#196980=CARTESIAN_POINT('Ctrl Pts',(-62.69431542765,-34.5868810019287,-213.257393287646));
#196981=CARTESIAN_POINT('Ctrl Pts',(-62.6950609186327,-34.5414369958665,
-213.267448588158));
#196982=CARTESIAN_POINT('Ctrl Pts',(-62.695805991523,-34.4959951029827,
-213.277359001672));
#196983=CARTESIAN_POINT('Ctrl Pts',(-62.6965506762908,-34.450555335486,
-213.28712284428));
#196984=CARTESIAN_POINT('Ctrl Pts',(-62.6973051981915,-34.4045153179852,
-213.297015665244));
#196985=CARTESIAN_POINT('Ctrl Pts',(-62.6980593192824,-34.3584776267204,
-213.306757986266));
#196986=CARTESIAN_POINT('Ctrl Pts',(-62.6988130699629,-34.3124423208934,
-213.316348049998));
#196987=CARTESIAN_POINT('Ctrl Pts',(-62.7009988974643,-34.1789429554945,
-213.34415860538));
#196988=CARTESIAN_POINT('Ctrl Pts',(-62.7031812969114,-34.0454633873908,
-213.370706259291));
#196989=CARTESIAN_POINT('Ctrl Pts',(-62.7053612372101,-33.9120052530651,
-213.395935334588));
#196990=CARTESIAN_POINT('Ctrl Pts',(-62.7241252898362,-32.7632511071928,
-213.61309710589));
#196991=CARTESIAN_POINT('Ctrl Pts',(-62.7427109555555,-31.6158500572718,
-213.732605675668));
#196992=CARTESIAN_POINT('Ctrl Pts',(-62.7617431230016,-30.4704148960704,
-213.718959479368));
#196993=CARTESIAN_POINT('Ctrl Pts',(-62.7647391297308,-30.2901027240271,
-213.716811321726));
#196994=CARTESIAN_POINT('Ctrl Pts',(-62.7677462013119,-30.1098392611621,
-213.711363635705));
#196995=CARTESIAN_POINT('Ctrl Pts',(-62.7707667754261,-29.929626890117,
-213.702478069896));
#196996=CARTESIAN_POINT('Ctrl Pts',(-62.7725414402335,-29.8237474974438,
-213.697257571958));
#196997=CARTESIAN_POINT('Ctrl Pts',(-62.7743209052534,-29.7178858577744,
-213.690842589644));
#196998=CARTESIAN_POINT('Ctrl Pts',(-62.7761057740119,-29.6120425444018,
-213.683199054813));
#196999=CARTESIAN_POINT('Ctrl Pts',(-62.7866097971823,-28.9891504629465,
-213.638216550309));
#197000=CARTESIAN_POINT('Ctrl Pts',(-62.7973012895261,-28.3668822616518,
-213.550676253008));
#197001=CARTESIAN_POINT('Ctrl Pts',(-62.8083033340944,-27.7453414694755,
-213.413639151456));
#197002=CARTESIAN_POINT('Ctrl Pts',(-62.8099338015368,-27.6532311331213,
-213.39333069596));
#197003=CARTESIAN_POINT('Ctrl Pts',(-62.811571077252,-27.5611367494673,
-213.371935988235));
#197004=CARTESIAN_POINT('Ctrl Pts',(-62.8132156027367,-27.4690586781088,
-213.349430181199));
#197005=CARTESIAN_POINT('Ctrl Pts',(-62.8148166574625,-27.3794145633366,
-213.327519284075));
#197006=CARTESIAN_POINT('Ctrl Pts',(-62.8164245864001,-27.2897858690337,
-213.304555131303));
#197007=CARTESIAN_POINT('Ctrl Pts',(-62.8180397952864,-27.2001730524582,
-213.280514793433));
#197008=CARTESIAN_POINT('Ctrl Pts',(-62.8188583605629,-27.1547585301661,
-213.268331486382));
#197009=CARTESIAN_POINT('Ctrl Pts',(-62.8196787972069,-27.1093480871546,
-213.25587168702));
#197010=CARTESIAN_POINT('Ctrl Pts',(-62.8205011614669,-27.063941785938,
-213.243132215583));
#197011=CARTESIAN_POINT('Ctrl Pts',(-62.820603956966,-27.0582660001277,
-213.241539782171));
#197012=CARTESIAN_POINT('Ctrl Pts',(-62.8207068130078,-27.0525903054942,
-213.23994121606));
#197013=CARTESIAN_POINT('Ctrl Pts',(-62.8208096296675,-27.0469146151422,
-213.238342307309));
#197014=CARTESIAN_POINT('Ctrl Pts',(-62.8209124463233,-27.0412389250094,
-213.23674339862));
#197015=CARTESIAN_POINT('Ctrl Pts',(-62.8210151618557,-27.0355631854498,
-213.23514772473));
#197016=CARTESIAN_POINT('Ctrl Pts',(-62.8211177763469,-27.0298873965555,
-213.233555280697));
#197017=CARTESIAN_POINT('Ctrl Pts',(-62.8213230053217,-27.0185358191958,
-213.23037039275));
#197018=CARTESIAN_POINT('Ctrl Pts',(-62.8215278301311,-27.007184044526,
-213.227198424317));
#197019=CARTESIAN_POINT('Ctrl Pts',(-62.821732251428,-26.9958320733605,
-213.224039336346));
#197020=CARTESIAN_POINT('Ctrl Pts',(-62.8221023145257,-26.9752816430542,
-213.218320451383));
#197021=CARTESIAN_POINT('Ctrl Pts',(-62.8224710552457,-26.9547305687705,
-213.212643777776));
#197022=CARTESIAN_POINT('Ctrl Pts',(-62.8228384774044,-26.9341788553176,
-213.207009087125));
#197023=CARTESIAN_POINT('Ctrl Pts',(-62.8228769801512,-26.9320252088911,
-213.206418619016));
#197024=CARTESIAN_POINT('Ctrl Pts',(-62.8229154684173,-26.9298715555,-213.205828611962));
#197025=CARTESIAN_POINT('Ctrl Pts',(-62.822953942207,-26.927717895148,-213.205239065704));
#197026=CARTESIAN_POINT('Ctrl Pts',(-62.8245764233091,-26.8368957212836,
-213.18037726579));
#197027=CARTESIAN_POINT('Ctrl Pts',(-62.8261731614531,-26.7460611681188,
-213.156334842912));
#197028=CARTESIAN_POINT('Ctrl Pts',(-62.8277444695765,-26.6552145055689,
-213.133093149386));
#197029=CARTESIAN_POINT('Ctrl Pts',(-62.8292202126583,-26.56989302612,-213.111264987285));
#197030=CARTESIAN_POINT('Ctrl Pts',(-62.8306735455578,-26.4845608838021,
-213.090141906315));
#197031=CARTESIAN_POINT('Ctrl Pts',(-62.8321046858337,-26.3992182785356,
-213.069710892685));
#197032=CARTESIAN_POINT('Ctrl Pts',(-62.8367688988908,-26.1210791607003,
-213.003124407662));
#197033=CARTESIAN_POINT('Ctrl Pts',(-62.8411971255009,-25.8428597458171,
-212.943883039818));
#197034=CARTESIAN_POINT('Ctrl Pts',(-62.8453976824702,-25.5644780440306,
-212.891551576526));
#197035=CARTESIAN_POINT('Ctrl Pts',(-62.8465846366303,-25.485815542499,
-212.876764240343));
#197036=CARTESIAN_POINT('Ctrl Pts',(-62.8477534065635,-25.4071494583571,
-212.862521456415));
#197037=CARTESIAN_POINT('Ctrl Pts',(-62.8489040944972,-25.3284786414784,
-212.848818315903));
#197038=CARTESIAN_POINT('Ctrl Pts',(-62.8589719385762,-24.6401551658149,
-212.728923878816));
#197039=CARTESIAN_POINT('Ctrl Pts',(-62.8676537352891,-23.9520875862977,
-212.65003766299));
#197040=CARTESIAN_POINT('Ctrl Pts',(-62.8750146865604,-23.2647003090938,
-212.608425061387));
#197041=CARTESIAN_POINT('Ctrl Pts',(-62.8823756378316,-22.5773130318898,
-212.566812459785));
#197042=CARTESIAN_POINT('Ctrl Pts',(-62.8884156923501,-21.8906064258753,
-212.562474309898));
#197043=CARTESIAN_POINT('Ctrl Pts',(-62.8931986251439,-21.205051121817,
-212.591707581156));
#197044=CARTESIAN_POINT('Ctrl Pts',(-62.8935577382081,-21.1535781288823,
-212.593902479154));
#197045=CARTESIAN_POINT('Ctrl Pts',(-62.8939097569274,-21.1021052395342,
-212.596289051621));
#197046=CARTESIAN_POINT('Ctrl Pts',(-62.8942546885952,-21.0506330432678,
-212.598866899387));
#197047=CARTESIAN_POINT('Ctrl Pts',(-62.8968212608728,-20.6676380203933,
-212.618048184355));
#197048=CARTESIAN_POINT('Ctrl Pts',(-62.898993894224,-20.2848774438099,
-212.64782882147));
#197049=CARTESIAN_POINT('Ctrl Pts',(-62.900778786722,-19.9023518511943,
-212.687972680865));
#197050=CARTESIAN_POINT('Ctrl Pts',(-62.9023087147126,-19.5744684565834,
-212.722382156061));
#197051=CARTESIAN_POINT('Ctrl Pts',(-62.9035537360166,-19.2467573919575,
-212.764406500889));
#197052=CARTESIAN_POINT('Ctrl Pts',(-62.9045166573415,-18.9192122497013,
-212.81392668013));
#197053=CARTESIAN_POINT('Ctrl Pts',(-62.9053466520591,-18.6368831218561,
-212.856610839387));
#197054=CARTESIAN_POINT('Ctrl Pts',(-62.9059670124065,-18.3545500700678,
-212.904900139621));
#197055=CARTESIAN_POINT('Ctrl Pts',(-62.9063776080623,-18.0726457860301,
-212.95869124202));
#197056=CARTESIAN_POINT('Ctrl Pts',(-62.9064830589281,-18.0002459678509,
-212.972506094273));
#197057=CARTESIAN_POINT('Ctrl Pts',(-62.9065746841136,-17.9278744301204,
-212.986683569855));
#197058=CARTESIAN_POINT('Ctrl Pts',(-62.9066525023395,-17.8555384962728,
-213.00122136616));
#197059=CARTESIAN_POINT('Ctrl Pts',(-62.9070069220114,-17.5260876814359,
-213.06743311714));
#197060=CARTESIAN_POINT('Ctrl Pts',(-62.9070749640207,-17.197340288906,
-213.141130341411));
#197061=CARTESIAN_POINT('Ctrl Pts',(-62.9068586171446,-16.8692921444043,
-213.222255473336));
#197062=CARTESIAN_POINT('Ctrl Pts',(-62.9068512161578,-16.8580699810933,
-213.225030674155));
#197063=CARTESIAN_POINT('Ctrl Pts',(-62.9068434310689,-16.8468489287218,
-213.227817504345));
#197064=CARTESIAN_POINT('Ctrl Pts',(-62.9068354227292,-16.8356281229708,
-213.230606932774));
#197065=CARTESIAN_POINT('Ctrl Pts',(-62.9068274143987,-16.824407330074,
-213.233396358007));
#197066=CARTESIAN_POINT('Ctrl Pts',(-62.9068194222443,-16.81318550769,-213.236174929377));
#197067=CARTESIAN_POINT('Ctrl Pts',(-62.9068114465212,-16.8019626469682,
-213.238942628495));
#197068=CARTESIAN_POINT('Ctrl Pts',(-62.9068100308831,-16.7999706633578,
-213.239433876798));
#197069=CARTESIAN_POINT('Ctrl Pts',(-62.9068086157626,-16.7979786470357,
-213.239924782582));
#197070=CARTESIAN_POINT('Ctrl Pts',(-62.9068072011611,-16.7959865979527,
-213.240415345746));
#197071=CARTESIAN_POINT('Ctrl Pts',(-62.9067926759976,-16.7755321875305,
-213.245452460734));
#197072=CARTESIAN_POINT('Ctrl Pts',(-62.9067782084953,-16.7550743640961,
-213.250453275771));
#197073=CARTESIAN_POINT('Ctrl Pts',(-62.9067638003454,-16.7346131155667,
-213.255417662646));
#197074=CARTESIAN_POINT('Ctrl Pts',(-62.9067321774736,-16.6897049597551,
-213.266313452264));
#197075=CARTESIAN_POINT('Ctrl Pts',(-62.9067008405294,-16.6447803048274,
-213.277033762557));
#197076=CARTESIAN_POINT('Ctrl Pts',(-62.9066698070808,-16.5998390244792,
-213.287577252305));
#197077=CARTESIAN_POINT('Ctrl Pts',(-62.9066077395427,-16.5099555355157,
-213.308664449577));
#197078=CARTESIAN_POINT('Ctrl Pts',(-62.9065468864317,-16.4200055414544,
-213.329044330242));
#197079=CARTESIAN_POINT('Ctrl Pts',(-62.9064873833149,-16.3299880540902,
-213.348706398678));
#197080=CARTESIAN_POINT('Ctrl Pts',(-62.9063683745862,-16.14994930492,-213.388031359981));
#197081=CARTESIAN_POINT('Ctrl Pts',(-62.9062547727652,-15.9696405404297,
-213.424484631685));
#197082=CARTESIAN_POINT('Ctrl Pts',(-62.9061475795573,-15.7890542301186,
-213.457986204279));
#197083=CARTESIAN_POINT('Ctrl Pts',(-62.9059331838863,-15.4278660176369,
-213.524992242));
#197084=CARTESIAN_POINT('Ctrl Pts',(-62.9057445834296,-15.0655667619647,
-213.58018242881));
#197085=CARTESIAN_POINT('Ctrl Pts',(-62.905589362047,-14.7020974635233,
-213.622929699832));
#197086=CARTESIAN_POINT('Ctrl Pts',(-62.9052798509934,-13.9773405794218,
-213.708167652755));
#197087=CARTESIAN_POINT('Ctrl Pts',(-62.9051047269463,-13.2479237446018,
-213.743849925036));
#197088=CARTESIAN_POINT('Ctrl Pts',(-62.9051090261727,-12.5134449350678,
-213.725695782834));
#197089=CARTESIAN_POINT('Ctrl Pts',(-62.9051090395082,-12.5111666950214,
-213.725639471484));
#197090=CARTESIAN_POINT('Ctrl Pts',(-62.9051090545696,-12.5088884062743,
-213.725582642177));
#197091=CARTESIAN_POINT('Ctrl Pts',(-62.9051090713583,-12.5066100688143,
-213.725525294786));
#197092=CARTESIAN_POINT('Ctrl Pts',(-62.9051117186635,-12.1473516978959,
-213.716482503419));
#197093=CARTESIAN_POINT('Ctrl Pts',(-62.9051569926989,-11.7868835043618,
-213.694572753784));
#197094=CARTESIAN_POINT('Ctrl Pts',(-62.9052478305722,-11.4251692471516,
-213.659411822611));
#197095=CARTESIAN_POINT('Ctrl Pts',(-62.9052501495695,-11.4159350548302,
-213.658514200263));
#197096=CARTESIAN_POINT('Ctrl Pts',(-62.905252498141,-11.4066999814362,
-213.657607942971));
#197097=CARTESIAN_POINT('Ctrl Pts',(-62.9052548763439,-11.3974640308012,
-213.656693043944));
#197098=CARTESIAN_POINT('Ctrl Pts',(-62.9053396597116,-11.0682006948933,
-213.624076725649));
#197099=CARTESIAN_POINT('Ctrl Pts',(-62.9054625664031,-10.7375855896767,
-213.580337710378));
#197100=CARTESIAN_POINT('Ctrl Pts',(-62.9056218033686,-10.4097786632115,
-213.526208718246));
#197101=CARTESIAN_POINT('Ctrl Pts',(-62.9056341733888,-10.3843136067641,
-213.522003810635));
#197102=CARTESIAN_POINT('Ctrl Pts',(-62.905646762572,-10.3588654933522,
-213.517736228732));
#197103=CARTESIAN_POINT('Ctrl Pts',(-62.9056595700396,-10.3334362698611,
-213.513406328741));
#197104=CARTESIAN_POINT('Ctrl Pts',(-62.9056676765601,-10.317340775653,
-213.510665707099));
#197105=CARTESIAN_POINT('Ctrl Pts',(-62.9056758700813,-10.3012520481916,
-213.507900031565));
#197106=CARTESIAN_POINT('Ctrl Pts',(-62.9056841503679,-10.2851705845394,
-213.505109387712));
#197107=CARTESIAN_POINT('Ctrl Pts',(-62.9058495001971,-9.96403831223826,
-213.449382756037));
#197108=CARTESIAN_POINT('Ctrl Pts',(-62.9060495440864,-9.64477667567909,
-213.383630454477));
#197109=CARTESIAN_POINT('Ctrl Pts',(-62.9062818494613,-9.32750692225147,
-213.308308849077));
#197110=CARTESIAN_POINT('Ctrl Pts',(-62.9062995203884,-9.30337295347418,
-213.302579310559));
#197111=CARTESIAN_POINT('Ctrl Pts',(-62.9063173779087,-9.27925050600288,
-213.296794425733));
#197112=CARTESIAN_POINT('Ctrl Pts',(-62.9063354209129,-9.25513963110861,
-213.290954407383));
#197113=CARTESIAN_POINT('Ctrl Pts',(-62.9063523663721,-9.23249540595939,
-213.28546963377));
#197114=CARTESIAN_POINT('Ctrl Pts',(-62.9063694755794,-9.20986097578642,
-213.279936139709));
#197115=CARTESIAN_POINT('Ctrl Pts',(-62.9063867476374,-9.18723633851541,
-213.274354087607));
#197116=CARTESIAN_POINT('Ctrl Pts',(-62.9064214242477,-9.14181351020547,
-213.263147163439));
#197117=CARTESIAN_POINT('Ctrl Pts',(-62.9064567545313,-9.09643013343645,
-213.251744618045));
#197118=CARTESIAN_POINT('Ctrl Pts',(-62.9064927284741,-9.05108616789961,
-213.240147881952));
#197119=CARTESIAN_POINT('Ctrl Pts',(-62.9065017219161,-9.03975023169194,
-213.23724871204));
#197120=CARTESIAN_POINT('Ctrl Pts',(-62.906510755583,-9.02841675862167,
-213.23433740548));
#197121=CARTESIAN_POINT('Ctrl Pts',(-62.9065198293118,-9.01708574800018,
-213.231413985003));
#197122=CARTESIAN_POINT('Ctrl Pts',(-62.9065289030347,-9.00575474453466,
-213.228490566373));
#197123=CARTESIAN_POINT('Ctrl Pts',(-62.9065377477119,-8.99442319446877,
-213.225569813864));
#197124=CARTESIAN_POINT('Ctrl Pts',(-62.9065461779452,-8.98308903056771,
-213.222661899751));
#197125=CARTESIAN_POINT('Ctrl Pts',(-62.9065630384181,-8.96042069442155,
-213.216846069384));
#197126=CARTESIAN_POINT('Ctrl Pts',(-62.9065784765558,-8.93774453557201,
-213.211068662567));
#197127=CARTESIAN_POINT('Ctrl Pts',(-62.9065924909309,-8.91506058486269,
-213.205329682185));
#197128=CARTESIAN_POINT('Ctrl Pts',(-62.906632507978,-8.85028818379569,
-213.188942433607));
#197129=CARTESIAN_POINT('Ctrl Pts',(-62.9066609166417,-8.7854522548987,
-213.172868479925));
#197130=CARTESIAN_POINT('Ctrl Pts',(-62.9066776826504,-8.72055350098855,
-213.157107960246));
#197131=CARTESIAN_POINT('Ctrl Pts',(-62.9066844034019,-8.69453846021989,
-213.1507902648));
#197132=CARTESIAN_POINT('Ctrl Pts',(-62.9066892533842,-8.66851311367876,
-213.144522883906));
#197133=CARTESIAN_POINT('Ctrl Pts',(-62.9066922303343,-8.64247748890024,
-213.13830582419));
#197134=CARTESIAN_POINT('Ctrl Pts',(-62.9067096741274,-8.48991865034706,
-213.101876223688));
#197135=CARTESIAN_POINT('Ctrl Pts',(-62.9066627545095,-8.33741593724109,
-213.067272060264));
#197136=CARTESIAN_POINT('Ctrl Pts',(-62.906552054195,-8.18500124845787,
-213.034473300197));
#197137=CARTESIAN_POINT('Ctrl Pts',(-62.9065307100423,-8.15561413774858,
-213.02814936383));
#197138=CARTESIAN_POINT('Ctrl Pts',(-62.906506993431,-8.12623007030402,
-213.021892565579));
#197139=CARTESIAN_POINT('Ctrl Pts',(-62.9064809085264,-8.09684923724608,
-213.015702751583));
#197140=CARTESIAN_POINT('Ctrl Pts',(-62.9056899601275,-7.20596145140544,
-212.828014755284));
#197141=CARTESIAN_POINT('Ctrl Pts',(-62.9027366747181,-6.31764267915001,
-212.700961335132));
#197142=CARTESIAN_POINT('Ctrl Pts',(-62.8976715771841,-5.43185195165884,
-212.632707606633));
#197143=CARTESIAN_POINT('Ctrl Pts',(-62.8947900085007,-4.92791953904604,
-212.593877592946));
#197144=CARTESIAN_POINT('Ctrl Pts',(-62.8912249487153,-4.42480439538553,
-212.574078170132));
#197145=CARTESIAN_POINT('Ctrl Pts',(-62.8869856905768,-3.92249156539548,
-212.572970530223));
#197146=CARTESIAN_POINT('Ctrl Pts',(-62.8865147226824,-3.8666862314995,
-212.572847475005));
#197147=CARTESIAN_POINT('Ctrl Pts',(-62.8860354164368,-3.81089071961118,
-212.572956060008));
#197148=CARTESIAN_POINT('Ctrl Pts',(-62.885547785291,-3.75510503118202,
-212.573295788909));
#197149=CARTESIAN_POINT('Ctrl Pts',(-62.8793243758262,-3.04313824163478,
-212.577631590838));
#197150=CARTESIAN_POINT('Ctrl Pts',(-62.8717459291031,-2.33277234486263,
-212.619539913621));
#197151=CARTESIAN_POINT('Ctrl Pts',(-62.862782948286,-1.62412895620602,
-212.701365863942));
#197152=CARTESIAN_POINT('Ctrl Pts',(-62.8546488502804,-0.981019828565347,
-212.775624675034));
#197153=CARTESIAN_POINT('Ctrl Pts',(-62.8453744839341,-0.339328956700993,
-212.882759122652));
#197154=CARTESIAN_POINT('Ctrl Pts',(-62.8349373318117,0.300889820690812,
-213.0245235881));
#197155=CARTESIAN_POINT('Ctrl Pts',(-62.833607314137,0.382473597532965,
-213.0425887885));
#197156=CARTESIAN_POINT('Ctrl Pts',(-62.8322582595392,0.46403334488501,
-213.0612252722));
#197157=CARTESIAN_POINT('Ctrl Pts',(-62.8308901810048,0.545568613619919,
-213.080433504715));
#197158=CARTESIAN_POINT('Ctrl Pts',(-62.8293216865052,0.639048349842208,
-213.102455637426));
#197159=CARTESIAN_POINT('Ctrl Pts',(-62.8277279878957,0.732495388151248,
-213.125241286058));
#197160=CARTESIAN_POINT('Ctrl Pts',(-62.8261090055383,0.82590908127445,
-213.148796974995));
#197161=CARTESIAN_POINT('Ctrl Pts',(-62.8246401331401,0.910661577071861,
-213.170168610789));
#197162=CARTESIAN_POINT('Ctrl Pts',(-62.8231504392872,0.995387120797636,
-213.192174253453));
#197163=CARTESIAN_POINT('Ctrl Pts',(-62.8216398034464,1.08008493804872,
-213.214822482476));
#197164=CARTESIAN_POINT('Ctrl Pts',(-62.8212428495944,1.10234121179649,
-213.220773818666));
#197165=CARTESIAN_POINT('Ctrl Pts',(-62.8208444494788,1.12459557042322,
-213.226769539358));
#197166=CARTESIAN_POINT('Ctrl Pts',(-62.8204446007164,1.14684799932478,
-213.232809812555));
#197167=CARTESIAN_POINT('Ctrl Pts',(-62.8202446762939,1.15797421607791,
-213.235829949778));
#197168=CARTESIAN_POINT('Ctrl Pts',(-62.8200446532189,1.16910062229217,
-213.238845621168));
#197169=CARTESIAN_POINT('Ctrl Pts',(-62.8198447802283,1.18022785110057,
-213.241842094701));
#197170=CARTESIAN_POINT('Ctrl Pts',(-62.8196449071673,1.19135508383139,
-213.24483856929));
#197171=CARTESIAN_POINT('Ctrl Pts',(-62.8194451061373,1.20248294022561,
-213.247820468072));
#197172=CARTESIAN_POINT('Ctrl Pts',(-62.8192453767934,1.21361141859872,
-213.250787808694));
#197173=CARTESIAN_POINT('Ctrl Pts',(-62.818446458071,1.25812540713443,-213.262657191196));
#197174=CARTESIAN_POINT('Ctrl Pts',(-62.8176486863071,1.30264934734857,
-213.274293643791));
#197175=CARTESIAN_POINT('Ctrl Pts',(-62.8168520397829,1.34718313255572,
-213.285698279351));
#197176=CARTESIAN_POINT('Ctrl Pts',(-62.8168331493294,1.3482391384167,-213.285968711382));
#197177=CARTESIAN_POINT('Ctrl Pts',(-62.8168142595085,1.3492951498132,-213.28623901307));
#197178=CARTESIAN_POINT('Ctrl Pts',(-62.8167953703201,1.35035116674384,
-213.28650918443));
#197179=CARTESIAN_POINT('Ctrl Pts',(-62.8152210633639,1.43836420130322,
-213.30902643819));
#197180=CARTESIAN_POINT('Ctrl Pts',(-62.8136511488777,1.52641572029817,
-213.330638365248));
#197181=CARTESIAN_POINT('Ctrl Pts',(-62.8120854563785,1.61450537353331,
-213.351353373466));
#197182=CARTESIAN_POINT('Ctrl Pts',(-62.8074297466586,1.87644688184623,
-213.412951078736));
#197183=CARTESIAN_POINT('Ctrl Pts',(-62.8028113125303,2.13872544174752,
-213.466621196678));
#197184=CARTESIAN_POINT('Ctrl Pts',(-62.7982260322374,2.40133274732117,
-213.512564584869));
#197185=CARTESIAN_POINT('Ctrl Pts',(-62.7965691479007,2.49622551363434,
-213.529166161088));
#197186=CARTESIAN_POINT('Ctrl Pts',(-62.7949165988104,2.59116092814595,
-213.544758707681));
#197187=CARTESIAN_POINT('Ctrl Pts',(-62.7932681861794,2.6861388388309,-213.559351754428));
#197188=CARTESIAN_POINT('Ctrl Pts',(-62.7870578081227,3.04396716487013,
-213.614330911704));
#197189=CARTESIAN_POINT('Ctrl Pts',(-62.7808961247399,3.40303459050701,
-213.655110348145));
#197190=CARTESIAN_POINT('Ctrl Pts',(-62.7748157638915,3.76060806585584,
-213.682219323134));
#197191=CARTESIAN_POINT('Ctrl Pts',(-62.7705733532615,4.01009548126256,
-213.701133891944));
#197192=CARTESIAN_POINT('Ctrl Pts',(-62.7663688307484,4.25893819616316,
-213.713443335564));
#197193=CARTESIAN_POINT('Ctrl Pts',(-62.7621968858993,4.50717455612263,
-213.719490676914));
#197194=CARTESIAN_POINT('Ctrl Pts',(-62.7603897273271,4.61470293486237,
-213.722110199739));
#197195=CARTESIAN_POINT('Ctrl Pts',(-62.7585886940891,4.72211697152003,
-213.723554528341));
#197196=CARTESIAN_POINT('Ctrl Pts',(-62.756793361705,4.82941936939531,-213.723851522444));
#197197=CARTESIAN_POINT('Ctrl Pts',(-62.7449145685473,5.53938427674049,
-213.72581658003));
#197198=CARTESIAN_POINT('Ctrl Pts',(-62.7332829196989,6.24447623947785,
-213.677701667467));
#197199=CARTESIAN_POINT('Ctrl Pts',(-62.7217741472389,6.94546014142215,
-213.58738262144));
#197200=CARTESIAN_POINT('Ctrl Pts',(-62.7160202469306,7.29592249555901,
-213.542226911863));
#197201=CARTESIAN_POINT('Ctrl Pts',(-62.7102974318188,7.64535562415708,
-213.486497387223));
#197202=CARTESIAN_POINT('Ctrl Pts',(-62.7045905440093,7.99385039894269,
-213.42112885562));
#197203=CARTESIAN_POINT('Ctrl Pts',(-62.7017372091525,8.16809112725469,
-213.388445838889));
#197204=CARTESIAN_POINT('Ctrl Pts',(-62.6988879008502,8.34209702777322,
-213.353350616143));
#197205=CARTESIAN_POINT('Ctrl Pts',(-62.6960409729441,8.51587804140929,
-213.31594549485));
#197206=CARTESIAN_POINT('Ctrl Pts',(-62.6953306860554,8.55923508435002,
-213.306613201199));
#197207=CARTESIAN_POINT('Ctrl Pts',(-62.6946205479401,8.60257812546093,
-213.297137089371));
#197208=CARTESIAN_POINT('Ctrl Pts',(-62.693910534767,8.64590730924635,-213.287518647044));
#197209=CARTESIAN_POINT('Ctrl Pts',(-62.6931976571302,8.68941129946275,
-213.277861400257));
#197210=CARTESIAN_POINT('Ctrl Pts',(-62.6924849069969,8.73290123523708,
-213.268060682277));
#197211=CARTESIAN_POINT('Ctrl Pts',(-62.6917722569378,8.77637732701844,
-213.258118114802));
#197212=CARTESIAN_POINT('Ctrl Pts',(-62.6914166494633,8.79807159758174,
-213.253156842064));
#197213=CARTESIAN_POINT('Ctrl Pts',(-62.6910610669502,8.8197624208846,-213.248160247015));
#197214=CARTESIAN_POINT('Ctrl Pts',(-62.6907055060663,8.84144982288414,
-213.243128526156));
#197215=CARTESIAN_POINT('Ctrl Pts',(-62.6903499459702,8.86313717683234,
-213.238096816445));
#197216=CARTESIAN_POINT('Ctrl Pts',(-62.6899947488889,8.88481939248657,
-213.233012444837));
#197217=CARTESIAN_POINT('Ctrl Pts',(-62.6896387405559,8.90650238461306,
-213.227935756798));
#197218=CARTESIAN_POINT('Ctrl Pts',(-62.6889267268058,8.94986819125594,
-213.217782422304));
#197219=CARTESIAN_POINT('Ctrl Pts',(-62.6882099166076,8.99324491620445,
-213.20773948302));
#197220=CARTESIAN_POINT('Ctrl Pts',(-62.6874882954834,9.03663265289044,
-213.197807426414));
#197221=CARTESIAN_POINT('Ctrl Pts',(-62.6868204901171,9.0767846972564,-213.1886160648));
#197222=CARTESIAN_POINT('Ctrl Pts',(-62.6861485996542,9.11694554599575,
-213.179518348821));
#197223=CARTESIAN_POINT('Ctrl Pts',(-62.6854726096978,9.15711522005327,
-213.170514913905));
#197224=CARTESIAN_POINT('Ctrl Pts',(-62.6826037415343,9.3275933432039,-213.132304778465));
#197225=CARTESIAN_POINT('Ctrl Pts',(-62.6796606062759,9.49823764842399,
-213.0958088569));
#197226=CARTESIAN_POINT('Ctrl Pts',(-62.6766425417446,9.66904980342632,
-213.061049681902));
#197227=CARTESIAN_POINT('Ctrl Pts',(-62.6706064126818,10.010674113431,-212.991531331906));
#197228=CARTESIAN_POINT('Ctrl Pts',(-62.664270812359,10.3529550669585,-212.928960848345));
#197229=CARTESIAN_POINT('Ctrl Pts',(-62.6576327768096,10.6957266313347,
-212.873621170708));
#197230=CARTESIAN_POINT('Ctrl Pts',(-62.6473143570134,11.2285440393067,
-212.787599030422));
#197231=CARTESIAN_POINT('Ctrl Pts',(-62.6362643202696,11.7626593744732,
-212.718966127623));
#197232=CARTESIAN_POINT('Ctrl Pts',(-62.6244492722702,12.2981837916612,
-212.669131165341));
#197233=CARTESIAN_POINT('Ctrl Pts',(-62.6210626304399,12.4516854441724,
-212.654846570993));
#197234=CARTESIAN_POINT('Ctrl Pts',(-62.6176131332117,12.6053025653781,
-212.642106558566));
#197235=CARTESIAN_POINT('Ctrl Pts',(-62.6140999935327,12.7590370278545,
-212.630944584506));
#197236=CARTESIAN_POINT('Ctrl Pts',(-62.6105014211192,12.9165100139118,
-212.619511172914));
#197237=CARTESIAN_POINT('Ctrl Pts',(-62.6068362958068,13.0740938080764,
-212.609737755954));
#197238=CARTESIAN_POINT('Ctrl Pts',(-62.6031038882691,13.2317919256033,
-212.60165208257));
#197239=CARTESIAN_POINT('Ctrl Pts',(-62.5920978382562,13.6968090361302,
-212.577809207764));
#197240=CARTESIAN_POINT('Ctrl Pts',(-62.5804979951207,14.1630944923736,
-212.568752968315));
#197241=CARTESIAN_POINT('Ctrl Pts',(-62.5682752556912,14.6305393235299,
-212.576049312116));
#197242=CARTESIAN_POINT('Ctrl Pts',(-62.5664789097222,14.69923854133,-212.577121637829));
#197243=CARTESIAN_POINT('Ctrl Pts',(-62.5646691057699,14.7679628409678,
-212.57854725337));
#197244=CARTESIAN_POINT('Ctrl Pts',(-62.5628457474452,14.8367119180636,
-212.580331218974));
#197245=CARTESIAN_POINT('Ctrl Pts',(-62.5582940634694,15.0083315434174,
-212.584784566154));
#197246=CARTESIAN_POINT('Ctrl Pts',(-62.5536582189233,15.1800866651594,
-212.591481763734));
#197247=CARTESIAN_POINT('Ctrl Pts',(-62.5489369347187,15.3519656949738,
-212.600500512768));
#197248=CARTESIAN_POINT('Ctrl Pts',(-62.5345339878628,15.8763070446555,
-212.628013485384));
#197249=CARTESIAN_POINT('Ctrl Pts',(-62.5194888785073,16.3962308632549,
-212.67684339347));
#197250=CARTESIAN_POINT('Ctrl Pts',(-62.5037997387389,16.9113773860642,
-212.748829194443));
#197251=CARTESIAN_POINT('Ctrl Pts',(-62.4982710429057,17.0929098649718,
-212.774196270251));
#197252=CARTESIAN_POINT('Ctrl Pts',(-62.4926620464246,17.2738497478374,
-212.802456316522));
#197253=CARTESIAN_POINT('Ctrl Pts',(-62.4869727360513,17.4541800510744,
-212.833687547544));
#197254=CARTESIAN_POINT('Ctrl Pts',(-62.471224815544,17.9533314585636,-212.920135097635));
#197255=CARTESIAN_POINT('Ctrl Pts',(-62.4548621630433,18.4478214139081,
-213.029285839066));
#197256=CARTESIAN_POINT('Ctrl Pts',(-62.4378715929549,18.937051788145,-213.164110067595));
#197257=CARTESIAN_POINT('Ctrl Pts',(-62.4313084944047,19.1260311539449,
-213.216189820905));
#197258=CARTESIAN_POINT('Ctrl Pts',(-62.4246524255105,19.3141920754881,
-213.272116519071));
#197259=CARTESIAN_POINT('Ctrl Pts',(-62.4179027766836,19.501499283875,-213.33205678481));
#197260=CARTESIAN_POINT('Ctrl Pts',(-62.4127593088451,19.6442339100696,
-213.377733358061));
#197261=CARTESIAN_POINT('Ctrl Pts',(-62.4075533326539,19.7866395914389,
-213.425870497305));
#197262=CARTESIAN_POINT('Ctrl Pts',(-62.4022963811676,19.9284129896732,
-213.476422874392));
#197263=CARTESIAN_POINT('Ctrl Pts',(-62.3923400029528,20.1969240416179,
-213.572166308062));
#197264=CARTESIAN_POINT('Ctrl Pts',(-62.3821761384096,20.4638252096883,
-213.676819486359));
#197265=CARTESIAN_POINT('Ctrl Pts',(-62.3718829556573,20.7269505848268,
-213.79019579402));
#197266=CARTESIAN_POINT('Ctrl Pts',(-62.3696094190237,20.7850691662223,
-213.815238115239));
#197267=CARTESIAN_POINT('Ctrl Pts',(-62.3673295817903,20.8430033470654,
-213.840705944902));
#197268=CARTESIAN_POINT('Ctrl Pts',(-62.3650443003751,20.9007294710183,
-213.866597158632));
#197269=CARTESIAN_POINT('Ctrl Pts',(-61.713103822739,20.0389506617614,-216.160137831685));
#197270=CARTESIAN_POINT('Ctrl Pts',(-61.7321110912357,20.3496658649069,
-216.247078381677));
#197271=CARTESIAN_POINT('Ctrl Pts',(-61.6907486315906,20.6657286340102,
-216.300532529068));
#197272=CARTESIAN_POINT('Ctrl Pts',(-61.9252463833055,20.1793980393595,
-215.812042320923));
#197273=CARTESIAN_POINT('Ctrl Pts',(-61.9373844794568,20.4413798330517,
-215.880084558757));
#197274=CARTESIAN_POINT('Ctrl Pts',(-61.9064790936528,20.7060595729952,
-215.92903923894));
#197275=CARTESIAN_POINT('Ctrl Pts',(-62.0850713031281,20.3222903717942,
-215.445236972404));
#197276=CARTESIAN_POINT('Ctrl Pts',(-62.0914940184093,20.5335632238432,
-215.496856996578));
#197277=CARTESIAN_POINT('Ctrl Pts',(-62.0699842872639,20.7460043187545,
-215.538658319552));
#197278=CARTESIAN_POINT('Ctrl Pts',(-62.3043696537349,20.611682425576,-214.675676922536));
#197279=CARTESIAN_POINT('Ctrl Pts',(-62.3035607512221,20.7183157084577,
-214.699282243487));
#197280=CARTESIAN_POINT('Ctrl Pts',(-62.2967890390184,20.824939865421,-214.721940813782));
#197281=CARTESIAN_POINT('Ctrl Pts',(-62.3625010497726,20.7591101230298,
-214.269920324208));
#197282=CARTESIAN_POINT('Ctrl Pts',(-62.36063660277,20.8116268449194,-214.281171503343));
#197283=CARTESIAN_POINT('Ctrl Pts',(-62.3587717320579,20.8641365401031,
-214.2924597236));
#197284=CARTESIAN_POINT('Ctrl Pts',(-62.3650472056256,20.9007985863674,
-213.86644416092));
#197285=CARTESIAN_POINT('Ctrl Pts',(-62.3650472056256,20.9007985863674,
-213.86644416092));
#197286=CARTESIAN_POINT('Ctrl Pts',(-62.3650472056256,20.9007985863674,
-213.86644416092));
#197287=CARTESIAN_POINT('',(-61.6907486315871,20.6657286340098,-216.300532529074));
#197288=CARTESIAN_POINT('Origin',(-59.1013738165116,20.5826972454933,-214.78783829177));
#197289=CARTESIAN_POINT('Ctrl Pts',(-61.6907486315871,20.66572863401,-216.300532529074));
#197290=CARTESIAN_POINT('Ctrl Pts',(-61.7776458854704,20.6819741262679,
-216.150893248708));
#197291=CARTESIAN_POINT('Ctrl Pts',(-61.8667307948559,20.7002117978156,
-215.979723760535));
#197292=CARTESIAN_POINT('Ctrl Pts',(-61.9936363408029,20.7302399848448,
-215.687912889814));
#197293=CARTESIAN_POINT('Ctrl Pts',(-62.034784576062,20.7406936090083,-215.584820111112));
#197294=CARTESIAN_POINT('Ctrl Pts',(-62.0932494709526,20.7569920861929,
-215.421377131638));
#197295=CARTESIAN_POINT('Ctrl Pts',(-62.121664872513,20.7652957504502,-215.337458316968));
#197296=CARTESIAN_POINT('Ctrl Pts',(-62.1530272418572,20.7752422475622,
-215.235736062925));
#197297=CARTESIAN_POINT('Ctrl Pts',(-62.166045121126,20.7795592499655,-215.191329117645));
#197298=CARTESIAN_POINT('Ctrl Pts',(-62.1746252349796,20.7824491595449,
-215.161544906292));
#197299=CARTESIAN_POINT('Ctrl Pts',(-62.179454484566,20.7841046857491,-215.144446131259));
#197300=CARTESIAN_POINT('Ctrl Pts',(-62.2982778852125,20.8254239556915,
-214.716977329717));
#197301=CARTESIAN_POINT('Ctrl Pts',(-62.3588454290314,20.8638984988155,
-214.288283562016));
#197302=CARTESIAN_POINT('Ctrl Pts',(-62.365046045184,20.9007916780701,-213.866523136266));
#197303=CARTESIAN_POINT('Ctrl Pts',(-61.6377935655245,19.9815886122025,
-216.280755810351));
#197304=CARTESIAN_POINT('Ctrl Pts',(-61.6055583132384,20.2909606839632,
-216.465410556112));
#197305=CARTESIAN_POINT('Ctrl Pts',(-61.499388181455,20.6071190721679,-216.605481304297));
#197306=CARTESIAN_POINT('Ctrl Pts',(-61.6652027952659,20.0090334790696,
-216.239468240032));
#197307=CARTESIAN_POINT('Ctrl Pts',(-61.6507949119044,20.3194192931518,
-216.390568004079));
#197308=CARTESIAN_POINT('Ctrl Pts',(-61.5691908701262,20.6359350302665,
-216.502281627839));
#197309=CARTESIAN_POINT('Ctrl Pts',(-61.6926044944854,20.0301302514809,
-216.195652941672));
#197310=CARTESIAN_POINT('Ctrl Pts',(-61.6967727624885,20.3410293418827,
-216.311297779654));
#197311=CARTESIAN_POINT('Ctrl Pts',(-61.6387815649118,20.6575029215266,
-216.391600777262));
#197312=CARTESIAN_POINT('Ctrl Pts',(-61.7199387591116,20.0421410735216,
-216.14839440092));
#197313=CARTESIAN_POINT('Ctrl Pts',(-61.7438559996858,20.35282222204,-216.225852774313));
#197314=CARTESIAN_POINT('Ctrl Pts',(-61.7080768938385,20.6687713493049,
-216.270467388274));
#197315=CARTESIAN_POINT('',(-61.516838435879,20.6141575017552,-216.579518431174));
#197316=CARTESIAN_POINT('',(-61.6446456814072,19.9883159925442,-216.270380726959));
#197317=CARTESIAN_POINT('Origin',(-59.0326817073425,20.5344053061246,-214.899457439615));
#197318=CARTESIAN_POINT('Ctrl Pts',(-61.6446456814073,19.9883159925441,
-216.270380726959));
#197319=CARTESIAN_POINT('Ctrl Pts',(-61.6589899513843,20.0021161049564,
-216.24854827085));
#197320=CARTESIAN_POINT('Ctrl Pts',(-61.6733754040443,20.0141614250312,
-216.225936040046));
#197321=CARTESIAN_POINT('Ctrl Pts',(-61.6878163893671,20.0240270532932,
-216.202356326574));
#197322=CARTESIAN_POINT('Ctrl Pts',(-61.6962257996766,20.0297720986736,
-216.18862516619));
#197323=CARTESIAN_POINT('Ctrl Pts',(-61.7046540329176,20.034777214409,-216.174565637937));
#197324=CARTESIAN_POINT('Ctrl Pts',(-61.7131038227345,20.0389506617863,
-216.160137831703));
#197325=CARTESIAN_POINT('Ctrl Pts',(-61.516838435851,20.614157501844,-216.579518431211));
#197326=CARTESIAN_POINT('Ctrl Pts',(-61.5771479675576,20.6380049970577,
-216.489212055522));
#197327=CARTESIAN_POINT('Ctrl Pts',(-61.6351552038294,20.6553354111624,
-216.396265812028));
#197328=CARTESIAN_POINT('Ctrl Pts',(-61.6907486315871,20.66572863401,-216.300532529074));
#197329=CARTESIAN_POINT('Ctrl Pts',(-61.235107328202,28.3894013135675,-216.583947161644));
#197330=CARTESIAN_POINT('Ctrl Pts',(-62.0737483304577,28.4205138141115,
-215.350417820742));
#197331=CARTESIAN_POINT('Ctrl Pts',(-62.0998335778874,28.4197995297673,
-213.858707258037));
#197332=CARTESIAN_POINT('Ctrl Pts',(-61.3394317178759,25.782537982878,-216.582300349965));
#197333=CARTESIAN_POINT('Ctrl Pts',(-62.1750190192476,25.8120069501401,
-215.350359724707));
#197334=CARTESIAN_POINT('Ctrl Pts',(-62.2010617731482,25.8108994796242,
-213.861712475948));
#197335=CARTESIAN_POINT('Ctrl Pts',(-61.4338508567495,23.1751069333097,
-216.580828347939));
#197336=CARTESIAN_POINT('Ctrl Pts',(-62.2667395005803,23.2024779691083,
-215.350312870121));
#197337=CARTESIAN_POINT('Ctrl Pts',(-62.2927210668524,23.2015642400677,
-213.864398964149));
#197338=CARTESIAN_POINT('Ctrl Pts',(-61.5183514407949,20.5675003107738,
-216.579494546858));
#197339=CARTESIAN_POINT('Ctrl Pts',(-62.3488810204336,20.5925259779214,
-215.350234406272));
#197340=CARTESIAN_POINT('Ctrl Pts',(-62.3748047396227,20.5920154834281,
-213.866720382044));
#197341=CARTESIAN_POINT('',(-62.099833577893,28.4197995297552,-213.858707258032));
#197342=CARTESIAN_POINT('Origin',(1003.25098428815,-12.9621320438613,-174.780968069139));
#197343=CARTESIAN_POINT('',(-61.2351073280272,28.3894013125172,-216.583947161963));
#197344=CARTESIAN_POINT('Origin',(-57.1043579940171,28.2258690560256,-213.771445225846));
#197345=CARTESIAN_POINT('Origin',(967.060476622167,-12.7722155952905,-232.807288933329));
#197346=CARTESIAN_POINT('Ctrl Pts',(-61.0271214515746,29.6036708476845,
-216.705447812142));
#197347=CARTESIAN_POINT('Ctrl Pts',(-62.0328771597131,29.432010466984,-215.416461273176));
#197348=CARTESIAN_POINT('Ctrl Pts',(-62.0715435503805,29.1708764678268,
-213.793867031503));
#197349=CARTESIAN_POINT('Ctrl Pts',(-61.0627413621019,29.4095488042208,
-216.699316444474));
#197350=CARTESIAN_POINT('Ctrl Pts',(-62.0394002938428,29.2676078599798,
-215.416801443606));
#197351=CARTESIAN_POINT('Ctrl Pts',(-62.0761251487726,29.0460828494865,
-213.81396536355));
#197352=CARTESIAN_POINT('Ctrl Pts',(-61.0959751735216,29.2176086084485,
-216.688979075795));
#197353=CARTESIAN_POINT('Ctrl Pts',(-62.045900321156,29.1044853538962,-215.413559895334));
#197354=CARTESIAN_POINT('Ctrl Pts',(-62.0807624949799,28.9211132693028,
-213.830014605952));
#197355=CARTESIAN_POINT('Ctrl Pts',(-61.1660917025604,28.812533486502,-216.649425062049));
#197356=CARTESIAN_POINT('Ctrl Pts',(-62.059522361877,28.7670896367546,-215.392285581265));
#197357=CARTESIAN_POINT('Ctrl Pts',(-62.0901763780839,28.6707891288636,
-213.852481398947));
#197358=CARTESIAN_POINT('Ctrl Pts',(-61.2033761954606,28.5977249793428,
-216.618438059186));
#197359=CARTESIAN_POINT('Ctrl Pts',(-62.0666989989455,28.5919001092215,
-215.373070477725));
#197360=CARTESIAN_POINT('Ctrl Pts',(-62.094959380688,28.5454196012504,-213.858562559592));
#197361=CARTESIAN_POINT('Ctrl Pts',(-61.2351073279008,28.3894013132804,
-216.583947162106));
#197362=CARTESIAN_POINT('Ctrl Pts',(-62.0737483304886,28.4205138133222,
-215.350417821044));
#197363=CARTESIAN_POINT('Ctrl Pts',(-62.0998335779475,28.4197995283645,
-213.858707258032));
#197364=CARTESIAN_POINT('',(-61.0271214515743,29.6036708476852,-216.705447812142));
#197365=CARTESIAN_POINT('',(-62.0715435503803,29.170876467827,-213.793867031503));
#197366=CARTESIAN_POINT('Origin',(-57.0762058255522,28.9734268472959,-213.706604999317));
#197367=CARTESIAN_POINT('Ctrl Pts',(-61.0271214515743,29.6036708476852,
-216.705447812142));
#197368=CARTESIAN_POINT('Ctrl Pts',(-61.0627413621019,29.4095488042208,
-216.699316444474));
#197369=CARTESIAN_POINT('Ctrl Pts',(-61.0959751735216,29.2176086084485,
-216.688979075795));
#197370=CARTESIAN_POINT('Ctrl Pts',(-61.1660917025604,28.812533486502,-216.649425062049));
#197371=CARTESIAN_POINT('Ctrl Pts',(-61.2033761954606,28.5977249793428,
-216.618438059186));
#197372=CARTESIAN_POINT('Ctrl Pts',(-61.2351073279234,28.3894013132814,
-216.583947162069));
#197373=CARTESIAN_POINT('Ctrl Pts',(-62.0998335778935,28.4197995297553,
-213.858707258032));
#197374=CARTESIAN_POINT('Ctrl Pts',(-62.094949600635,28.5456716573278,-213.858562269211));
#197375=CARTESIAN_POINT('Ctrl Pts',(-62.0901675429821,28.6710240626564,
-213.85246031345));
#197376=CARTESIAN_POINT('Ctrl Pts',(-62.0854694365319,28.7959511990832,
-213.841248002449));
#197377=CARTESIAN_POINT('Ctrl Pts',(-62.0807548271223,28.9213171649583,
-213.829996306153));
#197378=CARTESIAN_POINT('Ctrl Pts',(-62.0761182844883,29.0462698189252,
-213.813935251642));
#197379=CARTESIAN_POINT('Ctrl Pts',(-62.0715435503805,29.1708764678268,
-213.793867031503));
#197380=CARTESIAN_POINT('Ctrl Pts',(-62.0722753176769,29.1511380815083,
-213.795657702395));
#197381=CARTESIAN_POINT('Ctrl Pts',(-62.0340745338293,29.4127097517032,
-215.416670061812));
#197382=CARTESIAN_POINT('Ctrl Pts',(-61.030221352118,29.5865570284964,-216.704939048052));
#197383=CARTESIAN_POINT('Ctrl Pts',(-62.0620320829829,29.4340729912048,
-213.769970033114));
#197384=CARTESIAN_POINT('Ctrl Pts',(-62.0171383824692,29.6895867289819,
-215.413872853516));
#197385=CARTESIAN_POINT('Ctrl Pts',(-60.9858182348534,29.8316477735471,
-216.712544680079));
#197386=CARTESIAN_POINT('Ctrl Pts',(-62.0412495434026,29.7158438578209,
-213.745237314573));
#197387=CARTESIAN_POINT('Ctrl Pts',(-61.9892647258148,29.9729902357752,
-215.414291487854));
#197388=CARTESIAN_POINT('Ctrl Pts',(-60.9270407929623,30.0877775086874,
-216.723516257042));
#197389=CARTESIAN_POINT('Ctrl Pts',(-61.9794688757743,30.2707145068829,
-213.698186104697));
#197390=CARTESIAN_POINT('Ctrl Pts',(-61.9159025865061,30.5129372076058,
-215.407258353661));
#197391=CARTESIAN_POINT('Ctrl Pts',(-60.8096093037007,30.5582220616567,
-216.733419187575));
#197392=CARTESIAN_POINT('Ctrl Pts',(-61.938926317498,30.5439708220038,-213.676343773128));
#197393=CARTESIAN_POINT('Ctrl Pts',(-61.8707327962001,30.775264549444,-215.402898488695));
#197394=CARTESIAN_POINT('Ctrl Pts',(-60.747409441142,30.7826838238242,-216.736387709467));
#197395=CARTESIAN_POINT('Ctrl Pts',(-61.837636032495,31.0884065478961,-213.634598566576));
#197396=CARTESIAN_POINT('Ctrl Pts',(-61.7592484376381,31.3083441263931,
-215.399426388486));
#197397=CARTESIAN_POINT('Ctrl Pts',(-60.5980527039995,31.2446203390114,
-216.747650397627));
#197398=CARTESIAN_POINT('Ctrl Pts',(-61.7769096374044,31.3595164244479,
-213.614424841566));
#197399=CARTESIAN_POINT('Ctrl Pts',(-61.6932454520362,31.5755832712924,
-215.398384202842));
#197400=CARTESIAN_POINT('Ctrl Pts',(-60.5138367274016,31.4762486370728,
-216.753526488075));
#197401=CARTESIAN_POINT('Ctrl Pts',(-61.6347983988434,31.899450706002,-213.575433990368));
#197402=CARTESIAN_POINT('Ctrl Pts',(-61.5426774850893,32.1020267212171,
-215.393731279353));
#197403=CARTESIAN_POINT('Ctrl Pts',(-60.3359793889894,31.9259601738048,
-216.76111570899));
#197404=CARTESIAN_POINT('Ctrl Pts',(-61.5531858863137,32.1688271147634,
-213.556786982595));
#197405=CARTESIAN_POINT('Ctrl Pts',(-61.458472596998,32.3604331023391,-215.389897348667));
#197406=CARTESIAN_POINT('Ctrl Pts',(-60.2437451595173,32.1426522013982,
-216.762577010636));
#197407=CARTESIAN_POINT('Ctrl Pts',(-61.4159587545849,32.5674954665022,
-213.530743809019));
#197408=CARTESIAN_POINT('Ctrl Pts',(-61.3177400835575,32.7449412296482,
-215.385939876134));
#197409=CARTESIAN_POINT('Ctrl Pts',(-60.0928857706128,32.4655283166213,
-216.766110440268));
#197410=CARTESIAN_POINT('Ctrl Pts',(-61.3676767622843,32.6997212687758,
-213.522342385503));
#197411=CARTESIAN_POINT('Ctrl Pts',(-61.2682838922593,32.872909821302,-215.384883950169));
#197412=CARTESIAN_POINT('Ctrl Pts',(-60.0403931405282,32.572987171916,-216.767475838973));
#197413=CARTESIAN_POINT('Ctrl Pts',(-61.2664764445886,32.9616854374991,
-213.505934868461));
#197414=CARTESIAN_POINT('Ctrl Pts',(-61.16400924397,33.1287467154492,-215.383607108532));
#197415=CARTESIAN_POINT('Ctrl Pts',(-59.9294247387107,32.7889935283979,
-216.770953998618));
#197416=CARTESIAN_POINT('Ctrl Pts',(-61.2135447672718,33.091483145622,-213.497857516746));
#197417=CARTESIAN_POINT('Ctrl Pts',(-61.108560223271,33.2579834247729,-215.383794009871));
#197418=CARTESIAN_POINT('Ctrl Pts',(-59.8692253143189,32.8995596733306,
-216.773542513475));
#197419=CARTESIAN_POINT('Ctrl Pts',(-61.0478125873863,33.4773667643361,
-213.47408238772));
#197420=CARTESIAN_POINT('Ctrl Pts',(-60.939655477163,33.6324724880252,-215.380343496444));
#197421=CARTESIAN_POINT('Ctrl Pts',(-59.6963317184513,33.2127149517822,
-216.776352933466));
#197422=CARTESIAN_POINT('Ctrl Pts',(-60.9280440899178,33.7300206143803,
-213.459385328777));
#197423=CARTESIAN_POINT('Ctrl Pts',(-60.8222945421723,33.8691785847138,
-215.375378456549));
#197424=CARTESIAN_POINT('Ctrl Pts',(-59.5857444814115,33.4045989682938,
-216.77471811873));
#197425=CARTESIAN_POINT('Ctrl Pts',(-60.7344672841107,34.1022007074626,
-213.439632708162));
#197426=CARTESIAN_POINT('Ctrl Pts',(-60.6302881857557,34.2248170372617,
-215.371749277836));
#197427=CARTESIAN_POINT('Ctrl Pts',(-59.4018730546303,33.6971462711828,
-216.77599109459));
#197428=CARTESIAN_POINT('Ctrl Pts',(-60.6676250274419,34.2251152634526,
-213.433348725261));
#197429=CARTESIAN_POINT('Ctrl Pts',(-60.5629875662736,34.3444216969835,
-215.371371877201));
#197430=CARTESIAN_POINT('Ctrl Pts',(-59.3362053418023,33.7967893027105,
-216.777264657507));
#197431=CARTESIAN_POINT('Ctrl Pts',(-60.5293279502117,34.4685916588927,
-213.420959244589));
#197432=CARTESIAN_POINT('Ctrl Pts',(-60.4230895229254,34.5826588364461,
-215.370625427342));
#197433=CARTESIAN_POINT('Ctrl Pts',(-59.1998648193908,33.9959954562112,
-216.779653928204));
#197434=CARTESIAN_POINT('Ctrl Pts',(-60.4578772193282,34.5891494281844,
-213.414818675441));
#197435=CARTESIAN_POINT('Ctrl Pts',(-60.3505501995765,34.7010803776926,
-215.370127825967));
#197436=CARTESIAN_POINT('Ctrl Pts',(-59.1294078669496,34.095271216951,-216.780624801763));
#197437=CARTESIAN_POINT('Ctrl Pts',(-60.3471832550081,34.768251943839,-213.406087731132));
#197438=CARTESIAN_POINT('Ctrl Pts',(-60.2427301457655,34.8702456283936,
-215.36729429493));
#197439=CARTESIAN_POINT('Ctrl Pts',(-59.0316233263315,34.2327858157498,
-216.779602213422));
#197440=CARTESIAN_POINT('Ctrl Pts',(-60.3096963328013,34.8276667088433,
-213.403282057557));
#197441=CARTESIAN_POINT('Ctrl Pts',(-60.2073956626117,34.9245822814321,
-215.365838464165));
#197442=CARTESIAN_POINT('Ctrl Pts',(-59.0013384113356,34.2757719021763,
-216.778662998653));
#197443=CARTESIAN_POINT('Ctrl Pts',(-60.2335269589641,34.945932810334,-213.397980978197));
#197444=CARTESIAN_POINT('Ctrl Pts',(-60.1350035456452,35.0338818623324,
-215.363515549055));
#197445=CARTESIAN_POINT('Ctrl Pts',(-58.9384240938482,34.3630029801402,
-216.777376929373));
#197446=CARTESIAN_POINT('Ctrl Pts',(-60.1948462340149,35.0047819102021,
-213.395467604637));
#197447=CARTESIAN_POINT('Ctrl Pts',(-60.098003280493,35.0887243625003,-215.362587120194));
#197448=CARTESIAN_POINT('Ctrl Pts',(-58.9059517617724,34.4070761172112,
-216.776964413499));
#197449=CARTESIAN_POINT('Ctrl Pts',(-60.0732701737662,35.1860378427238,
-213.388026309707));
#197450=CARTESIAN_POINT('Ctrl Pts',(-59.9811145129592,35.2587196749933,
-215.360184867158));
#197451=CARTESIAN_POINT('Ctrl Pts',(-58.80275485317,34.5444172631871,-216.776133900962));
#197452=CARTESIAN_POINT('Ctrl Pts',(-59.9883366029424,35.3074524979782,
-213.38343869169));
#197453=CARTESIAN_POINT('Ctrl Pts',(-59.8985377265825,35.374186215073,-215.359237777425));
#197454=CARTESIAN_POINT('Ctrl Pts',(-58.7288550087989,34.6388163213973,
-216.776220299507));
#197455=CARTESIAN_POINT('Ctrl Pts',(-59.9016315893045,35.4263976750195,
-213.37931837001));
#197456=CARTESIAN_POINT('Ctrl Pts',(-59.8155211638331,35.4858202289832,
-215.357783188893));
#197457=CARTESIAN_POINT('Ctrl Pts',(-58.6567202300399,34.7293397325179,
-216.775594469212));
#197458=CARTESIAN_POINT('',(-58.6665914736623,34.7169872964315,-216.775646223556));
#197459=CARTESIAN_POINT('',(-59.9134443065973,35.4101621769153,-213.379883144535));
#197460=CARTESIAN_POINT('Origin',(-55.8698139418538,32.470529749032,-213.292621112349));
#197461=CARTESIAN_POINT('Ctrl Pts',(-58.6665914736623,34.7169872964315,
-216.775646223557));
#197462=CARTESIAN_POINT('Ctrl Pts',(-58.68891411473,34.6889262212036,-216.775820369084));
#197463=CARTESIAN_POINT('Ctrl Pts',(-58.7113614970553,34.6605567043895,
-216.775932488694));
#197464=CARTESIAN_POINT('Ctrl Pts',(-58.7337888387604,34.6319802064989,
-216.776022661718));
#197465=CARTESIAN_POINT('Ctrl Pts',(-58.7552226821379,34.6046696055318,
-216.776108840209));
#197466=CARTESIAN_POINT('Ctrl Pts',(-58.7766384767105,34.5771695739528,
-216.77617497345));
#197467=CARTESIAN_POINT('Ctrl Pts',(-58.7978896199004,34.5496113066691,
-216.776256046869));
#197468=CARTESIAN_POINT('Ctrl Pts',(-58.818445685349,34.5229544091615,-216.776334468557));
#197469=CARTESIAN_POINT('Ctrl Pts',(-58.8388478025107,34.4962428910996,
-216.776426869088));
#197470=CARTESIAN_POINT('Ctrl Pts',(-58.8589413273301,34.4696399854441,
-216.77656491206));
#197471=CARTESIAN_POINT('Ctrl Pts',(-58.8635229652065,34.4635741069449,
-216.776596388017));
#197472=CARTESIAN_POINT('Ctrl Pts',(-58.8680884632319,34.4575140665269,
-216.776630236976));
#197473=CARTESIAN_POINT('Ctrl Pts',(-58.8726358156898,34.4514621421053,
-216.776666834302));
#197474=CARTESIAN_POINT('Ctrl Pts',(-58.8993737676191,34.4158774660199,
-216.776882022713));
#197475=CARTESIAN_POINT('Ctrl Pts',(-58.9255521608924,34.3804868678643,
-216.777189950846));
#197476=CARTESIAN_POINT('Ctrl Pts',(-58.951098376918,34.3453668781434,-216.77763514187));
#197477=CARTESIAN_POINT('Ctrl Pts',(-58.9574067387464,34.3366943764177,
-216.77774507698));
#197478=CARTESIAN_POINT('Ctrl Pts',(-58.9636764242332,34.328038594042,-216.777863382238));
#197479=CARTESIAN_POINT('Ctrl Pts',(-58.9699061024711,34.3194010903381,
-216.777990728079));
#197480=CARTESIAN_POINT('Ctrl Pts',(-58.982028851275,34.3025927924298,-216.778238538894));
#197481=CARTESIAN_POINT('Ctrl Pts',(-58.9939827439098,34.2858621186605,
-216.778530335959));
#197482=CARTESIAN_POINT('Ctrl Pts',(-59.005958458314,34.2690364739751,-216.778814923197));
#197483=CARTESIAN_POINT('Ctrl Pts',(-59.0196242261173,34.2498363372941,
-216.77913967235));
#197484=CARTESIAN_POINT('Ctrl Pts',(-59.033317885381,34.2305136307765,-216.779455033138));
#197485=CARTESIAN_POINT('Ctrl Pts',(-59.047339665745,34.2107575527891,-216.779684931869));
#197486=CARTESIAN_POINT('Ctrl Pts',(-59.0529154730659,34.2029014830594,
-216.779776351859));
#197487=CARTESIAN_POINT('Ctrl Pts',(-59.0585434000204,34.1949763905612,
-216.779854257892));
#197488=CARTESIAN_POINT('Ctrl Pts',(-59.0642433014168,34.1869605874501,
-216.77991386644));
#197489=CARTESIAN_POINT('Ctrl Pts',(-59.0832958083669,34.1601669407071,
-216.780113114147));
#197490=CARTESIAN_POINT('Ctrl Pts',(-59.102779151996,34.1327728264599,-216.78017120186));
#197491=CARTESIAN_POINT('Ctrl Pts',(-59.1225303078593,34.1048954334528,
-216.780123799295));
#197492=CARTESIAN_POINT('Ctrl Pts',(-59.1415464599063,34.0780554475924,
-216.780078160731));
#197493=CARTESIAN_POINT('Ctrl Pts',(-59.1608108973337,34.0507670685685,
-216.779934737065));
#197494=CARTESIAN_POINT('Ctrl Pts',(-59.1801602203819,34.0231784383873,
-216.779725362211));
#197495=CARTESIAN_POINT('Ctrl Pts',(-59.1988920056233,33.9964703052722,
-216.7795226696));
#197496=CARTESIAN_POINT('Ctrl Pts',(-59.2177033230583,33.9694806014766,
-216.779258168316));
#197497=CARTESIAN_POINT('Ctrl Pts',(-59.2364287245647,33.9423895910669,
-216.778960740555));
#197498=CARTESIAN_POINT('Ctrl Pts',(-59.2470111671479,33.9270794220388,
-216.778792652719));
#197499=CARTESIAN_POINT('Ctrl Pts',(-59.2575658550351,33.9117377574434,
-216.77861404878));
#197500=CARTESIAN_POINT('Ctrl Pts',(-59.2680604524456,33.8964041258495,
-216.77843014182));
#197501=CARTESIAN_POINT('Ctrl Pts',(-59.2998335102196,33.8499805858637,
-216.777873351861));
#197502=CARTESIAN_POINT('Ctrl Pts',(-59.3310391548654,33.8035995166105,
-216.777299416541));
#197503=CARTESIAN_POINT('Ctrl Pts',(-59.3615252914712,33.7573947953899,
-216.776802311717));
#197504=CARTESIAN_POINT('Ctrl Pts',(-59.3795446970365,33.7300846241643,
-216.776508488542));
#197505=CARTESIAN_POINT('Ctrl Pts',(-59.3973125982864,33.7028372954064,
-216.776241507053));
#197506=CARTESIAN_POINT('Ctrl Pts',(-59.4147969421915,33.675688640263,-216.776020773));
#197507=CARTESIAN_POINT('Ctrl Pts',(-59.4311986392249,33.6502210551514,
-216.775813707006));
#197508=CARTESIAN_POINT('Ctrl Pts',(-59.4473498031528,33.6248420237438,
-216.775647338403));
#197509=CARTESIAN_POINT('Ctrl Pts',(-59.4631890571003,33.5996410081924,
-216.775537686686));
#197510=CARTESIAN_POINT('Ctrl Pts',(-59.4834075864701,33.5674723546204,
-216.775397718195));
#197511=CARTESIAN_POINT('Ctrl Pts',(-59.5033327223937,33.5352944108817,
-216.775325313048));
#197512=CARTESIAN_POINT('Ctrl Pts',(-59.5230054610261,33.5031054017674,
-216.775293584259));
#197513=CARTESIAN_POINT('Ctrl Pts',(-59.5438616272312,33.4689800399348,
-216.775259946801));
#197514=CARTESIAN_POINT('Ctrl Pts',(-59.5644345215814,33.4348418935606,
-216.775272026729));
#197515=CARTESIAN_POINT('Ctrl Pts',(-59.5847982540677,33.4006346487011,
-216.775297787095));
#197516=CARTESIAN_POINT('Ctrl Pts',(-59.607298462236,33.3628385260738,-216.77532625013));
#197517=CARTESIAN_POINT('Ctrl Pts',(-59.6295437657375,33.3249579524366,
-216.775371414775));
#197518=CARTESIAN_POINT('Ctrl Pts',(-59.6516573645725,33.2868558376646,
-216.77539006563));
#197519=CARTESIAN_POINT('Ctrl Pts',(-59.6753100926277,33.2461017765208,
-216.775410014604));
#197520=CARTESIAN_POINT('Ctrl Pts',(-59.6988130119915,33.2050936700177,
-216.775399630573));
#197521=CARTESIAN_POINT('Ctrl Pts',(-59.72233137803,33.1636031936252,-216.775306032011));
#197522=CARTESIAN_POINT('Ctrl Pts',(-59.7482947804579,33.1177992490086,
-216.775202702675));
#197523=CARTESIAN_POINT('Ctrl Pts',(-59.7742785554707,33.0714067381163,
-216.774997956963));
#197524=CARTESIAN_POINT('Ctrl Pts',(-59.8005028618899,33.0240569092213,
-216.77462064611));
#197525=CARTESIAN_POINT('Ctrl Pts',(-59.8042035822122,33.0173749985065,
-216.774567400777));
#197526=CARTESIAN_POINT('Ctrl Pts',(-59.807909064699,33.0106739440499,-216.774510718933));
#197527=CARTESIAN_POINT('Ctrl Pts',(-59.811619893991,33.003952637821,-216.774450400634));
#197528=CARTESIAN_POINT('Ctrl Pts',(-59.833977195716,32.9634575733704,-216.774086990108));
#197529=CARTESIAN_POINT('Ctrl Pts',(-59.8567504991726,32.9220364044774,
-216.773475005287));
#197530=CARTESIAN_POINT('Ctrl Pts',(-59.8794666670023,32.8801912149089,
-216.772760470042));
#197531=CARTESIAN_POINT('Ctrl Pts',(-59.8830729275937,32.8735481640557,
-216.772647035403));
#197532=CARTESIAN_POINT('Ctrl Pts',(-59.8866777641604,32.8668945322141,
-216.772531016234));
#197533=CARTESIAN_POINT('Ctrl Pts',(-59.8902793094997,32.8602324399893,
-216.772412996774));
#197534=CARTESIAN_POINT('Ctrl Pts',(-59.9147369266354,32.8149910545269,
-216.771611542259));
#197535=CARTESIAN_POINT('Ctrl Pts',(-59.9390402310768,32.7693558218133,
-216.770717842538));
#197536=CARTESIAN_POINT('Ctrl Pts',(-59.9626984288671,32.723963924159,-216.769914861649));
#197537=CARTESIAN_POINT('Ctrl Pts',(-59.9701796860638,32.7096099795344,
-216.769660940931));
#197538=CARTESIAN_POINT('Ctrl Pts',(-59.9775966733613,32.695280690391,-216.769416091802));
#197539=CARTESIAN_POINT('Ctrl Pts',(-59.9849345594905,32.6809970052011,
-216.769186099808));
#197540=CARTESIAN_POINT('Ctrl Pts',(-60.019976886076,32.6127847772576,-216.768087765163));
#197541=CARTESIAN_POINT('Ctrl Pts',(-60.0538230741447,32.5447837722497,
-216.767138487128));
#197542=CARTESIAN_POINT('Ctrl Pts',(-60.0866775699529,32.4768286872757,
-216.76629138433));
#197543=CARTESIAN_POINT('Ctrl Pts',(-60.1058431236745,32.4371873292306,
-216.765797229914));
#197544=CARTESIAN_POINT('Ctrl Pts',(-60.124670852594,32.3975605116188,-216.765337845025));
#197545=CARTESIAN_POINT('Ctrl Pts',(-60.143197685769,32.3579083385831,-216.7649039233));
#197546=CARTESIAN_POINT('Ctrl Pts',(-60.1789309577007,32.2814299750988,
-216.764067005147));
#197547=CARTESIAN_POINT('Ctrl Pts',(-60.2136112483601,32.2046803722813,
-216.76334298333));
#197548=CARTESIAN_POINT('Ctrl Pts',(-60.2474734670841,32.1274737896909,
-216.762587094311));
#197549=CARTESIAN_POINT('Ctrl Pts',(-60.2748213223657,32.0651200950118,
-216.761976622101));
#197550=CARTESIAN_POINT('Ctrl Pts',(-60.3016350479361,32.0024671247304,
-216.761345364431));
#197551=CARTESIAN_POINT('Ctrl Pts',(-60.3280143860689,31.9394105099008,
-216.760617063764));
#197552=CARTESIAN_POINT('Ctrl Pts',(-60.3609034404128,31.8607932064096,
-216.759709037941));
#197553=CARTESIAN_POINT('Ctrl Pts',(-60.3931182697554,31.7815511857832,
-216.758650164247));
#197554=CARTESIAN_POINT('Ctrl Pts',(-60.424932988713,31.7011072820459,-216.757292652615));
#197555=CARTESIAN_POINT('Ctrl Pts',(-60.455870616552,31.6228811138668,-216.755972565842));
#197556=CARTESIAN_POINT('Ctrl Pts',(-60.4862672508109,31.5438480239397,
-216.754400559193));
#197557=CARTESIAN_POINT('Ctrl Pts',(-60.5158738472255,31.4643026910919,
-216.752674579628));
#197558=CARTESIAN_POINT('Ctrl Pts',(-60.5449572973019,31.3861629183096,
-216.750979097992));
#197559=CARTESIAN_POINT('Ctrl Pts',(-60.5732787670902,31.3075277945667,
-216.749135036746));
#197560=CARTESIAN_POINT('Ctrl Pts',(-60.6006489223964,31.2286922513233,
-216.747235241906));
#197561=CARTESIAN_POINT('Ctrl Pts',(-60.6255053702117,31.1570970577745,
-216.745509926476));
#197562=CARTESIAN_POINT('Ctrl Pts',(-60.6495779600038,31.0853362075051,
-216.743738644629));
#197563=CARTESIAN_POINT('Ctrl Pts',(-60.6727550228659,31.0136526708201,
-216.741990938608));
#197564=CARTESIAN_POINT('Ctrl Pts',(-60.6750801349789,31.0064614119259,
-216.741815609557));
#197565=CARTESIAN_POINT('Ctrl Pts',(-60.6773925737596,30.9992764828879,
-216.741642861846));
#197566=CARTESIAN_POINT('Ctrl Pts',(-60.6796927546667,30.9920971874804,
-216.741472557014));
#197567=CARTESIAN_POINT('Ctrl Pts',(-60.7005717089029,30.926930060931,-216.739926684351));
#197568=CARTESIAN_POINT('Ctrl Pts',(-60.7204435599204,30.8622313445984,
-216.738582089287));
#197569=CARTESIAN_POINT('Ctrl Pts',(-60.739541788745,30.7977002662527,-216.73733521714));
#197570=CARTESIAN_POINT('Ctrl Pts',(-60.7595264935239,30.7301738709184,
-216.736030469355));
#197571=CARTESIAN_POINT('Ctrl Pts',(-60.7786648263104,30.6628289056779,
-216.734832726975));
#197572=CARTESIAN_POINT('Ctrl Pts',(-60.7971797973658,30.595283631511,-216.733623335648));
#197573=CARTESIAN_POINT('Ctrl Pts',(-60.8147795981204,30.5310770300697,
-216.73247372292));
#197574=CARTESIAN_POINT('Ctrl Pts',(-60.8318162353816,30.4666873557856,
-216.731313584368));
#197575=CARTESIAN_POINT('Ctrl Pts',(-60.8484370244407,30.4017854464693,
-216.730041005063));
#197576=CARTESIAN_POINT('Ctrl Pts',(-60.8549049587336,30.3765290471826,
-216.729545784331));
#197577=CARTESIAN_POINT('Ctrl Pts',(-60.8613094191775,30.3511952223564,
-216.729033536068));
#197578=CARTESIAN_POINT('Ctrl Pts',(-60.8676570670374,30.325765519308,-216.728498254352));
#197579=CARTESIAN_POINT('Ctrl Pts',(-60.8843043256454,30.2590739112798,
-216.727094431495));
#197580=CARTESIAN_POINT('Ctrl Pts',(-60.9009917813059,30.1909296264927,
-216.725222439664));
#197581=CARTESIAN_POINT('Ctrl Pts',(-60.9173043394106,30.1220021183896,
-216.723087543031));
#197582=CARTESIAN_POINT('Ctrl Pts',(-60.9255062185316,30.0873456846193,
-216.722014126832));
#197583=CARTESIAN_POINT('Ctrl Pts',(-60.9336138051568,30.0524920317603,
-216.720874247456));
#197584=CARTESIAN_POINT('Ctrl Pts',(-60.9415777804195,30.0175296824247,
-216.71969399568));
#197585=CARTESIAN_POINT('Ctrl Pts',(-60.9572804382746,29.9485940326622,
-216.717366880237));
#197586=CARTESIAN_POINT('Ctrl Pts',(-60.9724208023033,29.8792370463633,
-216.714882811262));
#197587=CARTESIAN_POINT('Ctrl Pts',(-60.9867512024517,29.8100625396009,
-216.712441782693));
#197588=CARTESIAN_POINT('Ctrl Pts',(-61.0003153409054,29.7445868670811,
-216.71013127851));
#197589=CARTESIAN_POINT('Ctrl Pts',(-61.0131545031479,29.6792758917845,
-216.707859334961));
#197590=CARTESIAN_POINT('Ctrl Pts',(-61.0251046935149,29.614621768833,-216.705795549183));
#197591=CARTESIAN_POINT('Ctrl Pts',(-61.0257797804844,29.6109693453498,
-216.705678962347));
#197592=CARTESIAN_POINT('Ctrl Pts',(-61.0264520416984,29.6073190097918,
-216.705563039808));
#197593=CARTESIAN_POINT('Ctrl Pts',(-61.0271214515743,29.6036708476852,
-216.705447812142));
#197594=CARTESIAN_POINT('Ctrl Pts',(-62.0715435503803,29.170876467827,-213.793867031503));
#197595=CARTESIAN_POINT('Ctrl Pts',(-62.0610597588881,29.4471784510282,
-213.768820140639));
#197596=CARTESIAN_POINT('Ctrl Pts',(-62.0405226885833,29.7223719582909,
-213.744683753079));
#197597=CARTESIAN_POINT('Ctrl Pts',(-61.9794688757743,30.2707145068829,
-213.698186104697));
#197598=CARTESIAN_POINT('Ctrl Pts',(-61.938926317498,30.5439708220038,-213.676343773128));
#197599=CARTESIAN_POINT('Ctrl Pts',(-61.837636032495,31.0884065478961,-213.634598566576));
#197600=CARTESIAN_POINT('Ctrl Pts',(-61.7769096374044,31.3595164244479,
-213.614424841566));
#197601=CARTESIAN_POINT('Ctrl Pts',(-61.6347983988434,31.899450706002,-213.575433990368));
#197602=CARTESIAN_POINT('Ctrl Pts',(-61.5531858863137,32.1688271147634,
-213.556786982595));
#197603=CARTESIAN_POINT('Ctrl Pts',(-61.4159587545849,32.5674954665022,
-213.530743809019));
#197604=CARTESIAN_POINT('Ctrl Pts',(-61.3676767622843,32.6997212687758,
-213.522342385503));
#197605=CARTESIAN_POINT('Ctrl Pts',(-61.2664764445886,32.9616854374991,
-213.505934868461));
#197606=CARTESIAN_POINT('Ctrl Pts',(-61.2135447672718,33.091483145622,-213.497857516746));
#197607=CARTESIAN_POINT('Ctrl Pts',(-61.0478125873863,33.4773667643361,
-213.47408238772));
#197608=CARTESIAN_POINT('Ctrl Pts',(-60.9280440899178,33.7300206143803,
-213.459385328777));
#197609=CARTESIAN_POINT('Ctrl Pts',(-60.7344672841107,34.1022007074626,
-213.439632708162));
#197610=CARTESIAN_POINT('Ctrl Pts',(-60.6676250274419,34.2251152634526,
-213.433348725261));
#197611=CARTESIAN_POINT('Ctrl Pts',(-60.5293279502117,34.4685916588927,
-213.420959244589));
#197612=CARTESIAN_POINT('Ctrl Pts',(-60.4578772193282,34.5891494281844,
-213.414818675441));
#197613=CARTESIAN_POINT('Ctrl Pts',(-60.3471832550081,34.768251943839,-213.406087731132));
#197614=CARTESIAN_POINT('Ctrl Pts',(-60.3096963328013,34.8276667088433,
-213.403282057557));
#197615=CARTESIAN_POINT('Ctrl Pts',(-60.2335269589641,34.945932810334,-213.397980978197));
#197616=CARTESIAN_POINT('Ctrl Pts',(-60.1948462340149,35.0047819102021,
-213.395467604637));
#197617=CARTESIAN_POINT('Ctrl Pts',(-60.0770110939153,35.180460560743,-213.388255279868));
#197618=CARTESIAN_POINT('Ctrl Pts',(-59.9960526307283,35.2964118099283,
-213.383856689781));
#197619=CARTESIAN_POINT('Ctrl Pts',(-59.9134443065973,35.4101621769153,
-213.379883144535));
#197620=CARTESIAN_POINT('Ctrl Pts',(-58.4265182736836,35.031835198701,-216.764384131257));
#197621=CARTESIAN_POINT('Ctrl Pts',(-59.4820528027665,35.9125166648153,
-215.346308247144));
#197622=CARTESIAN_POINT('Ctrl Pts',(-59.4999643211654,35.9450057402374,
-213.371639708519));
#197623=CARTESIAN_POINT('Ctrl Pts',(-58.5101635386642,34.9284713760212,
-216.764533686556));
#197624=CARTESIAN_POINT('Ctrl Pts',(-59.6013542567605,35.7669646494546,
-215.346152352703));
#197625=CARTESIAN_POINT('Ctrl Pts',(-59.6440986517759,35.7696968033849,
-213.370755972398));
#197626=CARTESIAN_POINT('Ctrl Pts',(-58.5901397589755,34.8235003567058,
-216.768336879113));
#197627=CARTESIAN_POINT('Ctrl Pts',(-59.716223702441,35.6196247157672,-215.350089533733));
#197628=CARTESIAN_POINT('Ctrl Pts',(-59.7818407313686,35.591378236295,-213.37355288053));
#197629=CARTESIAN_POINT('Ctrl Pts',(-58.6665914736623,34.7169872964315,
-216.775646223556));
#197630=CARTESIAN_POINT('Ctrl Pts',(-59.8268417476682,35.4705704696998,
-215.357954892849));
#197631=CARTESIAN_POINT('Ctrl Pts',(-59.9134443065992,35.4101621769128,
-213.379883144535));
#197632=CARTESIAN_POINT('',(-58.4265182736835,35.0318351987012,-216.764384131257));
#197633=CARTESIAN_POINT('',(-59.4999643211654,35.9450057402376,-213.371639708519));
#197634=CARTESIAN_POINT('Origin',(-55.6381166865346,32.7703375395218,-213.284377676332));
#197635=CARTESIAN_POINT('Origin',(-55.6093041639685,32.7570348834843,-220.18888881533));
#197636=CARTESIAN_POINT('Origin',(-52.7506200812507,30.3721960348575,-218.064222059651));
#197637=CARTESIAN_POINT('Ctrl Pts',(-59.4999643211654,35.9450057402375,
-213.371639708519));
#197638=CARTESIAN_POINT('Ctrl Pts',(-59.4820528027664,35.9125166648155,
-215.346308247144));
#197639=CARTESIAN_POINT('Ctrl Pts',(-58.4265182736835,35.0318351987011,
-216.764384131257));
#197640=CARTESIAN_POINT('Ctrl Pts',(-58.5926451028781,37.0484655333583,
-213.380920503251));
#197641=CARTESIAN_POINT('Ctrl Pts',(-58.5785030823812,37.0120312878948,
-215.346864153085));
#197642=CARTESIAN_POINT('Ctrl Pts',(-57.5486529224783,36.1166487545866,
-216.762814542594));
#197643=CARTESIAN_POINT('Ctrl Pts',(-57.6483853099767,38.133634981491,-213.391180664217));
#197644=CARTESIAN_POINT('Ctrl Pts',(-57.6304520414564,38.1023651317606,
-215.347861259614));
#197645=CARTESIAN_POINT('Ctrl Pts',(-56.6223825642859,37.199049975754,-216.761500614303));
#197646=CARTESIAN_POINT('Ctrl Pts',(-56.6821911570462,39.1835711849512,
-213.399142265953));
#197647=CARTESIAN_POINT('Ctrl Pts',(-56.6650296771565,39.1519706625635,
-215.348455523392));
#197648=CARTESIAN_POINT('Ctrl Pts',(-55.6813080372832,38.2352492592492,
-216.760202274403));
#197649=CARTESIAN_POINT('Origin',(-55.9261752750931,34.4804203345293,-216.774342624392));
#197650=CARTESIAN_POINT('Ctrl Pts',(-59.4999643211654,35.9450057402376,
-213.371639708519));
#197651=CARTESIAN_POINT('Ctrl Pts',(-58.5980606988345,37.0418792159154,
-213.380865108156));
#197652=CARTESIAN_POINT('Ctrl Pts',(-57.6596561667371,38.1206800373646,
-213.391058217659));
#197653=CARTESIAN_POINT('Ctrl Pts',(-56.6994898617306,39.1647669078403,
-213.398999669105));
#197654=CARTESIAN_POINT('Ctrl Pts',(-32.8165183688975,-74.6541274212728,
-216.51122887497));
#197655=CARTESIAN_POINT('Ctrl Pts',(-33.0091444114044,-74.6582518783947,
-216.541274916939));
#197656=CARTESIAN_POINT('Ctrl Pts',(-33.2026950400511,-74.6410958794286,
-216.55765515809));
#197657=CARTESIAN_POINT('Ctrl Pts',(-32.9887489376153,-75.1686242635311,
-215.738182558023));
#197658=CARTESIAN_POINT('Ctrl Pts',(-33.1223658470707,-75.1686649637887,
-215.755874084856));
#197659=CARTESIAN_POINT('Ctrl Pts',(-33.2561102111421,-75.1596478279591,
-215.769886156826));
#197660=CARTESIAN_POINT('Ctrl Pts',(-33.1761299750104,-75.4501086463177,
-214.823392642664));
#197661=CARTESIAN_POINT('Ctrl Pts',(-33.2421742173859,-75.4479136121607,
-214.830806918362));
#197662=CARTESIAN_POINT('Ctrl Pts',(-33.3081522704534,-75.4457107575812,
-214.838787544289));
#197663=CARTESIAN_POINT('Ctrl Pts',(-33.3513928282978,-75.4608560063641,
-213.894101968638));
#197664=CARTESIAN_POINT('Ctrl Pts',(-33.3513928282978,-75.4608560063641,
-213.894101968638));
#197665=CARTESIAN_POINT('Ctrl Pts',(-33.3513928282978,-75.4608560063641,
-213.894101968638));
#197666=CARTESIAN_POINT('',(-32.8638506286442,-74.7886412857388,-216.296958652099));
#197667=CARTESIAN_POINT('',(-33.2148661077876,-74.7769245833719,-216.339144130374));
#197668=CARTESIAN_POINT('Origin',(-33.132841491033,-72.1913959359691,-214.819830610287));
#197669=CARTESIAN_POINT('',(-33.3513928264996,-75.4608559488301,-213.894101967632));
#197670=CARTESIAN_POINT('Ctrl Pts',(-32.8638506286442,-74.7886412857387,
-216.296958652099));
#197671=CARTESIAN_POINT('Ctrl Pts',(-32.8933260548794,-74.8682190505126,
-216.162404628958));
#197672=CARTESIAN_POINT('Ctrl Pts',(-32.9231745954811,-74.9411675841871,
-216.02417466485));
#197673=CARTESIAN_POINT('Ctrl Pts',(-32.9532524920876,-75.0072119742557,
-215.88285862242));
#197674=CARTESIAN_POINT('Ctrl Pts',(-32.986261903726,-75.0796933211633,
-215.727769339525));
#197675=CARTESIAN_POINT('Ctrl Pts',(-33.0195475005087,-75.1438591184812,
-215.568962618225));
#197676=CARTESIAN_POINT('Ctrl Pts',(-33.0529294896422,-75.199412086906,
-215.407221678871));
#197677=CARTESIAN_POINT('Ctrl Pts',(-33.0852131460734,-75.2531372540669,
-215.250802332615));
#197678=CARTESIAN_POINT('Ctrl Pts',(-33.1175871783702,-75.2988078108743,
-215.091637931136));
#197679=CARTESIAN_POINT('Ctrl Pts',(-33.1498964378058,-75.3362055632975,
-214.930449437084));
#197680=CARTESIAN_POINT('Ctrl Pts',(-33.1812470981023,-75.372493743607,
-214.774043322893));
#197681=CARTESIAN_POINT('Ctrl Pts',(-33.2125369672066,-75.4009928593788,
-214.615730725899));
#197682=CARTESIAN_POINT('Ctrl Pts',(-33.2436284013859,-75.4215458554388,
-214.456193093629));
#197683=CARTESIAN_POINT('Ctrl Pts',(-33.2728936047542,-75.4408916214159,
-214.306026291212));
#197684=CARTESIAN_POINT('Ctrl Pts',(-33.3019831259178,-75.4531972400418,
-214.154773836299));
#197685=CARTESIAN_POINT('Ctrl Pts',(-33.3307835805188,-75.4583694968115,
-214.003031469667));
#197686=CARTESIAN_POINT('Ctrl Pts',(-33.3376703705436,-75.4596062913975,
-213.96674670155));
#197687=CARTESIAN_POINT('Ctrl Pts',(-33.3445406344615,-75.4604353932884,
-213.930434060699));
#197688=CARTESIAN_POINT('Ctrl Pts',(-33.3513928247577,-75.4608558931301,
-213.894101966659));
#197689=CARTESIAN_POINT('Ctrl Pts',(-33.214866107757,-74.7769245823989,
-216.339144129802));
#197690=CARTESIAN_POINT('Ctrl Pts',(-33.2161008212724,-74.7878219958422,
-216.320532532356));
#197691=CARTESIAN_POINT('Ctrl Pts',(-33.2175661619688,-74.8004930397082,
-216.298622713186));
#197692=CARTESIAN_POINT('Ctrl Pts',(-33.2192576796893,-74.8147968984671,
-216.273316347388));
#197693=CARTESIAN_POINT('Ctrl Pts',(-33.2209398407141,-74.8290216348776,
-216.248149964733));
#197694=CARTESIAN_POINT('Ctrl Pts',(-33.2228456900929,-74.8448613909909,
-216.219624134786));
#197695=CARTESIAN_POINT('Ctrl Pts',(-33.2249693770086,-74.8621308073514,
-216.187621059665));
#197696=CARTESIAN_POINT('Ctrl Pts',(-33.2270703464035,-74.8792154891719,
-216.155960328097));
#197697=CARTESIAN_POINT('Ctrl Pts',(-33.2293845234151,-74.8976995978964,
-216.120895865541));
#197698=CARTESIAN_POINT('Ctrl Pts',(-33.2319047062494,-74.9173546654421,
-216.082299276337));
#197699=CARTESIAN_POINT('Ctrl Pts',(-33.2322639276174,-74.9201562559283,
-216.07679780264));
#197700=CARTESIAN_POINT('Ctrl Pts',(-33.2326273317533,-74.922981551917,
-216.071224549988));
#197701=CARTESIAN_POINT('Ctrl Pts',(-33.232994895118,-74.9258298060492,
-216.065579132006));
#197702=CARTESIAN_POINT('Ctrl Pts',(-33.235521708764,-74.9454101236201,
-216.02676971692));
#197703=CARTESIAN_POINT('Ctrl Pts',(-33.2382452115044,-74.9660795535131,
-215.984549980128));
#197704=CARTESIAN_POINT('Ctrl Pts',(-33.2411568577201,-74.9875665385017,
-215.938792794573));
#197705=CARTESIAN_POINT('Ctrl Pts',(-33.2440204091037,-75.0086985995535,
-215.893791430295));
#197706=CARTESIAN_POINT('Ctrl Pts',(-33.2470659410344,-75.0306214817497,
-215.845367893565));
#197707=CARTESIAN_POINT('Ctrl Pts',(-33.2502837771814,-75.0530272134654,
-215.793405196313));
#197708=CARTESIAN_POINT('Ctrl Pts',(-33.2534413473024,-75.0750133139911,
-215.742415695061));
#197709=CARTESIAN_POINT('Ctrl Pts',(-33.2567648260833,-75.097464297192,
-215.688017709565));
#197710=CARTESIAN_POINT('Ctrl Pts',(-33.2602435735815,-75.1200409653675,
-215.630113880679));
#197711=CARTESIAN_POINT('Ctrl Pts',(-33.2636148807263,-75.1419203580994,
-215.573998398844));
#197712=CARTESIAN_POINT('Ctrl Pts',(-33.2671320060908,-75.1639175549083,
-215.514589701032));
#197713=CARTESIAN_POINT('Ctrl Pts',(-33.2707839210029,-75.1856803680515,
-215.45182058607));
#197714=CARTESIAN_POINT('Ctrl Pts',(-33.2743682890001,-75.2070406496675,
-215.390212467508));
#197715=CARTESIAN_POINT('Ctrl Pts',(-33.2780824983859,-75.2281748902149,
-215.325366493977));
#197716=CARTESIAN_POINT('Ctrl Pts',(-33.2819149163973,-75.2487109574915,
-215.257248779496));
#197717=CARTESIAN_POINT('Ctrl Pts',(-33.2856358268015,-75.2686495096442,
-215.191113010441));
#197718=CARTESIAN_POINT('Ctrl Pts',(-33.2894681543121,-75.288023788226,
-215.121892651973));
#197719=CARTESIAN_POINT('Ctrl Pts',(-33.2934002616768,-75.3064608341125,
-215.049592577771));
#197720=CARTESIAN_POINT('Ctrl Pts',(-33.2968272599527,-75.3225295012684,
-214.986579997834));
#197721=CARTESIAN_POINT('Ctrl Pts',(-33.3003300294583,-75.3378856082417,
-214.921228394508));
#197722=CARTESIAN_POINT('Ctrl Pts',(-33.3039003488338,-75.3522651902505,
-214.853568530225));
#197723=CARTESIAN_POINT('Ctrl Pts',(-33.3078221575319,-75.3680604073912,
-214.779247715656));
#197724=CARTESIAN_POINT('Ctrl Pts',(-33.3118254668097,-75.3826772453835,
-214.702140725086));
#197725=CARTESIAN_POINT('Ctrl Pts',(-33.3158988721731,-75.3957488225826,
-214.622330942384));
#197726=CARTESIAN_POINT('Ctrl Pts',(-33.3199055351263,-75.4086062230697,
-214.543828836376));
#197727=CARTESIAN_POINT('Ctrl Pts',(-33.3239799985301,-75.4199680325328,
-214.462711510984));
#197728=CARTESIAN_POINT('Ctrl Pts',(-33.3281111209217,-75.4294750184256,
-214.379106717126));
#197729=CARTESIAN_POINT('Ctrl Pts',(-33.3321439448228,-75.4387557891946,
-214.297491267632));
#197730=CARTESIAN_POINT('Ctrl Pts',(-33.3362307450562,-75.4462683685185,
-214.213505231994));
#197731=CARTESIAN_POINT('Ctrl Pts',(-33.3403611424482,-75.4516772452927,
-214.127316474386));
#197732=CARTESIAN_POINT('Ctrl Pts',(-33.3440067390281,-75.4564512611557,
-214.051244026592));
#197733=CARTESIAN_POINT('Ctrl Pts',(-33.3476862895492,-75.4595861164654,
-213.973456225545));
#197734=CARTESIAN_POINT('Ctrl Pts',(-33.3513928282415,-75.4608560045305,
-213.894101968605));
#197735=CARTESIAN_POINT('Ctrl Pts',(-32.8237598256931,-74.7342241033955,
-216.385388039321));
#197736=CARTESIAN_POINT('Ctrl Pts',(-32.9990492150883,-74.6974990623407,
-216.482388336084));
#197737=CARTESIAN_POINT('Ctrl Pts',(-33.1752262860966,-74.6372704537069,
-216.564961398279));
#197738=CARTESIAN_POINT('Ctrl Pts',(-32.8430811295134,-74.7517232841371,
-216.358132577358));
#197739=CARTESIAN_POINT('Ctrl Pts',(-33.0186275335316,-74.7272821064456,
-216.433478854629));
#197740=CARTESIAN_POINT('Ctrl Pts',(-33.1949631872871,-74.6820694401031,
-216.496303691409));
#197741=CARTESIAN_POINT('Ctrl Pts',(-32.8576392293324,-74.7701076430446,
-216.328432913936));
#197742=CARTESIAN_POINT('Ctrl Pts',(-33.0332084422395,-74.759074042344,
-216.380020841617));
#197743=CARTESIAN_POINT('Ctrl Pts',(-33.2094670740838,-74.7292736488408,
-216.42052674827));
#197744=CARTESIAN_POINT('Ctrl Pts',(-32.8638454862961,-74.788639230448,
-216.296979356596));
#197745=CARTESIAN_POINT('Ctrl Pts',(-33.0390297214682,-74.7918205915911,
-216.32328753345));
#197746=CARTESIAN_POINT('Ctrl Pts',(-33.2148661078031,-74.7769245838569,
-216.339144130663));
#197747=CARTESIAN_POINT('',(-33.1752262860962,-74.6372704537073,-216.564961398278));
#197748=CARTESIAN_POINT('',(-32.8237598256931,-74.7342241033955,-216.385388039321));
#197749=CARTESIAN_POINT('Origin',(-33.095784450501,-72.1361943004091,-214.910178309726));
#197750=CARTESIAN_POINT('Origin',(-31.6882418561644,-74.6383695538455,-216.347659410123));
#197751=CARTESIAN_POINT('Origin',(-32.1378318913552,-74.4550490310553,-216.331724211812));
#197752=CARTESIAN_POINT('Ctrl Pts',(-40.9214983009346,-74.359273050182,
-216.569709261874));
#197753=CARTESIAN_POINT('Ctrl Pts',(-40.9511754288283,-75.1706180168058,
-215.350418326104));
#197754=CARTESIAN_POINT('Ctrl Pts',(-40.9503927122519,-75.1962323486437,
-213.885776709122));
#197755=CARTESIAN_POINT('Ctrl Pts',(-38.3243446255231,-74.4622360878715,
-216.567950323542));
#197756=CARTESIAN_POINT('Ctrl Pts',(-38.3524464104668,-75.2704427049198,
-215.350356210397));
#197757=CARTESIAN_POINT('Ctrl Pts',(-38.3512480421798,-75.2960131238996,
-213.888896037155));
#197758=CARTESIAN_POINT('Ctrl Pts',(-35.7265937516252,-74.5554064320832,
-216.566381833796));
#197759=CARTESIAN_POINT('Ctrl Pts',(-35.7526446696953,-75.3607900950907,
-215.350336416776));
#197760=CARTESIAN_POINT('Ctrl Pts',(-35.75158731892,-75.3862982053642,-213.891764704332));
#197761=CARTESIAN_POINT('Ctrl Pts',(-33.1287433582892,-74.6387629869627,
-216.564935505388));
#197762=CARTESIAN_POINT('Ctrl Pts',(-33.152500416473,-75.4416278685767,
-215.350281850593));
#197763=CARTESIAN_POINT('Ctrl Pts',(-33.1518661790636,-75.4670741746134,
-213.89429696046));
#197764=CARTESIAN_POINT('',(-40.9503927122327,-75.1962323486441,-213.885776709122));
#197765=CARTESIAN_POINT('Origin',(0.00137741249504053,990.512728685443,
-181.064224899351));
#197766=CARTESIAN_POINT('',(-40.9214982998565,-74.359273049611,-216.569709262805));
#197767=CARTESIAN_POINT('Origin',(-40.758509388043,-70.2006777120066,-213.798514676938));
#197768=CARTESIAN_POINT('Origin',(0.00331736233953883,957.648657693644,
-233.042565174374));
#197769=CARTESIAN_POINT('Ctrl Pts',(-42.6506409244545,-73.9423397713714,
-216.824911934325));
#197770=CARTESIAN_POINT('Ctrl Pts',(-42.3889675192146,-75.111938779609,
-215.496580546143));
#197771=CARTESIAN_POINT('Ctrl Pts',(-41.9926628230245,-75.1580153204876,
-213.752528187964));
#197772=CARTESIAN_POINT('Ctrl Pts',(-42.5223146433586,-73.9743057102224,
-216.82138777715));
#197773=CARTESIAN_POINT('Ctrl Pts',(-42.2773680112826,-75.1163504965845,
-215.497499167852));
#197774=CARTESIAN_POINT('Ctrl Pts',(-41.9066793323656,-75.1610610934853,
-213.772054913983));
#197775=CARTESIAN_POINT('Ctrl Pts',(-42.3813794284866,-74.0123061097096,
-216.810485774898));
#197776=CARTESIAN_POINT('Ctrl Pts',(-42.1584887885793,-75.1211304958,-215.492781710654));
#197777=CARTESIAN_POINT('Ctrl Pts',(-41.8205323433735,-75.1641318505825,
-213.789924116924));
#197778=CARTESIAN_POINT('Ctrl Pts',(-42.1071714176858,-74.0810920561383,
-216.786773384891));
#197779=CARTESIAN_POINT('Ctrl Pts',(-41.9257553840099,-75.130477399032,
-215.482136500678));
#197780=CARTESIAN_POINT('Ctrl Pts',(-41.6477999581334,-75.1703415381604,
-213.821539717991));
#197781=CARTESIAN_POINT('Ctrl Pts',(-41.9710574680775,-74.1134796538365,
-216.773245626096));
#197782=CARTESIAN_POINT('Ctrl Pts',(-41.8102296619904,-75.1351214208382,
-215.475611436836));
#197783=CARTESIAN_POINT('Ctrl Pts',(-41.5612314342439,-75.1734777382292,
-213.835404439875));
#197784=CARTESIAN_POINT('Ctrl Pts',(-41.6930958560016,-74.1786675398529,
-216.738185296847));
#197785=CARTESIAN_POINT('Ctrl Pts',(-41.5763451014596,-75.1445888151811,
-215.456563678656));
#197786=CARTESIAN_POINT('Ctrl Pts',(-41.3876518834474,-75.1798203744337,
-213.85888373828));
#197787=CARTESIAN_POINT('Ctrl Pts',(-41.550883114529,-74.2117857468627,
-216.716530930408));
#197788=CARTESIAN_POINT('Ctrl Pts',(-41.4577834622525,-75.1494218955762,
-215.443955718173));
#197789=CARTESIAN_POINT('Ctrl Pts',(-41.3006463902462,-75.1830256709096,
-213.868551556967));
#197790=CARTESIAN_POINT('Ctrl Pts',(-41.242598522617,-74.2859889768,-216.652644382786));
#197791=CARTESIAN_POINT('Ctrl Pts',(-41.2077086856973,-75.1598056161709,
-215.404074252949));
#197792=CARTESIAN_POINT('Ctrl Pts',(-41.1260290981951,-75.1895400074146,
-213.882061105839));
#197793=CARTESIAN_POINT('Ctrl Pts',(-41.0767448132029,-74.3265280314252,
-216.609717214661));
#197794=CARTESIAN_POINT('Ctrl Pts',(-41.0764186051261,-75.16535240508,-215.376453037305));
#197795=CARTESIAN_POINT('Ctrl Pts',(-41.0384011165336,-75.1928537189709,
-213.885671097976));
#197796=CARTESIAN_POINT('Ctrl Pts',(-40.9214983001269,-74.359273049532,
-216.569709262896));
#197797=CARTESIAN_POINT('Ctrl Pts',(-40.9511754272514,-75.170618016854,
-215.350418326772));
#197798=CARTESIAN_POINT('Ctrl Pts',(-40.9503927097334,-75.1962323487397,
-213.885776709125));
#197799=CARTESIAN_POINT('',(-42.6506409244548,-73.9423397713703,-216.824911934326));
#197800=CARTESIAN_POINT('',(-41.992662823025,-75.1580153204871,-213.752528187964));
#197801=CARTESIAN_POINT('Origin',(-41.7958961124187,-70.1626506491805,-213.665266155779));
#197802=CARTESIAN_POINT('Ctrl Pts',(-42.6506409244548,-73.9423397713703,
-216.824911934326));
#197803=CARTESIAN_POINT('Ctrl Pts',(-42.5223146433586,-73.9743057102224,
-216.82138777715));
#197804=CARTESIAN_POINT('Ctrl Pts',(-42.3813794284866,-74.0123061097096,
-216.810485774898));
#197805=CARTESIAN_POINT('Ctrl Pts',(-42.1071714176858,-74.0810920561383,
-216.786773384891));
#197806=CARTESIAN_POINT('Ctrl Pts',(-41.9710574680775,-74.1134796538365,
-216.773245626096));
#197807=CARTESIAN_POINT('Ctrl Pts',(-41.6930958560016,-74.1786675398529,
-216.738185296847));
#197808=CARTESIAN_POINT('Ctrl Pts',(-41.550883114529,-74.2117857468627,
-216.716530930408));
#197809=CARTESIAN_POINT('Ctrl Pts',(-41.242598522617,-74.2859889768,-216.652644382786));
#197810=CARTESIAN_POINT('Ctrl Pts',(-41.0767448132029,-74.3265280314252,
-216.609717214661));
#197811=CARTESIAN_POINT('Ctrl Pts',(-40.921498300133,-74.359273049617,-216.569709262785));
#197812=CARTESIAN_POINT('Ctrl Pts',(-40.9503927122327,-75.1962323486438,
-213.885776709122));
#197813=CARTESIAN_POINT('Ctrl Pts',(-41.038474251468,-75.1928509113325,
-213.885671010147));
#197814=CARTESIAN_POINT('Ctrl Pts',(-41.1260976159204,-75.1895374500551,
-213.882055874295));
#197815=CARTESIAN_POINT('Ctrl Pts',(-41.2133377538232,-75.1862828366116,
-213.875306456161));
#197816=CARTESIAN_POINT('Ctrl Pts',(-41.3007070198063,-75.1830234058673,
-213.868547047908));
#197817=CARTESIAN_POINT('Ctrl Pts',(-41.3877081322113,-75.1798183151619,
-213.858876354798));
#197818=CARTESIAN_POINT('Ctrl Pts',(-41.4744416790084,-75.1766490529395,
-213.847144238352));
#197819=CARTESIAN_POINT('Ctrl Pts',(-41.5612776272754,-75.1734760489456,
-213.835398270449));
#197820=CARTESIAN_POINT('Ctrl Pts',(-41.6478454293514,-75.1703399027888,
-213.821531434941));
#197821=CARTESIAN_POINT('Ctrl Pts',(-41.7341661542901,-75.1672366938954,
-213.805731936782));
#197822=CARTESIAN_POINT('Ctrl Pts',(-41.8205769753023,-75.1641302460704,
-213.789915948114));
#197823=CARTESIAN_POINT('Ctrl Pts',(-41.9067233040908,-75.1610595358852,
-213.772044928068));
#197824=CARTESIAN_POINT('Ctrl Pts',(-41.9926628230246,-75.1580153204876,
-213.752528187964));
#197825=CARTESIAN_POINT('Ctrl Pts',(-41.9926628230233,-75.1580153204872,
-213.752528187965));
#197826=CARTESIAN_POINT('Ctrl Pts',(-42.3889675192142,-75.1119387796086,
-215.496580546144));
#197827=CARTESIAN_POINT('Ctrl Pts',(-42.650640924455,-73.9423397713704,
-216.824911934326));
#197828=CARTESIAN_POINT('Ctrl Pts',(-42.2441904201252,-75.1486693658634,
-213.720374383032));
#197829=CARTESIAN_POINT('Ctrl Pts',(-42.6352341484771,-75.0934987178605,
-215.491846788295));
#197830=CARTESIAN_POINT('Ctrl Pts',(-42.8635176930321,-73.8893123883119,
-216.830758067302));
#197831=CARTESIAN_POINT('Ctrl Pts',(-42.4949766531494,-75.1309696159339,
-213.689703299478));
#197832=CARTESIAN_POINT('Ctrl Pts',(-42.8751575352819,-75.0674875232695,
-215.483919014076));
#197833=CARTESIAN_POINT('Ctrl Pts',(-43.0658447951879,-73.8361356612473,
-216.831614746056));
#197834=CARTESIAN_POINT('Ctrl Pts',(-42.9950456426682,-75.0789259129276,
-213.631395393625));
#197835=CARTESIAN_POINT('Ctrl Pts',(-43.3573635301376,-74.9997783248717,
-215.472578146401));
#197836=CARTESIAN_POINT('Ctrl Pts',(-43.4723745746873,-73.7138512147641,
-216.837059076436));
#197837=CARTESIAN_POINT('Ctrl Pts',(-43.244282955429,-75.0445859118617,
-213.603599246343));
#197838=CARTESIAN_POINT('Ctrl Pts',(-43.6008375706358,-74.9576518167014,
-215.469588054037));
#197839=CARTESIAN_POINT('Ctrl Pts',(-43.6783947191598,-73.6431300259591,
-216.842077816832));
#197840=CARTESIAN_POINT('Ctrl Pts',(-43.7407999450918,-74.9592348987093,
-213.549700262593));
#197841=CARTESIAN_POINT('Ctrl Pts',(-44.0847915726919,-74.8574180597928,
-215.462932027522));
#197842=CARTESIAN_POINT('Ctrl Pts',(-44.0841000052998,-73.4910414674771,
-216.849773863078));
#197843=CARTESIAN_POINT('Ctrl Pts',(-43.9880896420054,-74.9082283395953,
-213.523624316504));
#197844=CARTESIAN_POINT('Ctrl Pts',(-44.3242556788489,-74.7995069031645,
-215.458703822069));
#197845=CARTESIAN_POINT('Ctrl Pts',(-44.2823909841006,-73.4109348364935,
-216.851832092541));
#197846=CARTESIAN_POINT('Ctrl Pts',(-44.4808857844271,-74.7891870797402,
-213.473791302964));
#197847=CARTESIAN_POINT('Ctrl Pts',(-44.7955537966533,-74.6692676550458,
-215.447631213062));
#197848=CARTESIAN_POINT('Ctrl Pts',(-44.6664888328127,-73.2472194754336,
-216.851891665016));
#197849=CARTESIAN_POINT('Ctrl Pts',(-44.7267891899937,-74.7210209447827,
-213.450088190094));
#197850=CARTESIAN_POINT('Ctrl Pts',(-45.0291379688623,-74.5965659081431,
-215.441811276339));
#197851=CARTESIAN_POINT('Ctrl Pts',(-44.8547955882521,-73.161697166002,
-216.851063156481));
#197852=CARTESIAN_POINT('Ctrl Pts',(-45.0928291473126,-74.606027152532,
-213.416036405768));
#197853=CARTESIAN_POINT('Ctrl Pts',(-45.3816384584871,-74.4740602974644,
-215.436515048508));
#197854=CARTESIAN_POINT('Ctrl Pts',(-45.1406078814123,-73.0181691132047,
-216.852776982251));
#197855=CARTESIAN_POINT('Ctrl Pts',(-45.2142260714279,-74.5656241152041,
-213.404928397061));
#197856=CARTESIAN_POINT('Ctrl Pts',(-45.5004898449934,-74.4305954967414,
-215.435878858443));
#197857=CARTESIAN_POINT('Ctrl Pts',(-45.2377029692462,-72.9663736632951,
-216.854423557714));
#197858=CARTESIAN_POINT('Ctrl Pts',(-45.4557176198781,-74.4806914809372,
-213.382939645029));
#197859=CARTESIAN_POINT('Ctrl Pts',(-45.7358730844374,-74.3399851570232,
-215.4337505975));
#197860=CARTESIAN_POINT('Ctrl Pts',(-45.4288319445799,-72.8615155438485,
-216.85653065457));
#197861=CARTESIAN_POINT('Ctrl Pts',(-45.5757446359476,-74.4361813329049,
-213.372122623239));
#197862=CARTESIAN_POINT('Ctrl Pts',(-45.8501188293173,-74.2937160035012,
-215.431078613902));
#197863=CARTESIAN_POINT('Ctrl Pts',(-45.5198481005889,-72.8116610800095,
-216.855759513965));
#197864=CARTESIAN_POINT('Ctrl Pts',(-45.9328087572912,-74.2968675255704,
-213.340776903277));
#197865=CARTESIAN_POINT('Ctrl Pts',(-46.1873653169248,-74.1508282744403,
-215.422045951277));
#197866=CARTESIAN_POINT('Ctrl Pts',(-45.7862796787808,-72.6630395831569,
-216.852106972262));
#197867=CARTESIAN_POINT('Ctrl Pts',(-46.1672258662825,-74.1961452862474,
-213.321432015398));
#197868=CARTESIAN_POINT('Ctrl Pts',(-46.4036505792935,-74.0508269587878,
-215.414220291772));
#197869=CARTESIAN_POINT('Ctrl Pts',(-45.9538518097036,-72.5669178021949,
-216.847424766396));
#197870=CARTESIAN_POINT('Ctrl Pts',(-46.5133864112104,-74.0333951639031,
-213.29438225272));
#197871=CARTESIAN_POINT('Ctrl Pts',(-46.7325370368903,-73.8859308362923,
-215.40853678471));
#197872=CARTESIAN_POINT('Ctrl Pts',(-46.2132892873817,-72.4014855733941,
-216.846116620724));
#197873=CARTESIAN_POINT('Ctrl Pts',(-46.6278478339336,-73.977206798173,
-213.285618874285));
#197874=CARTESIAN_POINT('Ctrl Pts',(-46.8439967269085,-73.8278355227286,
-215.408064094516));
#197875=CARTESIAN_POINT('Ctrl Pts',(-46.3023963850082,-72.3411661322158,
-216.847039252521));
#197876=CARTESIAN_POINT('Ctrl Pts',(-46.8548608425726,-73.8609873091134,
-213.268274976754));
#197877=CARTESIAN_POINT('Ctrl Pts',(-47.0648456467714,-73.7079559631609,
-215.406504660188));
#197878=CARTESIAN_POINT('Ctrl Pts',(-46.478613276723,-72.2185871221317,
-216.848037413775));
#197879=CARTESIAN_POINT('Ctrl Pts',(-46.9674078997609,-73.8009605736129,
-213.259666405965));
#197880=CARTESIAN_POINT('Ctrl Pts',(-47.1733859838122,-73.6465693372023,
-215.404947296863));
#197881=CARTESIAN_POINT('Ctrl Pts',(-46.5646834624717,-72.1575736757065,
-216.847643933755));
#197882=CARTESIAN_POINT('Ctrl Pts',(-47.1348908422149,-73.7079618268568,
-213.247450860245));
#197883=CARTESIAN_POINT('Ctrl Pts',(-47.3249946652538,-73.5575902386026,
-215.398041248184));
#197884=CARTESIAN_POINT('Ctrl Pts',(-46.6799581763352,-72.0805586557944,
-216.842417562875));
#197885=CARTESIAN_POINT('Ctrl Pts',(-47.1904997834943,-73.6764658823064,
-213.243519901462));
#197886=CARTESIAN_POINT('Ctrl Pts',(-47.3742816457676,-73.5281301342516,
-215.395327330629));
#197887=CARTESIAN_POINT('Ctrl Pts',(-46.7168699475549,-72.05633006151,-216.840249166734));
#197888=CARTESIAN_POINT('Ctrl Pts',(-47.3012779792568,-73.612476222395,
-213.235940031067));
#197889=CARTESIAN_POINT('Ctrl Pts',(-47.4738788426063,-73.4675943998322,
-215.39080987434));
#197890=CARTESIAN_POINT('Ctrl Pts',(-46.7922015926475,-72.005114703694,
-216.836785542713));
#197891=CARTESIAN_POINT('Ctrl Pts',(-47.3564465382692,-73.5799829806332,
-213.232287185893));
#197892=CARTESIAN_POINT('Ctrl Pts',(-47.5236661359778,-73.4368125264023,
-215.388740875334));
#197893=CARTESIAN_POINT('Ctrl Pts',(-46.8299530635768,-71.9789628961022,
-216.835225967646));
#197894=CARTESIAN_POINT('Ctrl Pts',(-47.5212831512919,-73.4810018009163,
-213.221720566444));
#197895=CARTESIAN_POINT('Ctrl Pts',(-47.6725708647175,-73.3431501790447,
-215.382801668109));
#197896=CARTESIAN_POINT('Ctrl Pts',(-46.9429621731836,-71.8996192326861,
-216.830756524433));
#197897=CARTESIAN_POINT('Ctrl Pts',(-47.6302808905533,-73.4130142912104,
-213.215183926779));
#197898=CARTESIAN_POINT('Ctrl Pts',(-47.7711941360104,-73.2789527469259,
-215.379175449449));
#197899=CARTESIAN_POINT('Ctrl Pts',(-47.017973525604,-71.8455276788576,
-216.82803305392));
#197900=CARTESIAN_POINT('Ctrl Pts',(-47.7383831769164,-73.3429891884104,
-213.20923907124));
#197901=CARTESIAN_POINT('Ctrl Pts',(-47.8674267413588,-73.2141877251374,
-215.374920075633));
#197902=CARTESIAN_POINT('Ctrl Pts',(-47.090555767608,-71.7934728593479,
-216.824560386716));
#197903=CARTESIAN_POINT('',(-47.0905557676078,-71.7934728593479,-216.824560386716));
#197904=CARTESIAN_POINT('',(-47.738383176916,-73.3429891884109,-213.20923907124));
#197905=CARTESIAN_POINT('Origin',(-45.0170666017296,-69.1493247484068,-213.121977039054));
#197906=CARTESIAN_POINT('Ctrl Pts',(-47.0905557676078,-71.7934728593479,
-216.824560386716));
#197907=CARTESIAN_POINT('Ctrl Pts',(-47.017973525604,-71.8455276788576,
-216.82803305392));
#197908=CARTESIAN_POINT('Ctrl Pts',(-46.9429621731836,-71.8996192326861,
-216.830756524433));
#197909=CARTESIAN_POINT('Ctrl Pts',(-46.8299530635768,-71.9789628961022,
-216.835225967646));
#197910=CARTESIAN_POINT('Ctrl Pts',(-46.7922015926475,-72.005114703694,
-216.836785542713));
#197911=CARTESIAN_POINT('Ctrl Pts',(-46.7168699475549,-72.05633006151,-216.840249166734));
#197912=CARTESIAN_POINT('Ctrl Pts',(-46.6799581763352,-72.0805586557944,
-216.842417562875));
#197913=CARTESIAN_POINT('Ctrl Pts',(-46.5646834624717,-72.1575736757065,
-216.847643933755));
#197914=CARTESIAN_POINT('Ctrl Pts',(-46.478613276723,-72.2185871221317,
-216.848037413775));
#197915=CARTESIAN_POINT('Ctrl Pts',(-46.3023963850082,-72.3411661322158,
-216.847039252521));
#197916=CARTESIAN_POINT('Ctrl Pts',(-46.2132892873817,-72.4014855733941,
-216.846116620724));
#197917=CARTESIAN_POINT('Ctrl Pts',(-45.9538518097036,-72.5669178021949,
-216.847424766396));
#197918=CARTESIAN_POINT('Ctrl Pts',(-45.7862796787808,-72.6630395831569,
-216.852106972262));
#197919=CARTESIAN_POINT('Ctrl Pts',(-45.5198481005889,-72.8116610800095,
-216.855759513965));
#197920=CARTESIAN_POINT('Ctrl Pts',(-45.4288319445799,-72.8615155438485,
-216.85653065457));
#197921=CARTESIAN_POINT('Ctrl Pts',(-45.2377029692462,-72.9663736632951,
-216.854423557714));
#197922=CARTESIAN_POINT('Ctrl Pts',(-45.1406078814123,-73.0181691132047,
-216.852776982251));
#197923=CARTESIAN_POINT('Ctrl Pts',(-44.8547955882521,-73.161697166002,
-216.851063156481));
#197924=CARTESIAN_POINT('Ctrl Pts',(-44.6664888328127,-73.2472194754336,
-216.851891665016));
#197925=CARTESIAN_POINT('Ctrl Pts',(-44.2823909841006,-73.4109348364935,
-216.851832092541));
#197926=CARTESIAN_POINT('Ctrl Pts',(-44.0841000052998,-73.4910414674771,
-216.849773863078));
#197927=CARTESIAN_POINT('Ctrl Pts',(-43.6783947191598,-73.6431300259591,
-216.842077816832));
#197928=CARTESIAN_POINT('Ctrl Pts',(-43.4723745746873,-73.7138512147641,
-216.837059076436));
#197929=CARTESIAN_POINT('Ctrl Pts',(-43.0658447951879,-73.8361356612473,
-216.831614746056));
#197930=CARTESIAN_POINT('Ctrl Pts',(-42.8635176930321,-73.8893123883119,
-216.830758067302));
#197931=CARTESIAN_POINT('Ctrl Pts',(-42.6506409244548,-73.9423397713703,
-216.824911934326));
#197932=CARTESIAN_POINT('Ctrl Pts',(-41.992662823025,-75.1580153204871,
-213.752528187964));
#197933=CARTESIAN_POINT('Ctrl Pts',(-42.2441904201252,-75.1486693658634,
-213.720374383032));
#197934=CARTESIAN_POINT('Ctrl Pts',(-42.4949766531494,-75.1309696159339,
-213.689703299478));
#197935=CARTESIAN_POINT('Ctrl Pts',(-42.9950456426682,-75.0789259129276,
-213.631395393625));
#197936=CARTESIAN_POINT('Ctrl Pts',(-43.244282955429,-75.0445859118617,
-213.603599246343));
#197937=CARTESIAN_POINT('Ctrl Pts',(-43.7407999450918,-74.9592348987093,
-213.549700262593));
#197938=CARTESIAN_POINT('Ctrl Pts',(-43.9880896420054,-74.9082283395953,
-213.523624316504));
#197939=CARTESIAN_POINT('Ctrl Pts',(-44.4808857844271,-74.7891870797402,
-213.473791302964));
#197940=CARTESIAN_POINT('Ctrl Pts',(-44.7267891899937,-74.7210209447827,
-213.450088190094));
#197941=CARTESIAN_POINT('Ctrl Pts',(-45.0928291473126,-74.606027152532,
-213.416036405768));
#197942=CARTESIAN_POINT('Ctrl Pts',(-45.2142260714279,-74.5656241152041,
-213.404928397061));
#197943=CARTESIAN_POINT('Ctrl Pts',(-45.4557176198781,-74.4806914809372,
-213.382939645029));
#197944=CARTESIAN_POINT('Ctrl Pts',(-45.5757446359476,-74.4361813329049,
-213.372122623239));
#197945=CARTESIAN_POINT('Ctrl Pts',(-45.9328087572912,-74.2968675255704,
-213.340776903277));
#197946=CARTESIAN_POINT('Ctrl Pts',(-46.1672258662825,-74.1961452862474,
-213.321432015398));
#197947=CARTESIAN_POINT('Ctrl Pts',(-46.5133864112104,-74.0333951639031,
-213.29438225272));
#197948=CARTESIAN_POINT('Ctrl Pts',(-46.6278478339336,-73.977206798173,
-213.285618874285));
#197949=CARTESIAN_POINT('Ctrl Pts',(-46.8548608425726,-73.8609873091134,
-213.268274976754));
#197950=CARTESIAN_POINT('Ctrl Pts',(-46.9674078997609,-73.8009605736129,
-213.259666405965));
#197951=CARTESIAN_POINT('Ctrl Pts',(-47.1348908422149,-73.7079618268568,
-213.247450860245));
#197952=CARTESIAN_POINT('Ctrl Pts',(-47.1904997834943,-73.6764658823064,
-213.243519901462));
#197953=CARTESIAN_POINT('Ctrl Pts',(-47.3012779792568,-73.612476222395,
-213.235940031067));
#197954=CARTESIAN_POINT('Ctrl Pts',(-47.3564465382692,-73.5799829806332,
-213.232287185893));
#197955=CARTESIAN_POINT('Ctrl Pts',(-47.5212831512919,-73.4810018009163,
-213.221720566444));
#197956=CARTESIAN_POINT('Ctrl Pts',(-47.6302808905533,-73.4130142912104,
-213.215183926779));
#197957=CARTESIAN_POINT('Ctrl Pts',(-47.738383176916,-73.3429891884109,
-213.20923907124));
#197958=CARTESIAN_POINT('Ctrl Pts',(-47.6826029798323,-71.3710801272352,
-216.791855002172));
#197959=CARTESIAN_POINT('Ctrl Pts',(-48.7033558856732,-72.5944415704724,
-215.339600005589));
#197960=CARTESIAN_POINT('Ctrl Pts',(-48.7454044931546,-72.6086641314349,
-213.184229057458));
#197961=CARTESIAN_POINT('Ctrl Pts',(-47.4907935026769,-71.5238447202,-216.792044585111));
#197962=CARTESIAN_POINT('Ctrl Pts',(-48.4312469413224,-72.815727223767,
-215.339098369127));
#197963=CARTESIAN_POINT('Ctrl Pts',(-48.4201758660461,-72.8745352082661,
-213.18165597563));
#197964=CARTESIAN_POINT('Ctrl Pts',(-47.2933342138992,-71.6644126162078,
-216.803168697205));
#197965=CARTESIAN_POINT('Ctrl Pts',(-48.1524733410987,-73.0220158932609,
-215.351128153924));
#197966=CARTESIAN_POINT('Ctrl Pts',(-48.0843074405244,-73.1189108367624,
-213.190215709169));
#197967=CARTESIAN_POINT('Ctrl Pts',(-47.0905557676078,-71.7934728593478,
-216.824560386716));
#197968=CARTESIAN_POINT('Ctrl Pts',(-47.8674267413582,-73.2141877251378,
-215.374920075632));
#197969=CARTESIAN_POINT('Ctrl Pts',(-47.7383831769152,-73.3429891884114,
-213.20923907124));
#197970=CARTESIAN_POINT('',(-47.6826029798323,-71.3710801272351,-216.791855002172));
#197971=CARTESIAN_POINT('',(-48.7454044931547,-72.6086641314348,-213.184229057458));
#197972=CARTESIAN_POINT('Origin',(-45.5817163713881,-68.7378163165586,-213.096967025272));
#197973=CARTESIAN_POINT('Ctrl Pts',(-47.6826029798323,-71.3710801272352,
-216.791855002172));
#197974=CARTESIAN_POINT('Ctrl Pts',(-47.5930241853469,-71.4424241944854,
-216.791943540536));
#197975=CARTESIAN_POINT('Ctrl Pts',(-47.5017703583274,-71.5114565089323,
-216.794420184509));
#197976=CARTESIAN_POINT('Ctrl Pts',(-47.4089903165443,-71.5780732055786,
-216.799270679166));
#197977=CARTESIAN_POINT('Ctrl Pts',(-47.3150167558955,-71.6455468568316,
-216.804183570399));
#197978=CARTESIAN_POINT('Ctrl Pts',(-47.21947748162,-71.7105423794927,-216.811531734658));
#197979=CARTESIAN_POINT('Ctrl Pts',(-47.1225445138657,-71.7729893063581,
-216.821266633423));
#197980=CARTESIAN_POINT('Ctrl Pts',(-47.1118983132863,-71.7798478863064,
-216.82233582265));
#197981=CARTESIAN_POINT('Ctrl Pts',(-47.1012353177767,-71.7866757595247,
-216.823433769832));
#197982=CARTESIAN_POINT('Ctrl Pts',(-47.0905557676078,-71.7934728593478,
-216.824560386716));
#197983=CARTESIAN_POINT('Origin',(-42.892397296669,-65.4915301102559,-217.548968570462));
#197984=CARTESIAN_POINT('Ctrl Pts',(-48.7454044931547,-72.6086641314348,
-213.184229057458));
#197985=CARTESIAN_POINT('Ctrl Pts',(-48.7033558856732,-72.5944415704724,
-215.339600005589));
#197986=CARTESIAN_POINT('Ctrl Pts',(-47.6826029798322,-71.3710801272353,
-216.791855002172));
#197987=CARTESIAN_POINT('Ctrl Pts',(-49.8084038141049,-71.7395463911352,
-213.19825784801));
#197988=CARTESIAN_POINT('Ctrl Pts',(-49.7617328576239,-71.7299417528012,
-215.340395531801));
#197989=CARTESIAN_POINT('Ctrl Pts',(-48.7278636856231,-70.5385934819214,
-216.79082188204));
#197990=CARTESIAN_POINT('Ctrl Pts',(-50.8549407258151,-70.835967150169,
-213.213888015999));
#197991=CARTESIAN_POINT('Ctrl Pts',(-50.8130965389169,-70.8232845235791,
-215.341943634174));
#197992=CARTESIAN_POINT('Ctrl Pts',(-49.772756291054,-69.6608348552585,
-216.790293600156));
#197993=CARTESIAN_POINT('Ctrl Pts',(-51.8687937432179,-69.9121576054873,
-213.227785479717));
#197994=CARTESIAN_POINT('Ctrl Pts',(-51.8269633350129,-69.9002951910831,
-215.34395680141));
#197995=CARTESIAN_POINT('Ctrl Pts',(-50.7746555306532,-68.7687177611616,
-216.79041881877));
#197996=CARTESIAN_POINT('Origin',(-46.9277583887874,-69.2440043695137,-216.824274994638));
#197997=CARTESIAN_POINT('Ctrl Pts',(-48.7454044931547,-72.6086641314348,
-213.184229057458));
#197998=CARTESIAN_POINT('Ctrl Pts',(-49.8020589781625,-71.7447339856784,
-213.198174112891));
#197999=CARTESIAN_POINT('Ctrl Pts',(-50.8424469892599,-70.8467524994813,
-213.213701486193));
#198000=CARTESIAN_POINT('Ctrl Pts',(-51.8506358032439,-69.9286975854465,
-213.227536545096));
#198001=CARTESIAN_POINT('Origin',(5.34244157628528E-6,47.3246585720436,
-196.660871591801));
#198002=CARTESIAN_POINT('',(0.,53.3225191912041,-213.879601465234));
#198003=CARTESIAN_POINT('',(-1.6965687653276E-15,52.4792326277482,-216.572278947217));
#198004=CARTESIAN_POINT('Origin',(1.82415280199159E-13,48.3232807154221,
-213.792339433049));
#198005=CARTESIAN_POINT('',(-0.0544835933803365,52.4792219709058,-216.572215033819));
#198006=CARTESIAN_POINT('Origin',(-0.0318049166815379,52.4691014048544,
-216.511517174968));
#198007=CARTESIAN_POINT('',(-0.0473571427401393,53.3225154460666,-213.879539002147));
#198008=CARTESIAN_POINT('Origin',(-0.0463362411570871,48.3232770745245,
-213.79227696996));
#198009=CARTESIAN_POINT('Origin',(-0.46976145343121,53.0041184688829,-208.56971754274));
#198010=CARTESIAN_POINT('Ctrl Pts',(-0.0544838121610982,52.4791654811938,
-216.572299482171));
#198011=CARTESIAN_POINT('Ctrl Pts',(-0.0513170628758878,53.2968486113713,
-215.349944618211));
#198012=CARTESIAN_POINT('Ctrl Pts',(-0.0473571427401181,53.3225154460666,
-213.879539002147));
#198013=CARTESIAN_POINT('Ctrl Pts',(-1.72631364479056,52.4785114930465,
-216.568377409431));
#198014=CARTESIAN_POINT('Ctrl Pts',(-1.6261124312647,53.2965689361806,-215.346119637512));
#198015=CARTESIAN_POINT('Ctrl Pts',(-1.50078629177953,53.3222855571144,
-213.875705279281));
#198016=CARTESIAN_POINT('Ctrl Pts',(-3.36619303951308,52.4477003743405,
-216.38454765132));
#198017=CARTESIAN_POINT('Ctrl Pts',(-3.17354336684182,53.2833995412461,
-215.166295535093));
#198018=CARTESIAN_POINT('Ctrl Pts',(-2.92702243085717,53.3114912412646,
-213.695947807356));
#198019=CARTESIAN_POINT('Ctrl Pts',(-5.02403903766868,52.3888604794127,
-216.029604597611));
#198020=CARTESIAN_POINT('Ctrl Pts',(-4.73705181005364,53.2579964078456,
-214.820557484925));
#198021=CARTESIAN_POINT('Ctrl Pts',(-4.37281940663811,53.2905575229658,
-213.348880503444));
#198022=CARTESIAN_POINT('Ctrl Pts',(-5.07424920625965,52.3870512560605,
-216.018691745657));
#198023=CARTESIAN_POINT('Ctrl Pts',(-4.78447983975736,53.2572141001589,
-214.809911386444));
#198024=CARTESIAN_POINT('Ctrl Pts',(-4.4166077184939,53.289913868413,-213.338209943704));
#198025=CARTESIAN_POINT('Ctrl Pts',(-5.1369792265556,52.3847567936962,-216.004854723837));
#198026=CARTESIAN_POINT('Ctrl Pts',(-4.84373380419663,53.2562221185161,
-214.79641336836));
#198027=CARTESIAN_POINT('Ctrl Pts',(-4.47131352346949,53.2890977177666,
-213.324680435774));
#198028=CARTESIAN_POINT('Ctrl Pts',(-5.14483151826084,52.385083371175,-216.002211218262));
#198029=CARTESIAN_POINT('Ctrl Pts',(-4.8529857001896,53.2560738876406,-214.793661486801));
#198030=CARTESIAN_POINT('Ctrl Pts',(-4.48225430767022,53.2889337622212,
-213.321972140265));
#198031=CARTESIAN_POINT('Ctrl Pts',(-5.16354659654888,52.3852300457096,
-215.996869330628));
#198032=CARTESIAN_POINT('Ctrl Pts',(-4.87315904092074,53.2557430575767,
-214.788216412269));
#198033=CARTESIAN_POINT('Ctrl Pts',(-4.50414007083122,53.2886037420393,
-213.316582951083));
#198034=CARTESIAN_POINT('Ctrl Pts',(-5.17290526355219,52.3853021345043,
-215.994206794316));
#198035=CARTESIAN_POINT('Ctrl Pts',(-4.88324702370802,53.2555768088776,
-214.78550260211));
#198036=CARTESIAN_POINT('Ctrl Pts',(-4.51508431353993,53.2884377751688,
-213.313897267951));
#198037=CARTESIAN_POINT('Ctrl Pts',(-5.20098465409101,52.385514651656,-215.986244424357));
#198038=CARTESIAN_POINT('Ctrl Pts',(-4.91351451474929,53.2550755663235,
-214.777387478169));
#198039=CARTESIAN_POINT('Ctrl Pts',(-4.54792112758205,53.2879370021236,
-213.30586696962));
#198040=CARTESIAN_POINT('Ctrl Pts',(-5.21970876708894,52.38565133079,-215.980969829665));
#198041=CARTESIAN_POINT('Ctrl Pts',(-4.93369836198372,53.254738063078,-214.772012254543));
#198042=CARTESIAN_POINT('Ctrl Pts',(-4.56981778482713,53.2875993235168,
-213.300549105442));
#198043=CARTESIAN_POINT('Ctrl Pts',(-5.31335200957375,52.3863096810235,
-215.954765336006));
#198044=CARTESIAN_POINT('Ctrl Pts',(-5.03463605558215,53.253033966418,-214.745313113829));
#198045=CARTESIAN_POINT('Ctrl Pts',(-4.67932834466443,53.2858917529302,
-213.274138348232));
#198046=CARTESIAN_POINT('Ctrl Pts',(-5.38833916300533,52.3867562150194,
-215.934340872373));
#198047=CARTESIAN_POINT('Ctrl Pts',(-5.11547694549389,53.2516171105571,
-214.724511598889));
#198048=CARTESIAN_POINT('Ctrl Pts',(-4.76702406702058,53.2844643286531,
-213.253581139954));
#198049=CARTESIAN_POINT('Ctrl Pts',(-5.61352154702286,52.3878534578465,
-215.874693437342));
#198050=CARTESIAN_POINT('Ctrl Pts',(-5.35822907168792,53.2472055317345,
-214.663801477364));
#198051=CARTESIAN_POINT('Ctrl Pts',(-5.03037439099589,53.2799968687432,
-213.193632432869));
#198052=CARTESIAN_POINT('Ctrl Pts',(-5.76393762412216,52.3882617916828,
-215.837096372224));
#198053=CARTESIAN_POINT('Ctrl Pts',(-5.52042156751042,53.2440489818281,
-214.625572928414));
#198054=CARTESIAN_POINT('Ctrl Pts',(-5.20629213894649,53.2767716505112,
-213.155963782957));
#198055=CARTESIAN_POINT('Ctrl Pts',(-6.21609808576436,52.3885024391131,
-215.730879287284));
#198056=CARTESIAN_POINT('Ctrl Pts',(-6.00793734859214,53.2339271751484,
-214.517735436117));
#198057=CARTESIAN_POINT('Ctrl Pts',(-5.7351090490271,53.2663464299268,-213.049921731156));
#198058=CARTESIAN_POINT('Ctrl Pts',(-6.51897325761332,52.3873481165059,
-215.6687950942));
#198059=CARTESIAN_POINT('Ctrl Pts',(-6.33464333385786,53.226300180748,-214.45488048842));
#198060=CARTESIAN_POINT('Ctrl Pts',(-6.08932836962055,53.2583903798102,
-212.988474563998));
#198061=CARTESIAN_POINT('Ctrl Pts',(-7.43009426840034,52.3798510205839,
-215.509670650059));
#198062=CARTESIAN_POINT('Ctrl Pts',(-7.31716856464453,53.2007824433048,
-214.294545088556));
#198063=CARTESIAN_POINT('Ctrl Pts',(-7.15467547994453,53.2314932970166,
-212.832839779496));
#198064=CARTESIAN_POINT('Ctrl Pts',(-8.03670071712731,52.3695847260312,
-215.440224224832));
#198065=CARTESIAN_POINT('Ctrl Pts',(-7.97197058059872,53.1803550515563,
-214.225561760305));
#198066=CARTESIAN_POINT('Ctrl Pts',(-7.86408306340235,53.2096427750673,
-212.767811172676));
#198067=CARTESIAN_POINT('Ctrl Pts',(-9.85173860809738,52.3231412296717,
-215.343152516339));
#198068=CARTESIAN_POINT('Ctrl Pts',(-9.93187025910714,53.108960624321,-214.134202008953));
#198069=CARTESIAN_POINT('Ctrl Pts',(-9.98981135051243,53.1323666949439,
-212.690409355922));
#198070=CARTESIAN_POINT('Ctrl Pts',(-11.0568111525605,52.2713911945477,
-215.42554273729));
#198071=CARTESIAN_POINT('Ctrl Pts',(-11.2368319229789,53.0477276627447,
-214.225816329401));
#198072=CARTESIAN_POINT('Ctrl Pts',(-11.4039030903532,53.0652276040471,
-212.794256396899));
#198073=CARTESIAN_POINT('Ctrl Pts',(-12.5473914277697,52.1795355667477,
-215.729436635764));
#198074=CARTESIAN_POINT('Ctrl Pts',(-12.8548033121088,52.9546875149451,
-214.549327186523));
#198075=CARTESIAN_POINT('Ctrl Pts',(-13.1664443334459,52.9616798229913,
-213.138287858349));
#198076=CARTESIAN_POINT('Ctrl Pts',(-12.8444100738279,52.1598101428135,
-215.800296334662));
#198077=CARTESIAN_POINT('Ctrl Pts',(-13.1775953389357,52.935263628279,-214.624547564513));
#198078=CARTESIAN_POINT('Ctrl Pts',(-13.5182905195363,52.9400113359771,
-213.217839110357));
#198079=CARTESIAN_POINT('Ctrl Pts',(-13.1588676265443,52.1373853379567,
-215.886637060861));
#198080=CARTESIAN_POINT('Ctrl Pts',(-13.5195142127268,52.9137765318947,
-214.715953380887));
#198081=CARTESIAN_POINT('Ctrl Pts',(-13.8914034372555,52.9159732378538,
-213.314153161469));
#198082=CARTESIAN_POINT('Ctrl Pts',(-13.1773609898638,52.1360608428166,
-215.891756568308));
#198083=CARTESIAN_POINT('Ctrl Pts',(-13.5396265714153,52.9125092524799,
-214.72137332412));
#198084=CARTESIAN_POINT('Ctrl Pts',(-13.913348594832,52.9145554991733,-213.319862053586));
#198085=CARTESIAN_POINT('Ctrl Pts',(-13.2143394524504,52.1334010639901,
-215.902077029165));
#198086=CARTESIAN_POINT('Ctrl Pts',(-13.5798441312398,52.9099684160984,
-214.732298003386));
#198087=CARTESIAN_POINT('Ctrl Pts',(-13.9572335779769,52.911712557551,-213.331366738555));
#198088=CARTESIAN_POINT('Ctrl Pts',(-13.2429336797444,52.1319007516476,
-215.909182860407));
#198089=CARTESIAN_POINT('Ctrl Pts',(-13.6054337990796,52.9083475768503,
-214.73874381139));
#198090=CARTESIAN_POINT('Ctrl Pts',(-13.9791751707463,52.9102878010619,
-213.337130942174));
#198091=CARTESIAN_POINT('Ctrl Pts',(-13.3196525905457,52.1275217648837,
-215.928540678133));
#198092=CARTESIAN_POINT('Ctrl Pts',(-13.6772913107925,52.9037880649127,
-214.756990320156));
#198093=CARTESIAN_POINT('Ctrl Pts',(-14.0450114907347,52.9060072619919,
-213.354204614097));
#198094=CARTESIAN_POINT('Ctrl Pts',(-13.3707958087157,52.1245713270207,
-215.94124689702));
#198095=CARTESIAN_POINT('Ctrl Pts',(-13.7251992193788,52.9007367776418,
-214.76896183255));
#198096=CARTESIAN_POINT('Ctrl Pts',(-14.088912169659,52.9031437987813,-213.36539506595));
#198097=CARTESIAN_POINT('Ctrl Pts',(-13.5242193311591,52.1156270333207,
-215.978772604734));
#198098=CARTESIAN_POINT('Ctrl Pts',(-13.8689295059075,52.891548129523,-214.804300670642));
#198099=CARTESIAN_POINT('Ctrl Pts',(-14.2206434120783,52.894523997485,-213.398393774552));
#198100=CARTESIAN_POINT('Ctrl Pts',(-13.6264935272095,52.109540209161,-216.002999208033));
#198101=CARTESIAN_POINT('Ctrl Pts',(-13.9647632011014,52.8853756812463,
-214.827093567687));
#198102=CARTESIAN_POINT('Ctrl Pts',(-14.3085031783526,52.8887382469479,
-213.419629432868));
#198103=CARTESIAN_POINT('Ctrl Pts',(-13.9333070017177,52.0909102906718,
-216.07333725522));
#198104=CARTESIAN_POINT('Ctrl Pts',(-14.2523014370409,52.8667178365155,
-214.893197226102));
#198105=CARTESIAN_POINT('Ctrl Pts',(-14.5721978639792,52.8712625751263,
-213.481070862543));
#198106=CARTESIAN_POINT('Ctrl Pts',(-14.1378374819569,52.0779979063538,
-216.117107824054));
#198107=CARTESIAN_POINT('Ctrl Pts',(-14.4440621069193,52.8540907200264,
-214.934238234567));
#198108=CARTESIAN_POINT('Ctrl Pts',(-14.7481481314415,52.8594542225781,
-213.519011772409));
#198109=CARTESIAN_POINT('Ctrl Pts',(-15.1606137321987,52.0109959618191,
-216.320693501189));
#198110=CARTESIAN_POINT('Ctrl Pts',(-15.4032365304224,52.7900018371231,
-215.124595810338));
#198111=CARTESIAN_POINT('Ctrl Pts',(-15.628651977767,52.799613377438,-213.693903709864));
#198112=CARTESIAN_POINT('Ctrl Pts',(-15.9800466985321,51.9494919248635,
-216.434735900354));
#198113=CARTESIAN_POINT('Ctrl Pts',(-16.1727115912884,52.7356122605164,
-215.22941057846));
#198114=CARTESIAN_POINT('Ctrl Pts',(-16.3354684202618,52.7491845407374,
-213.786320807126));
#198115=CARTESIAN_POINT('Ctrl Pts',(-18.4347031718877,51.7430432922917,
-216.639213100253));
#198116=CARTESIAN_POINT('Ctrl Pts',(-18.4831202248674,52.5631013698916,
-215.410445297568));
#198117=CARTESIAN_POINT('Ctrl Pts',(-18.4626009436692,52.5898921039121,
-213.930740442329));
#198118=CARTESIAN_POINT('Ctrl Pts',(-20.0708093960321,51.5754935237252,
-216.5932389759));
#198119=CARTESIAN_POINT('Ctrl Pts',(-20.0302851577021,52.4352453396046,
-215.353542049237));
#198120=CARTESIAN_POINT('Ctrl Pts',(-19.8895768543743,52.4730122776837,
-213.850322288872));
#198121=CARTESIAN_POINT('Ctrl Pts',(-22.106942925778,51.3343802180279,-216.337037616295));
#198122=CARTESIAN_POINT('Ctrl Pts',(-21.961050385352,52.2595837051689,-215.091027749643));
#198123=CARTESIAN_POINT('Ctrl Pts',(-21.6827252055939,52.3125514421292,
-213.558099210826));
#198124=CARTESIAN_POINT('Ctrl Pts',(-22.5140029611996,51.2845488712585,
-216.275810860144));
#198125=CARTESIAN_POINT('Ctrl Pts',(-22.3483346833126,52.2235374473467,
-215.028730453821));
#198126=CARTESIAN_POINT('Ctrl Pts',(-22.042080438038,52.2797161015951,-213.490009648206));
#198127=CARTESIAN_POINT('Ctrl Pts',(-23.020123969084,51.2205746604136,-216.187808497287));
#198128=CARTESIAN_POINT('Ctrl Pts',(-22.830207401887,52.1776766786295,-214.939815041818));
#198129=CARTESIAN_POINT('Ctrl Pts',(-22.4896859299856,52.237965427953,-213.393843363057));
#198130=CARTESIAN_POINT('Ctrl Pts',(-23.1212414946463,51.207692183615,-216.169631097871));
#198131=CARTESIAN_POINT('Ctrl Pts',(-22.9265597686305,52.1684559716392,
-214.921463855732));
#198132=CARTESIAN_POINT('Ctrl Pts',(-22.5791527085491,52.2295777954781,
-213.374053497716));
#198133=CARTESIAN_POINT('Ctrl Pts',(-23.2475111366351,51.1914790355507,
-216.146197182102));
#198134=CARTESIAN_POINT('Ctrl Pts',(-23.0468999380045,52.1568764972718,
-214.897838328728));
#198135=CARTESIAN_POINT('Ctrl Pts',(-22.690919027762,52.2190463850866,-213.34862868516));
#198136=CARTESIAN_POINT('Ctrl Pts',(-23.2727587011446,51.1882309027779,
-216.141474787588));
#198137=CARTESIAN_POINT('Ctrl Pts',(-23.0709668523537,52.1545575467334,
-214.893078113741));
#198138=CARTESIAN_POINT('Ctrl Pts',(-22.7132689336659,52.216937759573,-213.343509345961));
#198139=CARTESIAN_POINT('Ctrl Pts',(-23.3106206153721,51.1833504374298,
-216.134337938203));
#198140=CARTESIAN_POINT('Ctrl Pts',(-23.1070601888508,52.1510750563128,
-214.885886361002));
#198141=CARTESIAN_POINT('Ctrl Pts',(-22.7467887689227,52.2137713063518,
-213.335778919634));
#198142=CARTESIAN_POINT('Ctrl Pts',(-23.323239681318,51.1817222379552,-216.131950112096));
#198143=CARTESIAN_POINT('Ctrl Pts',(-23.1190905197751,52.1499135108851,
-214.88348045923));
#198144=CARTESIAN_POINT('Ctrl Pts',(-22.7579612100687,52.2127152361208,
-213.333193541222));
#198145=CARTESIAN_POINT('Ctrl Pts',(-23.3484746877927,51.1784630815982,
-216.127156733402));
#198146=CARTESIAN_POINT('Ctrl Pts',(-23.143149110136,52.1475890391182,-214.878651485124));
#198147=CARTESIAN_POINT('Ctrl Pts',(-22.7803044200115,52.2106019240511,
-213.328005669353));
#198148=CARTESIAN_POINT('Ctrl Pts',(-23.3634428804975,51.1759647735806,
-216.125067970779));
#198149=CARTESIAN_POINT('Ctrl Pts',(-23.1565316045267,52.1462872653411,
-214.876515197103));
#198150=CARTESIAN_POINT('Ctrl Pts',(-22.7914750239788,52.2095447316335,
-213.325401286811));
#198151=CARTESIAN_POINT('Ctrl Pts',(-23.4120169921601,51.1731488430113,
-216.111042278681));
#198152=CARTESIAN_POINT('Ctrl Pts',(-23.2083148973916,52.1413255461524,
-214.862589766122));
#198153=CARTESIAN_POINT('Ctrl Pts',(-22.8473256024096,52.204255320697,-213.312356521225));
#198154=CARTESIAN_POINT('Ctrl Pts',(-23.4508800621557,51.1708771222298,
-216.099941976412));
#198155=CARTESIAN_POINT('Ctrl Pts',(-23.2497524300108,52.1373416940334,
-214.851574226443));
#198156=CARTESIAN_POINT('Ctrl Pts',(-22.8920158443542,52.2000074805641,
-213.302049206936));
#198157=CARTESIAN_POINT('Ctrl Pts',(-23.6452138197032,51.1594235544229,
-216.045044240048));
#198158=CARTESIAN_POINT('Ctrl Pts',(-23.4569298224344,52.1173561427463,
-214.797140469721));
#198159=CARTESIAN_POINT('Ctrl Pts',(-23.1155161868917,52.1786865508139,
-213.251157958141));
#198160=CARTESIAN_POINT('Ctrl Pts',(-23.8007397230343,51.1499568445754,
-216.003057863675));
#198161=CARTESIAN_POINT('Ctrl Pts',(-23.6228464558013,52.1011357232831,
-214.755597580258));
#198162=CARTESIAN_POINT('Ctrl Pts',(-23.2944736580691,52.1613682854175,
-213.212509671925));
#198163=CARTESIAN_POINT('Ctrl Pts',(-24.5786315814621,51.1010976638087,
-215.802956909761));
#198164=CARTESIAN_POINT('Ctrl Pts',(-24.4522745552879,52.0189656145359,
-214.558346148694));
#198165=CARTESIAN_POINT('Ctrl Pts',(-24.1900632291284,52.0734578840123,
-213.029785590209));
#198166=CARTESIAN_POINT('Ctrl Pts',(-25.2017886349748,51.057136405924,-215.674251388706));
#198167=CARTESIAN_POINT('Ctrl Pts',(-25.1186390175671,51.9494941764341,
-214.433049242548));
#198168=CARTESIAN_POINT('Ctrl Pts',(-24.9090934498146,51.9989121398783,
-212.917162893819));
#198169=CARTESIAN_POINT('Ctrl Pts',(-26.4489126716066,50.9591801161871,
-215.485243101151));
#198170=CARTESIAN_POINT('Ctrl Pts',(-26.4549089350885,51.8030345541437,
-214.254227764677));
#198171=CARTESIAN_POINT('Ctrl Pts',(-26.3528137916878,51.8410386164186,
-212.765468959114));
#198172=CARTESIAN_POINT('Ctrl Pts',(-27.0728715321185,50.905194894437,-215.424895423793));
#198173=CARTESIAN_POINT('Ctrl Pts',(-27.1250812825516,51.7260329324047,
-214.200467363498));
#198174=CARTESIAN_POINT('Ctrl Pts',(-27.0774998387683,51.7577126118315,
-212.726350375003));
#198175=CARTESIAN_POINT('Ctrl Pts',(-28.0085736911846,50.8162816305668,
-215.391931350205));
#198176=CARTESIAN_POINT('Ctrl Pts',(-28.1331634770288,51.6046724004521,
-214.180352486964));
#198177=CARTESIAN_POINT('Ctrl Pts',(-28.1693846366018,51.6257897144443,
-212.730030329888));
#198178=CARTESIAN_POINT('Ctrl Pts',(-28.3204349415701,50.7853183616886,
-215.390561027108));
#198179=CARTESIAN_POINT('Ctrl Pts',(-28.4695064538021,51.5632633940243,
-214.183737492164));
#198180=CARTESIAN_POINT('Ctrl Pts',(-28.5341580008858,51.5806587006086,
-212.741678726193));
#198181=CARTESIAN_POINT('Ctrl Pts',(-28.9439153079118,50.7206314629095,
-215.408483182069));
#198182=CARTESIAN_POINT('Ctrl Pts',(-29.1429916828581,51.4784709974454,
-214.212257584902));
#198183=CARTESIAN_POINT('Ctrl Pts',(-29.2654690941946,51.4880085266708,
-212.78747147059));
#198184=CARTESIAN_POINT('Ctrl Pts',(-29.2565395236243,50.686794162671,-215.427879478665));
#198185=CARTESIAN_POINT('Ctrl Pts',(-29.4812692925636,51.4349391049166,
-214.237504523825));
#198186=CARTESIAN_POINT('Ctrl Pts',(-29.6331976033025,51.4403305324129,
-212.821772692263));
#198187=CARTESIAN_POINT('Ctrl Pts',(-30.806459665517,50.5117195096438,-215.579673099401));
#198188=CARTESIAN_POINT('Ctrl Pts',(-31.1599649096486,51.2141679617287,
-214.421214926244));
#198189=CARTESIAN_POINT('Ctrl Pts',(-31.462411304102,51.1976497020186,-213.05276291922));
#198190=CARTESIAN_POINT('Ctrl Pts',(-31.9843584339507,50.3555651024278,
-215.871251464859));
#198191=CARTESIAN_POINT('Ctrl Pts',(-32.4487874910326,51.0294672908337,
-214.747007973179));
#198192=CARTESIAN_POINT('Ctrl Pts',(-32.8718379543183,50.9930622692594,
-213.421070504801));
#198193=CARTESIAN_POINT('Ctrl Pts',(-33.0838397730299,50.1837035797222,
-216.356359025309));
#198194=CARTESIAN_POINT('Ctrl Pts',(-33.6643488510553,50.8420575943128,
-215.277907585224));
#198195=CARTESIAN_POINT('Ctrl Pts',(-34.2185104850841,50.7818638678805,
-214.004031647198));
#198196=CARTESIAN_POINT('',(-5.13104565674618,52.3850329666526,-216.006074884366));
#198197=CARTESIAN_POINT('',(-13.2064804354037,52.1340237047487,-215.899796183989));
#198198=CARTESIAN_POINT('Ctrl Pts',(-5.13104565674618,52.3850329666526,
-216.006074884366));
#198199=CARTESIAN_POINT('Ctrl Pts',(-5.13996129572555,52.3849305551879,
-216.003777638489));
#198200=CARTESIAN_POINT('Ctrl Pts',(-5.14656866651012,52.3851571564325,
-216.001626363912));
#198201=CARTESIAN_POINT('Ctrl Pts',(-5.16352658620013,52.3852900305971,
-215.996786043511));
#198202=CARTESIAN_POINT('Ctrl Pts',(-5.19160273719641,52.3855062500636,
-215.988798420711));
#198203=CARTESIAN_POINT('Ctrl Pts',(-5.21968905682423,52.3857112220787,
-215.980886515042));
#198204=CARTESIAN_POINT('Ctrl Pts',(-5.31333279951823,52.3863694172317,
-215.954681976519));
#198205=CARTESIAN_POINT('Ctrl Pts',(-5.38832035449837,52.3868158288539,
-215.93425747843));
#198206=CARTESIAN_POINT('Ctrl Pts',(-5.61350394434034,52.3879127096803,
-215.874609945188));
#198207=CARTESIAN_POINT('Ctrl Pts',(-5.76392083021292,52.3883208090405,
-215.837012820505));
#198208=CARTESIAN_POINT('Ctrl Pts',(-6.2160837221702,52.3885607740694,-215.730795577584));
#198209=CARTESIAN_POINT('Ctrl Pts',(-6.51896053409861,52.3874060244112,
-215.668711303004));
#198210=CARTESIAN_POINT('Ctrl Pts',(-7.43008646643842,52.3799077366994,
-215.509586698213));
#198211=CARTESIAN_POINT('Ctrl Pts',(-8.036696242775,52.3696407673332,-215.440140264245));
#198212=CARTESIAN_POINT('Ctrl Pts',(-9.85174415293088,52.3231956049535,
-215.343068860401));
#198213=CARTESIAN_POINT('Ctrl Pts',(-11.056823612227,52.2714449257332,-215.425459700954));
#198214=CARTESIAN_POINT('Ctrl Pts',(-12.5474126952812,52.1795891926595,
-215.729354992607));
#198215=CARTESIAN_POINT('Ctrl Pts',(-12.8444331215652,52.1598637829641,
-215.800215003222));
#198216=CARTESIAN_POINT('Ctrl Pts',(-13.1588925696086,52.1374390337435,
-215.886556093702));
#198217=CARTESIAN_POINT('Ctrl Pts',(-13.1773860446445,52.1361145420097,
-215.891675622758));
#198218=CARTESIAN_POINT('Ctrl Pts',(-13.199128592437,52.1345506623852,-215.897743822643));
#198219=CARTESIAN_POINT('Ctrl Pts',(-13.2026946227731,52.1343113922399,
-215.898712001111));
#198220=CARTESIAN_POINT('Ctrl Pts',(-13.2064791900476,52.1340213385469,
-215.899799904774));
#198221=CARTESIAN_POINT('',(-23.3713119210585,51.1755743233668,-216.12270611168));
#198222=CARTESIAN_POINT('Ctrl Pts',(-13.206503688621,52.1340678863285,-215.899726709711));
#198223=CARTESIAN_POINT('Ctrl Pts',(-13.224334936536,52.1329279875711,-215.9044768025));
#198224=CARTESIAN_POINT('Ctrl Pts',(-13.2474589747328,52.1316975834026,
-215.910237414342));
#198225=CARTESIAN_POINT('Ctrl Pts',(-13.268531608982,52.1304947844112,-215.915554491141));
#198226=CARTESIAN_POINT('Ctrl Pts',(-13.3196773257302,52.1275754523624,
-215.928459650536));
#198227=CARTESIAN_POINT('Ctrl Pts',(-13.3708203204711,52.1246250082557,
-215.941165817504));
#198228=CARTESIAN_POINT('Ctrl Pts',(-13.4219612714471,52.121643572068,-215.953674335297));
#198229=CARTESIAN_POINT('Ctrl Pts',(-13.524243173399,52.1156806996926,-215.978691370885));
#198230=CARTESIAN_POINT('Ctrl Pts',(-13.6265169244848,52.1095938707609,
-216.002917873277));
#198231=CARTESIAN_POINT('Ctrl Pts',(-13.7287876386344,52.1033838982336,
-216.02636378994));
#198232=CARTESIAN_POINT('Ctrl Pts',(-13.9333290669337,52.0909639531789,
-216.073255623266));
#198233=CARTESIAN_POINT('Ctrl Pts',(-14.1378586642913,52.0780515896709,
-216.117026001651));
#198234=CARTESIAN_POINT('Ctrl Pts',(-14.3424130345253,52.0646512413527,
-216.157742953632));
#198235=CARTESIAN_POINT('Ctrl Pts',(-15.1606305154611,52.0110498480797,
-216.320610761555));
#198236=CARTESIAN_POINT('Ctrl Pts',(-15.9800600230911,51.9495462915113,
-216.43465254041));
#198237=CARTESIAN_POINT('Ctrl Pts',(-16.7982755207299,51.8807308388097,
-216.502811102887));
#198238=CARTESIAN_POINT('Ctrl Pts',(-18.4347065160074,51.7430999334064,
-216.639128227839));
#198239=CARTESIAN_POINT('Ctrl Pts',(-20.0708066016568,51.5755528046511,
-216.593153495422));
#198240=CARTESIAN_POINT('Ctrl Pts',(-21.6997076367388,51.3826656205631,
-216.388192261383));
#198241=CARTESIAN_POINT('Ctrl Pts',(-22.1069328955093,51.3344438245411,
-216.336951952873));
#198242=CARTESIAN_POINT('Ctrl Pts',(-22.5139915785022,51.2846133848892,
-216.275725177028));
#198243=CARTESIAN_POINT('Ctrl Pts',(-22.9188870606657,51.2334349680578,
-216.205323293599));
#198244=CARTESIAN_POINT('Ctrl Pts',(-23.0201109312066,51.2206403638499,
-216.187722822743));
#198245=CARTESIAN_POINT('Ctrl Pts',(-23.121228131896,51.2077581272943,-216.169545425857));
#198246=CARTESIAN_POINT('Ctrl Pts',(-23.2222435222512,51.1947878519363,
-216.150798297381));
#198247=CARTESIAN_POINT('Ctrl Pts',(-23.2474973698401,51.1915452830968,
-216.146111515263));
#198248=CARTESIAN_POINT('Ctrl Pts',(-23.2727448539233,51.1882972112394,
-216.141389121832));
#198249=CARTESIAN_POINT('Ctrl Pts',(-23.2979860497664,51.1850436287764,
-216.136631223406));
#198250=CARTESIAN_POINT('Ctrl Pts',(-23.310606647688,51.1834168375448,-216.134252274193));
#198251=CARTESIAN_POINT('Ctrl Pts',(-23.3232256735435,51.1817886686391,
-216.131864448716));
#198252=CARTESIAN_POINT('Ctrl Pts',(-23.3358431367254,51.1801591210892,
-216.129467759999));
#198253=CARTESIAN_POINT('Ctrl Pts',(-23.3476897986568,51.1786291226539,
-216.127217485076));
#198254=CARTESIAN_POINT('Ctrl Pts',(-23.3616086485301,51.1763333384333,
-216.125238663377));
#198255=CARTESIAN_POINT('Ctrl Pts',(-23.3713060248739,51.1755923752032,
-216.122683482436));
#198256=CARTESIAN_POINT('',(-32.9259640526745,50.2082425591298,-216.288164109342));
#198257=CARTESIAN_POINT('Ctrl Pts',(-23.3713119210585,51.1755743233668,
-216.12270611168));
#198258=CARTESIAN_POINT('Ctrl Pts',(-23.3719383148078,51.1755440742727,
-216.122516863379));
#198259=CARTESIAN_POINT('Ctrl Pts',(-23.3725507139463,51.1755024990986,
-216.122348351235));
#198260=CARTESIAN_POINT('Ctrl Pts',(-23.4120030149939,51.1732152730112,
-216.110956616071));
#198261=CARTESIAN_POINT('Ctrl Pts',(-23.4508662604922,51.1709434402525,
-216.099856312516));
#198262=CARTESIAN_POINT('Ctrl Pts',(-23.6452008940486,51.1594893141098,
-216.044958572661));
#198263=CARTESIAN_POINT('Ctrl Pts',(-23.8007275067389,51.1500221617809,
-216.002972199005));
#198264=CARTESIAN_POINT('Ctrl Pts',(-24.5786228904514,51.1011607936348,
-215.802871305082));
#198265=CARTESIAN_POINT('Ctrl Pts',(-25.2017829090892,51.0571978530063,
-215.674165918587));
#198266=CARTESIAN_POINT('Ctrl Pts',(-26.4489130852517,50.9592383471587,
-215.485158151918));
#198267=CARTESIAN_POINT('Ctrl Pts',(-27.0728751382963,50.9052515915225,
-215.424810848009));
#198268=CARTESIAN_POINT('Ctrl Pts',(-28.0085823077969,50.8163361552934,
-215.391847556155));
#198269=CARTESIAN_POINT('Ctrl Pts',(-28.3204452554017,50.7853721850659,
-215.390477529248));
#198270=CARTESIAN_POINT('Ctrl Pts',(-28.9439290913914,50.7206839329619,
-215.408400357933));
#198271=CARTESIAN_POINT('Ctrl Pts',(-29.2565550883999,50.6868459785135,
-215.427797032548));
#198272=CARTESIAN_POINT('Ctrl Pts',(-30.7473218723846,50.518451120397,-215.57379855617));
#198273=CARTESIAN_POINT('Ctrl Pts',(-31.8718448202371,50.3704768331421,
-215.843735990856));
#198274=CARTESIAN_POINT('Ctrl Pts',(-32.9259571993476,50.2082406704928,
-216.288179546395));
#198275=CARTESIAN_POINT('',(-33.8288256170145,50.8425199003324,-213.842075049522));
#198276=CARTESIAN_POINT('Ctrl Pts',(-33.8288255478926,50.8425194315114,
-213.842075041245));
#198277=CARTESIAN_POINT('Ctrl Pts',(-33.7970774697237,50.8454126628531,
-213.943330969591));
#198278=CARTESIAN_POINT('Ctrl Pts',(-33.7646338917884,50.8450038051801,
-214.044775431056));
#198279=CARTESIAN_POINT('Ctrl Pts',(-33.7315935110065,50.8412526174688,
-214.146057915126));
#198280=CARTESIAN_POINT('Ctrl Pts',(-33.6986141665251,50.837508359418,-214.247153297596));
#198281=CARTESIAN_POINT('Ctrl Pts',(-33.6650404319365,50.8304340345761,
-214.348086736041));
#198282=CARTESIAN_POINT('Ctrl Pts',(-33.6309839083423,50.8200397985673,
-214.448509146524));
#198283=CARTESIAN_POINT('Ctrl Pts',(-33.5969409221117,50.8096496942354,
-214.548891639407));
#198284=CARTESIAN_POINT('Ctrl Pts',(-33.5624157675524,50.7959423557587,
-214.648762951211));
#198285=CARTESIAN_POINT('Ctrl Pts',(-33.5275300116972,50.7789783952727,
-214.747782348801));
#198286=CARTESIAN_POINT('Ctrl Pts',(-33.4925921263582,50.761989085687,-214.846949710222));
#198287=CARTESIAN_POINT('Ctrl Pts',(-33.4572928164849,50.7417335604387,
-214.945262074432));
#198288=CARTESIAN_POINT('Ctrl Pts',(-33.4217606234739,50.718321968533,-215.0423933864));
#198289=CARTESIAN_POINT('Ctrl Pts',(-33.4122602220973,50.712062306488,-215.068363819737));
#198290=CARTESIAN_POINT('Ctrl Pts',(-33.4027431956259,50.7055772843654,
-215.094249934778));
#198291=CARTESIAN_POINT('Ctrl Pts',(-33.3932120420313,50.6988695765327,
-215.120045768538));
#198292=CARTESIAN_POINT('Ctrl Pts',(-33.355198383497,50.672116832222,-215.222928804308));
#198293=CARTESIAN_POINT('Ctrl Pts',(-33.3169504134669,50.6418178055739,
-215.324410349766));
#198294=CARTESIAN_POINT('Ctrl Pts',(-33.2784700659473,50.6080102934018,
-215.424514371539));
#198295=CARTESIAN_POINT('Ctrl Pts',(-33.2404166725892,50.5745778884971,
-215.523507700935));
#198296=CARTESIAN_POINT('Ctrl Pts',(-33.2021355491518,50.5377139435189,
-215.621154855899));
#198297=CARTESIAN_POINT('Ctrl Pts',(-33.1636281482726,50.4974055580181,
-215.717462013326));
#198298=CARTESIAN_POINT('Ctrl Pts',(-33.1244726752926,50.4564187901941,
-215.815390001565));
#198299=CARTESIAN_POINT('Ctrl Pts',(-33.0850827260538,50.4118701743681,
-215.911933509871));
#198300=CARTESIAN_POINT('Ctrl Pts',(-33.0454669545182,50.3637017224098,
-216.00706645164));
#198301=CARTESIAN_POINT('Ctrl Pts',(-33.0058511829825,50.3155332704514,
-216.102199393409));
#198302=CARTESIAN_POINT('Ctrl Pts',(-32.9660090942418,50.2637441385916,
-216.195922559663));
#198303=CARTESIAN_POINT('Ctrl Pts',(-32.9259640526745,50.2082425591299,
-216.288164109342));
#198304=CARTESIAN_POINT('Ctrl Pts',(-33.8288255478898,50.8425194315119,
-213.842075041244));
#198305=CARTESIAN_POINT('Ctrl Pts',(-33.4284854297646,50.9043645560048,
-213.682497556561));
#198306=CARTESIAN_POINT('Ctrl Pts',(-33.0234151328446,50.9655031281662,
-213.541601729915));
#198307=CARTESIAN_POINT('Ctrl Pts',(-32.613891113486,51.0258461323052,-213.41828489294));
#198308=CARTESIAN_POINT('Ctrl Pts',(-32.3314320696816,51.0674662240305,
-213.33323016059));
#198309=CARTESIAN_POINT('Ctrl Pts',(-32.0468532024027,51.1087080491179,
-213.256538361901));
#198310=CARTESIAN_POINT('Ctrl Pts',(-31.760231540292,51.1495445945208,-213.187851585035));
#198311=CARTESIAN_POINT('Ctrl Pts',(-31.4098748863998,51.1994618104719,
-213.10389118535));
#198312=CARTESIAN_POINT('Ctrl Pts',(-31.0565047381091,51.2487669119008,
-213.031971638878));
#198313=CARTESIAN_POINT('Ctrl Pts',(-30.7001071876422,51.2974288982541,
-212.971577846918));
#198314=CARTESIAN_POINT('Ctrl Pts',(-30.4677048549224,51.3291607637747,
-212.932195819418));
#198315=CARTESIAN_POINT('Ctrl Pts',(-30.2340152995371,51.3606190826065,
-212.89771588442));
#198316=CARTESIAN_POINT('Ctrl Pts',(-29.9990356615488,51.3917943388598,
-212.868006986083));
#198317=CARTESIAN_POINT('Ctrl Pts',(-29.8721559396975,51.4086277456857,
-212.851965354604));
#198318=CARTESIAN_POINT('Ctrl Pts',(-29.7450788398495,51.4253538896652,
-212.837366281476));
#198319=CARTESIAN_POINT('Ctrl Pts',(-29.617962992439,51.4419530974049,-212.824189892615));
#198320=CARTESIAN_POINT('Ctrl Pts',(-29.3784059473116,51.4732352485967,
-212.799358238301));
#198321=CARTESIAN_POINT('Ctrl Pts',(-29.1386589564598,51.5040741022661,
-212.779534675774));
#198322=CARTESIAN_POINT('Ctrl Pts',(-28.899813341109,51.5343335838556,-212.764578265057));
#198323=CARTESIAN_POINT('Ctrl Pts',(-28.5341328390394,51.5806618465861,
-212.741679507747));
#198324=CARTESIAN_POINT('Ctrl Pts',(-28.1693740006546,51.6257909648441,
-212.730032265418));
#198325=CARTESIAN_POINT('Ctrl Pts',(-27.8054230251461,51.6697639760348,
-212.728805896948));
#198326=CARTESIAN_POINT('Ctrl Pts',(-27.2316173838903,51.7390918899084,
-212.72687240262));
#198327=CARTESIAN_POINT('Ctrl Pts',(-26.659813477437,51.8055490574399,-212.750767886994));
#198328=CARTESIAN_POINT('Ctrl Pts',(-26.0896437383804,51.8692665746801,
-212.798150758929));
#198329=CARTESIAN_POINT('Ctrl Pts',(-25.9366321166225,51.8863659048961,
-212.810866498789));
#198330=CARTESIAN_POINT('Ctrl Pts',(-25.783738207763,51.9032678957084,-212.825274044136));
#198331=CARTESIAN_POINT('Ctrl Pts',(-25.6309549565992,51.919975004434,-212.841328746581));
#198332=CARTESIAN_POINT('Ctrl Pts',(-25.5252626824023,51.9315326346259,
-212.852435055682));
#198333=CARTESIAN_POINT('Ctrl Pts',(-25.4196234520871,51.9429969636603,
-212.864330645339));
#198334=CARTESIAN_POINT('Ctrl Pts',(-25.3140353742909,51.954368608782,-212.877005898427));
#198335=CARTESIAN_POINT('Ctrl Pts',(-24.6986753884515,52.0206417669556,
-212.950876393311));
#198336=CARTESIAN_POINT('Ctrl Pts',(-24.0852465518143,52.0837464971762,
-213.051177399378));
#198337=CARTESIAN_POINT('Ctrl Pts',(-23.4735918363939,52.1437861556343,
-213.175966145474));
#198338=CARTESIAN_POINT('Ctrl Pts',(-23.3778558249174,52.1531835448578,
-213.195498042355));
#198339=CARTESIAN_POINT('Ctrl Pts',(-23.2821634538011,52.1625057785251,
-213.215631611061));
#198340=CARTESIAN_POINT('Ctrl Pts',(-23.186514300368,52.1717531873608,-213.236361158368));
#198341=CARTESIAN_POINT('Ctrl Pts',(-23.1032160300045,52.1798065065351,
-213.254413962539));
#198342=CARTESIAN_POINT('Ctrl Pts',(-23.0199493662676,52.1878031958512,
-213.27291866346));
#198343=CARTESIAN_POINT('Ctrl Pts',(-22.9367159200589,52.1957432933471,
-213.291870988623));
#198344=CARTESIAN_POINT('Ctrl Pts',(-22.8920159948608,52.2000074657478,
-213.302049198894));
#198345=CARTESIAN_POINT('Ctrl Pts',(-22.8473256517326,52.2042553156825,
-213.31235652924));
#198346=CARTESIAN_POINT('Ctrl Pts',(-22.8026451428253,52.2084868488979,
-213.322792347151));
#198347=CARTESIAN_POINT('Ctrl Pts',(-22.7914750218732,52.2095447316075,
-213.325401300163));
#198348=CARTESIAN_POINT('Ctrl Pts',(-22.7803044160517,52.2106019242221,
-213.328005681871));
#198349=CARTESIAN_POINT('Ctrl Pts',(-22.7691328173551,52.2116585796836,
-213.330599615203));
#198350=CARTESIAN_POINT('Ctrl Pts',(-22.7579612024765,52.2127152366757,
-213.333193552293));
#198351=CARTESIAN_POINT('Ctrl Pts',(-22.7467887595382,52.2137713070932,
-213.335778930067));
#198352=CARTESIAN_POINT('Ctrl Pts',(-22.7356154921234,52.2148267904768,
-213.338355735395));
#198353=CARTESIAN_POINT('Ctrl Pts',(-22.7132688713499,52.2169377653627,
-213.34350936587));
#198354=CARTESIAN_POINT('Ctrl Pts',(-22.690918952669,52.2190463920883,-213.348628706464));
#198355=CARTESIAN_POINT('Ctrl Pts',(-22.6685657646952,52.2211526670292,
-213.353713651063));
#198356=CARTESIAN_POINT('Ctrl Pts',(-22.6646488913256,52.2215217424486,
-213.354604668671));
#198357=CARTESIAN_POINT('Ctrl Pts',(-22.6607319175818,52.2218907456563,
-213.355494630255));
#198358=CARTESIAN_POINT('Ctrl Pts',(-22.6568148436157,52.2222596766335,
-213.356383535216));
#198359=CARTESIAN_POINT('Ctrl Pts',(-22.5713095630331,52.230313021297,-213.375787322021));
#198360=CARTESIAN_POINT('Ctrl Pts',(-22.4857590592482,52.2383317076775,
-213.394687120908));
#198361=CARTESIAN_POINT('Ctrl Pts',(-22.4001649179091,52.2463155472972,
-213.413077019702));
#198362=CARTESIAN_POINT('Ctrl Pts',(-22.3089921278341,52.2548197383815,
-213.432665491016));
#198363=CARTESIAN_POINT('Ctrl Pts',(-22.2177437865543,52.2632866458112,
-213.451679464809));
#198364=CARTESIAN_POINT('Ctrl Pts',(-22.1264553921399,52.2717131158806,
-213.470105691494));
#198365=CARTESIAN_POINT('Ctrl Pts',(-21.8592067817176,52.2963817764619,
-213.524048840657));
#198366=CARTESIAN_POINT('Ctrl Pts',(-21.5914443579229,52.3207197108699,
-213.572977568728));
#198367=CARTESIAN_POINT('Ctrl Pts',(-21.324095772452,52.3446435619462,-213.616545275384));
#198368=CARTESIAN_POINT('Ctrl Pts',(-21.2373298036558,52.3524078675337,
-213.630684846273));
#198369=CARTESIAN_POINT('Ctrl Pts',(-21.1505925461958,52.3601300382446,
-213.64426337592));
#198370=CARTESIAN_POINT('Ctrl Pts',(-21.0638877077023,52.367809951321,-213.657275547301));
#198371=CARTESIAN_POINT('Ctrl Pts',(-19.9403620371655,52.4673266523355,
-213.825887920386));
#198372=CARTESIAN_POINT('Ctrl Pts',(-18.8212977891659,52.5598365227201,
-213.899469703825));
#198373=CARTESIAN_POINT('Ctrl Pts',(-17.7073210864199,52.6457202413902,
-213.86667189224));
#198374=CARTESIAN_POINT('Ctrl Pts',(-17.4861825445344,52.6627692517255,
-213.860161109552));
#198375=CARTESIAN_POINT('Ctrl Pts',(-17.26524445948,52.6795571452203,-213.849458033042));
#198376=CARTESIAN_POINT('Ctrl Pts',(-17.0445116841459,52.6960869022231,
-213.834473635959));
#198377=CARTESIAN_POINT('Ctrl Pts',(-16.9763221692116,52.7011933306195,
-213.829844605372));
#198378=CARTESIAN_POINT('Ctrl Pts',(-16.9081523016014,52.7062751479287,
-213.824806041867));
#198379=CARTESIAN_POINT('Ctrl Pts',(-16.8400022396715,52.7113324526888,
-213.819355050391));
#198380=CARTESIAN_POINT('Ctrl Pts',(-16.1996233055735,52.7588539272107,
-213.768134258918));
#198381=CARTESIAN_POINT('Ctrl Pts',(-15.5609952942025,52.8042113945112,
-213.680469263933));
#198382=CARTESIAN_POINT('Ctrl Pts',(-14.9242487810738,52.8474860509722,
-213.553990748348));
#198383=CARTESIAN_POINT('Ctrl Pts',(-14.8649438022494,52.8515165443194,
-213.542210855512));
#198384=CARTESIAN_POINT('Ctrl Pts',(-14.8056550939682,52.8555289645465,
-213.53009494545));
#198385=CARTESIAN_POINT('Ctrl Pts',(-14.7463827693234,52.8595233836131,
-213.517640823917));
#198386=CARTESIAN_POINT('Ctrl Pts',(-14.6296583420251,52.8673895552326,
-213.493115040389));
#198387=CARTESIAN_POINT('Ctrl Pts',(-14.5129975854062,52.8751859177496,
-213.467277078931));
#198388=CARTESIAN_POINT('Ctrl Pts',(-14.3964014059856,52.8829130229972,
-213.440109913242));
#198389=CARTESIAN_POINT('Ctrl Pts',(-14.3392716131932,52.8866991498144,
-213.426798546143));
#198390=CARTESIAN_POINT('Ctrl Pts',(-14.2821573282444,52.8904686504834,
-213.413167990812));
#198391=CARTESIAN_POINT('Ctrl Pts',(-14.2250586750741,52.8942215948614,
-213.399215938864));
#198392=CARTESIAN_POINT('Ctrl Pts',(-14.1943088494084,52.8962427000705,
-213.391702221092));
#198393=CARTESIAN_POINT('Ctrl Pts',(-14.1635634419837,52.8982590111405,
-213.384095232765));
#198394=CARTESIAN_POINT('Ctrl Pts',(-14.1328225823483,52.9002705316721,
-213.376394641147));
#198395=CARTESIAN_POINT('Ctrl Pts',(-14.0889125166663,52.9031437759375,
-213.365395160724));
#198396=CARTESIAN_POINT('Ctrl Pts',(-14.0450117306304,52.9060072461915,
-213.354204687972));
#198397=CARTESIAN_POINT('Ctrl Pts',(-14.0011206054635,52.9088609546764,
-213.342822186058));
#198398=CARTESIAN_POINT('Ctrl Pts',(-13.97917518517,52.9102877996674,-213.337130972003));
#198399=CARTESIAN_POINT('Ctrl Pts',(-13.9572335774899,52.9117125570173,
-213.331366770807));
#198400=CARTESIAN_POINT('Ctrl Pts',(-13.9352910762425,52.9131340283109,
-213.325614433985));
#198401=CARTESIAN_POINT('Ctrl Pts',(-13.9133485638327,52.9145555003276,
-213.319862094238));
#198402=CARTESIAN_POINT('Ctrl Pts',(-13.8914033905366,52.9159732398363,
-213.314153208263));
#198403=CARTESIAN_POINT('Ctrl Pts',(-13.8694556009261,52.9173872435139,
-213.308487695886));
#198404=CARTESIAN_POINT('Ctrl Pts',(-13.814453489134,52.9209307980009,-213.294289676376));
#198405=CARTESIAN_POINT('Ctrl Pts',(-13.759434949972,52.9244508908472,-213.280363986675));
#198406=CARTESIAN_POINT('Ctrl Pts',(-13.7044006823105,52.9279474706966,
-213.266709421035));
#198407=CARTESIAN_POINT('Ctrl Pts',(-13.4080399531724,52.9467766292867,
-213.193179287882));
#198408=CARTESIAN_POINT('Ctrl Pts',(-13.1112381993239,52.9649231366514,
-213.127512319229));
#198409=CARTESIAN_POINT('Ctrl Pts',(-12.8139330465278,52.9823892815607,
-213.069496767474));
#198410=CARTESIAN_POINT('Ctrl Pts',(-12.762879858688,52.985388564851,-213.059534347269));
#198411=CARTESIAN_POINT('Ctrl Pts',(-12.7118203984012,52.9883673151379,
-213.049796876756));
#198412=CARTESIAN_POINT('Ctrl Pts',(-12.6607543476392,52.9913255531846,
-213.040283642668));
#198413=CARTESIAN_POINT('Ctrl Pts',(-11.9341248848113,53.0334189379416,
-212.904917855179));
#198414=CARTESIAN_POINT('Ctrl Pts',(-11.2065831243644,53.0713381842672,
-212.814853635294));
#198415=CARTESIAN_POINT('Ctrl Pts',(-10.4781602304721,53.1051020165539,
-212.767914849581));
#198416=CARTESIAN_POINT('Ctrl Pts',(-9.84364980408828,53.1345128214588,
-212.727027681994));
#198417=CARTESIAN_POINT('Ctrl Pts',(-9.20847120771161,53.1607704847659,
-212.718863838119));
#198418=CARTESIAN_POINT('Ctrl Pts',(-8.57265926894805,53.1838840251076,
-212.742013573981));
#198419=CARTESIAN_POINT('Ctrl Pts',(-8.53829774072196,53.1851331626599,
-212.743264667667));
#198420=CARTESIAN_POINT('Ctrl Pts',(-8.50393420974279,53.186373110042,-212.744608085481));
#198421=CARTESIAN_POINT('Ctrl Pts',(-8.46956866922752,53.1876038661027,
-212.746043776936));
#198422=CARTESIAN_POINT('Ctrl Pts',(-8.05134105999317,53.2025821308736,
-212.76351609939));
#198423=CARTESIAN_POINT('Ctrl Pts',(-7.63294373530001,53.2161951626093,
-212.794632608455));
#198424=CARTESIAN_POINT('Ctrl Pts',(-7.21417793555685,53.2284476001672,
-212.839302228768));
#198425=CARTESIAN_POINT('Ctrl Pts',(-6.95775348626208,53.2359501816941,
-212.866654946674));
#198426=CARTESIAN_POINT('Ctrl Pts',(-6.70119085797075,53.2429425029054,
-212.899090463671));
#198427=CARTESIAN_POINT('Ctrl Pts',(-6.44444424425753,53.2494246606916,
-212.936597453296));
#198428=CARTESIAN_POINT('Ctrl Pts',(-6.41857408693467,53.2500778122144,
-212.940376711406));
#198429=CARTESIAN_POINT('Ctrl Pts',(-6.39270791173976,53.2507256250243,
-212.944206865458));
#198430=CARTESIAN_POINT('Ctrl Pts',(-6.36684597343844,53.2513681007524,
-212.948087807708));
#198431=CARTESIAN_POINT('Ctrl Pts',(-6.07745447347717,53.2585573149735,
-212.991515012816));
#198432=CARTESIAN_POINT('Ctrl Pts',(-5.78889206506211,53.2650712747836,
-213.041253050323));
#198433=CARTESIAN_POINT('Ctrl Pts',(-5.50128321713575,53.2709193635982,
-213.097172231798));
#198434=CARTESIAN_POINT('Ctrl Pts',(-5.46169210092698,53.2717243887757,
-213.104869848988));
#198435=CARTESIAN_POINT('Ctrl Pts',(-5.4221190644421,53.2725167877183,-213.112684673472));
#198436=CARTESIAN_POINT('Ctrl Pts',(-5.38256444434725,53.2732965767615,
-213.120616442334));
#198437=CARTESIAN_POINT('Ctrl Pts',(-5.36110255433366,53.273719681487,-213.124920130513));
#198438=CARTESIAN_POINT('Ctrl Pts',(-5.33964513566361,53.2741390978143,
-213.129258387298));
#198439=CARTESIAN_POINT('Ctrl Pts',(-5.31819206008382,53.2745548325864,
-213.133631201848));
#198440=CARTESIAN_POINT('Ctrl Pts',(-5.16346960690779,53.2775531674209,
-213.165168525801));
#198441=CARTESIAN_POINT('Ctrl Pts',(-5.00900884762652,53.2803593125378,
-213.198496059744));
#198442=CARTESIAN_POINT('Ctrl Pts',(-4.85480750872648,53.2829751753132,
-213.233598239231));
#198443=CARTESIAN_POINT('Ctrl Pts',(-4.83548667519202,53.2833029328385,
-213.237996407052));
#198444=CARTESIAN_POINT('Ctrl Pts',(-4.81616991445761,53.2836277030469,
-213.242422436056));
#198445=CARTESIAN_POINT('Ctrl Pts',(-4.79685722222938,53.2839494896215,
-213.246876296773));
#198446=CARTESIAN_POINT('Ctrl Pts',(-4.7284277801666,53.2850896556584,-213.262657380025));
#198447=CARTESIAN_POINT('Ctrl Pts',(-4.66004791849701,53.2861923861427,
-213.278788317341));
#198448=CARTESIAN_POINT('Ctrl Pts',(-4.59171994251615,53.287257805251,-213.295267139756));
#198449=CARTESIAN_POINT('Ctrl Pts',(-4.56981793503112,53.2875993171567,
-213.300549299614));
#198450=CARTESIAN_POINT('Ctrl Pts',(-4.5479212585868,53.2879369954791,-213.305867203351));
#198451=CARTESIAN_POINT('Ctrl Pts',(-4.52602998880579,53.2882708445055,
-213.311220784633));
#198452=CARTESIAN_POINT('Ctrl Pts',(-4.51508439514851,53.2884377683898,
-213.313897565189));
#198453=CARTESIAN_POINT('Ctrl Pts',(-4.50414015314487,53.2886037349588,
-213.316583265059));
#198454=CARTESIAN_POINT('Ctrl Pts',(-4.49319727224013,53.2887687447573,
-213.319277875872));
#198455=CARTESIAN_POINT('Ctrl Pts',(-4.48225439119486,53.288933754558,-213.32197248672));
#198456=CARTESIAN_POINT('Ctrl Pts',(-4.47131360771902,53.2890977098182,
-213.324680797965));
#198457=CARTESIAN_POINT('Ctrl Pts',(-4.46037245702204,53.2892609395381,
-213.327386711908));
#198458=CARTESIAN_POINT('Ctrl Pts',(-4.41660743855001,53.2899138646194,
-213.338210470483));
#198459=CARTESIAN_POINT('Ctrl Pts',(-4.37281891468896,53.2905575212915,
-213.348881124148));
#198460=CARTESIAN_POINT('Ctrl Pts',(-4.32900749630775,53.2911918673437,
-213.359398181113));
#198461=CARTESIAN_POINT('Ctrl Pts',(-4.31174898704184,53.2914417535064,
-213.36354113589));
#198462=CARTESIAN_POINT('Ctrl Pts',(-4.29448693048956,53.2916901975378,
-213.367660294877));
#198463=CARTESIAN_POINT('Ctrl Pts',(-4.27722136169741,53.2919371969757,
-213.371755612804));
#198464=CARTESIAN_POINT('Ctrl Pts',(-3.34936233527052,53.305211052053,-213.591839743871));
#198465=CARTESIAN_POINT('Ctrl Pts',(-2.41131193880081,53.3143129931199,
-213.743095767743));
#198466=CARTESIAN_POINT('Ctrl Pts',(-1.46228217018108,53.3189491272515,
-213.820197476167));
#198467=CARTESIAN_POINT('Ctrl Pts',(-0.993352427707391,53.3212399101714,
-213.858294578566));
#198468=CARTESIAN_POINT('Ctrl Pts',(-0.521742197160567,53.3224404125564,
-213.878287712818));
#198469=CARTESIAN_POINT('Ctrl Pts',(-0.0473571427401393,53.3225154460666,
-213.879539002147));
#198470=CARTESIAN_POINT('Ctrl Pts',(-0.0544835933803345,52.4792219709059,
-216.57221503382));
#198471=CARTESIAN_POINT('Ctrl Pts',(-0.911160817479643,52.4788868661666,
-216.570205286074));
#198472=CARTESIAN_POINT('Ctrl Pts',(-1.76241895715707,52.4706614931604,
-216.520914925994));
#198473=CARTESIAN_POINT('Ctrl Pts',(-3.03147279341818,52.4469055640949,
-216.37863656052));
#198474=CARTESIAN_POINT('Ctrl Pts',(-3.45317987983679,52.437124954073,-216.319765648019));
#198475=CARTESIAN_POINT('Ctrl Pts',(-4.08382026129649,52.4196309296523,
-216.214709957797));
#198476=CARTESIAN_POINT('Ctrl Pts',(-4.29371035972386,52.4133485556671,
-216.176866822026));
#198477=CARTESIAN_POINT('Ctrl Pts',(-4.71285393159547,52.3998755739423,
-216.095622991724));
#198478=CARTESIAN_POINT('Ctrl Pts',(-4.92331707557612,52.3926407185815,
-216.051954867598));
#198479=CARTESIAN_POINT('Ctrl Pts',(-5.13104565674618,52.3850329666526,
-216.006074884366));
#198480=CARTESIAN_POINT('Ctrl Pts',(-33.4754093737626,49.9711874412034,
-216.637340091396));
#198481=CARTESIAN_POINT('Ctrl Pts',(-33.1531183251102,50.0508442845748,
-216.592238632432));
#198482=CARTESIAN_POINT('Ctrl Pts',(-32.8299704770403,50.0687939509079,
-216.505612191758));
#198483=CARTESIAN_POINT('Ctrl Pts',(-33.5583226571475,50.2807044023955,
-216.184599119136));
#198484=CARTESIAN_POINT('Ctrl Pts',(-33.2915590096021,50.3430190640451,
-216.141689042293));
#198485=CARTESIAN_POINT('Ctrl Pts',(-33.0227471817627,50.3616651708532,
-216.076225280147));
#198486=CARTESIAN_POINT('Ctrl Pts',(-33.6313141818038,50.506914657348,-215.69830350431));
#198487=CARTESIAN_POINT('Ctrl Pts',(-33.4219976724055,50.5521550190162,
-215.66141909055));
#198488=CARTESIAN_POINT('Ctrl Pts',(-33.2107462999537,50.5704649897337,
-215.613887593034));
#198489=CARTESIAN_POINT('Ctrl Pts',(-33.7472696093515,50.7753900150999,
-214.748451183307));
#198490=CARTESIAN_POINT('Ctrl Pts',(-33.6465861931775,50.793335292441,-214.728940081455));
#198491=CARTESIAN_POINT('Ctrl Pts',(-33.5452672954357,50.8058893973708,
-214.708515271655));
#198492=CARTESIAN_POINT('Ctrl Pts',(-33.7929819292232,50.8398470125736,
-214.293134446626));
#198493=CARTESIAN_POINT('Ctrl Pts',(-33.7432476178557,50.8473526001343,
-214.283376890363));
#198494=CARTESIAN_POINT('Ctrl Pts',(-33.6935058134431,50.8548585528471,
-214.273661258903));
#198495=CARTESIAN_POINT('Ctrl Pts',(-33.8288256585371,50.8425201819751,
-213.84207505449));
#198496=CARTESIAN_POINT('Ctrl Pts',(-33.8288256585371,50.8425201819751,
-213.84207505449));
#198497=CARTESIAN_POINT('Ctrl Pts',(-33.8288256585371,50.8425201819751,
-213.84207505449));
#198498=CARTESIAN_POINT('',(-33.5148860365099,50.1192982504879,-216.408010067648));
#198499=CARTESIAN_POINT('Ctrl Pts',(-33.828825603085,50.8425198058687,-213.84207504786));
#198500=CARTESIAN_POINT('Ctrl Pts',(-33.8198990676264,50.841864888462,-213.953795522105));
#198501=CARTESIAN_POINT('Ctrl Pts',(-33.8103998023479,50.8374948224705,
-214.066003151697));
#198502=CARTESIAN_POINT('Ctrl Pts',(-33.8003172610997,50.8293303724465,
-214.178318063006));
#198503=CARTESIAN_POINT('Ctrl Pts',(-33.7902347198515,50.8211659224224,
-214.290632974314));
#198504=CARTESIAN_POINT('Ctrl Pts',(-33.7795688729459,50.8092068754561,
-214.403054603578));
#198505=CARTESIAN_POINT('Ctrl Pts',(-33.7683167158641,50.7934249502469,
-214.515189821211));
#198506=CARTESIAN_POINT('Ctrl Pts',(-33.7570645587824,50.7776430250376,
-214.627325038844));
#198507=CARTESIAN_POINT('Ctrl Pts',(-33.7452260788453,50.7580381233537,
-214.739173241889));
#198508=CARTESIAN_POINT('Ctrl Pts',(-33.7328061316649,50.7346352575027,
-214.850336859306));
#198509=CARTESIAN_POINT('Ctrl Pts',(-33.7276482294165,50.7249162391657,
-214.896502198328));
#198510=CARTESIAN_POINT('Ctrl Pts',(-33.7223506794607,50.7144658367585,
-214.942895181462));
#198511=CARTESIAN_POINT('Ctrl Pts',(-33.7169619229803,50.7033744704336,
-214.989054517627));
#198512=CARTESIAN_POINT('Ctrl Pts',(-33.7115530693517,50.6922417393088,
-215.035386003159));
#198513=CARTESIAN_POINT('Ctrl Pts',(-33.7060523392326,50.6804633260605,
-215.081481730492));
#198514=CARTESIAN_POINT('Ctrl Pts',(-33.7005161572489,50.6681815307265,
-215.126887248828));
#198515=CARTESIAN_POINT('Ctrl Pts',(-33.6982866588628,50.6632354789248,
-215.145172689976));
#198516=CARTESIAN_POINT('Ctrl Pts',(-33.6960514937747,50.6582083562969,
-215.16334636011));
#198517=CARTESIAN_POINT('Ctrl Pts',(-33.6938146735602,50.6531116925866,
-215.181379319307));
#198518=CARTESIAN_POINT('Ctrl Pts',(-33.6804897647656,50.622750477744,-215.288803034027));
#198519=CARTESIAN_POINT('Ctrl Pts',(-33.6667462391996,50.5887152013327,
-215.395417267767));
#198520=CARTESIAN_POINT('Ctrl Pts',(-33.6525966745785,50.5510853335532,
-215.5008453749));
#198521=CARTESIAN_POINT('Ctrl Pts',(-33.63847268782,50.5135234884733,-215.606082901919));
#198522=CARTESIAN_POINT('Ctrl Pts',(-33.6239441491839,50.4723801664616,
-215.710138014617));
#198523=CARTESIAN_POINT('Ctrl Pts',(-33.6090308027503,50.4277843910374,
-215.812648418761));
#198524=CARTESIAN_POINT('Ctrl Pts',(-33.5940769452841,50.3830674743979,
-215.915437285043));
#198525=CARTESIAN_POINT('Ctrl Pts',(-33.5787362184851,50.3348795312152,
-216.01667248325));
#198526=CARTESIAN_POINT('Ctrl Pts',(-33.5630354218095,50.2833984427878,
-216.11600966241));
#198527=CARTESIAN_POINT('Ctrl Pts',(-33.5473346251338,50.2319173543604,
-216.21534684157));
#198528=CARTESIAN_POINT('Ctrl Pts',(-33.5312738087232,50.1771434563596,
-216.312785512755));
#198529=CARTESIAN_POINT('Ctrl Pts',(-33.5148860340387,50.1192982336582,
-216.408010056999));
#198530=CARTESIAN_POINT('Origin',(-33.1454591002416,47.6034469977721,-214.816150729402));
#198531=CARTESIAN_POINT('Ctrl Pts',(-42.5875626890161,49.379257463449,-213.836967828456));
#198532=CARTESIAN_POINT('Ctrl Pts',(-42.583706717545,49.3531444934432,-215.348104479787));
#198533=CARTESIAN_POINT('Ctrl Pts',(-42.4267736782988,48.5085693923201,
-216.591605848694));
#198534=CARTESIAN_POINT('Ctrl Pts',(-39.5843350108952,49.94028798542,-213.838955482324));
#198535=CARTESIAN_POINT('Ctrl Pts',(-39.5811128233999,49.9141052312931,
-215.348112574685));
#198536=CARTESIAN_POINT('Ctrl Pts',(-39.4353118162506,49.0695244128664,
-216.590608342324));
#198537=CARTESIAN_POINT('Ctrl Pts',(-36.5662930978432,50.4425286599318,
-213.840777098729));
#198538=CARTESIAN_POINT('Ctrl Pts',(-36.5632179392903,50.4163761409703,
-215.348234795315));
#198539=CARTESIAN_POINT('Ctrl Pts',(-36.4288305177724,49.5716582573572,
-216.589864155774));
#198540=CARTESIAN_POINT('Ctrl Pts',(-33.5455787101075,50.8841045229765,
-213.842210502424));
#198541=CARTESIAN_POINT('Ctrl Pts',(-33.542491458609,50.8579889698439,-215.348218150781));
#198542=CARTESIAN_POINT('Ctrl Pts',(-33.4195851394632,50.0130984955555,
-216.589106829638));
#198543=CARTESIAN_POINT('',(-33.4734406974179,50.0051916640197,-216.589120385861));
#198544=CARTESIAN_POINT('',(-42.426773677794,48.5085693922785,-216.591605848887));
#198545=CARTESIAN_POINT('Ctrl Pts',(-33.473440697418,50.0051916640197,-216.589120385862));
#198546=CARTESIAN_POINT('Ctrl Pts',(-36.464700907296,49.5656651085226,-216.589873039672));
#198547=CARTESIAN_POINT('Ctrl Pts',(-39.4531576785992,49.0661779829877,
-216.590614288892));
#198548=CARTESIAN_POINT('Ctrl Pts',(-42.4267736781731,48.508569392226,-216.591605848995));
#198549=CARTESIAN_POINT('',(-42.5875626890161,49.379257463449,-213.836967828456));
#198550=CARTESIAN_POINT('Origin',(-41.6694842675319,44.465041620637,-213.749705796269));
#198551=CARTESIAN_POINT('Origin',(-32.5100718388913,16.8405580785956,-213.686622269807));
#198552=CARTESIAN_POINT('Origin',(-31.3861213810748,49.6296476280943,-215.743606971984));
#198553=CARTESIAN_POINT('Ctrl Pts',(-33.4734406974176,50.0051916640201,
-216.589120385861));
#198554=CARTESIAN_POINT('Ctrl Pts',(-33.1846932575851,50.1143213461432,
-216.493132115846));
#198555=CARTESIAN_POINT('Ctrl Pts',(-32.8943360433596,50.1648136138274,
-216.360311415042));
#198556=CARTESIAN_POINT('Ctrl Pts',(-33.4901672823065,50.0432442151986,
-216.530872105694));
#198557=CARTESIAN_POINT('Ctrl Pts',(-33.1995861132119,50.1392297940238,
-216.451282693354));
#198558=CARTESIAN_POINT('Ctrl Pts',(-32.9074380702232,50.1790964451629,
-216.336991557182));
#198559=CARTESIAN_POINT('Ctrl Pts',(-33.5041153010602,50.0812800820291,
-216.470595425696));
#198560=CARTESIAN_POINT('Ctrl Pts',(-33.2118808797811,50.164531590063,-216.408280615884));
#198561=CARTESIAN_POINT('Ctrl Pts',(-32.9180956124776,50.1935640066322,
-216.312978006505));
#198562=CARTESIAN_POINT('Ctrl Pts',(-33.514886037746,50.119298258903,-216.408010072973));
#198563=CARTESIAN_POINT('Ctrl Pts',(-33.2211981697206,50.1902923385545,
-216.363964513645));
#198564=CARTESIAN_POINT('Ctrl Pts',(-32.9259571993478,50.2082406704929,
-216.288179546395));
#198565=CARTESIAN_POINT('',(-32.8943360433598,50.1648136138275,-216.360311415041));
#198566=CARTESIAN_POINT('Ctrl Pts',(-32.9259571993478,50.2082406704928,
-216.288179546395));
#198567=CARTESIAN_POINT('Ctrl Pts',(-32.9213942090144,50.1997220625587,
-216.302573035674));
#198568=CARTESIAN_POINT('Ctrl Pts',(-32.9158742467513,50.1912547814706,
-216.31673368404));
#198569=CARTESIAN_POINT('Ctrl Pts',(-32.9095161991152,50.1828980466778,
-216.330573580415));
#198570=CARTESIAN_POINT('Ctrl Pts',(-32.9048796509829,50.1768039742025,
-216.340666198364));
#198571=CARTESIAN_POINT('Ctrl Pts',(-32.8997987066695,50.1707685931225,
-216.350588603965));
#198572=CARTESIAN_POINT('Ctrl Pts',(-32.8943360433598,50.1648136138275,
-216.360311415041));
#198573=CARTESIAN_POINT('Origin',(-33.114566694526,47.5599010752717,-214.888601821826));
#198574=CARTESIAN_POINT('Ctrl Pts',(-43.4427334535925,49.2193110042462,
-213.753761106585));
#198575=CARTESIAN_POINT('Ctrl Pts',(-43.7363359520915,49.1333974713924,
-215.43762891935));
#198576=CARTESIAN_POINT('Ctrl Pts',(-43.7719279964167,48.0354975596101,
-216.750009718969));
#198577=CARTESIAN_POINT('Ctrl Pts',(-43.371956206762,49.2325823249756,-213.766498377489));
#198578=CARTESIAN_POINT('Ctrl Pts',(-43.6452593901831,49.1508522358615,
-215.438175221839));
#198579=CARTESIAN_POINT('Ctrl Pts',(-43.6692517245548,48.0727799897406,
-216.747093832485));
#198580=CARTESIAN_POINT('Ctrl Pts',(-43.3010795363893,49.2458600286701,
-213.778022394282));
#198581=CARTESIAN_POINT('Ctrl Pts',(-43.5493764245827,49.1692272064718,
-215.435455532993));
#198582=CARTESIAN_POINT('Ctrl Pts',(-43.5584791373048,48.11436895475,-216.739913980388));
#198583=CARTESIAN_POINT('Ctrl Pts',(-43.1590773754588,49.2724456764462,
-213.798159517644));
#198584=CARTESIAN_POINT('Ctrl Pts',(-43.3605441394919,49.205331988453,-215.428289388641));
#198585=CARTESIAN_POINT('Ctrl Pts',(-43.341150895191,48.1932191507075,-216.723471556235));
#198586=CARTESIAN_POINT('Ctrl Pts',(-43.0879593352488,49.2857509575935,
-213.806842606532));
#198587=CARTESIAN_POINT('Ctrl Pts',(-43.2666336864127,49.2232502933301,
-215.423678316261));
#198588=CARTESIAN_POINT('Ctrl Pts',(-43.2329905076982,48.2313985113306,
-216.713986670805));
#198589=CARTESIAN_POINT('Ctrl Pts',(-42.9454754545039,49.312391427417,-213.821265740755));
#198590=CARTESIAN_POINT('Ctrl Pts',(-43.0770958183574,49.2593635928723,
-215.410701334327));
#198591=CARTESIAN_POINT('Ctrl Pts',(-43.0131914262865,48.3080912144091,
-216.690257289732));
#198592=CARTESIAN_POINT('Ctrl Pts',(-42.8741106150187,49.3257262125301,
-213.827018288813));
#198593=CARTESIAN_POINT('Ctrl Pts',(-42.9810928107897,49.2776332485339,
-215.402139971414));
#198594=CARTESIAN_POINT('Ctrl Pts',(-42.9009270350625,48.3470115783392,
-216.675727916603));
#198595=CARTESIAN_POINT('Ctrl Pts',(-42.7310769616701,49.3524479316748,
-213.834879555374));
#198596=CARTESIAN_POINT('Ctrl Pts',(-42.7835366995418,49.3152096382395,
-215.378441131484));
#198597=CARTESIAN_POINT('Ctrl Pts',(-42.6662831546448,48.4283526107962,
-216.637893960711));
#198598=CARTESIAN_POINT('Ctrl Pts',(-42.6594046914523,49.3658367172642,
-213.836920285803));
#198599=CARTESIAN_POINT('Ctrl Pts',(-42.6823983172108,49.334434791349,-215.36340665766));
#198600=CARTESIAN_POINT('Ctrl Pts',(-42.5445646683703,48.470275506698,-216.614703255093));
#198601=CARTESIAN_POINT('Ctrl Pts',(-42.587562688342,49.3792574635749,-213.836967828456));
#198602=CARTESIAN_POINT('Ctrl Pts',(-42.5837067171795,49.3531444935084,
-215.348104479964));
#198603=CARTESIAN_POINT('Ctrl Pts',(-42.4267736781597,48.5085693921588,
-216.59160584896));
#198604=CARTESIAN_POINT('',(-43.4427334535923,49.2193110042465,-213.753761106585));
#198605=CARTESIAN_POINT('',(-43.7719279964152,48.0354975596111,-216.750009718968));
#198606=CARTESIAN_POINT('Origin',(-42.506225613034,44.3085739513886,-213.666499074398));
#198607=CARTESIAN_POINT('Ctrl Pts',(-43.4427334535923,49.2193110042462,
-213.753761106585));
#198608=CARTESIAN_POINT('Ctrl Pts',(-43.3719706400421,49.2325796186159,
-213.766495780036));
#198609=CARTESIAN_POINT('Ctrl Pts',(-43.3010945110548,49.2458572251129,
-213.778020270746));
#198610=CARTESIAN_POINT('Ctrl Pts',(-43.230078455924,49.2591528525582,-213.788090955963));
#198611=CARTESIAN_POINT('Ctrl Pts',(-43.1590933274853,49.2724426899074,
-213.79815725551));
#198612=CARTESIAN_POINT('Ctrl Pts',(-43.0879758381621,49.2857478720138,
-213.806840936001));
#198613=CARTESIAN_POINT('Ctrl Pts',(-43.0167173948763,49.2990711925053,
-213.814054173644));
#198614=CARTESIAN_POINT('Ctrl Pts',(-42.9454929340409,49.3123881592362,
-213.821263971364));
#198615=CARTESIAN_POINT('Ctrl Pts',(-42.874128659976,49.3257228413495,-213.827017297045));
#198616=CARTESIAN_POINT('Ctrl Pts',(-42.8025937883444,49.3390870721025,
-213.830948922093));
#198617=CARTESIAN_POINT('Ctrl Pts',(-42.7310959828176,49.3524443781212,
-213.834878509953));
#198618=CARTESIAN_POINT('Ctrl Pts',(-42.6594242987725,49.3658330544366,
-213.836920272815));
#198619=CARTESIAN_POINT('Ctrl Pts',(-42.5875626890161,49.379257463449,-213.836967828456));
#198620=CARTESIAN_POINT('Ctrl Pts',(-42.4267736781616,48.5085693921643,
-216.591605848952));
#198621=CARTESIAN_POINT('Ctrl Pts',(-42.4415254954543,48.503773861373,-216.594498092432));
#198622=CARTESIAN_POINT('Ctrl Pts',(-42.4593143860255,48.4979659020317,
-216.597960778204));
#198623=CARTESIAN_POINT('Ctrl Pts',(-42.480186767919,48.491088268847,-216.601973535425));
#198624=CARTESIAN_POINT('Ctrl Pts',(-42.4967271814369,48.4856380572956,
-216.60515346305));
#198625=CARTESIAN_POINT('Ctrl Pts',(-42.5152045567958,48.4795155730946,
-216.608678838495));
#198626=CARTESIAN_POINT('Ctrl Pts',(-42.5356174624875,48.4727022574992,
-216.612519977972));
#198627=CARTESIAN_POINT('Ctrl Pts',(-42.5515113833177,48.4673972656328,
-216.615510770546));
#198628=CARTESIAN_POINT('Ctrl Pts',(-42.5685785070712,48.461673503796,-216.618692765583));
#198629=CARTESIAN_POINT('Ctrl Pts',(-42.5868009760644,48.4555306364492,
-216.622040459405));
#198630=CARTESIAN_POINT('Ctrl Pts',(-42.6061677456185,48.4490020207962,
-216.625598375448));
#198631=CARTESIAN_POINT('Ctrl Pts',(-42.6262776792176,48.4421873747635,
-216.629237691355));
#198632=CARTESIAN_POINT('Ctrl Pts',(-42.645645819722,48.4355945626524,-216.632682797186));
#198633=CARTESIAN_POINT('Ctrl Pts',(-42.6618596565057,48.4300754587668,
-216.635566831594));
#198634=CARTESIAN_POINT('Ctrl Pts',(-42.6775524999369,48.4247129541951,
-216.638314861844));
#198635=CARTESIAN_POINT('Ctrl Pts',(-42.6918693280422,48.4198061888257,
-216.640789613044));
#198636=CARTESIAN_POINT('Ctrl Pts',(-42.715278653753,48.4117831778716,-216.644836058001));
#198637=CARTESIAN_POINT('Ctrl Pts',(-42.7364349552496,48.404496253462,-216.648396283454));
#198638=CARTESIAN_POINT('Ctrl Pts',(-42.7553494105702,48.3979643916984,
-216.651514294509));
#198639=CARTESIAN_POINT('Ctrl Pts',(-42.7618210576182,48.3957294923485,
-216.652581132897));
#198640=CARTESIAN_POINT('Ctrl Pts',(-42.7680306396195,48.3935827167038,
-216.653596337291));
#198641=CARTESIAN_POINT('Ctrl Pts',(-42.7739796041737,48.3915240995609,
-216.654561986672));
#198642=CARTESIAN_POINT('Ctrl Pts',(-42.7772862698949,48.3903798401393,
-216.65509873213));
#198643=CARTESIAN_POINT('Ctrl Pts',(-42.7805124230816,48.3892628125201,
-216.655620169018));
#198644=CARTESIAN_POINT('Ctrl Pts',(-42.7836583565613,48.3881729872862,
-216.656126663382));
#198645=CARTESIAN_POINT('Ctrl Pts',(-42.7916131605315,48.3854172563868,
-216.657407384481));
#198646=CARTESIAN_POINT('Ctrl Pts',(-42.7990521658508,48.3828376767049,
-216.658592151102));
#198647=CARTESIAN_POINT('Ctrl Pts',(-42.8059840566176,48.3804311709214,
-216.659688355632));
#198648=CARTESIAN_POINT('Ctrl Pts',(-42.8084023782922,48.3795916156987,
-216.660070787391));
#198649=CARTESIAN_POINT('Ctrl Pts',(-42.8095099314098,48.3792066589871,
-216.660245512224));
#198650=CARTESIAN_POINT('Ctrl Pts',(-42.8101772587533,48.3789746817772,
-216.660350971608));
#198651=CARTESIAN_POINT('Ctrl Pts',(-42.8108445860968,48.3787427045672,
-216.660456430992));
#198652=CARTESIAN_POINT('Ctrl Pts',(-42.8110716594233,48.3786635842834,
-216.660492534598));
#198653=CARTESIAN_POINT('Ctrl Pts',(-42.8117287721884,48.3784346229387,
-216.660596928192));
#198654=CARTESIAN_POINT('Ctrl Pts',(-42.8130429977186,48.3779767002494,
-216.660805715378));
#198655=CARTESIAN_POINT('Ctrl Pts',(-42.8151127707912,48.377255336016,-216.661134478143));
#198656=CARTESIAN_POINT('Ctrl Pts',(-42.8179347829778,48.3762716511989,
-216.661580299639));
#198657=CARTESIAN_POINT('Ctrl Pts',(-42.8239652219253,48.3741695868416,
-216.662532988406));
#198658=CARTESIAN_POINT('Ctrl Pts',(-42.8334335081744,48.3708687545685,
-216.664022789577));
#198659=CARTESIAN_POINT('Ctrl Pts',(-42.8462734480989,48.3663912789057,
-216.665990600897));
#198660=CARTESIAN_POINT('Ctrl Pts',(-42.8574678892586,48.3624876128337,
-216.667706227931));
#198661=CARTESIAN_POINT('Ctrl Pts',(-42.8712239810185,48.3576900086163,
-216.669784249758));
#198662=CARTESIAN_POINT('Ctrl Pts',(-42.8874753033194,48.3520199169081,
-216.672163514063));
#198663=CARTESIAN_POINT('Ctrl Pts',(-42.9049210367745,48.3459330947545,
-216.674717645359));
#198664=CARTESIAN_POINT('Ctrl Pts',(-42.9252414131555,48.338841234417,-216.677618487984));
#198665=CARTESIAN_POINT('Ctrl Pts',(-42.9483405988423,48.3307731838733,
-216.680772624931));
#198666=CARTESIAN_POINT('Ctrl Pts',(-42.9598901916857,48.3267391586014,
-216.682349693404));
#198667=CARTESIAN_POINT('Ctrl Pts',(-42.9721343606286,48.3224610817444,
-216.683989858753));
#198668=CARTESIAN_POINT('Ctrl Pts',(-42.9850612664934,48.3179421430536,
-216.685680657929));
#198669=CARTESIAN_POINT('Ctrl Pts',(-42.9896525342021,48.3163371451133,
-216.686281181499));
#198670=CARTESIAN_POINT('Ctrl Pts',(-42.995750004829,48.3142051330221,-216.687071085619));
#198671=CARTESIAN_POINT('Ctrl Pts',(-42.9995737114364,48.3128679604388,
-216.687562687561));
#198672=CARTESIAN_POINT('Ctrl Pts',(-43.0011329076028,48.3123227004124,
-216.687763148513));
#198673=CARTESIAN_POINT('Ctrl Pts',(-43.002314534652,48.3119094533396,-216.687914505546));
#198674=CARTESIAN_POINT('Ctrl Pts',(-43.0028633815164,48.3117175253772,
-216.68798476227));
#198675=CARTESIAN_POINT('Ctrl Pts',(-43.0047581971739,48.3110549214129,
-216.688227313606));
#198676=CARTESIAN_POINT('Ctrl Pts',(-43.0067444288693,48.3103606366143,
-216.688480302491));
#198677=CARTESIAN_POINT('Ctrl Pts',(-43.0088218770899,48.3096346619737,
-216.688743543246));
#198678=CARTESIAN_POINT('Ctrl Pts',(-43.0244229399528,48.3041827927562,
-216.690720408674));
#198679=CARTESIAN_POINT('Ctrl Pts',(-43.0451686616728,48.2969462008756,
-216.693276848829));
#198680=CARTESIAN_POINT('Ctrl Pts',(-43.0709184477644,48.2879624492166,
-216.696263099913));
#198681=CARTESIAN_POINT('Ctrl Pts',(-43.0725995349496,48.2873759406633,
-216.696458058753));
#198682=CARTESIAN_POINT('Ctrl Pts',(-43.0743019430858,48.2867819844123,
-216.696654834268));
#198683=CARTESIAN_POINT('Ctrl Pts',(-43.0760256312567,48.2861805899518,
-216.696853379208));
#198684=CARTESIAN_POINT('Ctrl Pts',(-43.0902687344933,48.2812111740613,
-216.698493986909));
#198685=CARTESIAN_POINT('Ctrl Pts',(-43.1059646008994,48.2757340625106,
-216.700255469844));
#198686=CARTESIAN_POINT('Ctrl Pts',(-43.1230914003588,48.2697535114062,
-216.702110542323));
#198687=CARTESIAN_POINT('Ctrl Pts',(-43.1397850747307,48.2639242043639,
-216.703918701284));
#198688=CARTESIAN_POINT('Ctrl Pts',(-43.157852453777,48.2576074670258,-216.705822337881));
#198689=CARTESIAN_POINT('Ctrl Pts',(-43.1772837610085,48.2507976758426,
-216.707797320349));
#198690=CARTESIAN_POINT('Ctrl Pts',(-43.1871254531832,48.247348609457,-216.70879762204));
#198691=CARTESIAN_POINT('Ctrl Pts',(-43.1965283228607,48.2440488814785,
-216.709734433479));
#198692=CARTESIAN_POINT('Ctrl Pts',(-43.2036246682312,48.2415563362908,
-216.710434118825));
#198693=CARTESIAN_POINT('Ctrl Pts',(-43.2816844673068,48.2141383392263,
-216.718130657632));
#198694=CARTESIAN_POINT('Ctrl Pts',(-43.3591363015399,48.1866286965368,
-216.724750583296));
#198695=CARTESIAN_POINT('Ctrl Pts',(-43.436799842652,48.1585111211586,-216.730701790525));
#198696=CARTESIAN_POINT('Ctrl Pts',(-43.441137525833,48.1569406914297,-216.731034178814));
#198697=CARTESIAN_POINT('Ctrl Pts',(-43.4454758694279,48.1553683652711,
-216.731364481053));
#198698=CARTESIAN_POINT('Ctrl Pts',(-43.4498150162479,48.1537940527302,
-216.73169276831));
#198699=CARTESIAN_POINT('Ctrl Pts',(-43.5584791373049,48.11436895475,-216.739913980388));
#198700=CARTESIAN_POINT('Ctrl Pts',(-43.6692517245548,48.0727799897407,
-216.747093832484));
#198701=CARTESIAN_POINT('Ctrl Pts',(-43.7719279964153,48.0354975596113,
-216.750009718968));
#198702=CARTESIAN_POINT('Ctrl Pts',(-47.5938143592254,47.5353276146289,
-213.404748058676));
#198703=CARTESIAN_POINT('Ctrl Pts',(-47.7151968771187,47.4137062867167,
-215.373807350724));
#198704=CARTESIAN_POINT('Ctrl Pts',(-47.0575921287075,46.1983743823902,
-216.787046295788));
#198705=CARTESIAN_POINT('Ctrl Pts',(-47.4361974911963,47.6395334582591,
-213.413799790385));
#198706=CARTESIAN_POINT('Ctrl Pts',(-47.5710170575155,47.5124761588416,
-215.378572627199));
#198707=CARTESIAN_POINT('Ctrl Pts',(-46.9439936233544,46.2838138436724,
-216.79016068369));
#198708=CARTESIAN_POINT('Ctrl Pts',(-47.2763792783413,47.7395307126687,
-213.423893656191));
#198709=CARTESIAN_POINT('Ctrl Pts',(-47.423589902594,47.6084784638584,-215.382114459135));
#198710=CARTESIAN_POINT('Ctrl Pts',(-46.8280682259696,46.3702652294506,
-216.791559853189));
#198711=CARTESIAN_POINT('Ctrl Pts',(-46.9524663169781,47.9311597954933,
-213.446422385042));
#198712=CARTESIAN_POINT('Ctrl Pts',(-47.1294827939091,47.7906783086273,
-215.393841476156));
#198713=CARTESIAN_POINT('Ctrl Pts',(-46.5987238205652,46.5304864276265,
-216.799043822533));
#198714=CARTESIAN_POINT('Ctrl Pts',(-46.7883227793929,48.0228296206103,
-213.458567219485));
#198715=CARTESIAN_POINT('Ctrl Pts',(-46.9655745538276,47.8868680864696,
-215.393218617728));
#198716=CARTESIAN_POINT('Ctrl Pts',(-46.4620613130109,46.632173235984,-216.795234897512));
#198717=CARTESIAN_POINT('Ctrl Pts',(-46.4554564499389,48.1980381642472,
-213.483257157288));
#198718=CARTESIAN_POINT('Ctrl Pts',(-46.645778329932,48.0640244167292,-215.396857720889));
#198719=CARTESIAN_POINT('Ctrl Pts',(-46.2017889155362,46.8105029195329,
-216.79265356856));
#198720=CARTESIAN_POINT('Ctrl Pts',(-46.2867982818254,48.281531361303,-213.496222696253));
#198721=CARTESIAN_POINT('Ctrl Pts',(-46.4887900152057,48.1462008970494,
-215.401226143536));
#198722=CARTESIAN_POINT('Ctrl Pts',(-46.0766746938607,46.8895727080125,
-216.794026584048));
#198723=CARTESIAN_POINT('Ctrl Pts',(-46.0305084677278,48.4005429744912,
-213.516940454077));
#198724=CARTESIAN_POINT('Ctrl Pts',(-46.2457844526878,48.2661209388548,
-215.406453553964));
#198725=CARTESIAN_POINT('Ctrl Pts',(-45.879944168228,47.0110043640158,-216.794144611354));
#198726=CARTESIAN_POINT('Ctrl Pts',(-45.9444636231603,48.4392026490648,
-213.524043422999));
#198727=CARTESIAN_POINT('Ctrl Pts',(-46.1636628855248,48.3054429426302,
-215.408017074389));
#198728=CARTESIAN_POINT('Ctrl Pts',(-45.8130123122325,47.051733779581,-216.79390894265));
#198729=CARTESIAN_POINT('Ctrl Pts',(-45.7716909901656,48.5142583186062,
-213.538427044995));
#198730=CARTESIAN_POINT('Ctrl Pts',(-45.9955375795966,48.3833424179063,
-215.409512738422));
#198731=CARTESIAN_POINT('Ctrl Pts',(-45.6738311416741,47.1362644708882,
-216.791413446998));
#198732=CARTESIAN_POINT('Ctrl Pts',(-45.6849221753783,48.5506755813429,
-213.545667919357));
#198733=CARTESIAN_POINT('Ctrl Pts',(-45.909485781788,48.4219041276403,-215.409378455852));
#198734=CARTESIAN_POINT('Ctrl Pts',(-45.6014976347732,47.180066238931,-216.789070533814));
#198735=CARTESIAN_POINT('Ctrl Pts',(-45.4234990388523,48.6566004797362,
-213.567641621074));
#198736=CARTESIAN_POINT('Ctrl Pts',(-45.6556174915683,48.5320412262081,
-215.411600281523));
#198737=CARTESIAN_POINT('Ctrl Pts',(-45.3906894073598,47.3016094353054,
-216.784909295631));
#198738=CARTESIAN_POINT('Ctrl Pts',(-45.2477531991542,48.7227706699221,
-213.582727977866));
#198739=CARTESIAN_POINT('Ctrl Pts',(-45.4876251235724,48.6001398788528,
-215.414556338723));
#198740=CARTESIAN_POINT('Ctrl Pts',(-45.2524231606292,47.3757390551069,
-216.783601115577));
#198741=CARTESIAN_POINT('Ctrl Pts',(-44.8934628219101,48.8462330088764,
-213.614222279575));
#198742=CARTESIAN_POINT('Ctrl Pts',(-45.1474114702805,48.7286790378217,
-215.42032956369));
#198743=CARTESIAN_POINT('Ctrl Pts',(-44.9704049771277,47.5202154420337,
-216.780178404985));
#198744=CARTESIAN_POINT('Ctrl Pts',(-44.7149101066689,48.9035307363901,
-213.630594481069));
#198745=CARTESIAN_POINT('Ctrl Pts',(-44.9742711452602,48.7893976468135,
-215.422593536637));
#198746=CARTESIAN_POINT('Ctrl Pts',(-44.8252363083432,47.5917545322963,
-216.777394875566));
#198747=CARTESIAN_POINT('Ctrl Pts',(-44.3548749878035,49.0092996064988,
-213.664137638318));
#198748=CARTESIAN_POINT('Ctrl Pts',(-44.622095897551,48.9031602696537,-215.425466313217));
#198749=CARTESIAN_POINT('Ctrl Pts',(-44.5266355180431,47.7322685705669,
-216.769090779705));
#198750=CARTESIAN_POINT('Ctrl Pts',(-44.1732412415974,49.0577948170664,
-213.681295718698));
#198751=CARTESIAN_POINT('Ctrl Pts',(-44.4434391165651,48.9560293640203,
-215.426301418401));
#198752=CARTESIAN_POINT('Ctrl Pts',(-44.3737734347551,47.8005712765384,
-216.763825997473));
#198753=CARTESIAN_POINT('Ctrl Pts',(-43.8089789068828,49.1454472082473,
-213.716585287098));
#198754=CARTESIAN_POINT('Ctrl Pts',(-44.0903037035521,49.0513958700251,
-215.431155804495));
#198755=CARTESIAN_POINT('Ctrl Pts',(-44.0737062319855,47.9238489048316,
-216.756518873734));
#198756=CARTESIAN_POINT('Ctrl Pts',(-43.6261771610655,49.1846631278254,
-213.734854145951));
#198757=CARTESIAN_POINT('Ctrl Pts',(-43.9151392929898,49.0942498031829,
-215.435089586124));
#198758=CARTESIAN_POINT('Ctrl Pts',(-43.9256354120413,47.9796853812831,
-216.75437483532));
#198759=CARTESIAN_POINT('Ctrl Pts',(-43.442733453593,49.219311004246,-213.753761106585));
#198760=CARTESIAN_POINT('Ctrl Pts',(-43.7363359520915,49.1333974713923,
-215.43762891935));
#198761=CARTESIAN_POINT('Ctrl Pts',(-43.7719279964163,48.0354975596104,
-216.750009718968));
#198762=CARTESIAN_POINT('',(-47.5938143592265,47.5353276146283,-213.404748058676));
#198763=CARTESIAN_POINT('',(-47.0575921287078,46.1983743823903,-216.787046295788));
#198764=CARTESIAN_POINT('Origin',(-44.8332438581234,43.3673981711062,-213.31748602649));
#198765=CARTESIAN_POINT('Ctrl Pts',(-47.5938143592265,47.5353276146283,
-213.404748058676));
#198766=CARTESIAN_POINT('Ctrl Pts',(-47.4361974915317,47.639533457943,-213.413799795273));
#198767=CARTESIAN_POINT('Ctrl Pts',(-47.2763792787077,47.7395307123426,
-213.423893661064));
#198768=CARTESIAN_POINT('Ctrl Pts',(-46.9524663174189,47.9311597951435,
-213.44642238989));
#198769=CARTESIAN_POINT('Ctrl Pts',(-46.7883227798346,48.0228296202715,
-213.458567224306));
#198770=CARTESIAN_POINT('Ctrl Pts',(-46.4554564504138,48.1980381639128,
-213.483257162063));
#198771=CARTESIAN_POINT('Ctrl Pts',(-46.2867982823297,48.2815313609651,
-213.496222701009));
#198772=CARTESIAN_POINT('Ctrl Pts',(-46.0305084682658,48.4005429741553,
-213.516940458798));
#198773=CARTESIAN_POINT('Ctrl Pts',(-45.9444636237083,48.4392026487304,
-213.524043427709));
#198774=CARTESIAN_POINT('Ctrl Pts',(-45.7716909907256,48.5142583182786,
-213.538427049676));
#198775=CARTESIAN_POINT('Ctrl Pts',(-45.6849221759404,48.5506755810206,
-213.545667924022));
#198776=CARTESIAN_POINT('Ctrl Pts',(-45.4234990394341,48.656600479424,-213.567641625695));
#198777=CARTESIAN_POINT('Ctrl Pts',(-45.2477531997558,48.7227706696145,
-213.58272798246));
#198778=CARTESIAN_POINT('Ctrl Pts',(-44.8934628225481,48.8462330085811,
-213.614222284111));
#198779=CARTESIAN_POINT('Ctrl Pts',(-44.7149101073209,48.9035307361032,
-213.630594485574));
#198780=CARTESIAN_POINT('Ctrl Pts',(-44.3548749884766,49.0092996062315,
-213.664137642754));
#198781=CARTESIAN_POINT('Ctrl Pts',(-44.1732412422787,49.0577948168098,
-213.681295723098));
#198782=CARTESIAN_POINT('Ctrl Pts',(-43.8089789075934,49.1454472080097,
-213.716585291428));
#198783=CARTESIAN_POINT('Ctrl Pts',(-43.626177161796,49.1846631275968,-213.734854150249));
#198784=CARTESIAN_POINT('Ctrl Pts',(-43.4427334535923,49.2193110042465,
-213.753761106585));
#198785=CARTESIAN_POINT('Ctrl Pts',(-43.7719279964163,48.0354975596108,
-216.750009718968));
#198786=CARTESIAN_POINT('Ctrl Pts',(-43.7811851272337,48.0321362342387,
-216.750272610989));
#198787=CARTESIAN_POINT('Ctrl Pts',(-43.7893021651862,48.0291829772161,
-216.750497126067));
#198788=CARTESIAN_POINT('Ctrl Pts',(-43.799178039926,48.0255804797839,-216.750762626771));
#198789=CARTESIAN_POINT('Ctrl Pts',(-43.8080192155758,48.0223554173551,
-216.751000310866));
#198790=CARTESIAN_POINT('Ctrl Pts',(-43.8182703799996,48.0186106696607,
-216.751270916601));
#198791=CARTESIAN_POINT('Ctrl Pts',(-43.831972963223,48.0135818234643,-216.751616944973));
#198792=CARTESIAN_POINT('Ctrl Pts',(-43.8335766018061,48.0129932883204,
-216.751657441312));
#198793=CARTESIAN_POINT('Ctrl Pts',(-43.835227458279,48.0123871498841,-216.751698951233));
#198794=CARTESIAN_POINT('Ctrl Pts',(-43.8369287587511,48.0117621670366,
-216.751741526661));
#198795=CARTESIAN_POINT('Ctrl Pts',(-43.8694055058916,47.9998316408073,
-216.752554264576));
#198796=CARTESIAN_POINT('Ctrl Pts',(-43.9008759562454,47.9881558224337,
-216.753270615293));
#198797=CARTESIAN_POINT('Ctrl Pts',(-43.9314332824726,47.976692143459,-216.753932760624));
#198798=CARTESIAN_POINT('Ctrl Pts',(-43.9686297051458,47.9627377861517,
-216.754738768236));
#198799=CARTESIAN_POINT('Ctrl Pts',(-44.0044739958948,47.9490971801564,
-216.755464878702));
#198800=CARTESIAN_POINT('Ctrl Pts',(-44.039093110119,47.9357219781021,-216.756167305868));
#198801=CARTESIAN_POINT('Ctrl Pts',(-44.0613540661284,47.9271213887681,
-216.756618984098));
#198802=CARTESIAN_POINT('Ctrl Pts',(-44.0831075367369,47.9186311582294,
-216.75706043696));
#198803=CARTESIAN_POINT('Ctrl Pts',(-44.1043786370355,47.9102443146154,
-216.757502456408));
#198804=CARTESIAN_POINT('Ctrl Pts',(-44.1397067224319,47.8963150338897,
-216.758236583959));
#198805=CARTESIAN_POINT('Ctrl Pts',(-44.1737062936049,47.8826695844048,
-216.758973260723));
#198806=CARTESIAN_POINT('Ctrl Pts',(-44.2064569138943,47.8692997410846,
-216.759744918243));
#198807=CARTESIAN_POINT('Ctrl Pts',(-44.2122572129562,47.8669318747974,
-216.759881582658));
#198808=CARTESIAN_POINT('Ctrl Pts',(-44.2180182348011,47.8645727207277,
-216.760019295337));
#198809=CARTESIAN_POINT('Ctrl Pts',(-44.2237402936187,47.8622223169866,
-216.760158175401));
#198810=CARTESIAN_POINT('Ctrl Pts',(-44.2579874141509,47.8481549047516,
-216.760989387112));
#198811=CARTESIAN_POINT('Ctrl Pts',(-44.2908804989542,47.8343590266573,
-216.761866207695));
#198812=CARTESIAN_POINT('Ctrl Pts',(-44.3223252327681,47.8209640907791,
-216.762743124348));
#198813=CARTESIAN_POINT('Ctrl Pts',(-44.3552906472565,47.8069213701161,
-216.763662449062));
#198814=CARTESIAN_POINT('Ctrl Pts',(-44.3866645471589,47.7933191305206,
-216.764582006858));
#198815=CARTESIAN_POINT('Ctrl Pts',(-44.4163794113386,47.7802696795038,
-216.765467472998));
#198816=CARTESIAN_POINT('Ctrl Pts',(-44.4487846007203,47.7660387569268,
-216.766433107496));
#198817=CARTESIAN_POINT('Ctrl Pts',(-44.479216953245,47.7524652205429,-216.767358276128));
#198818=CARTESIAN_POINT('Ctrl Pts',(-44.507632885208,47.7396533298788,-216.768218009436));
#198819=CARTESIAN_POINT('Ctrl Pts',(-44.5379039054705,47.726005035591,-216.769133869046));
#198820=CARTESIAN_POINT('Ctrl Pts',(-44.5658872349512,47.7132207550825,
-216.769975716415));
#198821=CARTESIAN_POINT('Ctrl Pts',(-44.5915712306527,47.7013845848144,
-216.770731900668));
#198822=CARTESIAN_POINT('Ctrl Pts',(-44.6203528538254,47.6881209090055,
-216.771579284793));
#198823=CARTESIAN_POINT('Ctrl Pts',(-44.6462477864905,47.6760476263165,
-216.772319371972));
#198824=CARTESIAN_POINT('Ctrl Pts',(-44.6692792696536,47.6652358761871,
-216.77295425634));
#198825=CARTESIAN_POINT('Ctrl Pts',(-44.6715286117851,47.6641799596007,
-216.773016261559));
#198826=CARTESIAN_POINT('Ctrl Pts',(-44.6737506639533,47.6631360444201,
-216.773077274141));
#198827=CARTESIAN_POINT('Ctrl Pts',(-44.6759454607542,47.6621041776483,
-216.773137302419));
#198828=CARTESIAN_POINT('Ctrl Pts',(-44.7037765107572,47.6490196243496,
-216.773898489067));
#198829=CARTESIAN_POINT('Ctrl Pts',(-44.7272086156641,47.6378971602701,
-216.774493853777));
#198830=CARTESIAN_POINT('Ctrl Pts',(-44.7463533295129,47.628772462078,-216.774960914982));
#198831=CARTESIAN_POINT('Ctrl Pts',(-44.7627930443094,47.6209370127176,
-216.775361984075));
#198832=CARTESIAN_POINT('Ctrl Pts',(-44.7760706843893,47.6145742802803,
-216.775668131786));
#198833=CARTESIAN_POINT('Ctrl Pts',(-44.7862332044631,47.6096979005449,
-216.775894447614));
#198834=CARTESIAN_POINT('Ctrl Pts',(-44.7941357857176,47.605905928986,-216.776070435381));
#198835=CARTESIAN_POINT('Ctrl Pts',(-44.8002363598239,47.6029767264898,
-216.776199286723));
#198836=CARTESIAN_POINT('Ctrl Pts',(-44.8083943648565,47.5990461730887,
-216.776372924679));
#198837=CARTESIAN_POINT('Ctrl Pts',(-44.8107273484308,47.5979221340024,
-216.776422580753));
#198838=CARTESIAN_POINT('Ctrl Pts',(-44.813228321892,47.5967161299053,-216.776475815531));
#198839=CARTESIAN_POINT('Ctrl Pts',(-44.8159867801204,47.5953843600175,
-216.776534542052));
#198840=CARTESIAN_POINT('Ctrl Pts',(-44.8314774654733,47.5879055343162,
-216.77686433282));
#198841=CARTESIAN_POINT('Ctrl Pts',(-44.8515740904643,47.5781633376041,
-216.777288516625));
#198842=CARTESIAN_POINT('Ctrl Pts',(-44.8761685367022,47.5661316606375,
-216.777775113872));
#198843=CARTESIAN_POINT('Ctrl Pts',(-44.9008453820597,47.5540596737741,
-216.778263341372));
#198844=CARTESIAN_POINT('Ctrl Pts',(-44.9300502849462,47.5396824427546,
-216.778814204285));
#198845=CARTESIAN_POINT('Ctrl Pts',(-44.9636231565079,47.522967707742,-216.779383698168));
#198846=CARTESIAN_POINT('Ctrl Pts',(-44.9971675948681,47.506267128606,-216.779952709741));
#198847=CARTESIAN_POINT('Ctrl Pts',(-45.0350726258933,47.4872324509082,
-216.780540039179));
#198848=CARTESIAN_POINT('Ctrl Pts',(-45.0771274087593,47.4658327612458,
-216.781093734266));
#198849=CARTESIAN_POINT('Ctrl Pts',(-45.0882843165739,47.4601555386197,
-216.781240626596));
#198850=CARTESIAN_POINT('Ctrl Pts',(-45.0997330089618,47.4543118970314,
-216.781385121284));
#198851=CARTESIAN_POINT('Ctrl Pts',(-45.1114689410713,47.4483013575709,
-216.781526195445));
#198852=CARTESIAN_POINT('Ctrl Pts',(-45.1395076970411,47.43394135211,-216.781863241017));
#198853=CARTESIAN_POINT('Ctrl Pts',(-45.1692394690722,47.4185847768683,
-216.78220619853));
#198854=CARTESIAN_POINT('Ctrl Pts',(-45.2006758201389,47.4021448352045,
-216.782569451285));
#198855=CARTESIAN_POINT('Ctrl Pts',(-45.2297367262886,47.3869471552708,
-216.782905255342));
#198856=CARTESIAN_POINT('Ctrl Pts',(-45.2602541421359,47.3708237485339,
-216.783258343756));
#198857=CARTESIAN_POINT('Ctrl Pts',(-45.2922640264201,47.3536723445899,
-216.783651004601));
#198858=CARTESIAN_POINT('Ctrl Pts',(-45.3230081294446,47.3371991663308,
-216.784028138281));
#198859=CARTESIAN_POINT('Ctrl Pts',(-45.3551287236645,47.3197779207588,
-216.784441678969));
#198860=CARTESIAN_POINT('Ctrl Pts',(-45.3886869395199,47.3012829987608,
-216.784923057149));
#198861=CARTESIAN_POINT('Ctrl Pts',(-45.4205801588626,47.2837057054223,
-216.785380551669));
#198862=CARTESIAN_POINT('Ctrl Pts',(-45.4537717327481,47.2651587428511,
-216.785899268647));
#198863=CARTESIAN_POINT('Ctrl Pts',(-45.4883440225305,47.2454997119075,
-216.786517961527));
#198864=CARTESIAN_POINT('Ctrl Pts',(-45.5024319813569,47.2374887985361,
-216.786770074415));
#198865=CARTESIAN_POINT('Ctrl Pts',(-45.5167495780152,47.2292928036801,
-216.787038933162));
#198866=CARTESIAN_POINT('Ctrl Pts',(-45.5313040065756,47.220900253631,-216.787327793623));
#198867=CARTESIAN_POINT('Ctrl Pts',(-45.5524181644651,47.2087251533791,
-216.787746844453));
#198868=CARTESIAN_POINT('Ctrl Pts',(-45.5741687627386,47.195992392959,-216.788262454171));
#198869=CARTESIAN_POINT('Ctrl Pts',(-45.5964324915328,47.1828114367862,
-216.788822892069));
#198870=CARTESIAN_POINT('Ctrl Pts',(-45.6157937849015,47.1713488304231,
-216.789310267865));
#198871=CARTESIAN_POINT('Ctrl Pts',(-45.6355427436437,47.1595476586865,
-216.789831377012));
#198872=CARTESIAN_POINT('Ctrl Pts',(-45.6555763820031,47.1475015125382,
-216.790342880917));
#198873=CARTESIAN_POINT('Ctrl Pts',(-45.6701261773398,47.1387527791373,
-216.79071436996));
#198874=CARTESIAN_POINT('Ctrl Pts',(-45.6848257139981,47.1298752419371,
-216.791080614918));
#198875=CARTESIAN_POINT('Ctrl Pts',(-45.6996282190663,47.1209119881337,
-216.791421896849));
#198876=CARTESIAN_POINT('Ctrl Pts',(-45.7074284250483,47.1161887858369,
-216.79160173596));
#198877=CARTESIAN_POINT('Ctrl Pts',(-45.7159680071028,47.1110106337719,
-216.791789776501));
#198878=CARTESIAN_POINT('Ctrl Pts',(-45.7236196209688,47.1063670490713,
-216.791947909506));
#198879=CARTESIAN_POINT('Ctrl Pts',(-45.7304885278804,47.1021984708337,
-216.792089866603));
#198880=CARTESIAN_POINT('Ctrl Pts',(-45.7366426222728,47.0984607701403,
-216.792208001644));
#198881=CARTESIAN_POINT('Ctrl Pts',(-45.7409359950755,47.0958528577209,
-216.792287234039));
#198882=CARTESIAN_POINT('Ctrl Pts',(-45.7417914642226,47.0953332222931,
-216.792303021364));
#198883=CARTESIAN_POINT('Ctrl Pts',(-45.7426465236319,47.094813812412,-216.792318647381));
#198884=CARTESIAN_POINT('Ctrl Pts',(-45.7435011644022,47.0942946370179,
-216.792334108291));
#198885=CARTESIAN_POINT('Ctrl Pts',(-45.7607808911895,47.0837975846006,
-216.792646707813));
#198886=CARTESIAN_POINT('Ctrl Pts',(-45.7778946723447,47.0733963572817,
-216.792896935563));
#198887=CARTESIAN_POINT('Ctrl Pts',(-45.7948624693683,47.0630713747316,
-216.793096051197));
#198888=CARTESIAN_POINT('Ctrl Pts',(-45.8304764893881,47.0414000797056,
-216.793513978649));
#198889=CARTESIAN_POINT('Ctrl Pts',(-45.8654477034202,47.0200642850446,
-216.793706933556));
#198890=CARTESIAN_POINT('Ctrl Pts',(-45.8999611384402,46.9988822608762,
-216.793779337632));
#198891=CARTESIAN_POINT('Ctrl Pts',(-45.9152590167607,46.9894934524855,
-216.793811430316));
#198892=CARTESIAN_POINT('Ctrl Pts',(-45.930466950287,46.9801348616291,-216.793819834911));
#198893=CARTESIAN_POINT('Ctrl Pts',(-45.945601020205,46.9707906928819,-216.793813626992));
#198894=CARTESIAN_POINT('Ctrl Pts',(-46.0405434277073,46.9121707788883,
-216.793774682097));
#198895=CARTESIAN_POINT('Ctrl Pts',(-46.1322571207837,46.8545743515597,
-216.793059832473));
#198896=CARTESIAN_POINT('Ctrl Pts',(-46.2249336316376,46.793472214907,-216.793167151654));
#198897=CARTESIAN_POINT('Ctrl Pts',(-46.2604025545799,46.7700873576591,
-216.793208224583));
#198898=CARTESIAN_POINT('Ctrl Pts',(-46.2960121446703,46.7461893965824,
-216.793369593332));
#198899=CARTESIAN_POINT('Ctrl Pts',(-46.3319960343607,46.7215258716012,
-216.793734755349));
#198900=CARTESIAN_POINT('Ctrl Pts',(-46.4053341178352,46.6712596088539,
-216.794478985135));
#198901=CARTESIAN_POINT('Ctrl Pts',(-46.4807017416469,46.6170461208078,
-216.796022478167));
#198902=CARTESIAN_POINT('Ctrl Pts',(-46.5530043796985,46.5649816566545,
-216.796566096102));
#198903=CARTESIAN_POINT('Ctrl Pts',(-46.6091179757941,46.5245747726023,
-216.796987994364));
#198904=CARTESIAN_POINT('Ctrl Pts',(-46.6633861233768,46.4854615099449,
-216.796807880319));
#198905=CARTESIAN_POINT('Ctrl Pts',(-46.7134409425736,46.4504754816595,
-216.795189569808));
#198906=CARTESIAN_POINT('Ctrl Pts',(-46.7687398835747,46.4118240521855,
-216.793401712837));
#198907=CARTESIAN_POINT('Ctrl Pts',(-46.8243036818415,46.3717158107884,
-216.792159988029));
#198908=CARTESIAN_POINT('Ctrl Pts',(-46.8797310108264,46.3309773553498,
-216.791008925619));
#198909=CARTESIAN_POINT('Ctrl Pts',(-46.9393413748466,46.2871644168086,
-216.789770993888));
#198910=CARTESIAN_POINT('Ctrl Pts',(-46.99879386052,46.2426226178321,-216.788637887748));
#198911=CARTESIAN_POINT('Ctrl Pts',(-47.0575921287076,46.1983743823903,
-216.787046295788));
#198912=CARTESIAN_POINT('Ctrl Pts',(-48.4710160211071,46.8924605148108,
-213.380827300298));
#198913=CARTESIAN_POINT('Ctrl Pts',(-48.4386236174112,46.8746099006705,
-215.343430354514));
#198914=CARTESIAN_POINT('Ctrl Pts',(-47.5746165801345,45.8238283676803,
-216.758537654376));
#198915=CARTESIAN_POINT('Ctrl Pts',(-48.18620705838,47.1231145402147,-213.379368669215));
#198916=CARTESIAN_POINT('Ctrl Pts',(-48.2020433443809,47.0656079993335,
-215.343093772686));
#198917=CARTESIAN_POINT('Ctrl Pts',(-47.4063346114126,45.9580463783679,
-216.758691640524));
#198918=CARTESIAN_POINT('Ctrl Pts',(-47.8936638370735,47.3370869807156,
-213.387528102977));
#198919=CARTESIAN_POINT('Ctrl Pts',(-47.960805927574,47.2450787050587,-215.353433308545));
#198920=CARTESIAN_POINT('Ctrl Pts',(-47.2339088845747,46.0827106122408,
-216.768384423919));
#198921=CARTESIAN_POINT('Ctrl Pts',(-47.5938143592261,47.5353276146285,
-213.404748058676));
#198922=CARTESIAN_POINT('Ctrl Pts',(-47.7151968771192,47.4137062867165,
-215.373807350724));
#198923=CARTESIAN_POINT('Ctrl Pts',(-47.0575921287078,46.1983743823903,
-216.787046295788));
#198924=CARTESIAN_POINT('',(-48.4710160211073,46.8924605148106,-213.380827300298));
#198925=CARTESIAN_POINT('',(-47.5746165801346,45.8238283676801,-216.758537654376));
#198926=CARTESIAN_POINT('Origin',(-45.3249961798233,43.0072392217583,-213.293565268111));
#198927=CARTESIAN_POINT('Origin',(-42.9552659882971,40.1115177027145,-218.083290145329));
#198928=CARTESIAN_POINT('Origin',(-45.3085773682635,42.9783608246564,-220.208955299598));
#198929=CARTESIAN_POINT('Ctrl Pts',(-51.7300796834963,44.0990078745201,
-213.405670914582));
#198930=CARTESIAN_POINT('Ctrl Pts',(-51.7004178351443,44.0801543735296,
-215.34722316631));
#198931=CARTESIAN_POINT('Ctrl Pts',(-50.7984099663007,43.0953291376926,
-216.756961257354));
#198932=CARTESIAN_POINT('Ctrl Pts',(-50.6732101690724,45.0571976655731,
-213.399273427569));
#198933=CARTESIAN_POINT('Ctrl Pts',(-50.6433589272572,45.0381703096645,
-215.345619228023));
#198934=CARTESIAN_POINT('Ctrl Pts',(-49.7561440689249,44.0321489495878,
-216.756606633385));
#198935=CARTESIAN_POINT('Ctrl Pts',(-49.5810652140705,45.993396027885,-213.390312554607));
#198936=CARTESIAN_POINT('Ctrl Pts',(-49.5465852937888,45.9777566735705,
-215.344527068816));
#198937=CARTESIAN_POINT('Ctrl Pts',(-48.6689534025116,44.9510092870384,
-216.757536292416));
#198938=CARTESIAN_POINT('Ctrl Pts',(-48.471016021107,46.8924605148109,-213.380827300298));
#198939=CARTESIAN_POINT('Ctrl Pts',(-48.4386236174111,46.8746099006705,
-215.343430354514));
#198940=CARTESIAN_POINT('Ctrl Pts',(-47.5746165801344,45.8238283676802,
-216.758537654376));
#198941=CARTESIAN_POINT('Ctrl Pts',(-51.7111509881036,44.1161634878024,
-213.405556127478));
#198942=CARTESIAN_POINT('Ctrl Pts',(-50.6601717838604,45.0683724383644,
-213.399166479425));
#198943=CARTESIAN_POINT('Ctrl Pts',(-49.5744394718705,45.9987624282913,
-213.390255981635));
#198944=CARTESIAN_POINT('Ctrl Pts',(-48.4710160211073,46.8924605148106,
-213.380827300298));
#198945=CARTESIAN_POINT('Ctrl Pts',(-47.5746165801346,45.8238283676801,
-216.758537654376));
#198946=CARTESIAN_POINT('Ctrl Pts',(-48.2691158909411,45.2699109287623,
-216.75790215973));
#198947=CARTESIAN_POINT('Ctrl Pts',(-48.960736291415,44.6974523761734,-216.757294260093));
#198948=CARTESIAN_POINT('Ctrl Pts',(-49.6398238003658,44.1136236554352,
-216.757027743291));
#198949=CARTESIAN_POINT('Ctrl Pts',(-33.311755802625,-74.7642469038882,
-216.366493231411));
#198950=CARTESIAN_POINT('Ctrl Pts',(-33.1370520886648,-74.8239894378111,
-216.284592934174));
#198951=CARTESIAN_POINT('Ctrl Pts',(-32.9632085045191,-74.8606208373411,
-216.188495172326));
#198952=CARTESIAN_POINT('Ctrl Pts',(-31.1602774969193,-72.7635470433165,
-219.49364146861));
#198953=CARTESIAN_POINT('Ctrl Pts',(-30.9603372594918,-72.8299657459105,
-219.402724042838));
#198954=CARTESIAN_POINT('Ctrl Pts',(-30.7643643263463,-72.869370950888,
-219.290077373128));
#198955=CARTESIAN_POINT('Ctrl Pts',(-29.0180188301449,-70.7601533693957,
-222.625390207514));
#198956=CARTESIAN_POINT('Ctrl Pts',(-28.7897411455683,-70.83439285059,-222.523822671102));
#198957=CARTESIAN_POINT('Ctrl Pts',(-28.568544162562,-70.8754191108834,
-222.392137619968));
#198958=CARTESIAN_POINT('Ctrl Pts',(-24.7728929630407,-66.7728546038162,
-228.85960306067));
#198959=CARTESIAN_POINT('Ctrl Pts',(-24.4825290072419,-66.8674311471827,
-228.729735935856));
#198960=CARTESIAN_POINT('Ctrl Pts',(-24.2020295713952,-66.9044734350692,
-228.556369888754));
#198961=CARTESIAN_POINT('Ctrl Pts',(-22.6699986370471,-64.7889483543043,
-231.9620410804));
#198962=CARTESIAN_POINT('Ctrl Pts',(-22.342807556714,-64.8931064786587,
-231.819117937466));
#198963=CARTESIAN_POINT('Ctrl Pts',(-22.031404906377,-64.9275141607773,
-231.618589156426));
#198964=CARTESIAN_POINT('Ctrl Pts',(-20.5752479313931,-62.80283290697,-235.068543705361));
#198965=CARTESIAN_POINT('Ctrl Pts',(-20.2128373512436,-62.9236980507114,
-234.901590690922));
#198966=CARTESIAN_POINT('Ctrl Pts',(-19.8613391097003,-62.9451022381765,
-234.678400237559));
#198967=CARTESIAN_POINT('Ctrl Pts',(-20.0008767707151,-63.0723812833681,
-234.482033933863));
#198968=CARTESIAN_POINT('Ctrl Pts',(-20.6994986722916,-63.7105120854193,
-233.496935192946));
#198969=CARTESIAN_POINT('Ctrl Pts',(-21.3982133314812,-64.3480811557091,
-232.511588190799));
#198970=CARTESIAN_POINT('Ctrl Pts',(-22.09694219437,-64.9851687951656,-231.52601338522));
#198971=CARTESIAN_POINT('Ctrl Pts',(-22.8095499458537,-65.6349109403151,
-230.520862054818));
#198972=CARTESIAN_POINT('Ctrl Pts',(-23.5221722228719,-66.2841526165371,
-229.515473781363));
#198973=CARTESIAN_POINT('Ctrl Pts',(-24.2347817439218,-66.9329758189411,
-228.509870266089));
#198974=CARTESIAN_POINT('Ctrl Pts',(-24.9473912649716,-67.5817990213451,
-227.504266750816));
#198975=CARTESIAN_POINT('Ctrl Pts',(-25.6599879657153,-68.2302039689098,
-226.498447993724));
#198976=CARTESIAN_POINT('Ctrl Pts',(-26.3726021547331,-68.8782657659646,
-225.492435696049));
#198977=CARTESIAN_POINT('Ctrl Pts',(-27.0584834080819,-69.502016239168,
-224.524162840629));
#198978=CARTESIAN_POINT('Ctrl Pts',(-27.7443776014784,-70.1254486506369,
-223.555710117061));
#198979=CARTESIAN_POINT('Ctrl Pts',(-28.4303298112128,-70.7485890029029,
-222.587148305811));
#198980=CARTESIAN_POINT('Ctrl Pts',(-29.113962572594,-71.3696222960424,
-221.621861546477));
#198981=CARTESIAN_POINT('Ctrl Pts',(-29.7976529446887,-71.9903656062306,
-220.656466435943));
#198982=CARTESIAN_POINT('Ctrl Pts',(-30.4814962405759,-72.6108344008091,
-219.691033039098));
#198983=CARTESIAN_POINT('Ctrl Pts',(-31.1627382119588,-73.2289429460596,
-218.729272129163));
#198984=CARTESIAN_POINT('Ctrl Pts',(-31.8441319441618,-73.8467791355826,
-217.767473223644));
#198985=CARTESIAN_POINT('Ctrl Pts',(-32.5258221696848,-74.4643467152214,
-216.805705590893));
#198986=CARTESIAN_POINT('Ctrl Pts',(-32.625128162791,-74.5543115695057,
-216.665599005333));
#198987=CARTESIAN_POINT('Ctrl Pts',(-32.7244405356851,-74.6442707023382,
-216.525493083429));
#198988=CARTESIAN_POINT('Ctrl Pts',(-32.8237598256929,-74.7342241033977,
-216.385388039322));
#198989=CARTESIAN_POINT('Ctrl Pts',(-33.175226286096,-74.6372704537072,
-216.564961398278));
#198990=CARTESIAN_POINT('Ctrl Pts',(-31.0696461183976,-72.6787866297426,
-219.626141064238));
#198991=CARTESIAN_POINT('Ctrl Pts',(-28.9728566675979,-70.7177341242162,
-222.691713455173));
#198992=CARTESIAN_POINT('Ctrl Pts',(-26.8829915137441,-68.754796626235,
-225.760801301184));
#198993=CARTESIAN_POINT('Ctrl Pts',(-24.8618782439252,-66.8564353766208,
-228.728923029217));
#198994=CARTESIAN_POINT('Ctrl Pts',(-22.8473703074868,-64.9562682462704,
-231.700386778281));
#198995=CARTESIAN_POINT('Ctrl Pts',(-20.8402917355536,-63.0540784606782,
-234.675571320252));
#198996=CARTESIAN_POINT('Ctrl Pts',(-48.394724810452,-30.9589748864444,
-236.571980303288));
#198997=CARTESIAN_POINT('Ctrl Pts',(-48.5327606194891,-30.5978875071193,
-236.384422495983));
#198998=CARTESIAN_POINT('Ctrl Pts',(-48.5655760584043,-30.2484467958801,
-236.13656993524));
#198999=CARTESIAN_POINT('Ctrl Pts',(-53.1357762583618,-36.5300914807295,
-229.349840256805));
#199000=CARTESIAN_POINT('Ctrl Pts',(-53.2603596661385,-36.1854606467053,
-229.182436919715));
#199001=CARTESIAN_POINT('Ctrl Pts',(-53.3041702101809,-35.8631937708939,
-228.944594002505));
#199002=CARTESIAN_POINT('Ctrl Pts',(-57.8701242734414,-42.1160518009944,
-222.134994554844));
#199003=CARTESIAN_POINT('Ctrl Pts',(-57.9936838628245,-41.7882503199416,
-221.968743812371));
#199004=CARTESIAN_POINT('Ctrl Pts',(-58.0357658478494,-41.4733525338354,
-221.746435886425));
#199005=CARTESIAN_POINT('Ctrl Pts',(-62.6038224850394,-47.7030040725398,
-214.920479869356));
#199006=CARTESIAN_POINT('Ctrl Pts',(-62.725814975539,-47.3874591829502,
-214.756341305096));
#199007=CARTESIAN_POINT('Ctrl Pts',(-62.767435183335,-47.0792819180526,
-214.544947314852));
#199008=CARTESIAN_POINT('Ctrl Pts',(-49.628292311974,-32.4090169808449,
-234.692797218109));
#199009=CARTESIAN_POINT('Ctrl Pts',(-53.5927125130264,-37.0706922464491,
-228.653306547473));
#199010=CARTESIAN_POINT('Ctrl Pts',(-57.552810123003,-41.7419121172879,
-222.6184966732));
#199011=CARTESIAN_POINT('Ctrl Pts',(-61.5121276273779,-46.414570793914,
-216.584292819144));
#199012=CARTESIAN_POINT('Ctrl Pts',(-61.6760242364037,-45.7878268313144,
-216.206690793879));
#199013=CARTESIAN_POINT('Ctrl Pts',(-61.1290793515412,-45.1397569490598,
-217.039067196821));
#199014=CARTESIAN_POINT('Ctrl Pts',(-60.5821634713164,-44.4918554909971,
-217.871396329666));
#199015=CARTESIAN_POINT('Ctrl Pts',(-60.0352403841908,-43.8439595660193,
-218.703673746095));
#199016=CARTESIAN_POINT('Ctrl Pts',(-59.4881996162324,-43.1959242339954,
-219.53613024273));
#199017=CARTESIAN_POINT('Ctrl Pts',(-58.9411516343724,-42.5478944393375,
-220.36853500069));
#199018=CARTESIAN_POINT('Ctrl Pts',(-58.3940681475654,-41.8997587412459,
-221.200883570786));
#199019=CARTESIAN_POINT('Ctrl Pts',(-57.8468424352846,-41.251454547104,
-222.033448526813));
#199020=CARTESIAN_POINT('Ctrl Pts',(-57.2995811930056,-40.6030443972108,
-222.865957265757));
#199021=CARTESIAN_POINT('Ctrl Pts',(-56.7522641358422,-39.9544683058983,
-223.698405334957));
#199022=CARTESIAN_POINT('Ctrl Pts',(-56.2047806782684,-39.3056950284643,
-224.531106492743));
#199023=CARTESIAN_POINT('Ctrl Pts',(-55.6572413649869,-38.6567557119309,
-225.363746943889));
#199024=CARTESIAN_POINT('Ctrl Pts',(-55.1096340281199,-38.0076418378489,
-226.196322231672));
#199025=CARTESIAN_POINT('Ctrl Pts',(-54.5617391016561,-37.3581870654904,
-227.02933476705));
#199026=CARTESIAN_POINT('Ctrl Pts',(-54.0137760751197,-36.7085575539615,
-227.862282070602));
#199027=CARTESIAN_POINT('Ctrl Pts',(-53.4657409963451,-36.0587963044242,
-228.695159678579));
#199028=CARTESIAN_POINT('Ctrl Pts',(-52.917521126298,-35.4088159626922,
-229.528318123531));
#199029=CARTESIAN_POINT('Ctrl Pts',(-52.3692291552187,-34.7587037974105,
-230.361406825898));
#199030=CARTESIAN_POINT('Ctrl Pts',(-51.8208694062986,-34.1085543663928,
-231.194421317416));
#199031=CARTESIAN_POINT('Ctrl Pts',(-51.272227397378,-33.4580702806543,
-232.027864590717));
#199032=CARTESIAN_POINT('Ctrl Pts',(-50.7235175473517,-32.8075488919341,
-232.861233576751));
#199033=CARTESIAN_POINT('Ctrl Pts',(-50.1747524277536,-32.1571364299523,
-233.694523800349));
#199034=CARTESIAN_POINT('Ctrl Pts',(-50.0025400417543,-31.9530252757239,
-233.956025292537));
#199035=CARTESIAN_POINT('Ctrl Pts',(-49.8303222731896,-31.7489252297835,
-234.217519028063));
#199036=CARTESIAN_POINT('Ctrl Pts',(-49.6580996754575,-31.5448418565169,
-234.479004868619));
#199037=CARTESIAN_POINT('Ctrl Pts',(-62.7235255475978,21.7695413998821,
-214.740437532627));
#199038=CARTESIAN_POINT('Ctrl Pts',(-62.8230072917154,21.4551226732318,
-214.60836056406));
#199039=CARTESIAN_POINT('Ctrl Pts',(-62.8511336743851,21.1472686270111,
-214.433330258979));
#199040=CARTESIAN_POINT('Ctrl Pts',(-57.9208187259037,17.1708899867545,
-222.060179301836));
#199041=CARTESIAN_POINT('Ctrl Pts',(-58.021494482598,16.8444023505525,-221.926546858332));
#199042=CARTESIAN_POINT('Ctrl Pts',(-58.0497358031121,16.5287545279998,
-221.741752515028));
#199043=CARTESIAN_POINT('Ctrl Pts',(-53.1176466678688,12.5728508607834,
-229.37998710404));
#199044=CARTESIAN_POINT('Ctrl Pts',(-53.218552259156,12.2298050378563,-229.246394945677));
#199045=CARTESIAN_POINT('Ctrl Pts',(-53.2484412443996,11.9055419092803,
-229.047156021484));
#199046=CARTESIAN_POINT('Ctrl Pts',(-48.3085599855162,7.99018616088097,
-236.705793683792));
#199047=CARTESIAN_POINT('Ctrl Pts',(-48.4218941664573,7.62742728044422,
-236.553636438645));
#199048=CARTESIAN_POINT('Ctrl Pts',(-48.4402788929552,7.27533655185505,
-236.345585245331));
#199049=CARTESIAN_POINT('Ctrl Pts',(-49.6480781836461,8.44024209637812,
-234.512742074857));
#199050=CARTESIAN_POINT('Ctrl Pts',(-50.20384928812,8.97542501790977,-233.668782076087));
#199051=CARTESIAN_POINT('Ctrl Pts',(-50.7595723119519,9.51073706975706,
-232.824733121525));
#199052=CARTESIAN_POINT('Ctrl Pts',(-51.3152323625987,10.0460216112609,
-231.980601369281));
#199053=CARTESIAN_POINT('Ctrl Pts',(-51.8706442281392,10.5810670683631,
-231.136846647792));
#199054=CARTESIAN_POINT('Ctrl Pts',(-52.4259931689815,11.1160850375145,
-230.293009202567));
#199055=CARTESIAN_POINT('Ctrl Pts',(-52.9812725114739,11.650970496052,-229.449095183471));
#199056=CARTESIAN_POINT('Ctrl Pts',(-53.5363226339063,12.1856351531522,
-228.605529533217));
#199057=CARTESIAN_POINT('Ctrl Pts',(-54.0913032149207,12.7201674059514,
-227.761887372297));
#199058=CARTESIAN_POINT('Ctrl Pts',(-54.6462158429117,13.2545137793697,
-226.918174842962));
#199059=CARTESIAN_POINT('Ctrl Pts',(-55.2296271481594,13.8163026078182,
-226.031131724526));
#199060=CARTESIAN_POINT('Ctrl Pts',(-55.8129632662219,14.3778854664311,
-225.144010824245));
#199061=CARTESIAN_POINT('Ctrl Pts',(-56.3962358505564,14.9392616066232,
-224.256819280148));
#199062=CARTESIAN_POINT('Ctrl Pts',(-56.9505543180094,15.4727705869074,
-223.413668632801));
#199063=CARTESIAN_POINT('Ctrl Pts',(-57.5048154823728,16.0060933155577,
-222.570454181187));
#199064=CARTESIAN_POINT('Ctrl Pts',(-58.0590376778228,16.539281928092,-221.727182052217));
#199065=CARTESIAN_POINT('Ctrl Pts',(-58.6131392156513,17.0723544621467,
-220.884093508838));
#199066=CARTESIAN_POINT('Ctrl Pts',(-59.1672018083433,17.6052929351375,
-220.040947313213));
#199067=CARTESIAN_POINT('Ctrl Pts',(-59.7212517903796,18.1382009308084,
-219.197749588254));
#199068=CARTESIAN_POINT('Ctrl Pts',(-60.2751697034323,18.6709818971143,
-218.354752856472));
#199069=CARTESIAN_POINT('Ctrl Pts',(-60.8290750163752,19.2037323987446,
-217.511704619919));
#199070=CARTESIAN_POINT('Ctrl Pts',(-61.3830019667998,19.7366074479272,
-216.668610997126));
#199071=CARTESIAN_POINT('Ctrl Pts',(-61.470215935575,19.8205068643843,-216.535868690877));
#199072=CARTESIAN_POINT('Ctrl Pts',(-61.5574304566285,19.9044094721162,
-216.403125259528));
#199073=CARTESIAN_POINT('Ctrl Pts',(-61.6446456814072,19.9883159925441,
-216.270380726959));
#199074=CARTESIAN_POINT('Ctrl Pts',(-61.516838435851,20.614157501844,-216.579518431211));
#199075=CARTESIAN_POINT('Ctrl Pts',(-57.5570112912469,16.8228354627662,
-222.614535941297));
#199076=CARTESIAN_POINT('Ctrl Pts',(-53.5965576606815,13.0327700456284,
-228.64993609011));
#199077=CARTESIAN_POINT('Ctrl Pts',(-49.6324230235363,9.25223577675679,
-234.689044294154));
#199078=CARTESIAN_POINT('Ctrl Pts',(-23.9003793742247,38.8880062428322,
-234.874538682189));
#199079=CARTESIAN_POINT('Ctrl Pts',(-23.6220334826828,38.9711510838488,
-234.795483705848));
#199080=CARTESIAN_POINT('Ctrl Pts',(-23.3436315228967,39.0028243075697,
-234.685354940774));
#199081=CARTESIAN_POINT('Ctrl Pts',(-25.3613763022199,40.7570726350447,
-231.772074582798));
#199082=CARTESIAN_POINT('Ctrl Pts',(-25.0911791370723,40.8413872876637,
-231.69349554685));
#199083=CARTESIAN_POINT('Ctrl Pts',(-24.8211729610243,40.8777894793531,
-231.583592072777));
#199084=CARTESIAN_POINT('Ctrl Pts',(-26.8976008470641,42.6201313632963,
-228.700804953167));
#199085=CARTESIAN_POINT('Ctrl Pts',(-26.6295221643462,42.7083584759227,
-228.618927707697));
#199086=CARTESIAN_POINT('Ctrl Pts',(-26.3601999892212,42.7472524558864,
-228.507951791168));
#199087=CARTESIAN_POINT('Ctrl Pts',(-30.0998495294269,46.3266672929645,
-222.608682403592));
#199088=CARTESIAN_POINT('Ctrl Pts',(-29.8266052300516,46.4238562842224,
-222.520666200209));
#199089=CARTESIAN_POINT('Ctrl Pts',(-29.5516593753034,46.4688062321367,
-222.401370424925));
#199090=CARTESIAN_POINT('Ctrl Pts',(-31.7641932541652,48.1699050147461,
-219.588919241872));
#199091=CARTESIAN_POINT('Ctrl Pts',(-31.4847343983961,48.2732692238746,
-219.496139318467));
#199092=CARTESIAN_POINT('Ctrl Pts',(-31.2025135348749,48.3205140505153,
-219.371535847534));
#199093=CARTESIAN_POINT('Ctrl Pts',(-33.4734406974175,50.0051916640201,
-216.589120385861));
#199094=CARTESIAN_POINT('Ctrl Pts',(-33.1846932575851,50.1143213461433,
-216.493132115845));
#199095=CARTESIAN_POINT('Ctrl Pts',(-32.8943360433596,50.1648136138276,
-216.360311415042));
#199096=CARTESIAN_POINT('Ctrl Pts',(-23.9972286658434,39.0117605909834,
-234.66915169881));
#199097=CARTESIAN_POINT('Ctrl Pts',(-25.4292211151269,40.839311165325,-231.636508421791));
#199098=CARTESIAN_POINT('Ctrl Pts',(-26.9329390257305,42.6610372183491,
-228.633571847125));
#199099=CARTESIAN_POINT('Ctrl Pts',(-30.0998477125744,46.3266679391917,
-222.608681818355));
#199100=CARTESIAN_POINT('Ctrl Pts',(-31.7641913965495,48.1699057018269,
-219.588918625145));
#199101=CARTESIAN_POINT('Ctrl Pts',(-33.473440697418,50.0051916640197,-216.589120385862));
#199102=CARTESIAN_POINT('Ctrl Pts',(-32.8943360433598,50.1648136138275,
-216.360311415042));
#199103=CARTESIAN_POINT('Ctrl Pts',(-31.2025135348749,48.3205140505153,
-219.371535847534));
#199104=CARTESIAN_POINT('Ctrl Pts',(-29.5516593753034,46.4688062321367,
-222.401370424925));
#199105=CARTESIAN_POINT('Ctrl Pts',(-26.3792344265555,42.76944847143,-228.471531042451));
#199106=CARTESIAN_POINT('Ctrl Pts',(-24.8578971641406,40.9223874961028,
-231.510220567283));
#199107=CARTESIAN_POINT('Ctrl Pts',(-23.3965311730097,39.0699180251917,
-234.574369193282));
#199108=CARTESIAN_POINT('Origin',(-7.99493453126772,-4.92182388367686,-192.281986444803));
#199109=CARTESIAN_POINT('',(-7.45184924284871,-4.40456343718705,-229.35005));
#199110=CARTESIAN_POINT('',(-8.57396770167424,-4.44514727677342,-229.35005));
#199111=CARTESIAN_POINT('Origin',(-7.99493453126772,-4.92182388367686,-229.35005));
#199112=CARTESIAN_POINT('',(-8.57396770167424,-4.44514727677342,-192.281986444803));
#199113=CARTESIAN_POINT('',(-7.45184924284871,-4.40456343718705,-192.281986444803));
#199114=CARTESIAN_POINT('Origin',(-1.25,-20.2703558849778,-192.281986444803));
#199115=CARTESIAN_POINT('',(-0.5,-20.2703558849778,-229.35005));
#199116=CARTESIAN_POINT('',(-0.5,-20.2703558849778,-235.35005));
#199117=CARTESIAN_POINT('',(-1.14413406213993,-19.5278652094801,-229.35005));
#199118=CARTESIAN_POINT('Origin',(-1.25,-20.2703558849778,-229.35005));
#199119=CARTESIAN_POINT('',(-1.14413406213993,-19.5278652094801,-192.281986444803));
#199120=CARTESIAN_POINT('Origin',(-10.2798200094577,-12.7534818258363,-192.281986444803));
#199121=CARTESIAN_POINT('',(-10.2798200094577,-12.0034818258363,-229.35005));
#199122=CARTESIAN_POINT('',(-10.2798200094577,-12.0034818258363,-229.35005));
#199123=CARTESIAN_POINT('',(-11.0243360211906,-12.844013081618,-229.35005));
#199124=CARTESIAN_POINT('Origin',(-10.2798200094577,-12.7534818258363,-229.35005));
#199125=CARTESIAN_POINT('',(-11.0243360211906,-12.844013081618,-192.281986444803));
#199126=CARTESIAN_POINT('Origin',(-8.76687405914144,-12.7534818258363,-192.281986444803));
#199127=CARTESIAN_POINT('',(-8.02438338364376,-12.6476158879763,-229.35005));
#199128=CARTESIAN_POINT('',(-8.02438338364376,-12.6476158879763,-192.281986444803));
#199129=CARTESIAN_POINT('',(-8.76687405914144,-12.0034818258363,-229.35005));
#199130=CARTESIAN_POINT('Origin',(-8.76687405914144,-12.7534818258363,-229.35005));
#199131=CARTESIAN_POINT('',(-8.76687405914144,-12.0034818258363,-235.35005));
#199132=CARTESIAN_POINT('Origin',(-8.76687405914145,-10.2534818258363,-192.281986444803));
#199133=CARTESIAN_POINT('',(-8.76687405914145,-11.0034818258363,-229.35005));
#199134=CARTESIAN_POINT('',(-8.76687405914145,-11.0034818258363,-229.35005));
#199135=CARTESIAN_POINT('',(-8.02438338364376,-10.3593477636964,-229.35005));
#199136=CARTESIAN_POINT('Origin',(-8.76687405914145,-10.2534818258363,-229.35005));
#199137=CARTESIAN_POINT('',(-8.02438338364376,-10.3593477636964,-192.281986444803));
#199138=CARTESIAN_POINT('Origin',(-10.2798200094577,-10.2534818258363,-192.281986444803));
#199139=CARTESIAN_POINT('',(-11.0243360211906,-10.1629505700546,-229.35005));
#199140=CARTESIAN_POINT('',(-11.0243360211906,-10.1629505700546,-192.281986444803));
#199141=CARTESIAN_POINT('',(-10.2798200094577,-11.0034818258363,-229.35005));
#199142=CARTESIAN_POINT('Origin',(-10.2798200094577,-10.2534818258363,-229.35005));
#199143=CARTESIAN_POINT('',(-10.2798200094577,-11.0034818258363,-229.35005));
#199144=CARTESIAN_POINT('Origin',(-6.95148506756697,-6.01736880073006,-192.281986444803));
#199145=CARTESIAN_POINT('',(-6.36274467860838,-6.48200280121742,-229.35005));
#199146=CARTESIAN_POINT('',(-6.36274467860838,-6.48200280121742,-192.281986444803));
#199147=CARTESIAN_POINT('',(-6.40839977914796,-5.50010835424024,-229.35005));
#199148=CARTESIAN_POINT('Origin',(-6.95148506756697,-6.01736880073006,-229.35005));
#199149=CARTESIAN_POINT('',(-6.40839977914796,-5.50010835424024,-235.35005));
#199150=CARTESIAN_POINT('Origin',(-5.14120077283694,-4.29316731243069,-192.281986444803));
#199151=CARTESIAN_POINT('',(-5.68428606125595,-4.81042775892049,-229.35005));
#199152=CARTESIAN_POINT('',(-5.68428606125595,-4.81042775892049,-229.35005));
#199153=CARTESIAN_POINT('',(-4.70577833960231,-4.90382867901287,-229.35005));
#199154=CARTESIAN_POINT('Origin',(-5.14120077283694,-4.29316731243068,-229.35005));
#199155=CARTESIAN_POINT('',(-4.70577833960231,-4.90382867901288,-192.281986444803));
#199156=CARTESIAN_POINT('Origin',(-1.25,-2.73660776669488,-192.281986444803));
#199157=CARTESIAN_POINT('',(-1.14413406213993,-3.47909844219256,-229.35005));
#199158=CARTESIAN_POINT('',(-1.14413406213993,-3.47909844219257,-192.281986444803));
#199159=CARTESIAN_POINT('',(-0.5,-2.73660776669487,-229.35005));
#199160=CARTESIAN_POINT('Origin',(-1.25,-2.73660776669487,-229.35005));
#199161=CARTESIAN_POINT('',(-0.5,-2.73660776669487,-235.35005));
#199162=CARTESIAN_POINT('Origin',(-8.87499999999985,-23.3741205625531,-192.281986444803));
#199163=CARTESIAN_POINT('',(-8.83216440217218,-22.6253448207192,-229.35005));
#199164=CARTESIAN_POINT('',(-9.62499999999985,-23.3741205625531,-229.35005));
#199165=CARTESIAN_POINT('Origin',(-8.87499999999985,-23.3741205625531,-229.35005));
#199166=CARTESIAN_POINT('',(-9.62499999999985,-23.3741205625531,-235.35005));
#199167=CARTESIAN_POINT('',(-8.83216440217218,-22.6253448207192,-192.281986444803));
#199168=CARTESIAN_POINT('Origin',(-12.7946237611812,-12.7534818258363,-192.281986444803));
#199169=CARTESIAN_POINT('',(-12.0481776255232,-12.6805560652209,-229.35005));
#199170=CARTESIAN_POINT('',(-12.0481776255232,-12.6805560652209,-192.281986444803));
#199171=CARTESIAN_POINT('',(-12.7946237611812,-12.0034818258363,-229.35005));
#199172=CARTESIAN_POINT('Origin',(-12.7946237611812,-12.7534818258363,-229.35005));
#199173=CARTESIAN_POINT('',(-12.7946237611812,-12.0034818258363,-235.35005));
#199174=CARTESIAN_POINT('Origin',(-11.3749999999999,-20.8590213785032,-229.35005));
#199175=CARTESIAN_POINT('',(-11.3749999999999,-21.6090213785032,-229.35005));
#199176=CARTESIAN_POINT('',(-11.3749999999999,-21.6090213785032,-229.35005));
#199177=CARTESIAN_POINT('',(-10.6249999999999,-20.8590213785032,-229.35005));
#199178=CARTESIAN_POINT('Origin',(-11.3749999999999,-20.8590213785032,-229.35005));
#199179=CARTESIAN_POINT('',(-10.6249999999999,-20.8590213785032,-235.35005));
#199180=CARTESIAN_POINT('Origin',(-19.,-20.8590213785032,-229.35005));
#199181=CARTESIAN_POINT('',(-19.75,-20.8590213785032,-229.35005));
#199182=CARTESIAN_POINT('',(-19.75,-20.8590213785032,-235.35005));
#199183=CARTESIAN_POINT('',(-19.,-21.6090213785031,-229.35005));
#199184=CARTESIAN_POINT('Origin',(-19.,-20.8590213785032,-229.35005));
#199185=CARTESIAN_POINT('',(-19.,-21.6090213785031,-229.35005));
#199186=CARTESIAN_POINT('Origin',(-19.,-12.7534818258363,-229.35005));
#199187=CARTESIAN_POINT('',(-19.,-12.0034818258363,-229.35005));
#199188=CARTESIAN_POINT('',(-19.,-12.0034818258363,-229.35005));
#199189=CARTESIAN_POINT('',(-19.75,-12.7534818258363,-229.35005));
#199190=CARTESIAN_POINT('Origin',(-19.,-12.7534818258363,-229.35005));
#199191=CARTESIAN_POINT('',(-19.75,-12.7534818258363,-235.35005));
#199192=CARTESIAN_POINT('Origin',(-12.7946237611812,-10.2534818258363,-192.281986444803));
#199193=CARTESIAN_POINT('',(-12.7946237611812,-11.0034818258363,-229.35005));
#199194=CARTESIAN_POINT('',(-12.7946237611812,-11.0034818258363,-229.35005));
#199195=CARTESIAN_POINT('',(-12.0481776255232,-10.3264075864518,-229.35005));
#199196=CARTESIAN_POINT('Origin',(-12.7946237611812,-10.2534818258363,-229.35005));
#199197=CARTESIAN_POINT('',(-12.0481776255232,-10.3264075864518,-192.281986444803));
#199198=CARTESIAN_POINT('Origin',(-19.,-10.2534818258363,-229.35005));
#199199=CARTESIAN_POINT('',(-19.75,-10.2534818258363,-229.35005));
#199200=CARTESIAN_POINT('',(-19.75,-10.2534818258363,-235.35005));
#199201=CARTESIAN_POINT('',(-19.,-11.0034818258363,-229.35005));
#199202=CARTESIAN_POINT('Origin',(-19.,-10.2534818258363,-229.35005));
#199203=CARTESIAN_POINT('',(-19.,-11.0034818258363,-229.35005));
#199204=CARTESIAN_POINT('Origin',(-19.,-2.14794227316951,-229.35005));
#199205=CARTESIAN_POINT('',(-19.,-1.39794227316951,-229.35005));
#199206=CARTESIAN_POINT('',(-19.,-1.39794227316951,-229.35005));
#199207=CARTESIAN_POINT('',(-19.75,-2.14794227316951,-229.35005));
#199208=CARTESIAN_POINT('Origin',(-19.,-2.14794227316951,-229.35005));
#199209=CARTESIAN_POINT('',(-19.75,-2.14794227316951,-235.35005));
#199210=CARTESIAN_POINT('Origin',(-11.3749999999999,-2.14794227316951,-229.35005));
#199211=CARTESIAN_POINT('',(-10.6249999999999,-2.14794227316951,-229.35005));
#199212=CARTESIAN_POINT('',(-10.6249999999999,-2.14794227316951,-235.35005));
#199213=CARTESIAN_POINT('',(-11.3749999999999,-1.3979422731695,-229.35005));
#199214=CARTESIAN_POINT('Origin',(-11.3749999999999,-2.14794227316951,-229.35005));
#199215=CARTESIAN_POINT('',(-11.3749999999999,-1.3979422731695,-229.35005));
#199216=CARTESIAN_POINT('Origin',(-8.87499999999985,0.367156910880378,-192.281986444803));
#199217=CARTESIAN_POINT('',(-9.62499999999985,0.367156910880385,-229.35005));
#199218=CARTESIAN_POINT('',(-9.62499999999985,0.367156910880383,-229.35005));
#199219=CARTESIAN_POINT('',(-8.83216440217218,-0.38161883095341,-229.35005));
#199220=CARTESIAN_POINT('Origin',(-8.87499999999985,0.367156910880383,-229.35005));
#199221=CARTESIAN_POINT('',(-8.83216440217218,-0.381618830953416,-192.281986444803));
#199222=CARTESIAN_POINT('Origin',(-8.87499999999986,8.45759727949731,-229.35005));
#199223=CARTESIAN_POINT('',(-8.87499999999986,9.20759727949731,-229.35005));
#199224=CARTESIAN_POINT('',(-8.87499999999986,9.20759727949731,-229.35005));
#199225=CARTESIAN_POINT('',(-9.62499999999986,8.45759727949731,-229.35005));
#199226=CARTESIAN_POINT('Origin',(-8.87499999999986,8.45759727949731,-229.35005));
#199227=CARTESIAN_POINT('',(-9.62499999999986,8.45759727949731,-235.35005));
#199228=CARTESIAN_POINT('Origin',(-1.25,8.45759727949731,-229.35005));
#199229=CARTESIAN_POINT('',(-0.5,8.45759727949731,-229.35005));
#199230=CARTESIAN_POINT('',(-0.5,8.45759727949731,-235.35005));
#199231=CARTESIAN_POINT('',(-1.25,9.20759727949731,-229.35005));
#199232=CARTESIAN_POINT('Origin',(-1.25,8.45759727949731,-229.35005));
#199233=CARTESIAN_POINT('',(-1.25,9.20759727949731,-229.35005));
#199234=CARTESIAN_POINT('Origin',(-1.25,2.29555713691451,-192.281986444803));
#199235=CARTESIAN_POINT('',(-1.18233753211584,1.54861551239502,-229.35005));
#199236=CARTESIAN_POINT('',(-1.18233753211584,1.54861551239501,-192.281986444803));
#199237=CARTESIAN_POINT('',(-0.5,2.29555713691451,-229.35005));
#199238=CARTESIAN_POINT('Origin',(-1.25,2.29555713691451,-229.35005));
#199239=CARTESIAN_POINT('',(-0.5,2.29555713691451,-235.35005));
#199240=CARTESIAN_POINT('Origin',(-1.25,-25.3025207885872,-192.281986444803));
#199241=CARTESIAN_POINT('',(-0.5,-25.3025207885872,-229.35005));
#199242=CARTESIAN_POINT('',(-0.5,-25.3025207885872,-235.35005));
#199243=CARTESIAN_POINT('',(-1.18233753211584,-24.5555791640676,-229.35005));
#199244=CARTESIAN_POINT('Origin',(-1.25,-25.3025207885872,-229.35005));
#199245=CARTESIAN_POINT('',(-1.18233753211584,-24.5555791640676,-192.281986444803));
#199246=CARTESIAN_POINT('Origin',(-1.25,-31.46456093117,-229.35005));
#199247=CARTESIAN_POINT('',(-1.25,-32.21456093117,-229.35005));
#199248=CARTESIAN_POINT('',(-1.25,-32.21456093117,-229.35005));
#199249=CARTESIAN_POINT('',(-0.5,-31.46456093117,-229.35005));
#199250=CARTESIAN_POINT('Origin',(-1.25,-31.46456093117,-229.35005));
#199251=CARTESIAN_POINT('',(-0.5,-31.46456093117,-235.35005));
#199252=CARTESIAN_POINT('Origin',(-8.87499999999984,-31.46456093117,-229.35005));
#199253=CARTESIAN_POINT('',(-9.62499999999984,-31.46456093117,-229.35005));
#199254=CARTESIAN_POINT('',(-9.62499999999984,-31.46456093117,-235.35005));
#199255=CARTESIAN_POINT('',(-8.87499999999984,-32.21456093117,-229.35005));
#199256=CARTESIAN_POINT('Origin',(-8.87499999999984,-31.46456093117,-229.35005));
#199257=CARTESIAN_POINT('',(-8.87499999999984,-32.21456093117,-229.35005));
#199258=CARTESIAN_POINT('Origin',(-31.625,21.5631368321642,-229.35005));
#199259=CARTESIAN_POINT('',(-31.625,20.8131368321642,-229.35005));
#199260=CARTESIAN_POINT('',(-31.625,20.8131368321642,-229.35005));
#199261=CARTESIAN_POINT('',(-30.875,21.5631368321642,-229.35005));
#199262=CARTESIAN_POINT('Origin',(-31.625,21.5631368321642,-229.35005));
#199263=CARTESIAN_POINT('',(-30.875,21.5631368321642,-235.35005));
#199264=CARTESIAN_POINT('Origin',(-33.751462642771,21.5631368321642,-229.35005));
#199265=CARTESIAN_POINT('',(-34.2872001450371,22.0880037949896,-229.35005));
#199266=CARTESIAN_POINT('',(-34.2872001450371,22.0880037949896,-229.35005));
#199267=CARTESIAN_POINT('',(-33.751462642771,20.8131368321642,-229.35005));
#199268=CARTESIAN_POINT('Origin',(-33.751462642771,21.5631368321642,-229.35005));
#199269=CARTESIAN_POINT('',(-33.751462642771,20.8131368321642,-229.35005));
#199270=CARTESIAN_POINT('Origin',(-31.625,23.6023848491226,-229.35005));
#199271=CARTESIAN_POINT('',(-30.875,23.6023848491226,-229.35005));
#199272=CARTESIAN_POINT('',(-32.1269841269841,24.1596208280901,-229.35005));
#199273=CARTESIAN_POINT('Origin',(-31.625,23.6023848491226,-229.35005));
#199274=CARTESIAN_POINT('',(-32.1269841269841,24.1596208280901,-229.35005));
#199275=CARTESIAN_POINT('',(-30.875,23.6023848491226,-229.35005));
#199276=CARTESIAN_POINT('Origin',(-29.125,19.0631368321642,-229.35005));
#199277=CARTESIAN_POINT('',(-29.125,19.8131368321642,-229.35005));
#199278=CARTESIAN_POINT('',(-29.125,19.8131368321642,-229.35005));
#199279=CARTESIAN_POINT('',(-29.875,19.0631368321642,-229.35005));
#199280=CARTESIAN_POINT('Origin',(-29.125,19.0631368321642,-229.35005));
#199281=CARTESIAN_POINT('',(-29.875,19.0631368321642,-235.35005));
#199282=CARTESIAN_POINT('Origin',(-21.5,19.0631368321642,-229.35005));
#199283=CARTESIAN_POINT('',(-20.75,19.0631368321642,-229.35005));
#199284=CARTESIAN_POINT('',(-20.75,19.0631368321642,-235.35005));
#199285=CARTESIAN_POINT('',(-21.5,19.8131368321642,-229.35005));
#199286=CARTESIAN_POINT('Origin',(-21.5,19.0631368321642,-229.35005));
#199287=CARTESIAN_POINT('',(-21.5,19.8131368321642,-229.35005));
#199288=CARTESIAN_POINT('Origin',(-21.5,10.9575972794973,-229.35005));
#199289=CARTESIAN_POINT('',(-21.5,10.2075972794973,-229.35005));
#199290=CARTESIAN_POINT('',(-21.5,10.2075972794973,-229.35005));
#199291=CARTESIAN_POINT('',(-20.75,10.9575972794973,-229.35005));
#199292=CARTESIAN_POINT('Origin',(-21.5,10.9575972794973,-229.35005));
#199293=CARTESIAN_POINT('',(-20.75,10.9575972794973,-235.35005));
#199294=CARTESIAN_POINT('Origin',(-29.125,10.9575972794973,-229.35005));
#199295=CARTESIAN_POINT('',(-29.875,10.9575972794973,-229.35005));
#199296=CARTESIAN_POINT('',(-29.875,10.9575972794973,-235.35005));
#199297=CARTESIAN_POINT('',(-29.125,10.2075972794973,-229.35005));
#199298=CARTESIAN_POINT('Origin',(-29.125,10.9575972794973,-229.35005));
#199299=CARTESIAN_POINT('',(-29.125,10.2075972794973,-229.35005));
#199300=CARTESIAN_POINT('Origin',(-29.125,8.45759727949731,-229.35005));
#199301=CARTESIAN_POINT('',(-29.125,9.20759727949731,-229.35005));
#199302=CARTESIAN_POINT('',(-29.125,9.20759727949731,-229.35005));
#199303=CARTESIAN_POINT('',(-29.875,8.45759727949731,-229.35005));
#199304=CARTESIAN_POINT('Origin',(-29.125,8.45759727949731,-229.35005));
#199305=CARTESIAN_POINT('',(-29.875,8.45759727949731,-235.35005));
#199306=CARTESIAN_POINT('Origin',(-21.5,8.45759727949731,-229.35005));
#199307=CARTESIAN_POINT('',(-20.75,8.45759727949731,-229.35005));
#199308=CARTESIAN_POINT('',(-20.75,8.45759727949731,-235.35005));
#199309=CARTESIAN_POINT('',(-21.5,9.20759727949731,-229.35005));
#199310=CARTESIAN_POINT('Origin',(-21.5,8.45759727949731,-229.35005));
#199311=CARTESIAN_POINT('',(-21.5,9.20759727949731,-229.35005));
#199312=CARTESIAN_POINT('Origin',(-21.5,0.35205772683049,-229.35005));
#199313=CARTESIAN_POINT('',(-21.5,-0.39794227316951,-229.35005));
#199314=CARTESIAN_POINT('',(-21.5,-0.39794227316951,-229.35005));
#199315=CARTESIAN_POINT('',(-20.75,0.352057726830487,-229.35005));
#199316=CARTESIAN_POINT('Origin',(-21.5,0.35205772683049,-229.35005));
#199317=CARTESIAN_POINT('',(-20.75,0.352057726830487,-235.35005));
#199318=CARTESIAN_POINT('Origin',(-29.125,0.352057726830493,-229.35005));
#199319=CARTESIAN_POINT('',(-29.875,0.352057726830494,-229.35005));
#199320=CARTESIAN_POINT('',(-29.875,0.352057726830494,-235.35005));
#199321=CARTESIAN_POINT('',(-29.125,-0.397942273169507,-229.35005));
#199322=CARTESIAN_POINT('Origin',(-29.125,0.352057726830493,-229.35005));
#199323=CARTESIAN_POINT('',(-29.125,-0.397942273169507,-229.35005));
#199324=CARTESIAN_POINT('Origin',(-29.125,-44.5701004838368,-229.35005));
#199325=CARTESIAN_POINT('',(-29.125,-43.8201004838368,-229.35005));
#199326=CARTESIAN_POINT('',(-29.125,-43.8201004838368,-229.35005));
#199327=CARTESIAN_POINT('',(-29.875,-44.5701004838368,-229.35005));
#199328=CARTESIAN_POINT('Origin',(-29.125,-44.5701004838368,-229.35005));
#199329=CARTESIAN_POINT('',(-29.875,-44.5701004838368,-235.35005));
#199330=CARTESIAN_POINT('Origin',(-21.5,-44.5701004838368,-229.35005));
#199331=CARTESIAN_POINT('',(-20.75,-44.5701004838368,-229.35005));
#199332=CARTESIAN_POINT('',(-20.75,-44.5701004838368,-235.35005));
#199333=CARTESIAN_POINT('',(-21.5,-43.8201004838368,-229.35005));
#199334=CARTESIAN_POINT('Origin',(-21.5,-44.5701004838368,-229.35005));
#199335=CARTESIAN_POINT('',(-21.5,-43.8201004838368,-229.35005));
#199336=CARTESIAN_POINT('Origin',(-21.5,-52.8339989151841,-229.35005));
#199337=CARTESIAN_POINT('',(-21.5238294101153,-53.5836202590728,-229.35005));
#199338=CARTESIAN_POINT('',(-21.5238294101154,-53.5836202590729,-229.35005));
#199339=CARTESIAN_POINT('',(-20.75,-52.8339989151841,-229.35005));
#199340=CARTESIAN_POINT('Origin',(-21.5,-52.8339989151841,-229.35005));
#199341=CARTESIAN_POINT('',(-20.75,-52.8339989151841,-235.35005));
#199342=CARTESIAN_POINT('Origin',(-29.125,-48.7096221120845,-229.35005));
#199343=CARTESIAN_POINT('',(-29.875,-48.7096221120845,-229.35005));
#199344=CARTESIAN_POINT('',(-29.875,-48.7096221120845,-229.35005));
#199345=CARTESIAN_POINT('',(-29.5873015873016,-49.3001957674217,-229.35005));
#199346=CARTESIAN_POINT('Origin',(-29.125,-48.7096221120845,-229.35005));
#199347=CARTESIAN_POINT('',(-29.5873015873016,-49.3001957674217,-229.35005));
#199348=CARTESIAN_POINT('Origin',(-31.625,-42.0701004838368,-229.35005));
#199349=CARTESIAN_POINT('',(-31.625,-42.8201004838368,-229.35005));
#199350=CARTESIAN_POINT('',(-31.625,-42.8201004838368,-229.35005));
#199351=CARTESIAN_POINT('',(-30.875,-42.0701004838368,-229.35005));
#199352=CARTESIAN_POINT('Origin',(-31.625,-42.0701004838368,-229.35005));
#199353=CARTESIAN_POINT('',(-30.875,-42.0701004838368,-235.35005));
#199354=CARTESIAN_POINT('Origin',(-36.0311576807678,-42.0701004838368,-229.35005));
#199355=CARTESIAN_POINT('',(-36.6030808185578,-42.5552849069797,-229.35005));
#199356=CARTESIAN_POINT('',(-36.6030808185578,-42.5552849069797,-229.35005));
#199357=CARTESIAN_POINT('',(-36.0311576807678,-42.8201004838368,-229.35005));
#199358=CARTESIAN_POINT('Origin',(-36.0311576807678,-42.0701004838368,-229.35005));
#199359=CARTESIAN_POINT('',(-36.0311576807678,-42.8201004838368,-229.35005));
#199360=CARTESIAN_POINT('Origin',(-39.3771239584772,-33.96456093117,-229.35005));
#199361=CARTESIAN_POINT('',(-39.3771239584772,-33.21456093117,-229.35005));
#199362=CARTESIAN_POINT('',(-39.3771239584772,-33.21456093117,-229.35005));
#199363=CARTESIAN_POINT('',(-40.1267106833091,-33.9894555481763,-229.35005));
#199364=CARTESIAN_POINT('Origin',(-39.3771239584772,-33.96456093117,-229.35005));
#199365=CARTESIAN_POINT('',(-40.1267106833092,-33.9894555481763,-229.35005));
#199366=CARTESIAN_POINT('Origin',(-31.625,-33.96456093117,-229.35005));
#199367=CARTESIAN_POINT('',(-30.875,-33.96456093117,-229.35005));
#199368=CARTESIAN_POINT('',(-30.875,-33.96456093117,-235.35005));
#199369=CARTESIAN_POINT('',(-31.625,-33.21456093117,-229.35005));
#199370=CARTESIAN_POINT('Origin',(-31.625,-33.96456093117,-229.35005));
#199371=CARTESIAN_POINT('',(-31.625,-33.21456093117,-229.35005));
#199372=CARTESIAN_POINT('Origin',(-29.125,-2.14794227316952,-229.35005));
#199373=CARTESIAN_POINT('',(-29.125,-1.39794227316951,-229.35005));
#199374=CARTESIAN_POINT('',(-29.125,-1.39794227316951,-229.35005));
#199375=CARTESIAN_POINT('',(-29.875,-2.14794227316951,-229.35005));
#199376=CARTESIAN_POINT('Origin',(-29.125,-2.14794227316952,-229.35005));
#199377=CARTESIAN_POINT('',(-29.875,-2.14794227316951,-235.35005));
#199378=CARTESIAN_POINT('Origin',(-21.5,-2.14794227316951,-229.35005));
#199379=CARTESIAN_POINT('',(-20.75,-2.14794227316951,-229.35005));
#199380=CARTESIAN_POINT('',(-20.75,-2.14794227316951,-235.35005));
#199381=CARTESIAN_POINT('',(-21.5,-1.39794227316951,-229.35005));
#199382=CARTESIAN_POINT('Origin',(-21.5,-2.14794227316951,-229.35005));
#199383=CARTESIAN_POINT('',(-21.5,-1.39794227316951,-229.35005));
#199384=CARTESIAN_POINT('Origin',(-21.5,-10.2534818258363,-229.35005));
#199385=CARTESIAN_POINT('',(-21.5,-11.0034818258363,-229.35005));
#199386=CARTESIAN_POINT('',(-21.5,-11.0034818258363,-229.35005));
#199387=CARTESIAN_POINT('',(-20.75,-10.2534818258363,-229.35005));
#199388=CARTESIAN_POINT('Origin',(-21.5,-10.2534818258363,-229.35005));
#199389=CARTESIAN_POINT('',(-20.75,-10.2534818258363,-235.35005));
#199390=CARTESIAN_POINT('Origin',(-29.125,-10.2534818258363,-229.35005));
#199391=CARTESIAN_POINT('',(-29.875,-10.2534818258363,-229.35005));
#199392=CARTESIAN_POINT('',(-29.875,-10.2534818258363,-235.35005));
#199393=CARTESIAN_POINT('',(-29.125,-11.0034818258363,-229.35005));
#199394=CARTESIAN_POINT('Origin',(-29.125,-10.2534818258363,-229.35005));
#199395=CARTESIAN_POINT('',(-29.125,-11.0034818258363,-229.35005));
#199396=CARTESIAN_POINT('Origin',(-29.125,-12.7534818258363,-229.35005));
#199397=CARTESIAN_POINT('',(-29.125,-12.0034818258363,-229.35005));
#199398=CARTESIAN_POINT('',(-29.125,-12.0034818258363,-229.35005));
#199399=CARTESIAN_POINT('',(-29.875,-12.7534818258363,-229.35005));
#199400=CARTESIAN_POINT('Origin',(-29.125,-12.7534818258363,-229.35005));
#199401=CARTESIAN_POINT('',(-29.875,-12.7534818258363,-235.35005));
#199402=CARTESIAN_POINT('Origin',(-21.5,-12.7534818258363,-229.35005));
#199403=CARTESIAN_POINT('',(-20.75,-12.7534818258363,-229.35005));
#199404=CARTESIAN_POINT('',(-20.75,-12.7534818258363,-235.35005));
#199405=CARTESIAN_POINT('',(-21.5,-12.0034818258363,-229.35005));
#199406=CARTESIAN_POINT('Origin',(-21.5,-12.7534818258363,-229.35005));
#199407=CARTESIAN_POINT('',(-21.5,-12.0034818258363,-229.35005));
#199408=CARTESIAN_POINT('Origin',(-21.5,-20.8590213785032,-229.35005));
#199409=CARTESIAN_POINT('',(-21.5,-21.6090213785031,-229.35005));
#199410=CARTESIAN_POINT('',(-21.5,-21.6090213785031,-229.35005));
#199411=CARTESIAN_POINT('',(-20.75,-20.8590213785032,-229.35005));
#199412=CARTESIAN_POINT('Origin',(-21.5,-20.8590213785032,-229.35005));
#199413=CARTESIAN_POINT('',(-20.75,-20.8590213785032,-235.35005));
#199414=CARTESIAN_POINT('Origin',(-29.125,-20.8590213785032,-229.35005));
#199415=CARTESIAN_POINT('',(-29.875,-20.8590213785032,-229.35005));
#199416=CARTESIAN_POINT('',(-29.875,-20.8590213785032,-235.35005));
#199417=CARTESIAN_POINT('',(-29.125,-21.6090213785031,-229.35005));
#199418=CARTESIAN_POINT('Origin',(-29.125,-20.8590213785032,-229.35005));
#199419=CARTESIAN_POINT('',(-29.125,-21.6090213785031,-229.35005));
#199420=CARTESIAN_POINT('Origin',(-29.125,-23.3590213785032,-229.35005));
#199421=CARTESIAN_POINT('',(-29.125,-22.6090213785032,-229.35005));
#199422=CARTESIAN_POINT('',(-29.125,-22.6090213785032,-229.35005));
#199423=CARTESIAN_POINT('',(-29.875,-23.3590213785032,-229.35005));
#199424=CARTESIAN_POINT('Origin',(-29.125,-23.3590213785032,-229.35005));
#199425=CARTESIAN_POINT('',(-29.875,-23.3590213785032,-235.35005));
#199426=CARTESIAN_POINT('Origin',(-21.5,-23.3590213785032,-229.35005));
#199427=CARTESIAN_POINT('',(-20.75,-23.3590213785032,-229.35005));
#199428=CARTESIAN_POINT('',(-20.75,-23.3590213785032,-235.35005));
#199429=CARTESIAN_POINT('',(-21.5,-22.6090213785032,-229.35005));
#199430=CARTESIAN_POINT('Origin',(-21.5,-23.3590213785032,-229.35005));
#199431=CARTESIAN_POINT('',(-21.5,-22.6090213785032,-229.35005));
#199432=CARTESIAN_POINT('Origin',(-21.5,-31.46456093117,-229.35005));
#199433=CARTESIAN_POINT('',(-21.5,-32.21456093117,-229.35005));
#199434=CARTESIAN_POINT('',(-21.5,-32.21456093117,-229.35005));
#199435=CARTESIAN_POINT('',(-20.75,-31.46456093117,-229.35005));
#199436=CARTESIAN_POINT('Origin',(-21.5,-31.46456093117,-229.35005));
#199437=CARTESIAN_POINT('',(-20.75,-31.46456093117,-235.35005));
#199438=CARTESIAN_POINT('Origin',(-29.125,-31.46456093117,-229.35005));
#199439=CARTESIAN_POINT('',(-29.875,-31.46456093117,-229.35005));
#199440=CARTESIAN_POINT('',(-29.875,-31.46456093117,-235.35005));
#199441=CARTESIAN_POINT('',(-29.125,-32.21456093117,-229.35005));
#199442=CARTESIAN_POINT('Origin',(-29.125,-31.46456093117,-229.35005));
#199443=CARTESIAN_POINT('',(-29.125,-32.21456093117,-229.35005));
#199444=CARTESIAN_POINT('Origin',(-31.625,-44.5701004838368,-229.35005));
#199445=CARTESIAN_POINT('',(-30.875,-44.5701004838368,-229.35005));
#199446=CARTESIAN_POINT('',(-30.875,-44.5701004838368,-235.35005));
#199447=CARTESIAN_POINT('',(-31.625,-43.8201004838368,-229.35005));
#199448=CARTESIAN_POINT('Origin',(-31.625,-44.5701004838368,-229.35005));
#199449=CARTESIAN_POINT('',(-31.625,-43.8201004838368,-229.35005));
#199450=CARTESIAN_POINT('Origin',(-31.625,-46.609348500795,-229.35005));
#199451=CARTESIAN_POINT('',(-32.1269841269841,-47.1665844797626,-229.35005));
#199452=CARTESIAN_POINT('',(-32.1269841269841,-47.1665844797626,-229.35005));
#199453=CARTESIAN_POINT('',(-30.875,-46.609348500795,-229.35005));
#199454=CARTESIAN_POINT('Origin',(-31.625,-46.609348500795,-229.35005));
#199455=CARTESIAN_POINT('',(-30.875,-46.609348500795,-235.35005));
#199456=CARTESIAN_POINT('Origin',(-33.7514626427707,-44.5701004838368,-229.35005));
#199457=CARTESIAN_POINT('',(-33.7514626427707,-43.8201004838368,-229.35005));
#199458=CARTESIAN_POINT('',(-33.7514626427707,-43.8201004838368,-229.35005));
#199459=CARTESIAN_POINT('',(-34.2872001450369,-45.0949674466622,-229.35005));
#199460=CARTESIAN_POINT('Origin',(-33.7514626427707,-44.5701004838368,-229.35005));
#199461=CARTESIAN_POINT('',(-34.2872001450369,-45.0949674466622,-229.35005));
#199462=CARTESIAN_POINT('Origin',(-29.125,-42.0701004838368,-229.35005));
#199463=CARTESIAN_POINT('',(-29.875,-42.0701004838368,-229.35005));
#199464=CARTESIAN_POINT('',(-29.875,-42.0701004838368,-235.35005));
#199465=CARTESIAN_POINT('',(-29.125,-42.8201004838368,-229.35005));
#199466=CARTESIAN_POINT('Origin',(-29.125,-42.0701004838368,-229.35005));
#199467=CARTESIAN_POINT('',(-29.125,-42.8201004838368,-229.35005));
#199468=CARTESIAN_POINT('Origin',(-29.125,-33.96456093117,-229.35005));
#199469=CARTESIAN_POINT('',(-29.125,-33.21456093117,-229.35005));
#199470=CARTESIAN_POINT('',(-29.125,-33.21456093117,-229.35005));
#199471=CARTESIAN_POINT('',(-29.875,-33.96456093117,-229.35005));
#199472=CARTESIAN_POINT('Origin',(-29.125,-33.96456093117,-229.35005));
#199473=CARTESIAN_POINT('',(-29.875,-33.96456093117,-235.35005));
#199474=CARTESIAN_POINT('Origin',(-21.5,-33.96456093117,-229.35005));
#199475=CARTESIAN_POINT('',(-20.75,-33.96456093117,-229.35005));
#199476=CARTESIAN_POINT('',(-20.75,-33.96456093117,-235.35005));
#199477=CARTESIAN_POINT('',(-21.5,-33.21456093117,-229.35005));
#199478=CARTESIAN_POINT('Origin',(-21.5,-33.96456093117,-229.35005));
#199479=CARTESIAN_POINT('',(-21.5,-33.21456093117,-229.35005));
#199480=CARTESIAN_POINT('Origin',(-21.5,-42.0701004838368,-229.35005));
#199481=CARTESIAN_POINT('',(-21.5,-42.8201004838368,-229.35005));
#199482=CARTESIAN_POINT('',(-21.5,-42.8201004838368,-229.35005));
#199483=CARTESIAN_POINT('',(-20.75,-42.0701004838368,-229.35005));
#199484=CARTESIAN_POINT('Origin',(-21.5,-42.0701004838368,-229.35005));
#199485=CARTESIAN_POINT('',(-20.75,-42.0701004838368,-235.35005));
#199486=CARTESIAN_POINT('Origin',(-31.625,-23.3590213785032,-229.35005));
#199487=CARTESIAN_POINT('',(-30.875,-23.3590213785032,-229.35005));
#199488=CARTESIAN_POINT('',(-30.875,-23.3590213785032,-235.35005));
#199489=CARTESIAN_POINT('',(-31.625,-22.6090213785032,-229.35005));
#199490=CARTESIAN_POINT('Origin',(-31.625,-23.3590213785032,-229.35005));
#199491=CARTESIAN_POINT('',(-31.625,-22.6090213785032,-229.35005));
#199492=CARTESIAN_POINT('Origin',(-31.625,-31.46456093117,-229.35005));
#199493=CARTESIAN_POINT('',(-31.625,-32.21456093117,-229.35005));
#199494=CARTESIAN_POINT('',(-31.625,-32.21456093117,-229.35005));
#199495=CARTESIAN_POINT('',(-30.875,-31.46456093117,-229.35005));
#199496=CARTESIAN_POINT('Origin',(-31.625,-31.46456093117,-229.35005));
#199497=CARTESIAN_POINT('',(-30.875,-31.46456093117,-235.35005));
#199498=CARTESIAN_POINT('Origin',(-39.4555265729267,-31.46456093117,-229.35005));
#199499=CARTESIAN_POINT('',(-40.2052001948773,-31.486684686535,-229.35005));
#199500=CARTESIAN_POINT('',(-40.2052001948774,-31.486684686535,-229.35005));
#199501=CARTESIAN_POINT('',(-39.4555265729267,-32.21456093117,-229.35005));
#199502=CARTESIAN_POINT('Origin',(-39.4555265729267,-31.46456093117,-229.35005));
#199503=CARTESIAN_POINT('',(-39.4555265729267,-32.21456093117,-229.35005));
#199504=CARTESIAN_POINT('Origin',(-39.6461373136998,-23.3590213785032,-229.35005));
#199505=CARTESIAN_POINT('',(-39.6461373136998,-22.6090213785032,-229.35005));
#199506=CARTESIAN_POINT('',(-39.6461373136998,-22.6090213785032,-229.35005));
#199507=CARTESIAN_POINT('',(-40.3960221980464,-23.3721614024167,-229.35005));
#199508=CARTESIAN_POINT('Origin',(-39.6461373136998,-23.3590213785032,-229.35005));
#199509=CARTESIAN_POINT('',(-40.3960221980465,-23.3721614024167,-229.35005));
#199510=CARTESIAN_POINT('Origin',(-31.625,-12.7534818258363,-229.35005));
#199511=CARTESIAN_POINT('',(-30.875,-12.7534818258363,-229.35005));
#199512=CARTESIAN_POINT('',(-30.875,-12.7534818258363,-235.35005));
#199513=CARTESIAN_POINT('',(-31.625,-12.0034818258363,-229.35005));
#199514=CARTESIAN_POINT('Origin',(-31.625,-12.7534818258363,-229.35005));
#199515=CARTESIAN_POINT('',(-31.625,-12.0034818258363,-229.35005));
#199516=CARTESIAN_POINT('Origin',(-31.625,-20.8590213785032,-229.35005));
#199517=CARTESIAN_POINT('',(-31.625,-21.6090213785031,-229.35005));
#199518=CARTESIAN_POINT('',(-31.625,-21.6090213785031,-229.35005));
#199519=CARTESIAN_POINT('',(-30.875,-20.8590213785032,-229.35005));
#199520=CARTESIAN_POINT('Origin',(-31.625,-20.8590213785032,-229.35005));
#199521=CARTESIAN_POINT('',(-30.875,-20.8590213785032,-235.35005));
#199522=CARTESIAN_POINT('Origin',(-39.6853241707135,-20.8590213785032,-229.35005));
#199523=CARTESIAN_POINT('',(-40.4352524876037,-20.8693905407753,-229.35005));
#199524=CARTESIAN_POINT('',(-40.4352524876037,-20.8693905407753,-229.35005));
#199525=CARTESIAN_POINT('',(-39.6853241707135,-21.6090213785031,-229.35005));
#199526=CARTESIAN_POINT('Origin',(-39.6853241707135,-20.8590213785032,-229.35005));
#199527=CARTESIAN_POINT('',(-39.6853241707135,-21.6090213785031,-229.35005));
#199528=CARTESIAN_POINT('Origin',(-39.7488454733312,-12.7534818258363,-229.35005));
#199529=CARTESIAN_POINT('',(-39.7488454733312,-12.0034818258363,-229.35005));
#199530=CARTESIAN_POINT('',(-39.7488454733312,-12.0034818258363,-229.35005));
#199531=CARTESIAN_POINT('',(-40.4988441937178,-12.754867256657,-229.35005));
#199532=CARTESIAN_POINT('Origin',(-39.7488454733312,-12.7534818258363,-229.35005));
#199533=CARTESIAN_POINT('',(-40.4988441937178,-12.754867256657,-229.35005));
#199534=CARTESIAN_POINT('Origin',(-31.625,-2.14794227316952,-229.35005));
#199535=CARTESIAN_POINT('',(-30.875,-2.14794227316951,-229.35005));
#199536=CARTESIAN_POINT('',(-30.875,-2.14794227316951,-235.35005));
#199537=CARTESIAN_POINT('',(-31.625,-1.39794227316951,-229.35005));
#199538=CARTESIAN_POINT('Origin',(-31.625,-2.14794227316952,-229.35005));
#199539=CARTESIAN_POINT('',(-31.625,-1.39794227316951,-229.35005));
#199540=CARTESIAN_POINT('Origin',(-31.625,-10.2534818258363,-229.35005));
#199541=CARTESIAN_POINT('',(-31.625,-11.0034818258363,-229.35005));
#199542=CARTESIAN_POINT('',(-31.625,-11.0034818258363,-229.35005));
#199543=CARTESIAN_POINT('',(-30.875,-10.2534818258363,-229.35005));
#199544=CARTESIAN_POINT('Origin',(-31.625,-10.2534818258363,-229.35005));
#199545=CARTESIAN_POINT('',(-30.875,-10.2534818258363,-235.35005));
#199546=CARTESIAN_POINT('Origin',(-39.7488454733312,-10.2534818258363,-229.35005));
#199547=CARTESIAN_POINT('',(-40.4988441937178,-10.2520963950157,-229.35005));
#199548=CARTESIAN_POINT('',(-40.4988441937178,-10.2520963950157,-229.35005));
#199549=CARTESIAN_POINT('',(-39.7488454733312,-11.0034818258363,-229.35005));
#199550=CARTESIAN_POINT('Origin',(-39.7488454733312,-10.2534818258363,-229.35005));
#199551=CARTESIAN_POINT('',(-39.7488454733312,-11.0034818258363,-229.35005));
#199552=CARTESIAN_POINT('Origin',(-39.6853241707135,-2.14794227316952,-229.35005));
#199553=CARTESIAN_POINT('',(-39.6853241707135,-1.39794227316952,-229.35005));
#199554=CARTESIAN_POINT('',(-39.6853241707135,-1.39794227316952,-229.35005));
#199555=CARTESIAN_POINT('',(-40.4352524876037,-2.13757311089736,-229.35005));
#199556=CARTESIAN_POINT('Origin',(-39.6853241707135,-2.14794227316952,-229.35005));
#199557=CARTESIAN_POINT('',(-40.4352524876037,-2.13757311089736,-229.35005));
#199558=CARTESIAN_POINT('Origin',(-31.625,8.45759727949731,-229.35005));
#199559=CARTESIAN_POINT('',(-30.875,8.45759727949731,-229.35005));
#199560=CARTESIAN_POINT('',(-30.875,8.45759727949731,-235.35005));
#199561=CARTESIAN_POINT('',(-31.625,9.20759727949731,-229.35005));
#199562=CARTESIAN_POINT('Origin',(-31.625,8.45759727949731,-229.35005));
#199563=CARTESIAN_POINT('',(-31.625,9.20759727949731,-229.35005));
#199564=CARTESIAN_POINT('Origin',(-31.625,0.352057726830494,-229.35005));
#199565=CARTESIAN_POINT('',(-31.625,-0.397942273169506,-229.35005));
#199566=CARTESIAN_POINT('',(-31.625,-0.397942273169506,-229.35005));
#199567=CARTESIAN_POINT('',(-30.875,0.352057726830494,-229.35005));
#199568=CARTESIAN_POINT('Origin',(-31.625,0.352057726830494,-229.35005));
#199569=CARTESIAN_POINT('',(-30.875,0.352057726830494,-235.35005));
#199570=CARTESIAN_POINT('Origin',(-39.6461373136998,0.352057726830498,-229.35005));
#199571=CARTESIAN_POINT('',(-40.3960221980465,0.365197750743975,-229.35005));
#199572=CARTESIAN_POINT('',(-40.3960221980464,0.365197750743973,-229.35005));
#199573=CARTESIAN_POINT('',(-39.6461373136998,-0.397942273169503,-229.35005));
#199574=CARTESIAN_POINT('Origin',(-39.6461373136998,0.352057726830498,-229.35005));
#199575=CARTESIAN_POINT('',(-39.6461373136998,-0.397942273169503,-229.35005));
#199576=CARTESIAN_POINT('Origin',(-39.4555265729267,8.45759727949731,-229.35005));
#199577=CARTESIAN_POINT('',(-39.4555265729267,9.20759727949731,-229.35005));
#199578=CARTESIAN_POINT('',(-39.4555265729267,9.20759727949731,-229.35005));
#199579=CARTESIAN_POINT('',(-40.2052001948774,8.47972103486228,-229.35005));
#199580=CARTESIAN_POINT('Origin',(-39.4555265729267,8.45759727949731,-229.35005));
#199581=CARTESIAN_POINT('',(-40.2052001948774,8.47972103486227,-229.35005));
#199582=CARTESIAN_POINT('Origin',(-31.625,19.0631368321642,-229.35005));
#199583=CARTESIAN_POINT('',(-30.875,19.0631368321642,-229.35005));
#199584=CARTESIAN_POINT('',(-30.875,19.0631368321642,-235.35005));
#199585=CARTESIAN_POINT('',(-31.625,19.8131368321642,-229.35005));
#199586=CARTESIAN_POINT('Origin',(-31.625,19.0631368321642,-229.35005));
#199587=CARTESIAN_POINT('',(-31.625,19.8131368321642,-229.35005));
#199588=CARTESIAN_POINT('Origin',(-31.625,10.9575972794973,-229.35005));
#199589=CARTESIAN_POINT('',(-31.625,10.2075972794973,-229.35005));
#199590=CARTESIAN_POINT('',(-31.625,10.2075972794973,-229.35005));
#199591=CARTESIAN_POINT('',(-30.875,10.9575972794973,-229.35005));
#199592=CARTESIAN_POINT('Origin',(-31.625,10.9575972794973,-229.35005));
#199593=CARTESIAN_POINT('',(-30.875,10.9575972794973,-235.35005));
#199594=CARTESIAN_POINT('Origin',(-39.3771239584772,10.9575972794973,-229.35005));
#199595=CARTESIAN_POINT('',(-40.1267106833092,10.9824918965036,-229.35005));
#199596=CARTESIAN_POINT('',(-40.1267106833092,10.9824918965036,-229.35005));
#199597=CARTESIAN_POINT('',(-39.3771239584772,10.2075972794973,-229.35005));
#199598=CARTESIAN_POINT('Origin',(-39.3771239584772,10.9575972794973,-229.35005));
#199599=CARTESIAN_POINT('',(-39.3771239584772,10.2075972794973,-229.35005));
#199600=CARTESIAN_POINT('Origin',(-36.0311576807679,19.0631368321642,-229.35005));
#199601=CARTESIAN_POINT('',(-36.0311576807679,19.8131368321642,-229.35005));
#199602=CARTESIAN_POINT('',(-36.0311576807679,19.8131368321642,-229.35005));
#199603=CARTESIAN_POINT('',(-36.6030808185579,19.548321255307,-229.35005));
#199604=CARTESIAN_POINT('Origin',(-36.0311576807679,19.0631368321642,-229.35005));
#199605=CARTESIAN_POINT('',(-36.6030808185579,19.548321255307,-229.35005));
#199606=CARTESIAN_POINT('Origin',(-29.125,21.5631368321642,-229.35005));
#199607=CARTESIAN_POINT('',(-29.875,21.5631368321642,-229.35005));
#199608=CARTESIAN_POINT('',(-29.875,21.5631368321642,-235.35005));
#199609=CARTESIAN_POINT('',(-29.125,20.8131368321642,-229.35005));
#199610=CARTESIAN_POINT('Origin',(-29.125,21.5631368321642,-229.35005));
#199611=CARTESIAN_POINT('',(-29.125,20.8131368321642,-229.35005));
#199612=CARTESIAN_POINT('Origin',(-29.125,25.702658460412,-229.35005));
#199613=CARTESIAN_POINT('',(-29.5873015873016,26.2932321157492,-229.35005));
#199614=CARTESIAN_POINT('',(-29.5873015873016,26.2932321157492,-229.35005));
#199615=CARTESIAN_POINT('',(-29.875,25.702658460412,-229.35005));
#199616=CARTESIAN_POINT('Origin',(-29.125,25.702658460412,-229.35005));
#199617=CARTESIAN_POINT('',(-29.875,25.702658460412,-235.35005));
#199618=CARTESIAN_POINT('Origin',(-21.5,29.0311209585238,-229.35005));
#199619=CARTESIAN_POINT('',(-20.75,29.0311209585238,-229.35005));
#199620=CARTESIAN_POINT('',(-21.5791427781145,29.776933549375,-229.35005));
#199621=CARTESIAN_POINT('Origin',(-21.5,29.0311209585238,-229.35005));
#199622=CARTESIAN_POINT('',(-21.5791427781145,29.7769335493751,-229.35005));
#199623=CARTESIAN_POINT('',(-20.75,29.0311209585238,-229.35005));
#199624=CARTESIAN_POINT('Origin',(-21.5,21.5631368321642,-229.35005));
#199625=CARTESIAN_POINT('',(-21.5,20.8131368321642,-229.35005));
#199626=CARTESIAN_POINT('',(-21.5,20.8131368321642,-229.35005));
#199627=CARTESIAN_POINT('',(-20.75,21.5631368321642,-229.35005));
#199628=CARTESIAN_POINT('Origin',(-21.5,21.5631368321642,-229.35005));
#199629=CARTESIAN_POINT('',(-20.75,21.5631368321642,-235.35005));
#199630=CARTESIAN_POINT('Origin',(-19.,-52.9088458284789,-229.35005));
#199631=CARTESIAN_POINT('',(-19.75,-52.9088458284789,-229.35005));
#199632=CARTESIAN_POINT('',(-19.75,-52.9088458284789,-229.35005));
#199633=CARTESIAN_POINT('',(-19.021058548474,-53.658550128544,-229.35005));
#199634=CARTESIAN_POINT('Origin',(-19.,-52.9088458284789,-229.35005));
#199635=CARTESIAN_POINT('',(-19.021058548474,-53.6585501285442,-229.35005));
#199636=CARTESIAN_POINT('Origin',(-19.,-44.5701004838368,-229.35005));
#199637=CARTESIAN_POINT('',(-19.,-43.8201004838368,-229.35005));
#199638=CARTESIAN_POINT('',(-19.,-43.8201004838368,-229.35005));
#199639=CARTESIAN_POINT('',(-19.75,-44.5701004838368,-229.35005));
#199640=CARTESIAN_POINT('Origin',(-19.,-44.5701004838368,-229.35005));
#199641=CARTESIAN_POINT('',(-19.75,-44.5701004838368,-235.35005));
#199642=CARTESIAN_POINT('Origin',(-11.3749999999999,-44.5701004838369,-229.35005));
#199643=CARTESIAN_POINT('',(-10.6249999999999,-44.5701004838369,-229.35005));
#199644=CARTESIAN_POINT('',(-10.6249999999999,-44.5701004838369,-235.35005));
#199645=CARTESIAN_POINT('',(-11.3749999999999,-43.8201004838368,-229.35005));
#199646=CARTESIAN_POINT('Origin',(-11.3749999999999,-44.5701004838369,-229.35005));
#199647=CARTESIAN_POINT('',(-11.3749999999999,-43.8201004838368,-229.35005));
#199648=CARTESIAN_POINT('Origin',(-11.3749999999999,-53.08002700974,-229.35005));
#199649=CARTESIAN_POINT('',(-11.3876074204679,-53.8299210375528,-229.35005));
#199650=CARTESIAN_POINT('',(-11.3876074204679,-53.8299210375529,-229.35005));
#199651=CARTESIAN_POINT('',(-10.6249999999999,-53.08002700974,-229.35005));
#199652=CARTESIAN_POINT('Origin',(-11.3749999999999,-53.08002700974,-229.35005));
#199653=CARTESIAN_POINT('',(-10.6249999999999,-53.08002700974,-235.35005));
#199654=CARTESIAN_POINT('Origin',(-19.,19.0631368321642,-229.35005));
#199655=CARTESIAN_POINT('',(-19.,19.8131368321642,-229.35005));
#199656=CARTESIAN_POINT('',(-19.,19.8131368321642,-229.35005));
#199657=CARTESIAN_POINT('',(-19.75,19.0631368321642,-229.35005));
#199658=CARTESIAN_POINT('Origin',(-19.,19.0631368321642,-229.35005));
#199659=CARTESIAN_POINT('',(-19.75,19.0631368321642,-235.35005));
#199660=CARTESIAN_POINT('Origin',(-11.3749999999999,19.0631368321642,-229.35005));
#199661=CARTESIAN_POINT('',(-10.6249999999999,19.0631368321642,-229.35005));
#199662=CARTESIAN_POINT('',(-10.6249999999999,19.0631368321642,-235.35005));
#199663=CARTESIAN_POINT('',(-11.3749999999999,19.8131368321642,-229.35005));
#199664=CARTESIAN_POINT('Origin',(-11.3749999999999,19.0631368321642,-229.35005));
#199665=CARTESIAN_POINT('',(-11.3749999999999,19.8131368321642,-229.35005));
#199666=CARTESIAN_POINT('Origin',(-11.3749999999999,10.9575972794973,-229.35005));
#199667=CARTESIAN_POINT('',(-11.3749999999999,10.2075972794973,-229.35005));
#199668=CARTESIAN_POINT('',(-11.3749999999999,10.2075972794973,-229.35005));
#199669=CARTESIAN_POINT('',(-10.6249999999999,10.9575972794973,-229.35005));
#199670=CARTESIAN_POINT('Origin',(-11.3749999999999,10.9575972794973,-229.35005));
#199671=CARTESIAN_POINT('',(-10.6249999999999,10.9575972794973,-235.35005));
#199672=CARTESIAN_POINT('Origin',(-19.,10.9575972794973,-229.35005));
#199673=CARTESIAN_POINT('',(-19.75,10.9575972794973,-229.35005));
#199674=CARTESIAN_POINT('',(-19.75,10.9575972794973,-235.35005));
#199675=CARTESIAN_POINT('',(-19.,10.2075972794973,-229.35005));
#199676=CARTESIAN_POINT('Origin',(-19.,10.9575972794973,-229.35005));
#199677=CARTESIAN_POINT('',(-19.,10.2075972794973,-229.35005));
#199678=CARTESIAN_POINT('Origin',(-19.,8.45759727949731,-229.35005));
#199679=CARTESIAN_POINT('',(-19.,9.20759727949731,-229.35005));
#199680=CARTESIAN_POINT('',(-19.,9.20759727949731,-229.35005));
#199681=CARTESIAN_POINT('',(-19.75,8.45759727949731,-229.35005));
#199682=CARTESIAN_POINT('Origin',(-19.,8.45759727949731,-229.35005));
#199683=CARTESIAN_POINT('',(-19.75,8.45759727949731,-235.35005));
#199684=CARTESIAN_POINT('Origin',(-11.3749999999999,8.45759727949731,-229.35005));
#199685=CARTESIAN_POINT('',(-10.6249999999999,8.45759727949731,-229.35005));
#199686=CARTESIAN_POINT('',(-10.6249999999999,8.45759727949731,-235.35005));
#199687=CARTESIAN_POINT('',(-11.3749999999999,9.20759727949731,-229.35005));
#199688=CARTESIAN_POINT('Origin',(-11.3749999999999,8.45759727949731,-229.35005));
#199689=CARTESIAN_POINT('',(-11.3749999999999,9.20759727949731,-229.35005));
#199690=CARTESIAN_POINT('Origin',(-11.3749999999999,0.352057726830486,-229.35005));
#199691=CARTESIAN_POINT('',(-11.3749999999999,-0.397942273169514,-229.35005));
#199692=CARTESIAN_POINT('',(-11.3749999999999,-0.397942273169514,-229.35005));
#199693=CARTESIAN_POINT('',(-10.6249999999999,0.352057726830487,-229.35005));
#199694=CARTESIAN_POINT('Origin',(-11.3749999999999,0.352057726830486,-229.35005));
#199695=CARTESIAN_POINT('',(-10.6249999999999,0.352057726830487,-235.35005));
#199696=CARTESIAN_POINT('Origin',(-19.,0.352057726830489,-229.35005));
#199697=CARTESIAN_POINT('',(-19.75,0.352057726830487,-229.35005));
#199698=CARTESIAN_POINT('',(-19.75,0.352057726830487,-235.35005));
#199699=CARTESIAN_POINT('',(-19.,-0.397942273169511,-229.35005));
#199700=CARTESIAN_POINT('Origin',(-19.,0.352057726830489,-229.35005));
#199701=CARTESIAN_POINT('',(-19.,-0.397942273169511,-229.35005));
#199702=CARTESIAN_POINT('Origin',(-19.,-23.3590213785032,-229.35005));
#199703=CARTESIAN_POINT('',(-19.,-22.6090213785032,-229.35005));
#199704=CARTESIAN_POINT('',(-19.,-22.6090213785032,-229.35005));
#199705=CARTESIAN_POINT('',(-19.75,-23.3590213785032,-229.35005));
#199706=CARTESIAN_POINT('Origin',(-19.,-23.3590213785032,-229.35005));
#199707=CARTESIAN_POINT('',(-19.75,-23.3590213785032,-235.35005));
#199708=CARTESIAN_POINT('Origin',(-11.3749999999999,-23.3590213785032,-229.35005));
#199709=CARTESIAN_POINT('',(-10.6249999999999,-23.3590213785032,-229.35005));
#199710=CARTESIAN_POINT('',(-10.6249999999999,-23.3590213785032,-235.35005));
#199711=CARTESIAN_POINT('',(-11.3749999999999,-22.6090213785032,-229.35005));
#199712=CARTESIAN_POINT('Origin',(-11.3749999999999,-23.3590213785032,-229.35005));
#199713=CARTESIAN_POINT('',(-11.3749999999999,-22.6090213785032,-229.35005));
#199714=CARTESIAN_POINT('Origin',(-11.3749999999999,-31.46456093117,-229.35005));
#199715=CARTESIAN_POINT('',(-11.3749999999999,-32.21456093117,-229.35005));
#199716=CARTESIAN_POINT('',(-11.3749999999999,-32.21456093117,-229.35005));
#199717=CARTESIAN_POINT('',(-10.6249999999999,-31.46456093117,-229.35005));
#199718=CARTESIAN_POINT('Origin',(-11.3749999999999,-31.46456093117,-229.35005));
#199719=CARTESIAN_POINT('',(-10.6249999999999,-31.46456093117,-235.35005));
#199720=CARTESIAN_POINT('Origin',(-19.,-31.46456093117,-229.35005));
#199721=CARTESIAN_POINT('',(-19.75,-31.46456093117,-229.35005));
#199722=CARTESIAN_POINT('',(-19.75,-31.46456093117,-235.35005));
#199723=CARTESIAN_POINT('',(-19.,-32.21456093117,-229.35005));
#199724=CARTESIAN_POINT('Origin',(-19.,-31.46456093117,-229.35005));
#199725=CARTESIAN_POINT('',(-19.,-32.21456093117,-229.35005));
#199726=CARTESIAN_POINT('Origin',(-19.,-42.0701004838368,-229.35005));
#199727=CARTESIAN_POINT('',(-19.75,-42.0701004838368,-229.35005));
#199728=CARTESIAN_POINT('',(-19.75,-42.0701004838368,-235.35005));
#199729=CARTESIAN_POINT('',(-19.,-42.8201004838368,-229.35005));
#199730=CARTESIAN_POINT('Origin',(-19.,-42.0701004838368,-229.35005));
#199731=CARTESIAN_POINT('',(-19.,-42.8201004838368,-229.35005));
#199732=CARTESIAN_POINT('Origin',(-19.,-33.96456093117,-229.35005));
#199733=CARTESIAN_POINT('',(-19.,-33.21456093117,-229.35005));
#199734=CARTESIAN_POINT('',(-19.,-33.21456093117,-229.35005));
#199735=CARTESIAN_POINT('',(-19.75,-33.96456093117,-229.35005));
#199736=CARTESIAN_POINT('Origin',(-19.,-33.96456093117,-229.35005));
#199737=CARTESIAN_POINT('',(-19.75,-33.96456093117,-235.35005));
#199738=CARTESIAN_POINT('Origin',(-11.3749999999999,-33.96456093117,-229.35005));
#199739=CARTESIAN_POINT('',(-10.6249999999999,-33.96456093117,-229.35005));
#199740=CARTESIAN_POINT('',(-10.6249999999999,-33.96456093117,-235.35005));
#199741=CARTESIAN_POINT('',(-11.3749999999999,-33.21456093117,-229.35005));
#199742=CARTESIAN_POINT('Origin',(-11.3749999999999,-33.96456093117,-229.35005));
#199743=CARTESIAN_POINT('',(-11.3749999999999,-33.21456093117,-229.35005));
#199744=CARTESIAN_POINT('Origin',(-11.3749999999999,-42.0701004838369,-229.35005));
#199745=CARTESIAN_POINT('',(-11.3749999999999,-42.8201004838369,-229.35005));
#199746=CARTESIAN_POINT('',(-11.3749999999999,-42.8201004838369,-229.35005));
#199747=CARTESIAN_POINT('',(-10.6249999999999,-42.0701004838368,-229.35005));
#199748=CARTESIAN_POINT('Origin',(-11.3749999999999,-42.0701004838369,-229.35005));
#199749=CARTESIAN_POINT('',(-10.6249999999999,-42.0701004838368,-235.35005));
#199750=CARTESIAN_POINT('Origin',(-19.,21.5631368321642,-229.35005));
#199751=CARTESIAN_POINT('',(-19.75,21.5631368321642,-229.35005));
#199752=CARTESIAN_POINT('',(-19.75,21.5631368321642,-235.35005));
#199753=CARTESIAN_POINT('',(-19.,20.8131368321642,-229.35005));
#199754=CARTESIAN_POINT('Origin',(-19.,21.5631368321642,-229.35005));
#199755=CARTESIAN_POINT('',(-19.,20.8131368321642,-229.35005));
#199756=CARTESIAN_POINT('Origin',(-19.,29.2808336449858,-229.35005));
#199757=CARTESIAN_POINT('',(-19.0699401294965,30.0275654430807,-229.35005));
#199758=CARTESIAN_POINT('',(-19.0699401294965,30.0275654430807,-229.35005));
#199759=CARTESIAN_POINT('',(-19.75,29.2808336449858,-229.35005));
#199760=CARTESIAN_POINT('Origin',(-19.,29.2808336449858,-229.35005));
#199761=CARTESIAN_POINT('',(-19.75,29.2808336449858,-235.35005));
#199762=CARTESIAN_POINT('Origin',(-11.3749999999999,29.8508988479304,-229.35005));
#199763=CARTESIAN_POINT('',(-10.6249999999999,29.8508988479304,-229.35005));
#199764=CARTESIAN_POINT('',(-11.4168720512116,30.5997290899261,-229.35005));
#199765=CARTESIAN_POINT('Origin',(-11.3749999999999,29.8508988479304,-229.35005));
#199766=CARTESIAN_POINT('',(-11.4168720512116,30.5997290899261,-229.35005));
#199767=CARTESIAN_POINT('',(-10.6249999999999,29.8508988479304,-229.35005));
#199768=CARTESIAN_POINT('Origin',(-11.3749999999999,21.5631368321642,-229.35005));
#199769=CARTESIAN_POINT('',(-11.3749999999999,20.8131368321642,-229.35005));
#199770=CARTESIAN_POINT('',(-11.3749999999999,20.8131368321642,-229.35005));
#199771=CARTESIAN_POINT('',(-10.6249999999999,21.5631368321642,-229.35005));
#199772=CARTESIAN_POINT('Origin',(-11.3749999999999,21.5631368321642,-229.35005));
#199773=CARTESIAN_POINT('',(-10.6249999999999,21.5631368321642,-235.35005));
#199774=CARTESIAN_POINT('Origin',(-8.87499999999984,-53.1174378937751,-229.35005));
#199775=CARTESIAN_POINT('',(-9.62499999999984,-53.1174378937751,-229.35005));
#199776=CARTESIAN_POINT('',(-9.62499999999984,-53.1174378937751,-229.35005));
#199777=CARTESIAN_POINT('',(-8.88483655882654,-53.8673733857413,-229.35005));
#199778=CARTESIAN_POINT('Origin',(-8.87499999999984,-53.1174378937751,-229.35005));
#199779=CARTESIAN_POINT('',(-8.88483655882654,-53.8673733857413,-229.35005));
#199780=CARTESIAN_POINT('Origin',(-8.87499999999984,-44.5701004838369,-229.35005));
#199781=CARTESIAN_POINT('',(-8.87499999999984,-43.8201004838368,-229.35005));
#199782=CARTESIAN_POINT('',(-8.87499999999984,-43.8201004838368,-229.35005));
#199783=CARTESIAN_POINT('',(-9.62499999999984,-44.5701004838369,-229.35005));
#199784=CARTESIAN_POINT('Origin',(-8.87499999999984,-44.5701004838369,-229.35005));
#199785=CARTESIAN_POINT('',(-9.62499999999984,-44.5701004838369,-235.35005));
#199786=CARTESIAN_POINT('Origin',(-1.25,-44.5701004838369,-229.35005));
#199787=CARTESIAN_POINT('',(-0.5,-44.5701004838369,-229.35005));
#199788=CARTESIAN_POINT('',(-0.5,-44.5701004838369,-235.35005));
#199789=CARTESIAN_POINT('',(-1.25,-43.8201004838368,-229.35005));
#199790=CARTESIAN_POINT('Origin',(-1.25,-44.5701004838369,-229.35005));
#199791=CARTESIAN_POINT('',(-1.25,-43.8201004838368,-229.35005));
#199792=CARTESIAN_POINT('Origin',(-1.25,-53.1744855098348,-229.35005));
#199793=CARTESIAN_POINT('',(-1.25138543082066,-53.9244842302215,-229.35005));
#199794=CARTESIAN_POINT('',(-1.25138543082066,-53.9244842302215,-229.35005));
#199795=CARTESIAN_POINT('',(-0.5,-53.1744855098348,-229.35005));
#199796=CARTESIAN_POINT('Origin',(-1.25,-53.1744855098348,-229.35005));
#199797=CARTESIAN_POINT('',(-0.5,-53.1744855098348,-235.35005));
#199798=CARTESIAN_POINT('Origin',(-8.87499999999986,19.0631368321642,-229.35005));
#199799=CARTESIAN_POINT('',(-8.87499999999986,19.8131368321642,-229.35005));
#199800=CARTESIAN_POINT('',(-8.87499999999986,19.8131368321642,-229.35005));
#199801=CARTESIAN_POINT('',(-9.62499999999986,19.0631368321642,-229.35005));
#199802=CARTESIAN_POINT('Origin',(-8.87499999999986,19.0631368321642,-229.35005));
#199803=CARTESIAN_POINT('',(-9.62499999999986,19.0631368321642,-235.35005));
#199804=CARTESIAN_POINT('Origin',(-1.25,19.0631368321642,-229.35005));
#199805=CARTESIAN_POINT('',(-0.5,19.0631368321642,-229.35005));
#199806=CARTESIAN_POINT('',(-0.5,19.0631368321642,-235.35005));
#199807=CARTESIAN_POINT('',(-1.25,19.8131368321642,-229.35005));
#199808=CARTESIAN_POINT('Origin',(-1.25,19.0631368321642,-229.35005));
#199809=CARTESIAN_POINT('',(-1.25,19.8131368321642,-229.35005));
#199810=CARTESIAN_POINT('Origin',(-1.25,10.9575972794973,-229.35005));
#199811=CARTESIAN_POINT('',(-1.25,10.2075972794973,-229.35005));
#199812=CARTESIAN_POINT('',(-1.25,10.2075972794973,-229.35005));
#199813=CARTESIAN_POINT('',(-0.5,10.9575972794973,-229.35005));
#199814=CARTESIAN_POINT('Origin',(-1.25,10.9575972794973,-229.35005));
#199815=CARTESIAN_POINT('',(-0.5,10.9575972794973,-235.35005));
#199816=CARTESIAN_POINT('Origin',(-8.87499999999986,10.9575972794973,-229.35005));
#199817=CARTESIAN_POINT('',(-9.62499999999986,10.9575972794973,-229.35005));
#199818=CARTESIAN_POINT('',(-9.62499999999986,10.9575972794973,-235.35005));
#199819=CARTESIAN_POINT('',(-8.87499999999986,10.2075972794973,-229.35005));
#199820=CARTESIAN_POINT('Origin',(-8.87499999999986,10.9575972794973,-229.35005));
#199821=CARTESIAN_POINT('',(-8.87499999999986,10.2075972794973,-229.35005));
#199822=CARTESIAN_POINT('Origin',(-8.87499999999984,-42.0701004838369,-229.35005));
#199823=CARTESIAN_POINT('',(-9.62499999999984,-42.0701004838368,-229.35005));
#199824=CARTESIAN_POINT('',(-9.62499999999984,-42.0701004838368,-235.35005));
#199825=CARTESIAN_POINT('',(-8.87499999999984,-42.8201004838369,-229.35005));
#199826=CARTESIAN_POINT('Origin',(-8.87499999999984,-42.0701004838369,-229.35005));
#199827=CARTESIAN_POINT('',(-8.87499999999984,-42.8201004838369,-229.35005));
#199828=CARTESIAN_POINT('Origin',(-8.87499999999984,-33.96456093117,-229.35005));
#199829=CARTESIAN_POINT('',(-8.87499999999984,-33.21456093117,-229.35005));
#199830=CARTESIAN_POINT('',(-8.87499999999984,-33.21456093117,-229.35005));
#199831=CARTESIAN_POINT('',(-9.62499999999984,-33.96456093117,-229.35005));
#199832=CARTESIAN_POINT('Origin',(-8.87499999999984,-33.96456093117,-229.35005));
#199833=CARTESIAN_POINT('',(-9.62499999999984,-33.96456093117,-235.35005));
#199834=CARTESIAN_POINT('Origin',(-1.25,-33.96456093117,-229.35005));
#199835=CARTESIAN_POINT('',(-0.5,-33.96456093117,-229.35005));
#199836=CARTESIAN_POINT('',(-0.5,-33.96456093117,-235.35005));
#199837=CARTESIAN_POINT('',(-1.25,-33.21456093117,-229.35005));
#199838=CARTESIAN_POINT('Origin',(-1.25,-33.96456093117,-229.35005));
#199839=CARTESIAN_POINT('',(-1.25,-33.21456093117,-229.35005));
#199840=CARTESIAN_POINT('Origin',(-1.25,-42.0701004838369,-229.35005));
#199841=CARTESIAN_POINT('',(-1.25,-42.8201004838369,-229.35005));
#199842=CARTESIAN_POINT('',(-1.25,-42.8201004838369,-229.35005));
#199843=CARTESIAN_POINT('',(-0.5,-42.0701004838369,-229.35005));
#199844=CARTESIAN_POINT('Origin',(-1.25,-42.0701004838369,-229.35005));
#199845=CARTESIAN_POINT('',(-0.5,-42.0701004838369,-235.35005));
#199846=CARTESIAN_POINT('Origin',(-8.87499999999986,21.5631368321642,-229.35005));
#199847=CARTESIAN_POINT('',(-9.62499999999986,21.5631368321642,-229.35005));
#199848=CARTESIAN_POINT('',(-9.62499999999986,21.5631368321642,-235.35005));
#199849=CARTESIAN_POINT('',(-8.87499999999986,20.8131368321642,-229.35005));
#199850=CARTESIAN_POINT('Origin',(-8.87499999999986,21.5631368321642,-229.35005));
#199851=CARTESIAN_POINT('',(-8.87499999999986,20.8131368321642,-229.35005));
#199852=CARTESIAN_POINT('Origin',(-8.87499999999986,29.9752906431998,-229.35005));
#199853=CARTESIAN_POINT('',(-8.90766940259363,30.7245787787886,-229.35005));
#199854=CARTESIAN_POINT('',(-8.90766940259363,30.7245787787886,-229.35005));
#199855=CARTESIAN_POINT('',(-9.62499999999986,29.9752906431998,-229.35005));
#199856=CARTESIAN_POINT('Origin',(-8.87499999999986,29.9752906431998,-229.35005));
#199857=CARTESIAN_POINT('',(-9.62499999999986,29.9752906431998,-235.35005));
#199858=CARTESIAN_POINT('Origin',(-1.25,30.1648419118246,-229.35005));
#199859=CARTESIAN_POINT('',(-0.5,30.1648419118246,-229.35005));
#199860=CARTESIAN_POINT('',(-1.25460132430898,30.9148277969016,-229.35005));
#199861=CARTESIAN_POINT('Origin',(-1.25,30.1648419118246,-229.35005));
#199862=CARTESIAN_POINT('',(-1.25460132430898,30.9148277969016,-229.35005));
#199863=CARTESIAN_POINT('',(-0.5,30.1648419118246,-229.35005));
#199864=CARTESIAN_POINT('Origin',(-1.25,21.5631368321642,-229.35005));
#199865=CARTESIAN_POINT('',(-1.25,20.8131368321642,-229.35005));
#199866=CARTESIAN_POINT('',(-1.25,20.8131368321642,-229.35005));
#199867=CARTESIAN_POINT('',(-0.5,21.5631368321642,-229.35005));
#199868=CARTESIAN_POINT('Origin',(-1.25,21.5631368321642,-229.35005));
#199869=CARTESIAN_POINT('',(-0.5,21.5631368321642,-235.35005));
#199870=CARTESIAN_POINT('Origin',(-7.99493453126771,-18.0851397679958,-192.281986444803));
#199871=CARTESIAN_POINT('',(-8.57396770167423,-18.5618163748993,-229.35005));
#199872=CARTESIAN_POINT('',(-8.57396770167423,-18.5618163748993,-192.281986444803));
#199873=CARTESIAN_POINT('',(-7.4518492428487,-18.6024002144856,-229.35005));
#199874=CARTESIAN_POINT('Origin',(-7.99493453126771,-18.0851397679958,-229.35005));
#199875=CARTESIAN_POINT('',(-7.4518492428487,-18.6024002144856,-235.35005));
#199876=CARTESIAN_POINT('Origin',(-6.18465023653768,-19.8093412562951,-192.281986444803));
#199877=CARTESIAN_POINT('',(-6.72773552495669,-19.2920808098054,-229.35005));
#199878=CARTESIAN_POINT('',(-6.72773552495669,-19.2920808098054,-229.35005));
#199879=CARTESIAN_POINT('',(-6.63257355852516,-20.4108931639637,-229.35005));
#199880=CARTESIAN_POINT('Origin',(-6.18465023653768,-19.8093412562951,-229.35005));
#199881=CARTESIAN_POINT('',(-6.63257355852516,-20.4108931639637,-192.281986444803));
#199882=CARTESIAN_POINT('Origin',(-6.18465023653769,-3.19762239537749,-192.281986444803));
#199883=CARTESIAN_POINT('',(-6.63257355852517,-2.59607048770891,-229.35005));
#199884=CARTESIAN_POINT('',(-6.63257355852517,-2.59607048770891,-192.281986444803));
#199885=CARTESIAN_POINT('',(-6.7277355249567,-3.7148828418673,-229.35005));
#199886=CARTESIAN_POINT('Origin',(-6.18465023653769,-3.19762239537748,-229.35005));
#199887=CARTESIAN_POINT('',(-6.7277355249567,-3.7148828418673,-192.281986444803));
#199888=CARTESIAN_POINT('Origin',(-1.25,-1.22366181637858,-192.281986444803));
#199889=CARTESIAN_POINT('',(-0.5,-1.22366181637858,-229.35005));
#199890=CARTESIAN_POINT('',(-1.3405312557817,-0.479145804645729,-229.35005));
#199891=CARTESIAN_POINT('Origin',(-1.25,-1.22366181637858,-229.35005));
#199892=CARTESIAN_POINT('',(-1.3405312557817,-0.479145804645732,-192.281986444803));
#199893=CARTESIAN_POINT('',(-0.5,-1.22366181637858,-229.35005));
#199894=CARTESIAN_POINT('Origin',(-1.25,-21.7833018352941,-192.281986444803));
#199895=CARTESIAN_POINT('',(-1.3405312557817,-22.5278178470269,-229.35005));
#199896=CARTESIAN_POINT('',(-1.3405312557817,-22.5278178470269,-192.281986444803));
#199897=CARTESIAN_POINT('',(-0.5,-21.7833018352941,-229.35005));
#199898=CARTESIAN_POINT('Origin',(-1.25,-21.7833018352941,-229.35005));
#199899=CARTESIAN_POINT('',(-0.5,-21.7833018352941,-235.35005));
#199900=CARTESIAN_POINT('Origin',(-5.14120077283693,-18.713796339242,-192.281986444803));
#199901=CARTESIAN_POINT('',(-4.7057783396023,-18.1031349726598,-229.35005));
#199902=CARTESIAN_POINT('',(-5.68428606125594,-18.1965358927522,-229.35005));
#199903=CARTESIAN_POINT('Origin',(-5.14120077283693,-18.713796339242,-229.35005));
#199904=CARTESIAN_POINT('',(-5.68428606125594,-18.1965358927522,-192.281986444803));
#199905=CARTESIAN_POINT('',(-4.7057783396023,-18.1031349726598,-192.281986444803));
#199906=CARTESIAN_POINT('Origin',(-6.95148506756696,-16.9895948509426,-192.281986444803));
#199907=CARTESIAN_POINT('',(-6.40839977914796,-17.5068552974324,-229.35005));
#199908=CARTESIAN_POINT('',(-6.40839977914795,-17.5068552974324,-192.281986444803));
#199909=CARTESIAN_POINT('',(-6.36274467860837,-16.5249608504553,-229.35005));
#199910=CARTESIAN_POINT('Origin',(-6.95148506756696,-16.9895948509426,-229.35005));
#199911=CARTESIAN_POINT('',(-6.36274467860837,-16.5249608504553,-192.281986444803));
#199912=CARTESIAN_POINT('Origin',(-20.625,-3.54959888009691,-192.281986444803));
#199913=CARTESIAN_POINT('',(-11.294759518486,-7.14773903260897,-229.35005));
#199914=CARTESIAN_POINT('',(-11.294759518486,-7.14773903260897,-192.281986444803));
#199915=CARTESIAN_POINT('',(-10.6249999999999,-3.54959888009691,-229.35005));
#199916=CARTESIAN_POINT('Origin',(-20.625,-3.54959888009691,-229.35005));
#199917=CARTESIAN_POINT('',(-10.6249999999999,-3.54959888009691,-235.35005));
#199918=CARTESIAN_POINT('Origin',(-20.625,-19.4573647715757,-192.281986444803));
#199919=CARTESIAN_POINT('',(-10.6249999999999,-19.4573647715757,-229.35005));
#199920=CARTESIAN_POINT('',(-10.6249999999999,-19.4573647715757,-235.35005));
#199921=CARTESIAN_POINT('',(-11.294759518486,-15.8592246190636,-229.35005));
#199922=CARTESIAN_POINT('Origin',(-20.625,-19.4573647715757,-229.35005));
#199923=CARTESIAN_POINT('',(-11.294759518486,-15.8592246190636,-192.281986444803));
#199924=CARTESIAN_POINT('Origin',(-9.40330570654103,-32.6090213785032,-192.281986444803));
#199925=CARTESIAN_POINT('',(-5.33358654455951,-23.474614668563,-229.35005));
#199926=CARTESIAN_POINT('',(-5.33358654455951,-23.474614668563,-192.281986444803));
#199927=CARTESIAN_POINT('Origin',(-9.40330570654103,-32.6090213785032,-229.35005));
#199928=CARTESIAN_POINT('Origin',(-9.40330570654115,9.60205772683048,-192.281986444803));
#199929=CARTESIAN_POINT('',(-5.33358654455957,0.46765101689032,-229.35005));
#199930=CARTESIAN_POINT('Origin',(-9.40330570654115,9.60205772683049,-229.35005));
#199931=CARTESIAN_POINT('',(-5.33358654455957,0.467651016890315,-192.281986444803));
#199932=CARTESIAN_POINT('Origin',(0.,-11.5034818258363,-192.281986444803));
#199933=CARTESIAN_POINT('Origin',(0.,-11.5034818258363,-229.35005));
#199934=CARTESIAN_POINT('Origin',(0.,-11.5034818258363,-192.281986444803));
#199935=CARTESIAN_POINT('Origin',(0.,-11.5034818258363,-229.35005));
#199936=CARTESIAN_POINT('Origin',(0.,-11.5034818258363,-192.281986444803));
#199937=CARTESIAN_POINT('Origin',(0.,-11.5034818258363,-229.35005));
#199938=CARTESIAN_POINT('Origin',(6.10697827817036,-5.81657868152891,-192.281986444803));
#199939=CARTESIAN_POINT('',(6.10697827817036,-5.81657868152891,-229.35005));
#199940=CARTESIAN_POINT('Origin',(5.38286456027835,-5.12689808620917,-192.281986444803));
#199941=CARTESIAN_POINT('',(5.38286456027835,-5.12689808620916,-229.35005));
#199942=CARTESIAN_POINT('Origin',(0.,-11.5034818258363,-192.281986444803));
#199943=CARTESIAN_POINT('Origin',(0.,-11.5034818258363,-229.35005));
#199944=CARTESIAN_POINT('Origin',(0.,-11.5034818258363,-192.281986444803));
#199945=CARTESIAN_POINT('Origin',(0.,-11.5034818258363,-229.35005));
#199946=CARTESIAN_POINT('Origin',(0.,-11.5034818258363,-192.281986444803));
#199947=CARTESIAN_POINT('Origin',(0.,-11.5034818258363,-229.35005));
#199948=CARTESIAN_POINT('Origin',(-5.38286456027834,-5.12689808620917,-192.281986444803));
#199949=CARTESIAN_POINT('',(-5.38286456027834,-5.12689808620916,-229.35005));
#199950=CARTESIAN_POINT('Origin',(-6.10697827817035,-5.81657868152891,-192.281986444803));
#199951=CARTESIAN_POINT('',(-6.10697827817035,-5.81657868152891,-229.35005));
#199952=CARTESIAN_POINT('Origin',(0.,-11.5034818258363,-192.281986444803));
#199953=CARTESIAN_POINT('Origin',(0.,-11.5034818258363,-229.35005));
#199954=CARTESIAN_POINT('Origin',(0.,-11.5034818258363,-192.281986444803));
#199955=CARTESIAN_POINT('Origin',(0.,-11.5034818258363,-229.35005));
#199956=CARTESIAN_POINT('Origin',(-29.875,26.0662450163965,-235.35005));
#199957=CARTESIAN_POINT('',(-29.875,26.0662450163965,-229.35005));
#199958=CARTESIAN_POINT('Origin',(-30.875,26.0662450163965,-235.35005));
#199959=CARTESIAN_POINT('',(-30.875,26.0662450163965,-229.35005));
#199960=CARTESIAN_POINT('Origin',(-30.875,26.0662450163965,-235.35005));
#199961=CARTESIAN_POINT('',(-30.875,26.0662450163965,-229.35005));
#199962=CARTESIAN_POINT('Origin',(-29.875,26.0662450163965,-235.35005));
#199963=CARTESIAN_POINT('',(-29.875,26.0662450163965,-229.35005));
#199964=CARTESIAN_POINT('Origin',(-30.875,26.0662450163965,-235.35005));
#199965=CARTESIAN_POINT('',(-30.875,26.0662450163965,-229.35005));
#199966=CARTESIAN_POINT('Origin',(-29.875,26.0662450163965,-235.35005));
#199967=CARTESIAN_POINT('',(-29.875,26.0662450163965,-229.35005));
#199968=CARTESIAN_POINT('Origin',(-30.875,26.0662450163965,-235.35005));
#199969=CARTESIAN_POINT('',(-30.875,26.0662450163965,-229.35005));
#199970=CARTESIAN_POINT('Origin',(-29.875,26.0662450163965,-235.35005));
#199971=CARTESIAN_POINT('',(-29.875,26.0662450163965,-229.35005));
#199972=CARTESIAN_POINT('Origin',(-30.875,26.0662450163965,-235.35005));
#199973=CARTESIAN_POINT('',(-30.875,26.0662450163965,-229.35005));
#199974=CARTESIAN_POINT('Origin',(-29.875,26.0662450163965,-235.35005));
#199975=CARTESIAN_POINT('',(-29.875,26.0662450163965,-229.35005));
#199976=CARTESIAN_POINT('Origin',(-30.875,26.0662450163965,-235.35005));
#199977=CARTESIAN_POINT('',(-30.875,26.0662450163965,-229.35005));
#199978=CARTESIAN_POINT('Origin',(-29.875,26.0662450163965,-235.35005));
#199979=CARTESIAN_POINT('',(-29.875,26.0662450163965,-229.35005));
#199980=CARTESIAN_POINT('Origin',(-30.875,26.0662450163965,-235.35005));
#199981=CARTESIAN_POINT('',(-30.875,26.0662450163965,-229.35005));
#199982=CARTESIAN_POINT('Origin',(-29.875,26.0662450163965,-235.35005));
#199983=CARTESIAN_POINT('',(-29.875,26.0662450163965,-229.35005));
#199984=CARTESIAN_POINT('Origin',(-30.875,26.0662450163965,-235.35005));
#199985=CARTESIAN_POINT('',(-30.875,26.0662450163965,-229.35005));
#199986=CARTESIAN_POINT('Origin',(-29.875,26.0662450163965,-235.35005));
#199987=CARTESIAN_POINT('',(-29.875,26.0662450163965,-229.35005));
#199988=CARTESIAN_POINT('Origin',(-19.75,32.818676384831,-235.35005));
#199989=CARTESIAN_POINT('',(-19.75,32.818676384831,-229.35005));
#199990=CARTESIAN_POINT('Origin',(-20.75,32.818676384831,-235.35005));
#199991=CARTESIAN_POINT('',(-20.75,32.818676384831,-229.35005));
#199992=CARTESIAN_POINT('Origin',(-20.75,32.818676384831,-235.35005));
#199993=CARTESIAN_POINT('',(-20.75,32.818676384831,-229.35005));
#199994=CARTESIAN_POINT('Origin',(-19.75,32.818676384831,-235.35005));
#199995=CARTESIAN_POINT('',(-19.75,32.818676384831,-229.35005));
#199996=CARTESIAN_POINT('Origin',(-20.75,32.818676384831,-235.35005));
#199997=CARTESIAN_POINT('',(-20.75,32.818676384831,-229.35005));
#199998=CARTESIAN_POINT('Origin',(-19.75,32.818676384831,-235.35005));
#199999=CARTESIAN_POINT('',(-19.75,32.818676384831,-229.35005));
#200000=CARTESIAN_POINT('Origin',(-20.75,32.818676384831,-235.35005));
#200001=CARTESIAN_POINT('',(-20.75,32.818676384831,-229.35005));
#200002=CARTESIAN_POINT('Origin',(-19.75,32.818676384831,-235.35005));
#200003=CARTESIAN_POINT('',(-19.75,32.818676384831,-229.35005));
#200004=CARTESIAN_POINT('Origin',(-20.75,32.818676384831,-235.35005));
#200005=CARTESIAN_POINT('',(-20.75,32.818676384831,-229.35005));
#200006=CARTESIAN_POINT('Origin',(-19.75,32.818676384831,-235.35005));
#200007=CARTESIAN_POINT('',(-19.75,32.818676384831,-229.35005));
#200008=CARTESIAN_POINT('Origin',(-20.75,32.818676384831,-235.35005));
#200009=CARTESIAN_POINT('',(-20.75,32.818676384831,-229.35005));
#200010=CARTESIAN_POINT('Origin',(-19.75,32.818676384831,-235.35005));
#200011=CARTESIAN_POINT('',(-19.75,32.818676384831,-229.35005));
#200012=CARTESIAN_POINT('Origin',(-20.75,32.818676384831,-235.35005));
#200013=CARTESIAN_POINT('',(-20.75,32.818676384831,-229.35005));
#200014=CARTESIAN_POINT('Origin',(-19.75,32.818676384831,-235.35005));
#200015=CARTESIAN_POINT('',(-19.75,32.818676384831,-229.35005));
#200016=CARTESIAN_POINT('Origin',(-20.75,32.818676384831,-235.35005));
#200017=CARTESIAN_POINT('',(-20.75,32.818676384831,-229.35005));
#200018=CARTESIAN_POINT('Origin',(-19.75,32.818676384831,-235.35005));
#200019=CARTESIAN_POINT('',(-19.75,32.818676384831,-229.35005));
#200020=CARTESIAN_POINT('Origin',(-20.75,32.818676384831,-235.35005));
#200021=CARTESIAN_POINT('',(-20.75,32.818676384831,-232.25005));
#200022=CARTESIAN_POINT('',(-20.75,32.818676384831,-229.35005));
#200023=CARTESIAN_POINT('',(-20.75,32.818676384831,-235.35005));
#200024=CARTESIAN_POINT('',(-19.75,32.818676384831,-229.35005));
#200025=CARTESIAN_POINT('',(-20.75,32.818676384831,-229.35005));
#200026=CARTESIAN_POINT('',(-19.75,32.818676384831,-232.25005));
#200027=CARTESIAN_POINT('',(-19.75,32.818676384831,-235.35005));
#200028=CARTESIAN_POINT('',(-11.4589044897296,32.818676384831,-232.25005));
#200029=CARTESIAN_POINT('Origin',(-20.75,32.818676384831,-235.35005));
#200030=CARTESIAN_POINT('',(-20.75,32.3760227311709,-232.25005));
#200031=CARTESIAN_POINT('',(-20.75,32.3760227311709,-229.35005));
#200032=CARTESIAN_POINT('',(-20.75,32.3760227311709,-229.35005));
#200033=CARTESIAN_POINT('',(-20.75,32.818676384831,-229.35005));
#200034=CARTESIAN_POINT('',(-20.75,-32.0203896799758,-232.25005));
#200035=CARTESIAN_POINT('Origin',(-19.75,32.818676384831,-235.35005));
#200036=CARTESIAN_POINT('',(-19.75,32.4743226583832,-229.35005));
#200037=CARTESIAN_POINT('',(-19.75,32.818676384831,-229.35005));
#200038=CARTESIAN_POINT('',(-19.75,32.4743226583831,-232.25005));
#200039=CARTESIAN_POINT('',(-19.75,32.4743226583832,-229.35005));
#200040=CARTESIAN_POINT('',(-19.75,-32.0203896799758,-232.25005));
#200041=CARTESIAN_POINT('Origin',(-9.62499999999986,32.818676384831,-235.35005));
#200042=CARTESIAN_POINT('',(-9.62499999999986,32.818676384831,-229.35005));
#200043=CARTESIAN_POINT('Origin',(-10.6249999999999,32.818676384831,-235.35005));
#200044=CARTESIAN_POINT('',(-10.6249999999999,32.818676384831,-229.35005));
#200045=CARTESIAN_POINT('Origin',(-10.6249999999999,32.818676384831,-235.35005));
#200046=CARTESIAN_POINT('',(-10.6249999999999,32.818676384831,-229.35005));
#200047=CARTESIAN_POINT('Origin',(-9.62499999999986,32.818676384831,-235.35005));
#200048=CARTESIAN_POINT('',(-9.62499999999986,32.818676384831,-229.35005));
#200049=CARTESIAN_POINT('Origin',(-10.6249999999999,32.818676384831,-235.35005));
#200050=CARTESIAN_POINT('',(-10.6249999999999,32.818676384831,-229.35005));
#200051=CARTESIAN_POINT('Origin',(-9.62499999999986,32.818676384831,-235.35005));
#200052=CARTESIAN_POINT('',(-9.62499999999986,32.818676384831,-229.35005));
#200053=CARTESIAN_POINT('Origin',(-10.6249999999999,32.818676384831,-235.35005));
#200054=CARTESIAN_POINT('',(-10.6249999999999,32.818676384831,-229.35005));
#200055=CARTESIAN_POINT('Origin',(-9.62499999999986,32.818676384831,-235.35005));
#200056=CARTESIAN_POINT('',(-9.62499999999986,32.818676384831,-229.35005));
#200057=CARTESIAN_POINT('Origin',(-10.6249999999999,32.818676384831,-235.35005));
#200058=CARTESIAN_POINT('',(-10.6249999999999,32.818676384831,-229.35005));
#200059=CARTESIAN_POINT('Origin',(-10.6249999999999,32.818676384831,-235.35005));
#200060=CARTESIAN_POINT('',(-10.6249999999999,32.818676384831,-229.35005));
#200061=CARTESIAN_POINT('Origin',(-10.6249999999999,32.818676384831,-235.35005));
#200062=CARTESIAN_POINT('',(-10.6249999999999,32.818676384831,-229.35005));
#200063=CARTESIAN_POINT('Origin',(-9.62499999999986,32.818676384831,-235.35005));
#200064=CARTESIAN_POINT('',(-9.62499999999986,32.818676384831,-229.35005));
#200065=CARTESIAN_POINT('Origin',(-10.6249999999999,32.818676384831,-235.35005));
#200066=CARTESIAN_POINT('',(-10.6249999999999,32.818676384831,-229.35005));
#200067=CARTESIAN_POINT('Origin',(-9.62499999999986,32.818676384831,-235.35005));
#200068=CARTESIAN_POINT('',(-9.62499999999986,32.818676384831,-229.35005));
#200069=CARTESIAN_POINT('Origin',(-0.5,32.818676384831,-235.35005));
#200070=CARTESIAN_POINT('',(-0.5,32.818676384831,-229.35005));
#200071=CARTESIAN_POINT('Origin',(-0.5,32.818676384831,-235.35005));
#200072=CARTESIAN_POINT('',(-0.5,32.818676384831,-229.35005));
#200073=CARTESIAN_POINT('Origin',(-0.5,32.818676384831,-235.35005));
#200074=CARTESIAN_POINT('',(-0.5,32.818676384831,-229.35005));
#200075=CARTESIAN_POINT('Origin',(-0.5,32.818676384831,-235.35005));
#200076=CARTESIAN_POINT('',(-0.5,32.818676384831,-229.35005));
#200077=CARTESIAN_POINT('Origin',(-0.5,32.818676384831,-235.35005));
#200078=CARTESIAN_POINT('',(-0.5,32.818676384831,-229.35005));
#200079=CARTESIAN_POINT('Origin',(-0.5,32.818676384831,-235.35005));
#200080=CARTESIAN_POINT('',(-0.5,32.818676384831,-229.35005));
#200081=CARTESIAN_POINT('Origin',(-0.5,32.818676384831,-235.35005));
#200082=CARTESIAN_POINT('',(-0.5,32.818676384831,-229.35005));
#200083=CARTESIAN_POINT('Origin',(-0.5,32.818676384831,-235.35005));
#200084=CARTESIAN_POINT('',(-0.5,32.818676384831,-229.35005));
#200085=CARTESIAN_POINT('Origin',(-24.838300653577,28.3971299569735,-229.35005));
#200086=CARTESIAN_POINT('',(-25.2655040598954,31.8709602996399,-229.35005));
#200087=CARTESIAN_POINT('',(-25.2655040598954,31.8709602996399,-232.25005));
#200088=CARTESIAN_POINT('',(-25.2655040598954,31.8709602996399,-229.35005));
#200089=CARTESIAN_POINT('',(-26.6879613405455,31.3684521110126,-232.25005));
#200090=CARTESIAN_POINT('Origin',(-24.838300653577,28.3971299569735,-232.25005));
#200091=CARTESIAN_POINT('',(-26.6879613405455,31.3684521110126,-229.35005));
#200092=CARTESIAN_POINT('',(-26.6879613405455,31.3684521110126,-229.35005));
#200093=CARTESIAN_POINT('Origin',(-24.838300653577,28.3971299569735,-229.35005));
#200094=CARTESIAN_POINT('Origin',(6.29739814579425E-15,-11.5034818258363,
-229.35005));
#200095=CARTESIAN_POINT('',(-41.8942895912773,16.6943638302095,-232.25005));
#200096=CARTESIAN_POINT('Origin',(6.29739814579425E-15,-11.5034818258363,
-232.25005));
#200097=CARTESIAN_POINT('',(-41.8942895912773,16.6943638302095,-229.35005));
#200098=CARTESIAN_POINT('',(-41.8942895912773,16.6943638302095,-229.35005));
#200099=CARTESIAN_POINT('Origin',(6.29739814579425E-15,-11.5034818258363,
-229.35005));
#200100=CARTESIAN_POINT('Origin',(-38.9907249661392,14.740057695632,-229.35005));
#200101=CARTESIAN_POINT('',(-42.4880898820539,14.8758466676788,-232.25005));
#200102=CARTESIAN_POINT('Origin',(-38.9907249661392,14.740057695632,-232.25005));
#200103=CARTESIAN_POINT('',(-42.4880898820539,14.8758466676788,-229.35005));
#200104=CARTESIAN_POINT('',(-42.4880898820538,14.8758466676788,-229.35005));
#200105=CARTESIAN_POINT('Origin',(-38.9907249661392,14.740057695632,-229.35005));
#200106=CARTESIAN_POINT('Origin',(636.934816028482,-11.5034818258361,-229.35005));
#200107=CARTESIAN_POINT('',(-42.4880898820539,-37.8828103193509,-232.25005));
#200108=CARTESIAN_POINT('Origin',(636.934816028482,-11.5034818258361,-232.25005));
#200109=CARTESIAN_POINT('',(-42.4880898820538,-37.8828103193512,-229.35005));
#200110=CARTESIAN_POINT('',(-42.4880898820539,-37.8828103193507,-229.35005));
#200111=CARTESIAN_POINT('Origin',(636.934816028482,-11.5034818258361,-229.35005));
#200112=CARTESIAN_POINT('Origin',(-38.9907249661392,-37.7470213473046,-229.35005));
#200113=CARTESIAN_POINT('',(-41.8942895912772,-39.701327481882,-232.25005));
#200114=CARTESIAN_POINT('Origin',(-38.9907249661392,-37.7470213473046,-232.25005));
#200115=CARTESIAN_POINT('',(-41.8942895912772,-39.701327481882,-229.35005));
#200116=CARTESIAN_POINT('',(-41.8942895912772,-39.701327481882,-229.35005));
#200117=CARTESIAN_POINT('Origin',(-38.9907249661392,-37.7470213473046,-229.35005));
#200118=CARTESIAN_POINT('Origin',(6.29739814579425E-15,-11.5034818258363,
-229.35005));
#200119=CARTESIAN_POINT('',(-24.6244543289934,-55.593007214519,-232.25005));
#200120=CARTESIAN_POINT('Origin',(6.29739814579425E-15,-11.5034818258363,
-232.25005));
#200121=CARTESIAN_POINT('',(-24.6244543289934,-55.593007214519,-229.35005));
#200122=CARTESIAN_POINT('',(-24.6244543289934,-55.593007214519,-229.35005));
#200123=CARTESIAN_POINT('Origin',(6.29739814579425E-15,-11.5034818258363,
-229.35005));
#200124=CARTESIAN_POINT('Origin',(-22.9178089794592,-52.5372975341153,-229.35005));
#200125=CARTESIAN_POINT('',(-23.036390000908,-56.0352881775208,-232.25005));
#200126=CARTESIAN_POINT('Origin',(-22.9178089794592,-52.5372975341153,-232.25005));
#200127=CARTESIAN_POINT('',(-23.0363900009079,-56.0352881775207,-229.35005));
#200128=CARTESIAN_POINT('',(-23.036390000908,-56.0352881775208,-229.35005));
#200129=CARTESIAN_POINT('Origin',(-22.9178089794592,-52.5372975341153,-229.35005));
#200130=CARTESIAN_POINT('Origin',(-0.127542579976414,-12.8706479699377,
-225.85005));
#200131=CARTESIAN_POINT('',(-45.4582832513426,-55.6286989103146,-225.85004999954));
#200132=CARTESIAN_POINT('',(-46.0196463796681,-56.2008156187296,-225.85005));
#200133=CARTESIAN_POINT('',(-1.84775995058105,-11.1827640290625,-225.85005));
#200134=CARTESIAN_POINT('',(-42.5792116384512,-59.576583500476,-225.85005));
#200135=CARTESIAN_POINT('Origin',(-48.1334350484927,-61.7961505568785,-225.85005));
#200136=CARTESIAN_POINT('',(-41.9650064389658,-58.9506113934371,-225.850044661983));
#200137=CARTESIAN_POINT('',(1.59267479062803,-14.5585319108126,-225.85005));
#200138=CARTESIAN_POINT('Ctrl Pts',(-45.4582832505119,-55.6286989095207,
-225.85005));
#200139=CARTESIAN_POINT('Ctrl Pts',(-44.9107918876255,-56.2015386026923,
-225.85005));
#200140=CARTESIAN_POINT('Ctrl Pts',(-44.349042231461,-56.7629778840832,
-225.85005));
#200141=CARTESIAN_POINT('Ctrl Pts',(-43.1825099491978,-57.8740631734374,
-225.85005));
#200142=CARTESIAN_POINT('Ctrl Pts',(-42.578325837185,-58.4209877839039,
-225.85005));
#200143=CARTESIAN_POINT('Ctrl Pts',(-41.9650009328216,-58.9506050170295,
-225.85005));
#200144=CARTESIAN_POINT('Origin',(-53.4203077633109,-63.7432454966418,-228.35005));
#200145=CARTESIAN_POINT('',(-46.030027498998,-56.2113956007998,-225.073027461918));
#200146=CARTESIAN_POINT('Ctrl Pts',(-46.030027499018,-56.2113956008005,
-225.073027461933));
#200147=CARTESIAN_POINT('Ctrl Pts',(-45.9347321456546,-56.1142747513013,
-225.202538647974));
#200148=CARTESIAN_POINT('Ctrl Pts',(-45.8394511612794,-56.0171685460456,
-225.332029751687));
#200149=CARTESIAN_POINT('Ctrl Pts',(-45.6488607659844,-55.8229271644452,
-225.591049471117));
#200150=CARTESIAN_POINT('Ctrl Pts',(-45.5535783484286,-55.7258194985544,
-225.720541401809));
#200151=CARTESIAN_POINT('Ctrl Pts',(-45.4582832511563,-55.6286989100522,
-225.850049999207));
#200152=CARTESIAN_POINT('',(-46.0300271011815,-56.2113951953429,-225.073057235855));
#200153=CARTESIAN_POINT('Origin',(-0.128459562639233,-12.6359082483571,
-225.85005));
#200154=CARTESIAN_POINT('',(-43.3207863665692,34.1152634411122,-225.85005));
#200155=CARTESIAN_POINT('',(-43.7661191577225,33.2092653453444,-225.850049986044));
#200156=CARTESIAN_POINT('Origin',(-48.892180948596,36.2913696007177,-225.85005));
#200157=CARTESIAN_POINT('',(-43.0713417429913,33.8649821651551,-225.850049999629));
#200158=CARTESIAN_POINT('Ctrl Pts',(-43.7661189699064,33.2092654881215,
-225.85005));
#200159=CARTESIAN_POINT('Ctrl Pts',(-43.6513378416623,33.3196167357978,
-225.85005));
#200160=CARTESIAN_POINT('Ctrl Pts',(-43.536034293583,33.4294426364236,-225.85005));
#200161=CARTESIAN_POINT('Ctrl Pts',(-43.3044413536273,33.6480087459458,
-225.85005));
#200162=CARTESIAN_POINT('Ctrl Pts',(-43.188133837425,33.7567660993298,-225.85005));
#200163=CARTESIAN_POINT('Ctrl Pts',(-43.0713417424048,33.8649821645222,
-225.85005));
#200164=CARTESIAN_POINT('',(-50.4030915963197,41.2213231498315,-225.85005));
#200165=CARTESIAN_POINT('Origin',(-50.4030915963197,41.2213231498315,-228.35005));
#200166=CARTESIAN_POINT('',(-43.3259173910555,34.1204116753589,-225.468974352258));
#200167=CARTESIAN_POINT('Ctrl Pts',(-43.3259173910559,34.1204116753647,
-225.468974352262));
#200168=CARTESIAN_POINT('Ctrl Pts',(-43.2834889553441,34.07784093212,-225.532489881091));
#200169=CARTESIAN_POINT('Ctrl Pts',(-43.2410614098359,34.0352710820648,
-225.59600200373));
#200170=CARTESIAN_POINT('Ctrl Pts',(-43.1562018220031,33.9501268700554,
-225.723028788387));
#200171=CARTESIAN_POINT('Ctrl Pts',(-43.1137729119589,33.9075556508875,
-225.786538761693));
#200172=CARTESIAN_POINT('Ctrl Pts',(-43.0713417427678,33.8649821649953,
-225.850049999372));
#200173=CARTESIAN_POINT('',(-43.3259171707406,34.1204114543102,-225.468990713749));
#200174=CARTESIAN_POINT('Origin',(-48.982196043432,-44.3222432618617,-167.906149834141));
#200175=CARTESIAN_POINT('',(-54.2707699605536,-64.1721709500326,-208.192630912054));
#200176=CARTESIAN_POINT('',(-54.238698329297,-64.0517945379221,-214.260116171494));
#200177=CARTESIAN_POINT('Ctrl Pts',(-54.2707699605539,-64.1721709500341,
-208.192630912048));
#200178=CARTESIAN_POINT('Ctrl Pts',(-54.2547227572974,-64.1119400013452,
-211.229354398965));
#200179=CARTESIAN_POINT('Ctrl Pts',(-54.2386983294438,-64.051794536968,
-214.260116171476));
#200180=CARTESIAN_POINT('',(-54.2707699605536,-64.1721709500326,-215.85005));
#200181=CARTESIAN_POINT('',(-54.2707699605536,-64.1721709500326,-208.192630912054));
#200182=CARTESIAN_POINT('',(-53.7300151844416,-62.1425230012532,-215.85005));
#200183=CARTESIAN_POINT('',(-53.272912245153,-60.426850603907,-215.85005));
#200184=CARTESIAN_POINT('Ctrl Pts',(-53.7300151844417,-62.1425230012532,
-215.85005));
#200185=CARTESIAN_POINT('Ctrl Pts',(-53.8150179700973,-62.461569151501,
-215.585784056343));
#200186=CARTESIAN_POINT('Ctrl Pts',(-53.8997787313594,-62.7797068968052,
-215.321544427158));
#200187=CARTESIAN_POINT('Ctrl Pts',(-54.0694761933671,-63.4166427518218,
-214.791113982276));
#200188=CARTESIAN_POINT('Ctrl Pts',(-54.1539754816099,-63.7337990944548,
-214.526290576097));
#200189=CARTESIAN_POINT('Ctrl Pts',(-54.238698329735,-64.0517945380611,
-214.260116171799));
#200190=CARTESIAN_POINT('Origin',(-52.3809255634408,-67.7420224291304,-167.906149834141));
#200191=CARTESIAN_POINT('',(-50.9302694872204,-67.3511117063321,-214.24934096818));
#200192=CARTESIAN_POINT('',(-51.0503406624406,-67.3834674874005,-208.192630912054));
#200193=CARTESIAN_POINT('Ctrl Pts',(-50.9302694862954,-67.35111170647,-214.249340968162));
#200194=CARTESIAN_POINT('Ctrl Pts',(-50.9902625163406,-67.3672781287523,
-211.223956213722));
#200195=CARTESIAN_POINT('Ctrl Pts',(-51.0503406624421,-67.3834674874009,
-208.192630912048));
#200196=CARTESIAN_POINT('',(-48.9715866554311,-66.8233021636441,-215.85005));
#200197=CARTESIAN_POINT('Ctrl Pts',(-50.930269487352,-67.3511117067548,
-214.249340968478));
#200198=CARTESIAN_POINT('Ctrl Pts',(-50.6074451104335,-67.2641196812418,
-214.515373951332));
#200199=CARTESIAN_POINT('Ctrl Pts',(-50.2841497321107,-67.1770007341929,
-214.780661946596));
#200200=CARTESIAN_POINT('Ctrl Pts',(-49.631251415414,-67.0010631313216,
-215.314234969152));
#200201=CARTESIAN_POINT('Ctrl Pts',(-49.3016472827222,-66.9122441536643,
-215.582485903116));
#200202=CARTESIAN_POINT('Ctrl Pts',(-48.9715866554311,-66.8233021636442,
-215.85005));
#200203=CARTESIAN_POINT('',(-51.0503406624406,-67.3834674874005,-215.85005));
#200204=CARTESIAN_POINT('',(-52.3809255634408,-67.7420224291304,-215.85005));
#200205=CARTESIAN_POINT('',(-51.0503406624406,-67.3834674874005,-208.192630912054));
#200206=CARTESIAN_POINT('Origin',(0.,-12.9675000200281,-167.906149834141));
#200207=CARTESIAN_POINT('Origin',(0.,-12.9675000200281,-208.192630912054));
#200208=CARTESIAN_POINT('Origin',(0.,-12.9675000200281,-215.85005));
#200209=CARTESIAN_POINT('Origin',(-48.9106432152246,18.4987427374335,-167.906149834141));
#200210=CARTESIAN_POINT('',(-54.1218033366501,38.2387592929899,-214.33352989342));
#200211=CARTESIAN_POINT('',(-54.1539855075907,38.3606662320892,-208.192630912062));
#200212=CARTESIAN_POINT('Ctrl Pts',(-54.1218033367874,38.2387592920601,
-214.333529893402));
#200213=CARTESIAN_POINT('Ctrl Pts',(-54.1378828568779,38.299668952361,-211.26613387672));
#200214=CARTESIAN_POINT('Ctrl Pts',(-54.1539855075911,38.3606662320908,
-208.192630912056));
#200215=CARTESIAN_POINT('',(-53.6858060762413,36.5871897873467,-215.85005));
#200216=CARTESIAN_POINT('Ctrl Pts',(-54.1218033370754,38.2387592931511,
-214.333529893716));
#200217=CARTESIAN_POINT('Ctrl Pts',(-54.0493242413351,37.964206503292,-214.587336490157));
#200218=CARTESIAN_POINT('Ctrl Pts',(-53.9768175206508,37.6895490693906,
-214.840391892303));
#200219=CARTESIAN_POINT('Ctrl Pts',(-53.8314491180661,37.1388895988311,
-215.346026703316));
#200220=CARTESIAN_POINT('Ctrl Pts',(-53.7586988751215,36.8633096959739,
-215.598218415201));
#200221=CARTESIAN_POINT('Ctrl Pts',(-53.6858060762413,36.5871897873468,
-215.85005));
#200222=CARTESIAN_POINT('',(-54.1539855075907,38.3606662320892,-215.85005));
#200223=CARTESIAN_POINT('',(-53.3004948454233,35.1276203445352,-215.85005));
#200224=CARTESIAN_POINT('',(-54.1539855075907,38.3606662320892,-208.192630912062));
#200225=CARTESIAN_POINT('Origin',(-52.2560139340206,41.9262034053684,-167.906149834141));
#200226=CARTESIAN_POINT('',(-50.9262492693411,41.5646183371225,-208.192630912063));
#200227=CARTESIAN_POINT('',(-50.8045364442235,41.5315226009329,-214.335913275013));
#200228=CARTESIAN_POINT('Ctrl Pts',(-50.9262492693426,41.5646183371229,
-208.192630912057));
#200229=CARTESIAN_POINT('Ctrl Pts',(-50.8653490995025,41.5480585708328,
-211.267327940101));
#200230=CARTESIAN_POINT('Ctrl Pts',(-50.8045364435665,41.5315226010249,
-214.335913275001));
#200231=CARTESIAN_POINT('',(-50.9262492693411,41.5646183371225,-215.85005));
#200232=CARTESIAN_POINT('',(-50.9262492693411,41.5646183371225,-208.192630912063));
#200233=CARTESIAN_POINT('',(-49.1680521502591,41.086535378401,-215.85005));
#200234=CARTESIAN_POINT('',(-47.6970590536189,40.6865479570431,-215.85005));
#200235=CARTESIAN_POINT('Ctrl Pts',(-49.1680521502592,41.086535378401,-215.85005));
#200236=CARTESIAN_POINT('Ctrl Pts',(-49.4414268426942,41.1608704915578,
-215.598356099776));
#200237=CARTESIAN_POINT('Ctrl Pts',(-49.7144017835719,41.2350969056357,
-215.346413106432));
#200238=CARTESIAN_POINT('Ctrl Pts',(-50.2599964077829,41.3834531333729,
-214.841609804261));
#200239=CARTESIAN_POINT('Ctrl Pts',(-50.532314182124,41.4575008529695,-214.589028866928));
#200240=CARTESIAN_POINT('Ctrl Pts',(-50.8045364443354,41.5315226012339,
-214.335913275222));
#200241=CARTESIAN_POINT('Origin',(0.,-12.9675000200281,-167.906149834141));
#200242=CARTESIAN_POINT('Origin',(0.,-12.9675000200281,-208.192630912063));
#200243=CARTESIAN_POINT('Origin',(0.,-12.9675000200281,-215.85005));
#200244=CARTESIAN_POINT('Origin',(-22.9178089794592,-52.5372975341153,-234.75005));
#200245=CARTESIAN_POINT('',(-27.0625191140422,-59.958306757953,-232.85005));
#200246=CARTESIAN_POINT('',(-23.2057914601203,-61.0324176680998,-232.85005));
#200247=CARTESIAN_POINT('Origin',(-22.9178089794592,-52.5372975341153,-232.85005));
#200248=CARTESIAN_POINT('',(-23.2057914601203,-61.0324176680998,-232.25005));
#200249=CARTESIAN_POINT('',(-23.2057914601203,-61.0324176680998,-234.75005));
#200250=CARTESIAN_POINT('',(-27.0625191140422,-59.958306757953,-232.25005));
#200251=CARTESIAN_POINT('Origin',(-22.9178089794592,-52.5372975341153,-232.25005));
#200252=CARTESIAN_POINT('',(-27.0625191140422,-59.958306757953,-234.75005));
#200253=CARTESIAN_POINT('Origin',(-24.838300653577,28.3971299569735,-234.75005));
#200254=CARTESIAN_POINT('',(-25.8757946403502,36.8335750748777,-232.85005));
#200255=CARTESIAN_POINT('',(-29.3303337505005,35.613198045354,-232.85005));
#200256=CARTESIAN_POINT('Origin',(-24.838300653577,28.3971299569735,-232.85005));
#200257=CARTESIAN_POINT('',(-29.3303337505005,35.613198045354,-232.25005));
#200258=CARTESIAN_POINT('',(-29.3303337505005,35.613198045354,-234.75005));
#200259=CARTESIAN_POINT('',(-25.8757946403502,36.8335750748777,-232.25005));
#200260=CARTESIAN_POINT('Origin',(-24.838300653577,28.3971299569735,-232.25005));
#200261=CARTESIAN_POINT('',(-25.8757946403502,36.8335750748777,-234.75005));
#200262=CARTESIAN_POINT('Origin',(6.29739814579425E-15,-11.5034818258363,
-234.75005));
#200263=CARTESIAN_POINT('',(-46.0422390557602,19.4862297367486,-232.85005));
#200264=CARTESIAN_POINT('Origin',(6.29739814579425E-15,-11.5034818258363,
-232.85005));
#200265=CARTESIAN_POINT('',(-46.0422390557602,19.4862297367486,-232.25005));
#200266=CARTESIAN_POINT('',(-46.0422390557602,19.4862297367486,-234.75005));
#200267=CARTESIAN_POINT('Origin',(6.29739814579425E-15,-11.5034818258363,
-232.25005));
#200268=CARTESIAN_POINT('Origin',(-38.9907249661392,14.740057695632,-234.75005));
#200269=CARTESIAN_POINT('',(-47.4843254762175,15.0698309134599,-232.85005));
#200270=CARTESIAN_POINT('Origin',(-38.9907249661392,14.740057695632,-232.85005));
#200271=CARTESIAN_POINT('',(-47.4843254762175,15.0698309134599,-232.25005));
#200272=CARTESIAN_POINT('',(-47.4843254762175,15.0698309134599,-234.75005));
#200273=CARTESIAN_POINT('Origin',(-38.9907249661392,14.740057695632,-232.25005));
#200274=CARTESIAN_POINT('Origin',(636.934816028482,-11.5034818258361,-234.75005));
#200275=CARTESIAN_POINT('',(-47.764411700877,6.45952891261038,-232.25005));
#200276=CARTESIAN_POINT('',(-47.7015217254648,8.71393888480408,-232.849988379285));
#200277=CARTESIAN_POINT('Ctrl Pts',(-47.764411700877,6.45952891261038,-232.25005));
#200278=CARTESIAN_POINT('Ctrl Pts',(-47.7543096879139,6.84458911076304,
-232.297638206554));
#200279=CARTESIAN_POINT('Ctrl Pts',(-47.743946362003,7.22712198577601,-232.368832317301));
#200280=CARTESIAN_POINT('Ctrl Pts',(-47.7228772190296,7.98214274175961,
-232.566012007014));
#200281=CARTESIAN_POINT('Ctrl Pts',(-47.7121682193403,8.3544760456171,-232.692635516398));
#200282=CARTESIAN_POINT('Ctrl Pts',(-47.7015533799491,8.71393371652249,
-232.849926758569));
#200283=CARTESIAN_POINT('Origin',(636.934816028482,-11.5034818258361,-232.25005));
#200284=CARTESIAN_POINT('Origin',(636.934816028482,-11.5034818258361,-232.85005));
#200285=CARTESIAN_POINT('Origin',(-38.9907249661392,-37.7470213473046,-234.75005));
#200286=CARTESIAN_POINT('',(-47.4843254762176,-38.0767945651323,-232.85005));
#200287=CARTESIAN_POINT('',(-46.0422390557601,-42.4931933884212,-232.85005));
#200288=CARTESIAN_POINT('Origin',(-38.9907249661392,-37.7470213473046,-232.85005));
#200289=CARTESIAN_POINT('',(-46.0422390557601,-42.4931933884212,-232.25005));
#200290=CARTESIAN_POINT('',(-46.0422390557601,-42.4931933884212,-234.75005));
#200291=CARTESIAN_POINT('',(-47.4843254762176,-38.0767945651323,-232.25005));
#200292=CARTESIAN_POINT('Origin',(-38.9907249661392,-37.7470213473046,-232.25005));
#200293=CARTESIAN_POINT('',(-47.4843254762176,-38.0767945651323,-234.75005));
#200294=CARTESIAN_POINT('Origin',(6.29739814579425E-15,-11.5034818258363,
-234.75005));
#200295=CARTESIAN_POINT('Origin',(6.29739814579425E-15,-11.5034818258363,
-232.85005));
#200296=CARTESIAN_POINT('Origin',(6.29739814579425E-15,-11.5034818258363,
-232.25005));
#200297=CARTESIAN_POINT('Ctrl Pts',(-47.269359813636,-39.9199414144257,
-233.323677937652));
#200298=CARTESIAN_POINT('Ctrl Pts',(-47.7852688958474,-40.5328114906027,
-232.537018038148));
#200299=CARTESIAN_POINT('Ctrl Pts',(-48.3011810934468,-41.1456737613432,
-231.750354102807));
#200300=CARTESIAN_POINT('Ctrl Pts',(-48.8170958227918,-41.7585296857986,
-230.963686885275));
#200301=CARTESIAN_POINT('Ctrl Pts',(-49.3330105521369,-42.3713856102541,
-230.177019667743));
#200302=CARTESIAN_POINT('Ctrl Pts',(-49.8489278162636,-42.9842351808713,
-229.390349164127));
#200303=CARTESIAN_POINT('Ctrl Pts',(-50.3648471682373,-43.5970795157942,
-228.603675952145));
#200304=CARTESIAN_POINT('Ctrl Pts',(-51.3966858721847,-44.82276818564,-227.03032952818));
#200305=CARTESIAN_POINT('Ctrl Pts',(-52.4285328613266,-46.0484360781329,
-225.456972356173));
#200306=CARTESIAN_POINT('Ctrl Pts',(-53.4603856521184,-47.2740894119757,
-223.883607650579));
#200307=CARTESIAN_POINT('Ctrl Pts',(-55.5240912337021,-49.7253960796616,
-220.736878239389));
#200308=CARTESIAN_POINT('Ctrl Pts',(-57.5878196113417,-52.1766455410871,
-217.590119225487));
#200309=CARTESIAN_POINT('Ctrl Pts',(-59.6515602724445,-54.6278641542595,
-214.443344242486));
#200310=CARTESIAN_POINT('Ctrl Pts',(-47.2844095710387,-40.0223529985484,
-233.29571384424));
#200311=CARTESIAN_POINT('Ctrl Pts',(-47.799865767177,-40.6397128949599,
-232.509454608122));
#200312=CARTESIAN_POINT('Ctrl Pts',(-48.3153486991529,-41.2570069665437,
-231.72316146998));
#200313=CARTESIAN_POINT('Ctrl Pts',(-48.8308531059458,-41.8742482184852,
-230.936841114977));
#200314=CARTESIAN_POINT('Ctrl Pts',(-49.3463575127387,-42.4914894704268,
-230.150520759975));
#200315=CARTESIAN_POINT('Ctrl Pts',(-49.8618834246415,-43.1086778283034,
-229.364173149988));
#200316=CARTESIAN_POINT('Ctrl Pts',(-50.3774268752988,-43.7258231065776,
-228.577803332719));
#200317=CARTESIAN_POINT('Ctrl Pts',(-51.4085137766134,-44.9601136631259,
-227.005063698182));
#200318=CARTESIAN_POINT('Ctrl Pts',(-52.4396702308542,-46.1942333889078,
-225.432235999036));
#200319=CARTESIAN_POINT('Ctrl Pts',(-53.4708746321289,-47.4282358136099,
-223.859347784982));
#200320=CARTESIAN_POINT('Ctrl Pts',(-55.5332834346784,-49.8962406630142,
-220.713571356874));
#200321=CARTESIAN_POINT('Ctrl Pts',(-57.5958804822797,-52.3637850919073,
-217.567557391373));
#200322=CARTESIAN_POINT('Ctrl Pts',(-59.658577156368,-54.831089092749,-214.42141923076));
#200323=CARTESIAN_POINT('Ctrl Pts',(-47.3011370887008,-40.083704476459,
-233.264807132349));
#200324=CARTESIAN_POINT('Ctrl Pts',(-47.8155006007713,-40.7086470422379,
-232.479276052542));
#200325=CARTESIAN_POINT('Ctrl Pts',(-48.330070971135,-41.3331587221332,
-231.693536730416));
#200326=CARTESIAN_POINT('Ctrl Pts',(-48.8447653455944,-41.957411102505,
-230.907671551986));
#200327=CARTESIAN_POINT('Ctrl Pts',(-49.3594597200538,-42.5816634828768,
-230.121806373556));
#200328=CARTESIAN_POINT('Ctrl Pts',(-49.8742800565343,-43.2056525867135,
-229.335813456774));
#200329=CARTESIAN_POINT('Ctrl Pts',(-50.3891818457356,-43.8294712170294,
-228.549737580672));
#200330=CARTESIAN_POINT('Ctrl Pts',(-51.4189854241382,-45.0771084776612,
-226.977585828468));
#200331=CARTESIAN_POINT('Ctrl Pts',(-52.4491078990803,-46.3240783396034,
-225.405109260953));
#200332=CARTESIAN_POINT('Ctrl Pts',(-53.4793832226061,-47.5707292968664,
-223.832476822232));
#200333=CARTESIAN_POINT('Ctrl Pts',(-55.5399338696578,-50.0640312113922,
-220.68721194479));
#200334=CARTESIAN_POINT('Ctrl Pts',(-57.6010852364915,-52.5560807120374,
-217.541335107067));
#200335=CARTESIAN_POINT('Ctrl Pts',(-59.6624305478473,-55.0477381521116,
-214.39526566237));
#200336=CARTESIAN_POINT('Ctrl Pts',(-47.3051413523369,-40.1629192793609,
-233.246904846954));
#200337=CARTESIAN_POINT('Ctrl Pts',(-47.819327369804,-40.7940757964512,
-232.460673323282));
#200338=CARTESIAN_POINT('Ctrl Pts',(-48.3336083951406,-41.4250391409392,
-231.674348554294));
#200339=CARTESIAN_POINT('Ctrl Pts',(-48.8479443642697,-42.0558912348621,
-230.88796994392));
#200340=CARTESIAN_POINT('Ctrl Pts',(-49.3622803333988,-42.6867433287849,
-230.101591333545));
#200341=CARTESIAN_POINT('Ctrl Pts',(-49.8766723259409,-43.3174819888763,
-229.315157839431));
#200342=CARTESIAN_POINT('Ctrl Pts',(-50.3910998220442,-43.9481493585103,
-228.52868979147));
#200343=CARTESIAN_POINT('Ctrl Pts',(-51.4199548142509,-45.2094840977783,
-226.955753695549));
#200344=CARTESIAN_POINT('Ctrl Pts',(-52.4489487693187,-46.4705399682764,
-225.382682428314));
#200345=CARTESIAN_POINT('Ctrl Pts',(-53.4780084556675,-47.7314680211233,
-223.809549063998));
#200346=CARTESIAN_POINT('Ctrl Pts',(-55.536127828365,-50.253324126817,-220.663282335366));
#200347=CARTESIAN_POINT('Ctrl Pts',(-57.5945065616385,-52.7746765489683,
-217.516770963173));
#200348=CARTESIAN_POINT('Ctrl Pts',(-59.6529740461698,-55.2958790062696,
-214.370186647608));
#200349=CARTESIAN_POINT('Ctrl Pts',(-47.3091454883712,-40.242131557965,
-233.229003132042));
#200350=CARTESIAN_POINT('Ctrl Pts',(-47.8231540168911,-40.8795018283497,
-232.442071186825));
#200351=CARTESIAN_POINT('Ctrl Pts',(-48.337145706421,-41.5169166318385,
-231.655160989632));
#200352=CARTESIAN_POINT('Ctrl Pts',(-48.8511232816408,-42.1543682290027,
-230.868268963674));
#200353=CARTESIAN_POINT('Ctrl Pts',(-49.3651008568606,-42.7918198261669,
-230.081376937717));
#200354=CARTESIAN_POINT('Ctrl Pts',(-49.8790645191143,-43.4293078274282,
-229.294502880311));
#200355=CARTESIAN_POINT('Ctrl Pts',(-50.3930177372337,-44.066823718135,
-228.507642672989));
#200356=CARTESIAN_POINT('Ctrl Pts',(-51.4209241734724,-45.3418554995486,
-226.933922258343));
#200357=CARTESIAN_POINT('Ctrl Pts',(-52.4487896446279,-46.616996929731,
-225.36025631034));
#200358=CARTESIAN_POINT('Ctrl Pts',(-53.4766337325378,-47.8922016232008,
-223.786622036391));
#200359=CARTESIAN_POINT('Ctrl Pts',(-55.5323219083575,-50.4426110101405,
-220.639353488495));
#200360=CARTESIAN_POINT('Ctrl Pts',(-57.5879280964248,-52.9932654200165,
-217.492207602051));
#200361=CARTESIAN_POINT('Ctrl Pts',(-59.6435178458378,-55.5440119530488,
-214.345108432027));
#200362=CARTESIAN_POINT('Ctrl Pts',(-47.3136637970655,-40.310070641192,
-233.20976892517));
#200363=CARTESIAN_POINT('Ctrl Pts',(-47.8271241660854,-40.955047815909,
-232.422048268856));
#200364=CARTESIAN_POINT('Ctrl Pts',(-48.3403579331886,-41.6004954572377,
-231.634553866964));
#200365=CARTESIAN_POINT('Ctrl Pts',(-48.8534714666716,-42.246191520782,
-230.847179503763));
#200366=CARTESIAN_POINT('Ctrl Pts',(-49.3665850001545,-42.8918875843263,
-230.059805140562));
#200367=CARTESIAN_POINT('Ctrl Pts',(-49.8795751912289,-43.537838701044,
-229.272553878112));
#200368=CARTESIAN_POINT('Ctrl Pts',(-50.3924934876008,-44.183938665318,
-228.485374488428));
#200369=CARTESIAN_POINT('Ctrl Pts',(-51.4183300803446,-45.476138593866,
-226.911015709061));
#200370=CARTESIAN_POINT('Ctrl Pts',(-52.4438863060015,-46.7689192505898,
-225.336937281619));
#200371=CARTESIAN_POINT('Ctrl Pts',(-53.4693312838495,-48.0619358471384,
-223.762972649457));
#200372=CARTESIAN_POINT('Ctrl Pts',(-55.5202212395457,-50.6479690402357,
-220.615043385133));
#200373=CARTESIAN_POINT('Ctrl Pts',(-57.5706688803884,-53.2349422023283,
-217.467567478191));
#200374=CARTESIAN_POINT('Ctrl Pts',(-59.6210250673444,-55.8221505796269,
-214.320205136697));
#200375=CARTESIAN_POINT('Ctrl Pts',(-47.3174213500927,-40.3725566206431,
-233.190758458866));
#200376=CARTESIAN_POINT('Ctrl Pts',(-47.8304331865629,-41.0247379875799,
-232.40178755381));
#200377=CARTESIAN_POINT('Ctrl Pts',(-48.3427237376172,-41.6782347797706,
-231.613445913152));
#200378=CARTESIAN_POINT('Ctrl Pts',(-48.8546863035239,-42.3323210585191,
-230.825382497106));
#200379=CARTESIAN_POINT('Ctrl Pts',(-49.3666488694307,-42.9864073372676,
-230.037319081059));
#200380=CARTESIAN_POINT('Ctrl Pts',(-49.8782662454544,-43.6411158354054,
-229.249550061497));
#200381=CARTESIAN_POINT('Ctrl Pts',(-50.3896983451462,-44.2961564367811,
-228.461936921534));
#200382=CARTESIAN_POINT('Ctrl Pts',(-51.4125625445298,-45.6062376395327,
-226.886710641608));
#200383=CARTESIAN_POINT('Ctrl Pts',(-52.4347028263001,-46.9176171020422,
-225.312093851176));
#200384=CARTESIAN_POINT('Ctrl Pts',(-53.4565811414505,-48.229468784563,
-223.737696459652));
#200385=CARTESIAN_POINT('Ctrl Pts',(-55.5003377717513,-50.8531721496045,
-220.588901676603));
#200386=CARTESIAN_POINT('Ctrl Pts',(-57.5430330553295,-53.4787928890259,
-217.440999537853));
#200387=CARTESIAN_POINT('Ctrl Pts',(-59.5855147104668,-56.1048379574655,
-214.293293254791));
#200388=CARTESIAN_POINT('Ctrl Pts',(-47.3211789031199,-40.4350426000942,
-233.171747992562));
#200389=CARTESIAN_POINT('Ctrl Pts',(-47.8337422070404,-41.0944281592508,
-232.381526838764));
#200390=CARTESIAN_POINT('Ctrl Pts',(-48.3450895420457,-41.7559741023036,
-231.59233795934));
#200391=CARTESIAN_POINT('Ctrl Pts',(-48.8559011403763,-42.4184505962563,
-230.803585490448));
#200392=CARTESIAN_POINT('Ctrl Pts',(-49.3667127387069,-43.080927090209,
-230.014833021558));
#200393=CARTESIAN_POINT('Ctrl Pts',(-49.87695729968,-43.7443929697667,-229.226546244883));
#200394=CARTESIAN_POINT('Ctrl Pts',(-50.3869032026916,-44.4083742082442,
-228.43849935464));
#200395=CARTESIAN_POINT('Ctrl Pts',(-51.4067950087149,-45.7363366851993,
-226.862405574156));
#200396=CARTESIAN_POINT('Ctrl Pts',(-52.4255193465988,-47.0663149534946,
-225.287250420734));
#200397=CARTESIAN_POINT('Ctrl Pts',(-53.4438309990515,-48.3970017219875,
-223.712420269846));
#200398=CARTESIAN_POINT('Ctrl Pts',(-55.4804543039569,-51.0583752589733,
-220.562759968072));
#200399=CARTESIAN_POINT('Ctrl Pts',(-57.5153972302706,-53.7226435757235,
-217.414431597513));
#200400=CARTESIAN_POINT('Ctrl Pts',(-59.5500043535892,-56.3875253353041,
-214.266381372884));
#200401=CARTESIAN_POINT('Ctrl Pts',(-47.320727875256,-40.4981900996217,
-233.155799645893));
#200402=CARTESIAN_POINT('Ctrl Pts',(-47.8322495334659,-41.1655802828307,
-232.364426098052));
#200403=CARTESIAN_POINT('Ctrl Pts',(-48.3419545189581,-41.8360548922265,
-231.574520658189));
#200404=CARTESIAN_POINT('Ctrl Pts',(-48.8509002126362,-42.507781144632,
-230.785196140269));
#200405=CARTESIAN_POINT('Ctrl Pts',(-49.3598459063144,-43.1795073970375,
-229.995871622349));
#200406=CARTESIAN_POINT('Ctrl Pts',(-49.8679794722695,-43.8525810620647,
-229.207175913618));
#200407=CARTESIAN_POINT('Ctrl Pts',(-50.3756978342709,-44.5263335458687,
-228.418792446769));
#200408=CARTESIAN_POINT('Ctrl Pts',(-51.3911345582736,-45.8738385134766,
-226.842025513071));
#200409=CARTESIAN_POINT('Ctrl Pts',(-52.4049464549377,-47.224002264507,
-225.266482347449));
#200410=CARTESIAN_POINT('Ctrl Pts',(-53.4182055248116,-48.5750603074809,
-223.691342941789));
#200411=CARTESIAN_POINT('Ctrl Pts',(-55.4447236645594,-51.2771763934287,
-220.541064130469));
#200412=CARTESIAN_POINT('Ctrl Pts',(-57.4689725824102,-53.9829798427017,
-217.392457267063));
#200413=CARTESIAN_POINT('Ctrl Pts',(-59.492784702789,-56.6895247738662,
-214.244180243974));
#200414=CARTESIAN_POINT('Ctrl Pts',(-47.3143897740156,-40.5659557077008,
-233.143618951735));
#200415=CARTESIAN_POINT('Ctrl Pts',(-47.8252832097387,-41.239862847313,
-232.350527479362));
#200416=CARTESIAN_POINT('Ctrl Pts',(-48.3335556171132,-41.9180591247534,
-231.559510554001));
#200417=CARTESIAN_POINT('Ctrl Pts',(-48.84072766068,-42.5979714018469,-230.769289654088));
#200418=CARTESIAN_POINT('Ctrl Pts',(-49.3478997042467,-43.2778836789405,
-229.979068754174));
#200419=CARTESIAN_POINT('Ctrl Pts',(-49.853896141919,-43.9596488205701,
-229.189715484531));
#200420=CARTESIAN_POINT('Ctrl Pts',(-50.3592905012865,-44.6423395873253,
-228.400785431186));
#200421=CARTESIAN_POINT('Ctrl Pts',(-51.3700792200214,-46.0077211208357,
-226.822925324494));
#200422=CARTESIAN_POINT('Ctrl Pts',(-52.3785121216331,-47.3767293468831,
-225.246725326938));
#200423=CARTESIAN_POINT('Ctrl Pts',(-53.3861409718259,-48.7469431347296,
-223.67105962423));
#200424=CARTESIAN_POINT('Ctrl Pts',(-55.4013986722116,-51.4873707104227,
-220.519728218813));
#200425=CARTESIAN_POINT('Ctrl Pts',(-57.4133569116451,-54.2327814391975,
-217.37062149599));
#200426=CARTESIAN_POINT('Ctrl Pts',(-59.4246687676614,-56.9791795051587,
-214.221940194738));
#200427=CARTESIAN_POINT('Ctrl Pts',(-47.3080516727752,-40.6337213157799,
-233.131438257577));
#200428=CARTESIAN_POINT('Ctrl Pts',(-47.8183168860115,-41.3141454117954,
-232.336628860671));
#200429=CARTESIAN_POINT('Ctrl Pts',(-48.3251567152684,-42.0000633572803,
-231.544500449812));
#200430=CARTESIAN_POINT('Ctrl Pts',(-48.8305551087238,-42.688161659062,
-230.753383167905));
#200431=CARTESIAN_POINT('Ctrl Pts',(-49.3359535021791,-43.3762599608436,
-229.962265885999));
#200432=CARTESIAN_POINT('Ctrl Pts',(-49.8398128115685,-44.0667165790755,
-229.172255055445));
#200433=CARTESIAN_POINT('Ctrl Pts',(-50.3428831683021,-44.7583456287819,
-228.382778415603));
#200434=CARTESIAN_POINT('Ctrl Pts',(-51.3490238817693,-46.1416037281948,
-226.803825135918));
#200435=CARTESIAN_POINT('Ctrl Pts',(-52.3520777883286,-47.5294564292592,
-225.226968306426));
#200436=CARTESIAN_POINT('Ctrl Pts',(-53.3540764188403,-48.9188259619783,
-223.65077630667));
#200437=CARTESIAN_POINT('Ctrl Pts',(-55.3580736798637,-51.6975650274167,
-220.498392307158));
#200438=CARTESIAN_POINT('Ctrl Pts',(-57.35774124088,-54.4825830356932,-217.348785724916));
#200439=CARTESIAN_POINT('Ctrl Pts',(-59.3565528325338,-57.2688342364512,
-214.199700145503));
#200440=CARTESIAN_POINT('Ctrl Pts',(-47.3048034248152,-40.692173181322,
-233.11661797197));
#200441=CARTESIAN_POINT('Ctrl Pts',(-47.8136028177951,-41.3798076595766,
-232.320613610482));
#200442=CARTESIAN_POINT('Ctrl Pts',(-48.3182607882955,-42.0738441576018,
-231.527752466761));
#200443=CARTESIAN_POINT('Ctrl Pts',(-48.8211728608215,-42.770397212734,
-230.736051725279));
#200444=CARTESIAN_POINT('Ctrl Pts',(-49.3240849333475,-43.4669502678662,
-229.944350983796));
#200445=CARTESIAN_POINT('Ctrl Pts',(-49.8251339017092,-44.1662308838252,
-229.153926426443));
#200446=CARTESIAN_POINT('Ctrl Pts',(-50.325227721477,-44.8668595754618,
-228.364110202531));
#200447=CARTESIAN_POINT('Ctrl Pts',(-51.3254153610126,-46.2681169587348,
-226.784477754705));
#200448=CARTESIAN_POINT('Ctrl Pts',(-52.3218662832923,-47.674658517871,
-225.207234282834));
#200449=CARTESIAN_POINT('Ctrl Pts',(-53.3170401441828,-49.0829298658951,
-223.630734549434));
#200450=CARTESIAN_POINT('Ctrl Pts',(-55.3073878659637,-51.8994725619434,
-220.477735082634));
#200451=CARTESIAN_POINT('Ctrl Pts',(-57.2924955409022,-54.7231886232885,
-217.327855954057));
#200452=CARTESIAN_POINT('Ctrl Pts',(-59.2765646638181,-57.5482976749593,
-214.178548151011));
#200453=CARTESIAN_POINT('Ctrl Pts',(-47.3009006987844,-40.7491010613005,
-233.101301752625));
#200454=CARTESIAN_POINT('Ctrl Pts',(-47.8070153253589,-41.445066041129,
-232.304686649286));
#200455=CARTESIAN_POINT('Ctrl Pts',(-48.3084583519731,-42.1479407187119,
-231.511460238167));
#200456=CARTESIAN_POINT('Ctrl Pts',(-48.8079303323174,-42.8535202192507,
-230.719470612188));
#200457=CARTESIAN_POINT('Ctrl Pts',(-49.3074023126618,-43.5590997197895,
-229.92748098621));
#200458=CARTESIAN_POINT('Ctrl Pts',(-49.8047715089351,-44.2676134042324,
-229.136855227393));
#200459=CARTESIAN_POINT('Ctrl Pts',(-50.3010627023117,-44.9775733943649,
-228.346875024182));
#200460=CARTESIAN_POINT('Ctrl Pts',(-51.293645089065,-46.3974933746299,
-226.766914617761));
#200461=CARTESIAN_POINT('Ctrl Pts',(-52.2820103247895,-47.8230831255928,
-225.189490258971));
#200462=CARTESIAN_POINT('Ctrl Pts',(-53.2689347752898,-49.2505213363517,
-223.612847133253));
#200463=CARTESIAN_POINT('Ctrl Pts',(-55.2427836762905,-52.1053977578695,
-220.459560881818));
#200464=CARTESIAN_POINT('Ctrl Pts',(-57.2107204090195,-54.9679461288674,
-217.309560330918));
#200465=CARTESIAN_POINT('Ctrl Pts',(-59.1774846171821,-57.8319751776559,
-214.160152831317));
#200466=CARTESIAN_POINT('Ctrl Pts',(-47.2969979727536,-40.8060289412791,
-233.085985533281));
#200467=CARTESIAN_POINT('Ctrl Pts',(-47.8004278329226,-41.5103244226814,
-232.28875968809));
#200468=CARTESIAN_POINT('Ctrl Pts',(-48.2986559156506,-42.2220372798219,
-231.495168009573));
#200469=CARTESIAN_POINT('Ctrl Pts',(-48.7946878038133,-42.9366432257674,
-230.702889499098));
#200470=CARTESIAN_POINT('Ctrl Pts',(-49.2907196919761,-43.6512491717128,
-229.910610988623));
#200471=CARTESIAN_POINT('Ctrl Pts',(-49.7844091161609,-44.3689959246396,
-229.119784028342));
#200472=CARTESIAN_POINT('Ctrl Pts',(-50.2768976831464,-45.088287213268,
-228.329639845834));
#200473=CARTESIAN_POINT('Ctrl Pts',(-51.2618748171174,-46.5268697905249,
-226.749351480816));
#200474=CARTESIAN_POINT('Ctrl Pts',(-52.2421543662867,-47.9715077333147,
-225.171746235109));
#200475=CARTESIAN_POINT('Ctrl Pts',(-53.2208294063969,-49.4181128068083,
-223.594959717073));
#200476=CARTESIAN_POINT('Ctrl Pts',(-55.1781794866173,-52.3113229537955,
-220.441386681001));
#200477=CARTESIAN_POINT('Ctrl Pts',(-57.1289452771368,-55.2127036344464,
-217.291264707778));
#200478=CARTESIAN_POINT('Ctrl Pts',(-59.078404570546,-58.1156526803525,
-214.141757511623));
#200479=CARTESIAN_POINT('Ctrl Pts',(-47.2838098592026,-40.8729843211449,
-233.075391456688));
#200480=CARTESIAN_POINT('Ctrl Pts',(-47.7845860001848,-41.584775131594,
-232.277142649072));
#200481=CARTESIAN_POINT('Ctrl Pts',(-48.2794983189707,-42.3046867305642,
-231.482901088115));
#200482=CARTESIAN_POINT('Ctrl Pts',(-48.7719103193318,-43.02777887034,-230.690101915866));
#200483=CARTESIAN_POINT('Ctrl Pts',(-49.2643223196929,-43.7508710101157,
-229.897302743617));
#200484=CARTESIAN_POINT('Ctrl Pts',(-49.7540733460123,-44.4774123295628,
-229.106099200524));
#200485=CARTESIAN_POINT('Ctrl Pts',(-50.2424538195015,-45.2056526956051,
-228.315643851313));
#200486=CARTESIAN_POINT('Ctrl Pts',(-51.2192147664799,-46.6621334276898,
-226.734733152891));
#200487=CARTESIAN_POINT('Ctrl Pts',(-52.1906157326061,-48.1252743043166,
-225.156762925491));
#200488=CARTESIAN_POINT('Ctrl Pts',(-53.160175528661,-49.5905823504069,
-223.57968507695));
#200489=CARTESIAN_POINT('Ctrl Pts',(-55.0992951207707,-52.5211984425875,
-220.425529379868));
#200490=CARTESIAN_POINT('Ctrl Pts',(-57.0308683476032,-55.4608117845694,
-217.275139764089));
#200491=CARTESIAN_POINT('Ctrl Pts',(-58.960931477471,-58.4021538834631,
-214.125415506933));
#200492=CARTESIAN_POINT('Ctrl Pts',(-47.2640162261029,-40.9447914059068,
-233.067937997558));
#200493=CARTESIAN_POINT('Ctrl Pts',(-47.7628369926546,-41.6622203630557,
-232.268067857029));
#200494=CARTESIAN_POINT('Ctrl Pts',(-48.2549965369399,-42.3887167282325,
-231.472771264582));
#200495=CARTESIAN_POINT('Ctrl Pts',(-48.7442220365055,-43.1188281595447,
-230.679129004258));
#200496=CARTESIAN_POINT('Ctrl Pts',(-49.2334475360712,-43.8489395908569,
-229.885486743933));
#200497=CARTESIAN_POINT('Ctrl Pts',(-49.7195709178301,-44.5829547593942,
-229.093671052645));
#200498=CARTESIAN_POINT('Ctrl Pts',(-50.2040684510243,-45.3189094985237,
-228.302711021656));
#200499=CARTESIAN_POINT('Ctrl Pts',(-51.1730635174128,-46.7908189767828,
-226.720790959677));
#200500=CARTESIAN_POINT('Ctrl Pts',(-52.1357048103052,-48.2703270275798,
-225.142232468079));
#200501=CARTESIAN_POINT('Ctrl Pts',(-53.0961142063379,-49.7523323833611,
-223.564687821978));
#200502=CARTESIAN_POINT('Ctrl Pts',(-55.0169329984032,-52.7163430949238,
-220.409598529776));
#200503=CARTESIAN_POINT('Ctrl Pts',(-56.9286455988057,-55.6906960308185,
-217.258791511269));
#200504=CARTESIAN_POINT('Ctrl Pts',(-58.8384812385968,-58.6670561134909,
-214.108729566325));
#200505=CARTESIAN_POINT('Ctrl Pts',(-47.2442225930031,-41.0165984906687,
-233.060484538427));
#200506=CARTESIAN_POINT('Ctrl Pts',(-47.7410879851243,-41.7396655945174,
-232.258993064984));
#200507=CARTESIAN_POINT('Ctrl Pts',(-48.2304947549091,-42.4727467259007,
-231.46264144105));
#200508=CARTESIAN_POINT('Ctrl Pts',(-48.7165337536793,-43.2098774487494,
-230.66815609265));
#200509=CARTESIAN_POINT('Ctrl Pts',(-49.2025727524494,-43.9470081715982,
-229.873670744249));
#200510=CARTESIAN_POINT('Ctrl Pts',(-49.6850684896479,-44.6884971892255,
-229.081242904766));
#200511=CARTESIAN_POINT('Ctrl Pts',(-50.1656830825472,-45.4321663014423,
-228.289778191998));
#200512=CARTESIAN_POINT('Ctrl Pts',(-51.1269122683457,-46.9195045258758,
-226.706848766463));
#200513=CARTESIAN_POINT('Ctrl Pts',(-52.0807938880043,-48.415379750843,
-225.127702010668));
#200514=CARTESIAN_POINT('Ctrl Pts',(-53.0320528840148,-49.9140824163154,
-223.549690567007));
#200515=CARTESIAN_POINT('Ctrl Pts',(-54.9345708760356,-52.9114877472602,
-220.393667679684));
#200516=CARTESIAN_POINT('Ctrl Pts',(-56.8264228500083,-55.9205802770675,
-217.24244325845));
#200517=CARTESIAN_POINT('Ctrl Pts',(-58.7160309997225,-58.9319583435186,
-214.092043625716));
#200518=CARTESIAN_POINT('Ctrl Pts',(-47.2331633716395,-41.074937962774,
-233.047719588827));
#200519=CARTESIAN_POINT('Ctrl Pts',(-47.7223958772293,-41.8099539540185,
-232.248012089236));
#200520=CARTESIAN_POINT('Ctrl Pts',(-48.2057678315329,-42.5524924864862,
-231.452175543568));
#200521=CARTESIAN_POINT('Ctrl Pts',(-48.6860560436761,-43.2986376795464,
-230.658029260724));
#200522=CARTESIAN_POINT('Ctrl Pts',(-49.1663442558194,-44.0447828726065,
-229.86388297788));
#200523=CARTESIAN_POINT('Ctrl Pts',(-49.6434655783611,-44.7946821653274,
-229.071521833792));
#200524=CARTESIAN_POINT('Ctrl Pts',(-50.1187524818162,-45.5466353134476,
-228.280074917719));
#200525=CARTESIAN_POINT('Ctrl Pts',(-51.0693262887264,-47.0505416096881,
-226.697181085572));
#200526=CARTESIAN_POINT('Ctrl Pts',(-52.0127499442126,-48.5624569502057,
-225.117853862002));
#200527=CARTESIAN_POINT('Ctrl Pts',(-52.9533507298994,-50.0773066236126,
-223.539705153474));
#200528=CARTESIAN_POINT('Ctrl Pts',(-54.8345523012729,-53.1070059704263,
-220.383407736418));
#200529=CARTESIAN_POINT('Ctrl Pts',(-56.7045075297636,-56.1485479679101,
-217.231955569755));
#200530=CARTESIAN_POINT('Ctrl Pts',(-58.5718893946176,-59.1926043098068,
-214.081397630038));
#200531=CARTESIAN_POINT('Ctrl Pts',(-47.2184619313714,-41.1386068777002,
-233.034226791445));
#200532=CARTESIAN_POINT('Ctrl Pts',(-47.6994633038231,-41.8843414973674,
-232.236899734718));
#200533=CARTESIAN_POINT('Ctrl Pts',(-48.1764662990288,-42.6351364657344,
-231.442184400327));
#200534=CARTESIAN_POINT('Ctrl Pts',(-48.6511105129755,-43.3886793381388,
-230.648777192266));
#200535=CARTESIAN_POINT('Ctrl Pts',(-49.1257547269221,-44.1422222105431,
-229.855369984204));
#200536=CARTESIAN_POINT('Ctrl Pts',(-49.5980020098404,-44.8985826028918,
-229.063316695606));
#200537=CARTESIAN_POINT('Ctrl Pts',(-50.0687290729088,-45.6566352866088,
-228.272029084797));
#200538=CARTESIAN_POINT('Ctrl Pts',(-51.0101831990457,-47.1727406540429,
-226.689453863181));
#200539=CARTESIAN_POINT('Ctrl Pts',(-51.9456932760972,-48.695455984225,
-225.109865596097));
#200540=CARTESIAN_POINT('Ctrl Pts',(-52.8784745199465,-50.2209883221406,
-223.531433290935));
#200541=CARTESIAN_POINT('Ctrl Pts',(-54.7440370076451,-53.2720529979718,
-220.374568680612));
#200542=CARTESIAN_POINT('Ctrl Pts',(-56.5988680832651,-56.3342829748578,
-217.222334895439));
#200543=CARTESIAN_POINT('Ctrl Pts',(-58.4505854057776,-59.3994904876393,
-214.071174978969));
#200544=CARTESIAN_POINT('Ctrl Pts',(-47.2037604911033,-41.2022757926265,
-233.020733994064));
#200545=CARTESIAN_POINT('Ctrl Pts',(-47.6765307304169,-41.9587290407164,
-232.2257873802));
#200546=CARTESIAN_POINT('Ctrl Pts',(-48.1471647665248,-42.7177804449826,
-231.432193257086));
#200547=CARTESIAN_POINT('Ctrl Pts',(-48.6161649822748,-43.4787209967311,
-230.639525123807));
#200548=CARTESIAN_POINT('Ctrl Pts',(-49.0851651980248,-44.2396615484797,
-229.846856990528));
#200549=CARTESIAN_POINT('Ctrl Pts',(-49.5525384413198,-45.0024830404561,
-229.055111557421));
#200550=CARTESIAN_POINT('Ctrl Pts',(-50.0187056640015,-45.76663525977,-228.263983251877));
#200551=CARTESIAN_POINT('Ctrl Pts',(-50.9510401093651,-47.2949396983977,
-226.68172664079));
#200552=CARTESIAN_POINT('Ctrl Pts',(-51.8786366079818,-48.8284550182444,
-225.101877330191));
#200553=CARTESIAN_POINT('Ctrl Pts',(-52.8035983099936,-50.3646700206687,
-223.523161428396));
#200554=CARTESIAN_POINT('Ctrl Pts',(-54.6535217140174,-53.4371000255173,
-220.365729624806));
#200555=CARTESIAN_POINT('Ctrl Pts',(-56.4932286367666,-56.5200179818056,
-217.212714221123));
#200556=CARTESIAN_POINT('Ctrl Pts',(-58.3292814169375,-59.6063766654718,
-214.060952327901));
#200557=CARTESIAN_POINT('Ctrl Pts',(-47.171541404707,-41.2857265086834,
-233.01310592162));
#200558=CARTESIAN_POINT('Ctrl Pts',(-47.639685387572,-42.0470753131842,
-232.218927162867));
#200559=CARTESIAN_POINT('Ctrl Pts',(-48.1062722861412,-42.8103918979816,
-231.425803682192));
#200560=CARTESIAN_POINT('Ctrl Pts',(-48.5716487660823,-43.5751432799917,
-230.633406080342));
#200561=CARTESIAN_POINT('Ctrl Pts',(-49.0370252460235,-44.3398946620018,
-229.841008478492));
#200562=CARTESIAN_POINT('Ctrl Pts',(-49.5011895680945,-45.1060858790577,
-229.049340752905));
#200563=CARTESIAN_POINT('Ctrl Pts',(-49.9644012667793,-45.8733524421474,
-228.25819056826));
#200564=CARTESIAN_POINT('Ctrl Pts',(-50.8908246641489,-47.4078855683268,
-226.675890198969));
#200565=CARTESIAN_POINT('Ctrl Pts',(-51.8134800494771,-48.9466583058251,
-225.095623133202));
#200566=CARTESIAN_POINT('Ctrl Pts',(-52.7337378890505,-50.4879249875678,
-223.516445892042));
#200567=CARTESIAN_POINT('Ctrl Pts',(-54.5742535681973,-53.5704583510531,
-220.358091409721));
#200568=CARTESIAN_POINT('Ctrl Pts',(-56.4054092509004,-56.6627147295212,
-217.203977876217));
#200569=CARTESIAN_POINT('Ctrl Pts',(-58.2323713080084,-59.7588964549113,
-214.051326981263));
#200570=CARTESIAN_POINT('Ctrl Pts',(-47.1301259245572,-41.3776365805516,
-233.007883276788));
#200571=CARTESIAN_POINT('Ctrl Pts',(-47.5942000936469,-42.1428559602882,
-232.214484939109));
#200572=CARTESIAN_POINT('Ctrl Pts',(-48.0571442886842,-42.9095264965149,
-231.42188110874));
#200573=CARTESIAN_POINT('Ctrl Pts',(-48.5191679953314,-43.677310151957,
-230.629855880101));
#200574=CARTESIAN_POINT('Ctrl Pts',(-48.9811917019786,-44.445093807399,
-229.837830651463));
#200575=CARTESIAN_POINT('Ctrl Pts',(-49.4422942329435,-45.2139930242057,
-229.046386055781));
#200576=CARTESIAN_POINT('Ctrl Pts',(-49.9026408989544,-45.9837637819335,
-228.255374275861));
#200577=CARTESIAN_POINT('Ctrl Pts',(-50.8233342309762,-47.5233052973892,
-226.673350716021));
#200578=CARTESIAN_POINT('Ctrl Pts',(-51.7410289944696,-49.0662933806299,
-225.093033330561));
#200579=CARTESIAN_POINT('Ctrl Pts',(-52.6566611088264,-50.611475717687,
-223.51371347964));
#200580=CARTESIAN_POINT('Ctrl Pts',(-54.4879253375398,-53.7018403918012,
-220.355073777797));
#200581=CARTESIAN_POINT('Ctrl Pts',(-56.3111024468989,-56.8007837303405,
-217.200320668143));
#200582=CARTESIAN_POINT('Ctrl Pts',(-58.1301468566089,-59.9036654708269,
-214.047106057761));
#200583=CARTESIAN_POINT('Ctrl Pts',(-47.1094181844823,-41.4235916164857,
-233.005271954373));
#200584=CARTESIAN_POINT('Ctrl Pts',(-47.5714574466843,-42.1907462838401,
-232.21226382723));
#200585=CARTESIAN_POINT('Ctrl Pts',(-48.0325802899557,-42.9590937957815,
-231.419919822014));
#200586=CARTESIAN_POINT('Ctrl Pts',(-48.4929276099559,-43.7283935879396,
-230.628080779981));
#200587=CARTESIAN_POINT('Ctrl Pts',(-48.9532749299561,-44.4976933800977,
-229.836241737948));
#200588=CARTESIAN_POINT('Ctrl Pts',(-49.4128465653679,-45.2679465967797,
-229.044908707219));
#200589=CARTESIAN_POINT('Ctrl Pts',(-49.8717607150419,-46.0389694518266,
-228.253966129662));
#200590=CARTESIAN_POINT('Ctrl Pts',(-50.7895890143898,-47.5810151619205,
-226.672080974546));
#200591=CARTESIAN_POINT('Ctrl Pts',(-51.7048034669659,-49.1261109180323,
-225.091738429241));
#200592=CARTESIAN_POINT('Ctrl Pts',(-52.6181227187143,-50.6732510827466,
-223.512347273439));
#200593=CARTESIAN_POINT('Ctrl Pts',(-54.4447612222111,-53.7675314121752,
-220.353564961834));
#200594=CARTESIAN_POINT('Ctrl Pts',(-56.2639490448981,-56.8698182307502,
-217.198492064106));
#200595=CARTESIAN_POINT('Ctrl Pts',(-58.0790346309092,-59.9760499787848,
-214.044995596012));
#200596=CARTESIAN_POINT('Ctrl Pts',(-47.1035243171495,-41.4544068124509,
-232.995787114217));
#200597=CARTESIAN_POINT('Ctrl Pts',(-47.5618182365402,-42.2252850495327,
-232.204165849507));
#200598=CARTESIAN_POINT('Ctrl Pts',(-48.0196603955539,-42.9967734838342,
-231.412895157786));
#200599=CARTESIAN_POINT('Ctrl Pts',(-48.4770833116826,-43.7688007487221,
-230.621922441887));
#200600=CARTESIAN_POINT('Ctrl Pts',(-48.9345062278113,-44.54082801361,-229.830949725988));
#200601=CARTESIAN_POINT('Ctrl Pts',(-49.391509938849,-45.313394184642,-229.040275082537));
#200602=CARTESIAN_POINT('Ctrl Pts',(-49.8481260220802,-46.0864367596275,
-228.249854204732));
#200603=CARTESIAN_POINT('Ctrl Pts',(-50.7613581885425,-47.6325219095984,
-226.669012449123));
#200604=CARTESIAN_POINT('Ctrl Pts',(-51.6730415942752,-49.1805060788742,
-225.089180182384));
#200605=CARTESIAN_POINT('Ctrl Pts',(-52.5834110903597,-50.7299791212212,
-223.510082333838));
#200606=CARTESIAN_POINT('Ctrl Pts',(-54.4041500825286,-53.8289252059152,
-220.351886636744));
#200607=CARTESIAN_POINT('Ctrl Pts',(-56.2196637687479,-56.9337600260798,
-217.196579358919));
#200608=CARTESIAN_POINT('Ctrl Pts',(-58.0314831441787,-60.0422631998226,
-214.04281865403));
#200609=CARTESIAN_POINT('Ctrl Pts',(-47.0912031843055,-41.4946844018168,
-232.986503298756));
#200610=CARTESIAN_POINT('Ctrl Pts',(-47.5465884139282,-42.2680813083878,
-232.195931935019));
#200611=CARTESIAN_POINT('Ctrl Pts',(-48.0017768129395,-43.0417829154583,
-231.40555195953));
#200612=CARTESIAN_POINT('Ctrl Pts',(-48.4567760318361,-43.8157641577748,
-230.615342754576));
#200613=CARTESIAN_POINT('Ctrl Pts',(-48.9117752507326,-44.5897454000911,
-229.825133549621));
#200614=CARTESIAN_POINT('Ctrl Pts',(-49.366585304478,-45.364006290321,-229.035095136287));
#200615=CARTESIAN_POINT('Ctrl Pts',(-49.8212141883276,-46.1385240104118,
-228.245209329223));
#200616=CARTESIAN_POINT('Ctrl Pts',(-50.7304719560267,-47.6875594505935,
-226.665437715093));
#200617=CARTESIAN_POINT('Ctrl Pts',(-51.6390050797513,-49.2376203690394,
-225.086274713309));
#200618=CARTESIAN_POINT('Ctrl Pts',(-52.5468787652607,-50.7885482821615,
-223.507599498114));
#200619=CARTESIAN_POINT('Ctrl Pts',(-54.3626261362793,-53.8904041084056,
-220.350249067725));
#200620=CARTESIAN_POINT('Ctrl Pts',(-56.1757402684043,-56.9957065400334,
-217.194831063113));
#200621=CARTESIAN_POINT('Ctrl Pts',(-57.9867151256432,-60.1034983677464,
-214.040672462087));
#200622=CARTESIAN_POINT('Ctrl Pts',(-47.0788820514615,-41.5349619911827,
-232.977219483294));
#200623=CARTESIAN_POINT('Ctrl Pts',(-47.5313585913162,-42.310877567243,
-232.187698020531));
#200624=CARTESIAN_POINT('Ctrl Pts',(-47.9838932303251,-43.0867923470826,
-231.398208761274));
#200625=CARTESIAN_POINT('Ctrl Pts',(-48.4364687519895,-43.8627275668274,
-230.608763067264));
#200626=CARTESIAN_POINT('Ctrl Pts',(-48.889044273654,-44.6386627865722,
-229.819317373254));
#200627=CARTESIAN_POINT('Ctrl Pts',(-49.3416606701069,-45.4146183959999,
-229.029915190037));
#200628=CARTESIAN_POINT('Ctrl Pts',(-49.7943023545749,-46.1906112611962,
-228.240564453713));
#200629=CARTESIAN_POINT('Ctrl Pts',(-50.6995857235109,-47.7425969915886,
-226.661862981063));
#200630=CARTESIAN_POINT('Ctrl Pts',(-51.6049685652275,-49.2947346592046,
-225.083369244233));
#200631=CARTESIAN_POINT('Ctrl Pts',(-52.5103464401617,-50.8471174431018,
-223.505116662391));
#200632=CARTESIAN_POINT('Ctrl Pts',(-54.3211021900301,-53.951883010896,
-220.348611498707));
#200633=CARTESIAN_POINT('Ctrl Pts',(-56.1318167680608,-57.0576530539869,
-217.193082767306));
#200634=CARTESIAN_POINT('Ctrl Pts',(-57.9419471071077,-60.1647335356702,
-214.038526270145));
#200635=CARTESIAN_POINT('Ctrl Pts',(-47.0588574073719,-41.5858000428048,
-232.968566523408));
#200636=CARTESIAN_POINT('Ctrl Pts',(-47.5093207248854,-42.363022265842,
-232.17977481419));
#200637=CARTESIAN_POINT('Ctrl Pts',(-47.9599297574655,-43.1401459593037,
-231.39096724535));
#200638=CARTESIAN_POINT('Ctrl Pts',(-48.4106907142535,-43.9171701566874,
-230.602146349555));
#200639=CARTESIAN_POINT('Ctrl Pts',(-48.8614516710415,-44.6941943540713,
-229.813325453759));
#200640=CARTESIAN_POINT('Ctrl Pts',(-49.3123645814213,-45.4711190318301,
-229.024491224305));
#200641=CARTESIAN_POINT('Ctrl Pts',(-49.7634348829592,-46.2479443404272,
-228.235646862402));
#200642=CARTESIAN_POINT('Ctrl Pts',(-50.6655754860351,-47.8015949576215,
-226.657958138597));
#200643=CARTESIAN_POINT('Ctrl Pts',(-51.5683478186111,-49.3548459662596,
-225.080227999184));
#200644=CARTESIAN_POINT('Ctrl Pts',(-52.4717770943224,-50.9077187028313,
-223.502491635481));
#200645=CARTESIAN_POINT('Ctrl Pts',(-54.2786356457449,-54.0134641759745,
-220.347018908076));
#200646=CARTESIAN_POINT('Ctrl Pts',(-56.0882389522679,-57.1176157229696,
-217.191507400736));
#200647=CARTESIAN_POINT('Ctrl Pts',(-57.8999640673718,-60.2209901065118,
-214.036411889894));
#200648=CARTESIAN_POINT('Ctrl Pts',(-47.0185565395742,-41.6609971057424,
-232.962224970815));
#200649=CARTESIAN_POINT('Ctrl Pts',(-47.4683098495203,-42.4379579278734,
-232.173885913265));
#200650=CARTESIAN_POINT('Ctrl Pts',(-47.9182404464189,-43.214781541947,
-231.385510833981));
#200651=CARTESIAN_POINT('Ctrl Pts',(-48.3683681238743,-43.9914549619569,
-230.597098052473));
#200652=CARTESIAN_POINT('Ctrl Pts',(-48.8184958013296,-44.7681283819668,
-229.808685270963));
#200653=CARTESIAN_POINT('Ctrl Pts',(-49.2688205234849,-45.5446516231764,
-229.020234782073));
#200654=CARTESIAN_POINT('Ctrl Pts',(-49.7193651569502,-46.321010055599,
-228.231745013587));
#200655=CARTESIAN_POINT('Ctrl Pts',(-50.6204544238808,-47.8737269204442,
-226.654765476616));
#200656=CARTESIAN_POINT('Ctrl Pts',(-51.5224188067103,-49.4257867780962,
-225.077628467932));
#200657=CARTESIAN_POINT('Ctrl Pts',(-52.4254879069396,-50.9770488729761,
-223.500324296104));
#200658=CARTESIAN_POINT('Ctrl Pts',(-54.2316261073984,-54.079573062736,
-220.345715952448));
#200659=CARTESIAN_POINT('Ctrl Pts',(-56.0420505223762,-57.178961519516,
-217.190418744692));
#200660=CARTESIAN_POINT('Ctrl Pts',(-57.8597736100785,-60.2735586547801,
-214.03449525351));
#200661=CARTESIAN_POINT('',(-47.5799752941295,-40.2889415902933,-232.85005));
#200662=CARTESIAN_POINT('',(-47.0825542278859,-41.7715518798765,-232.850050000968));
#200663=CARTESIAN_POINT('Ctrl Pts',(-47.5799752940314,-40.288941592692,
-232.85005));
#200664=CARTESIAN_POINT('Ctrl Pts',(-47.5775945735834,-40.3473480102004,
-232.85005));
#200665=CARTESIAN_POINT('Ctrl Pts',(-47.5746791399089,-40.3934055205313,
-232.85005));
#200666=CARTESIAN_POINT('Ctrl Pts',(-47.5660677925892,-40.4699741882521,
-232.85005));
#200667=CARTESIAN_POINT('Ctrl Pts',(-47.5635310902827,-40.4915421253747,
-232.850049999998));
#200668=CARTESIAN_POINT('Ctrl Pts',(-47.553195697107,-40.5727355795072,
-232.850049999998));
#200669=CARTESIAN_POINT('Ctrl Pts',(-47.5435314536243,-40.6342224880465,
-232.85005));
#200670=CARTESIAN_POINT('Ctrl Pts',(-47.4988634642814,-40.8512217221034,
-232.85005));
#200671=CARTESIAN_POINT('Ctrl Pts',(-47.4667238043787,-40.9561283632504,
-232.850050000041));
#200672=CARTESIAN_POINT('Ctrl Pts',(-47.4103530291719,-41.1136517563645,
-232.850050000041));
#200673=CARTESIAN_POINT('Ctrl Pts',(-47.388468896712,-41.1712462227268,
-232.850050000436));
#200674=CARTESIAN_POINT('Ctrl Pts',(-47.3415687150509,-41.2863061139755,
-232.850050000436));
#200675=CARTESIAN_POINT('Ctrl Pts',(-47.3098061173323,-41.3563636665165,
-232.850049999917));
#200676=CARTESIAN_POINT('Ctrl Pts',(-47.2385354932108,-41.4987551854794,
-232.850049999917));
#200677=CARTESIAN_POINT('Ctrl Pts',(-47.2078203686635,-41.5594829943073,
-232.850050000009));
#200678=CARTESIAN_POINT('Ctrl Pts',(-47.1722887236253,-41.6240970450122,
-232.850050000009));
#200679=CARTESIAN_POINT('Ctrl Pts',(-47.1600291819146,-41.6454764697112,
-232.85005));
#200680=CARTESIAN_POINT('Ctrl Pts',(-47.126386710567,-41.7020987848978,
-232.85005));
#200681=CARTESIAN_POINT('Ctrl Pts',(-47.1037445725666,-41.7383217641524,
-232.85005));
#200682=CARTESIAN_POINT('Ctrl Pts',(-47.0825542565969,-41.7715518684048,
-232.85005));
#200683=CARTESIAN_POINT('',(-59.5781472511572,-54.5406860123134,-214.555282751782));
#200684=CARTESIAN_POINT('Ctrl Pts',(-47.5799752942349,-40.2889415880665,
-232.85005));
#200685=CARTESIAN_POINT('Ctrl Pts',(-51.5792492625364,-45.0398156733569,
-226.7519456074));
#200686=CARTESIAN_POINT('Ctrl Pts',(-55.5786810873963,-49.7902940354523,
-220.653636556059));
#200687=CARTESIAN_POINT('Ctrl Pts',(-59.5781472511525,-54.540686011977,
-214.555282751822));
#200688=CARTESIAN_POINT('',(-59.5601545409129,-55.0066093843695,-214.536876504828));
#200689=CARTESIAN_POINT('Ctrl Pts',(-59.5601545409116,-55.0066093843695,
-214.53687650483));
#200690=CARTESIAN_POINT('Ctrl Pts',(-59.5631449158913,-54.928270959567,
-214.542949699432));
#200691=CARTESIAN_POINT('Ctrl Pts',(-59.566138639304,-54.8502579208168,
-214.547602707532));
#200692=CARTESIAN_POINT('Ctrl Pts',(-59.5721600832965,-54.6943310158058,
-214.553747671111));
#200693=CARTESIAN_POINT('Ctrl Pts',(-59.5751172054583,-54.6182288248312,
-214.555228314137));
#200694=CARTESIAN_POINT('Ctrl Pts',(-59.5781472511111,-54.540686012984,
-214.55528275182));
#200695=CARTESIAN_POINT('',(-57.733985310444,-60.0593815363208,-214.252907888001));
#200696=CARTESIAN_POINT('Ctrl Pts',(-59.5601545409136,-55.0066093843694,
-214.536876504827));
#200697=CARTESIAN_POINT('Ctrl Pts',(-59.5534103770657,-55.1832852782111,
-214.523179687618));
#200698=CARTESIAN_POINT('Ctrl Pts',(-59.5413857028285,-55.3595266936186,
-214.509940774979));
#200699=CARTESIAN_POINT('Ctrl Pts',(-59.5048392798775,-55.7306111572691,
-214.48359225017));
#200700=CARTESIAN_POINT('Ctrl Pts',(-59.4790426204911,-55.9255750604899,
-214.470456745239));
#200701=CARTESIAN_POINT('Ctrl Pts',(-59.4374186280887,-56.1761840160495,
-214.453298736124));
#200702=CARTESIAN_POINT('Ctrl Pts',(-59.4271923870096,-56.2341662571188,
-214.449364106516));
#200703=CARTESIAN_POINT('Ctrl Pts',(-59.3290041059246,-56.7600810924064,
-214.414327664565));
#200704=CARTESIAN_POINT('Ctrl Pts',(-59.2036000760255,-57.2212958977573,
-214.387817887296));
#200705=CARTESIAN_POINT('Ctrl Pts',(-58.9920439420377,-57.808059046763,
-214.354899874041));
#200706=CARTESIAN_POINT('Ctrl Pts',(-58.9383051097066,-57.9461281140529,
-214.347431324615));
#200707=CARTESIAN_POINT('Ctrl Pts',(-58.7834285639265,-58.3162123489879,
-214.328364513275));
#200708=CARTESIAN_POINT('Ctrl Pts',(-58.6754718372394,-58.5458967426817,
-214.316667298022));
#200709=CARTESIAN_POINT('Ctrl Pts',(-58.4793456692825,-58.9208033297017,
-214.298260215069));
#200710=CARTESIAN_POINT('Ctrl Pts',(-58.3955443144838,-59.0701807393182,
-214.291807992095));
#200711=CARTESIAN_POINT('Ctrl Pts',(-58.255439819926,-59.303876779064,-214.282137443959));
#200712=CARTESIAN_POINT('Ctrl Pts',(-58.2014468386663,-59.3905132232237,
-214.278624601648));
#200713=CARTESIAN_POINT('Ctrl Pts',(-58.0758641218483,-59.5844450019079,
-214.270199768697));
#200714=CARTESIAN_POINT('Ctrl Pts',(-58.0026577731471,-59.6923453371087,
-214.265296898901));
#200715=CARTESIAN_POINT('Ctrl Pts',(-57.8636814802857,-59.8874642716884,
-214.258285826271));
#200716=CARTESIAN_POINT('Ctrl Pts',(-57.7995878632373,-59.9740538268328,
-214.255565510063));
#200717=CARTESIAN_POINT('Ctrl Pts',(-57.7339853360531,-60.0593815526408,
-214.252907779837));
#200718=CARTESIAN_POINT('Ctrl Pts',(-47.0825542580294,-41.771551867666,
-232.85005));
#200719=CARTESIAN_POINT('Ctrl Pts',(-48.8467027002287,-44.8190048301195,
-229.757904206756));
#200720=CARTESIAN_POINT('Ctrl Pts',(-50.613532047441,-47.8643691189139,
-226.665199941971));
#200721=CARTESIAN_POINT('Ctrl Pts',(-54.1625939290642,-53.9611509924102,
-220.466183691575));
#200722=CARTESIAN_POINT('Ctrl Pts',(-55.944791066377,-57.0125677071401,
-217.359850769034));
#200723=CARTESIAN_POINT('Ctrl Pts',(-57.7339853814967,-60.059381488225,
-214.252907967141));
#200724=CARTESIAN_POINT('Ctrl Pts',(-26.4599578544128,-60.6835996873818,
-232.962469394759));
#200725=CARTESIAN_POINT('Ctrl Pts',(-27.3226882880111,-61.1109358874724,
-232.172413742166));
#200726=CARTESIAN_POINT('Ctrl Pts',(-28.1852243300615,-61.5385403473352,
-231.38229745923));
#200727=CARTESIAN_POINT('Ctrl Pts',(-29.0475520792886,-61.9664437404056,
-230.59212149004));
#200728=CARTESIAN_POINT('Ctrl Pts',(-29.9098798285159,-62.3943471334761,
-229.801945520851));
#200729=CARTESIAN_POINT('Ctrl Pts',(-30.7719992834121,-62.8225494254431,
-229.011709845514));
#200730=CARTESIAN_POINT('Ctrl Pts',(-31.6338956495273,-63.2510852212965,
-228.221416509758));
#200731=CARTESIAN_POINT('Ctrl Pts',(-33.3576883817577,-64.1081568130033,
-226.640829838246));
#200732=CARTESIAN_POINT('Ctrl Pts',(-35.0805895076854,-64.966557214572,
-225.060010587067));
#200733=CARTESIAN_POINT('Ctrl Pts',(-36.8024707859496,-65.826619215018,
-223.47899392047));
#200734=CARTESIAN_POINT('Ctrl Pts',(-40.2462333424779,-67.54674321591,-220.316960587274));
#200735=CARTESIAN_POINT('Ctrl Pts',(-43.6859139831841,-69.2733920499482,
-217.154070226751));
#200736=CARTESIAN_POINT('Ctrl Pts',(-47.1204141132129,-71.0104275193633,
-213.991161055977));
#200737=CARTESIAN_POINT('Ctrl Pts',(-26.3821787340349,-60.7171127522114,
-232.969564324364));
#200738=CARTESIAN_POINT('Ctrl Pts',(-27.2445605117317,-61.1462290233331,
-232.178536730278));
#200739=CARTESIAN_POINT('Ctrl Pts',(-28.1068458309989,-61.5755390840377,
-231.387516472179));
#200740=CARTESIAN_POINT('Ctrl Pts',(-28.9690444318655,-62.0050437616364,
-230.596514709636));
#200741=CARTESIAN_POINT('Ctrl Pts',(-29.8312430327322,-62.4345484392352,
-229.805512947091));
#200742=CARTESIAN_POINT('Ctrl Pts',(-30.6933548791156,-62.8642478097168,
-229.014529680654));
#200743=CARTESIAN_POINT('Ctrl Pts',(-31.5553928365677,-63.294139004949,
-228.223577554036));
#200744=CARTESIAN_POINT('Ctrl Pts',(-33.279468751472,-64.1539213954133,
-226.641673300801));
#200745=CARTESIAN_POINT('Ctrl Pts',(-35.0032446885496,-65.0144779934189,
-225.059892398919));
#200746=CARTESIAN_POINT('Ctrl Pts',(-36.7268700953622,-65.8757200976626,
-223.47835238333));
#200747=CARTESIAN_POINT('Ctrl Pts',(-40.1741209089872,-67.59820430615,-220.315272352152));
#200748=CARTESIAN_POINT('Ctrl Pts',(-43.6206707171006,-69.3236781200416,
-217.153178316448));
#200749=CARTESIAN_POINT('Ctrl Pts',(-47.0687185474759,-71.0494058698413,
-213.993041121244));
#200750=CARTESIAN_POINT('Ctrl Pts',(-26.3336571985367,-60.7298615784681,
-232.97989189577));
#200751=CARTESIAN_POINT('Ctrl Pts',(-27.1935442176352,-61.1624605165825,
-232.187307357553));
#200752=CARTESIAN_POINT('Ctrl Pts',(-28.0535703090899,-61.5950514826745,
-231.3948845311));
#200753=CARTESIAN_POINT('Ctrl Pts',(-28.9137915870808,-62.0275803216354,
-230.60265649712));
#200754=CARTESIAN_POINT('Ctrl Pts',(-29.7740128650717,-62.4601091605963,
-229.810428463141));
#200755=CARTESIAN_POINT('Ctrl Pts',(-30.6344288831099,-62.8925758112263,
-229.018394694299));
#200756=CARTESIAN_POINT('Ctrl Pts',(-31.4950740297321,-63.3249356024725,
-228.226569298064));
#200757=CARTESIAN_POINT('Ctrl Pts',(-33.2163643229766,-64.189655184965,
-226.642918505594));
#200758=CARTESIAN_POINT('Ctrl Pts',(-34.9385811609418,-65.0539386080163,
-225.060107632614));
#200759=CARTESIAN_POINT('Ctrl Pts',(-36.6618273110172,-65.9175410966594,
-223.478119078272));
#200760=CARTESIAN_POINT('Ctrl Pts',(-40.108319611168,-67.6447460739454,
-220.314141969587));
#200761=CARTESIAN_POINT('Ctrl Pts',(-43.5589622053215,-69.3691553263065,
-217.153452097777));
#200762=CARTESIAN_POINT('Ctrl Pts',(-47.01332562737,-71.0901106229208,-213.995220045295));
#200763=CARTESIAN_POINT('Ctrl Pts',(-26.2982843226441,-60.7344827742712,
-232.991392546795));
#200764=CARTESIAN_POINT('Ctrl Pts',(-27.1539710903761,-61.1717772412952,
-232.196575481186));
#200765=CARTESIAN_POINT('Ctrl Pts',(-28.0105205110111,-61.6084763232924,
-231.402405653547));
#200766=CARTESIAN_POINT('Ctrl Pts',(-28.8678178196021,-62.0446142255719,
-230.608774353877));
#200767=CARTESIAN_POINT('Ctrl Pts',(-29.725115128193,-62.4807521278514,
-229.815143054206));
#200768=CARTESIAN_POINT('Ctrl Pts',(-30.5831604852668,-62.9163290490967,
-229.022050566726));
#200769=CARTESIAN_POINT('Ctrl Pts',(-31.441855894783,-63.3513820288522,
-228.22940826535));
#200770=CARTESIAN_POINT('Ctrl Pts',(-33.1592467138153,-64.2214879883631,
-226.644123662598));
#200771=CARTESIAN_POINT('Ctrl Pts',(-34.879225924468,-65.0894996057218,
-225.060627483752));
#200772=CARTESIAN_POINT('Ctrl Pts',(-36.6011749254936,-65.955713208232,
-223.478393801851));
#200773=CARTESIAN_POINT('Ctrl Pts',(-40.045072927545,-67.6881404132524,
-220.313926438049));
#200774=CARTESIAN_POINT('Ctrl Pts',(-43.4967433028155,-69.4134193510673,
-217.154414312055));
#200775=CARTESIAN_POINT('Ctrl Pts',(-46.9530675926807,-71.1335421841428,
-213.997473502442));
#200776=CARTESIAN_POINT('Ctrl Pts',(-26.2629114467516,-60.7391039700744,
-233.002893197821));
#200777=CARTESIAN_POINT('Ctrl Pts',(-27.114397963117,-61.1810939660079,
-232.20584360482));
#200778=CARTESIAN_POINT('Ctrl Pts',(-27.9674707129322,-61.6219011639104,
-231.409926775993));
#200779=CARTESIAN_POINT('Ctrl Pts',(-28.8218440521233,-62.0616481295084,
-230.614892210633));
#200780=CARTESIAN_POINT('Ctrl Pts',(-29.6762173913143,-62.5013950951064,
-229.819857645272));
#200781=CARTESIAN_POINT('Ctrl Pts',(-30.5318920874236,-62.9400822869671,
-229.025706439153));
#200782=CARTESIAN_POINT('Ctrl Pts',(-31.3886377598337,-63.3778284552318,
-228.232247232636));
#200783=CARTESIAN_POINT('Ctrl Pts',(-33.102129104654,-64.2533207917612,
-226.645328819602));
#200784=CARTESIAN_POINT('Ctrl Pts',(-34.8198706879942,-65.1250606034272,
-225.061147334889));
#200785=CARTESIAN_POINT('Ctrl Pts',(-36.5405225399701,-65.9938853198046,
-223.478668525429));
#200786=CARTESIAN_POINT('Ctrl Pts',(-39.981826243922,-67.7315347525594,
-220.313710906511));
#200787=CARTESIAN_POINT('Ctrl Pts',(-43.4345244003096,-69.457683375828,
-217.155376526334));
#200788=CARTESIAN_POINT('Ctrl Pts',(-46.8928095579913,-71.1769737453648,
-213.999726959588));
#200789=CARTESIAN_POINT('Ctrl Pts',(-26.2384700826335,-60.7381106363183,
-233.014375819121));
#200790=CARTESIAN_POINT('Ctrl Pts',(-27.0842500022742,-61.1857245057431,
-232.21450624766));
#200791=CARTESIAN_POINT('Ctrl Pts',(-27.9329490724857,-61.6311192767247,
-231.416680870253));
#200792=CARTESIAN_POINT('Ctrl Pts',(-28.7837425502454,-62.0747440392428,
-230.620229257902));
#200793=CARTESIAN_POINT('Ctrl Pts',(-29.634536028005,-62.5183688017608,
-229.82377764555));
#200794=CARTESIAN_POINT('Ctrl Pts',(-30.487432035617,-62.960223154147,-229.028708571446));
#200795=CARTESIAN_POINT('Ctrl Pts',(-31.3418749575762,-63.4006637505655,
-228.234599595102));
#200796=CARTESIAN_POINT('Ctrl Pts',(-33.0507608014949,-64.2815449434024,
-226.646381642412));
#200797=CARTESIAN_POINT('Ctrl Pts',(-34.7657386962016,-65.1568306952181,
-225.061930422221));
#200798=CARTESIAN_POINT('Ctrl Pts',(-36.4842100442897,-66.0284770468812,
-223.479425721276));
#200799=CARTESIAN_POINT('Ctrl Pts',(-39.9211527404658,-67.7717697502073,
-220.314416319386));
#200800=CARTESIAN_POINT('Ctrl Pts',(-43.3717095799881,-69.5008533336608,
-217.156983031728));
#200801=CARTESIAN_POINT('Ctrl Pts',(-46.827583501196,-71.2232650351743,
-214.002012001263));
#200802=CARTESIAN_POINT('Ctrl Pts',(-26.1949495995768,-60.7559954632254,
-233.015310708939));
#200803=CARTESIAN_POINT('Ctrl Pts',(-27.0387644538443,-61.2057327308231,
-232.215070168042));
#200804=CARTESIAN_POINT('Ctrl Pts',(-27.8858336675415,-61.6529664487026,
-231.417079914153));
#200805=CARTESIAN_POINT('Ctrl Pts',(-28.7351647823697,-62.0982646553384,
-230.620551354198));
#200806=CARTESIAN_POINT('Ctrl Pts',(-29.5844958971979,-62.5435628619743,
-229.824022794242));
#200807=CARTESIAN_POINT('Ctrl Pts',(-30.4361008904608,-62.9869237960558,
-229.028968199982));
#200808=CARTESIAN_POINT('Ctrl Pts',(-31.2893382107612,-63.4287766497893,
-228.234911333144));
#200809=CARTESIAN_POINT('Ctrl Pts',(-32.9958128513619,-64.3124823572563,
-226.646797599469));
#200810=CARTESIAN_POINT('Ctrl Pts',(-34.7087066827471,-65.190229522585,
-225.062593091688));
#200811=CARTESIAN_POINT('Ctrl Pts',(-36.425148099657,-66.0642498543572,
-223.480334162157));
#200812=CARTESIAN_POINT('Ctrl Pts',(-39.8580309334768,-67.8122905179015,
-220.315816303095));
#200813=CARTESIAN_POINT('Ctrl Pts',(-43.304744476869,-69.545794357118,-217.158884043615));
#200814=CARTESIAN_POINT('Ctrl Pts',(-46.7566079538913,-71.2728084364657,
-214.004305067604));
#200815=CARTESIAN_POINT('Ctrl Pts',(-26.1079086334631,-60.7917651170397,
-233.017180488577));
#200816=CARTESIAN_POINT('Ctrl Pts',(-26.9477933569846,-61.2457491809832,
-232.216198008803));
#200817=CARTESIAN_POINT('Ctrl Pts',(-27.791602857653,-61.6966607926582,
-231.417878001952));
#200818=CARTESIAN_POINT('Ctrl Pts',(-28.6380092466183,-62.1453058875298,
-230.62119554679));
#200819=CARTESIAN_POINT('Ctrl Pts',(-29.4844156355837,-62.5939509824013,
-229.824513091628));
#200820=CARTESIAN_POINT('Ctrl Pts',(-30.3334386001484,-63.0403250798734,
-229.029487457053));
#200821=CARTESIAN_POINT('Ctrl Pts',(-31.1842647171309,-63.485002448237,
-228.23553480923));
#200822=CARTESIAN_POINT('Ctrl Pts',(-32.8859169510958,-64.3743571849642,
-226.647629513582));
#200823=CARTESIAN_POINT('Ctrl Pts',(-34.5946426558381,-65.2570271773188,
-225.063918430622));
#200824=CARTESIAN_POINT('Ctrl Pts',(-36.3070242103916,-66.1357954693092,
-223.482151043919));
#200825=CARTESIAN_POINT('Ctrl Pts',(-39.7317873194987,-67.8933320532899,
-220.318616270514));
#200826=CARTESIAN_POINT('Ctrl Pts',(-43.1708142706306,-69.6356764040323,
-217.162686067389));
#200827=CARTESIAN_POINT('Ctrl Pts',(-46.6146568592818,-71.3718952390485,
-214.008891200286));
#200828=CARTESIAN_POINT('Ctrl Pts',(-26.0271556717183,-60.8195050993445,
-233.023057709875));
#200829=CARTESIAN_POINT('Ctrl Pts',(-26.8614803279425,-61.2789736199002,
-232.220907138713));
#200830=CARTESIAN_POINT('Ctrl Pts',(-27.7006372905616,-61.7344790137215,
-231.421952061255));
#200831=CARTESIAN_POINT('Ctrl Pts',(-28.5430811002764,-62.1870353929875,
-230.62500928173));
#200832=CARTESIAN_POINT('Ctrl Pts',(-29.3855249099912,-62.6395917722535,
-229.828066502204));
#200833=CARTESIAN_POINT('Ctrl Pts',(-30.2312298015655,-63.0892242106365,
-229.033124256632));
#200834=CARTESIAN_POINT('Ctrl Pts',(-31.0790619662469,-63.5367969787612,
-228.239400097671));
#200835=CARTESIAN_POINT('Ctrl Pts',(-32.7747262956096,-64.4319425150107,
-226.651951779748));
#200836=CARTESIAN_POINT('Ctrl Pts',(-34.4786705837165,-65.3190393016261,
-225.069228384841));
#200837=CARTESIAN_POINT('Ctrl Pts',(-36.1863583725991,-66.202056470716,
-223.488410098027));
#200838=CARTESIAN_POINT('Ctrl Pts',(-39.6017339503642,-67.9680908088958,
-220.326773524398));
#200839=CARTESIAN_POINT('Ctrl Pts',(-43.0317527614028,-69.7182854025588,
-217.172664187274));
#200840=CARTESIAN_POINT('Ctrl Pts',(-46.4657689946141,-71.4633532268859,
-214.020279084284));
#200841=CARTESIAN_POINT('Ctrl Pts',(-25.9715990783732,-60.8263824397187,
-233.038076562284));
#200842=CARTESIAN_POINT('Ctrl Pts',(-26.7915895883623,-61.2972176688764,
-232.2311442104));
#200843=CARTESIAN_POINT('Ctrl Pts',(-27.6213469993979,-61.7602848222496,
-231.430540367037));
#200844=CARTESIAN_POINT('Ctrl Pts',(-28.4556335624375,-62.2192160084591,
-230.63258019833));
#200845=CARTESIAN_POINT('Ctrl Pts',(-29.289920125477,-62.6781471946685,
-229.834620029623));
#200846=CARTESIAN_POINT('Ctrl Pts',(-30.1289511322075,-63.1328363273331,
-229.039478997096));
#200847=CARTESIAN_POINT('Ctrl Pts',(-30.9705439434446,-63.5850360083551,
-228.245754373682));
#200848=CARTESIAN_POINT('Ctrl Pts',(-32.6537295659188,-64.4894353703992,
-226.658305126855));
#200849=CARTESIAN_POINT('Ctrl Pts',(-34.3469173915073,-65.3841225672083,
-225.076391213479));
#200850=CARTESIAN_POINT('Ctrl Pts',(-36.0437616605612,-66.2748188763012,
-223.496282027351));
#200851=CARTESIAN_POINT('Ctrl Pts',(-39.4374501986691,-68.0562114944868,
-220.336063655097));
#200852=CARTESIAN_POINT('Ctrl Pts',(-42.8459482063409,-69.8217123813687,
-217.183304075329));
#200853=CARTESIAN_POINT('Ctrl Pts',(-46.2577049582974,-71.5830236206181,
-214.031928620936));
#200854=CARTESIAN_POINT('Ctrl Pts',(-25.9160424850282,-60.8332597800929,
-233.053095414693));
#200855=CARTESIAN_POINT('Ctrl Pts',(-26.7216988487821,-61.3154617178527,
-232.241381282086));
#200856=CARTESIAN_POINT('Ctrl Pts',(-27.5420567082342,-61.7860906307777,
-231.439128672818));
#200857=CARTESIAN_POINT('Ctrl Pts',(-28.3681860245984,-62.2513966239306,
-230.64015111493));
#200858=CARTESIAN_POINT('Ctrl Pts',(-29.1943153409628,-62.7167026170834,
-229.841173557043));
#200859=CARTESIAN_POINT('Ctrl Pts',(-30.0266724628494,-63.1764484440297,
-229.045833737559));
#200860=CARTESIAN_POINT('Ctrl Pts',(-30.8620259206422,-63.633275037949,
-228.252108649693));
#200861=CARTESIAN_POINT('Ctrl Pts',(-32.5327328362278,-64.5469282257876,
-226.664658473961));
#200862=CARTESIAN_POINT('Ctrl Pts',(-34.215164199298,-65.4492058327905,
-225.083554042117));
#200863=CARTESIAN_POINT('Ctrl Pts',(-35.9011649485234,-66.3475812818863,
-223.504153956677));
#200864=CARTESIAN_POINT('Ctrl Pts',(-39.273166446974,-68.1443321800779,
-220.345353785796));
#200865=CARTESIAN_POINT('Ctrl Pts',(-42.6601436512792,-69.9251393601785,
-217.193943963384));
#200866=CARTESIAN_POINT('Ctrl Pts',(-46.0496409219808,-71.7026940143502,
-214.043578157589));
#200867=CARTESIAN_POINT('Ctrl Pts',(-25.8665286108953,-60.8381274420046,
-233.066411683095));
#200868=CARTESIAN_POINT('Ctrl Pts',(-26.6581633289744,-61.3291620138588,
-232.251762724729));
#200869=CARTESIAN_POINT('Ctrl Pts',(-27.4689810980677,-61.805659144746,
-231.449321410308));
#200870=CARTESIAN_POINT('Ctrl Pts',(-28.2858283440085,-62.276644660254,
-230.650185251577));
#200871=CARTESIAN_POINT('Ctrl Pts',(-29.1026755899493,-62.747630175762,
-229.851049092846));
#200872=CARTESIAN_POINT('Ctrl Pts',(-29.9264514304638,-63.2126139436637,
-229.055899144978));
#200873=CARTESIAN_POINT('Ctrl Pts',(-30.7532556538434,-63.6747328220346,
-228.26235895591));
#200874=CARTESIAN_POINT('Ctrl Pts',(-32.4068641006027,-64.5989705787766,
-226.675278577774));
#200875=CARTESIAN_POINT('Ctrl Pts',(-34.0724444645535,-65.5119690076117,
-225.094611701508));
#200876=CARTESIAN_POINT('Ctrl Pts',(-35.7413375761177,-66.4214664741137,
-223.515524234354));
#200877=CARTESIAN_POINT('Ctrl Pts',(-39.0791237992462,-68.2404614071178,
-220.357349300048));
#200878=CARTESIAN_POINT('Ctrl Pts',(-42.4312557792835,-70.0447514385552,
-217.206261484219));
#200879=CARTESIAN_POINT('Ctrl Pts',(-45.7856616296808,-71.8461945922107,
-214.056132477959));
#200880=CARTESIAN_POINT('Ctrl Pts',(-25.8011224073928,-60.8541224995348,
-233.072388186401));
#200881=CARTESIAN_POINT('Ctrl Pts',(-26.5882772139689,-61.345584476566,
-232.260902563554));
#200882=CARTESIAN_POINT('Ctrl Pts',(-27.3926111430279,-61.824140301072,
-231.460141397784));
#200883=CARTESIAN_POINT('Ctrl Pts',(-28.2023317845711,-62.2979002023416,
-230.662317129508));
#200884=CARTESIAN_POINT('Ctrl Pts',(-29.0120524261143,-62.7716601036112,
-229.864492861231));
#200885=CARTESIAN_POINT('Ctrl Pts',(-29.8279705672755,-63.2401673093096,
-229.070199114559));
#200886=CARTESIAN_POINT('Ctrl Pts',(-30.6466000725898,-63.7061844369386,
-228.277344321055));
#200887=CARTESIAN_POINT('Ctrl Pts',(-32.2838590832184,-64.6382186921966,
-226.691634734048));
#200888=CARTESIAN_POINT('Ctrl Pts',(-33.9318380253269,-65.5604762032412,
-225.111654172302));
#200889=CARTESIAN_POINT('Ctrl Pts',(-35.582792800409,-66.4797047104531,
-223.533108945327));
#200890=CARTESIAN_POINT('Ctrl Pts',(-38.884702350573,-68.3181617248767,
-220.376018491376));
#200891=CARTESIAN_POINT('Ctrl Pts',(-42.1994895547755,-70.143871943617,
-217.225335489343));
#200892=CARTESIAN_POINT('Ctrl Pts',(-45.5163300351324,-71.9671084389128,
-214.075544244624));
#200893=CARTESIAN_POINT('Ctrl Pts',(-25.7357162038904,-60.870117557065,
-233.078364689706));
#200894=CARTESIAN_POINT('Ctrl Pts',(-26.5183910989635,-61.3620069392732,
-232.270042402379));
#200895=CARTESIAN_POINT('Ctrl Pts',(-27.3162411879881,-61.842621457398,
-231.470961385261));
#200896=CARTESIAN_POINT('Ctrl Pts',(-28.1188352251337,-62.3191557444292,
-230.674449007438));
#200897=CARTESIAN_POINT('Ctrl Pts',(-28.9214292622792,-62.7956900314603,
-229.877936629616));
#200898=CARTESIAN_POINT('Ctrl Pts',(-29.7294897040872,-63.2677206749556,
-229.084499084141));
#200899=CARTESIAN_POINT('Ctrl Pts',(-30.5399444913362,-63.7376360518426,
-228.292329686201));
#200900=CARTESIAN_POINT('Ctrl Pts',(-32.1608540658341,-64.6774668056166,
-226.707990890321));
#200901=CARTESIAN_POINT('Ctrl Pts',(-33.7912315861003,-65.6089833988707,
-225.128696643096));
#200902=CARTESIAN_POINT('Ctrl Pts',(-35.4242480247001,-66.5379429467924,
-223.550693656299));
#200903=CARTESIAN_POINT('Ctrl Pts',(-38.6902809018998,-68.3958620426357,
-220.394687682705));
#200904=CARTESIAN_POINT('Ctrl Pts',(-41.9677233302676,-70.2429924486788,
-217.244409494466));
#200905=CARTESIAN_POINT('Ctrl Pts',(-45.2469984405841,-72.088022285615,
-214.09495601129));
#200906=CARTESIAN_POINT('Ctrl Pts',(-25.6764457543321,-60.8781185651427,
-233.089415099072));
#200907=CARTESIAN_POINT('Ctrl Pts',(-26.4517816472997,-61.3719375798059,
-232.282825348105));
#200908=CARTESIAN_POINT('Ctrl Pts',(-27.2411241731431,-61.8556224049542,
-231.484690141905));
#200909=CARTESIAN_POINT('Ctrl Pts',(-28.0348403941315,-62.3356735301276,
-230.688923056315));
#200910=CARTESIAN_POINT('Ctrl Pts',(-28.8285566151198,-62.8157246553009,
-229.893155970723));
#200911=CARTESIAN_POINT('Ctrl Pts',(-29.6273152575741,-63.2917540571251,
-229.100216973599));
#200912=CARTESIAN_POINT('Ctrl Pts',(-30.4282830173054,-63.7659009259987,
-228.308450386598));
#200913=CARTESIAN_POINT('Ctrl Pts',(-32.0302185367682,-64.7141946637459,
-226.724917212596));
#200914=CARTESIAN_POINT('Ctrl Pts',(-33.6408900276233,-65.6550862143651,
-225.14604576641));
#200915=CARTESIAN_POINT('Ctrl Pts',(-35.2539988230218,-66.5937075233338,
-223.568378062868));
#200916=CARTESIAN_POINT('Ctrl Pts',(-38.4802164138187,-68.4709501412712,
-220.413042655783));
#200917=CARTESIAN_POINT('Ctrl Pts',(-41.7169696970508,-70.3386046036742,
-217.263033043788));
#200918=CARTESIAN_POINT('Ctrl Pts',(-44.9554183644225,-72.2043881447385,
-214.113800504198));
#200919=CARTESIAN_POINT('Ctrl Pts',(-25.6298304748707,-60.8753734341798,
-233.107177069033));
#200920=CARTESIAN_POINT('Ctrl Pts',(-26.3965314717851,-61.3714239166506,
-232.301492490062));
#200921=CARTESIAN_POINT('Ctrl Pts',(-27.1765365083298,-61.8582017525339,
-231.503828898795));
#200922=CARTESIAN_POINT('Ctrl Pts',(-27.960699151696,-62.3416685933693,
-230.708430592375));
#200923=CARTESIAN_POINT('Ctrl Pts',(-28.7448617950622,-62.8251354342047,
-229.913032285956));
#200924=CARTESIAN_POINT('Ctrl Pts',(-29.5338172036037,-63.3049330183218,
-229.120332249855));
#200925=CARTESIAN_POINT('Ctrl Pts',(-30.3248744392529,-63.7830152939694,
-228.328756578445));
#200926=CARTESIAN_POINT('Ctrl Pts',(-31.9069889105511,-64.7391798452646,
-226.745605235623));
#200927=CARTESIAN_POINT('Ctrl Pts',(-33.4974147722857,-65.6885985452027,
-225.166922566632));
#200928=CARTESIAN_POINT('Ctrl Pts',(-35.0901638016772,-66.6359498673557,
-223.589403428947));
#200929=CARTESIAN_POINT('Ctrl Pts',(-38.2756618604604,-68.5306525116616,
-220.434365153576));
#200930=CARTESIAN_POINT('Ctrl Pts',(-41.4711974327502,-70.4166207416591,
-217.284462017333));
#200931=CARTESIAN_POINT('Ctrl Pts',(-44.6683526580257,-72.3008817462311,
-214.135317230106));
#200932=CARTESIAN_POINT('Ctrl Pts',(-25.5832151954094,-60.8726283032168,
-233.124939038994));
#200933=CARTESIAN_POINT('Ctrl Pts',(-26.3412812962705,-61.3709102534954,
-232.320159632019));
#200934=CARTESIAN_POINT('Ctrl Pts',(-27.1119488435164,-61.8607811001136,
-231.522967655684));
#200935=CARTESIAN_POINT('Ctrl Pts',(-27.8865579092606,-62.347663656611,
-230.727938128436));
#200936=CARTESIAN_POINT('Ctrl Pts',(-28.6611669750047,-62.8345462131084,
-229.932908601188));
#200937=CARTESIAN_POINT('Ctrl Pts',(-29.4403191496334,-63.3181119795184,
-229.140447526113));
#200938=CARTESIAN_POINT('Ctrl Pts',(-30.2214658612003,-63.8001296619401,
-228.349062770292));
#200939=CARTESIAN_POINT('Ctrl Pts',(-31.783759284334,-64.7641650267834,
-226.766293258651));
#200940=CARTESIAN_POINT('Ctrl Pts',(-33.353939516948,-65.7221108760403,
-225.187799366854));
#200941=CARTESIAN_POINT('Ctrl Pts',(-34.9263287803327,-66.6781922113775,
-223.610428795026));
#200942=CARTESIAN_POINT('Ctrl Pts',(-38.071107307102,-68.590354882052,-220.455687651369));
#200943=CARTESIAN_POINT('Ctrl Pts',(-41.2254251684497,-70.494636879644,
-217.305890990877));
#200944=CARTESIAN_POINT('Ctrl Pts',(-44.381286951629,-72.3973753477236,
-214.156833956015));
#200945=CARTESIAN_POINT('Ctrl Pts',(-25.5332663260497,-60.8715565679525,
-233.140620047442));
#200946=CARTESIAN_POINT('Ctrl Pts',(-26.2846593466459,-61.3702751859077,
-232.337976743902));
#200947=CARTESIAN_POINT('Ctrl Pts',(-27.0470683275914,-61.861877181739,
-231.541902635733));
#200948=CARTESIAN_POINT('Ctrl Pts',(-27.8129663979903,-62.3509604518928,
-230.747753285103));
#200949=CARTESIAN_POINT('Ctrl Pts',(-28.5788644683892,-62.8400437220466,
-229.953603934473));
#200950=CARTESIAN_POINT('Ctrl Pts',(-29.3487694431048,-63.3263269973223,
-229.161720142653));
#200951=CARTESIAN_POINT('Ctrl Pts',(-30.120445915247,-63.8113027794608,
-228.370799649172));
#200952=CARTESIAN_POINT('Ctrl Pts',(-31.6637988595316,-64.7812543437376,
-226.788958662211));
#200953=CARTESIAN_POINT('Ctrl Pts',(-33.2141526002521,-65.7460617730361,
-225.210938813702));
#200954=CARTESIAN_POINT('Ctrl Pts',(-34.7664868193848,-66.7092887992816,
-223.633944018777));
#200955=CARTESIAN_POINT('Ctrl Pts',(-37.8711552576499,-68.6357428517727,
-220.479954428925));
#200956=CARTESIAN_POINT('Ctrl Pts',(-40.9843522069086,-70.555519752599,
-217.330448431736));
#200957=CARTESIAN_POINT('Ctrl Pts',(-44.0989468098099,-72.4739730046678,
-214.18163152198));
#200958=CARTESIAN_POINT('Ctrl Pts',(-25.4734681104549,-60.8745649395491,
-233.152705479171));
#200959=CARTESIAN_POINT('Ctrl Pts',(-26.2191301593905,-61.3728030581697,
-232.352982827705));
#200960=CARTESIAN_POINT('Ctrl Pts',(-26.9737314089713,-61.8653651155087,
-231.558531400184));
#200961=CARTESIAN_POINT('Ctrl Pts',(-27.7312103498245,-62.3559170177131,
-230.765669056017));
#200962=CARTESIAN_POINT('Ctrl Pts',(-28.4886892906776,-62.8464689199175,
-229.972806711851));
#200963=CARTESIAN_POINT('Ctrl Pts',(-29.2494572009032,-63.3347856810085,
-229.181797847991));
#200964=CARTESIAN_POINT('Ctrl Pts',(-30.0116917876015,-63.8220563583486,
-228.391588810695));
#200965=CARTESIAN_POINT('Ctrl Pts',(-31.5361609609982,-64.7965977130286,
-226.811170736103));
#200966=CARTESIAN_POINT('Ctrl Pts',(-33.0664220838837,-65.7670232712464,
-225.233920858118));
#200967=CARTESIAN_POINT('Ctrl Pts',(-34.5983413220466,-66.7361768147042,
-223.657538786233));
#200968=CARTESIAN_POINT('Ctrl Pts',(-37.6621797983723,-68.6744839016197,
-220.504774642461));
#200969=CARTESIAN_POINT('Ctrl Pts',(-40.7331349268486,-70.6074216926982,
-217.355782960055));
#200970=CARTESIAN_POINT('Ctrl Pts',(-43.8052734509942,-72.5392749729601,
-214.207386766717));
#200971=CARTESIAN_POINT('Ctrl Pts',(-25.4136698948603,-60.8775733111457,
-233.1647909109));
#200972=CARTESIAN_POINT('Ctrl Pts',(-26.1536009721352,-61.3753309304317,
-232.367988911507));
#200973=CARTESIAN_POINT('Ctrl Pts',(-26.9003944903513,-61.8688530492783,
-231.575160164634));
#200974=CARTESIAN_POINT('Ctrl Pts',(-27.6494543016586,-62.3608735835334,
-230.783584826932));
#200975=CARTESIAN_POINT('Ctrl Pts',(-28.3985141129659,-62.8528941177885,
-229.992009489228));
#200976=CARTESIAN_POINT('Ctrl Pts',(-29.1501449587015,-63.3432443646947,
-229.201875553329));
#200977=CARTESIAN_POINT('Ctrl Pts',(-29.902937659956,-63.8328099372364,
-228.412377972218));
#200978=CARTESIAN_POINT('Ctrl Pts',(-31.4085230624649,-64.8119410823196,
-226.833382809995));
#200979=CARTESIAN_POINT('Ctrl Pts',(-32.9186915675153,-65.7879847694566,
-225.256902902535));
#200980=CARTESIAN_POINT('Ctrl Pts',(-34.4301958247084,-66.7630648301267,
-223.681133553689));
#200981=CARTESIAN_POINT('Ctrl Pts',(-37.4532043390948,-68.7132249514667,
-220.529594855996));
#200982=CARTESIAN_POINT('Ctrl Pts',(-40.4819176467888,-70.6593236327973,
-217.381117488375));
#200983=CARTESIAN_POINT('Ctrl Pts',(-43.5116000921785,-72.6045769412523,
-214.233142011455));
#200984=CARTESIAN_POINT('Ctrl Pts',(-25.3604578094675,-60.8735170241007,
-233.18242034351));
#200985=CARTESIAN_POINT('Ctrl Pts',(-26.0930283102741,-61.3713501637903,
-232.387708547763));
#200986=CARTESIAN_POINT('Ctrl Pts',(-26.8307495672501,-61.866135521907,
-231.595979029253));
#200987=CARTESIAN_POINT('Ctrl Pts',(-27.5702957875313,-62.3597741472074,
-230.805269005779));
#200988=CARTESIAN_POINT('Ctrl Pts',(-28.3098420078126,-62.8534127725078,
-230.014558982304));
#200989=CARTESIAN_POINT('Ctrl Pts',(-29.0514176428578,-63.3457952241198,
-229.224993612889));
#200990=CARTESIAN_POINT('Ctrl Pts',(-29.7939421742496,-63.8375690870219,
-228.435953327864));
#200991=CARTESIAN_POINT('Ctrl Pts',(-31.2789912370331,-64.8211168128261,
-226.857872757815));
#200992=CARTESIAN_POINT('Ctrl Pts',(-32.767772611159,-65.8022749106513,
-225.281860356042));
#200993=CARTESIAN_POINT('Ctrl Pts',(-34.2576895400343,-66.7826561972701,
-223.706461237247));
#200994=CARTESIAN_POINT('Ctrl Pts',(-37.237523397785,-68.7434187705077,
-220.555662999657));
#200995=CARTESIAN_POINT('Ctrl Pts',(-40.2221506876178,-70.7009385693032,
-217.407470987453));
#200996=CARTESIAN_POINT('Ctrl Pts',(-43.2076329024777,-72.657747925151,
-214.259730555427));
#200997=CARTESIAN_POINT('Ctrl Pts',(-25.3082796911041,-60.8654535469475,
-233.203637421846));
#200998=CARTESIAN_POINT('Ctrl Pts',(-26.0341343285133,-61.3629238744168,
-232.411039848471));
#200999=CARTESIAN_POINT('Ctrl Pts',(-26.7636013838676,-61.8583152760603,
-231.620533187723));
#201000=CARTESIAN_POINT('Ctrl Pts',(-27.4944243031966,-62.3528874641244,
-230.830789824077));
#201001=CARTESIAN_POINT('Ctrl Pts',(-28.2252472225255,-62.8474596521885,
-230.041046460431));
#201002=CARTESIAN_POINT('Ctrl Pts',(-28.9575562895767,-63.3411438699236,
-229.252145525666));
#201003=CARTESIAN_POINT('Ctrl Pts',(-29.6905827327532,-63.8343860369735,
-228.463645185323));
#201004=CARTESIAN_POINT('Ctrl Pts',(-31.1566356191065,-64.8208703710732,
-226.886644504638));
#201005=CARTESIAN_POINT('Ctrl Pts',(-32.6255046561051,-65.8056211821729,
-225.311217867621));
#201006=CARTESIAN_POINT('Ctrl Pts',(-34.0952688014063,-66.7897856212239,
-223.736281731367));
#201007=CARTESIAN_POINT('Ctrl Pts',(-37.034797092009,-68.7581144993257,
-220.58640945886));
#201008=CARTESIAN_POINT('Ctrl Pts',(-39.9780639773415,-70.7240153450236,
-217.438595831035));
#201009=CARTESIAN_POINT('Ctrl Pts',(-42.922034708619,-72.6893523415957,
-214.291161723059));
#201010=CARTESIAN_POINT('Ctrl Pts',(-25.2821906319223,-60.8614218083708,
-233.214245961014));
#201011=CARTESIAN_POINT('Ctrl Pts',(-26.0046873376329,-61.35871072973,-232.422705498826));
#201012=CARTESIAN_POINT('Ctrl Pts',(-26.7300272921764,-61.854405153137,
-231.632810266957));
#201013=CARTESIAN_POINT('Ctrl Pts',(-27.4564885610292,-62.3494441225829,
-230.843550233226));
#201014=CARTESIAN_POINT('Ctrl Pts',(-28.182949829882,-62.8444830920289,
-230.054290199494));
#201015=CARTESIAN_POINT('Ctrl Pts',(-28.9106256129361,-63.3388181928255,
-229.265721482054));
#201016=CARTESIAN_POINT('Ctrl Pts',(-29.6389030120051,-63.8327945119493,
-228.477491114052));
#201017=CARTESIAN_POINT('Ctrl Pts',(-31.0954578101431,-64.8207471501967,
-226.901030378049));
#201018=CARTESIAN_POINT('Ctrl Pts',(-32.5543706785782,-65.8072943179338,
-225.32589662341));
#201019=CARTESIAN_POINT('Ctrl Pts',(-34.0140584320924,-66.7933503332008,
-223.751191978427));
#201020=CARTESIAN_POINT('Ctrl Pts',(-36.933433939121,-68.7654623637348,
-220.60178268846));
#201021=CARTESIAN_POINT('Ctrl Pts',(-39.8560206222034,-70.7355537328838,
-217.454158252827));
#201022=CARTESIAN_POINT('Ctrl Pts',(-42.7792356116896,-72.705154549818,
-214.306877306875));
#201023=CARTESIAN_POINT('Ctrl Pts',(-25.2542808545004,-60.8576193179734,
-233.224589731722));
#201024=CARTESIAN_POINT('Ctrl Pts',(-25.9733613508541,-61.3547669345154,
-232.433994495002));
#201025=CARTESIAN_POINT('Ctrl Pts',(-26.6946341378572,-61.850707669122,
-231.644667681488));
#201026=CARTESIAN_POINT('Ctrl Pts',(-27.4168149846347,-62.3461306013993,
-230.855857430941));
#201027=CARTESIAN_POINT('Ctrl Pts',(-28.1389958314122,-62.8415535336766,
-230.067047180394));
#201028=CARTESIAN_POINT('Ctrl Pts',(-28.8621498208122,-63.3364251861756,
-229.278792485017));
#201029=CARTESIAN_POINT('Ctrl Pts',(-29.5857994425194,-63.8310086087711,
-228.490817987778));
#201030=CARTESIAN_POINT('Ctrl Pts',(-31.0330986859336,-64.8201754539622,
-226.914868993301));
#201031=CARTESIAN_POINT('Ctrl Pts',(-32.482338164911,-65.8082141619607,
-225.340017314949));
#201032=CARTESIAN_POINT('Ctrl Pts',(-33.9322394111677,-66.7958442294134,
-223.765535080096));
#201033=CARTESIAN_POINT('Ctrl Pts',(-36.8320419036812,-68.771104364319,
-220.61657061039));
#201034=CARTESIAN_POINT('Ctrl Pts',(-39.7345648061665,-70.7446942844296,
-217.469129121935));
#201035=CARTESIAN_POINT('Ctrl Pts',(-42.637644247718,-72.7178586955381,
-214.321995277256));
#201036=CARTESIAN_POINT('Ctrl Pts',(-25.2239774050683,-60.8541676049626,
-233.234470884236));
#201037=CARTESIAN_POINT('Ctrl Pts',(-25.9398083842247,-61.3511430455559,
-232.444758300872));
#201038=CARTESIAN_POINT('Ctrl Pts',(-26.6572825734193,-61.8472255929447,
-231.655996189968));
#201039=CARTESIAN_POINT('Ctrl Pts',(-27.3754647705453,-62.3429113806012,
-230.867638000096));
#201040=CARTESIAN_POINT('Ctrl Pts',(-28.0936469676712,-62.8385971682577,
-230.079279810225));
#201041=CARTESIAN_POINT('Ctrl Pts',(-28.8125820204444,-63.3338632665416,
-229.291352292986));
#201042=CARTESIAN_POINT('Ctrl Pts',(-29.5319096752348,-63.8289050323554,
-228.503647571677));
#201043=CARTESIAN_POINT('Ctrl Pts',(-30.9705649848157,-64.8189885639829,
-226.928238129057));
#201044=CARTESIAN_POINT('Ctrl Pts',(-32.4107560406701,-65.8081944618785,
-225.353700434162));
#201045=CARTESIAN_POINT('Ctrl Pts',(-33.8514884032197,-66.7970717553631,
-223.779466811102));
#201046=CARTESIAN_POINT('Ctrl Pts',(-36.732953128319,-68.7748263423323,
-220.630999564983));
#201047=CARTESIAN_POINT('Ctrl Pts',(-39.6166287632978,-70.7512448922044,
-217.483776946995));
#201048=CARTESIAN_POINT('Ctrl Pts',(-42.5007756355285,-72.7273057434785,
-214.336817183699));
#201049=CARTESIAN_POINT('Ctrl Pts',(-25.1936739556362,-60.8507158919519,
-233.244352036751));
#201050=CARTESIAN_POINT('Ctrl Pts',(-25.9062554175954,-61.3475191565963,
-232.455522106742));
#201051=CARTESIAN_POINT('Ctrl Pts',(-26.6199310089813,-61.8437435167674,
-231.667324698448));
#201052=CARTESIAN_POINT('Ctrl Pts',(-27.3341145564557,-62.3396921598031,
-230.879418569252));
#201053=CARTESIAN_POINT('Ctrl Pts',(-28.0482981039303,-62.8356408028389,
-230.091512440055));
#201054=CARTESIAN_POINT('Ctrl Pts',(-28.7630142200764,-63.3313013469077,
-229.303912100956));
#201055=CARTESIAN_POINT('Ctrl Pts',(-29.4780199079502,-63.8268014559396,
-228.516477155575));
#201056=CARTESIAN_POINT('Ctrl Pts',(-30.9080312836978,-64.8178016740036,
-226.941607264814));
#201057=CARTESIAN_POINT('Ctrl Pts',(-32.3391739164292,-65.8081747617964,
-225.367383553375));
#201058=CARTESIAN_POINT('Ctrl Pts',(-33.7707373952718,-66.7982992813128,
-223.793398542109));
#201059=CARTESIAN_POINT('Ctrl Pts',(-36.6338643529568,-68.7785483203456,
-220.645428519576));
#201060=CARTESIAN_POINT('Ctrl Pts',(-39.498692720429,-70.7577954999793,
-217.498424772054));
#201061=CARTESIAN_POINT('Ctrl Pts',(-42.363907023339,-72.7367527914189,
-214.351639090142));
#201062=CARTESIAN_POINT('Ctrl Pts',(-25.1598238196964,-60.8482202385386,
-233.25309688913));
#201063=CARTESIAN_POINT('Ctrl Pts',(-25.8694641248229,-61.3447486920278,
-232.465168808441));
#201064=CARTESIAN_POINT('Ctrl Pts',(-26.5797195835393,-61.8409546524082,
-231.677595750858));
#201065=CARTESIAN_POINT('Ctrl Pts',(-27.2902792575572,-62.3369977131888,
-230.890197499475));
#201066=CARTESIAN_POINT('Ctrl Pts',(-28.000838931575,-62.8330407739693,
-230.102799248092));
#201067=CARTESIAN_POINT('Ctrl Pts',(-28.711714550991,-63.3289150112138,
-229.315582660731));
#201068=CARTESIAN_POINT('Ctrl Pts',(-29.4227692929209,-63.8246912312197,
-228.528468791165));
#201069=CARTESIAN_POINT('Ctrl Pts',(-30.8448787767808,-64.8162436712314,
-226.954241052034));
#201070=CARTESIAN_POINT('Ctrl Pts',(-32.2676879017602,-65.8074128718581,
-225.380414529439));
#201071=CARTESIAN_POINT('Ctrl Pts',(-33.6907733702002,-66.7984195359043,
-223.806745992614));
#201072=CARTESIAN_POINT('Ctrl Pts',(-36.5369443070804,-68.7804328639968,
-220.659408918962));
#201073=CARTESIAN_POINT('Ctrl Pts',(-39.3842222584393,-70.7617958073898,
-217.512705107097));
#201074=CARTESIAN_POINT('Ctrl Pts',(-42.2317710074449,-72.7429480158072,
-214.366156356611));
#201075=CARTESIAN_POINT('Ctrl Pts',(-25.1256029177818,-60.8447964462213,
-233.262708527412));
#201076=CARTESIAN_POINT('Ctrl Pts',(-25.8323432559684,-61.3411439778804,
-232.475469715128));
#201077=CARTESIAN_POINT('Ctrl Pts',(-26.5393879179131,-61.8373317659467,
-231.688406549544));
#201078=CARTESIAN_POINT('Ctrl Pts',(-27.2465878469089,-62.3334358738351,
-230.90143275512));
#201079=CARTESIAN_POINT('Ctrl Pts',(-27.9537877759048,-62.8295399817235,
-230.114458960696));
#201080=CARTESIAN_POINT('Ctrl Pts',(-28.6611482655484,-63.3255577393973,
-229.327577621181));
#201081=CARTESIAN_POINT('Ctrl Pts',(-29.3686016850915,-63.8215238522036,
-228.540749713863));
#201082=CARTESIAN_POINT('Ctrl Pts',(-30.7835085241778,-64.8134560778162,
-226.967093899227));
#201083=CARTESIAN_POINT('Ctrl Pts',(-32.198778370749,-65.8051862301184,
-225.3936468087));
#201084=CARTESIAN_POINT('Ctrl Pts',(-33.6141958867398,-66.7968253706499,
-223.820284551445));
#201085=CARTESIAN_POINT('Ctrl Pts',(-36.4450309187215,-68.7801036517128,
-220.673560036935));
#201086=CARTESIAN_POINT('Ctrl Pts',(-39.2764551401188,-70.7630188613062,
-217.527174130311));
#201087=CARTESIAN_POINT('Ctrl Pts',(-42.1080287367154,-72.7457990899024,
-214.3808746454));
#201088=CARTESIAN_POINT('Ctrl Pts',(-25.0913820158672,-60.8413726539041,
-233.272320165694));
#201089=CARTESIAN_POINT('Ctrl Pts',(-25.7952223871138,-61.337539263733,
-232.485770621816));
#201090=CARTESIAN_POINT('Ctrl Pts',(-26.4990562522867,-61.8337088794851,
-231.699217348229));
#201091=CARTESIAN_POINT('Ctrl Pts',(-27.2028964362607,-62.3298740344814,
-230.912668010765));
#201092=CARTESIAN_POINT('Ctrl Pts',(-27.9067366202345,-62.8260391894777,
-230.126118673301));
#201093=CARTESIAN_POINT('Ctrl Pts',(-28.6105819801057,-63.3222004675808,
-229.339572581631));
#201094=CARTESIAN_POINT('Ctrl Pts',(-29.314434077262,-63.8183564731875,
-228.553030636562));
#201095=CARTESIAN_POINT('Ctrl Pts',(-30.7221382715748,-64.8106684844009,
-226.97994674642));
#201096=CARTESIAN_POINT('Ctrl Pts',(-32.1298688397377,-65.8029595883788,
-225.406879087961));
#201097=CARTESIAN_POINT('Ctrl Pts',(-33.5376184032793,-66.7952312053955,
-223.833823110276));
#201098=CARTESIAN_POINT('Ctrl Pts',(-36.3531175303626,-68.7797744394288,
-220.687711154908));
#201099=CARTESIAN_POINT('Ctrl Pts',(-39.1686880217984,-70.7642419152226,
-217.541643153526));
#201100=CARTESIAN_POINT('Ctrl Pts',(-41.9842864659859,-72.7486501639975,
-214.39559293419));
#201101=CARTESIAN_POINT('Ctrl Pts',(-25.0620255817184,-60.8342761915281,
-233.285941631018));
#201102=CARTESIAN_POINT('Ctrl Pts',(-25.7623705261304,-61.3306758976375,
-232.499505184585));
#201103=CARTESIAN_POINT('Ctrl Pts',(-26.4626944173704,-61.8270835434123,
-231.713056538299));
#201104=CARTESIAN_POINT('Ctrl Pts',(-27.1630058058958,-62.3234949649194,
-230.926600669881));
#201105=CARTESIAN_POINT('Ctrl Pts',(-27.8633171944211,-62.8199063864266,
-230.140144801462));
#201106=CARTESIAN_POINT('Ctrl Pts',(-28.5636158753459,-63.3163216831959,
-229.353681591601));
#201107=CARTESIAN_POINT('Ctrl Pts',(-29.2639064106539,-63.8127386310709,
-228.567213695831));
#201108=CARTESIAN_POINT('Ctrl Pts',(-30.6644874812699,-64.8055725268209,
-226.994277904292));
#201109=CARTESIAN_POINT('Ctrl Pts',(-32.0650366774472,-65.7984126816902,
-225.421323781149));
#201110=CARTESIAN_POINT('Ctrl Pts',(-33.4655708458739,-66.7912508691866,
-223.848361132451));
#201111=CARTESIAN_POINT('Ctrl Pts',(-36.2666391827274,-68.7769272441794,
-220.702435835054));
#201112=CARTESIAN_POINT('Ctrl Pts',(-39.0676484327315,-70.7625952457594,
-217.556477030254));
#201113=CARTESIAN_POINT('Ctrl Pts',(-41.8686390590285,-72.7482350521135,
-214.410508283843));
#201114=CARTESIAN_POINT('Ctrl Pts',(-25.028605078732,-60.8264461849104,
-233.300589177504));
#201115=CARTESIAN_POINT('Ctrl Pts',(-25.7257590504183,-61.3230773961178,
-232.514138876127));
#201116=CARTESIAN_POINT('Ctrl Pts',(-26.4228956738429,-61.8197151427821,
-231.727678440368));
#201117=CARTESIAN_POINT('Ctrl Pts',(-27.1200213189657,-62.3163563966737,
-230.941211605428));
#201118=CARTESIAN_POINT('Ctrl Pts',(-27.8171469640885,-62.8129976505652,
-230.154744770487));
#201119=CARTESIAN_POINT('Ctrl Pts',(-28.514261502952,-63.3096424726104,
-229.368271461406));
#201120=CARTESIAN_POINT('Ctrl Pts',(-29.2113685617452,-63.8062891397564,
-228.581793805278));
#201121=CARTESIAN_POINT('Ctrl Pts',(-30.6055826793317,-64.7995824740485,
-227.008838493021));
#201122=CARTESIAN_POINT('Ctrl Pts',(-31.9997674609787,-65.7928829112188,
-225.435866135329));
#201123=CARTESIAN_POINT('Ctrl Pts',(-33.393937296167,-66.786183616434,-223.862885177104));
#201124=CARTESIAN_POINT('Ctrl Pts',(-36.1822769665438,-68.7727850268643,
-220.716923260653));
#201125=CARTESIAN_POINT('Ctrl Pts',(-38.9705580867346,-70.7593869240872,
-217.570927667784));
#201126=CARTESIAN_POINT('Ctrl Pts',(-41.7588188049893,-72.745971187409,
-214.424920813073));
#201127=CARTESIAN_POINT('Ctrl Pts',(-25.0118948272389,-60.8225311816015,
-233.307912950748));
#201128=CARTESIAN_POINT('Ctrl Pts',(-25.7074533125622,-61.319278145358,
-232.521455721897));
#201129=CARTESIAN_POINT('Ctrl Pts',(-26.4029963020791,-61.8160309424671,
-231.734989391403));
#201130=CARTESIAN_POINT('Ctrl Pts',(-27.0985290755007,-62.3127871125508,
-230.948517073201));
#201131=CARTESIAN_POINT('Ctrl Pts',(-27.7940618489222,-62.8095432826346,
-230.162044755));
#201132=CARTESIAN_POINT('Ctrl Pts',(-28.489584316755,-63.3063028673177,
-229.375566396309));
#201133=CARTESIAN_POINT('Ctrl Pts',(-29.1850996372909,-63.8030643940992,
-228.589083860001));
#201134=CARTESIAN_POINT('Ctrl Pts',(-30.5761302783625,-64.7965874476622,
-227.016118787385));
#201135=CARTESIAN_POINT('Ctrl Pts',(-31.9671328527444,-65.7901180259831,
-225.443137312419));
#201136=CARTESIAN_POINT('Ctrl Pts',(-33.3581205213136,-66.7836499900577,
-223.870147199431));
#201137=CARTESIAN_POINT('Ctrl Pts',(-36.140095858452,-68.7707139182068,
-220.724166973453));
#201138=CARTESIAN_POINT('Ctrl Pts',(-38.9220129137361,-70.7577827632511,
-217.578152986549));
#201139=CARTESIAN_POINT('Ctrl Pts',(-41.7039086779697,-72.7448392550568,
-214.432127077688));
#201140=CARTESIAN_POINT('Ctrl Pts',(-24.9941555235601,-60.8184248975328,
-233.315484141906));
#201141=CARTESIAN_POINT('Ctrl Pts',(-25.6881907528502,-61.3152906961552,
-232.528985905911));
#201142=CARTESIAN_POINT('Ctrl Pts',(-26.3822204946216,-61.8121578773183,
-231.74248442401));
#201143=CARTESIAN_POINT('Ctrl Pts',(-27.0762463009327,-62.3090257464567,
-230.955980624069));
#201144=CARTESIAN_POINT('Ctrl Pts',(-27.7702721072438,-62.8058936155951,
-230.169476824128));
#201145=CARTESIAN_POINT('Ctrl Pts',(-28.4642939595846,-63.3027621809775,
-229.382970695078));
#201146=CARTESIAN_POINT('Ctrl Pts',(-29.1583128779801,-63.7996309859099,
-228.596462846723));
#201147=CARTESIAN_POINT('Ctrl Pts',(-30.5463507147712,-64.7933685957745,
-227.023447150014));
#201148=CARTESIAN_POINT('Ctrl Pts',(-31.9343769856396,-65.7871070878229,
-225.450424677593));
#201149=CARTESIAN_POINT('Ctrl Pts',(-33.3223964166864,-66.7808443446069,
-223.877398255344));
#201150=CARTESIAN_POINT('Ctrl Pts',(-36.0984352787801,-68.768318858175,
-220.731345410844));
#201151=CARTESIAN_POINT('Ctrl Pts',(-38.8744474110663,-70.7557881486592,
-217.585277143015));
#201152=CARTESIAN_POINT('Ctrl Pts',(-41.6504481618404,-72.7432453287128,
-214.439202637353));
#201153=CARTESIAN_POINT('Ctrl Pts',(-24.9744025307133,-60.8143487212353,
-233.322986925177));
#201154=CARTESIAN_POINT('Ctrl Pts',(-25.6670491804662,-61.3113173869818,
-232.536442059561));
#201155=CARTESIAN_POINT('Ctrl Pts',(-26.3596977749792,-61.8082844221729,
-231.749898382092));
#201156=CARTESIAN_POINT('Ctrl Pts',(-27.0523477402915,-62.3052500852752,
-230.96335555072));
#201157=CARTESIAN_POINT('Ctrl Pts',(-27.7449977056038,-62.8022157483775,
-230.176812719347));
#201158=CARTESIAN_POINT('Ctrl Pts',(-28.4376490490292,-63.2991800360968,
-229.390270738434));
#201159=CARTESIAN_POINT('Ctrl Pts',(-29.1303013990492,-63.7961431156999,
-228.603729386647));
#201160=CARTESIAN_POINT('Ctrl Pts',(-30.5156060990893,-64.7900692749063,
-227.030646683075));
#201161=CARTESIAN_POINT('Ctrl Pts',(-31.9009147636639,-65.7839906295158,
-225.45756645914));
#201162=CARTESIAN_POINT('Ctrl Pts',(-33.2862256991509,-66.777907941617,
-223.884487706564));
#201163=CARTESIAN_POINT('Ctrl Pts',(-36.0568475701252,-68.7657425658195,
-220.738330201412));
#201164=CARTESIAN_POINT('Ctrl Pts',(-38.827478307619,-70.7535611178629,
-217.592178452254));
#201165=CARTESIAN_POINT('Ctrl Pts',(-41.5981125175426,-72.7413660196969,
-214.446029255158));
#201166=CARTESIAN_POINT('Ctrl Pts',(-24.96452603429,-60.8123106330865,-233.326738316813));
#201167=CARTESIAN_POINT('Ctrl Pts',(-25.6564783942742,-61.3093307323952,
-232.540170136386));
#201168=CARTESIAN_POINT('Ctrl Pts',(-26.3484364151579,-61.8063476946002,
-231.753605361133));
#201169=CARTESIAN_POINT('Ctrl Pts',(-27.0403984599708,-62.3033622546844,
-230.967043014045));
#201170=CARTESIAN_POINT('Ctrl Pts',(-27.7323605047837,-62.8003768147686,
-230.180480666957));
#201171=CARTESIAN_POINT('Ctrl Pts',(-28.4243265937515,-63.2973889636564,
-229.393920760111));
#201172=CARTESIAN_POINT('Ctrl Pts',(-29.1162956595838,-63.794399180595,
-228.607362656609));
#201173=CARTESIAN_POINT('Ctrl Pts',(-30.5002337912484,-64.7884196144722,
-227.034246449605));
#201174=CARTESIAN_POINT('Ctrl Pts',(-31.8841836526759,-65.7824324003622,
-225.461137349913));
#201175=CARTESIAN_POINT('Ctrl Pts',(-33.2681403403832,-66.7764397401221,
-223.888032432174));
#201176=CARTESIAN_POINT('Ctrl Pts',(-36.0360537157978,-68.7644544196418,
-220.741822596696));
#201177=CARTESIAN_POINT('Ctrl Pts',(-38.8039937558954,-70.7524476024647,
-217.595629106873));
#201178=CARTESIAN_POINT('Ctrl Pts',(-41.5719446953938,-72.740426365189,
-214.449442564061));
#201179=CARTESIAN_POINT('Ctrl Pts',(-24.9541490838557,-60.8102778631162,
-233.330474075949));
#201180=CARTESIAN_POINT('Ctrl Pts',(-25.6454401441992,-61.307345800731,
-232.543880802852));
#201181=CARTESIAN_POINT('Ctrl Pts',(-26.3367401731056,-61.8044093273887,
-231.757292929005));
#201182=CARTESIAN_POINT('Ctrl Pts',(-27.0280467391398,-62.3014695196208,
-230.970708996412));
#201183=CARTESIAN_POINT('Ctrl Pts',(-27.719353305174,-62.7985297118529,
-230.18412506382));
#201184=CARTESIAN_POINT('Ctrl Pts',(-28.4106664345268,-63.2955865581015,
-229.397545088212));
#201185=CARTESIAN_POINT('Ctrl Pts',(-29.1019844928396,-63.7926407824983,
-228.610968089891));
#201186=CARTESIAN_POINT('Ctrl Pts',(-30.4846206094652,-64.7867492312918,
-227.037814093248));
#201187=CARTESIAN_POINT('Ctrl Pts',(-31.8672761708201,-65.7808473127859,
-225.464671843211));
#201188=CARTESIAN_POINT('Ctrl Pts',(-33.2499434120597,-66.7749384699927,
-223.891536687223));
#201189=CARTESIAN_POINT('Ctrl Pts',(-36.0152778945389,-68.7631207844063,
-220.745266375246));
#201190=CARTESIAN_POINT('Ctrl Pts',(-38.7806580129467,-70.7512758829813,
-217.599023790475));
#201191=CARTESIAN_POINT('Ctrl Pts',(-41.5460576771974,-72.7394153448676,
-214.45279331175));
#201192=CARTESIAN_POINT('Ctrl Pts',(-24.9431675857188,-60.8082654676189,
-233.334164524199));
#201193=CARTESIAN_POINT('Ctrl Pts',(-25.6338346604351,-61.3053771897629,
-232.547545996672));
#201194=CARTESIAN_POINT('Ctrl Pts',(-26.3245132764945,-61.8024835845448,
-231.760934436748));
#201195=CARTESIAN_POINT('Ctrl Pts',(-27.0152005013104,-62.2995859346266,
-230.97432807854));
#201196=CARTESIAN_POINT('Ctrl Pts',(-27.7058877261263,-62.7966882847084,
-230.187721720333));
#201197=CARTESIAN_POINT('Ctrl Pts',(-28.3965835877948,-63.2937865778419,
-229.401120580787));
#201198=CARTESIAN_POINT('Ctrl Pts',(-29.0872860637793,-63.7908816992324,
-228.614523442413));
#201199=CARTESIAN_POINT('Ctrl Pts',(-30.4686910157482,-64.7850719420134,
-227.041329165664));
#201200=CARTESIAN_POINT('Ctrl Pts',(-31.8501220936262,-65.7792496428099,
-225.468150694098));
#201201=CARTESIAN_POINT('Ctrl Pts',(-33.231569388313,-66.7734191417836,
-223.894982065188));
#201202=CARTESIAN_POINT('Ctrl Pts',(-35.9944639776866,-68.7617581397308,
-220.748644807367));
#201203=CARTESIAN_POINT('Ctrl Pts',(-38.7574219835962,-70.7500649666192,
-217.602346047653));
#201204=CARTESIAN_POINT('Ctrl Pts',(-41.5204085705364,-72.7383548951067,
-214.45606483788));
#201205=CARTESIAN_POINT('Ctrl Pts',(-24.9376768366503,-60.8072592698702,
-233.336009748324));
#201206=CARTESIAN_POINT('Ctrl Pts',(-25.6280319185531,-61.3043928842789,
-232.549378593582));
#201207=CARTESIAN_POINT('Ctrl Pts',(-26.318399828189,-61.8015207131228,
-231.762755190619));
#201208=CARTESIAN_POINT('Ctrl Pts',(-27.0087773823957,-62.2986441421295,
-230.976137619604));
#201209=CARTESIAN_POINT('Ctrl Pts',(-27.6991549366024,-62.7957675711362,
-230.189520048589));
#201210=CARTESIAN_POINT('Ctrl Pts',(-28.3895421644288,-63.2928865877122,
-229.402908327074));
#201211=CARTESIAN_POINT('Ctrl Pts',(-29.0799368492491,-63.7900021575995,
-228.616301118674));
#201212=CARTESIAN_POINT('Ctrl Pts',(-30.4607262188897,-64.7842332973742,
-227.043086701871));
#201213=CARTESIAN_POINT('Ctrl Pts',(-31.8415450550293,-65.778450807822,
-225.469890119541));
#201214=CARTESIAN_POINT('Ctrl Pts',(-33.2223823764397,-66.772659477679,
-223.89670475417));
#201215=CARTESIAN_POINT('Ctrl Pts',(-35.9840570192604,-68.7610768173931,
-220.750334023428));
#201216=CARTESIAN_POINT('Ctrl Pts',(-38.7458039689211,-70.7494595084382,
-217.604007176241));
#201217=CARTESIAN_POINT('Ctrl Pts',(-41.5075840172059,-72.7378246702262,
-214.457700600944));
#201218=CARTESIAN_POINT('Ctrl Pts',(-24.9320351560731,-60.8062580406183,
-233.337843753845));
#201219=CARTESIAN_POINT('Ctrl Pts',(-25.6220875425827,-61.3034125499849,
-232.551199913808));
#201220=CARTESIAN_POINT('Ctrl Pts',(-26.312153866782,-61.8005609014255,
-231.764564507522));
#201221=CARTESIAN_POINT('Ctrl Pts',(-27.0022307652976,-62.2977045512317,
-230.977935502733));
#201222=CARTESIAN_POINT('Ctrl Pts',(-27.6923076638132,-62.794848201038,
-230.191306497943));
#201223=CARTESIAN_POINT('Ctrl Pts',(-28.3823951656622,-63.2919871367077,
-229.404683912223));
#201224=CARTESIAN_POINT('Ctrl Pts',(-29.0724909030316,-63.7891223844269,
-228.618066315475));
#201225=CARTESIAN_POINT('Ctrl Pts',(-30.4526823777702,-64.7833928798651,
-227.044831121978));
#201226=CARTESIAN_POINT('Ctrl Pts',(-31.8329064109243,-65.7776487896842,
-225.471615652582));
#201227=CARTESIAN_POINT('Ctrl Pts',(-33.2131511215727,-66.7718952685571,
-223.898412735151));
#201228=CARTESIAN_POINT('Ctrl Pts',(-35.9736405428697,-68.7603882263028,
-220.752006900292));
#201229=CARTESIAN_POINT('Ctrl Pts',(-38.7342108749039,-70.7488442420639,
-217.605650187832));
#201230=CARTESIAN_POINT('Ctrl Pts',(-41.4948189193303,-72.737282086382,
-214.459316539654));
#201231=CARTESIAN_POINT('Ctrl Pts',(-24.9262307371789,-60.8052629613404,
-233.339663481057));
#201232=CARTESIAN_POINT('Ctrl Pts',(-25.6159901042832,-61.3024373924278,
-232.553007006783));
#201233=CARTESIAN_POINT('Ctrl Pts',(-26.3057643351287,-61.7996053791141,
-231.766359540212));
#201234=CARTESIAN_POINT('Ctrl Pts',(-26.9955499476215,-62.2967684208872,
-230.979718973407));
#201235=CARTESIAN_POINT('Ctrl Pts',(-27.6853355601145,-62.7939314626603,
-230.193078406603));
#201236=CARTESIAN_POINT('Ctrl Pts',(-28.3751325826488,-63.2910895473583,
-229.406444756795));
#201237=CARTESIAN_POINT('Ctrl Pts',(-29.0649385371855,-63.7882437431482,
-228.619816524538));
#201238=CARTESIAN_POINT('Ctrl Pts',(-30.4445504462589,-64.7825521347279,
-227.046560060024));
#201239=CARTESIAN_POINT('Ctrl Pts',(-31.8241976850135,-65.7768451422546,
-225.473325024605));
#201240=CARTESIAN_POINT('Ctrl Pts',(-33.2038676569546,-66.7711282018108,
-223.90010380027));
#201241=CARTESIAN_POINT('Ctrl Pts',(-35.9632076008367,-68.7596943209232,
-220.753661351601));
#201242=CARTESIAN_POINT('Ctrl Pts',(-38.7226365397166,-70.7482214856064,
-217.607272976111));
#201243=CARTESIAN_POINT('Ctrl Pts',(-41.4821077889028,-72.7367298763208,
-214.460910461991));
#201244=CARTESIAN_POINT('Ctrl Pts',(-24.9204263182847,-60.8042678820624,
-233.341483208271));
#201245=CARTESIAN_POINT('Ctrl Pts',(-25.6098926659838,-61.3014622348707,
-232.554814099759));
#201246=CARTESIAN_POINT('Ctrl Pts',(-26.2993748034754,-61.7986498568027,
-231.768154572902));
#201247=CARTESIAN_POINT('Ctrl Pts',(-26.9888691299455,-62.2958322905427,
-230.981502444082));
#201248=CARTESIAN_POINT('Ctrl Pts',(-27.6783634564157,-62.7930147242826,
-230.194850315263));
#201249=CARTESIAN_POINT('Ctrl Pts',(-28.3678699996353,-63.2901919580089,
-229.408205601368));
#201250=CARTESIAN_POINT('Ctrl Pts',(-29.0573861713395,-63.7873651018695,
-228.621566733601));
#201251=CARTESIAN_POINT('Ctrl Pts',(-30.4364185147476,-64.7817113895908,
-227.048288998068));
#201252=CARTESIAN_POINT('Ctrl Pts',(-31.8154889591027,-65.776041494825,
-225.475034396628));
#201253=CARTESIAN_POINT('Ctrl Pts',(-33.1945841923364,-66.7703611350645,
-223.901794865388));
#201254=CARTESIAN_POINT('Ctrl Pts',(-35.9527746588037,-68.7590004155436,
-220.755315802909));
#201255=CARTESIAN_POINT('Ctrl Pts',(-38.7110622045295,-70.7475987291489,
-217.608895764391));
#201256=CARTESIAN_POINT('Ctrl Pts',(-41.4693966584753,-72.7361776662597,
-214.462504384327));
#201257=CARTESIAN_POINT('Ctrl Pts',(-24.9106027465158,-60.8049715273879,
-233.340948124015));
#201258=CARTESIAN_POINT('Ctrl Pts',(-25.5998098315156,-61.3021744082037,
-232.554282687331));
#201259=CARTESIAN_POINT('Ctrl Pts',(-26.2890324103538,-61.7993707608737,
-231.767626642701));
#201260=CARTESIAN_POINT('Ctrl Pts',(-26.9782669268481,-62.2965621103122,
-230.980977835653));
#201261=CARTESIAN_POINT('Ctrl Pts',(-27.6675014433422,-62.7937534597507,
-230.194329028605));
#201262=CARTESIAN_POINT('Ctrl Pts',(-28.3567479253494,-63.2909397940828,
-229.407687476061));
#201263=CARTESIAN_POINT('Ctrl Pts',(-29.0460038234333,-63.7881222076912,
-228.621051634203));
#201264=CARTESIAN_POINT('Ctrl Pts',(-30.424515619601,-64.7824870349079,
-227.047779950486));
#201265=CARTESIAN_POINT('Ctrl Pts',(-31.8030646725822,-65.776836354002,
-225.474530862664));
#201266=CARTESIAN_POINT('Ctrl Pts',(-33.1816379091815,-66.771175783969,
-223.901296458627));
#201267=CARTESIAN_POINT('Ctrl Pts',(-35.9387843823801,-68.759854643903,
-220.754827650554));
#201268=CARTESIAN_POINT('Ctrl Pts',(-38.6960255585086,-70.7484948217514,
-217.608416348934));
#201269=CARTESIAN_POINT('Ctrl Pts',(-41.4533123673286,-72.737117447414,
-214.462032879015));
#201270=CARTESIAN_POINT('Ctrl Pts',(-24.9017054131522,-60.8052918727755,
-233.340945144186));
#201271=CARTESIAN_POINT('Ctrl Pts',(-25.5906443745351,-61.3025059726095,
-232.554279700873));
#201272=CARTESIAN_POINT('Ctrl Pts',(-26.2795988326832,-61.7997136258234,
-231.767623645885));
#201273=CARTESIAN_POINT('Ctrl Pts',(-26.9685652314336,-62.2969163567666,
-230.980974825615));
#201274=CARTESIAN_POINT('Ctrl Pts',(-27.6575316301841,-62.7941190877098,
-230.194326005343));
#201275=CARTESIAN_POINT('Ctrl Pts',(-28.346509997394,-63.2913168845119,
-229.407684436704));
#201276=CARTESIAN_POINT('Ctrl Pts',(-29.0354977836505,-63.7885108411498,
-228.621048576497));
#201277=CARTESIAN_POINT('Ctrl Pts',(-30.4134733561636,-64.7828987544258,
-227.047776856082));
#201278=CARTESIAN_POINT('Ctrl Pts',(-31.7914861973683,-65.7772714817533,
-225.474527722644));
#201279=CARTESIAN_POINT('Ctrl Pts',(-33.1695232342839,-66.7716346400439,
-223.90129326724));
#201280=CARTESIAN_POINT('Ctrl Pts',(-35.925597308115,-68.7603609566252,
-220.754824356431));
#201281=CARTESIAN_POINT('Ctrl Pts',(-38.6817661332381,-70.749049871159,
-217.608412929565));
#201282=CARTESIAN_POINT('Ctrl Pts',(-41.437980641355,-72.7377225056729,
-214.462029323759));
#201283=CARTESIAN_POINT('',(-26.5827141673278,-60.7444095340058,-232.85005));
#201284=CARTESIAN_POINT('',(-25.3523897646956,-61.114818041723,-232.850050017304));
#201285=CARTESIAN_POINT('Ctrl Pts',(-26.5827141673278,-60.7444095340058,
-232.85005));
#201286=CARTESIAN_POINT('Ctrl Pts',(-26.5523883211155,-60.7606145810421,
-232.85005));
#201287=CARTESIAN_POINT('Ctrl Pts',(-26.5182436214773,-60.7785813873836,
-232.85005));
#201288=CARTESIAN_POINT('Ctrl Pts',(-26.4690256747712,-60.8033306143011,
-232.85005));
#201289=CARTESIAN_POINT('Ctrl Pts',(-26.4527133286803,-60.8112699859099,
-232.850050000173));
#201290=CARTESIAN_POINT('Ctrl Pts',(-26.3977210282154,-60.8370309306803,
-232.850050000173));
#201291=CARTESIAN_POINT('Ctrl Pts',(-26.3580453525237,-60.8538506884452,
-232.85005));
#201292=CARTESIAN_POINT('Ctrl Pts',(-26.2130644838343,-60.9164277579278,
-232.85005));
#201293=CARTESIAN_POINT('Ctrl Pts',(-26.1545198953832,-60.9398574595328,
-232.85005));
#201294=CARTESIAN_POINT('Ctrl Pts',(-26.0680132927756,-60.971650599673,
-232.85005));
#201295=CARTESIAN_POINT('Ctrl Pts',(-26.0182912512482,-60.9885178579036,
-232.850050000019));
#201296=CARTESIAN_POINT('Ctrl Pts',(-25.9539874352103,-61.0096287447273,
-232.850050000019));
#201297=CARTESIAN_POINT('Ctrl Pts',(-25.9240201650144,-61.019154825783,
-232.85005));
#201298=CARTESIAN_POINT('Ctrl Pts',(-25.8612333031519,-61.0378499416973,
-232.85005));
#201299=CARTESIAN_POINT('Ctrl Pts',(-25.8258381809542,-61.047112084847,
-232.85005));
#201300=CARTESIAN_POINT('Ctrl Pts',(-25.7621933691786,-61.0617509830125,
-232.85005));
#201301=CARTESIAN_POINT('Ctrl Pts',(-25.7424556613749,-61.0661234399878,
-232.850049999971));
#201302=CARTESIAN_POINT('Ctrl Pts',(-25.6672523478798,-61.0820029852263,
-232.850049999971));
#201303=CARTESIAN_POINT('Ctrl Pts',(-25.6192423246462,-61.0902478978104,
-232.850050000018));
#201304=CARTESIAN_POINT('Ctrl Pts',(-25.528905053629,-61.1015857089327,
-232.850050000018));
#201305=CARTESIAN_POINT('Ctrl Pts',(-25.4898697688722,-61.1058736055181,
-232.85005));
#201306=CARTESIAN_POINT('Ctrl Pts',(-25.4126689239331,-61.1125397549223,
-232.85005));
#201307=CARTESIAN_POINT('Ctrl Pts',(-25.3781594362844,-61.1138848746439,
-232.85005));
#201308=CARTESIAN_POINT('Ctrl Pts',(-25.3523897698351,-61.1148181836303,
-232.85005));
#201309=CARTESIAN_POINT('',(-46.8664918972107,-70.8820281131858,-214.224994829282));
#201310=CARTESIAN_POINT('Ctrl Pts',(-26.5827166022082,-60.7444082350379,
-232.85005));
#201311=CARTESIAN_POINT('Ctrl Pts',(-27.4045094191061,-61.1514998298357,
-232.097461865351));
#201312=CARTESIAN_POINT('Ctrl Pts',(-28.2261252496076,-61.5588361613065,
-231.344818757035));
#201313=CARTESIAN_POINT('Ctrl Pts',(-29.9098798269229,-62.3943471342904,
-229.801945520923));
#201314=CARTESIAN_POINT('Ctrl Pts',(-30.7719992818189,-62.8225494262878,
-229.011709845571));
#201315=CARTESIAN_POINT('Ctrl Pts',(-33.3576883801732,-64.1081568139303,
-226.640829838263));
#201316=CARTESIAN_POINT('Ctrl Pts',(-35.0805895061186,-64.9665572155428,
-225.060010587065));
#201317=CARTESIAN_POINT('Ctrl Pts',(-40.1613675899462,-67.5043536465696,
-220.39488359422));
#201318=CARTESIAN_POINT('Ctrl Pts',(-43.5163811847326,-69.1882952855583,
-217.309957960225));
#201319=CARTESIAN_POINT('Ctrl Pts',(-46.8664918972107,-70.8820281131858,
-214.224994829282));
#201320=CARTESIAN_POINT('',(-41.8937014876592,-72.6456596144325,-214.55018589167));
#201321=CARTESIAN_POINT('Ctrl Pts',(-46.8664918907845,-70.8820281261857,
-214.224994454969));
#201322=CARTESIAN_POINT('Ctrl Pts',(-46.7744407826033,-70.9511131613608,
-214.228242207603));
#201323=CARTESIAN_POINT('Ctrl Pts',(-46.680727279368,-71.0186224423001,
-214.231828155425));
#201324=CARTESIAN_POINT('Ctrl Pts',(-46.5495229902255,-71.1092838966998,
-214.237663532247));
#201325=CARTESIAN_POINT('Ctrl Pts',(-46.5126373769831,-71.1343646694262,
-214.239393263808));
#201326=CARTESIAN_POINT('Ctrl Pts',(-46.3057923036224,-71.2726997131669,
-214.249757794819));
#201327=CARTESIAN_POINT('Ctrl Pts',(-46.1254151593501,-71.3847351190163,
-214.258939730943));
#201328=CARTESIAN_POINT('Ctrl Pts',(-45.7687595214659,-71.5880113826264,
-214.27689821422));
#201329=CARTESIAN_POINT('Ctrl Pts',(-45.5977961983387,-71.6781131955288,
-214.286477772573));
#201330=CARTESIAN_POINT('Ctrl Pts',(-45.3185014968499,-71.8138089272529,
-214.303180439003));
#201331=CARTESIAN_POINT('Ctrl Pts',(-45.2120152032011,-71.8629654501139,
-214.309490070308));
#201332=CARTESIAN_POINT('Ctrl Pts',(-45.046199455701,-71.935548692169,-214.319240105057));
#201333=CARTESIAN_POINT('Ctrl Pts',(-44.9874097476947,-71.9605279868894,
-214.322717043323));
#201334=CARTESIAN_POINT('Ctrl Pts',(-44.7920434623916,-72.0410490489618,
-214.334469550289));
#201335=CARTESIAN_POINT('Ctrl Pts',(-44.6545819295426,-72.0937224742825,
-214.343103618652));
#201336=CARTESIAN_POINT('Ctrl Pts',(-44.0770061022199,-72.298643730271,
-214.380774049869));
#201337=CARTESIAN_POINT('Ctrl Pts',(-43.6246516197569,-72.4199541122146,
-214.411162580962));
#201338=CARTESIAN_POINT('Ctrl Pts',(-43.0535644966474,-72.5255358982375,
-214.454758498776));
#201339=CARTESIAN_POINT('Ctrl Pts',(-42.9403769882396,-72.5441841202125,
-214.463730404288));
#201340=CARTESIAN_POINT('Ctrl Pts',(-42.7453484949782,-72.5724398999914,
-214.479262989124));
#201341=CARTESIAN_POINT('Ctrl Pts',(-42.663500340452,-72.5831344326424,
-214.485726488472));
#201342=CARTESIAN_POINT('Ctrl Pts',(-42.3528138938661,-72.6193128180556,
-214.510537926913));
#201343=CARTESIAN_POINT('Ctrl Pts',(-42.123906167336,-72.6369493090122,
-214.52972492121));
#201344=CARTESIAN_POINT('Ctrl Pts',(-41.8937014876739,-72.6456596144296,
-214.550185891837));
#201345=CARTESIAN_POINT('',(-41.3748964727292,-72.6655519634609,-214.574036901741));
#201346=CARTESIAN_POINT('Ctrl Pts',(-41.8937014876741,-72.6456596144277,
-214.55018589184));
#201347=CARTESIAN_POINT('Ctrl Pts',(-41.8073293516378,-72.6489276960371,
-214.557862789404));
#201348=CARTESIAN_POINT('Ctrl Pts',(-41.7213837775228,-72.6521985331045,
-214.563823000958));
#201349=CARTESIAN_POINT('Ctrl Pts',(-41.5899590748613,-72.6572360335019,
-214.569961528013));
#201350=CARTESIAN_POINT('Ctrl Pts',(-41.5458704327232,-72.6589321169506,
-214.571508890137));
#201351=CARTESIAN_POINT('Ctrl Pts',(-41.4802081830395,-72.6614677335481,
-214.573029139169));
#201352=CARTESIAN_POINT('Ctrl Pts',(-41.4590018913533,-72.6622881096249,
-214.573399452815));
#201353=CARTESIAN_POINT('Ctrl Pts',(-41.4169705066586,-72.6639170467841,
-214.573893334939));
#201354=CARTESIAN_POINT('Ctrl Pts',(-41.4044675732566,-72.6644020926304,
-214.574005833637));
#201355=CARTESIAN_POINT('Ctrl Pts',(-41.3748964708024,-72.6655518905447,
-214.574037743505));
#201356=CARTESIAN_POINT('Ctrl Pts',(-25.3523897720292,-61.114817956777,
-232.850049970045));
#201357=CARTESIAN_POINT('Ctrl Pts',(-30.6926995480076,-64.965287483333,
-226.757725855014));
#201358=CARTESIAN_POINT('Ctrl Pts',(-36.0337490039693,-68.8154400690564,
-220.665850944208));
#201359=CARTESIAN_POINT('Ctrl Pts',(-41.3748962564069,-72.665551761209,
-214.574036584249));
#201360=CARTESIAN_POINT('Ctrl Pts',(-27.4675166955088,36.501209334595,-233.2699618027));
#201361=CARTESIAN_POINT('Ctrl Pts',(-28.0986597880893,36.9344896240505,
-232.484645254214));
#201362=CARTESIAN_POINT('Ctrl Pts',(-28.7300030462673,37.3676977230337,
-231.69945191414));
#201363=CARTESIAN_POINT('Ctrl Pts',(-29.3615087464634,37.8008474937043,
-230.914358703846));
#201364=CARTESIAN_POINT('Ctrl Pts',(-29.9930144466596,38.2339972643749,
-230.129265493552));
#201365=CARTESIAN_POINT('Ctrl Pts',(-30.624682800611,38.6670886387032,-229.344272547955));
#201366=CARTESIAN_POINT('Ctrl Pts',(-31.2564852375126,39.1001323034766,
-228.559362491382));
#201367=CARTESIAN_POINT('Ctrl Pts',(-32.5200901113159,39.9662196330235,
-226.989542378236));
#201368=CARTESIAN_POINT('Ctrl Pts',(-33.7842270188127,40.8321176985828,
-225.420051188828));
#201369=CARTESIAN_POINT('Ctrl Pts',(-35.0487393284727,41.6978863030865,
-223.850794334856));
#201370=CARTESIAN_POINT('Ctrl Pts',(-37.5777639477929,43.429423512094,-220.712280626913));
#201371=CARTESIAN_POINT('Ctrl Pts',(-40.1082645173074,45.1604528702306,
-217.574688874121));
#201372=CARTESIAN_POINT('Ctrl Pts',(-42.6395909737856,46.8912293280373,
-214.437630225606));
#201373=CARTESIAN_POINT('Ctrl Pts',(-27.5495579756445,36.5028921654741,
-233.251051919951));
#201374=CARTESIAN_POINT('Ctrl Pts',(-28.1827688115622,36.9359521258547,
-232.465366213753));
#201375=CARTESIAN_POINT('Ctrl Pts',(-28.8164085091962,37.3688162618127,
-231.679931708896));
#201376=CARTESIAN_POINT('Ctrl Pts',(-29.45037829501,37.8015234896747,-230.894689344989));
#201377=CARTESIAN_POINT('Ctrl Pts',(-30.0843480808238,38.2342307175367,
-230.109446981082));
#201378=CARTESIAN_POINT('Ctrl Pts',(-30.7186486771531,38.6667807943463,
-229.324397213218));
#201379=CARTESIAN_POINT('Ctrl Pts',(-31.3532086585038,39.0992026045944,
-228.539497756859));
#201380=CARTESIAN_POINT('Ctrl Pts',(-32.6223286212052,39.9640462250905,
-226.96969884414));
#201381=CARTESIAN_POINT('Ctrl Pts',(-33.8924746608402,40.828381296436,-225.400494315711));
#201382=CARTESIAN_POINT('Ctrl Pts',(-35.1632781294504,41.6923616886714,
-223.831668727949));
#201383=CARTESIAN_POINT('Ctrl Pts',(-37.7048850666709,43.4203224731419,
-220.694017552425));
#201384=CARTESIAN_POINT('Ctrl Pts',(-40.2490633538194,45.1468896454712,
-217.55784834607));
#201385=CARTESIAN_POINT('Ctrl Pts',(-42.7944274621604,46.8726693939935,
-214.42236887553));
#201386=CARTESIAN_POINT('Ctrl Pts',(-27.6055780256448,36.5084909217888,
-233.228921976304));
#201387=CARTESIAN_POINT('Ctrl Pts',(-28.2423304860859,36.9411059500847,
-232.442898411838));
#201388=CARTESIAN_POINT('Ctrl Pts',(-28.8798608338247,37.3733283098348,
-231.657313855381));
#201389=CARTESIAN_POINT('Ctrl Pts',(-29.5179264655878,37.8052614858298,
-230.87202778373));
#201390=CARTESIAN_POINT('Ctrl Pts',(-30.1559920973509,38.2371946618249,
-230.08674171208));
#201391=CARTESIAN_POINT('Ctrl Pts',(-30.7945950027779,38.6688382551504,
-229.301755452856));
#201392=CARTESIAN_POINT('Ctrl Pts',(-31.433575412527,39.1002648835096,-228.516978390142));
#201393=CARTESIAN_POINT('Ctrl Pts',(-32.7115362320255,39.9631181402278,
-226.947424264716));
#201394=CARTESIAN_POINT('Ctrl Pts',(-33.9909784660999,40.82511685855,-225.378690793586));
#201395=CARTESIAN_POINT('Ctrl Pts',(-35.2712022810355,41.6865965771103,
-223.810389502773));
#201396=CARTESIAN_POINT('Ctrl Pts',(-37.8316499109069,43.4095560142309,
-220.673786921149));
#201397=CARTESIAN_POINT('Ctrl Pts',(-40.3951430863757,45.1304838440415,
-217.53887071552));
#201398=CARTESIAN_POINT('Ctrl Pts',(-42.9596694236649,46.8503990616624,
-214.404555343614));
#201399=CARTESIAN_POINT('Ctrl Pts',(-27.6544884050101,36.5134544997187,
-233.208489782041));
#201400=CARTESIAN_POINT('Ctrl Pts',(-28.2958883125488,36.9453045586868,
-232.422071262426));
#201401=CARTESIAN_POINT('Ctrl Pts',(-28.9385402233851,37.3764580517972,
-231.636337934604));
#201402=CARTESIAN_POINT('Ctrl Pts',(-29.5819207190053,37.8071775310161,
-230.850998973988));
#201403=CARTESIAN_POINT('Ctrl Pts',(-30.2253012146256,38.2378970102351,
-230.065660013372));
#201404=CARTESIAN_POINT('Ctrl Pts',(-30.8694237090864,38.6681763110842,
-229.280723186985));
#201405=CARTESIAN_POINT('Ctrl Pts',(-31.5140148312165,39.0981569518477,
-228.496039104459));
#201406=CARTESIAN_POINT('Ctrl Pts',(-32.8031970754766,39.9581182333748,
-226.926670939409));
#201407=CARTESIAN_POINT('Ctrl Pts',(-34.094212486763,40.8169068877022,-225.358291458816));
#201408=CARTESIAN_POINT('Ctrl Pts',(-35.3860663228485,41.675053386644,-223.79036645522));
#201409=CARTESIAN_POINT('Ctrl Pts',(-37.9697739950195,43.3913463845276,
-220.654516448028));
#201410=CARTESIAN_POINT('Ctrl Pts',(-40.5567806505099,45.1051056979372,
-217.520458021817));
#201411=CARTESIAN_POINT('Ctrl Pts',(-43.1447063347815,46.8176414904025,
-214.386944837765));
#201412=CARTESIAN_POINT('Ctrl Pts',(-27.7033987843753,36.5184180776487,
-233.188057587778));
#201413=CARTESIAN_POINT('Ctrl Pts',(-28.3494461390117,36.9495031672888,
-232.401244113014));
#201414=CARTESIAN_POINT('Ctrl Pts',(-28.9972196129455,37.3795877937595,
-231.615362013826));
#201415=CARTESIAN_POINT('Ctrl Pts',(-29.6459149724228,37.8090935762025,
-230.829970164246));
#201416=CARTESIAN_POINT('Ctrl Pts',(-30.2946103319002,38.2385993586454,
-230.044578314665));
#201417=CARTESIAN_POINT('Ctrl Pts',(-30.944252415395,38.6675143670179,-229.259690921114));
#201418=CARTESIAN_POINT('Ctrl Pts',(-31.5944542499059,39.0960490201859,
-228.475099818776));
#201419=CARTESIAN_POINT('Ctrl Pts',(-32.8948579189276,39.9531183265218,
-226.905917614101));
#201420=CARTESIAN_POINT('Ctrl Pts',(-34.1974465074261,40.8086969168544,
-225.337892124046));
#201421=CARTESIAN_POINT('Ctrl Pts',(-35.5009303646614,41.6635101961778,
-223.770343407667));
#201422=CARTESIAN_POINT('Ctrl Pts',(-38.1078980791321,43.3731367548243,
-220.635245974907));
#201423=CARTESIAN_POINT('Ctrl Pts',(-40.7184182146441,45.0797275518329,
-217.502045328114));
#201424=CARTESIAN_POINT('Ctrl Pts',(-43.329743245898,46.7848839191427,-214.369334331916));
#201425=CARTESIAN_POINT('Ctrl Pts',(-27.7467504913837,36.5219322799631,
-233.170032188139));
#201426=CARTESIAN_POINT('Ctrl Pts',(-28.3985217181101,36.9519116209705,
-232.382753952573));
#201427=CARTESIAN_POINT('Ctrl Pts',(-29.0525419525678,37.3805207587552,
-231.59666656708));
#201428=CARTESIAN_POINT('Ctrl Pts',(-29.707648099349,37.8084119595345,-230.811147097123));
#201429=CARTESIAN_POINT('Ctrl Pts',(-30.3627542461301,38.2363031603138,
-230.025627627167));
#201430=CARTESIAN_POINT('Ctrl Pts',(-31.0189916736704,38.6634523908632,
-229.240701082927));
#201431=CARTESIAN_POINT('Ctrl Pts',(-31.6758577488396,39.0901500013781,
-228.456102690314));
#201432=CARTESIAN_POINT('Ctrl Pts',(-32.9895898991783,39.9435452224079,
-226.886905905089));
#201433=CARTESIAN_POINT('Ctrl Pts',(-34.305776607248,40.7951703456425,-225.318990914817));
#201434=CARTESIAN_POINT('Ctrl Pts',(-35.6228886941575,41.6459326221272,
-223.751565966636));
#201435=CARTESIAN_POINT('Ctrl Pts',(-38.2571128679763,43.3474571750966,
-220.616716070273));
#201436=CARTESIAN_POINT('Ctrl Pts',(-40.8950551389346,45.0455299408185,
-217.483839750893));
#201437=CARTESIAN_POINT('Ctrl Pts',(-43.5337367396124,46.7419641904284,
-214.351434639915));
#201438=CARTESIAN_POINT('Ctrl Pts',(-27.8054264163448,36.5146074937637,
-233.160277704479));
#201439=CARTESIAN_POINT('Ctrl Pts',(-28.4608655062395,36.9445884335815,
-232.371247983632));
#201440=CARTESIAN_POINT('Ctrl Pts',(-29.1196314139931,37.372514313029,-231.584005383938));
#201441=CARTESIAN_POINT('Ctrl Pts',(-29.7799261927146,37.7994041715398,
-230.797562749801));
#201442=CARTESIAN_POINT('Ctrl Pts',(-30.4402209714361,38.2262940300507,
-230.011120115663));
#201443=CARTESIAN_POINT('Ctrl Pts',(-31.1021216515676,38.6521081108545,
-229.225521863909));
#201444=CARTESIAN_POINT('Ctrl Pts',(-31.7648888134181,39.0772864601489,
-228.440373573626));
#201445=CARTESIAN_POINT('Ctrl Pts',(-33.090423137119,39.9276431587379,-226.87007699306));
#201446=CARTESIAN_POINT('Ctrl Pts',(-34.4193423302246,40.7755094860917,
-225.301539303434));
#201447=CARTESIAN_POINT('Ctrl Pts',(-35.7494892631586,41.6222215800908,
-223.73364023664));
#201448=CARTESIAN_POINT('Ctrl Pts',(-38.4097831290267,43.3156457680889,
-220.597842103052));
#201449=CARTESIAN_POINT('Ctrl Pts',(-41.0750442414306,45.0044380406571,
-217.464638507897));
#201450=CARTESIAN_POINT('Ctrl Pts',(-43.7412542098013,46.69118281627,-214.332014574282));
#201451=CARTESIAN_POINT('Ctrl Pts',(-27.864102341306,36.5072827075644,-233.150523220819));
#201452=CARTESIAN_POINT('Ctrl Pts',(-28.523209294369,36.9372652461925,-232.359742014691));
#201453=CARTESIAN_POINT('Ctrl Pts',(-29.1867208754184,37.3645078673026,
-231.571344200798));
#201454=CARTESIAN_POINT('Ctrl Pts',(-29.8522042860804,37.7903963835451,
-230.783978402477));
#201455=CARTESIAN_POINT('Ctrl Pts',(-30.5176876967423,38.2162848997876,
-229.996612604157));
#201456=CARTESIAN_POINT('Ctrl Pts',(-31.1852516294648,38.6407638308456,
-229.210342644892));
#201457=CARTESIAN_POINT('Ctrl Pts',(-31.8539198779964,39.0644229189197,
-228.424644456938));
#201458=CARTESIAN_POINT('Ctrl Pts',(-33.1912563750597,39.9117410950679,
-226.853248081031));
#201459=CARTESIAN_POINT('Ctrl Pts',(-34.532908053201,40.7558486265409,-225.284087692051));
#201460=CARTESIAN_POINT('Ctrl Pts',(-35.8760898321597,41.5985105380543,
-223.715714506644));
#201461=CARTESIAN_POINT('Ctrl Pts',(-38.5624533900771,43.2838343610812,
-220.578968135829));
#201462=CARTESIAN_POINT('Ctrl Pts',(-41.2550333439266,44.9633461404957,
-217.4454372649));
#201463=CARTESIAN_POINT('Ctrl Pts',(-43.9487716799902,46.6404014421116,
-214.312594508648));
#201464=CARTESIAN_POINT('Ctrl Pts',(-27.9190830878262,36.5008900102226,
-233.139346077501));
#201465=CARTESIAN_POINT('Ctrl Pts',(-28.5832756511028,36.9299347713319,
-232.34736702198));
#201466=CARTESIAN_POINT('Ctrl Pts',(-29.2527286972829,37.3556305517945,
-231.558257704261));
#201467=CARTESIAN_POINT('Ctrl Pts',(-29.9244591932939,37.7797083909036,
-230.770340230532));
#201468=CARTESIAN_POINT('Ctrl Pts',(-30.5961896893049,38.2037862300127,
-229.982422756802));
#201469=CARTESIAN_POINT('Ctrl Pts',(-31.270338006197,38.626174417356,-229.195781239181));
#201470=CARTESIAN_POINT('Ctrl Pts',(-31.945743753703,39.0475951547582,-228.409789029494));
#201471=CARTESIAN_POINT('Ctrl Pts',(-33.2965552487149,39.8904366295628,
-226.837804610121));
#201472=CARTESIAN_POINT('Ctrl Pts',(-34.6522827270746,40.7294895383089,
-225.268361443424));
#201473=CARTESIAN_POINT('Ctrl Pts',(-36.0097034880497,41.5668741114757,
-223.699782360708));
#201474=CARTESIAN_POINT('Ctrl Pts',(-38.7245450099999,43.2416432578092,
-220.56262419528));
#201475=CARTESIAN_POINT('Ctrl Pts',(-41.4463029811519,44.9096878836177,
-217.429019852247));
#201476=CARTESIAN_POINT('Ctrl Pts',(-44.169290550113,46.5749498873242,-214.296143159535));
#201477=CARTESIAN_POINT('Ctrl Pts',(-27.9635611001738,36.4990952898012,
-233.124907406577));
#201478=CARTESIAN_POINT('Ctrl Pts',(-28.6335193341731,36.9265762879192,
-232.332215621801));
#201479=CARTESIAN_POINT('Ctrl Pts',(-29.3093382993415,37.3501779403658,
-231.542719800075));
#201480=CARTESIAN_POINT('Ctrl Pts',(-29.9876295989316,37.7719445682467,
-230.754510440041));
#201481=CARTESIAN_POINT('Ctrl Pts',(-30.6659208985218,38.1937111961276,
-229.966301080007));
#201482=CARTESIAN_POINT('Ctrl Pts',(-31.346850346985,38.6135550182896,-229.179478141202));
#201483=CARTESIAN_POINT('Ctrl Pts',(-32.0291309789057,39.032311940978,-228.393348201459));
#201484=CARTESIAN_POINT('Ctrl Pts',(-33.3936922427472,39.869825786355,-226.821088321973));
#201485=CARTESIAN_POINT('Ctrl Pts',(-34.7635386549114,40.7030825753783,
-225.251542754464));
#201486=CARTESIAN_POINT('Ctrl Pts',(-36.1351659076718,41.5344930728638,
-223.682897927105));
#201487=CARTESIAN_POINT('Ctrl Pts',(-38.8784204131928,43.1973140678347,
-220.545608272386));
#201488=CARTESIAN_POINT('Ctrl Pts',(-41.6289795635766,44.8526757118206,
-217.412042386738));
#201489=CARTESIAN_POINT('Ctrl Pts',(-44.3807833059246,46.5049749771785,
-214.279216302521));
#201490=CARTESIAN_POINT('Ctrl Pts',(-28.0080391125216,36.4973005693799,
-233.110468735653));
#201491=CARTESIAN_POINT('Ctrl Pts',(-28.6837630172434,36.9232178045066,
-232.317064221622));
#201492=CARTESIAN_POINT('Ctrl Pts',(-29.3659479014001,37.344725328937,-231.527181895889));
#201493=CARTESIAN_POINT('Ctrl Pts',(-30.0508000045693,37.7641807455897,
-230.73868064955));
#201494=CARTESIAN_POINT('Ctrl Pts',(-30.7356521077386,38.1836361622425,
-229.950179403211));
#201495=CARTESIAN_POINT('Ctrl Pts',(-31.423362687773,38.6009356192233,-229.163175043223));
#201496=CARTESIAN_POINT('Ctrl Pts',(-32.1125182041085,39.0170287271978,
-228.376907373423));
#201497=CARTESIAN_POINT('Ctrl Pts',(-33.4908292367796,39.849214943147,-226.804372033824));
#201498=CARTESIAN_POINT('Ctrl Pts',(-34.8747945827483,40.6766756124477,
-225.234724065505));
#201499=CARTESIAN_POINT('Ctrl Pts',(-36.2606283272941,41.5021120342519,
-223.666013493501));
#201500=CARTESIAN_POINT('Ctrl Pts',(-39.0322958163857,43.1529848778602,
-220.528592349493));
#201501=CARTESIAN_POINT('Ctrl Pts',(-41.8116561460013,44.7956635400236,
-217.395064921228));
#201502=CARTESIAN_POINT('Ctrl Pts',(-44.5922760617361,46.4350000670329,
-214.262289445508));
#201503=CARTESIAN_POINT('Ctrl Pts',(-28.0494437864605,36.495141074799,-233.096611018152));
#201504=CARTESIAN_POINT('Ctrl Pts',(-28.7308360120535,36.9193190689171,
-232.302532895241));
#201505=CARTESIAN_POINT('Ctrl Pts',(-29.4192203432693,37.3385601524366,
-231.512266925172));
#201506=CARTESIAN_POINT('Ctrl Pts',(-30.1104565561833,37.7555228770627,
-230.723470216585));
#201507=CARTESIAN_POINT('Ctrl Pts',(-30.8016927690973,38.1724856016888,
-229.934673507997));
#201508=CARTESIAN_POINT('Ctrl Pts',(-31.4959930724453,38.5870515082353,
-229.147475500813));
#201509=CARTESIAN_POINT('Ctrl Pts',(-32.1918313004172,39.0002838036336,
-228.361056572999));
#201510=CARTESIAN_POINT('Ctrl Pts',(-33.5835077563608,39.82674839443,-226.788218717371));
#201511=CARTESIAN_POINT('Ctrl Pts',(-34.981204076813,40.6479886792153,-225.218435880259));
#201512=CARTESIAN_POINT('Ctrl Pts',(-36.3808689058395,41.4670086872456,
-223.649631412145));
#201513=CARTESIAN_POINT('Ctrl Pts',(-39.1801985638925,43.1050487033063,
-220.512022475916));
#201514=CARTESIAN_POINT('Ctrl Pts',(-41.9876501636135,44.7340917680141,
-217.378490005261));
#201515=CARTESIAN_POINT('Ctrl Pts',(-44.7964013528814,46.3594930633657,
-214.245731113265));
#201516=CARTESIAN_POINT('Ctrl Pts',(-28.0986638608654,36.4864396316355,
-233.086219707902));
#201517=CARTESIAN_POINT('Ctrl Pts',(-28.7855090882708,36.908671912885,-232.291339757935));
#201518=CARTESIAN_POINT('Ctrl Pts',(-29.4797969634702,37.3255148395588,
-231.50054713919));
#201519=CARTESIAN_POINT('Ctrl Pts',(-30.1771392417705,37.7398414336408,
-230.711331015122));
#201520=CARTESIAN_POINT('Ctrl Pts',(-30.8744815200707,38.1541680277229,
-229.922114891055));
#201521=CARTESIAN_POINT('Ctrl Pts',(-31.5751008302705,38.565853402466,-229.134613456395));
#201522=CARTESIAN_POINT('Ctrl Pts',(-32.2773697651967,38.9760615626091,
-228.347946926293));
#201523=CARTESIAN_POINT('Ctrl Pts',(-33.6819076350491,39.7964778828953,
-226.77461386609));
#201524=CARTESIAN_POINT('Ctrl Pts',(-35.092901360331,40.6111090059392,-225.204554400508));
#201525=CARTESIAN_POINT('Ctrl Pts',(-36.506013012055,41.4232755079927,-223.635540355772));
#201526=CARTESIAN_POINT('Ctrl Pts',(-39.3322363155031,43.0476085120996,
-220.4975122663));
#201527=CARTESIAN_POINT('Ctrl Pts',(-42.1671908002668,44.6619661512638,
-217.363841724096));
#201528=CARTESIAN_POINT('Ctrl Pts',(-45.0035463653253,46.2723209746968,
-214.23099286058));
#201529=CARTESIAN_POINT('Ctrl Pts',(-28.1478839352704,36.477738188472,-233.075828397652));
#201530=CARTESIAN_POINT('Ctrl Pts',(-28.8401821644882,36.8980247568529,
-232.280146620628));
#201531=CARTESIAN_POINT('Ctrl Pts',(-29.5403735836712,37.3124695266811,
-231.488827353208));
#201532=CARTESIAN_POINT('Ctrl Pts',(-30.2438219273577,37.724159990219,-230.69919181366));
#201533=CARTESIAN_POINT('Ctrl Pts',(-30.9472702710442,38.1358504537568,
-229.909556274112));
#201534=CARTESIAN_POINT('Ctrl Pts',(-31.6542085880957,38.5446552966966,
-229.121751411976));
#201535=CARTESIAN_POINT('Ctrl Pts',(-32.3629082299762,38.9518393215846,
-228.334837279587));
#201536=CARTESIAN_POINT('Ctrl Pts',(-33.7803075137374,39.7662073713606,
-226.761009014808));
#201537=CARTESIAN_POINT('Ctrl Pts',(-35.204598643849,40.5742293326632,-225.190672920757));
#201538=CARTESIAN_POINT('Ctrl Pts',(-36.6311571182707,41.3795423287398,
-223.621449299399));
#201539=CARTESIAN_POINT('Ctrl Pts',(-39.4842740671139,42.9901683208929,
-220.483002056683));
#201540=CARTESIAN_POINT('Ctrl Pts',(-42.3467314369201,44.5898405345135,
-217.349193442931));
#201541=CARTESIAN_POINT('Ctrl Pts',(-45.2106913777692,46.1851488860278,
-214.216254607896));
#201542=CARTESIAN_POINT('Ctrl Pts',(-28.2012732840083,36.4651498400409,
-233.067037777728));
#201543=CARTESIAN_POINT('Ctrl Pts',(-28.8990579728149,36.8831408843765,
-232.270578628329));
#201544=CARTESIAN_POINT('Ctrl Pts',(-29.6051083171889,37.2948838670021,
-231.478729287174));
#201545=CARTESIAN_POINT('Ctrl Pts',(-30.3146028640688,37.7036388348153,
-230.688668141709));
#201546=CARTESIAN_POINT('Ctrl Pts',(-31.0240974109487,38.1123938026283,
-229.898606996244));
#201547=CARTESIAN_POINT('Ctrl Pts',(-31.7372746006804,38.5180264505524,
-229.110487353379));
#201548=CARTESIAN_POINT('Ctrl Pts',(-32.4523194990151,38.9218935751344,
-228.323313754114));
#201549=CARTESIAN_POINT('Ctrl Pts',(-33.8824092956843,39.7296278242987,
-226.748966555583));
#201550=CARTESIAN_POINT('Ctrl Pts',(-35.3198051784721,40.5304514518755,
-225.178327508987));
#201551=CARTESIAN_POINT('Ctrl Pts',(-36.7596189263893,41.3283116061093,
-223.608870010882));
#201552=CARTESIAN_POINT('Ctrl Pts',(-39.6392464222237,42.9240319145765,
-220.469955014674));
#201553=CARTESIAN_POINT('Ctrl Pts',(-42.5288205943682,44.5077862844145,
-217.335965063606));
#201554=CARTESIAN_POINT('Ctrl Pts',(-45.4200071428167,46.0868030777345,
-214.202896281505));
#201555=CARTESIAN_POINT('Ctrl Pts',(-28.2536248719719,36.45164456484,-233.058476234802));
#201556=CARTESIAN_POINT('Ctrl Pts',(-28.956246064681,36.8674691193729,-232.261151946464));
#201557=CARTESIAN_POINT('Ctrl Pts',(-29.6674872789167,37.2766580792002,
-231.468687139439));
#201558=CARTESIAN_POINT('Ctrl Pts',(-30.3823793991597,37.6826022896234,
-230.678128469586));
#201559=CARTESIAN_POINT('Ctrl Pts',(-31.0972715194027,38.0885465000466,
-229.887569799732));
#201560=CARTESIAN_POINT('Ctrl Pts',(-31.8160539135098,38.4911129154006,
-229.099074756418));
#201561=CARTESIAN_POINT('Ctrl Pts',(-32.5368266733684,38.8917474183737,
-228.311589632248));
#201562=CARTESIAN_POINT('Ctrl Pts',(-33.9783721930855,39.6930164243198,
-226.736619383908));
#201563=CARTESIAN_POINT('Ctrl Pts',(-35.4277003933768,40.4867262619234,
-225.16560579597));
#201564=CARTESIAN_POINT('Ctrl Pts',(-36.8796336124663,41.2771645198602,
-223.595856775541));
#201565=CARTESIAN_POINT('Ctrl Pts',(-39.7835000506455,42.8580410357338,
-220.456358734683));
#201566=CARTESIAN_POINT('Ctrl Pts',(-42.6980566108585,44.4257389283559,
-217.322125580858));
#201567=CARTESIAN_POINT('Ctrl Pts',(-45.6143789670139,45.9882588716253,
-214.18887606046));
#201568=CARTESIAN_POINT('Ctrl Pts',(-28.3059764599357,36.4381392896391,
-233.049914691876));
#201569=CARTESIAN_POINT('Ctrl Pts',(-29.0134341565471,36.8517973543695,
-232.2517252646));
#201570=CARTESIAN_POINT('Ctrl Pts',(-29.7298662406445,37.2584322913983,
-231.458644991706));
#201571=CARTESIAN_POINT('Ctrl Pts',(-30.4501559342506,37.6615657444315,
-230.667588797462));
#201572=CARTESIAN_POINT('Ctrl Pts',(-31.1704456278568,38.0646991974648,
-229.876532603218));
#201573=CARTESIAN_POINT('Ctrl Pts',(-31.8948332263391,38.464199380249,-229.087662159456));
#201574=CARTESIAN_POINT('Ctrl Pts',(-32.6213338477217,38.8616012616129,
-228.299865510382));
#201575=CARTESIAN_POINT('Ctrl Pts',(-34.0743350904866,39.6564050243409,
-226.724272212234));
#201576=CARTESIAN_POINT('Ctrl Pts',(-35.5355956082815,40.4430010719712,
-225.152884082953));
#201577=CARTESIAN_POINT('Ctrl Pts',(-36.9996482985433,41.2260174336112,
-223.582843540199));
#201578=CARTESIAN_POINT('Ctrl Pts',(-39.9277536790671,42.792050156891,-220.442762454692));
#201579=CARTESIAN_POINT('Ctrl Pts',(-42.8672926273489,44.3436915722972,
-217.308286098109));
#201580=CARTESIAN_POINT('Ctrl Pts',(-45.8087507912112,45.889714665516,-214.174855839415));
#201581=CARTESIAN_POINT('Ctrl Pts',(-28.3519546381049,36.428499297722,-233.038801999823));
#201582=CARTESIAN_POINT('Ctrl Pts',(-29.0685651860499,36.8359598776144,
-232.242286479252));
#201583=CARTESIAN_POINT('Ctrl Pts',(-29.7920661546429,37.237805899639,-231.449720689388));
#201584=CARTESIAN_POINT('Ctrl Pts',(-30.5189980352994,37.6364573834381,
-230.658986703413));
#201585=CARTESIAN_POINT('Ctrl Pts',(-31.2459299159559,38.0351088672372,
-229.868252717438));
#201586=CARTESIAN_POINT('Ctrl Pts',(-31.9764124958348,38.4305023582899,
-229.079433957463));
#201587=CARTESIAN_POINT('Ctrl Pts',(-32.7088796298207,38.8238619301343,
-228.291635917502));
#201588=CARTESIAN_POINT('Ctrl Pts',(-34.1738138977924,39.6105810738233,
-226.716039837583));
#201589=CARTESIAN_POINT('Ctrl Pts',(-35.6464836269217,40.3893479405787,
-225.144422997191));
#201590=CARTESIAN_POINT('Ctrl Pts',(-37.122025520744,41.1643408760019,-223.574201356819));
#201591=CARTESIAN_POINT('Ctrl Pts',(-40.0731093083885,42.7143267468484,
-220.433758076075));
#201592=CARTESIAN_POINT('Ctrl Pts',(-43.0357115526382,44.2493386577901,
-217.298984924306));
#201593=CARTESIAN_POINT('Ctrl Pts',(-46.0004325581354,45.7782515470524,
-214.165346999843));
#201594=CARTESIAN_POINT('Ctrl Pts',(-28.404523824249,36.4142111160726,-233.028222391732));
#201595=CARTESIAN_POINT('Ctrl Pts',(-29.1296788023777,36.8148442685854,
-232.23397055258));
#201596=CARTESIAN_POINT('Ctrl Pts',(-29.8595774687733,37.2115210846296,
-231.442464211111));
#201597=CARTESIAN_POINT('Ctrl Pts',(-30.5921210784794,37.6056911614944,
-230.652400010517));
#201598=CARTESIAN_POINT('Ctrl Pts',(-31.3246646881855,37.9998612383593,
-229.862335809922));
#201599=CARTESIAN_POINT('Ctrl Pts',(-32.0599114204536,38.3914951944436,
-229.073755169551));
#201600=CARTESIAN_POINT('Ctrl Pts',(-32.7968044445028,38.7814033859296,
-228.286041512615));
#201601=CARTESIAN_POINT('Ctrl Pts',(-34.2705904926014,39.5612197689016,
-226.710614198745));
#201602=CARTESIAN_POINT('Ctrl Pts',(-35.7508066075144,40.334264217189,-225.138570075993));
#201603=CARTESIAN_POINT('Ctrl Pts',(-37.2337704007868,41.1036371719424,
-223.567901121106));
#201604=CARTESIAN_POINT('Ctrl Pts',(-40.1996979873318,42.6423830814493,
-220.426563211331));
#201605=CARTESIAN_POINT('Ctrl Pts',(-43.1764747241572,44.166666266985,-217.290698996916));
#201606=CARTESIAN_POINT('Ctrl Pts',(-46.1558000266483,45.6842043061087,
-214.156194672008));
#201607=CARTESIAN_POINT('Ctrl Pts',(-28.4570930103932,36.3999229344231,
-233.01764278364));
#201608=CARTESIAN_POINT('Ctrl Pts',(-29.1907924187055,36.7937286595564,
-232.225654625907));
#201609=CARTESIAN_POINT('Ctrl Pts',(-29.9270887829037,37.1852362696201,
-231.435207732835));
#201610=CARTESIAN_POINT('Ctrl Pts',(-30.6652441216594,37.5749249395508,
-230.645813317621));
#201611=CARTESIAN_POINT('Ctrl Pts',(-31.403399460415,37.9646136094813,-229.856418902407));
#201612=CARTESIAN_POINT('Ctrl Pts',(-32.1434103450723,38.3524880305972,
-229.06807638164));
#201613=CARTESIAN_POINT('Ctrl Pts',(-32.884729259185,38.7389448417248,-228.280447107729));
#201614=CARTESIAN_POINT('Ctrl Pts',(-34.3673670874105,39.5118584639798,
-226.705188559907));
#201615=CARTESIAN_POINT('Ctrl Pts',(-35.8551295881073,40.2791804937992,
-225.132717154794));
#201616=CARTESIAN_POINT('Ctrl Pts',(-37.3455152808298,41.0429334678829,
-223.561600885392));
#201617=CARTESIAN_POINT('Ctrl Pts',(-40.3262866662749,42.5704394160502,
-220.419368346588));
#201618=CARTESIAN_POINT('Ctrl Pts',(-43.3172378956761,44.0839938761798,
-217.282413069526));
#201619=CARTESIAN_POINT('Ctrl Pts',(-46.3111674951612,45.590157065165,-214.147042344173));
#201620=CARTESIAN_POINT('Ctrl Pts',(-28.5214435153128,36.3758121500046,
-233.010309376466));
#201621=CARTESIAN_POINT('Ctrl Pts',(-29.2597711912192,36.7652926192596,
-232.219435748514));
#201622=CARTESIAN_POINT('Ctrl Pts',(-29.9999412300851,37.1531174751436,
-231.429684565593));
#201623=CARTESIAN_POINT('Ctrl Pts',(-30.741464839369,37.539582297854,-230.640726768058));
#201624=CARTESIAN_POINT('Ctrl Pts',(-31.482988448653,37.9260471205643,-229.851768970523));
#201625=CARTESIAN_POINT('Ctrl Pts',(-32.2258698218865,38.3111507874138,
-229.063608073021));
#201626=CARTESIAN_POINT('Ctrl Pts',(-32.9697681692284,38.6951211034311,
-228.276025525187));
#201627=CARTESIAN_POINT('Ctrl Pts',(-34.4575648639124,39.4630617354659,
-226.700860429518));
#201628=CARTESIAN_POINT('Ctrl Pts',(-35.9493723068607,40.2265053230493,
-225.12797096096));
#201629=CARTESIAN_POINT('Ctrl Pts',(-37.4435195048015,40.9866952819017,
-223.556350656432));
#201630=CARTESIAN_POINT('Ctrl Pts',(-40.4318139006829,42.5070751996064,
-220.413110047378));
#201631=CARTESIAN_POINT('Ctrl Pts',(-43.4292180728484,44.0146569196856,
-217.274809144726));
#201632=CARTESIAN_POINT('Ctrl Pts',(-46.4299697523172,45.5143458457586,
-214.138325398592));
#201633=CARTESIAN_POINT('Ctrl Pts',(-28.5917373044541,36.3459190971896,
-233.004412799005));
#201634=CARTESIAN_POINT('Ctrl Pts',(-29.3336456870839,36.7317236596899,
-232.214541575288));
#201635=CARTESIAN_POINT('Ctrl Pts',(-30.0768533355596,37.1163079376712,
-231.425484075423));
#201636=CARTESIAN_POINT('Ctrl Pts',(-30.8210649438641,37.4998384795814,
-230.63703601277));
#201637=CARTESIAN_POINT('Ctrl Pts',(-31.5652765521686,37.8833690214916,
-229.848587950118));
#201638=CARTESIAN_POINT('Ctrl Pts',(-32.3104940183536,38.2658454573702,
-229.060750983011));
#201639=CARTESIAN_POINT('Ctrl Pts',(-33.056499757863,38.6474031071304,-228.273381017246));
#201640=CARTESIAN_POINT('Ctrl Pts',(-34.5485112368819,39.4105184066505,
-226.698641085717));
#201641=CARTESIAN_POINT('Ctrl Pts',(-36.0436413480666,40.1699780267802,
-225.125745165631));
#201642=CARTESIAN_POINT('Ctrl Pts',(-37.5407436150405,40.9265749496157,
-223.553976309726));
#201643=CARTESIAN_POINT('Ctrl Pts',(-40.5349481489884,42.439768795287,-220.410438597917));
#201644=CARTESIAN_POINT('Ctrl Pts',(-43.536857304037,43.9416524034681,-217.271298591679));
#201645=CARTESIAN_POINT('Ctrl Pts',(-46.5420263558244,45.4357480033572,
-214.134039310084));
#201646=CARTESIAN_POINT('Ctrl Pts',(-28.6268841990247,36.3309725707821,
-233.001464510274));
#201647=CARTESIAN_POINT('Ctrl Pts',(-29.3705829350163,36.7149391799052,
-232.212094488675));
#201648=CARTESIAN_POINT('Ctrl Pts',(-30.1153093882969,37.097903168935,-231.423383830337));
#201649=CARTESIAN_POINT('Ctrl Pts',(-30.8608649961116,37.4799665704452,
-230.635190635126));
#201650=CARTESIAN_POINT('Ctrl Pts',(-31.6064206039263,37.8620299719552,
-229.846997439915));
#201651=CARTESIAN_POINT('Ctrl Pts',(-32.3528061165871,38.2431927923484,
-229.059322438005));
#201652=CARTESIAN_POINT('Ctrl Pts',(-33.0998655521803,38.6235441089799,
-228.272058763276));
#201653=CARTESIAN_POINT('Ctrl Pts',(-34.5939844233666,39.3842467422428,
-226.697531413816));
#201654=CARTESIAN_POINT('Ctrl Pts',(-36.0907758686695,40.1417143786457,
-225.124632267967));
#201655=CARTESIAN_POINT('Ctrl Pts',(-37.5893556701601,40.8965147834728,
-223.552789136373));
#201656=CARTESIAN_POINT('Ctrl Pts',(-40.5865152731412,42.4061155931272,
-220.409102873187));
#201657=CARTESIAN_POINT('Ctrl Pts',(-43.5906769196312,43.9051501453593,
-217.269543315155));
#201658=CARTESIAN_POINT('Ctrl Pts',(-46.598054657578,45.3964490821564,-214.13189626583));
#201659=CARTESIAN_POINT('Ctrl Pts',(-28.6518975580342,36.3261811548597,
-232.993056797812));
#201660=CARTESIAN_POINT('Ctrl Pts',(-29.398737821756,36.7070015779651,-232.205034899571));
#201661=CARTESIAN_POINT('Ctrl Pts',(-30.1460916201158,37.0872237185874,
-231.417368861425));
#201662=CARTESIAN_POINT('Ctrl Pts',(-30.8939024648147,37.4668637098655,
-230.6300135554));
#201663=CARTESIAN_POINT('Ctrl Pts',(-31.6417133095137,37.8465037011437,
-229.842658249374));
#201664=CARTESIAN_POINT('Ctrl Pts',(-32.3899812257617,38.225561587839,-229.055613721231));
#201665=CARTESIAN_POINT('Ctrl Pts',(-33.1386550153031,38.6040547581662,
-228.268840529801));
#201666=CARTESIAN_POINT('Ctrl Pts',(-34.6360025943859,39.3610410988206,
-226.69529414694));
#201667=CARTESIAN_POINT('Ctrl Pts',(-36.1349692411245,40.1157684838324,
-225.122828814917));
#201668=CARTESIAN_POINT('Ctrl Pts',(-37.6352027617429,40.8683822730397,
-223.551187160683));
#201669=CARTESIAN_POINT('Ctrl Pts',(-40.6356698029797,42.3736098514546,
-220.407903852216));
#201670=CARTESIAN_POINT('Ctrl Pts',(-43.6411528261178,43.8703944217154,
-217.267871204892));
#201671=CARTESIAN_POINT('Ctrl Pts',(-46.6495816719042,45.3598482038711,
-214.129724170691));
#201672=CARTESIAN_POINT('Ctrl Pts',(-28.6836693563314,36.3172916302978,
-232.984586371767));
#201673=CARTESIAN_POINT('Ctrl Pts',(-29.4328038186657,36.6955273714839,
-232.197666951892));
#201674=CARTESIAN_POINT('Ctrl Pts',(-30.1821597301324,37.0733995616469,
-231.410933917807));
#201675=CARTESIAN_POINT('Ctrl Pts',(-30.9317206554361,37.4509071831741,
-230.624372601034));
#201676=CARTESIAN_POINT('Ctrl Pts',(-31.6812815807397,37.8284148047014,
-229.83781128426));
#201677=CARTESIAN_POINT('Ctrl Pts',(-32.4310475185464,38.2055578694789,
-229.051421689267));
#201678=CARTESIAN_POINT('Ctrl Pts',(-33.1810027512314,38.5823363130566,
-228.265190292231));
#201679=CARTESIAN_POINT('Ctrl Pts',(-34.6809132166015,39.3358932002121,
-226.69272749816));
#201680=CARTESIAN_POINT('Ctrl Pts',(-36.1815801312299,40.0879909915779,
-225.120896504533));
#201681=CARTESIAN_POINT('Ctrl Pts',(-37.6828865095192,40.8386380933409,
-223.549601777981));
#201682=CARTESIAN_POINT('Ctrl Pts',(-40.6854992660978,42.3399322968669,
-220.407012324875));
#201683=CARTESIAN_POINT('Ctrl Pts',(-43.6906591856765,43.835419294533,-217.266555597716));
#201684=CARTESIAN_POINT('Ctrl Pts',(-46.6975653758367,45.3252553963054,
-214.127639057046));
#201685=CARTESIAN_POINT('Ctrl Pts',(-28.7154411546286,36.3084021057357,
-232.976115945722));
#201686=CARTESIAN_POINT('Ctrl Pts',(-29.4668698155753,36.6840531650027,
-232.190299004213));
#201687=CARTESIAN_POINT('Ctrl Pts',(-30.2182278401491,37.0595754047064,
-231.404498974189));
#201688=CARTESIAN_POINT('Ctrl Pts',(-30.9695388460574,37.4349506564828,
-230.618731646667));
#201689=CARTESIAN_POINT('Ctrl Pts',(-31.7208498519656,37.8103259082591,
-229.832964319146));
#201690=CARTESIAN_POINT('Ctrl Pts',(-32.4721138113312,38.1855541511188,
-229.047229657302));
#201691=CARTESIAN_POINT('Ctrl Pts',(-33.2233504871597,38.560617867947,-228.261540054661));
#201692=CARTESIAN_POINT('Ctrl Pts',(-34.7258238388169,39.3107453016035,
-226.690160849379));
#201693=CARTESIAN_POINT('Ctrl Pts',(-36.2281910213353,40.0602134993234,
-225.11896419415));
#201694=CARTESIAN_POINT('Ctrl Pts',(-37.7305702572955,40.808893913642,-223.548016395278));
#201695=CARTESIAN_POINT('Ctrl Pts',(-40.7353287292159,42.3062547422792,
-220.406120797533));
#201696=CARTESIAN_POINT('Ctrl Pts',(-43.7401655452353,43.8004441673505,
-217.265239990539));
#201697=CARTESIAN_POINT('Ctrl Pts',(-46.7455490797692,45.2906625887397,
-214.1255539434));
#201698=CARTESIAN_POINT('Ctrl Pts',(-28.7546828535794,36.2946048538794,
-232.967923270373));
#201699=CARTESIAN_POINT('Ctrl Pts',(-29.5075354964661,36.6682851435785,
-232.18296040294));
#201700=CARTESIAN_POINT('Ctrl Pts',(-30.260203356218,37.041928546648,-231.397949783602));
#201701=CARTESIAN_POINT('Ctrl Pts',(-31.012687072449,37.4155430678739,-230.612897000714));
#201702=CARTESIAN_POINT('Ctrl Pts',(-31.7651707886799,37.7891575890997,
-229.827844217825));
#201703=CARTESIAN_POINT('Ctrl Pts',(-32.5174703341753,38.1627432696007,
-229.042749264024));
#201704=CARTESIAN_POINT('Ctrl Pts',(-33.2695884278607,38.5363065970483,
-228.257619016064));
#201705=CARTESIAN_POINT('Ctrl Pts',(-34.7738246152316,39.2834332519434,
-226.687358520144));
#201706=CARTESIAN_POINT('Ctrl Pts',(-36.2773319082997,40.0304737792722,
-225.116955396868));
#201707=CARTESIAN_POINT('Ctrl Pts',(-37.7801639596043,40.7774501421753,
-223.546481445834));
#201708=CARTESIAN_POINT('Ctrl Pts',(-40.7858280622135,42.2714028679817,
-220.405533543764));
#201709=CARTESIAN_POINT('Ctrl Pts',(-43.788714991937,43.7652295475826,-217.264288793245));
#201710=CARTESIAN_POINT('Ctrl Pts',(-46.7899896154941,45.2580776239732,
-214.123556902107));
#201711=CARTESIAN_POINT('Ctrl Pts',(-28.811481324712,36.2672238003158,-232.961663720964));
#201712=CARTESIAN_POINT('Ctrl Pts',(-29.5645263655861,36.6399226415611,
-232.177270818232));
#201713=CARTESIAN_POINT('Ctrl Pts',(-30.3173414199567,37.0126142771829,
-231.392803581211));
#201714=CARTESIAN_POINT('Ctrl Pts',(-31.069911071871,37.385324556228,-230.608260371606));
#201715=CARTESIAN_POINT('Ctrl Pts',(-31.8224807237854,37.7580348352731,
-229.823717162));
#201716=CARTESIAN_POINT('Ctrl Pts',(-32.5748049718356,38.1307637318441,
-229.039097966911));
#201717=CARTESIAN_POINT('Ctrl Pts',(-33.326867581659,38.5035402264522,-228.254401763819));
#201718=CARTESIAN_POINT('Ctrl Pts',(-34.8309928013059,39.2490932156681,
-226.685009357635));
#201719=CARTESIAN_POINT('Ctrl Pts',(-36.3340721635766,39.9948325139069,
-225.115307761803));
#201720=CARTESIAN_POINT('Ctrl Pts',(-37.8359666905481,40.7410341111373,
-223.545299801334));
#201721=CARTESIAN_POINT('Ctrl Pts',(-40.8397557444911,42.233437305598,-220.405283880397));
#201722=CARTESIAN_POINT('Ctrl Pts',(-43.8388051696003,43.7275965705222,
-217.264000696622));
#201723=CARTESIAN_POINT('Ctrl Pts',(-46.8319258491792,45.2266492383781,
-214.121813627025));
#201724=CARTESIAN_POINT('',(-27.8050194937375,36.7328856011635,-232.85004997616));
#201725=CARTESIAN_POINT('',(-28.91863242939,36.3202559697984,-232.850049997099));
#201726=CARTESIAN_POINT('Ctrl Pts',(-27.8050195498509,36.7328855898013,
-232.85005));
#201727=CARTESIAN_POINT('Ctrl Pts',(-27.8949275165814,36.7209782096512,
-232.85005));
#201728=CARTESIAN_POINT('Ctrl Pts',(-27.9520459297408,36.7106005629156,
-232.850049999996));
#201729=CARTESIAN_POINT('Ctrl Pts',(-28.0460926671002,36.6880699552386,
-232.850049999996));
#201730=CARTESIAN_POINT('Ctrl Pts',(-28.0749971330459,36.6807536283026,
-232.85004999998));
#201731=CARTESIAN_POINT('Ctrl Pts',(-28.1941353499751,36.6493093982322,
-232.85004999998));
#201732=CARTESIAN_POINT('Ctrl Pts',(-28.2670565577019,36.626391907203,-232.85005000281));
#201733=CARTESIAN_POINT('Ctrl Pts',(-28.4092997003064,36.5718764626196,
-232.85005000281));
#201734=CARTESIAN_POINT('Ctrl Pts',(-28.4498501321219,36.5555397344433,
-232.850050000011));
#201735=CARTESIAN_POINT('Ctrl Pts',(-28.516992000843,36.5269407519737,-232.850050000011));
#201736=CARTESIAN_POINT('Ctrl Pts',(-28.5460646864076,36.5139050283581,
-232.850049999999));
#201737=CARTESIAN_POINT('Ctrl Pts',(-28.5974873610269,36.4900506389875,
-232.850049999999));
#201738=CARTESIAN_POINT('Ctrl Pts',(-28.6238785516589,36.4773923395039,
-232.85005));
#201739=CARTESIAN_POINT('Ctrl Pts',(-28.6914460343325,36.4443598397627,
-232.85005));
#201740=CARTESIAN_POINT('Ctrl Pts',(-28.7430990859246,36.4184125393908,
-232.850050000001));
#201741=CARTESIAN_POINT('Ctrl Pts',(-28.8244637237435,36.3756607678727,
-232.850050000001));
#201742=CARTESIAN_POINT('Ctrl Pts',(-28.8695136741866,36.3496498157912,
-232.85005));
#201743=CARTESIAN_POINT('Ctrl Pts',(-28.9186324246664,36.3202560005055,
-232.85005));
#201744=CARTESIAN_POINT('',(-42.5495440650111,46.8296601025756,-214.549225413994));
#201745=CARTESIAN_POINT('Ctrl Pts',(-27.8050194367111,36.7328856245227,
-232.850049943209));
#201746=CARTESIAN_POINT('Ctrl Pts',(-28.8113908504514,37.4236469909598,
-231.598047201307));
#201747=CARTESIAN_POINT('Ctrl Pts',(-29.8181679708266,38.1142366013137,
-230.346339471264));
#201748=CARTESIAN_POINT('Ctrl Pts',(-30.825311593422,38.8047002149063,-229.094849929364));
#201749=CARTESIAN_POINT('Ctrl Pts',(-32.0551345438968,39.647825246345,-227.566656207657));
#201750=CARTESIAN_POINT('Ctrl Pts',(-33.2855044821927,40.4907627392734,
-226.038787218309));
#201751=CARTESIAN_POINT('Ctrl Pts',(-34.5163077632667,41.3335669381032,
-224.511155775758));
#201752=CARTESIAN_POINT('Ctrl Pts',(-35.858766024936,42.2528279419423,-222.844941944213));
#201753=CARTESIAN_POINT('Ctrl Pts',(-37.2017438370567,43.1719331137164,
-221.179005741399));
#201754=CARTESIAN_POINT('Ctrl Pts',(-38.5450581953352,44.0909285309741,
-219.513278100248));
#201755=CARTESIAN_POINT('Ctrl Pts',(-39.87961658598,45.0039337687333,-217.858407975228));
#201756=CARTESIAN_POINT('Ctrl Pts',(-41.2145061144966,45.9168299735115,
-216.203744979336));
#201757=CARTESIAN_POINT('Ctrl Pts',(-42.5495440044243,46.8296601017195,
-214.549225420693));
#201758=CARTESIAN_POINT('',(-42.9717852817482,46.7498147039571,-214.534096350323));
#201759=CARTESIAN_POINT('Ctrl Pts',(-42.971785281757,46.7498147039532,-214.534096350459));
#201760=CARTESIAN_POINT('Ctrl Pts',(-42.9007346296511,46.763275910118,-214.539081896592));
#201761=CARTESIAN_POINT('Ctrl Pts',(-42.8299315204016,46.776675786459,-214.542916316407));
#201762=CARTESIAN_POINT('Ctrl Pts',(-42.6886800576438,46.8033850073215,
-214.547976621766));
#201763=CARTESIAN_POINT('Ctrl Pts',(-42.619734567264,46.8164109911115,-214.549201740479));
#201764=CARTESIAN_POINT('Ctrl Pts',(-42.5495441334904,46.8296600955011,
-214.549225427215));
#201765=CARTESIAN_POINT('',(-46.6391379650153,45.1301057079818,-214.324193082213));
#201766=CARTESIAN_POINT('Ctrl Pts',(-42.971785281757,46.749814703953,-214.534096350459));
#201767=CARTESIAN_POINT('Ctrl Pts',(-43.0986721931805,46.7257747996628,
-214.525192835446));
#201768=CARTESIAN_POINT('Ctrl Pts',(-43.2250603487763,46.698950689265,-214.516517597901));
#201769=CARTESIAN_POINT('Ctrl Pts',(-43.4873979542421,46.6372234999647,
-214.499052367715));
#201770=CARTESIAN_POINT('Ctrl Pts',(-43.6236733286717,46.60170761618,-214.490110644589));
#201771=CARTESIAN_POINT('Ctrl Pts',(-43.8528808069682,46.536136708902,-214.475014174647));
#201772=CARTESIAN_POINT('Ctrl Pts',(-43.9471502951446,46.5074540598357,
-214.468951067953));
#201773=CARTESIAN_POINT('Ctrl Pts',(-44.1657362375147,46.4369225437304,
-214.455376470205));
#201774=CARTESIAN_POINT('Ctrl Pts',(-44.2895719690723,46.3939046797032,
-214.44795935219));
#201775=CARTESIAN_POINT('Ctrl Pts',(-44.5758870683756,46.2872516658799,
-214.430838622384));
#201776=CARTESIAN_POINT('Ctrl Pts',(-44.7376694317707,46.2214844642399,
-214.421105848178));
#201777=CARTESIAN_POINT('Ctrl Pts',(-44.9968191999223,46.1070741801046,
-214.40608822588));
#201778=CARTESIAN_POINT('Ctrl Pts',(-45.0953309340452,46.061394556028,-214.400545485118));
#201779=CARTESIAN_POINT('Ctrl Pts',(-45.3586587291112,45.933337546142,-214.386175771088));
#201780=CARTESIAN_POINT('Ctrl Pts',(-45.5225973316144,45.847169815917,-214.377106637015));
#201781=CARTESIAN_POINT('Ctrl Pts',(-45.7910067952199,45.695231241578,-214.362880563465));
#201782=CARTESIAN_POINT('Ctrl Pts',(-45.8980961662255,45.6315653233674,
-214.357676228472));
#201783=CARTESIAN_POINT('Ctrl Pts',(-46.0677903916686,45.5257929940805,
-214.349632079152));
#201784=CARTESIAN_POINT('Ctrl Pts',(-46.1316130051584,45.4848666363269,
-214.346627166685));
#201785=CARTESIAN_POINT('Ctrl Pts',(-46.276213361064,45.3894937683197,-214.339569954199));
#201786=CARTESIAN_POINT('Ctrl Pts',(-46.3575523972629,45.3339263996382,
-214.335548815048));
#201787=CARTESIAN_POINT('Ctrl Pts',(-46.5062346419384,45.2285595756106,
-214.32924726228));
#201788=CARTESIAN_POINT('Ctrl Pts',(-46.5731746843278,45.1796922527548,
-214.326639483805));
#201789=CARTESIAN_POINT('Ctrl Pts',(-46.6391379870654,45.1301057439282,
-214.324192948162));
#201790=CARTESIAN_POINT('Ctrl Pts',(-28.9186324244905,36.3202560021114,
-232.85005));
#201791=CARTESIAN_POINT('Ctrl Pts',(-31.8738175305195,37.7828806767965,
-229.771729072198));
#201792=CARTESIAN_POINT('Ctrl Pts',(-34.8254630565706,39.2453536842348,
-226.692248678165));
#201793=CARTESIAN_POINT('Ctrl Pts',(-40.7330653074378,42.1803713539693,
-220.516897602703));
#201794=CARTESIAN_POINT('Ctrl Pts',(-43.6889686819812,43.6528974634763,
-217.42098942157));
#201795=CARTESIAN_POINT('Ctrl Pts',(-46.6391379591575,45.1301057601645,
-214.324193166304));
#201796=CARTESIAN_POINT('Ctrl Pts',(-46.9840049393815,18.6129810161854,
-232.962872244472));
#201797=CARTESIAN_POINT('Ctrl Pts',(-47.8808382771992,19.9304390734321,
-231.392237704844));
#201798=CARTESIAN_POINT('Ctrl Pts',(-48.7782728428765,21.247161929372,-229.821521522905));
#201799=CARTESIAN_POINT('Ctrl Pts',(-49.6764219919997,22.5630778387597,
-228.250728876356));
#201800=CARTESIAN_POINT('Ctrl Pts',(-50.5745711411229,23.8789937481474,
-226.679936229808));
#201801=CARTESIAN_POINT('Ctrl Pts',(-51.4734343837544,25.1941028059552,
-225.109066921118));
#201802=CARTESIAN_POINT('Ctrl Pts',(-52.3731538889575,26.508321667889,-223.538132682591));
#201803=CARTESIAN_POINT('Ctrl Pts',(-54.1725928993637,29.1367593917566,
-220.396264205537));
#201804=CARTESIAN_POINT('Ctrl Pts',(-55.9754067618462,31.7616502024816,
-217.254119255235));
#201805=CARTESIAN_POINT('Ctrl Pts',(-57.7832199428974,34.3821699572177,
-214.111935079921));
#201806=CARTESIAN_POINT('Ctrl Pts',(-46.9913120403997,18.6016320696042,
-232.962809737275));
#201807=CARTESIAN_POINT('Ctrl Pts',(-47.8881017068652,19.919347208754,-231.392174086571));
#201808=CARTESIAN_POINT('Ctrl Pts',(-48.7854927208081,21.2363283107576,
-229.821456748291));
#201809=CARTESIAN_POINT('Ctrl Pts',(-49.6835984491062,22.5525036430274,
-228.250662893886));
#201810=CARTESIAN_POINT('Ctrl Pts',(-50.5817041774044,23.8686789752972,
-226.679869039482));
#201811=CARTESIAN_POINT('Ctrl Pts',(-51.480524130202,25.1840486327538,-225.108998471456));
#201812=CARTESIAN_POINT('Ctrl Pts',(-52.3802004849816,26.4985292873713,
-223.538062914284));
#201813=CARTESIAN_POINT('Ctrl Pts',(-54.1795531945409,29.1274905966065,
-220.396191799938));
#201814=CARTESIAN_POINT('Ctrl Pts',(-55.9822813208348,31.7529097593695,
-217.254043978496));
#201815=CARTESIAN_POINT('Ctrl Pts',(-57.7900093367969,34.3739628192697,
-214.111856605281));
#201816=CARTESIAN_POINT('Ctrl Pts',(-46.9993592918125,18.5895020464233,
-232.962537246545));
#201817=CARTESIAN_POINT('Ctrl Pts',(-47.8960185439573,19.9075721396807,
-231.391930728925));
#201818=CARTESIAN_POINT('Ctrl Pts',(-48.7932866262407,21.2248997369702,
-229.821238456431));
#201819=CARTESIAN_POINT('Ctrl Pts',(-49.6912806705268,22.5414098682959,
-228.250464972721));
#201820=CARTESIAN_POINT('Ctrl Pts',(-50.5892747148128,23.8579199996217,
-226.679691489012));
#201821=CARTESIAN_POINT('Ctrl Pts',(-51.4879942010195,25.1736127697718,
-225.108836587826));
#201822=CARTESIAN_POINT('Ctrl Pts',(-52.3875865131366,26.4884007882765,
-223.537911482743));
#201823=CARTESIAN_POINT('Ctrl Pts',(-54.1867711373708,29.117976825286,-220.396061272575));
#201824=CARTESIAN_POINT('Ctrl Pts',(-55.9893940924071,31.7439488367061,
-217.25391286698));
#201825=CARTESIAN_POINT('Ctrl Pts',(-57.7971476360592,34.365448302035,-214.11170390739));
#201826=CARTESIAN_POINT('Ctrl Pts',(-47.0041643855294,18.580762838696,-232.963218170749));
#201827=CARTESIAN_POINT('Ctrl Pts',(-47.9010716022698,19.8987644772325,
-231.392505287657));
#201828=CARTESIAN_POINT('Ctrl Pts',(-48.7985636253896,21.2160564611115,
-229.821719884836));
#201829=CARTESIAN_POINT('Ctrl Pts',(-49.6967438426135,22.5325760511435,
-228.250869035074));
#201830=CARTESIAN_POINT('Ctrl Pts',(-50.5949240598375,23.8490956411754,
-226.680018185312));
#201831=CARTESIAN_POINT('Ctrl Pts',(-51.4937920916948,25.1648428846195,
-225.10910171349));
#201832=CARTESIAN_POINT('Ctrl Pts',(-52.3934756614324,26.4797462844595,
-223.53813309987));
#201833=CARTESIAN_POINT('Ctrl Pts',(-54.1928428009075,29.1095530841393,
-220.396195872632));
#201834=CARTESIAN_POINT('Ctrl Pts',(-55.9954317595172,31.7359937276413,
-217.254034998605));
#201835=CARTESIAN_POINT('Ctrl Pts',(-57.8026630300816,34.3583854144121,
-214.111890802731));
#201836=CARTESIAN_POINT('Ctrl Pts',(-47.0089694792463,18.5720236309689,
-232.963899094952));
#201837=CARTESIAN_POINT('Ctrl Pts',(-47.9061246605823,19.8899568147843,
-231.393079846389));
#201838=CARTESIAN_POINT('Ctrl Pts',(-48.8038406245385,21.2072131852528,
-229.822201313241));
#201839=CARTESIAN_POINT('Ctrl Pts',(-49.7022070147003,22.523742233991,-228.251273097427));
#201840=CARTESIAN_POINT('Ctrl Pts',(-50.6005734048621,23.8402712827293,
-226.680344881612));
#201841=CARTESIAN_POINT('Ctrl Pts',(-51.4995899823701,25.1560729994673,
-225.109366839153));
#201842=CARTESIAN_POINT('Ctrl Pts',(-52.3993648097282,26.4710917806424,
-223.538354716999));
#201843=CARTESIAN_POINT('Ctrl Pts',(-54.1989144644443,29.1011293429925,
-220.39633047269));
#201844=CARTESIAN_POINT('Ctrl Pts',(-56.0014694266273,31.7280386185765,
-217.25415713023));
#201845=CARTESIAN_POINT('Ctrl Pts',(-57.8081784241041,34.3513225267891,
-214.112077698071));
#201846=CARTESIAN_POINT('Ctrl Pts',(-47.0135037838248,18.5636186637907,
-232.964603901451));
#201847=CARTESIAN_POINT('Ctrl Pts',(-47.9109413268945,19.8814389765153,
-231.393671922464));
#201848=CARTESIAN_POINT('Ctrl Pts',(-48.8089116831402,21.1986202770561,
-229.822695902599));
#201849=CARTESIAN_POINT('Ctrl Pts',(-49.7074910913547,22.5151234922153,
-228.251687496631));
#201850=CARTESIAN_POINT('Ctrl Pts',(-50.6060704995693,23.8316267073747,
-226.680679090663));
#201851=CARTESIAN_POINT('Ctrl Pts',(-51.5052588130045,25.1474518025266,
-225.109638186271));
#201852=CARTESIAN_POINT('Ctrl Pts',(-52.4051458912763,26.4625572063643,
-223.538582055459));
#201853=CARTESIAN_POINT('Ctrl Pts',(-54.2049200478198,29.0927680140397,
-220.396469793837));
#201854=CARTESIAN_POINT('Ctrl Pts',(-56.0074702714946,31.7201003474161,
-217.254286107255));
#201855=CARTESIAN_POINT('Ctrl Pts',(-57.8137160680311,34.3442051333583,
-214.11226899193));
#201856=CARTESIAN_POINT('Ctrl Pts',(-47.0177828560111,18.5555300817996,
-232.96533252157));
#201857=CARTESIAN_POINT('Ctrl Pts',(-47.9155370349421,19.8731929180949,
-231.394280823516));
#201858=CARTESIAN_POINT('Ctrl Pts',(-48.8137913023007,21.1902606020353,
-229.823202807664));
#201859=CARTESIAN_POINT('Ctrl Pts',(-49.7126093236726,22.5067040125525,
-228.252111396185));
#201860=CARTESIAN_POINT('Ctrl Pts',(-50.6114273450444,23.8231474230696,
-226.681019984706));
#201861=CARTESIAN_POINT('Ctrl Pts',(-51.5108090328418,25.1389665178458,
-225.109915092335));
#201862=CARTESIAN_POINT('Ctrl Pts',(-52.4108279627846,26.4541313607334,
-223.538814574431));
#201863=CARTESIAN_POINT('Ctrl Pts',(-54.2108658226704,29.0844610465087,
-220.396613538622));
#201864=CARTESIAN_POINT('Ctrl Pts',(-56.0134397408495,31.7121723231175,
-217.254421501589));
#201865=CARTESIAN_POINT('Ctrl Pts',(-57.8192783928772,34.3370299914758,
-214.112464332901));
#201866=CARTESIAN_POINT('Ctrl Pts',(-47.0263410003839,18.5393529178172,
-232.966789761807));
#201867=CARTESIAN_POINT('Ctrl Pts',(-47.9247284510372,19.856700801254,-231.395498625619));
#201868=CARTESIAN_POINT('Ctrl Pts',(-48.8235505406218,21.1735412519938,
-229.824216617793));
#201869=CARTESIAN_POINT('Ctrl Pts',(-49.7228457883083,22.4898650532266,
-228.252959195293));
#201870=CARTESIAN_POINT('Ctrl Pts',(-50.6221410359948,23.8061888544594,
-226.681701772792));
#201871=CARTESIAN_POINT('Ctrl Pts',(-51.5219094725163,25.1219959484843,
-225.110468904466));
#201872=CARTESIAN_POINT('Ctrl Pts',(-52.4221921058014,26.4372796694717,
-223.539279612374));
#201873=CARTESIAN_POINT('Ctrl Pts',(-54.2227573723716,29.0678471114466,
-220.396901028191));
#201874=CARTESIAN_POINT('Ctrl Pts',(-56.0253786795592,31.6963162745203,
-217.254692290257));
#201875=CARTESIAN_POINT('Ctrl Pts',(-57.8304030425693,34.3226797077107,
-214.112855014843));
#201876=CARTESIAN_POINT('Ctrl Pts',(-47.0338760075754,18.5244437003147,
-232.968343063198));
#201877=CARTESIAN_POINT('Ctrl Pts',(-47.9330342637239,19.8412977645685,
-231.396784393101));
#201878=CARTESIAN_POINT('Ctrl Pts',(-48.8325426907541,21.1577563020188,
-229.825280180548));
#201879=CARTESIAN_POINT('Ctrl Pts',(-49.7324178666844,22.4738242520981,
-228.253845361594));
#201880=CARTESIAN_POINT('Ctrl Pts',(-50.6322930426146,23.7898922021775,
-226.682410542641));
#201881=CARTESIAN_POINT('Ctrl Pts',(-51.5325349868385,25.1055695505858,
-225.111045116373));
#201882=CARTESIAN_POINT('Ctrl Pts',(-52.4331598468605,26.4208632806089,
-223.539765492053));
#201883=CARTESIAN_POINT('Ctrl Pts',(-54.2344095669047,29.0514507406552,
-220.397206243413));
#201884=CARTESIAN_POINT('Ctrl Pts',(-56.0371921164241,31.6805012272399,
-217.254988767415));
#201885=CARTESIAN_POINT('Ctrl Pts',(-57.8416264681079,34.3080984038517,
-214.113261878824));
#201886=CARTESIAN_POINT('Ctrl Pts',(-47.0405353763693,18.5106352292473,
-232.969983979348));
#201887=CARTESIAN_POINT('Ctrl Pts',(-47.9405971515569,19.8268187140002,
-231.398125716493));
#201888=CARTESIAN_POINT('Ctrl Pts',(-48.8408986391317,21.1427526567519,
-229.826381496195));
#201889=CARTESIAN_POINT('Ctrl Pts',(-49.7414431123329,22.4584427038901,
-228.254759191353));
#201890=CARTESIAN_POINT('Ctrl Pts',(-50.6419875855342,23.7741327510283,
-226.683136886512));
#201891=CARTESIAN_POINT('Ctrl Pts',(-51.5427750540585,25.0895788993504,
-225.111636500013));
#201892=CARTESIAN_POINT('Ctrl Pts',(-52.443808131774,26.4047878990792,-223.540266455142));
#201893=CARTESIAN_POINT('Ctrl Pts',(-54.2458742872048,29.0352058985368,
-220.397526365399));
#201894=CARTESIAN_POINT('Ctrl Pts',(-56.0489238784563,31.6646741163143,
-217.255307216989));
#201895=CARTESIAN_POINT('Ctrl Pts',(-57.852967529916,34.2932604357928,-214.113682169595));
#201896=CARTESIAN_POINT('Ctrl Pts',(-47.0538541139573,18.4830182871128,
-232.973265811648));
#201897=CARTESIAN_POINT('Ctrl Pts',(-47.955722927223,19.7978606128634,-231.400808363276));
#201898=CARTESIAN_POINT('Ctrl Pts',(-48.8576105358869,21.1127453662178,
-229.828584127488));
#201899=CARTESIAN_POINT('Ctrl Pts',(-49.7594936036301,22.4276796074738,
-228.256586850871));
#201900=CARTESIAN_POINT('Ctrl Pts',(-50.6613766713732,23.7426138487298,
-226.684589574255));
#201901=CARTESIAN_POINT('Ctrl Pts',(-51.5632551884987,25.0575975968797,
-225.112819267293));
#201902=CARTESIAN_POINT('Ctrl Pts',(-52.4651047016009,26.3726371360198,
-223.541268381319));
#201903=CARTESIAN_POINT('Ctrl Pts',(-54.2688037278052,29.0027162143,-220.398166609371));
#201904=CARTESIAN_POINT('Ctrl Pts',(-56.0723874025208,31.6330198944631,
-217.255944116137));
#201905=CARTESIAN_POINT('Ctrl Pts',(-57.875649653532,34.2635844996751,-214.114522751136));
#201906=CARTESIAN_POINT('Ctrl Pts',(-47.0636230131447,18.4598625903094,
-232.976920051811));
#201907=CARTESIAN_POINT('Ctrl Pts',(-47.9678453495437,19.7726375200406,
-231.403727674415));
#201908=CARTESIAN_POINT('Ctrl Pts',(-48.8717566764505,21.0858891471629,
-229.830947114461));
#201909=CARTESIAN_POINT('Ctrl Pts',(-49.7753424176378,22.3995713001604,
-228.258531477614));
#201910=CARTESIAN_POINT('Ctrl Pts',(-50.6789281588252,23.713253453158,-226.686115840768));
#201911=CARTESIAN_POINT('Ctrl Pts',(-51.5821885259387,25.0273656345712,
-225.114064824849));
#201912=CARTESIAN_POINT('Ctrl Pts',(-52.4851199367133,26.3418548778766,
-223.54233208791));
#201913=CARTESIAN_POINT('Ctrl Pts',(-54.2909827582626,28.9708333644873,
-220.398866614033));
#201914=CARTESIAN_POINT('Ctrl Pts',(-56.0955252131014,31.6013169572485,
-217.256668942392));
#201915=CARTESIAN_POINT('Ctrl Pts',(-57.8988032731226,34.2328814256343,
-214.115416854107));
#201916=CARTESIAN_POINT('Ctrl Pts',(-47.07151283755,18.4392609475024,-232.980675631547));
#201917=CARTESIAN_POINT('Ctrl Pts',(-47.9784669049768,19.7494077885448,
-231.40663525448));
#201918=CARTESIAN_POINT('Ctrl Pts',(-48.8846403863511,21.0606622046162,
-229.833271513153));
#201919=CARTESIAN_POINT('Ctrl Pts',(-49.7901160730939,22.3727913382652,
-228.260434083043));
#201920=CARTESIAN_POINT('Ctrl Pts',(-50.6955917598367,23.6849204719142,
-226.687596652933));
#201921=CARTESIAN_POINT('Ctrl Pts',(-51.6003698589295,24.9979251551198,
-225.115286361312));
#201922=CARTESIAN_POINT('Ctrl Pts',(-52.5045272731894,26.3116209606581,
-223.543390841591));
#201923=CARTESIAN_POINT('Ctrl Pts',(-54.3128421017092,28.939012571735,-220.399599802148));
#201924=CARTESIAN_POINT('Ctrl Pts',(-56.1186826713171,31.569141738417,-217.257449700108));
#201925=CARTESIAN_POINT('Ctrl Pts',(-57.9225686339535,34.2009514305169,
-214.116344107367));
#201926=CARTESIAN_POINT('Ctrl Pts',(-47.0872924863604,18.3980576618883,
-232.988186791018));
#201927=CARTESIAN_POINT('Ctrl Pts',(-47.999710015843,19.7029483255535,-231.41245041461));
#201928=CARTESIAN_POINT('Ctrl Pts',(-48.9104078061524,21.0102083195229,
-229.837920310538));
#201929=CARTESIAN_POINT('Ctrl Pts',(-49.819663384006,22.3192314144748,-228.264239293901));
#201930=CARTESIAN_POINT('Ctrl Pts',(-50.7289189618596,23.6282545094267,
-226.690558277265));
#201931=CARTESIAN_POINT('Ctrl Pts',(-51.636732524911,24.9390441962169,-225.117729434238));
#201932=CARTESIAN_POINT('Ctrl Pts',(-52.5433419461414,26.2511531262214,
-223.545508348952));
#201933=CARTESIAN_POINT('Ctrl Pts',(-54.3565607886023,28.8753709862302,
-220.401066178378));
#201934=CARTESIAN_POINT('Ctrl Pts',(-56.1649975877485,31.5047913007538,
-217.259011215537));
#201935=CARTESIAN_POINT('Ctrl Pts',(-57.9700993556152,34.1370914402818,
-214.118198613889));
#201936=CARTESIAN_POINT('Ctrl Pts',(-47.0957039619647,18.3671243104028,
-232.996174969848));
#201937=CARTESIAN_POINT('Ctrl Pts',(-48.0152404739711,19.6642406239314,
-231.41815251762));
#201938=CARTESIAN_POINT('Ctrl Pts',(-48.9313836399292,20.966064710906,-229.842352705242));
#201939=CARTESIAN_POINT('Ctrl Pts',(-49.8451267410034,22.2708048165049,
-228.267820632962));
#201940=CARTESIAN_POINT('Ctrl Pts',(-50.7588698420775,23.575544922104,-226.693288560683));
#201941=CARTESIAN_POINT('Ctrl Pts',(-51.6702057869443,24.8832308760699,
-225.12004558303));
#201942=CARTESIAN_POINT('Ctrl Pts',(-52.5798100280734,26.1928111185938,
-223.547584934865));
#201943=CARTESIAN_POINT('Ctrl Pts',(-54.3990185103318,28.8119716036413,
-220.402663638535));
#201944=CARTESIAN_POINT('Ctrl Pts',(-56.2114230943841,31.438531247625,-217.260790636888));
#201945=CARTESIAN_POINT('Ctrl Pts',(-58.0200925469402,34.0683156133792,
-214.120181154191));
#201946=CARTESIAN_POINT('Ctrl Pts',(-47.1150642483994,18.3236858273299,
-232.999295710587));
#201947=CARTESIAN_POINT('Ctrl Pts',(-48.0392206238659,19.6158965079908,
-231.420362484156));
#201948=CARTESIAN_POINT('Ctrl Pts',(-48.9590100671071,20.9141580894346,
-229.844205156969));
#201949=CARTESIAN_POINT('Ctrl Pts',(-49.8759725739142,22.2158319633755,
-228.269472472139));
#201950=CARTESIAN_POINT('Ctrl Pts',(-50.7929350807213,23.5175058373164,
-226.694739787308));
#201951=CARTESIAN_POINT('Ctrl Pts',(-51.7070476323962,24.8226580511233,
-225.12147447558));
#201952=CARTESIAN_POINT('Ctrl Pts',(-52.6192352667853,26.1299128826243,
-223.549042364026));
#201953=CARTESIAN_POINT('Ctrl Pts',(-54.4436105355637,28.7444225456263,
-220.404178140919));
#201954=CARTESIAN_POINT('Ctrl Pts',(-56.2604448907417,31.367132192526,-217.262559371757));
#201955=CARTESIAN_POINT('Ctrl Pts',(-58.0734857403641,33.9931206393803,
-214.122173015364));
#201956=CARTESIAN_POINT('Ctrl Pts',(-47.1344245348341,18.280247344257,-233.002416451326));
#201957=CARTESIAN_POINT('Ctrl Pts',(-48.0632007737606,19.5675523920502,
-231.422572450694));
#201958=CARTESIAN_POINT('Ctrl Pts',(-48.9866364942849,20.8622514679632,
-229.846057608697));
#201959=CARTESIAN_POINT('Ctrl Pts',(-49.906818406825,22.1608591102461,-228.271124311316));
#201960=CARTESIAN_POINT('Ctrl Pts',(-50.8270003193651,23.459466752529,-226.696191013934));
#201961=CARTESIAN_POINT('Ctrl Pts',(-51.7438894778481,24.7620852261766,
-225.12290336813));
#201962=CARTESIAN_POINT('Ctrl Pts',(-52.6586605054972,26.0670146466549,
-223.550499793187));
#201963=CARTESIAN_POINT('Ctrl Pts',(-54.4882025607956,28.6768734876113,
-220.405692643303));
#201964=CARTESIAN_POINT('Ctrl Pts',(-56.3094666870994,31.2957331374271,
-217.264328106627));
#201965=CARTESIAN_POINT('Ctrl Pts',(-58.1268789337879,33.9179256653815,
-214.124164876537));
#201966=CARTESIAN_POINT('Ctrl Pts',(-47.1550475881779,18.2351214015296,
-233.004587184861));
#201967=CARTESIAN_POINT('Ctrl Pts',(-48.0879494927851,19.5179208547626,
-231.424215169804));
#201968=CARTESIAN_POINT('Ctrl Pts',(-49.0146228296911,20.8093049547191,
-229.847633981322));
#201969=CARTESIAN_POINT('Ctrl Pts',(-49.9377435309543,22.1049290587682,
-228.272719230379));
#201970=CARTESIAN_POINT('Ctrl Pts',(-50.8608642322175,23.4005531628173,
-226.697804479436));
#201971=CARTESIAN_POINT('Ctrl Pts',(-51.7803719924673,24.7005632099661,
-225.124644811749));
#201972=CARTESIAN_POINT('Ctrl Pts',(-52.6976719303263,26.0029791484965,
-223.55238064694));
#201973=CARTESIAN_POINT('Ctrl Pts',(-54.5322718060444,28.6078110255573,
-220.407852317323));
#201974=CARTESIAN_POINT('Ctrl Pts',(-56.3582589004816,31.2220093923588,
-217.266815267618));
#201975=CARTESIAN_POINT('Ctrl Pts',(-58.1805302372139,33.8394259727705,
-214.126915573344));
#201976=CARTESIAN_POINT('Ctrl Pts',(-47.1711020320382,18.1951169691784,
-233.008152197064));
#201977=CARTESIAN_POINT('Ctrl Pts',(-48.1091754301695,19.471620881615,-231.426873602798));
#201978=CARTESIAN_POINT('Ctrl Pts',(-49.0396359981975,20.7586423084589,
-229.850155627119));
#201979=CARTESIAN_POINT('Ctrl Pts',(-49.9662083070876,22.0502814645383,
-228.275198729438));
#201980=CARTESIAN_POINT('Ctrl Pts',(-50.8927806159777,23.3419206206176,
-226.700241831756));
#201981=CARTESIAN_POINT('Ctrl Pts',(-51.8153427493086,24.6384368291909,
-225.12719326289));
#201982=CARTESIAN_POINT('Ctrl Pts',(-52.7356127602431,25.9374582798656,
-223.555055698046));
#201983=CARTESIAN_POINT('Ctrl Pts',(-54.5761527821122,28.535501181215,-220.410780568357));
#201984=CARTESIAN_POINT('Ctrl Pts',(-56.4077512436301,31.1433164616566,
-217.270071905955));
#201985=CARTESIAN_POINT('Ctrl Pts',(-58.2358086912436,33.7542064961608,
-214.130435725157));
#201986=CARTESIAN_POINT('Ctrl Pts',(-47.1871564758985,18.1551125368272,
-233.011717209266));
#201987=CARTESIAN_POINT('Ctrl Pts',(-48.1304013675538,19.4253209084676,
-231.429532035792));
#201988=CARTESIAN_POINT('Ctrl Pts',(-49.0646491667038,20.7079796621986,
-229.852677272917));
#201989=CARTESIAN_POINT('Ctrl Pts',(-49.9946730832209,21.9956338703083,
-228.277678228496));
#201990=CARTESIAN_POINT('Ctrl Pts',(-50.924696999738,23.283288078418,-226.702679184075));
#201991=CARTESIAN_POINT('Ctrl Pts',(-51.8503135061499,24.5763104484158,
-225.129741714031));
#201992=CARTESIAN_POINT('Ctrl Pts',(-52.7735535901599,25.8719374112347,
-223.557730749151));
#201993=CARTESIAN_POINT('Ctrl Pts',(-54.62003375818,28.4631913368726,-220.413708819391));
#201994=CARTESIAN_POINT('Ctrl Pts',(-56.4572435867786,31.0646235309543,
-217.273328544292));
#201995=CARTESIAN_POINT('Ctrl Pts',(-58.2910871452732,33.6689870195509,
-214.133955876969));
#201996=CARTESIAN_POINT('Ctrl Pts',(-47.2003193864821,18.1182964298664,
-233.015989564334));
#201997=CARTESIAN_POINT('Ctrl Pts',(-48.1493988764852,19.3809230047756,
-231.432724300644));
#201998=CARTESIAN_POINT('Ctrl Pts',(-49.0877568643722,20.6584395224563,
-229.855761293683));
#201999=CARTESIAN_POINT('Ctrl Pts',(-50.0215848134126,21.9412987456968,
-228.28073090895));
#202000=CARTESIAN_POINT('Ctrl Pts',(-50.9554127624531,23.2241579689375,
-226.705700524218));
#202001=CARTESIAN_POINT('Ctrl Pts',(-51.8844304624717,24.5129032830703,
-225.132894527219));
#202002=CARTESIAN_POINT('Ctrl Pts',(-52.811027126582,25.8043188185571,-223.561022084209));
#202003=CARTESIAN_POINT('Ctrl Pts',(-54.6642204548024,28.3871498895308,
-220.417277198188));
#202004=CARTESIAN_POINT('Ctrl Pts',(-56.5079518327106,30.9804583526794,
-217.27722687764));
#202005=CARTESIAN_POINT('Ctrl Pts',(-58.3485555395427,33.5765033299539,
-214.138113904034));
#202006=CARTESIAN_POINT('Ctrl Pts',(-47.2098674957262,18.0858618424364,
-233.021306146667));
#202007=CARTESIAN_POINT('Ctrl Pts',(-48.1660577345037,19.3384804806313,
-231.436445859109));
#202008=CARTESIAN_POINT('Ctrl Pts',(-49.1090703108757,20.6096704873925,
-229.859386110464));
#202009=CARTESIAN_POINT('Ctrl Pts',(-50.0473336065433,21.8864233995054,
-228.284270940977));
#202010=CARTESIAN_POINT('Ctrl Pts',(-50.9855969022109,23.1631763116183,
-226.709155771488));
#202011=CARTESIAN_POINT('Ctrl Pts',(-51.9186177626333,24.4464108695765,
-225.136458640789));
#202012=CARTESIAN_POINT('Ctrl Pts',(-52.8491949026841,25.7323667348012,
-223.564699625624));
#202013=CARTESIAN_POINT('Ctrl Pts',(-54.7103491827856,28.3042784652506,
-220.421181595292));
#202014=CARTESIAN_POINT('Ctrl Pts',(-56.5618994916621,30.8869590362523,
-217.281419567094));
#202015=CARTESIAN_POINT('Ctrl Pts',(-58.4105543383496,33.4721882778783,
-214.142529225918));
#202016=CARTESIAN_POINT('Ctrl Pts',(-47.2289637142144,18.0209926675766,
-233.031939311332));
#202017=CARTESIAN_POINT('Ctrl Pts',(-48.1993754505405,19.2535954323428,
-231.443888976038));
#202018=CARTESIAN_POINT('Ctrl Pts',(-49.1516972038829,20.512132417265,-229.866635744028));
#202019=CARTESIAN_POINT('Ctrl Pts',(-50.0988311928047,21.7766727071225,
-228.291351005029));
#202020=CARTESIAN_POINT('Ctrl Pts',(-51.0459651817265,23.0412129969801,
-226.716066266029));
#202021=CARTESIAN_POINT('Ctrl Pts',(-51.9869923629565,24.3134260425889,
-225.14358686793));
#202022=CARTESIAN_POINT('Ctrl Pts',(-52.9255304548883,25.5884625672894,
-223.572054708453));
#202023=CARTESIAN_POINT('Ctrl Pts',(-54.802606638752,28.1385356166903,-220.4289903895));
#202024=CARTESIAN_POINT('Ctrl Pts',(-56.6697948095651,30.6999604033981,
-217.289804946001));
#202025=CARTESIAN_POINT('Ctrl Pts',(-58.5345519359632,33.2635581737269,
-214.151359869686));
#202026=CARTESIAN_POINT('Ctrl Pts',(-47.2430220815907,17.9624777113029,
-233.042540471425));
#202027=CARTESIAN_POINT('Ctrl Pts',(-48.2273551133025,19.1720899539984,
-231.451949485653));
#202028=CARTESIAN_POINT('Ctrl Pts',(-49.1896659714189,20.4147736143863,
-229.87503540962));
#202029=CARTESIAN_POINT('Ctrl Pts',(-50.1472740382399,21.6628174682499,
-228.299725265682));
#202030=CARTESIAN_POINT('Ctrl Pts',(-51.1048821050609,22.9108613221134,
-226.724415121745));
#202031=CARTESIAN_POINT('Ctrl Pts',(-52.0562292256746,24.1671081729364,
-225.152079490178));
#202032=CARTESIAN_POINT('Ctrl Pts',(-53.0052546893374,25.4261024980228,
-223.580661790924));
#202033=CARTESIAN_POINT('Ctrl Pts',(-54.9033056166631,27.9440911481955,
-220.437826392414));
#202034=CARTESIAN_POINT('Ctrl Pts',(-56.7919721995556,30.4733633447205,
-217.298842424047));
#202035=CARTESIAN_POINT('Ctrl Pts',(-58.6785207415017,33.0046199530293,
-214.16054151441));
#202036=CARTESIAN_POINT('Ctrl Pts',(-47.2636279462708,17.8918194961353,
-233.049292072559));
#202037=CARTESIAN_POINT('Ctrl Pts',(-48.2527927601426,19.0896993463335,
-231.461117845357));
#202038=CARTESIAN_POINT('Ctrl Pts',(-49.2222701184903,20.3177090530585,
-229.885189443365));
#202039=CARTESIAN_POINT('Ctrl Pts',(-50.1877928495361,21.5503879875109,
-228.310673435979));
#202040=CARTESIAN_POINT('Ctrl Pts',(-51.1533155805818,22.7830669219633,
-226.736157428594));
#202041=CARTESIAN_POINT('Ctrl Pts',(-52.1134152350247,24.0230769225979,
-225.164293315049));
#202042=CARTESIAN_POINT('Ctrl Pts',(-53.0715402305708,25.265515738592,-223.593249605752));
#202043=CARTESIAN_POINT('Ctrl Pts',(-54.9877902216631,27.75039337058,-220.451162187155));
#202044=CARTESIAN_POINT('Ctrl Pts',(-56.8960314270369,30.2452705785478,
-217.312517061756));
#202045=CARTESIAN_POINT('Ctrl Pts',(-58.8025041724956,32.7418818204746,
-214.174488273677));
#202046=CARTESIAN_POINT('Ctrl Pts',(-47.2842338109509,17.8211612809678,
-233.056043673691));
#202047=CARTESIAN_POINT('Ctrl Pts',(-48.2782304069827,19.0073087386684,
-231.47028620506));
#202048=CARTESIAN_POINT('Ctrl Pts',(-49.2548742655618,20.2206444917306,
-229.89534347711));
#202049=CARTESIAN_POINT('Ctrl Pts',(-50.2283116608323,21.437958506772,-228.321621606276));
#202050=CARTESIAN_POINT('Ctrl Pts',(-51.2017490561027,22.6552725218134,
-226.747899735443));
#202051=CARTESIAN_POINT('Ctrl Pts',(-52.1706012443748,23.8790456722595,
-225.176507139922));
#202052=CARTESIAN_POINT('Ctrl Pts',(-53.1378257718042,25.1049289791612,
-223.60583742058));
#202053=CARTESIAN_POINT('Ctrl Pts',(-55.072274826663,27.5566955929646,-220.464497981896));
#202054=CARTESIAN_POINT('Ctrl Pts',(-57.0000906545182,30.0171778123751,
-217.326191699464));
#202055=CARTESIAN_POINT('Ctrl Pts',(-58.9264876034895,32.47914368792,-214.188435032943));
#202056=CARTESIAN_POINT('Ctrl Pts',(-47.2994830625051,17.7544372214138,
-233.064985179967));
#202057=CARTESIAN_POINT('Ctrl Pts',(-48.2988763150662,18.9260864440995,
-231.481022299027));
#202058=CARTESIAN_POINT('Ctrl Pts',(-49.2831180301545,20.12226670526,-229.90673458038));
#202059=CARTESIAN_POINT('Ctrl Pts',(-50.264622038348,21.3220097502749,-228.333564088779));
#202060=CARTESIAN_POINT('Ctrl Pts',(-51.2461260465415,22.5217527952899,
-226.760393597177));
#202061=CARTESIAN_POINT('Ctrl Pts',(-52.2236675241889,23.7273082081328,
-225.189324740538));
#202062=CARTESIAN_POINT('Ctrl Pts',(-53.199809818472,24.9347623794372,-223.618913074665));
#202063=CARTESIAN_POINT('Ctrl Pts',(-55.1520944070382,27.3496707220463,
-220.478089742921));
#202064=CARTESIAN_POINT('Ctrl Pts',(-57.0986707756308,29.7724235792233,
-217.34001940174));
#202065=CARTESIAN_POINT('Ctrl Pts',(-59.0440358271753,32.1965198188522,
-214.20245343815));
#202066=CARTESIAN_POINT('Ctrl Pts',(-47.3068095033878,17.6967086574683,
-233.077497779098));
#202067=CARTESIAN_POINT('Ctrl Pts',(-48.3116549954781,18.8520796703188,
-231.494638672248));
#202068=CARTESIAN_POINT('Ctrl Pts',(-49.3030451918381,20.0301039514678,
-229.920713549775));
#202069=CARTESIAN_POINT('Ctrl Pts',(-50.2920112564435,21.2114530404761,
-228.347855989514));
#202070=CARTESIAN_POINT('Ctrl Pts',(-51.280977321049,22.3928021294844,-226.774998429254));
#202071=CARTESIAN_POINT('Ctrl Pts',(-52.2664287923936,23.5795439345552,
-225.204106117501));
#202072=CARTESIAN_POINT('Ctrl Pts',(-53.2506399867227,24.7680561731562,
-223.633834433041));
#202073=CARTESIAN_POINT('Ctrl Pts',(-55.2190623753812,27.1450806503585,
-220.493291064124));
#202074=CARTESIAN_POINT('Ctrl Pts',(-57.1824244494106,29.5294142243635,
-217.355341819955));
#202075=CARTESIAN_POINT('Ctrl Pts',(-59.1447159484551,31.9150218118753,
-214.217874373197));
#202076=CARTESIAN_POINT('Ctrl Pts',(-47.3141359442706,17.638980093523,-233.090010378228));
#202077=CARTESIAN_POINT('Ctrl Pts',(-48.32443367589,18.7780728965381,-231.50825504547));
#202078=CARTESIAN_POINT('Ctrl Pts',(-49.3229723535216,19.9379411976756,
-229.93469251917));
#202079=CARTESIAN_POINT('Ctrl Pts',(-50.3194004745391,21.1008963306773,
-228.36214789025));
#202080=CARTESIAN_POINT('Ctrl Pts',(-51.3158285955566,22.2638514636789,
-226.78960326133));
#202081=CARTESIAN_POINT('Ctrl Pts',(-52.3091900605982,23.4317796609776,
-225.218887494463));
#202082=CARTESIAN_POINT('Ctrl Pts',(-53.3014701549735,24.6013499668753,
-223.648755791418));
#202083=CARTESIAN_POINT('Ctrl Pts',(-55.2860303437241,26.9404905786706,
-220.508492385326));
#202084=CARTESIAN_POINT('Ctrl Pts',(-57.2661781231904,29.2864048695037,
-217.370664238171));
#202085=CARTESIAN_POINT('Ctrl Pts',(-59.2453960697349,31.6335238048983,
-214.233295308244));
#202086=CARTESIAN_POINT('Ctrl Pts',(-47.3205362764709,17.5794518606674,
-233.102169725448));
#202087=CARTESIAN_POINT('Ctrl Pts',(-48.3341251295478,18.7044081787822,
-231.522433893026));
#202088=CARTESIAN_POINT('Ctrl Pts',(-49.338165710491,19.8469474114891,-229.949581699504));
#202089=CARTESIAN_POINT('Ctrl Pts',(-50.3405072447859,20.99216003676,-228.377642387885));
#202090=CARTESIAN_POINT('Ctrl Pts',(-51.3428487790808,22.1373726620309,
-226.805703076266));
#202091=CARTESIAN_POINT('Ctrl Pts',(-52.3427094024845,23.2868368796911,
-225.235339740797));
#202092=CARTESIAN_POINT('Ctrl Pts',(-53.3416967030123,24.4377161128276,
-223.665489068171));
#202093=CARTESIAN_POINT('Ctrl Pts',(-55.3396713040681,26.7394745791004,
-220.525787722919));
#202094=CARTESIAN_POINT('Ctrl Pts',(-57.334081396471,29.0470612357366,-217.388215315384));
#202095=CARTESIAN_POINT('Ctrl Pts',(-59.3277447200742,31.3557006527919,
-214.251054208451));
#202096=CARTESIAN_POINT('Ctrl Pts',(-47.3285982419782,17.5118110061916,
-233.112766042078));
#202097=CARTESIAN_POINT('Ctrl Pts',(-48.3441007183216,18.6236888893903,
-231.535741196264));
#202098=CARTESIAN_POINT('Ctrl Pts',(-49.3524346981868,19.7490902161012,
-229.963964803722));
#202099=CARTESIAN_POINT('Ctrl Pts',(-50.3595015772335,20.8765891331594,
-228.392921090687));
#202100=CARTESIAN_POINT('Ctrl Pts',(-51.3665684562802,22.0040880502176,
-226.821877377652));
#202101=CARTESIAN_POINT('Ctrl Pts',(-52.3717783622527,23.1348854144855,
-225.252060380076));
#202102=CARTESIAN_POINT('Ctrl Pts',(-53.3763360684624,24.2667864286898,
-223.682648344784));
#202103=CARTESIAN_POINT('Ctrl Pts',(-55.3854514808819,26.5305884570984,
-220.5438242742));
#202104=CARTESIAN_POINT('Ctrl Pts',(-57.3919042457265,28.7989304812669,
-217.40667659104));
#202105=CARTESIAN_POINT('Ctrl Pts',(-59.397804330835,31.0680944254412,-214.269858953779));
#202106=CARTESIAN_POINT('Ctrl Pts',(-47.3366602074855,17.444170151716,-233.123362358707));
#202107=CARTESIAN_POINT('Ctrl Pts',(-48.3540763070954,18.5429695999985,
-231.549048499502));
#202108=CARTESIAN_POINT('Ctrl Pts',(-49.3667036858826,19.6512330207133,
-229.97834790794));
#202109=CARTESIAN_POINT('Ctrl Pts',(-50.378495909681,20.7610182295588,-228.40819979349));
#202110=CARTESIAN_POINT('Ctrl Pts',(-51.3902881334795,21.8708034384043,
-226.83805167904));
#202111=CARTESIAN_POINT('Ctrl Pts',(-52.4008473220208,22.9829339492799,
-225.268781019355));
#202112=CARTESIAN_POINT('Ctrl Pts',(-53.4109754339125,24.0958567445521,
-223.699807621397));
#202113=CARTESIAN_POINT('Ctrl Pts',(-55.4312316576958,26.3217023350964,
-220.561860825481));
#202114=CARTESIAN_POINT('Ctrl Pts',(-57.4497270949821,28.5507997267972,
-217.425137866697));
#202115=CARTESIAN_POINT('Ctrl Pts',(-59.4678639415957,30.7804881980906,
-214.288663699106));
#202116=CARTESIAN_POINT('Ctrl Pts',(-47.3394631111059,17.3809856982998,
-233.13701868782));
#202117=CARTESIAN_POINT('Ctrl Pts',(-48.3594374346572,18.4637008192816,
-231.564473009033));
#202118=CARTESIAN_POINT('Ctrl Pts',(-49.3763048521849,19.5528780490395,
-229.994408187512));
#202119=CARTESIAN_POINT('Ctrl Pts',(-50.3925482040264,20.6432779103424,
-228.424798520261));
#202120=CARTESIAN_POINT('Ctrl Pts',(-51.4087915558678,21.7336777716453,
-226.85518885301));
#202121=CARTESIAN_POINT('Ctrl Pts',(-52.4241774034375,22.8258062072129,
-225.286233875719));
#202122=CARTESIAN_POINT('Ctrl Pts',(-53.4392506767952,23.9185477700511,
-223.717512563418));
#202123=CARTESIAN_POINT('Ctrl Pts',(-55.4693972235108,26.1040308957274,
-220.580069938817));
#202124=CARTESIAN_POINT('Ctrl Pts',(-57.4982777107523,28.2920062253737,
-217.443579202073));
#202125=CARTESIAN_POINT('Ctrl Pts',(-59.526890391898,30.4804660465043,-214.307294206909));
#202126=CARTESIAN_POINT('Ctrl Pts',(-47.3388947489722,17.3172597414177,
-233.15277350217));
#202127=CARTESIAN_POINT('Ctrl Pts',(-48.3602977670814,18.3855423142397,
-231.582083581833));
#202128=CARTESIAN_POINT('Ctrl Pts',(-49.3799313248768,19.4576103826212,
-230.012850342708));
#202129=CARTESIAN_POINT('Ctrl Pts',(-50.3991818891466,20.5304657339301,
-228.443915670914));
#202130=CARTESIAN_POINT('Ctrl Pts',(-51.4184324534164,21.6033210852391,
-226.874980999121));
#202131=CARTESIAN_POINT('Ctrl Pts',(-52.4371748506907,22.6772399564986,
-225.306453273624));
#202132=CARTESIAN_POINT('Ctrl Pts',(-53.4557277384216,23.7515480681017,
-223.738076580824));
#202133=CARTESIAN_POINT('Ctrl Pts',(-55.4928335138835,25.9001642913079,
-220.601323195224));
#202134=CARTESIAN_POINT('Ctrl Pts',(-57.529175347697,28.050353188994,-217.465180895102));
#202135=CARTESIAN_POINT('Ctrl Pts',(-59.5653551090103,30.2008561303528,
-214.329177297802));
#202136=CARTESIAN_POINT('Ctrl Pts',(-47.3383263868385,17.2535337845356,
-233.16852831652));
#202137=CARTESIAN_POINT('Ctrl Pts',(-48.3611580995056,18.3073838091979,
-231.599694154632));
#202138=CARTESIAN_POINT('Ctrl Pts',(-49.3835577975687,19.3623427162029,
-230.031292497904));
#202139=CARTESIAN_POINT('Ctrl Pts',(-50.4058155742669,20.4176535575179,
-228.463032821567));
#202140=CARTESIAN_POINT('Ctrl Pts',(-51.4280733509651,21.4729643988329,
-226.894773145231));
#202141=CARTESIAN_POINT('Ctrl Pts',(-52.4501722979439,22.5286737057843,
-225.326672671531));
#202142=CARTESIAN_POINT('Ctrl Pts',(-53.472204800048,23.5845483661524,-223.75864059823));
#202143=CARTESIAN_POINT('Ctrl Pts',(-55.5162698042562,25.6962976868884,
-220.622576451631));
#202144=CARTESIAN_POINT('Ctrl Pts',(-57.5600729846415,27.8087001526143,
-217.486782588132));
#202145=CARTESIAN_POINT('Ctrl Pts',(-59.6038198261226,29.9212462142014,
-214.351060388696));
#202146=CARTESIAN_POINT('Ctrl Pts',(-47.3375387814793,17.1823623301207,
-233.18377696202));
#202147=CARTESIAN_POINT('Ctrl Pts',(-48.3615298096416,18.2217514970558,
-231.616266612933));
#202148=CARTESIAN_POINT('Ctrl Pts',(-49.3856802662736,19.2607945266738,
-230.048626531198));
#202149=CARTESIAN_POINT('Ctrl Pts',(-50.4098664093718,20.299771974626,-228.480964758552));
#202150=CARTESIAN_POINT('Ctrl Pts',(-51.43405255247,21.3387494225781,-226.913302985906));
#202151=CARTESIAN_POINT('Ctrl Pts',(-52.4582849722416,22.377636554534,-225.34560994901));
#202152=CARTESIAN_POINT('Ctrl Pts',(-53.4825352205651,23.4164945474948,
-223.777908916675));
#202153=CARTESIAN_POINT('Ctrl Pts',(-55.5310357172121,25.4942105334166,
-220.642506852006));
#202154=CARTESIAN_POINT('Ctrl Pts',(-57.5796085089827,27.5718067803009,
-217.507071482923));
#202155=CARTESIAN_POINT('Ctrl Pts',(-59.6282062333003,29.6493743968087,
-214.371636285096));
#202156=CARTESIAN_POINT('Ctrl Pts',(-47.3352334252266,17.1035049830549,
-233.199529035477));
#202157=CARTESIAN_POINT('Ctrl Pts',(-48.3600042849483,18.1301783396072,
-231.632852310436));
#202158=CARTESIAN_POINT('Ctrl Pts',(-49.3851454200133,19.1559450105208,
-230.065825712809));
#202159=CARTESIAN_POINT('Ctrl Pts',(-50.4104205557466,20.1813828669923,
-228.498672133956));
#202160=CARTESIAN_POINT('Ctrl Pts',(-51.4356956914798,21.2068207234638,
-226.931518555102));
#202161=CARTESIAN_POINT('Ctrl Pts',(-52.4611193627566,22.2318946684557,
-225.364224580397));
#202162=CARTESIAN_POINT('Ctrl Pts',(-53.4866146769212,23.2567945291104,
-223.79686392097));
#202163=CARTESIAN_POINT('Ctrl Pts',(-55.5376053052503,25.3065942504197,
-220.662142602115));
#202164=CARTESIAN_POINT('Ctrl Pts',(-57.5888779614229,27.3557092766758,
-217.527159175984));
#202165=CARTESIAN_POINT('Ctrl Pts',(-59.6402468289299,29.4046011172088,
-214.392093753442));
#202166=CARTESIAN_POINT('Ctrl Pts',(-47.3340807471002,17.0640763095221,
-233.207405072206));
#202167=CARTESIAN_POINT('Ctrl Pts',(-48.3592415226016,18.084391760883,-231.641145159187));
#202168=CARTESIAN_POINT('Ctrl Pts',(-49.3848779968831,19.1035202524442,
-230.074425303614));
#202169=CARTESIAN_POINT('Ctrl Pts',(-50.4106976289339,20.1221883131755,
-228.507525821657));
#202170=CARTESIAN_POINT('Ctrl Pts',(-51.4365172609848,21.1408563739068,
-226.9406263397));
#202171=CARTESIAN_POINT('Ctrl Pts',(-52.4625365580142,22.1590237254166,
-225.373531896091));
#202172=CARTESIAN_POINT('Ctrl Pts',(-53.4886544050993,23.1769445199182,
-223.806341423117));
#202173=CARTESIAN_POINT('Ctrl Pts',(-55.5408900992694,25.2127861089213,
-220.671960477169));
#202174=CARTESIAN_POINT('Ctrl Pts',(-57.593512687643,27.2476605248632,-217.537203022514));
#202175=CARTESIAN_POINT('Ctrl Pts',(-59.6462671267447,29.2822144774089,
-214.402322487616));
#202176=CARTESIAN_POINT('Ctrl Pts',(-47.3300959856285,17.0287621384219,
-233.217844880347));
#202177=CARTESIAN_POINT('Ctrl Pts',(-48.3560378107335,18.0419554383925,
-231.651416226232));
#202178=CARTESIAN_POINT('Ctrl Pts',(-49.3823066249335,19.0542905470043,
-230.08464943573));
#202179=CARTESIAN_POINT('Ctrl Pts',(-50.4087248511739,20.0662312984004,
-228.517726367742));
#202180=CARTESIAN_POINT('Ctrl Pts',(-51.4351430774143,21.0781720497965,
-226.950803299753));
#202181=CARTESIAN_POINT('Ctrl Pts',(-52.4617184722238,22.0896985728052,
-225.383716267118));
#202182=CARTESIAN_POINT('Ctrl Pts',(-53.4883790234851,23.1010010173179,
-223.816540379752));
#202183=CARTESIAN_POINT('Ctrl Pts',(-55.5417001260078,25.1236059063434,
-220.68218860502));
#202184=CARTESIAN_POINT('Ctrl Pts',(-57.5953541578395,27.1453352451054,
-217.54748972819));
#202185=CARTESIAN_POINT('Ctrl Pts',(-59.6491347229493,29.1667389675576,
-214.412662365356));
#202186=CARTESIAN_POINT('Ctrl Pts',(-47.3252263828413,16.9896223025012,
-233.229110072315));
#202187=CARTESIAN_POINT('Ctrl Pts',(-48.3518314896857,17.9964142568803,
-231.662398987523));
#202188=CARTESIAN_POINT('Ctrl Pts',(-49.3786544580299,19.0026193721543,
-230.095454289591));
#202189=CARTESIAN_POINT('Ctrl Pts',(-50.4055851760868,20.0085325545711,
-228.528392739382));
#202190=CARTESIAN_POINT('Ctrl Pts',(-51.4325158941438,21.0144457369877,
-226.961331189173));
#202191=CARTESIAN_POINT('Ctrl Pts',(-52.459558588544,22.0200559113108,-225.394148461867));
#202192=CARTESIAN_POINT('Ctrl Pts',(-53.4866652007083,23.0254932317529,
-223.826896445521));
#202193=CARTESIAN_POINT('Ctrl Pts',(-55.5408784250369,25.0363678726369,
-220.692392412828));
#202194=CARTESIAN_POINT('Ctrl Pts',(-57.5953414810798,27.046567195329,-217.557617709049));
#202195=CARTESIAN_POINT('Ctrl Pts',(-59.6499065909155,29.0564953668167,
-214.422734451764));
#202196=CARTESIAN_POINT('Ctrl Pts',(-47.3227915814476,16.9700523845408,
-233.234742668299));
#202197=CARTESIAN_POINT('Ctrl Pts',(-48.3497283291618,17.9736436661242,
-231.667890368169));
#202198=CARTESIAN_POINT('Ctrl Pts',(-49.3768283745781,18.9767837847294,
-230.100856716523));
#202199=CARTESIAN_POINT('Ctrl Pts',(-50.4040153385433,19.9796831826563,
-228.533725925203));
#202200=CARTESIAN_POINT('Ctrl Pts',(-51.4312023025085,20.9825825805833,
-226.966595133883));
#202201=CARTESIAN_POINT('Ctrl Pts',(-52.4584786467041,21.9852345805636,
-225.399364559241));
#202202=CARTESIAN_POINT('Ctrl Pts',(-53.4858082893199,22.9877393389703,
-223.832074478405));
#202203=CARTESIAN_POINT('Ctrl Pts',(-55.5404675745514,24.9927488557837,
-220.697494316732));
#202204=CARTESIAN_POINT('Ctrl Pts',(-57.5953351427,26.9971831704407,-217.562681699479));
#202205=CARTESIAN_POINT('Ctrl Pts',(-59.6502925248986,29.0013735664462,
-214.427770494967));
#202206=CARTESIAN_POINT('Ctrl Pts',(-47.3201275842246,16.9495165547055,
-233.240576377928));
#202207=CARTESIAN_POINT('Ctrl Pts',(-48.3473719504709,17.9500807957729,
-231.67355223474));
#202208=CARTESIAN_POINT('Ctrl Pts',(-49.3747299988842,18.9503241764231,
-230.106397960498));
#202209=CARTESIAN_POINT('Ctrl Pts',(-50.4021522240997,19.9503861234,-228.539169864665));
#202210=CARTESIAN_POINT('Ctrl Pts',(-51.4295744493152,20.9504480703769,
-226.97194176883));
#202211=CARTESIAN_POINT('Ctrl Pts',(-52.4570622538851,21.9503247000739,
-225.40463829887));
#202212=CARTESIAN_POINT('Ctrl Pts',(-53.4845908245458,22.9500863858554,
-223.837287994071));
#202213=CARTESIAN_POINT('Ctrl Pts',(-55.539647965867,24.9496097574185,-220.702587384473));
#202214=CARTESIAN_POINT('Ctrl Pts',(-57.5948645555888,26.9486836845843,
-217.56770364283));
#202215=CARTESIAN_POINT('Ctrl Pts',(-59.6501540472924,28.9475552769007,
-214.432737386764));
#202216=CARTESIAN_POINT('Ctrl Pts',(-47.317375174873,16.9271166732568,-233.246414795271));
#202217=CARTESIAN_POINT('Ctrl Pts',(-48.3448826696721,17.9249382396269,
-231.679221637881));
#202218=CARTESIAN_POINT('Ctrl Pts',(-49.3724670545446,18.9225395323645,
-230.111938592781));
#202219=CARTESIAN_POINT('Ctrl Pts',(-50.4000965635423,19.9200114073275,
-228.544602587596));
#202220=CARTESIAN_POINT('Ctrl Pts',(-51.42772607254,20.9174832822903,-226.977266582412));
#202221=CARTESIAN_POINT('Ctrl Pts',(-52.4554015221151,21.9148234426101,
-225.409876692422));
#202222=CARTESIAN_POINT('Ctrl Pts',(-53.4831063385788,22.9120795922463,
-223.842452376097));
#202223=CARTESIAN_POINT('Ctrl Pts',(-55.5385159715063,24.9065918915186,
-220.707603743446));
#202224=CARTESIAN_POINT('Ctrl Pts',(-57.5940405653775,26.9007754041514,
-217.572620374409));
#202225=CARTESIAN_POINT('Ctrl Pts',(-59.6496198849772,28.8948045789125,
-214.437573677779));
#202226=CARTESIAN_POINT('Ctrl Pts',(-47.3159989701972,16.9159167325326,
-233.249334003942));
#202227=CARTESIAN_POINT('Ctrl Pts',(-48.3436380292726,17.9123669615539,
-231.682056339452));
#202228=CARTESIAN_POINT('Ctrl Pts',(-49.3713355823747,18.9086472103352,
-230.114708908922));
#202229=CARTESIAN_POINT('Ctrl Pts',(-50.3990687332636,19.9048240492912,
-228.547318949062));
#202230=CARTESIAN_POINT('Ctrl Pts',(-51.4268018841524,20.9010008882471,
-226.979928989203));
#202231=CARTESIAN_POINT('Ctrl Pts',(-52.45457115623,21.8970728138782,-225.412495889199));
#202232=CARTESIAN_POINT('Ctrl Pts',(-53.4823640955953,22.8930761954416,
-223.84503456711));
#202233=CARTESIAN_POINT('Ctrl Pts',(-55.537949974326,24.8850829585685,-220.710111922933));
#202234=CARTESIAN_POINT('Ctrl Pts',(-57.5936285702719,26.8768212639349,
-217.575078740198));
#202235=CARTESIAN_POINT('Ctrl Pts',(-59.6493528038196,28.8684292299185,
-214.439991823286));
#202236=CARTESIAN_POINT('Ctrl Pts',(-47.3145992078122,16.9042529363287,
-233.252255026597));
#202237=CARTESIAN_POINT('Ctrl Pts',(-48.342359204181,17.8994019124442,-231.684893211564));
#202238=CARTESIAN_POINT('Ctrl Pts',(-49.3701622440295,18.8944243694381,
-230.117479224879));
#202239=CARTESIAN_POINT('Ctrl Pts',(-50.3979922061516,19.8893677455407,
-228.55003257268));
#202240=CARTESIAN_POINT('Ctrl Pts',(-51.4258221682736,20.8843111216433,
-226.982585920481));
#202241=CARTESIAN_POINT('Ctrl Pts',(-52.4536793921196,21.8791744293876,
-225.41510619931));
#202242=CARTESIAN_POINT('Ctrl Pts',(-53.4815548458549,22.8739843484231,
-223.847604402904));
#202243=CARTESIAN_POINT('Ctrl Pts',(-55.5373057533255,24.8636041864943,
-220.712600810094));
#202244=CARTESIAN_POINT('Ctrl Pts',(-57.5931281378066,26.8530147412008,
-217.577510678694));
#202245=CARTESIAN_POINT('Ctrl Pts',(-59.6489867620326,28.8423205147682,
-214.442377165073));
#202246=CARTESIAN_POINT('Ctrl Pts',(-47.3131850756779,16.8920273532507,
-233.255157881008));
#202247=CARTESIAN_POINT('Ctrl Pts',(-48.3410552958596,17.8859535740668,
-231.68771449894));
#202248=CARTESIAN_POINT('Ctrl Pts',(-49.3689559345468,18.8797895866585,
-230.120233792132));
#202249=CARTESIAN_POINT('Ctrl Pts',(-50.3968759670817,19.8735681235901,
-228.552729269786));
#202250=CARTESIAN_POINT('Ctrl Pts',(-51.4247959996165,20.8673466605217,
-226.98522474744));
#202251=CARTESIAN_POINT('Ctrl Pts',(-52.4527356437508,21.8610670819393,
-225.417696146955));
#202252=CARTESIAN_POINT('Ctrl Pts',(-53.4806885888443,22.8547481865589,
-223.850151240679));
#202253=CARTESIAN_POINT('Ctrl Pts',(-55.5365944790313,24.8421103957982,
-220.715061428126));
#202254=CARTESIAN_POINT('Ctrl Pts',(-57.5925525533974,26.8293183807281,
-217.579907651647));
#202255=CARTESIAN_POINT('Ctrl Pts',(-59.6485376230928,28.8164474339779,
-214.444721098757));
#202256=CARTESIAN_POINT('Ctrl Pts',(-47.3124780096108,16.8859145617117,
-233.256609308214));
#202257=CARTESIAN_POINT('Ctrl Pts',(-48.3404033416989,17.879229404878,-231.689125142628));
#202258=CARTESIAN_POINT('Ctrl Pts',(-49.3683527798054,18.8724721952687,
-230.121611075758));
#202259=CARTESIAN_POINT('Ctrl Pts',(-50.3963178475467,19.8656683126149,
-228.554077618338));
#202260=CARTESIAN_POINT('Ctrl Pts',(-51.424282915288,20.8588644299609,-226.986544160919));
#202261=CARTESIAN_POINT('Ctrl Pts',(-52.4522637695665,21.8520134082152,
-225.418991120778));
#202262=CARTESIAN_POINT('Ctrl Pts',(-53.480255460339,22.8451301056268,-223.851424659566));
#202263=CARTESIAN_POINT('Ctrl Pts',(-55.5362388418842,24.83136350045,-220.716291737142));
#202264=CARTESIAN_POINT('Ctrl Pts',(-57.5922647611927,26.8174702004918,
-217.581106138124));
#202265=CARTESIAN_POINT('Ctrl Pts',(-59.6483130536229,28.8035108935828,
-214.4458930656));
#202266=CARTESIAN_POINT('Ctrl Pts',(-47.3117672667176,16.8796614828891,
-233.258056246654));
#202267=CARTESIAN_POINT('Ctrl Pts',(-48.3397450538273,17.8723845217414,
-231.690531924442));
#202268=CARTESIAN_POINT('Ctrl Pts',(-49.3677413331199,18.8650518969515,
-230.122984445821));
#202269=CARTESIAN_POINT('Ctrl Pts',(-50.3957497606693,19.8576827301003,
-228.555421751598));
#202270=CARTESIAN_POINT('Ctrl Pts',(-51.4237581882186,20.8503135632492,
-226.987859057374));
#202271=CARTESIAN_POINT('Ctrl Pts',(-52.4517788757404,21.8429075199303,
-225.420281009185));
#202272=CARTESIAN_POINT('Ctrl Pts',(-53.4798080609562,22.835475963723,-223.852692331251));
#202273=CARTESIAN_POINT('Ctrl Pts',(-55.5358664313876,24.8206128513086,
-220.717514975384));
#202274=CARTESIAN_POINT('Ctrl Pts',(-57.5919581746568,26.8056495551953,
-217.582295877378));
#202275=CARTESIAN_POINT('Ctrl Pts',(-59.6480677075794,28.790633246673,-214.447054670791));
#202276=CARTESIAN_POINT('Ctrl Pts',(-47.3110535174895,16.873256830116,-233.259496526039));
#202277=CARTESIAN_POINT('Ctrl Pts',(-48.3390812029547,17.8654084135782,
-231.691932847844));
#202278=CARTESIAN_POINT('Ctrl Pts',(-49.3671224159146,18.8575190179354,
-230.124352092621));
#202279=CARTESIAN_POINT('Ctrl Pts',(-50.3951725945636,19.8496024611769,
-228.556760010403));
#202280=CARTESIAN_POINT('Ctrl Pts',(-51.4232227732125,20.8416859044184,
-226.989167928185));
#202281=CARTESIAN_POINT('Ctrl Pts',(-52.4512819949066,21.8337419536198,
-225.421564422348));
#202282=CARTESIAN_POINT('Ctrl Pts',(-53.4793475235956,22.8257789108232,
-223.853952950714));
#202283=CARTESIAN_POINT('Ctrl Pts',(-55.5354785809735,24.8098528252302,
-220.718730007446));
#202284=CARTESIAN_POINT('Ctrl Pts',(-57.5916344152767,26.7938517410564,
-217.583475771517));
#202285=CARTESIAN_POINT('Ctrl Pts',(-59.6478035550371,28.7778105309341,
-214.448204781494));
#202286=CARTESIAN_POINT('Ctrl Pts',(-47.3103397682614,16.8668521773429,
-233.260936805424));
#202287=CARTESIAN_POINT('Ctrl Pts',(-48.3384173520821,17.8584323054149,
-231.693333771247));
#202288=CARTESIAN_POINT('Ctrl Pts',(-49.3665034987094,18.8499861389194,
-230.125719739421));
#202289=CARTESIAN_POINT('Ctrl Pts',(-50.3945954284579,19.8415221922535,
-228.558098269208));
#202290=CARTESIAN_POINT('Ctrl Pts',(-51.4226873582065,20.8330582455877,
-226.990476798996));
#202291=CARTESIAN_POINT('Ctrl Pts',(-52.4507851140727,21.8245763873091,
-225.422847835511));
#202292=CARTESIAN_POINT('Ctrl Pts',(-53.4788869862349,22.8160818579234,
-223.855213570177));
#202293=CARTESIAN_POINT('Ctrl Pts',(-55.5350907305594,24.7990927991518,
-220.719945039509));
#202294=CARTESIAN_POINT('Ctrl Pts',(-57.5913106558967,26.7820539269176,
-217.584655665656));
#202295=CARTESIAN_POINT('Ctrl Pts',(-59.6475394024948,28.7649878151953,
-214.449354892196));
#202296=CARTESIAN_POINT('Ctrl Pts',(-47.3110520982437,16.8559465263517,
-233.26053824229));
#202297=CARTESIAN_POINT('Ctrl Pts',(-48.3391380137511,17.8470909658639,
-231.692946212383));
#202298=CARTESIAN_POINT('Ctrl Pts',(-49.3672339116285,18.8382047449221,
-230.125341393407));
#202299=CARTESIAN_POINT('Ctrl Pts',(-50.3953364602535,19.82929801124,-228.55772801405));
#202300=CARTESIAN_POINT('Ctrl Pts',(-51.4234390088786,20.8203912775578,
-226.990114634692));
#202301=CARTESIAN_POINT('Ctrl Pts',(-52.4515482625761,21.8114638664511,
-225.422492626496));
#202302=CARTESIAN_POINT('Ctrl Pts',(-53.4796622004807,22.8025219415151,
-223.854864559695));
#202303=CARTESIAN_POINT('Ctrl Pts',(-55.5358900762899,24.7846380916432,
-220.719608426093));
#202304=CARTESIAN_POINT('Ctrl Pts',(-57.5921363546469,26.7666972063695,
-217.58432848346));
#202305=CARTESIAN_POINT('Ctrl Pts',(-59.6483924596735,28.7487254799229,
-214.449035662994));
#202306=CARTESIAN_POINT('Ctrl Pts',(-47.3114554705886,16.8460380888807,
-233.260539515782));
#202307=CARTESIAN_POINT('Ctrl Pts',(-48.3395590816568,17.8367146054412,
-231.692947455239));
#202308=CARTESIAN_POINT('Ctrl Pts',(-49.3676726219367,18.8273604593628,
-230.125342611939));
#202309=CARTESIAN_POINT('Ctrl Pts',(-50.3957927612346,19.8179857984423,
-228.557729212486));
#202310=CARTESIAN_POINT('Ctrl Pts',(-51.4239129005325,20.8086111375217,
-226.990115813032));
#202311=CARTESIAN_POINT('Ctrl Pts',(-52.4520396931497,21.7992157970736,
-225.422493789));
#202312=CARTESIAN_POINT('Ctrl Pts',(-53.480171119088,22.7898059407486,-223.854865709355));
#202313=CARTESIAN_POINT('Ctrl Pts',(-55.5364339709647,24.7709862280985,
-220.719609550066));
#202314=CARTESIAN_POINT('Ctrl Pts',(-57.5927150219887,26.7521094718628,
-217.584329593504));
#202315=CARTESIAN_POINT('Ctrl Pts',(-59.6490056999632,28.7332018665566,
-214.449036765473));
#202316=CARTESIAN_POINT('',(-47.0649767742812,18.6816981840219,-232.850050031414));
#202317=CARTESIAN_POINT('',(-47.5797438888055,17.1282946860168,-232.850050025775));
#202318=CARTESIAN_POINT('Ctrl Pts',(-47.0649772746806,18.681698503234,-232.85005));
#202319=CARTESIAN_POINT('Ctrl Pts',(-47.0897739050568,18.6428271142161,
-232.85005));
#202320=CARTESIAN_POINT('Ctrl Pts',(-47.1311006982707,18.5775957466655,
-232.850050000004));
#202321=CARTESIAN_POINT('Ctrl Pts',(-47.194785050436,18.4616925010307,-232.850050000004));
#202322=CARTESIAN_POINT('Ctrl Pts',(-47.2287770053728,18.3950676863438,
-232.850049999972));
#202323=CARTESIAN_POINT('Ctrl Pts',(-47.294963678024,18.2630532098196,-232.850049999972));
#202324=CARTESIAN_POINT('Ctrl Pts',(-47.3298979480949,18.1874159971604,
-232.850050000077));
#202325=CARTESIAN_POINT('Ctrl Pts',(-47.3845235381683,18.0516462813532,
-232.850050000077));
#202326=CARTESIAN_POINT('Ctrl Pts',(-47.4068726947903,17.992614936778,-232.850050003188));
#202327=CARTESIAN_POINT('Ctrl Pts',(-47.4814502842607,17.7794293002805,
-232.850050003188));
#202328=CARTESIAN_POINT('Ctrl Pts',(-47.5068744752097,17.6686904849674,
-232.85005000024));
#202329=CARTESIAN_POINT('Ctrl Pts',(-47.5415713170795,17.4960000874156,
-232.85005000024));
#202330=CARTESIAN_POINT('Ctrl Pts',(-47.5519413173953,17.4283876884363,
-232.85005));
#202331=CARTESIAN_POINT('Ctrl Pts',(-47.5744439294891,17.2490905556932,
-232.85005));
#202332=CARTESIAN_POINT('Ctrl Pts',(-47.5778164032854,17.1751517854889,
-232.85005));
#202333=CARTESIAN_POINT('Ctrl Pts',(-47.5797441362696,17.1282946961977,
-232.85005));
#202334=CARTESIAN_POINT('',(-57.6802384504567,34.1916870210802,-214.317651768483));
#202335=CARTESIAN_POINT('Ctrl Pts',(-47.0649765291407,18.6816980387269,
-232.850049769526));
#202336=CARTESIAN_POINT('Ctrl Pts',(-48.8271545273793,21.2716434707432,
-229.763670058287));
#202337=CARTESIAN_POINT('Ctrl Pts',(-50.591632449928,23.8587524581056,-226.676983143055));
#202338=CARTESIAN_POINT('Ctrl Pts',(-52.3593744293695,26.4424372048812,
-223.590052929728));
#202339=CARTESIAN_POINT('Ctrl Pts',(-54.1292305723972,29.029211957027,-220.499430845344));
#202340=CARTESIAN_POINT('Ctrl Pts',(-55.9023386650238,31.6125563678527,
-217.408555364207));
#202341=CARTESIAN_POINT('Ctrl Pts',(-57.6802383718549,34.1916869226675,
-214.317651641153));
#202342=CARTESIAN_POINT('',(-59.5599473199192,29.0716011550534,-214.548757454512));
#202343=CARTESIAN_POINT('Ctrl Pts',(-57.6802384190918,34.1916870036612,
-214.317652095804));
#202344=CARTESIAN_POINT('Ctrl Pts',(-57.711076640637,34.1523839213935,-214.318515519703));
#202345=CARTESIAN_POINT('Ctrl Pts',(-57.7444787407025,34.1091244974209,
-214.319516304586));
#202346=CARTESIAN_POINT('Ctrl Pts',(-57.8155385849082,34.015034636639,-214.321768181642));
#202347=CARTESIAN_POINT('Ctrl Pts',(-57.8508234071904,33.9673227106125,
-214.32296093355));
#202348=CARTESIAN_POINT('Ctrl Pts',(-57.9661234018488,33.808083144089,-214.32727701056));
#202349=CARTESIAN_POINT('Ctrl Pts',(-58.0434074298098,33.6958767305163,
-214.331195699283));
#202350=CARTESIAN_POINT('Ctrl Pts',(-58.1756532244509,33.494224655047,-214.338033936497));
#202351=CARTESIAN_POINT('Ctrl Pts',(-58.232181736934,33.4045586829591,-214.340952245208));
#202352=CARTESIAN_POINT('Ctrl Pts',(-58.3756461184004,33.1676840614597,
-214.348689659445));
#202353=CARTESIAN_POINT('Ctrl Pts',(-58.4602479257778,33.0184255663356,
-214.353756590895));
#202354=CARTESIAN_POINT('Ctrl Pts',(-58.6568844792436,32.6464976653465,
-214.368544945655));
#202355=CARTESIAN_POINT('Ctrl Pts',(-58.7646217839408,32.4201536609433,
-214.377793138464));
#202356=CARTESIAN_POINT('Ctrl Pts',(-58.9195386091013,32.0554702583991,
-214.392846705456));
#202357=CARTESIAN_POINT('Ctrl Pts',(-58.9732785720301,31.9197057886375,
-214.398754579606));
#202358=CARTESIAN_POINT('Ctrl Pts',(-59.1078149579114,31.5535708296281,
-214.415391307452));
#202359=CARTESIAN_POINT('Ctrl Pts',(-59.1824588553433,31.3211191065939,
-214.426591762046));
#202360=CARTESIAN_POINT('Ctrl Pts',(-59.2717173594901,30.9979484732358,
-214.442018247786));
#202361=CARTESIAN_POINT('Ctrl Pts',(-59.2947355260442,30.9092561462526,
-214.446284061646));
#202362=CARTESIAN_POINT('Ctrl Pts',(-59.3544699104766,30.6634680433675,
-214.458293748765));
#202363=CARTESIAN_POINT('Ctrl Pts',(-59.3882196655572,30.5059342511556,
-214.466398394897));
#202364=CARTESIAN_POINT('Ctrl Pts',(-59.4590872539795,30.1244208307377,
-214.487274531048));
#202365=CARTESIAN_POINT('Ctrl Pts',(-59.492072393894,29.8990070152149,-214.499666866019));
#202366=CARTESIAN_POINT('Ctrl Pts',(-59.5376880887931,29.4727426572454,
-214.524039704186));
#202367=CARTESIAN_POINT('Ctrl Pts',(-59.5522340174229,29.2722643299,-214.536262708201));
#202368=CARTESIAN_POINT('Ctrl Pts',(-59.559947319918,29.0716011550592,-214.548757454604));
#202369=CARTESIAN_POINT('',(-59.5744430571196,28.6979747816093,-214.56059856522));
#202370=CARTESIAN_POINT('Ctrl Pts',(-59.5599473199158,29.0716011550593,
-214.548757454608));
#202371=CARTESIAN_POINT('Ctrl Pts',(-59.562335847696,29.0094631058835,-214.552626620787));
#202372=CARTESIAN_POINT('Ctrl Pts',(-59.5647394386419,28.9472090864927,
-214.555583575921));
#202373=CARTESIAN_POINT('Ctrl Pts',(-59.5683821822733,28.8533107884066,
-214.558574296067));
#202374=CARTESIAN_POINT('Ctrl Pts',(-59.5696089211159,28.8217653832972,
-214.559329741406));
#202375=CARTESIAN_POINT('Ctrl Pts',(-59.5720174159227,28.7599810676145,
-214.560318279807));
#202376=CARTESIAN_POINT('Ctrl Pts',(-59.5727190081475,28.7420025676919,
-214.5605526967));
#202377=CARTESIAN_POINT('Ctrl Pts',(-59.5744429767042,28.6979747794686,
-214.560599513176));
#202378=CARTESIAN_POINT('Ctrl Pts',(-59.5744427861971,28.6979745676234,
-214.560598252186));
#202379=CARTESIAN_POINT('Ctrl Pts',(-55.5761465166849,24.8416079159138,
-220.657162906121));
#202380=CARTESIAN_POINT('Ctrl Pts',(-51.5778799971753,20.9851500975526,
-226.753689417593));
#202381=CARTESIAN_POINT('Ctrl Pts',(-47.5797437329671,17.1282947147807,
-232.85004994177));
#202382=CARTESIAN_POINT('Origin',(-41.5452362233251,-63.7990866568863,-205.306318983907));
#202383=CARTESIAN_POINT('',(-47.2772325636527,-70.8123207858077,-202.84995));
#202384=CARTESIAN_POINT('',(-41.9017397792002,-72.8497297394107,-202.84995));
#202385=CARTESIAN_POINT('Origin',(-41.5452362233251,-63.7990866568863,-202.84995));
#202386=CARTESIAN_POINT('',(-41.9000522051254,-72.8068868830794,-205.306318983907));
#202387=CARTESIAN_POINT('',(-47.1516276096018,-70.6586401308143,-214.220867040027));
#202388=CARTESIAN_POINT('Ctrl Pts',(-47.1516276096073,-70.658640130818,
-214.220867039664));
#202389=CARTESIAN_POINT('Ctrl Pts',(-47.1049465298323,-70.69680049246,-214.220539579083));
#202390=CARTESIAN_POINT('Ctrl Pts',(-47.0581254645236,-70.7342797725851,
-214.220714572147));
#202391=CARTESIAN_POINT('Ctrl Pts',(-46.9626662222933,-70.8090665014231,
-214.222095580797));
#202392=CARTESIAN_POINT('Ctrl Pts',(-46.9147757072847,-70.8457911604741,
-214.22327290135));
#202393=CARTESIAN_POINT('Ctrl Pts',(-46.8664918175106,-70.8820283127247,
-214.224988432219));
#202394=CARTESIAN_POINT('',(-47.250099122033,-70.7791223733342,-205.306318983907));
#202395=CARTESIAN_POINT('Origin',(0.,-12.9675000200281,-205.306318983907));
#202396=CARTESIAN_POINT('Ctrl Pts',(-50.9302694868398,-67.3511117059353,
-214.24934096937));
#202397=CARTESIAN_POINT('Ctrl Pts',(-50.6301450874489,-67.632232782722,
-214.247062743179));
#202398=CARTESIAN_POINT('Ctrl Pts',(-50.3277270490238,-67.9108411525188,
-214.244646208669));
#202399=CARTESIAN_POINT('Ctrl Pts',(-49.7080810419159,-68.4722815054349,
-214.240153263143));
#202400=CARTESIAN_POINT('Ctrl Pts',(-49.3907687173044,-68.7548784334755,
-214.238095007483));
#202401=CARTESIAN_POINT('Ctrl Pts',(-48.4391587456012,-69.5878975441349,
-214.231198509907));
#202402=CARTESIAN_POINT('Ctrl Pts',(-47.7996962354631,-70.1288637578241,
-214.22541314119));
#202403=CARTESIAN_POINT('Ctrl Pts',(-47.1516276096073,-70.658640130818,
-214.220867039664));
#202404=CARTESIAN_POINT('',(-57.55661147574,-60.2824542804282,-214.249782619794));
#202405=CARTESIAN_POINT('Ctrl Pts',(-57.5566114760922,-60.2824542808246,
-214.249782589791));
#202406=CARTESIAN_POINT('Ctrl Pts',(-57.0250153197209,-60.929054875926,
-214.252086125668));
#202407=CARTESIAN_POINT('Ctrl Pts',(-56.4825490090204,-61.5666907434623,
-214.255305282271));
#202408=CARTESIAN_POINT('Ctrl Pts',(-55.3753515248431,-62.8244435222611,
-214.258374348072));
#202409=CARTESIAN_POINT('Ctrl Pts',(-54.8117226671775,-63.4434099521044,
-214.259195881147));
#202410=CARTESIAN_POINT('Ctrl Pts',(-54.2386983288856,-64.0517945375328,
-214.260116172733));
#202411=CARTESIAN_POINT('',(-57.7103246972002,-60.4088156810276,-202.84995));
#202412=CARTESIAN_POINT('',(-57.677203474973,-60.3815880685163,-205.306318983907));
#202413=CARTESIAN_POINT('Origin',(0.,-12.9675000200281,-202.84995));
#202414=CARTESIAN_POINT('Origin',(-50.7133971693864,-54.6569255427236,-205.306318983907));
#202415=CARTESIAN_POINT('',(-59.7639914300581,-55.014666400457,-202.84995));
#202416=CARTESIAN_POINT('Origin',(-50.7133971693864,-54.6569255427236,-202.84995));
#202417=CARTESIAN_POINT('Origin',(-53.6115278221397,-57.0237333927552,-218.549922256745));
#202418=CARTESIAN_POINT('',(-59.7211488048338,-55.0129729693901,-205.306318983907));
#202419=CARTESIAN_POINT('Origin',(-50.7133971693864,28.7219255026674,-205.306318983907));
#202420=CARTESIAN_POINT('',(-57.7103246972002,34.4738156409714,-202.84995));
#202421=CARTESIAN_POINT('',(-59.7639914300583,29.0796663604006,-202.84995));
#202422=CARTESIAN_POINT('Origin',(-50.7133971693864,28.7219255026674,-202.84995));
#202423=CARTESIAN_POINT('',(-59.7211488048339,29.0779729293336,-205.306318983907));
#202424=CARTESIAN_POINT('',(-57.555715349607,34.3467175710979,-214.316254908503));
#202425=CARTESIAN_POINT('Origin',(-53.918424535989,31.3368194791983,-218.660877916293));
#202426=CARTESIAN_POINT('',(-57.677203474973,34.44658802846,-205.306318983907));
#202427=CARTESIAN_POINT('Origin',(0.,-12.9675000200281,-205.306318983907));
#202428=CARTESIAN_POINT('',(-46.8872094279775,44.936516366183,-214.320099730218));
#202429=CARTESIAN_POINT('Ctrl Pts',(-46.8872094285464,44.9365163666477,
-214.32009968902));
#202430=CARTESIAN_POINT('Ctrl Pts',(-47.5890114515051,44.368165416605,-214.323378596591));
#202431=CARTESIAN_POINT('Ctrl Pts',(-48.2806521881363,43.7869284638981,
-214.327270067522));
#202432=CARTESIAN_POINT('Ctrl Pts',(-49.2784687584601,42.9168915640759,
-214.330851585581));
#202433=CARTESIAN_POINT('Ctrl Pts',(-49.5914691205952,42.6393040561203,
-214.331776628684));
#202434=CARTESIAN_POINT('Ctrl Pts',(-50.2053425551683,42.0855623761046,
-214.333899644539));
#202435=CARTESIAN_POINT('Ctrl Pts',(-50.506054266235,41.8097922959792,-214.335007679769));
#202436=CARTESIAN_POINT('Ctrl Pts',(-50.804536443953,41.5315226006458,-214.335913275952));
#202437=CARTESIAN_POINT('',(-47.0132029332902,45.0921138114136,-202.84995));
#202438=CARTESIAN_POINT('',(-46.9862210240714,45.0587921244845,-205.306318983907));
#202439=CARTESIAN_POINT('Origin',(0.,-12.9675000200281,-202.84995));
#202440=CARTESIAN_POINT('Ctrl Pts',(-54.1218033362461,38.2387592926023,
-214.333529894748));
#202441=CARTESIAN_POINT('Ctrl Pts',(-54.3992526046939,37.9455431189732,
-214.332337047462));
#202442=CARTESIAN_POINT('Ctrl Pts',(-54.6742923213544,37.6501031166571,
-214.331036263298));
#202443=CARTESIAN_POINT('Ctrl Pts',(-55.2277092285518,37.0458584843467,
-214.328741493667));
#202444=CARTESIAN_POINT('Ctrl Pts',(-55.5058839842676,36.7369811431027,
-214.327762901693));
#202445=CARTESIAN_POINT('Ctrl Pts',(-56.3870207183081,35.7419812347418,
-214.323805214881));
#202446=CARTESIAN_POINT('Ctrl Pts',(-56.9779401341808,35.0494690118534,
-214.319418635742));
#202447=CARTESIAN_POINT('Ctrl Pts',(-57.5557151719484,34.346717423436,-214.316255263493));
#202448=CARTESIAN_POINT('Origin',(-41.3132181298675,38.0528376956935,-205.306318983907));
#202449=CARTESIAN_POINT('',(-43.0099907914441,46.9501517582364,-202.84995));
#202450=CARTESIAN_POINT('Origin',(-41.3132181298675,38.0528376956935,-202.84995));
#202451=CARTESIAN_POINT('Origin',(-43.9075665164217,41.2822320849722,-218.664372653694));
#202452=CARTESIAN_POINT('',(-43.001958811097,46.9080347125589,-205.306318983907));
#202453=CARTESIAN_POINT('Origin',(1004.,-12.967500020028,-179.606318983907));
#202454=CARTESIAN_POINT('',(-62.6666822880186,29.1944003864053,-179.64995));
#202455=CARTESIAN_POINT('',(-62.6666822880186,-55.1294004264619,-179.64995));
#202456=CARTESIAN_POINT('Origin',(1004.,-12.967500020028,-179.64995));
#202457=CARTESIAN_POINT('',(-62.2620407574844,-55.1134062492798,-202.84995));
#202458=CARTESIAN_POINT('',(-62.6674432759983,-55.1294305058671,-179.606318983907));
#202459=CARTESIAN_POINT('',(-62.2620407574844,29.1784062092233,-202.84995));
#202460=CARTESIAN_POINT('Origin',(1004.,-12.967500020028,-202.84995));
#202461=CARTESIAN_POINT('',(-62.6674432759984,29.1944304658105,-179.606318983907));
#202462=CARTESIAN_POINT('Origin',(-50.7133971693864,28.7219255026673,-179.606318983907));
#202463=CARTESIAN_POINT('',(-59.9543671306402,36.3185518471891,-179.64995));
#202464=CARTESIAN_POINT('Origin',(-50.7133971693864,28.7219255026673,-179.64995));
#202465=CARTESIAN_POINT('',(-59.6415426483635,36.0613915368278,-202.84995));
#202466=CARTESIAN_POINT('Origin',(-50.7133971693864,28.7219255026674,-202.84995));
#202467=CARTESIAN_POINT('',(-59.9549554431411,36.3190354750184,-179.606318983907));
#202468=CARTESIAN_POINT('Origin',(0.,-12.9675000200281,-179.606318983907));
#202469=CARTESIAN_POINT('',(-48.8412921507357,47.3497382103492,-179.64995));
#202470=CARTESIAN_POINT('Origin',(0.,-12.9675000200281,-179.64995));
#202471=CARTESIAN_POINT('',(-48.5864524674565,47.0350203720195,-202.84995));
#202472=CARTESIAN_POINT('Origin',(0.,-12.9675000200281,-202.84995));
#202473=CARTESIAN_POINT('',(-48.8417714142841,47.3503300835849,-179.606318983907));
#202474=CARTESIAN_POINT('Origin',(-41.3132181298675,38.0528376956935,-179.606318983907));
#202475=CARTESIAN_POINT('',(-43.5541767698386,49.8036828575113,-179.64995));
#202476=CARTESIAN_POINT('Origin',(-41.3132181298675,38.0528376956935,-179.64995));
#202477=CARTESIAN_POINT('',(-43.478316039927,49.4058943061501,-202.84995));
#202478=CARTESIAN_POINT('Origin',(-41.3132181298675,38.0528376956935,-202.84995));
#202479=CARTESIAN_POINT('',(-43.5543194371113,49.8044309574546,-179.606318983907));
#202480=CARTESIAN_POINT('Origin',(-41.5452362233251,-63.7990866568863,-179.606318983907));
#202481=CARTESIAN_POINT('',(-49.1155884655664,-73.0615930440079,-179.64995));
#202482=CARTESIAN_POINT('',(-42.0160769799045,-75.7524362554308,-179.64995));
#202483=CARTESIAN_POINT('Origin',(-41.5452362233251,-63.7990866568863,-179.64995));
#202484=CARTESIAN_POINT('',(-42.0001381210477,-75.3477925421285,-202.84995));
#202485=CARTESIAN_POINT('',(-42.0161069552755,-75.7531972475156,-179.606318983907));
#202486=CARTESIAN_POINT('',(-48.8593175837476,-72.7480395125837,-202.84995));
#202487=CARTESIAN_POINT('Origin',(-41.5452362233251,-63.7990866568863,-202.84995));
#202488=CARTESIAN_POINT('',(-49.1160704206943,-73.0621827275931,-179.606318983907));
#202489=CARTESIAN_POINT('Origin',(0.,-12.9675000200281,-179.606318983907));
#202490=CARTESIAN_POINT('',(-59.9543671306402,-62.2535518872453,-179.64995));
#202491=CARTESIAN_POINT('Origin',(0.,-12.9675000200281,-179.64995));
#202492=CARTESIAN_POINT('',(-59.6415426483635,-61.9963915768841,-202.84995));
#202493=CARTESIAN_POINT('Origin',(0.,-12.9675000200281,-202.84995));
#202494=CARTESIAN_POINT('',(-59.9549554431411,-62.2540355150746,-179.606318983907));
#202495=CARTESIAN_POINT('Origin',(-50.7133971693864,-54.6569255427236,-179.606318983907));
#202496=CARTESIAN_POINT('Origin',(-50.7133971693864,-54.6569255427236,-179.64995));
#202497=CARTESIAN_POINT('Origin',(-50.7133971693864,-54.6569255427236,-202.84995));
#202498=CARTESIAN_POINT('Ctrl Pts',(-47.7724784290048,-32.4865586987341,
-232.970973990925));
#202499=CARTESIAN_POINT('Ctrl Pts',(-51.8616631458841,-35.9897429718971,
-226.798709657862));
#202500=CARTESIAN_POINT('Ctrl Pts',(-55.9509791745034,-39.4923578424338,
-220.626231304292));
#202501=CARTESIAN_POINT('Ctrl Pts',(-60.0403077603802,-42.9948148700989,
-214.453693714461));
#202502=CARTESIAN_POINT('Ctrl Pts',(-47.6970999179399,-35.0937046824551,
-232.967721023846));
#202503=CARTESIAN_POINT('Ctrl Pts',(-51.7757137841176,-39.0045377390498,
-226.795568831742));
#202504=CARTESIAN_POINT('Ctrl Pts',(-55.8544675412487,-42.9147019697459,
-220.623140932772));
#202505=CARTESIAN_POINT('Ctrl Pts',(-59.9332050840609,-46.8246892042479,
-214.450640245293));
#202506=CARTESIAN_POINT('Ctrl Pts',(-47.6083941910801,-37.6707809958978,
-232.96396511673));
#202507=CARTESIAN_POINT('Ctrl Pts',(-51.6738491177805,-42.0114382175837,
-226.791891649754));
#202508=CARTESIAN_POINT('Ctrl Pts',(-55.7393519427245,-46.3514436774691,
-220.61950573142));
#202509=CARTESIAN_POINT('Ctrl Pts',(-59.8047170999058,-50.6912943906935,
-214.447047813144));
#202510=CARTESIAN_POINT('Ctrl Pts',(-47.5079779560868,-40.2034134198457,
-232.959831751742));
#202511=CARTESIAN_POINT('Ctrl Pts',(-51.5558271984379,-45.0119998619165,
-226.787659137649));
#202512=CARTESIAN_POINT('Ctrl Pts',(-55.603839292235,-49.8201780781628,
-220.615275392699));
#202513=CARTESIAN_POINT('Ctrl Pts',(-59.6518858770376,-54.6282695245469,
-214.442846690034));
#202514=CARTESIAN_POINT('',(-47.8511644985019,-32.6020541825732,-232.850071652982));
#202515=CARTESIAN_POINT('Ctrl Pts',(-47.8511937435036,-32.6021335774055,
-232.85005));
#202516=CARTESIAN_POINT('Ctrl Pts',(-47.8129987256184,-33.8832172184026,
-232.85005));
#202517=CARTESIAN_POINT('Ctrl Pts',(-47.7712743196189,-35.1649732916811,
-232.850050000001));
#202518=CARTESIAN_POINT('Ctrl Pts',(-47.6808913011582,-37.7267114902632,
-232.850050000001));
#202519=CARTESIAN_POINT('Ctrl Pts',(-47.632174582744,-39.0083318774293,
-232.85005));
#202520=CARTESIAN_POINT('Ctrl Pts',(-47.5799752941153,-40.2889415902927,
-232.85005));
#202521=CARTESIAN_POINT('',(-59.8539584057532,-46.7516625814213,-214.560265665659));
#202522=CARTESIAN_POINT('Ctrl Pts',(-47.8511937435036,-32.6021335774055,
-232.85005));
#202523=CARTESIAN_POINT('Ctrl Pts',(-49.7758731964884,-34.8662384268529,
-229.917938361341));
#202524=CARTESIAN_POINT('Ctrl Pts',(-52.006472582506,-37.4944438055142,
-226.519199319976));
#202525=CARTESIAN_POINT('Ctrl Pts',(-55.7540093824077,-41.913096923482,
-220.808621189981));
#202526=CARTESIAN_POINT('Ctrl Pts',(-57.9042257962353,-44.4502782877339,
-217.531776051457));
#202527=CARTESIAN_POINT('Ctrl Pts',(-59.8539550780142,-46.7516786354062,
-214.560279194377));
#202528=CARTESIAN_POINT('Ctrl Pts',(-59.8539609358732,-46.7516610380903,
-214.560271423235));
#202529=CARTESIAN_POINT('Ctrl Pts',(-59.8127437126638,-48.0499861504054,
-214.559533037022));
#202530=CARTESIAN_POINT('Ctrl Pts',(-59.769150621426,-49.34823472919,-214.558748583908));
#202531=CARTESIAN_POINT('Ctrl Pts',(-59.6772124392589,-51.9445894630669,
-214.557078958964));
#202532=CARTESIAN_POINT('Ctrl Pts',(-59.6288676637842,-53.242684640561,
-214.556193992093));
#202533=CARTESIAN_POINT('Ctrl Pts',(-59.5781472511379,-54.5406860123126,
-214.555282751789));
#202534=CARTESIAN_POINT('Ctrl Pts',(-47.5077687575999,17.0588630313157,
-232.959797430566));
#202535=CARTESIAN_POINT('Ctrl Pts',(-51.5543587613359,20.962467251341,-226.789554159174));
#202536=CARTESIAN_POINT('Ctrl Pts',(-55.6010831372117,24.8656613676635,
-220.619139657106));
#202537=CARTESIAN_POINT('Ctrl Pts',(-59.6478359854379,28.7687682426261,
-214.448688656128));
#202538=CARTESIAN_POINT('Ctrl Pts',(-47.6093150514154,14.5106669763354,
-232.963237198889));
#202539=CARTESIAN_POINT('Ctrl Pts',(-51.673625611954,17.943733161272,-226.793068881834));
#202540=CARTESIAN_POINT('Ctrl Pts',(-55.7379386239558,21.3761434795959,
-220.622650915033));
#202541=CARTESIAN_POINT('Ctrl Pts',(-59.8021028749556,24.8083979649139,
-214.45217527183));
#202542=CARTESIAN_POINT('Ctrl Pts',(-47.6990097155228,11.9175493678758,
-232.966275794525));
#202543=CARTESIAN_POINT('Ctrl Pts',(-51.7765308861555,14.9186157818217,
-226.796020622489));
#202544=CARTESIAN_POINT('Ctrl Pts',(-55.8541462985605,17.9190127102163,
-220.625556640966));
#202545=CARTESIAN_POINT('Ctrl Pts',(-59.9317344440901,20.9192322601435,
-214.455037317351));
#202546=CARTESIAN_POINT('Ctrl Pts',(-47.7752156818158,9.29411691894321,
-232.968782926844));
#202547=CARTESIAN_POINT('Ctrl Pts',(-51.8633248967382,11.8855265874929,
-226.79842796189));
#202548=CARTESIAN_POINT('Ctrl Pts',(-55.9515262957967,14.4763668580276,
-220.627916411389));
#202549=CARTESIAN_POINT('Ctrl Pts',(-60.0397300597283,17.0670490879089,
-214.457361414306));
#202550=CARTESIAN_POINT('',(-59.8522817919913,20.8670659745804,-214.56462304469));
#202551=CARTESIAN_POINT('Ctrl Pts',(-59.5744430045609,28.6979747791781,
-214.56059791914));
#202552=CARTESIAN_POINT('Ctrl Pts',(-59.6255523742397,27.3929948773216,
-214.561350802779));
#202553=CARTESIAN_POINT('Ctrl Pts',(-59.6742602842767,26.0879255239807,
-214.562076913704));
#202554=CARTESIAN_POINT('Ctrl Pts',(-59.7668739992229,23.4776071864522,
-214.563426526416));
#202555=CARTESIAN_POINT('Ctrl Pts',(-59.8107792490354,22.1723754160636,
-214.56404982166));
#202556=CARTESIAN_POINT('Ctrl Pts',(-59.8522830098483,20.8670660146469,
-214.564626087537));
#202557=CARTESIAN_POINT('',(-47.8524647801522,9.39110652846791,-232.850060330937));
#202558=CARTESIAN_POINT('Ctrl Pts',(-59.8522792844971,20.8670810655101,
-214.564630881667));
#202559=CARTESIAN_POINT('Ctrl Pts',(-57.9231698177518,19.0197028269434,
-217.504721577749));
#202560=CARTESIAN_POINT('Ctrl Pts',(-55.7588762173457,16.9478029332325,
-220.803047120975));
#202561=CARTESIAN_POINT('Ctrl Pts',(-52.0105370781302,13.362350606817,-226.514897697653));
#202562=CARTESIAN_POINT('Ctrl Pts',(-49.7764856318141,11.2269580602607,
-229.918931539958));
#202563=CARTESIAN_POINT('Ctrl Pts',(-47.8524795676142,9.39114590592674,
-232.85005));
#202564=CARTESIAN_POINT('Ctrl Pts',(-47.5797436947461,17.1282946781069,
-232.85005));
#202565=CARTESIAN_POINT('Ctrl Pts',(-47.6322830986109,15.839317171622,-232.85005));
#202566=CARTESIAN_POINT('Ctrl Pts',(-47.6812964150147,14.5493107491118,
-232.850050000002));
#202567=CARTESIAN_POINT('Ctrl Pts',(-47.7721850391671,11.9708027192453,
-232.850050000002));
#202568=CARTESIAN_POINT('Ctrl Pts',(-47.8141193819828,10.6806307165552,
-232.85005));
#202569=CARTESIAN_POINT('Ctrl Pts',(-47.8524795676142,9.39114590592674,
-232.85005));
#202570=CARTESIAN_POINT('Origin',(1004.,-12.967500020028,-205.306318983907));
#202571=CARTESIAN_POINT('Ctrl Pts',(-59.852283684575,20.8670529899755,-214.564611171477));
#202572=CARTESIAN_POINT('Ctrl Pts',(-59.9408921983977,18.6616086582029,
-213.507172831477));
#202573=CARTESIAN_POINT('Ctrl Pts',(-60.0187430617361,16.1586269377748,
-213.171736592191));
#202574=CARTESIAN_POINT('Ctrl Pts',(-60.0783440471533,13.709584889334,-213.274710076528));
#202575=CARTESIAN_POINT('Ctrl Pts',(-60.0869371638556,13.3564883090716,
-213.289556528511));
#202576=CARTESIAN_POINT('Ctrl Pts',(-60.0951902283565,13.0034719450298,
-213.313678069836));
#202577=CARTESIAN_POINT('Ctrl Pts',(-60.1030981576493,12.6512459219475,
-213.346442200715));
#202578=CARTESIAN_POINT('Ctrl Pts',(-60.1182284170081,11.9773310594209,
-213.409129887912));
#202579=CARTESIAN_POINT('Ctrl Pts',(-60.1324253703542,11.283793184265,-213.510071155534));
#202580=CARTESIAN_POINT('Ctrl Pts',(-60.1429164546448,10.7356826748675,
-213.608457606495));
#202581=CARTESIAN_POINT('Ctrl Pts',(-60.1466440184685,10.5409347489484,
-213.643415077543));
#202582=CARTESIAN_POINT('Ctrl Pts',(-60.1500513021095,10.3579630053009,
-213.678691006502));
#202583=CARTESIAN_POINT('Ctrl Pts',(-60.1532641850396,10.1814317298332,
-213.714618736487));
#202584=CARTESIAN_POINT('Ctrl Pts',(-60.1571763074451,9.96648086699788,
-213.758365639348));
#202585=CARTESIAN_POINT('Ctrl Pts',(-60.1608006466485,9.76108925215573,
-213.803062347838));
#202586=CARTESIAN_POINT('Ctrl Pts',(-60.1643187438617,9.55589232998761,
-213.850313921784));
#202587=CARTESIAN_POINT('Ctrl Pts',(-60.1647663228057,9.52978679163152,
-213.856325355888));
#202588=CARTESIAN_POINT('Ctrl Pts',(-60.1652121278246,9.50368446580759,
-213.862379491625));
#202589=CARTESIAN_POINT('Ctrl Pts',(-60.1656564875316,9.47756602057091,
-213.868480820893));
#202590=CARTESIAN_POINT('Ctrl Pts',(-60.1660491443594,9.4544865520864,-213.873872238157));
#202591=CARTESIAN_POINT('Ctrl Pts',(-60.1664410470052,9.43139075002581,
-213.879283604594));
#202592=CARTESIAN_POINT('Ctrl Pts',(-60.1668339732077,9.40824978917481,
-213.884647521255));
#202593=CARTESIAN_POINT('Ctrl Pts',(-60.1675888932482,9.36378959540123,
-213.894953090485));
#202594=CARTESIAN_POINT('Ctrl Pts',(-60.1683459618837,9.3191789651964,-213.905157368098));
#202595=CARTESIAN_POINT('Ctrl Pts',(-60.1691067978077,9.27432300489259,
-213.91527730166));
#202596=CARTESIAN_POINT('Ctrl Pts',(-60.1705954940517,9.1865551990907,-213.935078557894));
#202597=CARTESIAN_POINT('Ctrl Pts',(-60.1720986097152,9.09784859398886,
-213.954559217709));
#202598=CARTESIAN_POINT('Ctrl Pts',(-60.1736282672258,9.00748926176064,
-213.973818634937));
#202599=CARTESIAN_POINT('Ctrl Pts',(-60.1792151276392,8.67746442109373,
-214.044160966443));
#202600=CARTESIAN_POINT('Ctrl Pts',(-60.1853553620157,8.31350519984393,
-214.113465883351));
#202601=CARTESIAN_POINT('Ctrl Pts',(-60.1914134093591,7.95361934628412,
-214.171719071268));
#202602=CARTESIAN_POINT('Ctrl Pts',(-60.2137472534458,6.62684950003347,
-214.386477646555));
#202603=CARTESIAN_POINT('Ctrl Pts',(-60.236418104203,5.27038456544881,-214.469588956065));
#202604=CARTESIAN_POINT('Ctrl Pts',(-60.2591685013589,3.93463693001197,
-214.381568911362));
#202605=CARTESIAN_POINT('Ctrl Pts',(-60.270567951341,3.26533923579523,-214.337465061652));
#202606=CARTESIAN_POINT('Ctrl Pts',(-60.2826202444475,2.56566381511999,
-214.241040503758));
#202607=CARTESIAN_POINT('Ctrl Pts',(-60.292057365503,2.02427812018546,-214.137294054647));
#202608=CARTESIAN_POINT('Ctrl Pts',(-60.2979421316394,1.68668276821483,
-214.072600215613));
#202609=CARTESIAN_POINT('Ctrl Pts',(-60.3031851011954,1.38822157870232,
-214.004609259433));
#202610=CARTESIAN_POINT('Ctrl Pts',(-60.3084747241416,1.08920916466888,
-213.927821213477));
#202611=CARTESIAN_POINT('Ctrl Pts',(-60.3091581982913,1.05057365935602,
-213.917899401477));
#202612=CARTESIAN_POINT('Ctrl Pts',(-60.3098424352801,1.01193290476609,
-213.907817486517));
#202613=CARTESIAN_POINT('Ctrl Pts',(-60.3105289330055,0.973203341285052,
-213.897551739282));
#202614=CARTESIAN_POINT('Ctrl Pts',(-60.3112345718811,0.933393907674668,
-213.886999759185));
#202615=CARTESIAN_POINT('Ctrl Pts',(-60.3119438877354,0.893513565114719,
-213.87616273221));
#202616=CARTESIAN_POINT('Ctrl Pts',(-60.3126540303503,0.853391001986712,
-213.865328893283));
#202617=CARTESIAN_POINT('Ctrl Pts',(-60.3142387111128,0.763857642627992,
-213.841153219592));
#202618=CARTESIAN_POINT('Ctrl Pts',(-60.3158218668931,0.673014957611186,
-213.817396808284));
#202619=CARTESIAN_POINT('Ctrl Pts',(-60.3174186631854,0.579830242826638,
-213.793870865919));
#202620=CARTESIAN_POINT('Ctrl Pts',(-60.3203923825932,0.406292017450701,
-213.750058419878));
#202621=CARTESIAN_POINT('Ctrl Pts',(-60.3234151563687,0.224650876049034,
-213.706988287318));
#202622=CARTESIAN_POINT('Ctrl Pts',(-60.3265631280972,0.0280980835395926,
-213.664136837394));
#202623=CARTESIAN_POINT('Ctrl Pts',(-60.3339383732068,-0.432396846778452,
-213.563742051876));
#202624=CARTESIAN_POINT('Ctrl Pts',(-60.3416644856382,-0.959964067856175,
-213.470756377755));
#202625=CARTESIAN_POINT('Ctrl Pts',(-60.3482721133978,-1.46527456786017,
-213.40505861675));
#202626=CARTESIAN_POINT('Ctrl Pts',(-60.3615553279344,-2.48109265317286,
-213.272987397582));
#202627=CARTESIAN_POINT('Ctrl Pts',(-60.3719858564929,-3.50919761377231,
-213.2277198046));
#202628=CARTESIAN_POINT('Ctrl Pts',(-60.3794425164094,-4.53314772643593,
-213.26537659776));
#202629=CARTESIAN_POINT('Ctrl Pts',(-60.3850857563185,-5.30807862114162,
-213.293875459232));
#202630=CARTESIAN_POINT('Ctrl Pts',(-60.389031621255,-6.08056089768348,
-213.369825212479));
#202631=CARTESIAN_POINT('Ctrl Pts',(-60.3913108160445,-6.84593414020724,
-213.491429597462));
#202632=CARTESIAN_POINT('Ctrl Pts',(-60.3924832204613,-7.23963764205741,
-213.553982179063));
#202633=CARTESIAN_POINT('Ctrl Pts',(-60.393210861424,-7.65045599543644,
-213.633390155679));
#202634=CARTESIAN_POINT('Ctrl Pts',(-60.3934920217241,-7.99285084597502,
-213.708959851915));
#202635=CARTESIAN_POINT('Ctrl Pts',(-60.3936603081493,-8.19778875984029,
-213.754191536544));
#202636=CARTESIAN_POINT('Ctrl Pts',(-60.3936984229566,-8.3833292016282,
-213.798440546674));
#202637=CARTESIAN_POINT('Ctrl Pts',(-60.3936519031611,-8.56176805395006,
-213.843419246262));
#202638=CARTESIAN_POINT('Ctrl Pts',(-60.3936457152461,-8.58550342183554,
-213.849402169644));
#202639=CARTESIAN_POINT('Ctrl Pts',(-60.3936379471922,-8.60911262131742,
-213.855400254366));
#202640=CARTESIAN_POINT('Ctrl Pts',(-60.3936286330974,-8.63262423355809,
-213.86141955001));
#202641=CARTESIAN_POINT('Ctrl Pts',(-60.3936240106306,-8.64429274776344,
-213.864406849902));
#202642=CARTESIAN_POINT('Ctrl Pts',(-60.3936189488047,-8.65593645131671,
-213.867402543179));
#202643=CARTESIAN_POINT('Ctrl Pts',(-60.3936136334464,-8.66756126923334,
-213.870397484014));
#202644=CARTESIAN_POINT('Ctrl Pts',(-60.3936089954616,-8.67770465498888,
-213.873010758511));
#202645=CARTESIAN_POINT('Ctrl Pts',(-60.3936043793879,-8.68783651798293,
-213.875611805623));
#202646=CARTESIAN_POINT('Ctrl Pts',(-60.3935997841399,-8.69795915571533,
-213.878201268307));
#202647=CARTESIAN_POINT('Ctrl Pts',(-60.3935813536365,-8.73855877228209,
-213.888587019024));
#202648=CARTESIAN_POINT('Ctrl Pts',(-60.3935632575531,-8.77901001068333,
-213.898786760883));
#202649=CARTESIAN_POINT('Ctrl Pts',(-60.3935454305536,-8.81946085570323,
-213.9088392194));
#202650=CARTESIAN_POINT('Ctrl Pts',(-60.3935099629075,-8.89993969675822,
-213.928839054034));
#202651=CARTESIAN_POINT('Ctrl Pts',(-60.3934755529649,-8.9804162770879,
-213.948259982409));
#202652=CARTESIAN_POINT('Ctrl Pts',(-60.3934417749187,-9.06205842258958,
-213.967356720238));
#202653=CARTESIAN_POINT('Ctrl Pts',(-60.3932972840641,-9.41129541870198,
-214.049045991312));
#202654=CARTESIAN_POINT('Ctrl Pts',(-60.3931553384559,-9.79419688676307,
-214.129239831576));
#202655=CARTESIAN_POINT('Ctrl Pts',(-60.3930255323827,-10.2663428839057,
-214.205320185781));
#202656=CARTESIAN_POINT('Ctrl Pts',(-60.3927844696473,-11.1431647675559,
-214.346608939443));
#202657=CARTESIAN_POINT('Ctrl Pts',(-60.3926875276504,-12.0266701068567,
-214.418412123761));
#202658=CARTESIAN_POINT('Ctrl Pts',(-60.3927142613204,-12.9140676164264,
-214.419432663803));
#202659=CARTESIAN_POINT('Ctrl Pts',(-60.392740601048,-13.7883885989459,
-214.420438165354));
#202660=CARTESIAN_POINT('Ctrl Pts',(-60.392886297565,-14.6625510241356,
-214.352549769935));
#202661=CARTESIAN_POINT('Ctrl Pts',(-60.3930924113226,-15.5293465961958,
-214.221220332185));
#202662=CARTESIAN_POINT('Ctrl Pts',(-60.3931958927294,-15.9645297022867,
-214.155285116912));
#202663=CARTESIAN_POINT('Ctrl Pts',(-60.3933106563195,-16.3866140396118,
-214.073965655162));
#202664=CARTESIAN_POINT('Ctrl Pts',(-60.3934060177548,-16.7332476949765,
-213.998244468936));
#202665=CARTESIAN_POINT('Ctrl Pts',(-60.3934150872653,-16.7662148746455,
-213.991042877537));
#202666=CARTESIAN_POINT('Ctrl Pts',(-60.3934240727474,-16.7988175394096,
-213.983832359438));
#202667=CARTESIAN_POINT('Ctrl Pts',(-60.393432985145,-16.8311197866803,
-213.976604381314));
#202668=CARTESIAN_POINT('Ctrl Pts',(-60.3934565432233,-16.9165040912771,
-213.95749871722));
#202669=CARTESIAN_POINT('Ctrl Pts',(-60.3934796365262,-16.9997898733479,
-213.938272995079));
#202670=CARTESIAN_POINT('Ctrl Pts',(-60.3935024947112,-17.0821483260315,
-213.918723916564));
#202671=CARTESIAN_POINT('Ctrl Pts',(-60.3935141968302,-17.1243112718211,
-213.908715875971));
#202672=CARTESIAN_POINT('Ctrl Pts',(-60.3935258376587,-17.1662309100974,
-213.898622064381));
#202673=CARTESIAN_POINT('Ctrl Pts',(-60.3935374491214,-17.2080633558844,
-213.888408909728));
#202674=CARTESIAN_POINT('Ctrl Pts',(-60.3935432880669,-17.2290992392795,
-213.883273117969));
#202675=CARTESIAN_POINT('Ctrl Pts',(-60.393549119591,-17.2501130687726,
-213.878107082029));
#202676=CARTESIAN_POINT('Ctrl Pts',(-60.393554947749,-17.2711246845471,
-213.872906131118));
#202677=CARTESIAN_POINT('Ctrl Pts',(-60.3935615224738,-17.294827815679,
-213.867038956371));
#202678=CARTESIAN_POINT('Ctrl Pts',(-60.3935675567514,-17.3185350501926,
-213.861156493035));
#202679=CARTESIAN_POINT('Ctrl Pts',(-60.3935716543076,-17.3422928483403,
-213.855327567938));
#202680=CARTESIAN_POINT('Ctrl Pts',(-60.3936041243251,-17.5305553343483,
-213.809137768578));
#202681=CARTESIAN_POINT('Ctrl Pts',(-60.3935458845432,-17.7216373314316,
-213.764774682049));
#202682=CARTESIAN_POINT('Ctrl Pts',(-60.3933602461435,-17.9298338823286,
-213.719802565618));
#202683=CARTESIAN_POINT('Ctrl Pts',(-60.39306103192,-18.2654076075664,-213.647315963041));
#202684=CARTESIAN_POINT('Ctrl Pts',(-60.3923553391732,-18.6775129550165,
-213.567607646049));
#202685=CARTESIAN_POINT('Ctrl Pts',(-60.3910564967462,-19.1075296034981,
-213.499906653704));
#202686=CARTESIAN_POINT('Ctrl Pts',(-60.3887092138914,-19.8846605974918,
-213.377556647813));
#202687=CARTESIAN_POINT('Ctrl Pts',(-60.3846983903846,-20.669134581579,
-213.299096394904));
#202688=CARTESIAN_POINT('Ctrl Pts',(-60.3789612071656,-21.4554845530463,
-213.268525469849));
#202689=CARTESIAN_POINT('Ctrl Pts',(-60.3679012957513,-22.971378449573,
-213.209592068205));
#202690=CARTESIAN_POINT('Ctrl Pts',(-60.3502984944823,-24.5000103406804,
-213.329130293887));
#202691=CARTESIAN_POINT('Ctrl Pts',(-60.3264857554363,-25.9796130521886,
-213.6570101885));
#202692=CARTESIAN_POINT('Ctrl Pts',(-60.3234504544024,-26.1682112487739,
-213.698803540418));
#202693=CARTESIAN_POINT('Ctrl Pts',(-60.32045653301,-26.3472746066239,-213.742037759623));
#202694=CARTESIAN_POINT('Ctrl Pts',(-60.3175367315418,-26.516649532719,
-213.78578065973));
#202695=CARTESIAN_POINT('Ctrl Pts',(-60.3159762978469,-26.6071688178869,
-213.809158240699));
#202696=CARTESIAN_POINT('Ctrl Pts',(-60.3144291687252,-26.6953838659087,
-213.832796220737));
#202697=CARTESIAN_POINT('Ctrl Pts',(-60.3128853379364,-26.7820351410227,
-213.856805411057));
#202698=CARTESIAN_POINT('Ctrl Pts',(-60.3124915944156,-26.8041349581721,
-213.862928791414));
#202699=CARTESIAN_POINT('Ctrl Pts',(-60.3120980566698,-26.8261330430226,
-213.86907659917));
#202700=CARTESIAN_POINT('Ctrl Pts',(-60.3117045402841,-26.8480416873385,
-213.875251256029));
#202701=CARTESIAN_POINT('Ctrl Pts',(-60.3115355397114,-26.857450630824,
-213.877903040255));
#202702=CARTESIAN_POINT('Ctrl Pts',(-60.3113666893836,-26.8668457943141,
-213.880549365385));
#202703=CARTESIAN_POINT('Ctrl Pts',(-60.311198146228,-26.8762313719384,
-213.883178158384));
#202704=CARTESIAN_POINT('Ctrl Pts',(-60.3110325273771,-26.8854541052786,
-213.88576134056));
#202705=CARTESIAN_POINT('Ctrl Pts',(-60.3108671528631,-26.8946666125183,
-213.888331312463));
#202706=CARTESIAN_POINT('Ctrl Pts',(-60.3107020058,-26.9038697912027,-213.890888412478));
#202707=CARTESIAN_POINT('Ctrl Pts',(-60.31003714784,-26.940920444689,-213.901182923738));
#202708=CARTESIAN_POINT('Ctrl Pts',(-60.3093759742382,-26.9778199604899,
-213.911268999765));
#202709=CARTESIAN_POINT('Ctrl Pts',(-60.3087174003261,-27.0146264313552,
-213.921167211129));
#202710=CARTESIAN_POINT('Ctrl Pts',(-60.3034328975208,-27.3099674628737,
-214.000592048282));
#202711=CARTESIAN_POINT('Ctrl Pts',(-60.2983146403094,-27.5991766863594,
-214.068573069903));
#202712=CARTESIAN_POINT('Ctrl Pts',(-60.2928256973099,-27.9124538529064,
-214.131004935625));
#202713=CARTESIAN_POINT('Ctrl Pts',(-60.2839179962429,-28.4208539858519,
-214.23232214678));
#202714=CARTESIAN_POINT('Ctrl Pts',(-60.2740350908591,-28.9922802878427,
-214.323849549146));
#202715=CARTESIAN_POINT('Ctrl Pts',(-60.2607587673068,-29.7735994708971,
-214.377595134823));
#202716=CARTESIAN_POINT('Ctrl Pts',(-60.2515599690423,-30.3149539744131,
-214.414833968173));
#202717=CARTESIAN_POINT('Ctrl Pts',(-60.2410136149577,-30.9417409026654,
-214.424736435113));
#202718=CARTESIAN_POINT('Ctrl Pts',(-60.2310558010096,-31.5353290509064,
-214.401902737164));
#202719=CARTESIAN_POINT('Ctrl Pts',(-60.2183577806209,-32.2922616917676,
-214.372785627362));
#202720=CARTESIAN_POINT('Ctrl Pts',(-60.2057261525619,-33.0473025715524,
-214.295280550927));
#202721=CARTESIAN_POINT('Ctrl Pts',(-60.1931159963307,-33.7953694742733,
-214.178967256063));
#202722=CARTESIAN_POINT('Ctrl Pts',(-60.1870407676876,-34.1557676637223,
-214.122930689379));
#202723=CARTESIAN_POINT('Ctrl Pts',(-60.1809699443646,-34.5145264949527,
-214.05797839233));
#202724=CARTESIAN_POINT('Ctrl Pts',(-60.1749016871998,-34.8710225250701,
-213.985271624848));
#202725=CARTESIAN_POINT('Ctrl Pts',(-60.1733510559208,-34.9621185152596,
-213.966692750421));
#202726=CARTESIAN_POINT('Ctrl Pts',(-60.1718496862813,-35.050193464265,
-213.948229706888));
#202727=CARTESIAN_POINT('Ctrl Pts',(-60.1702373704645,-35.1446172308779,
-213.927869919498));
#202728=CARTESIAN_POINT('Ctrl Pts',(-60.1694999096097,-35.1878059355493,
-213.918557509326));
#202729=CARTESIAN_POINT('Ctrl Pts',(-60.1687161169393,-35.23367491272,-213.908549231462));
#202730=CARTESIAN_POINT('Ctrl Pts',(-60.1678875012017,-35.2821213266033,
-213.897823414987));
#202731=CARTESIAN_POINT('Ctrl Pts',(-60.1675039091746,-35.3045486801587,
-213.892858100551));
#202732=CARTESIAN_POINT('Ctrl Pts',(-60.1671107108273,-35.3275283964073,
-213.887738985336));
#202733=CARTESIAN_POINT('Ctrl Pts',(-60.1667080521216,-35.3510503623432,
-213.882463780837));
#202734=CARTESIAN_POINT('Ctrl Pts',(-60.1665110501776,-35.3625585526502,
-213.879882871679));
#202735=CARTESIAN_POINT('Ctrl Pts',(-60.1663118308306,-35.3741960784184,
-213.877262456814));
#202736=CARTESIAN_POINT('Ctrl Pts',(-60.1661102633079,-35.385963215018,
-213.874608964427));
#202737=CARTESIAN_POINT('Ctrl Pts',(-60.1658814425207,-35.399321346446,
-213.871596702288));
#202738=CARTESIAN_POINT('Ctrl Pts',(-60.1656492765433,-35.4128496429709,
-213.868556305922));
#202739=CARTESIAN_POINT('Ctrl Pts',(-60.1654137561779,-35.4265466933703,
-213.865488895693));
#202740=CARTESIAN_POINT('Ctrl Pts',(-60.1622181589691,-35.6123915818273,
-213.82386953276));
#202741=CARTESIAN_POINT('Ctrl Pts',(-60.158406128703,-35.8293021918329,
-213.777246558444));
#202742=CARTESIAN_POINT('Ctrl Pts',(-60.1539472537289,-36.0737459393782,
-213.728630617293));
#202743=CARTESIAN_POINT('Ctrl Pts',(-60.1418239904498,-36.7383655857192,
-213.596448428388));
#202744=CARTESIAN_POINT('Ctrl Pts',(-60.1249235460772,-37.6062744383648,
-213.448897620045));
#202745=CARTESIAN_POINT('Ctrl Pts',(-60.1024025775609,-38.6088068260868,
-213.355157950907));
#202746=CARTESIAN_POINT('Ctrl Pts',(-60.0769094959091,-39.7436443442948,
-213.249047370555));
#202747=CARTESIAN_POINT('Ctrl Pts',(-60.0435573435545,-41.0613446239085,
-213.221088955402));
#202748=CARTESIAN_POINT('Ctrl Pts',(-60.0067973884015,-42.3155600514751,
-213.345100282712));
#202749=CARTESIAN_POINT('Ctrl Pts',(-59.9618223482237,-43.8500665276586,
-213.496825561076));
#202750=CARTESIAN_POINT('Ctrl Pts',(-59.9097381130811,-45.3772288239093,
-213.865683397748));
#202751=CARTESIAN_POINT('Ctrl Pts',(-59.8539617334923,-46.7516465274364,
-214.56025213694));
#202752=CARTESIAN_POINT('Origin',(1004.,-12.967500020028,-202.84995));
#202753=CARTESIAN_POINT('Ctrl Pts',(-21.8343359993853,37.3653585113446,
-232.959639066595));
#202754=CARTESIAN_POINT('Ctrl Pts',(-25.7068670980457,41.0171742382378,
-226.784363424386));
#202755=CARTESIAN_POINT('Ctrl Pts',(-29.5908265861273,44.7050007481411,
-220.612769983421));
#202756=CARTESIAN_POINT('Ctrl Pts',(-33.4823003440903,48.4301227180298,
-214.442258946369));
#202757=CARTESIAN_POINT('Ctrl Pts',(-23.8044899907809,37.1610589494743,
-232.959868581815));
#202758=CARTESIAN_POINT('Ctrl Pts',(-28.0381839166385,40.7424490125755,
-226.783608200302));
#202759=CARTESIAN_POINT('Ctrl Pts',(-32.283433258083,44.3482400615009,-220.611766381486));
#202760=CARTESIAN_POINT('Ctrl Pts',(-36.5352279127207,47.9802021638173,
-214.441141334719));
#202761=CARTESIAN_POINT('Ctrl Pts',(-25.7658626658342,36.9296719371149,
-232.9601933409));
#202762=CARTESIAN_POINT('Ctrl Pts',(-30.3639150200345,40.4303260414807,
-226.78272680046));
#202763=CARTESIAN_POINT('Ctrl Pts',(-34.9732667504195,43.9421267939794,
-220.610591760459));
#202764=CARTESIAN_POINT('Ctrl Pts',(-39.587510189865,47.4674439422847,-214.439830103812));
#202765=CARTESIAN_POINT('Ctrl Pts',(-27.7161624394018,36.671894066742,-232.960596901862));
#202766=CARTESIAN_POINT('Ctrl Pts',(-32.6826602701726,40.0809702013776,
-226.781662197074));
#202767=CARTESIAN_POINT('Ctrl Pts',(-37.6596812128995,43.4862512150987,
-220.609204852275));
#202768=CARTESIAN_POINT('Ctrl Pts',(-42.6390550299281,46.8908628802244,
-214.438294417841));
#202769=CARTESIAN_POINT('',(-23.9219380212091,37.2105892288189,-232.850059426121));
#202770=CARTESIAN_POINT('Origin',(-0.0818455390431216,-172.606491708452,
-232.85022953235));
#202771=CARTESIAN_POINT('',(-33.4675962034302,48.3558337693674,-214.551986533665));
#202772=CARTESIAN_POINT('Ctrl Pts',(-23.9219380212091,37.2105892288189,
-232.850059426121));
#202773=CARTESIAN_POINT('Ctrl Pts',(-24.1894337590953,37.5543763047846,
-232.280636433357));
#202774=CARTESIAN_POINT('Ctrl Pts',(-24.4678390241573,37.9086652249051,
-231.694544993519));
#202775=CARTESIAN_POINT('Ctrl Pts',(-24.7575586284418,38.2734572988675,
-231.091774329981));
#202776=CARTESIAN_POINT('Ctrl Pts',(-24.8338303793635,38.3694926716625,
-230.933088575782));
#202777=CARTESIAN_POINT('Ctrl Pts',(-24.910886561832,38.4662559972377,-230.773246849354));
#202778=CARTESIAN_POINT('Ctrl Pts',(-24.9887351655947,38.5637473465457,
-230.612248954828));
#202779=CARTESIAN_POINT('Ctrl Pts',(-25.1755142162996,38.7976544533602,
-230.225973126467));
#202780=CARTESIAN_POINT('Ctrl Pts',(-25.3668559491288,39.0357523185106,
-229.833042219166));
#202781=CARTESIAN_POINT('Ctrl Pts',(-25.5628869758507,39.2780421787683,
-229.433455789082));
#202782=CARTESIAN_POINT('Ctrl Pts',(-25.6609024892116,39.3991871088971,
-229.23366257404));
#202783=CARTESIAN_POINT('Ctrl Pts',(-25.7600905647287,39.521380045916,-229.032205503484));
#202784=CARTESIAN_POINT('Ctrl Pts',(-25.8604684704001,39.6446211959334,
-228.829084681626));
#202785=CARTESIAN_POINT('Ctrl Pts',(-25.9106574232357,39.706241770942,-228.727524270697));
#202786=CARTESIAN_POINT('Ctrl Pts',(-25.9611438336268,39.768124399285,-228.625547922004));
#202787=CARTESIAN_POINT('Ctrl Pts',(-26.0119299676247,39.8302691107557,
-228.523155661133));
#202788=CARTESIAN_POINT('Ctrl Pts',(-26.0373230346236,39.8613414664911,
-228.471959530698));
#202789=CARTESIAN_POINT('Ctrl Pts',(-26.0627910325259,39.8924793430169,
-228.420659422224));
#202790=CARTESIAN_POINT('Ctrl Pts',(-26.0883342475814,39.9236827441997,
-228.369255339306));
#202791=CARTESIAN_POINT('Ctrl Pts',(-26.1074916588731,39.9470852950868,
-228.330702277118));
#202792=CARTESIAN_POINT('Ctrl Pts',(-26.1266913798135,39.9705247035944,
-228.292090729306));
#202793=CARTESIAN_POINT('Ctrl Pts',(-26.1459335324298,39.9940009714088,
-228.253420697542));
#202794=CARTESIAN_POINT('Ctrl Pts',(-26.1523475833019,40.0018263940136,
-228.240530686954));
#202795=CARTESIAN_POINT('Ctrl Pts',(-26.159603988047,40.0106774358069,-228.225951592293));
#202796=CARTESIAN_POINT('Ctrl Pts',(-26.1651898335708,40.0174895257253,
-228.214731171203));
#202797=CARTESIAN_POINT('Ctrl Pts',(-26.4784456003041,40.3995134183188,
-227.585486843432));
#202798=CARTESIAN_POINT('Ctrl Pts',(-26.8042399378866,40.7928975113341,
-226.938117284709));
#202799=CARTESIAN_POINT('Ctrl Pts',(-27.1430237328783,41.1976515383687,
-226.272617727839));
#202800=CARTESIAN_POINT('Ctrl Pts',(-27.1908671777602,41.254811376795,-226.178635099866));
#202801=CARTESIAN_POINT('Ctrl Pts',(-27.2389697606827,41.3121979844456,
-226.084290897946));
#202802=CARTESIAN_POINT('Ctrl Pts',(-27.2873328347012,41.3698114029867,
-225.989585108865));
#202803=CARTESIAN_POINT('Ctrl Pts',(-27.4827460398511,41.6026010468474,
-225.60692205102));
#202804=CARTESIAN_POINT('Ctrl Pts',(-27.6824126124695,41.8390934527353,
-225.218356004158));
#202805=CARTESIAN_POINT('Ctrl Pts',(-27.8864313861877,42.0792915016639,
-224.823887988709));
#202806=CARTESIAN_POINT('Ctrl Pts',(-27.9884407730468,42.1993905261282,
-224.626653980985));
#202807=CARTESIAN_POINT('Ctrl Pts',(-28.0915382097496,42.3204159683605,
-224.427944485158));
#202808=CARTESIAN_POINT('Ctrl Pts',(-28.1957371229962,42.4423682592528,
-224.227759780574));
#202809=CARTESIAN_POINT('Ctrl Pts',(-28.2478365796194,42.5033444046989,
-224.127667428282));
#202810=CARTESIAN_POINT('Ctrl Pts',(-28.3002114053509,42.5645522628344,
-224.027206274105));
#202811=CARTESIAN_POINT('Ctrl Pts',(-28.3528633081307,42.6259918913164,
-223.926376358727));
#202812=CARTESIAN_POINT('Ctrl Pts',(-28.3791892595206,42.6567117055573,
-223.875961401039));
#202813=CARTESIAN_POINT('Ctrl Pts',(-28.4055844801704,42.6874894624216,
-223.825454253071));
#202814=CARTESIAN_POINT('Ctrl Pts',(-28.4320491872001,42.7183251694128,
-223.774854920477));
#202815=CARTESIAN_POINT('Ctrl Pts',(-28.4518977174724,42.7414519496563,
-223.736905421032));
#202816=CARTESIAN_POINT('Ctrl Pts',(-28.4717853338333,42.7646113268491,
-223.698904067736));
#202817=CARTESIAN_POINT('Ctrl Pts',(-28.4917121286658,42.7878033042288,
-223.660850863104));
#202818=CARTESIAN_POINT('Ctrl Pts',(-28.4983543936099,42.7955339633554,
-223.64816646156));
#202819=CARTESIAN_POINT('Ctrl Pts',(-28.5058234396025,42.8042250770556,
-223.633906381256));
#202820=CARTESIAN_POINT('Ctrl Pts',(-28.5116519864808,42.8110061484612,
-223.622780374796));
#202821=CARTESIAN_POINT('Ctrl Pts',(-28.8846789866944,43.2449947184182,
-222.910715961337));
#202822=CARTESIAN_POINT('Ctrl Pts',(-29.2740946136785,43.6935589406833,
-222.175300745994));
#202823=CARTESIAN_POINT('Ctrl Pts',(-29.6803694781413,44.1567272852874,
-221.416525967767));
#202824=CARTESIAN_POINT('Ctrl Pts',(-29.8835069103727,44.3883114575895,
-221.037138578654));
#202825=CARTESIAN_POINT('Ctrl Pts',(-30.0908607695619,44.6235468200016,
-220.65191152586));
#202826=CARTESIAN_POINT('Ctrl Pts',(-30.3024996229282,44.8624379324151,
-220.260845174858));
#202827=CARTESIAN_POINT('Ctrl Pts',(-30.4083190496114,44.9818834886218,
-220.065311999357));
#202828=CARTESIAN_POINT('Ctrl Pts',(-30.5152097241604,45.10224299076,-219.868319004086));
#202829=CARTESIAN_POINT('Ctrl Pts',(-30.6231809422163,45.2235170782419,
-219.669866346784));
#202830=CARTESIAN_POINT('Ctrl Pts',(-30.6771665512442,45.2841541219828,
-219.570640018133));
#202831=CARTESIAN_POINT('Ctrl Pts',(-30.7314222961001,45.3450198126418,
-219.471048774303));
#202832=CARTESIAN_POINT('Ctrl Pts',(-30.7859493585771,45.4061142340476,
-219.371092639537));
#202833=CARTESIAN_POINT('Ctrl Pts',(-30.8132128898157,45.4366614447505,
-219.321114572154));
#202834=CARTESIAN_POINT('Ctrl Pts',(-30.8405442504562,45.4672658381784,
-219.271045282059));
#202835=CARTESIAN_POINT('Ctrl Pts',(-30.8679435906687,45.4979274250916,
-219.220884772699));
#202836=CARTESIAN_POINT('Ctrl Pts',(-30.8884930958281,45.5209236152766,
-219.183264390679));
#202837=CARTESIAN_POINT('Ctrl Pts',(-30.9090808394965,45.5439519768002,
-219.145592697825));
#202838=CARTESIAN_POINT('Ctrl Pts',(-30.9297068855559,45.5670125142704,
-219.107869695687));
#202839=CARTESIAN_POINT('Ctrl Pts',(-30.9365822342424,45.5746993600938,
-219.095295361641));
#202840=CARTESIAN_POINT('Ctrl Pts',(-30.9443002873472,45.5833269031714,
-219.081182394694));
#202841=CARTESIAN_POINT('Ctrl Pts',(-30.9503457014926,45.5900837772301,
-219.070129590519));
#202842=CARTESIAN_POINT('Ctrl Pts',(-31.3783887818336,46.0685014862618,
-218.28754030354));
#202843=CARTESIAN_POINT('Ctrl Pts',(-31.826098659014,46.5643404167945,-217.477019211197));
#202844=CARTESIAN_POINT('Ctrl Pts',(-32.2939772733384,47.0776507896269,
-216.638564146678));
#202845=CARTESIAN_POINT('Ctrl Pts',(-32.6719260436299,47.4922989873653,
-215.96126655094));
#202846=CARTESIAN_POINT('Ctrl Pts',(-33.0630364837259,47.9183480882516,
-215.265741238066));
#202847=CARTESIAN_POINT('Ctrl Pts',(-33.4675962034302,48.3558337693674,
-214.551986533665));
#202848=CARTESIAN_POINT('Ctrl Pts',(-33.4676025732012,48.3558411518987,
-214.551991264071));
#202849=CARTESIAN_POINT('Ctrl Pts',(-34.986173088576,48.1318948779757,-214.551622026082));
#202850=CARTESIAN_POINT('Ctrl Pts',(-36.5024599607171,47.8927123635888,
-214.551192124683));
#202851=CARTESIAN_POINT('Ctrl Pts',(-39.5299978799685,47.3839481265764,
-214.550248248569));
#202852=CARTESIAN_POINT('Ctrl Pts',(-41.0411822924498,47.1143775777148,
-214.549734342702));
#202853=CARTESIAN_POINT('Ctrl Pts',(-42.5495440571184,46.8296601105062,
-214.549225394074));
#202854=CARTESIAN_POINT('Origin',(296.501483394397,-25.4138432731711,-232.85005));
#202855=CARTESIAN_POINT('',(-47.6963129660555,-31.8956500308477,-232.849931330248));
#202856=CARTESIAN_POINT('Origin',(636.934816028482,-11.5034818258361,-232.85005));
#202857=CARTESIAN_POINT('Ctrl Pts',(-47.696355285306,-31.8961636867541,
-232.85005));
#202858=CARTESIAN_POINT('Ctrl Pts',(-47.7198209970693,-32.0141643773229,
-232.85005));
#202859=CARTESIAN_POINT('Ctrl Pts',(-47.7444480612299,-32.1319277281148,
-232.850050000009));
#202860=CARTESIAN_POINT('Ctrl Pts',(-47.7960571707323,-32.367227820781,
-232.850050000009));
#202861=CARTESIAN_POINT('Ctrl Pts',(-47.8230417127441,-32.484751255595,
-232.85005));
#202862=CARTESIAN_POINT('Ctrl Pts',(-47.8511636801456,-32.6020082275457,
-232.85005));
#202863=CARTESIAN_POINT('Ctrl Pts',(-47.0825542034256,-41.7715518889728,
-232.85005));
#202864=CARTESIAN_POINT('Ctrl Pts',(-46.9318457802784,-42.0078889334137,
-232.85005));
#202865=CARTESIAN_POINT('Ctrl Pts',(-46.790407810866,-42.2260222196836,
-232.85005));
#202866=CARTESIAN_POINT('Ctrl Pts',(-46.4935676456938,-42.6770301149308,
-232.85005));
#202867=CARTESIAN_POINT('Ctrl Pts',(-46.3418104287299,-42.9039683374183,
-232.85005));
#202868=CARTESIAN_POINT('Ctrl Pts',(-45.8752836486906,-43.5906554858717,
-232.85005));
#202869=CARTESIAN_POINT('Ctrl Pts',(-45.5551891811036,-44.0469551839436,
-232.85005));
#202870=CARTESIAN_POINT('Ctrl Pts',(-44.5502158894675,-45.434541329739,
-232.85005));
#202871=CARTESIAN_POINT('Ctrl Pts',(-43.8423500925213,-46.3501756007727,
-232.85005));
#202872=CARTESIAN_POINT('Ctrl Pts',(-41.5657247068321,-49.1071648985542,
-232.85005));
#202873=CARTESIAN_POINT('Ctrl Pts',(-39.8686235209219,-50.9065939957953,
-232.85005));
#202874=CARTESIAN_POINT('Ctrl Pts',(-36.3067467607518,-54.2094198215295,
-232.85005));
#202875=CARTESIAN_POINT('Ctrl Pts',(-34.3620922232014,-55.779993285671,
-232.85005));
#202876=CARTESIAN_POINT('Ctrl Pts',(-29.6879673386845,-59.0721264532024,
-232.85005));
#202877=CARTESIAN_POINT('Ctrl Pts',(-27.4993617066061,-60.2539794127404,
-232.85005));
#202878=CARTESIAN_POINT('Ctrl Pts',(-26.5827048610815,-60.7443921296953,
-232.85005));
#202879=CARTESIAN_POINT('',(-21.0035766188647,-61.257476972142,-232.850047644298));
#202880=CARTESIAN_POINT('Origin',(-0.0517782018608104,643.799970559367,
-232.855108201462));
#202881=CARTESIAN_POINT('',(-20.3871357022546,-61.1221564407624,-232.850041788805));
#202882=CARTESIAN_POINT('Ctrl Pts',(-20.3871899403996,-61.1221588841743,
-232.85005));
#202883=CARTESIAN_POINT('Ctrl Pts',(-20.4903351182891,-61.1426979252124,
-232.85005));
#202884=CARTESIAN_POINT('Ctrl Pts',(-20.5932743876283,-61.1642481051797,
-232.850050000001));
#202885=CARTESIAN_POINT('Ctrl Pts',(-20.7987564077172,-61.2093548950234,
-232.850050000001));
#202886=CARTESIAN_POINT('Ctrl Pts',(-20.901290168981,-61.2329102063362,
-232.85005));
#202887=CARTESIAN_POINT('Ctrl Pts',(-21.0035920114341,-61.2574518715733,
-232.85005));
#202888=CARTESIAN_POINT('Origin',(-7.14692237356698E-14,623.509175991979,
-232.85005));
#202889=CARTESIAN_POINT('Ctrl Pts',(-25.2562521239792,-61.0455007230049,
-232.959725695103));
#202890=CARTESIAN_POINT('Ctrl Pts',(-30.6613188291079,-64.9426708583199,
-226.793511106062));
#202891=CARTESIAN_POINT('Ctrl Pts',(-36.0671479350067,-68.8395145916166,
-220.627759071707));
#202892=CARTESIAN_POINT('Ctrl Pts',(-41.4730739204624,-72.736318130574,
-214.462066626483));
#202893=CARTESIAN_POINT('Ctrl Pts',(-23.6900699183709,-61.1001919234539,
-232.961968408598));
#202894=CARTESIAN_POINT('Ctrl Pts',(-28.7297131786069,-65.012574288375,
-226.795902612053));
#202895=CARTESIAN_POINT('Ctrl Pts',(-33.7700272351411,-68.9255509631158,
-220.630194103463));
#202896=CARTESIAN_POINT('Ctrl Pts',(-38.8104606792061,-72.8393402290212,
-214.464534772546));
#202897=CARTESIAN_POINT('Ctrl Pts',(-22.115564575717,-61.1500631726904,
-232.964012351071));
#202898=CARTESIAN_POINT('Ctrl Pts',(-26.7965523266534,-65.0759017171342,
-226.798067164761));
#202899=CARTESIAN_POINT('Ctrl Pts',(-31.4781225651976,-69.0031581792391,
-220.632397171727));
#202900=CARTESIAN_POINT('Ctrl Pts',(-36.1598241774431,-72.9319991467586,
-214.466766784373));
#202901=CARTESIAN_POINT('Ctrl Pts',(-20.5341645416114,-61.1949426407512,
-232.965861592748));
#202902=CARTESIAN_POINT('Ctrl Pts',(-24.8619705593691,-65.1326290782542,
-226.800008788317));
#202903=CARTESIAN_POINT('Ctrl Pts',(-29.1902811104598,-69.0724625871147,
-220.634368994467));
#202904=CARTESIAN_POINT('Ctrl Pts',(-33.5187281767876,-73.0145710177392,
-214.468761046583));
#202905=CARTESIAN_POINT('',(-33.4888847838974,-72.9429804215028,-214.578390315157));
#202906=CARTESIAN_POINT('Ctrl Pts',(-21.0035766188647,-61.257476972142,
-232.850047644298));
#202907=CARTESIAN_POINT('Ctrl Pts',(-21.4855291169009,-61.7123302898789,
-232.13856112446));
#202908=CARTESIAN_POINT('Ctrl Pts',(-21.9854835224216,-62.1838047440078,
-231.401113733466));
#202909=CARTESIAN_POINT('Ctrl Pts',(-22.5035510757124,-62.6718647794899,
-230.637765485951));
#202910=CARTESIAN_POINT('Ctrl Pts',(-22.961623614274,-63.1034048325268,
-229.962817079465));
#202911=CARTESIAN_POINT('Ctrl Pts',(-23.4338577616424,-63.5479114810121,
-229.267619379724));
#202912=CARTESIAN_POINT('Ctrl Pts',(-23.9203643500785,-64.0053593573632,
-228.552213807771));
#202913=CARTESIAN_POINT('Ctrl Pts',(-24.4387307921192,-64.4927641196409,
-227.789958476056));
#202914=CARTESIAN_POINT('Ctrl Pts',(-24.9732848589469,-64.9948621266171,
-227.004760241598));
#202915=CARTESIAN_POINT('Ctrl Pts',(-25.5241023969115,-65.5116339688911,
-226.196655135222));
#202916=CARTESIAN_POINT('Ctrl Pts',(-25.7995111658937,-65.7700198900281,
-225.792602582035));
#202917=CARTESIAN_POINT('Ctrl Pts',(-26.078985368137,-66.03207440159,-225.38282313732));
#202918=CARTESIAN_POINT('Ctrl Pts',(-26.362531603249,-66.2977959631439,
-224.967320133644));
#202919=CARTESIAN_POINT('Ctrl Pts',(-26.504304720805,-66.4306567439208,
-224.759568631806));
#202920=CARTESIAN_POINT('Ctrl Pts',(-26.6470958466098,-66.5644342873659,
-224.550386240369));
#202921=CARTESIAN_POINT('Ctrl Pts',(-26.7909055674976,-66.699128475012,
-224.339773277289));
#202922=CARTESIAN_POINT('Ctrl Pts',(-26.8628104279415,-66.766475568835,
-224.234466795749));
#202923=CARTESIAN_POINT('Ctrl Pts',(-26.9349699371596,-66.8340518237192,
-224.128802671308));
#202924=CARTESIAN_POINT('Ctrl Pts',(-27.0073841607627,-66.9018572273527,
-224.022780940459));
#202925=CARTESIAN_POINT('Ctrl Pts',(-27.0435912725642,-66.9357599291695,
-223.969770075035));
#202926=CARTESIAN_POINT('Ctrl Pts',(-27.0798620629622,-66.9697199181742,
-223.916669808009));
#202927=CARTESIAN_POINT('Ctrl Pts',(-27.1161965393057,-67.0037371930959,
-223.863480143587));
#202928=CARTESIAN_POINT('Ctrl Pts',(-27.1502601108777,-67.0356283883349,
-223.813614833192));
#202929=CARTESIAN_POINT('Ctrl Pts',(-27.1843796564252,-67.0675699325244,
-223.763670950868));
#202930=CARTESIAN_POINT('Ctrl Pts',(-27.2185551816222,-67.0995618247377,
-223.71364849992));
#202931=CARTESIAN_POINT('Ctrl Pts',(-27.2208335499687,-67.1016946175519,
-223.710313669857));
#202932=CARTESIAN_POINT('Ctrl Pts',(-27.2236948361456,-67.1043730690699,
-223.706125650112));
#202933=CARTESIAN_POINT('Ctrl Pts',(-27.2253910330544,-67.1059608744884,
-223.703642962148));
#202934=CARTESIAN_POINT('Ctrl Pts',(-27.6762562132143,-67.5280145714332,
-223.043721021226));
#202935=CARTESIAN_POINT('Ctrl Pts',(-28.1506357027507,-67.9716482766551,
-222.350079919967));
#202936=CARTESIAN_POINT('Ctrl Pts',(-28.6486036964326,-68.4368359628475,
-221.622769209847));
#202937=CARTESIAN_POINT('Ctrl Pts',(-29.1347392918129,-68.8909701555265,
-220.912740393585));
#202938=CARTESIAN_POINT('Ctrl Pts',(-29.6433554842619,-69.365646209218,
-220.170623031685));
#202939=CARTESIAN_POINT('Ctrl Pts',(-30.1745694141053,-69.8608390978478,
-219.396463103265));
#202940=CARTESIAN_POINT('Ctrl Pts',(-30.6879409058229,-70.3393994247554,
-218.648305694445));
#202941=CARTESIAN_POINT('Ctrl Pts',(-31.2224175099817,-70.8371215031639,
-217.870222065641));
#202942=CARTESIAN_POINT('Ctrl Pts',(-31.7781526360163,-71.3539817960171,
-217.062253580961));
#202943=CARTESIAN_POINT('Ctrl Pts',(-32.3275541022051,-71.8649514817638,
-216.263493435486));
#202944=CARTESIAN_POINT('Ctrl Pts',(-32.8977320509018,-72.3946256494591,
-215.435525743744));
#202945=CARTESIAN_POINT('Ctrl Pts',(-33.4888847838974,-72.9429804215028,
-214.578390315157));
#202946=CARTESIAN_POINT('Ctrl Pts',(-41.3748964705093,-72.6655519150593,
-214.574036340781));
#202947=CARTESIAN_POINT('Ctrl Pts',(-40.0607372977895,-72.716660645803,
-214.574827132799));
#202948=CARTESIAN_POINT('Ctrl Pts',(-38.7464886157383,-72.7653339442144,
-214.575594614694));
#202949=CARTESIAN_POINT('Ctrl Pts',(-36.1178114852045,-72.8578102117473,
-214.577053530306));
#202950=CARTESIAN_POINT('Ctrl Pts',(-34.8033905902617,-72.9016129219457,
-214.577744931601));
#202951=CARTESIAN_POINT('Ctrl Pts',(-33.4888912371591,-72.9429802184569,
-214.578390311931));
#202952=CARTESIAN_POINT('Origin',(0.,-12.9675000200281,-215.85005));
#202953=CARTESIAN_POINT('',(-48.0827620446565,42.0414223951255,-215.85005));
#202954=CARTESIAN_POINT('Ctrl Pts',(-49.1680521502591,41.086535378401,-215.85005));
#202955=CARTESIAN_POINT('Ctrl Pts',(-48.9888707647949,41.2476479220656,
-215.85005));
#202956=CARTESIAN_POINT('Ctrl Pts',(-48.8088730843222,41.4077049862833,
-215.850050000001));
#202957=CARTESIAN_POINT('Ctrl Pts',(-48.4481130991412,41.725084481334,-215.850050000001));
#202958=CARTESIAN_POINT('Ctrl Pts',(-48.265340719459,41.8841953684814,-215.85005));
#202959=CARTESIAN_POINT('Ctrl Pts',(-48.0827620446564,42.0414223951254,
-215.85005));
#202960=CARTESIAN_POINT('',(-54.6458252041307,35.5078877047658,-215.85005));
#202961=CARTESIAN_POINT('Ctrl Pts',(-54.6458252041308,35.5078877047659,
-215.85005));
#202962=CARTESIAN_POINT('Ctrl Pts',(-54.4864708806764,35.6908450584155,
-215.85005));
#202963=CARTESIAN_POINT('Ctrl Pts',(-54.3265120584759,35.8725242596181,
-215.850050000225));
#202964=CARTESIAN_POINT('Ctrl Pts',(-54.0074980938231,36.2310904022842,
-215.850050000225));
#202965=CARTESIAN_POINT('Ctrl Pts',(-53.8465341367002,36.410205079622,-215.85005));
#202966=CARTESIAN_POINT('Ctrl Pts',(-53.6858060762413,36.5871897873468,
-215.85005));
#202967=CARTESIAN_POINT('Origin',(-48.892180948596,36.2913696007177,-215.85005));
#202968=CARTESIAN_POINT('Ctrl Pts',(-28.7632636728437,36.243359951239,-233.011888154992));
#202969=CARTESIAN_POINT('Ctrl Pts',(-31.7703631777874,37.7316226214323,
-229.879662179404));
#202970=CARTESIAN_POINT('Ctrl Pts',(-34.7738161809111,39.2196944596949,
-226.746236332649));
#202971=CARTESIAN_POINT('Ctrl Pts',(-37.7725662199917,40.7095348345317,
-223.611574672556));
#202972=CARTESIAN_POINT('Ctrl Pts',(-40.7713162590722,42.1993752093685,
-220.476913012461));
#202973=CARTESIAN_POINT('Ctrl Pts',(-43.7653510607838,43.6909491168262,
-217.340988222568));
#202974=CARTESIAN_POINT('Ctrl Pts',(-46.7534875501661,45.1873665995436,
-214.204156771482));
#202975=CARTESIAN_POINT('Ctrl Pts',(-28.818156654463,36.2102288606094,-233.012213872822));
#202976=CARTESIAN_POINT('Ctrl Pts',(-31.8223098653572,37.6990724529492,
-229.880007982271));
#202977=CARTESIAN_POINT('Ctrl Pts',(-34.8228081429799,39.18767633626,-226.746603037528));
#202978=CARTESIAN_POINT('Ctrl Pts',(-37.8185924512592,40.6780007601943,
-223.611963071785));
#202979=CARTESIAN_POINT('Ctrl Pts',(-40.8143767595385,42.1683251841286,
-220.477323106043));
#202980=CARTESIAN_POINT('Ctrl Pts',(-43.8054348260158,43.6603350812977,
-217.341420791685));
#202981=CARTESIAN_POINT('Ctrl Pts',(-46.7905804536569,45.1571425161278,
-214.2046126078));
#202982=CARTESIAN_POINT('Ctrl Pts',(-28.8701497243513,36.1801317847072,
-233.011182834863));
#202983=CARTESIAN_POINT('Ctrl Pts',(-31.871666643597,37.6692800952327,-229.879182435101));
#202984=CARTESIAN_POINT('Ctrl Pts',(-34.8695237116303,39.1581256922717,
-226.745980987327));
#202985=CARTESIAN_POINT('Ctrl Pts',(-37.8626041662257,40.6486877405231,
-223.611516219864));
#202986=CARTESIAN_POINT('Ctrl Pts',(-40.8556846208211,42.1392497887745,
-220.4770514524));
#202987=CARTESIAN_POINT('Ctrl Pts',(-43.8439779916275,43.6314868745012,
-217.341294913291));
#202988=CARTESIAN_POINT('Ctrl Pts',(-46.8261837881837,45.128675130066,-214.204570275934));
#202989=CARTESIAN_POINT('Ctrl Pts',(-28.9236494148868,36.1483017803918,
-233.01082974273));
#202990=CARTESIAN_POINT('Ctrl Pts',(-31.9223177157407,37.6379530768432,
-229.878939694123));
#202991=CARTESIAN_POINT('Ctrl Pts',(-34.9173208817124,39.1272459095225,
-226.745848865747));
#202992=CARTESIAN_POINT('Ctrl Pts',(-37.9075126656038,40.6182282999103,
-223.611482166239));
#202993=CARTESIAN_POINT('Ctrl Pts',(-40.8977044494953,42.109210690298,-220.477115466732));
#202994=CARTESIAN_POINT('Ctrl Pts',(-43.8830754570229,43.6018377843273,
-217.341443930439));
#202995=CARTESIAN_POINT('Ctrl Pts',(-46.8622654530928,45.0994691148216,
-214.204774369339));
#202996=CARTESIAN_POINT('Ctrl Pts',(-28.9771491054224,36.1164717760765,
-233.010476650599));
#202997=CARTESIAN_POINT('Ctrl Pts',(-31.9729687878842,37.6066260584536,
-229.878696953144));
#202998=CARTESIAN_POINT('Ctrl Pts',(-34.9651180517945,39.0963661267734,
-226.745716744168));
#202999=CARTESIAN_POINT('Ctrl Pts',(-37.952421164982,40.5877688592974,-223.611448112616));
#203000=CARTESIAN_POINT('Ctrl Pts',(-40.9397242781695,42.0791715918215,
-220.477179481064));
#203001=CARTESIAN_POINT('Ctrl Pts',(-43.9221729224182,43.5721886941534,
-217.341592947587));
#203002=CARTESIAN_POINT('Ctrl Pts',(-46.8983471180018,45.0702630995771,
-214.204978462744));
#203003=CARTESIAN_POINT('Ctrl Pts',(-29.030685932722,36.0844977879761,-233.010123307814));
#203004=CARTESIAN_POINT('Ctrl Pts',(-32.0236191310345,37.5751950097359,
-229.878452353611));
#203005=CARTESIAN_POINT('Ctrl Pts',(-35.012877532973,39.0654224083999,-226.745581710878));
#203006=CARTESIAN_POINT('Ctrl Pts',(-37.997256377555,40.5572850161139,-223.611410887796));
#203007=CARTESIAN_POINT('Ctrl Pts',(-40.9816352221372,42.0491476238279,
-220.477240064714));
#203008=CARTESIAN_POINT('Ctrl Pts',(-43.9611273848811,43.5425935498471,
-217.341739105347));
#203009=CARTESIAN_POINT('Ctrl Pts',(-46.934252483156,45.041149319151,-214.205180808032));
#203010=CARTESIAN_POINT('Ctrl Pts',(-29.0842579792521,36.0523797092374,
-233.009769824147));
#203011=CARTESIAN_POINT('Ctrl Pts',(-32.0742678787604,37.5436593534111,
-229.878206054095));
#203012=CARTESIAN_POINT('Ctrl Pts',(-35.0605994496261,39.0344137463011,
-226.745443927067));
#203013=CARTESIAN_POINT('Ctrl Pts',(-38.0420193927072,40.5267753480634,
-223.611370632498));
#203014=CARTESIAN_POINT('Ctrl Pts',(-41.0234393357883,42.0191369498257,
-220.477297337928));
#203015=CARTESIAN_POINT('Ctrl Pts',(-43.9999418407127,43.5130501216253,
-217.341882483075));
#203016=CARTESIAN_POINT('Ctrl Pts',(-46.9699855652835,45.0121250312964,
-214.205381478311));
#203017=CARTESIAN_POINT('Ctrl Pts',(-29.1914020723121,35.98814355176,-233.009062856813));
#203018=CARTESIAN_POINT('Ctrl Pts',(-32.1755653742122,37.4805880407614,
-229.877713455064));
#203019=CARTESIAN_POINT('Ctrl Pts',(-35.1560432829324,38.9723964221036,
-226.745168359446));
#203020=CARTESIAN_POINT('Ctrl Pts',(-38.1315454230114,40.4657560119625,
-223.611290121901));
#203021=CARTESIAN_POINT('Ctrl Pts',(-41.1070475630904,41.9591156018214,
-220.477411884356));
#203022=CARTESIAN_POINT('Ctrl Pts',(-44.0775707523758,43.4539632651818,
-217.342169238531));
#203023=CARTESIAN_POINT('Ctrl Pts',(-47.0414517295384,44.9540764555871,
-214.205782818867));
#203024=CARTESIAN_POINT('Ctrl Pts',(-29.2986870405764,35.9233310293129,
-233.008355328346));
#203025=CARTESIAN_POINT('Ctrl Pts',(-32.2768564887194,37.4170982945592,
-229.877214059559));
#203026=CARTESIAN_POINT('Ctrl Pts',(-35.2513368575648,38.9101193220809,
-226.744881791608));
#203027=CARTESIAN_POINT('Ctrl Pts',(-38.220782661284,40.4046333779168,-223.611197490097));
#203028=CARTESIAN_POINT('Ctrl Pts',(-41.1902284650032,41.8991474337527,
-220.477513188586));
#203029=CARTESIAN_POINT('Ctrl Pts',(-44.1546396323386,43.3950832783248,
-217.342444873235));
#203030=CARTESIAN_POINT('Ctrl Pts',(-47.1122287537746,44.8963858575329,
-214.206177460189));
#203031=CARTESIAN_POINT('Ctrl Pts',(-29.4060975644904,35.8579413159883,
-233.007648088092));
#203032=CARTESIAN_POINT('Ctrl Pts',(-32.3781342806196,37.3531855340767,
-229.87670909491));
#203033=CARTESIAN_POINT('Ctrl Pts',(-35.3464811752108,38.8475743913038,
-226.744585492565));
#203034=CARTESIAN_POINT('Ctrl Pts',(-38.3097398506307,40.3433960477796,
-223.611093856846));
#203035=CARTESIAN_POINT('Ctrl Pts',(-41.2729985260507,41.8392177042554,
-220.477602221127));
#203036=CARTESIAN_POINT('Ctrl Pts',(-44.231172512421,43.3363922589179,-217.342710032053));
#203037=CARTESIAN_POINT('Ctrl Pts',(-47.182348866173,44.8390312087872,-214.206565980874));
#203038=CARTESIAN_POINT('Ctrl Pts',(-29.6209186123181,35.727161889339,-233.006233607583));
#203039=CARTESIAN_POINT('Ctrl Pts',(-32.5806898644201,37.2253600131119,
-229.875699165609));
#203040=CARTESIAN_POINT('Ctrl Pts',(-35.5367698105028,38.7224845297496,
-226.743992894479));
#203041=CARTESIAN_POINT('Ctrl Pts',(-38.4876542293243,40.2209213875052,
-223.610886590344));
#203042=CARTESIAN_POINT('Ctrl Pts',(-41.4385386481458,41.7193582452608,
-220.477780286209));
#203043=CARTESIAN_POINT('Ctrl Pts',(-44.3842382725856,43.2190102201042,
-217.343240349689));
#203044=CARTESIAN_POINT('Ctrl Pts',(-47.3225890909698,44.7243219112958,
-214.207343022243));
#203045=CARTESIAN_POINT('Ctrl Pts',(-29.8362418555055,35.5940736601297,
-233.004820318005));
#203046=CARTESIAN_POINT('Ctrl Pts',(-32.7831921644516,37.0958423851614,
-229.874667015866));
#203047=CARTESIAN_POINT('Ctrl Pts',(-35.7264614073862,38.5963233250342,
-226.743361409764));
#203048=CARTESIAN_POINT('Ctrl Pts',(-38.664448374147,40.0979879599528,-223.610635340874));
#203049=CARTESIAN_POINT('Ctrl Pts',(-41.6024353409078,41.5996525948713,
-220.477909271983));
#203050=CARTESIAN_POINT('Ctrl Pts',(-44.5351599478724,43.1023841297568,
-217.343728766806));
#203051=CARTESIAN_POINT('Ctrl Pts',(-47.4602015413284,44.6109565161706,
-214.208095611128));
#203052=CARTESIAN_POINT('Ctrl Pts',(-30.0519450660363,35.4586704870703,
-233.00341455534));
#203053=CARTESIAN_POINT('Ctrl Pts',(-32.9855855312196,36.9645966036217,
-229.87362179639));
#203054=CARTESIAN_POINT('Ctrl Pts',(-35.9155640960709,38.4690265434296,
-226.742700788357));
#203055=CARTESIAN_POINT('Ctrl Pts',(-38.8401926838925,39.9745043257835,
-223.610348870589));
#203056=CARTESIAN_POINT('Ctrl Pts',(-41.7648212717142,41.4799821081373,
-220.477996952821));
#203057=CARTESIAN_POINT('Ctrl Pts',(-44.6841307999907,42.986369790773,-217.344180493823));
#203058=CARTESIAN_POINT('Ctrl Pts',(-47.5954455649975,44.4987574479709,
-214.208828131933));
#203059=CARTESIAN_POINT('Ctrl Pts',(-30.4833514870981,35.1878641409515,
-233.000603030011));
#203060=CARTESIAN_POINT('Ctrl Pts',(-33.3903722647552,36.7021050405422,
-229.871531357437));
#203061=CARTESIAN_POINT('Ctrl Pts',(-36.2937694734405,38.2144329802205,
-226.741379545545));
#203062=CARTESIAN_POINT('Ctrl Pts',(-39.1916813033838,39.727537057445,-223.60977593002));
#203063=CARTESIAN_POINT('Ctrl Pts',(-42.089593133327,41.2406411346694,-220.478172314495));
#203064=CARTESIAN_POINT('Ctrl Pts',(-44.9820725042275,42.7543411128055,
-217.345083947855));
#203065=CARTESIAN_POINT('Ctrl Pts',(-47.8659336123358,44.2743593115718,
-214.210293173543));
#203066=CARTESIAN_POINT('Ctrl Pts',(-30.916277333454,34.9077973812142,-232.997822214095));
#203067=CARTESIAN_POINT('Ctrl Pts',(-33.7947232111487,36.4327000734428,
-229.869389558127));
#203068=CARTESIAN_POINT('Ctrl Pts',(-36.6696189896331,37.9552966453494,
-226.739942596491));
#203069=CARTESIAN_POINT('Ctrl Pts',(-39.5389699559083,39.4783689999817,
-223.60906282344));
#203070=CARTESIAN_POINT('Ctrl Pts',(-42.4083209221835,41.001441354614,-220.47818305039));
#203071=CARTESIAN_POINT('Ctrl Pts',(-45.2722095136632,42.5247604673061,
-217.345841145671));
#203072=CARTESIAN_POINT('Ctrl Pts',(-48.1269460791978,44.0546275108218,
-214.211679022545));
#203073=CARTESIAN_POINT('Ctrl Pts',(-31.3497500510356,34.6184286458191,
-232.99511552399));
#203074=CARTESIAN_POINT('Ctrl Pts',(-34.1981927402684,36.1561028618858,
-229.86725871849));
#203075=CARTESIAN_POINT('Ctrl Pts',(-37.0431800113206,37.6911082882257,
-226.738459395528));
#203076=CARTESIAN_POINT('Ctrl Pts',(-39.8826292444588,39.2262665988641,
-223.608273410873));
#203077=CARTESIAN_POINT('Ctrl Pts',(-42.722078477597,40.7614249095024,-220.47808742622));
#203078=CARTESIAN_POINT('Ctrl Pts',(-45.5561045113048,42.2964603802716,
-217.34649079771));
#203079=CARTESIAN_POINT('Ctrl Pts',(-48.3805813576904,43.8381246360801,
-214.213011833879));
#203080=CARTESIAN_POINT('Ctrl Pts',(-32.216695486199,34.0396911750287,-232.98970214378));
#203081=CARTESIAN_POINT('Ctrl Pts',(-35.0051317985077,35.6029084387718,
-229.862997039215));
#203082=CARTESIAN_POINT('Ctrl Pts',(-37.7903020546954,37.1627315739784,
-226.7354929936));
#203083=CARTESIAN_POINT('Ctrl Pts',(-40.5699478215597,38.7220617966288,
-223.60669458574));
#203084=CARTESIAN_POINT('Ctrl Pts',(-43.3495935884239,40.2813920192791,
-220.477896177879));
#203085=CARTESIAN_POINT('Ctrl Pts',(-46.1238945065879,41.8398602062025,
-217.347790101788));
#203086=CARTESIAN_POINT('Ctrl Pts',(-48.8878519146755,43.4051188865968,
-214.215677456544));
#203087=CARTESIAN_POINT('Ctrl Pts',(-33.0858200844503,33.4237352208328,
-232.984594842862));
#203088=CARTESIAN_POINT('Ctrl Pts',(-35.8085395768491,35.0209330321244,
-229.858794403155));
#203089=CARTESIAN_POINT('Ctrl Pts',(-38.5282634124981,36.6141368109387,
-226.732360240482));
#203090=CARTESIAN_POINT('Ctrl Pts',(-41.2427386177898,38.2061131505809,
-223.604831267861));
#203091=CARTESIAN_POINT('Ctrl Pts',(-43.9572138230815,39.7980894902232,
-220.47730229524));
#203092=CARTESIAN_POINT('Ctrl Pts',(-46.6666957170646,41.3883883178512,
-217.348681905218));
#203093=CARTESIAN_POINT('Ctrl Pts',(-49.3656016298064,42.9850105281785,
-214.21816495405));
#203094=CARTESIAN_POINT('Ctrl Pts',(-33.949434877602,32.770352829909,-232.980025784665));
#203095=CARTESIAN_POINT('Ctrl Pts',(-36.6048862944054,34.4080943544835,
-229.854970428563));
#203096=CARTESIAN_POINT('Ctrl Pts',(-39.2576627597897,36.0413528393508,
-226.72942775857));
#203097=CARTESIAN_POINT('Ctrl Pts',(-41.9056884039802,37.6725825561817,
-223.603007266837));
#203098=CARTESIAN_POINT('Ctrl Pts',(-44.5537140481708,39.3038122730124,
-220.476586775106));
#203099=CARTESIAN_POINT('Ctrl Pts',(-47.1972705274053,40.9325619164058,
-217.349301164816));
#203100=CARTESIAN_POINT('Ctrl Pts',(-49.8308862116777,42.5662844245855,
-214.220385090245));
#203101=CARTESIAN_POINT('Ctrl Pts',(-35.6766644639054,31.4635880480613,
-232.97088766827));
#203102=CARTESIAN_POINT('Ctrl Pts',(-38.1975797295179,33.1824169992017,
-229.847322479379));
#203103=CARTESIAN_POINT('Ctrl Pts',(-40.7164614543727,34.8957848961753,
-226.723562794745));
#203104=CARTESIAN_POINT('Ctrl Pts',(-43.231587976361,36.605521367383,-223.599359264791));
#203105=CARTESIAN_POINT('Ctrl Pts',(-45.7467144983492,38.3152578385909,
-220.475155734837));
#203106=CARTESIAN_POINT('Ctrl Pts',(-48.2584201480868,40.0209091135152,
-217.350539684011));
#203107=CARTESIAN_POINT('Ctrl Pts',(-50.7614553754203,41.7288322173994,
-214.224825362635));
#203108=CARTESIAN_POINT('Ctrl Pts',(-37.3872308412151,30.0009912840992,
-232.96524155552));
#203109=CARTESIAN_POINT('Ctrl Pts',(-39.7663238105267,31.8283107595538,
-229.842276532991));
#203110=CARTESIAN_POINT('Ctrl Pts',(-42.1439828477997,33.6499110945716,
-226.719277469106));
#203111=CARTESIAN_POINT('Ctrl Pts',(-44.5191699020356,35.4667587805032,
-223.596189898099));
#203112=CARTESIAN_POINT('Ctrl Pts',(-46.8943569562715,37.2836064664347,
-220.473102327093));
#203113=CARTESIAN_POINT('Ctrl Pts',(-49.2672899419476,39.0954616111304,
-217.349938712546));
#203114=CARTESIAN_POINT('Ctrl Pts',(-51.6347775088331,40.905653234556,-214.226516638731));
#203115=CARTESIAN_POINT('Ctrl Pts',(-38.9866932910313,28.4456556381462,
-232.962790912271));
#203116=CARTESIAN_POINT('Ctrl Pts',(-41.2391357104746,30.3925039299732,
-229.839958591048));
#203117=CARTESIAN_POINT('Ctrl Pts',(-43.490849558744,32.3336071411576,-226.717133201801));
#203118=CARTESIAN_POINT('Ctrl Pts',(-45.7416073381742,34.2690638917383,
-223.59431099442));
#203119=CARTESIAN_POINT('Ctrl Pts',(-47.9923651176044,36.2045206423189,
-220.471488787039));
#203120=CARTESIAN_POINT('Ctrl Pts',(-50.2421837638693,38.1343124474224,
-217.348670714219));
#203121=CARTESIAN_POINT('Ctrl Pts',(-52.490668536736,40.0587201499459,-214.225843430884));
#203122=CARTESIAN_POINT('Ctrl Pts',(-40.5861557408476,26.890319992193,-232.960340269022));
#203123=CARTESIAN_POINT('Ctrl Pts',(-42.7119476104226,28.9566971003925,
-229.837640649106));
#203124=CARTESIAN_POINT('Ctrl Pts',(-44.8377162696882,31.0173031877438,
-226.714988934497));
#203125=CARTESIAN_POINT('Ctrl Pts',(-46.9640447743127,33.0713690029734,
-223.592432090741));
#203126=CARTESIAN_POINT('Ctrl Pts',(-49.0903732789372,35.1254348182031,
-220.469875246985));
#203127=CARTESIAN_POINT('Ctrl Pts',(-51.2170775857911,37.1731632837144,
-217.347402715892));
#203128=CARTESIAN_POINT('Ctrl Pts',(-53.3465595646389,39.2117870653358,
-214.225170223039));
#203129=CARTESIAN_POINT('Ctrl Pts',(-42.0829734536151,25.2333240584369,
-232.96163643903));
#203130=CARTESIAN_POINT('Ctrl Pts',(-44.0964019190368,27.4311852581839,
-229.838534751308));
#203131=CARTESIAN_POINT('Ctrl Pts',(-46.1104687275099,29.6236435023039,
-226.715389153373));
#203132=CARTESIAN_POINT('Ctrl Pts',(-48.1264950127556,31.8092762896688,
-223.592148794104));
#203133=CARTESIAN_POINT('Ctrl Pts',(-50.1425212980013,33.9949090770337,
-220.468908434835));
#203134=CARTESIAN_POINT('Ctrl Pts',(-52.1601585723181,36.1740231929721,
-217.345564448446));
#203135=CARTESIAN_POINT('Ctrl Pts',(-54.1842549207791,38.3419362669036,
-214.22207202995));
#203136=CARTESIAN_POINT('Ctrl Pts',(-43.422273991912,23.5661942096002,-232.965337149737));
#203137=CARTESIAN_POINT('Ctrl Pts',(-45.3530981989507,25.8862379834418,
-229.841157038659));
#203138=CARTESIAN_POINT('Ctrl Pts',(-47.2852714213136,28.2012404581192,
-226.716776130434));
#203139=CARTESIAN_POINT('Ctrl Pts',(-49.2205702668173,30.5094898312471,
-223.59207508571));
#203140=CARTESIAN_POINT('Ctrl Pts',(-51.155869112321,32.817739204375,-220.467374040986));
#203141=CARTESIAN_POINT('Ctrl Pts',(-53.0939569308302,35.1194950308581,
-217.342336617277));
#203142=CARTESIAN_POINT('Ctrl Pts',(-55.0403804700997,37.4099350168284,
-214.216875626567));
#203143=CARTESIAN_POINT('Ctrl Pts',(-44.7615745302087,21.8990643607635,
-232.969037860444));
#203144=CARTESIAN_POINT('Ctrl Pts',(-46.6097944788647,24.3412907086997,
-229.843779326009));
#203145=CARTESIAN_POINT('Ctrl Pts',(-48.4600741151173,26.7788374139345,
-226.718163107495));
#203146=CARTESIAN_POINT('Ctrl Pts',(-50.314645520879,29.2097033728254,-223.592001377317));
#203147=CARTESIAN_POINT('Ctrl Pts',(-52.1692169266407,31.6405693317163,
-220.465839647138));
#203148=CARTESIAN_POINT('Ctrl Pts',(-54.0277552893424,34.0649668687443,
-217.339108786108));
#203149=CARTESIAN_POINT('Ctrl Pts',(-55.8965060194204,36.4779337667532,
-214.211679223185));
#203150=CARTESIAN_POINT('Ctrl Pts',(-45.9478671932277,20.2170814818308,
-232.97487795833));
#203151=CARTESIAN_POINT('Ctrl Pts',(-47.742137018698,22.773387445697,-229.848036259254));
#203152=CARTESIAN_POINT('Ctrl Pts',(-49.5390933433176,25.3254669009981,
-226.72056760043));
#203153=CARTESIAN_POINT('Ctrl Pts',(-51.3405748716693,27.8719256903179,
-223.592376908212));
#203154=CARTESIAN_POINT('Ctrl Pts',(-53.1420564000211,30.4183844796377,
-220.464186215995));
#203155=CARTESIAN_POINT('Ctrl Pts',(-54.9479893176734,32.9592452374763,
-217.335250628456));
#203156=CARTESIAN_POINT('Ctrl Pts',(-56.7618317615675,35.4923074576668,
-214.205720218898));
#203157=CARTESIAN_POINT('Ctrl Pts',(-46.9910749481346,18.573078208412,-232.979487417878));
#203158=CARTESIAN_POINT('Ctrl Pts',(-48.777813963045,21.1992978212187,-229.849984990042));
#203159=CARTESIAN_POINT('Ctrl Pts',(-50.5669117785144,23.8226213730258,
-226.720151765023));
#203160=CARTESIAN_POINT('Ctrl Pts',(-52.3593746083135,26.4424369538029,
-223.59005292932));
#203161=CARTESIAN_POINT('Ctrl Pts',(-54.1518374381127,29.06225253458,-220.459954093617));
#203162=CARTESIAN_POINT('Ctrl Pts',(-55.9476448491922,31.678562291835,-217.329579884935));
#203163=CARTESIAN_POINT('Ctrl Pts',(-57.7483973817176,34.2905533170906,
-214.199162765268));
#203164=CARTESIAN_POINT('',(-46.7405472321667,30.7185439590785,-225.418940742796));
#203165=CARTESIAN_POINT('Ctrl Pts',(-54.6458252041307,35.5078877047659,
-215.85005));
#203166=CARTESIAN_POINT('Ctrl Pts',(-54.5943354599518,35.087122974679,-216.179655766524));
#203167=CARTESIAN_POINT('Ctrl Pts',(-54.4989704543799,34.6852639061865,
-216.528294351409));
#203168=CARTESIAN_POINT('Ctrl Pts',(-54.2127819561474,33.8548754265287,
-217.317195844329));
#203169=CARTESIAN_POINT('Ctrl Pts',(-54.0059798593604,33.4340164708342,
-217.764515858533));
#203170=CARTESIAN_POINT('Ctrl Pts',(-53.2992114913906,32.3315417127153,
-219.06879824846));
#203171=CARTESIAN_POINT('Ctrl Pts',(-52.6935858833432,31.7306722107994,
-219.957379377995));
#203172=CARTESIAN_POINT('Ctrl Pts',(-51.1420741771435,30.7313234767532,
-221.883755689445));
#203173=CARTESIAN_POINT('Ctrl Pts',(-50.1720763337667,30.4163412318132,
-222.887464054421));
#203174=CARTESIAN_POINT('Ctrl Pts',(-48.7953703137217,30.3299008816491,
-224.056790689196));
#203175=CARTESIAN_POINT('Ctrl Pts',(-48.3973293089683,30.3422930430152,
-224.368248807804));
#203176=CARTESIAN_POINT('Ctrl Pts',(-47.5822488325699,30.4570387032031,
-224.938952842351));
#203177=CARTESIAN_POINT('Ctrl Pts',(-47.1618710052275,30.5599614050353,
-225.200460248924));
#203178=CARTESIAN_POINT('Ctrl Pts',(-46.7405472321717,30.7185439590994,
-225.41894074279));
#203179=CARTESIAN_POINT('Ctrl Pts',(-28.918632420916,36.3202559369514,-232.85005));
#203180=CARTESIAN_POINT('Ctrl Pts',(-29.1405722429493,36.1874419307039,
-232.85005));
#203181=CARTESIAN_POINT('Ctrl Pts',(-29.3442027713454,36.0636271479823,
-232.85005));
#203182=CARTESIAN_POINT('Ctrl Pts',(-29.7663007847225,35.8033260589207,
-232.85005));
#203183=CARTESIAN_POINT('Ctrl Pts',(-29.9787466996519,35.6703265943611,
-232.85005));
#203184=CARTESIAN_POINT('Ctrl Pts',(-30.6209255013549,35.2622379995154,
-232.85005));
#203185=CARTESIAN_POINT('Ctrl Pts',(-31.0479818197497,34.98254405126,-232.85005));
#203186=CARTESIAN_POINT('Ctrl Pts',(-32.3437566649082,34.1080837663654,
-232.85005));
#203187=CARTESIAN_POINT('Ctrl Pts',(-33.2007785122789,33.4934899779856,
-232.85005));
#203188=CARTESIAN_POINT('Ctrl Pts',(-35.7754719960827,31.5304296840008,
-232.85005));
#203189=CARTESIAN_POINT('Ctrl Pts',(-37.4639373139644,30.0758667472214,
-232.85005));
#203190=CARTESIAN_POINT('Ctrl Pts',(-40.599089476002,27.0270783922592,-232.85005));
#203191=CARTESIAN_POINT('Ctrl Pts',(-42.1044452521513,25.3726646453487,
-232.85005));
#203192=CARTESIAN_POINT('Ctrl Pts',(-44.762707951181,22.0795000960731,-232.85005));
#203193=CARTESIAN_POINT('Ctrl Pts',(-45.9624973465495,20.4083241018545,
-232.85005));
#203194=CARTESIAN_POINT('Ctrl Pts',(-47.0649763530314,18.681697915047,-232.85005));
#203195=CARTESIAN_POINT('Ctrl Pts',(-48.0827620446564,42.0414223951255,
-215.85005));
#203196=CARTESIAN_POINT('Ctrl Pts',(-47.6918902578017,41.9918377458004,
-216.158510565779));
#203197=CARTESIAN_POINT('Ctrl Pts',(-47.3178589835132,41.9044704486574,
-216.48375532529));
#203198=CARTESIAN_POINT('Ctrl Pts',(-46.5278541133197,41.641234161018,-217.23269561852));
#203199=CARTESIAN_POINT('Ctrl Pts',(-46.1204261816762,41.4485202650992,
-217.663837570708));
#203200=CARTESIAN_POINT('Ctrl Pts',(-44.981799852587,40.7494982164702,-219.00027770574));
#203201=CARTESIAN_POINT('Ctrl Pts',(-44.3453100117826,40.1178561866307,
-219.946031814412));
#203202=CARTESIAN_POINT('Ctrl Pts',(-43.3187329856621,38.5182399992048,
-221.95430949443));
#203203=CARTESIAN_POINT('Ctrl Pts',(-43.002470525188,37.5284133107564,-222.985431129024));
#203204=CARTESIAN_POINT('Ctrl Pts',(-42.9307447595933,36.1378442916941,
-224.156404719787));
#203205=CARTESIAN_POINT('Ctrl Pts',(-42.9463038154314,35.7490409900809,
-224.457196959813));
#203206=CARTESIAN_POINT('Ctrl Pts',(-43.0642975219893,34.9494394058048,
-225.008393072148));
#203207=CARTESIAN_POINT('Ctrl Pts',(-43.1679394115819,34.535481911261,-225.260388542568));
#203208=CARTESIAN_POINT('Ctrl Pts',(-43.3259173910694,34.1204116753623,
-225.468974352254));
#203209=CARTESIAN_POINT('',(-45.7333210472294,31.2122413349066,-225.850044625489));
#203210=CARTESIAN_POINT('Ctrl Pts',(-45.7333215211538,31.2122476871429,
-225.850034142281));
#203211=CARTESIAN_POINT('Ctrl Pts',(-45.3380055594478,31.455444850938,-225.979526553824));
#203212=CARTESIAN_POINT('Ctrl Pts',(-44.9655439649494,31.7492431768137,
-226.049129920994));
#203213=CARTESIAN_POINT('Ctrl Pts',(-44.2903200744336,32.435009374361,-226.04918891067));
#203214=CARTESIAN_POINT('Ctrl Pts',(-44.0029189269882,32.8110299162004,
-225.979864418515));
#203215=CARTESIAN_POINT('Ctrl Pts',(-43.7661192040752,33.2092653547038,
-225.850049930202));
#203216=CARTESIAN_POINT('',(-46.4511396589728,30.4281656954993,-225.850049999692));
#203217=CARTESIAN_POINT('Ctrl Pts',(-46.4511396584396,30.4281656950206,
-225.85005));
#203218=CARTESIAN_POINT('Ctrl Pts',(-46.3327936013924,30.5600059653032,
-225.85005));
#203219=CARTESIAN_POINT('Ctrl Pts',(-46.2137942836441,30.6912801190928,
-225.85005));
#203220=CARTESIAN_POINT('Ctrl Pts',(-45.9745262548726,30.952635522043,-225.85005));
#203221=CARTESIAN_POINT('Ctrl Pts',(-45.8542372577667,31.0827388238805,
-225.85005));
#203222=CARTESIAN_POINT('Ctrl Pts',(-45.7333160870584,31.2122314463161,
-225.85005));
#203223=CARTESIAN_POINT('Ctrl Pts',(-46.4511396588545,30.4281656952996,
-225.850049999479));
#203224=CARTESIAN_POINT('Ctrl Pts',(-46.49937538757,30.476563209559,-225.778199404494));
#203225=CARTESIAN_POINT('Ctrl Pts',(-46.5476099273389,30.5249595308839,
-225.706349253907));
#203226=CARTESIAN_POINT('Ctrl Pts',(-46.6440796086263,30.6217527773017,
-225.562645429306));
#203227=CARTESIAN_POINT('Ctrl Pts',(-46.6923132700127,30.670148217298,-225.490793960134));
#203228=CARTESIAN_POINT('Ctrl Pts',(-46.7405472321751,30.7185439590791,
-225.418940742802));
#203229=CARTESIAN_POINT('Origin',(0.,-12.9675000200281,-215.85005));
#203230=CARTESIAN_POINT('',(-48.069978588367,-67.6025450148014,-215.850048907738));
#203231=CARTESIAN_POINT('Ctrl Pts',(-48.0699790801226,-67.6025411545956,
-215.85005));
#203232=CARTESIAN_POINT('Ctrl Pts',(-48.2216024642868,-67.4737675776872,
-215.85005));
#203233=CARTESIAN_POINT('Ctrl Pts',(-48.37313230858,-67.3439224269873,-215.850050000034));
#203234=CARTESIAN_POINT('Ctrl Pts',(-48.672769750555,-67.0849704871732,
-215.850050000034));
#203235=CARTESIAN_POINT('Ctrl Pts',(-48.8224593013279,-66.9544830612177,
-215.85005));
#203236=CARTESIAN_POINT('Ctrl Pts',(-48.9715866554311,-66.8233021636441,
-215.85005));
#203237=CARTESIAN_POINT('',(-53.9390346875574,-61.9113848028034,-215.85005));
#203238=CARTESIAN_POINT('Origin',(-48.1334350484927,-61.7961505568785,-215.85005));
#203239=CARTESIAN_POINT('Ctrl Pts',(-53.7300151844416,-62.1425230012532,
-215.85005));
#203240=CARTESIAN_POINT('Ctrl Pts',(-53.7649393991568,-62.1040873964405,
-215.85005));
#203241=CARTESIAN_POINT('Ctrl Pts',(-53.799816986159,-62.0656105112331,
-215.85005));
#203242=CARTESIAN_POINT('Ctrl Pts',(-53.8694902457089,-61.9885636960974,
-215.85005));
#203243=CARTESIAN_POINT('Ctrl Pts',(-53.9042848508542,-61.9499949024127,
-215.85005));
#203244=CARTESIAN_POINT('Ctrl Pts',(-53.9390346875574,-61.9113848028034,
-215.85005));
#203245=CARTESIAN_POINT('Ctrl Pts',(-46.9944270680642,-41.6193123752663,
-233.004519986905));
#203246=CARTESIAN_POINT('Ctrl Pts',(-48.7878616654988,-44.7175816808496,
-229.860902939557));
#203247=CARTESIAN_POINT('Ctrl Pts',(-50.5840414119712,-47.8137084153908,
-226.716710153573));
#203248=CARTESIAN_POINT('Ctrl Pts',(-52.3845374377678,-50.9067036630134,
-223.571849766529));
#203249=CARTESIAN_POINT('Ctrl Pts',(-54.1850334635645,-53.999698910636,
-220.426989379484));
#203250=CARTESIAN_POINT('Ctrl Pts',(-55.9897753069174,-57.0895865666151,
-217.281445207064));
#203251=CARTESIAN_POINT('Ctrl Pts',(-57.8017289442242,-60.1747340778167,
-214.135276372889));
#203252=CARTESIAN_POINT('Ctrl Pts',(-46.9566286849537,-41.6781739629451,
-233.004786483119));
#203253=CARTESIAN_POINT('Ctrl Pts',(-48.7510652266437,-44.7730579825931,
-229.861179418927));
#203254=CARTESIAN_POINT('Ctrl Pts',(-50.5482471004081,-47.8657963569279,
-226.716997721658));
#203255=CARTESIAN_POINT('Ctrl Pts',(-52.3497454436632,-50.9553990731154,
-223.572150029539));
#203256=CARTESIAN_POINT('Ctrl Pts',(-54.1512437869183,-54.045001789303,
-220.427302337419));
#203257=CARTESIAN_POINT('Ctrl Pts',(-55.9569880950718,-57.1314927928873,
-217.28177244287));
#203258=CARTESIAN_POINT('Ctrl Pts',(-57.7699448315789,-60.2132374154909,
-214.135620383829));
#203259=CARTESIAN_POINT('Ctrl Pts',(-46.9219121704599,-41.7340896317106,
-233.003924127997));
#203260=CARTESIAN_POINT('Ctrl Pts',(-48.7170243830511,-44.8259324838809,
-229.860501038468));
#203261=CARTESIAN_POINT('Ctrl Pts',(-50.5148833131725,-47.9156143059604,
-226.716492970748));
#203262=CARTESIAN_POINT('Ctrl Pts',(-52.3171186451179,-51.0020915740055,
-223.571790312035));
#203263=CARTESIAN_POINT('Ctrl Pts',(-54.1193539770633,-54.0885688420506,
-220.427087653323));
#203264=CARTESIAN_POINT('Ctrl Pts',(-55.9258862266926,-57.1718702110663,
-217.28167372519));
#203265=CARTESIAN_POINT('Ctrl Pts',(-57.7398613178177,-60.2502287004015,
-214.1355819053));
#203266=CARTESIAN_POINT('Ctrl Pts',(-46.8853928444761,-41.791544195152,
-233.003625168491));
#203267=CARTESIAN_POINT('Ctrl Pts',(-48.681427442577,-44.8800992987762,
-229.860296540463));
#203268=CARTESIAN_POINT('Ctrl Pts',(-50.4802079998591,-47.9664858608819,
-226.716379335157));
#203269=CARTESIAN_POINT('Ctrl Pts',(-52.2833924017896,-51.0496336439922,
-223.57175528194));
#203270=CARTESIAN_POINT('Ctrl Pts',(-54.0865768037201,-54.1327814271025,
-220.427131228723));
#203271=CARTESIAN_POINT('Ctrl Pts',(-55.8940807177617,-57.2127217368356,
-217.281783456688));
#203272=CARTESIAN_POINT('Ctrl Pts',(-57.7091409883845,-60.287618730288,
-214.135731970477));
#203273=CARTESIAN_POINT('Ctrl Pts',(-46.8488735184923,-41.8489987585935,
-233.003326208986));
#203274=CARTESIAN_POINT('Ctrl Pts',(-48.645830502103,-44.9342661136713,
-229.860092042457));
#203275=CARTESIAN_POINT('Ctrl Pts',(-50.4455326865456,-48.0173574158033,
-226.716265699565));
#203276=CARTESIAN_POINT('Ctrl Pts',(-52.2496661584613,-51.0971757139789,
-223.571720251843));
#203277=CARTESIAN_POINT('Ctrl Pts',(-54.053799630377,-54.1769940121544,
-220.427174804122));
#203278=CARTESIAN_POINT('Ctrl Pts',(-55.8622752088309,-57.2535732626049,
-217.281893188185));
#203279=CARTESIAN_POINT('Ctrl Pts',(-57.6784206589513,-60.3250087601744,
-214.135882035655));
#203280=CARTESIAN_POINT('Ctrl Pts',(-46.8121794637376,-41.9064965273971,
-233.003026620871));
#203281=CARTESIAN_POINT('Ctrl Pts',(-48.6101143190285,-44.9884269324132,
-229.859885255064));
#203282=CARTESIAN_POINT('Ctrl Pts',(-50.4107926169958,-48.0681748858937,
-226.716148772852));
#203283=CARTESIAN_POINT('Ctrl Pts',(-52.2159279111165,-51.1446171397359,
-223.571681746167));
#203284=CARTESIAN_POINT('Ctrl Pts',(-54.0210632052373,-54.221059393578,
-220.427214719482));
#203285=CARTESIAN_POINT('Ctrl Pts',(-55.8305612422911,-57.2942327369214,
-217.281999929988));
#203286=CARTESIAN_POINT('Ctrl Pts',(-57.6478412701604,-60.3621625545191,
-214.136030325987));
#203287=CARTESIAN_POINT('Ctrl Pts',(-46.7753102520778,-41.9640352485997,
-233.002726574857));
#203288=CARTESIAN_POINT('Ctrl Pts',(-48.5742777683907,-45.0425809377688,
-229.859676400769));
#203289=CARTESIAN_POINT('Ctrl Pts',(-50.3759860497308,-48.1189387987811,
-226.716028769071));
#203290=CARTESIAN_POINT('Ctrl Pts',(-52.1821753368859,-51.191959764097,
-223.571639944857));
#203291=CARTESIAN_POINT('Ctrl Pts',(-53.9883646240409,-54.264980729413,
-220.427251120643));
#203292=CARTESIAN_POINT('Ctrl Pts',(-55.7989353732621,-57.3347046065519,
-217.282103770803));
#203293=CARTESIAN_POINT('Ctrl Pts',(-57.6173986625019,-60.3990859831037,
-214.136176919604));
#203294=CARTESIAN_POINT('Ctrl Pts',(-46.7015718287581,-42.0791126910049,
-233.00212648283));
#203295=CARTESIAN_POINT('Ctrl Pts',(-48.5026046671152,-45.1508889484801,
-229.859258692179));
#203296=CARTESIAN_POINT('Ctrl Pts',(-50.3063729152009,-48.2204666245557,
-226.715788761507));
#203297=CARTESIAN_POINT('Ctrl Pts',(-52.1146701884246,-51.2866450128194,
-223.571556342237));
#203298=CARTESIAN_POINT('Ctrl Pts',(-53.9229674616482,-54.3528234010831,
-220.427323922968));
#203299=CARTESIAN_POINT('Ctrl Pts',(-55.7356836352042,-57.4156483458129,
-217.282311452432));
#203300=CARTESIAN_POINT('Ctrl Pts',(-57.5565134471849,-60.4729328402728,
-214.136470106837));
#203301=CARTESIAN_POINT('Ctrl Pts',(-46.6271327739678,-42.1943539415595,
-233.001524562797));
#203302=CARTESIAN_POINT('Ctrl Pts',(-48.4304500911505,-45.2591697072969,
-229.858832720452));
#203303=CARTESIAN_POINT('Ctrl Pts',(-50.2364937898458,-48.3217802201232,
-226.715536447315));
#203304=CARTESIAN_POINT('Ctrl Pts',(-52.0471077366989,-51.3809350513845,
-223.571459556911));
#203305=CARTESIAN_POINT('Ctrl Pts',(-53.857721683552,-54.4400898826458,
-220.427382666507));
#203306=CARTESIAN_POINT('Ctrl Pts',(-55.672784296813,-57.4958416576678,
-217.282507528118));
#203307=CARTESIAN_POINT('Ctrl Pts',(-57.4961753701015,-60.5458582201909,
-214.136756507531));
#203308=CARTESIAN_POINT('Ctrl Pts',(-46.5519897086414,-42.3097409936012,
-233.000922137489));
#203309=CARTESIAN_POINT('Ctrl Pts',(-48.3578050935127,-45.3674166545976,
-229.858400212826));
#203310=CARTESIAN_POINT('Ctrl Pts',(-50.166334738395,-48.4228838232303,
-226.715273522923));
#203311=CARTESIAN_POINT('Ctrl Pts',(-51.9794693444289,-51.4748446769843,
-223.571351034937));
#203312=CARTESIAN_POINT('Ctrl Pts',(-53.7926039504629,-54.5268055307383,
-220.427428546952));
#203313=CARTESIAN_POINT('Ctrl Pts',(-55.6102096831407,-57.5753202178,-217.28269273506));
#203314=CARTESIAN_POINT('Ctrl Pts',(-57.4363509894997,-60.6179092484165,
-214.137036747929));
#203315=CARTESIAN_POINT('Ctrl Pts',(-46.4017035779887,-42.5405150976846,
-232.999717286874));
#203316=CARTESIAN_POINT('Ctrl Pts',(-48.2125150982371,-45.5839105491989,
-229.857535197574));
#203317=CARTESIAN_POINT('Ctrl Pts',(-50.0260166354934,-48.6250910294446,
-226.714747674137));
#203318=CARTESIAN_POINT('Ctrl Pts',(-51.844192559889,-51.6626639281839,
-223.571133990991));
#203319=CARTESIAN_POINT('Ctrl Pts',(-53.6623684842846,-54.7002368269232,
-220.427520307844));
#203320=CARTESIAN_POINT('Ctrl Pts',(-55.4850604557961,-57.7342773380644,
-217.283063148945));
#203321=CARTESIAN_POINT('Ctrl Pts',(-57.3167022282962,-60.7620113048676,
-214.137597228726));
#203322=CARTESIAN_POINT('Ctrl Pts',(-46.2486013427642,-42.7718723828066,
-232.998510473058));
#203323=CARTESIAN_POINT('Ctrl Pts',(-48.0652633432344,-45.8002692151702,
-229.856644114599));
#203324=CARTESIAN_POINT('Ctrl Pts',(-49.8845788152544,-48.8264582428966,
-226.714179427834));
#203325=CARTESIAN_POINT('Ctrl Pts',(-51.708612066789,-51.848961452988,-223.570870018747));
#203326=CARTESIAN_POINT('Ctrl Pts',(-53.5326453183235,-54.8714646630795,
-220.427560609659));
#203327=CARTESIAN_POINT('Ctrl Pts',(-55.3612102766787,-57.8903753028513,
-217.283390075808));
#203328=CARTESIAN_POINT('Ctrl Pts',(-57.1991084585358,-60.9026157167782,
-214.13813310078));
#203329=CARTESIAN_POINT('Ctrl Pts',(-46.0926567139982,-43.0036690826345,
-232.997311586148));
#203330=CARTESIAN_POINT('Ctrl Pts',(-47.9159791152656,-46.0164399058077,
-229.855739900183));
#203331=CARTESIAN_POINT('Ctrl Pts',(-49.7419098599322,-49.0270196364001,
-226.713581949947));
#203332=CARTESIAN_POINT('Ctrl Pts',(-51.5725780231494,-52.0338565143131,
-223.570570609253));
#203333=CARTESIAN_POINT('Ctrl Pts',(-53.4032461863666,-55.0406933922261,
-220.427559268559));
#203334=CARTESIAN_POINT('Ctrl Pts',(-55.2384359222485,-58.0439012335412,
-217.283679691665));
#203335=CARTESIAN_POINT('Ctrl Pts',(-57.083299585097,-61.0401022731089,
-214.13864916931));
#203336=CARTESIAN_POINT('Ctrl Pts',(-45.7807674564663,-43.4672624822902,
-232.994913812328));
#203337=CARTESIAN_POINT('Ctrl Pts',(-47.617410659328,-46.4487812870827,
-229.853931471351));
#203338=CARTESIAN_POINT('Ctrl Pts',(-49.4565719492878,-49.4281424234071,
-226.71238699417));
#203339=CARTESIAN_POINT('Ctrl Pts',(-51.3005099358702,-52.4036466369632,
-223.569971790265));
#203340=CARTESIAN_POINT('Ctrl Pts',(-53.1444479224527,-55.3791508505193,
-220.427556586359));
#203341=CARTESIAN_POINT('Ctrl Pts',(-54.992887213388,-58.3509530949211,
-217.284258923378));
#203342=CARTESIAN_POINT('Ctrl Pts',(-56.8516818382195,-61.3150753857701,
-214.139681306367));
#203343=CARTESIAN_POINT('Ctrl Pts',(-45.457507604722,-43.9326130692061,
-232.99254867873));
#203344=CARTESIAN_POINT('Ctrl Pts',(-47.3107111022754,-46.8803707732786,
-229.852071833745));
#203345=CARTESIAN_POINT('Ctrl Pts',(-49.1663089215364,-49.8260415059931,
-226.711076271479));
#203346=CARTESIAN_POINT('Ctrl Pts',(-51.0266279973321,-52.7678256944002,
-223.569232172689));
#203347=CARTESIAN_POINT('Ctrl Pts',(-52.8869470731278,-55.7096098828074,
-220.427388073898));
#203348=CARTESIAN_POINT('Ctrl Pts',(-54.7516438900022,-58.6477142186619,
-217.284689472746));
#203349=CARTESIAN_POINT('Ctrl Pts',(-56.6272059226936,-61.5775733671438,
-214.14063576296));
#203350=CARTESIAN_POINT('Ctrl Pts',(-45.122678945944,-44.3985758751927,
-232.990284156912));
#203351=CARTESIAN_POINT('Ctrl Pts',(-46.9953289795326,-47.3107844763396,
-229.850249364904));
#203352=CARTESIAN_POINT('Ctrl Pts',(-48.8702338796761,-50.2209949619586,
-226.709744329754));
#203353=CARTESIAN_POINT('Ctrl Pts',(-50.7497258393681,-53.1273622037278,
-223.56843670589));
#203354=CARTESIAN_POINT('Ctrl Pts',(-52.62921779906,-56.033729445497,-220.427129082025));
#203355=CARTESIAN_POINT('Ctrl Pts',(-54.5128930537055,-58.9365113017985,
-217.285019110898));
#203356=CARTESIAN_POINT('Ctrl Pts',(-56.4076769323115,-61.8306798185293,
-214.141539423862));
#203357=CARTESIAN_POINT('Ctrl Pts',(-44.4530216283881,-45.330501487166,
-232.985755113274));
#203358=CARTESIAN_POINT('Ctrl Pts',(-46.364564734047,-48.1716118824616,
-229.846604427224));
#203359=CARTESIAN_POINT('Ctrl Pts',(-48.2780837959556,-51.0109018738896,
-226.707080446303));
#203360=CARTESIAN_POINT('Ctrl Pts',(-50.19592152344,-53.846435222383,-223.566845772292));
#203361=CARTESIAN_POINT('Ctrl Pts',(-52.1137592509244,-56.6819685708763,
-220.42661109828));
#203362=CARTESIAN_POINT('Ctrl Pts',(-54.0353913811122,-59.5141054680716,
-217.285678387203));
#203363=CARTESIAN_POINT('Ctrl Pts',(-55.9686189515471,-62.3368927213004,
-214.143346745665));
#203364=CARTESIAN_POINT('Ctrl Pts',(-43.7371085113763,-46.2648305947527,
-232.981637432207));
#203365=CARTESIAN_POINT('Ctrl Pts',(-45.6990794088443,-49.0277012666958,
-229.84312647621));
#203366=CARTESIAN_POINT('Ctrl Pts',(-47.6626881850455,-51.7889977645385,
-226.704357361211));
#203367=CARTESIAN_POINT('Ctrl Pts',(-49.6300299185432,-54.5469161187202,
-223.565063052865));
#203368=CARTESIAN_POINT('Ctrl Pts',(-51.5973716520409,-57.3048344729019,
-220.425768744518));
#203369=CARTESIAN_POINT('Ctrl Pts',(-53.5678464328781,-60.0598292382354,
-217.285973682359));
#203370=CARTESIAN_POINT('Ctrl Pts',(-55.5492457890124,-62.8055814665179,
-214.145012087778));
#203371=CARTESIAN_POINT('Ctrl Pts',(-42.9734424791526,-47.1926155685251,
-232.978313839575));
#203372=CARTESIAN_POINT('Ctrl Pts',(-44.9946071331279,-49.8757842370209,
-229.840273609375));
#203373=CARTESIAN_POINT('Ctrl Pts',(-47.0170439436796,-52.5576635978524,
-226.702063718992));
#203374=CARTESIAN_POINT('Ctrl Pts',(-49.0424058070309,-55.2367916852255,
-223.563495724472));
#203375=CARTESIAN_POINT('Ctrl Pts',(-51.0677676703821,-57.9159197725986,
-220.424927729951));
#203376=CARTESIAN_POINT('Ctrl Pts',(-53.0955326872786,-60.5927163347612,
-217.286025395512));
#203377=CARTESIAN_POINT('Ctrl Pts',(-55.1321416284158,-63.2617424152049,
-214.146274180285));
#203378=CARTESIAN_POINT('Ctrl Pts',(-41.4461104147051,-49.0481855160699,
-232.97166665431));
#203379=CARTESIAN_POINT('Ctrl Pts',(-43.5856625816949,-51.5719501776712,
-229.834567875703));
#203380=CARTESIAN_POINT('Ctrl Pts',(-45.725755460948,-54.09499526448,-226.697476434552));
#203381=CARTESIAN_POINT('Ctrl Pts',(-47.8671575840062,-56.616542818236,
-223.560361067685));
#203382=CARTESIAN_POINT('Ctrl Pts',(-50.0085597070645,-59.138090371992,
-220.423245700818));
#203383=CARTESIAN_POINT('Ctrl Pts',(-52.1509051960796,-61.6584905278127,
-217.286128821816));
#203384=CARTESIAN_POINT('Ctrl Pts',(-54.2979333072227,-64.1740643125789,
-214.148798365297));
#203385=CARTESIAN_POINT('Ctrl Pts',(-39.7224455239868,-50.8825869261812,
-232.968811623327));
#203386=CARTESIAN_POINT('Ctrl Pts',(-42.0166284209611,-53.2398821108309,
-229.831855736726));
#203387=CARTESIAN_POINT('Ctrl Pts',(-44.3107862632822,-55.5969218113776,
-226.694951854308));
#203388=CARTESIAN_POINT('Ctrl Pts',(-46.6046310902244,-57.9539261591375,
-223.55816686563));
#203389=CARTESIAN_POINT('Ctrl Pts',(-48.8984759171666,-60.3109305068973,
-220.421381876952));
#203390=CARTESIAN_POINT('Ctrl Pts',(-51.1921534761245,-62.6678044223395,
-217.284704907766));
#203391=CARTESIAN_POINT('Ctrl Pts',(-53.4842288420267,-65.0255514956176,
-214.148339440146));
#203392=CARTESIAN_POINT('Ctrl Pts',(-37.882123536986,-52.5752193780183,
-232.970806720566));
#203393=CARTESIAN_POINT('Ctrl Pts',(-40.3469003584876,-54.7858287675482,
-229.833381329414));
#203394=CARTESIAN_POINT('Ctrl Pts',(-42.8110087314114,-56.9968033268292,
-226.695906966754));
#203395=CARTESIAN_POINT('Ctrl Pts',(-45.2731441984033,-59.2095312210711,
-223.558332736904));
#203396=CARTESIAN_POINT('Ctrl Pts',(-47.7352796653952,-61.4222591153131,
-220.420758507053));
#203397=CARTESIAN_POINT('Ctrl Pts',(-50.1959790879104,-63.636130388643,
-217.283078469976));
#203398=CARTESIAN_POINT('Ctrl Pts',(-52.6494272678771,-65.857552778289,
-214.145217662806));
#203399=CARTESIAN_POINT('Ctrl Pts',(-36.0418015499852,-54.2678518298554,
-232.972801817804));
#203400=CARTESIAN_POINT('Ctrl Pts',(-38.677172296014,-56.3317754242655,
-229.834906922101));
#203401=CARTESIAN_POINT('Ctrl Pts',(-41.3112311995406,-58.3966848422808,
-226.696862079201));
#203402=CARTESIAN_POINT('Ctrl Pts',(-43.9416573065822,-60.4651362830048,
-223.558498608177));
#203403=CARTESIAN_POINT('Ctrl Pts',(-46.5720834136237,-62.5335877237288,
-220.420135137153));
#203404=CARTESIAN_POINT('Ctrl Pts',(-49.1998046996963,-64.6044563549465,
-217.281452032185));
#203405=CARTESIAN_POINT('Ctrl Pts',(-51.8146256937275,-66.6895540609604,
-214.142095885467));
#203406=CARTESIAN_POINT('Ctrl Pts',(-34.0754426298001,-55.8293718868815,
-232.978994680116));
#203407=CARTESIAN_POINT('Ctrl Pts',(-36.898122716604,-57.765479730986,-229.840093780616));
#203408=CARTESIAN_POINT('Ctrl Pts',(-39.7189124685042,-59.7032049990848,
-226.700797887619));
#203409=CARTESIAN_POINT('Ctrl Pts',(-42.5347347571142,-61.6462105210921,
-223.560608578979));
#203410=CARTESIAN_POINT('Ctrl Pts',(-45.3505570457242,-63.5892160430994,
-220.420419270338));
#203411=CARTESIAN_POINT('Ctrl Pts',(-48.1623968718184,-65.5360552707562,
-217.279358981544));
#203412=CARTESIAN_POINT('Ctrl Pts',(-50.9580697373535,-67.5028226458884,
-214.13623151235));
#203413=CARTESIAN_POINT('Ctrl Pts',(-32.1087006613968,-57.191646012686,
-232.989078118058));
#203414=CARTESIAN_POINT('Ctrl Pts',(-35.1076397475695,-59.0371491145894,
-229.847995786691));
#203415=CARTESIAN_POINT('Ctrl Pts',(-38.1040273439412,-60.8851347665649,
-226.706162642268));
#203416=CARTESIAN_POINT('Ctrl Pts',(-41.0945558666574,-62.7399255565489,
-223.562922655666));
#203417=CARTESIAN_POINT('Ctrl Pts',(-44.0850843893735,-64.5947163465329,
-220.419682669063));
#203418=CARTESIAN_POINT('Ctrl Pts',(-47.0704902905866,-66.4550539448948,
-217.275009748779));
#203419=CARTESIAN_POINT('Ctrl Pts',(-50.0397793224693,-68.3371871397263,
-214.127816818154));
#203420=CARTESIAN_POINT('Ctrl Pts',(-31.1253296771952,-57.8727830755883,
-232.994119837029));
#203421=CARTESIAN_POINT('Ctrl Pts',(-34.2123982630523,-59.6729838063912,
-229.851946789728));
#203422=CARTESIAN_POINT('Ctrl Pts',(-37.2965847816597,-61.4760996503049,
-226.708845019593));
#203423=CARTESIAN_POINT('Ctrl Pts',(-40.374466421429,-63.2867830742773,
-223.564079694009));
#203424=CARTESIAN_POINT('Ctrl Pts',(-43.4523480611983,-65.0974664982497,
-220.419314368426));
#203425=CARTESIAN_POINT('Ctrl Pts',(-46.5245369999706,-66.9145532819642,
-217.272835132396));
#203426=CARTESIAN_POINT('Ctrl Pts',(-49.5806341150271,-68.7543693866452,
-214.123609471056));
#203427=CARTESIAN_POINT('Ctrl Pts',(-30.1402892390281,-58.5059782041702,
-232.999787567079));
#203428=CARTESIAN_POINT('Ctrl Pts',(-33.312862968668,-60.2699670414456,
-229.856286548401));
#203429=CARTESIAN_POINT('Ctrl Pts',(-36.4822633143695,-62.0372971477581,
-226.711666225327));
#203430=CARTESIAN_POINT('Ctrl Pts',(-39.645238310907,-63.8126368978593,
-223.565198694695));
#203431=CARTESIAN_POINT('Ctrl Pts',(-42.8082133074446,-65.5879766479605,
-220.418731164063));
#203432=CARTESIAN_POINT('Ctrl Pts',(-45.9651478987472,-67.3704636405086,
-217.270335425737));
#203433=CARTESIAN_POINT('Ctrl Pts',(-49.1075700836515,-69.1744983835783,
-214.119318043209));
#203434=CARTESIAN_POINT('Ctrl Pts',(-29.1622830188973,-59.093703206177,
-233.005601149464));
#203435=CARTESIAN_POINT('Ctrl Pts',(-32.4119055964007,-60.8333256128672,
-229.860352517102));
#203436=CARTESIAN_POINT('Ctrl Pts',(-35.6582030143032,-62.5766317072687,
-226.713886241748));
#203437=CARTESIAN_POINT('Ctrl Pts',(-38.8983695571512,-64.3279278794606,
-223.565632722533));
#203438=CARTESIAN_POINT('Ctrl Pts',(-42.1385360999994,-66.0792240516524,
-220.417379203317));
#203439=CARTESIAN_POINT('Ctrl Pts',(-45.3727988408086,-67.8379178590787,
-217.267251393612));
#203440=CARTESIAN_POINT('Ctrl Pts',(-48.5947562955792,-69.6157591498535,
-214.114999659484));
#203441=CARTESIAN_POINT('Ctrl Pts',(-28.673279908832,-59.3875657071804,
-233.008507940657));
#203442=CARTESIAN_POINT('Ctrl Pts',(-31.9614269102671,-61.115004898578,
-229.862385501452));
#203443=CARTESIAN_POINT('Ctrl Pts',(-35.2461728642701,-62.846298987024,
-226.714996249958));
#203444=CARTESIAN_POINT('Ctrl Pts',(-38.5249351802734,-64.5855733702612,
-223.565849736452));
#203445=CARTESIAN_POINT('Ctrl Pts',(-41.8036974962768,-66.3248477534984,
-220.416703222945));
#203446=CARTESIAN_POINT('Ctrl Pts',(-45.0766243118393,-68.0716449683638,
-217.26570937755));
#203447=CARTESIAN_POINT('Ctrl Pts',(-48.338349401543,-69.8363895329911,
-214.112840467621));
#203448=CARTESIAN_POINT('Ctrl Pts',(-28.1860374776607,-59.6700652305358,
-233.011446770425));
#203449=CARTESIAN_POINT('Ctrl Pts',(-31.5105936078552,-61.3882833386183,
-229.864343520922));
#203450=CARTESIAN_POINT('Ctrl Pts',(-34.8317102236203,-63.1105042946341,
-226.715949123638));
#203451=CARTESIAN_POINT('Ctrl Pts',(-38.1470954909054,-64.8405791788429,
-223.565888981583));
#203452=CARTESIAN_POINT('Ctrl Pts',(-41.4624807581906,-66.5706540630517,
-220.415828839529));
#203453=CARTESIAN_POINT('Ctrl Pts',(-44.772220394414,-68.3082505831985,
-217.264016183284));
#203454=CARTESIAN_POINT('Ctrl Pts',(-48.0720115712419,-70.062309547184,
-214.110662164981));
#203455=CARTESIAN_POINT('Ctrl Pts',(-27.7016532108346,-59.9415372606891,
-233.014331652954));
#203456=CARTESIAN_POINT('Ctrl Pts',(-31.05976276075,-61.6538447557032,-229.866107695338));
#203457=CARTESIAN_POINT('Ctrl Pts',(-34.4144695478916,-63.3702479288391,
-226.716625256232));
#203458=CARTESIAN_POINT('Ctrl Pts',(-37.7638186351444,-65.0942396965474,
-223.565650201608));
#203459=CARTESIAN_POINT('Ctrl Pts',(-41.1131677223973,-66.8182314642556,
-220.414675146985));
#203460=CARTESIAN_POINT('Ctrl Pts',(-44.4572046958943,-68.5495754713907,
-217.262129974306));
#203461=CARTESIAN_POINT('Ctrl Pts',(-47.7925819070095,-70.295770952258,
-214.1084263508));
#203462=CARTESIAN_POINT('Ctrl Pts',(-27.4594610774215,-60.0772732757658,
-233.015774094218));
#203463=CARTESIAN_POINT('Ctrl Pts',(-30.8343473371973,-61.7866254642456,
-229.866989782546));
#203464=CARTESIAN_POINT('Ctrl Pts',(-34.2058492100272,-63.5001197459416,
-226.716963322528));
#203465=CARTESIAN_POINT('Ctrl Pts',(-37.5721802072639,-65.2210699553996,
-223.565530811621));
#203466=CARTESIAN_POINT('Ctrl Pts',(-40.9385112045005,-66.9420201648576,
-220.414098300713));
#203467=CARTESIAN_POINT('Ctrl Pts',(-44.2996968466345,-68.6702379154868,
-217.261186869816));
#203468=CARTESIAN_POINT('Ctrl Pts',(-47.6528670748933,-70.412501654795,
-214.107308443709));
#203469=CARTESIAN_POINT('Ctrl Pts',(-27.2179835587658,-60.2102526866361,
-233.017202782736));
#203470=CARTESIAN_POINT('Ctrl Pts',(-30.608932448567,-61.9174772218177,
-229.867823057804));
#203471=CARTESIAN_POINT('Ctrl Pts',(-33.9965344785202,-63.628876184999,
-226.717232037632));
#203472=CARTESIAN_POINT('Ctrl Pts',(-37.3791828237546,-65.3475636411034,
-223.565341878319));
#203473=CARTESIAN_POINT('Ctrl Pts',(-40.761831168989,-67.0662510972078,
-220.413451719006));
#203474=CARTESIAN_POINT('Ctrl Pts',(-44.1395366106154,-68.7920796018397,
-217.260195585412));
#203475=CARTESIAN_POINT('Ctrl Pts',(-47.509880204324,-70.5311169985697,
-214.10617593024));
#203476=CARTESIAN_POINT('Ctrl Pts',(-26.9773582084069,-60.3405190002037,
-233.018605415792));
#203477=CARTESIAN_POINT('Ctrl Pts',(-30.383562017878,-62.046487235826,-229.868590727832));
#203478=CARTESIAN_POINT('Ctrl Pts',(-33.786482884195,-63.7566420726074,
-226.717416049128));
#203479=CARTESIAN_POINT('Ctrl Pts',(-37.1846995203357,-65.4738805679581,
-223.56507131637));
#203480=CARTESIAN_POINT('Ctrl Pts',(-40.5829161564765,-67.1911190633088,
-220.412726583613));
#203481=CARTESIAN_POINT('Ctrl Pts',(-43.9764292691396,-68.9153271247727,
-217.259151804163));
#203482=CARTESIAN_POINT('Ctrl Pts',(-47.3632316759027,-70.6518934365393,
-214.105023471352));
#203483=CARTESIAN_POINT('Ctrl Pts',(-26.8570455332274,-60.4056521569874,
-233.019306732319));
#203484=CARTESIAN_POINT('Ctrl Pts',(-30.2708768025335,-62.1109922428301,
-229.868974562847));
#203485=CARTESIAN_POINT('Ctrl Pts',(-33.6814570870323,-63.8205250164116,
-226.717508054876));
#203486=CARTESIAN_POINT('Ctrl Pts',(-37.0874578686263,-65.5370390313854,
-223.564936035396));
#203487=CARTESIAN_POINT('Ctrl Pts',(-40.4934586502203,-67.2535530463592,
-220.412364015916));
#203488=CARTESIAN_POINT('Ctrl Pts',(-43.8948755984016,-68.9769508862391,
-217.258629913538));
#203489=CARTESIAN_POINT('Ctrl Pts',(-47.289907411692,-70.7122816555241,
-214.104447241908));
#203490=CARTESIAN_POINT('Ctrl Pts',(-26.7369459033605,-60.4701070554585,
-233.020001519128));
#203491=CARTESIAN_POINT('Ctrl Pts',(-30.1582026923428,-62.1750368311418,
-229.869341977822));
#203492=CARTESIAN_POINT('Ctrl Pts',(-33.5762470819994,-63.8841603164497,
-226.717578885404));
#203493=CARTESIAN_POINT('Ctrl Pts',(-36.9898447579513,-65.6001532805383,
-223.564780357348));
#203494=CARTESIAN_POINT('Ctrl Pts',(-40.4034424339031,-67.3161462446269,
-220.411981829292));
#203495=CARTESIAN_POINT('Ctrl Pts',(-43.8125851811644,-69.0389260700454,
-217.258094911949));
#203496=CARTESIAN_POINT('Ctrl Pts',(-47.2156677897142,-70.7732100898985,
-214.103866027175));
#203497=CARTESIAN_POINT('Ctrl Pts',(-26.6170765305167,-60.5338892284733,
-233.020688145171));
#203498=CARTESIAN_POINT('Ctrl Pts',(-30.045545113986,-62.238632000908,-229.869690768214));
#203499=CARTESIAN_POINT('Ctrl Pts',(-33.4708476093749,-63.9475635251553,
-226.717626646141));
#203500=CARTESIAN_POINT('Ctrl Pts',(-36.8918444428126,-65.6632431316632,
-223.564602851986));
#203501=CARTESIAN_POINT('Ctrl Pts',(-40.3128412762504,-67.378922738171,
-220.411579057831));
#203502=CARTESIAN_POINT('Ctrl Pts',(-43.7295213469238,-69.1012807810974,
-217.257546349595));
#203503=CARTESIAN_POINT('Ctrl Pts',(-47.140464436521,-70.8347129400802,
-214.103279186265));
#203504=CARTESIAN_POINT('Ctrl Pts',(-26.4972071576729,-60.5976714014882,
-233.021374771214));
#203505=CARTESIAN_POINT('Ctrl Pts',(-29.9328875356291,-62.3022271706743,
-229.870039558606));
#203506=CARTESIAN_POINT('Ctrl Pts',(-33.3654481367504,-64.010966733861,
-226.717674406878));
#203507=CARTESIAN_POINT('Ctrl Pts',(-36.793844127674,-65.7263329827881,
-223.564425346624));
#203508=CARTESIAN_POINT('Ctrl Pts',(-40.2222401185977,-67.4416992317152,
-220.411176286369));
#203509=CARTESIAN_POINT('Ctrl Pts',(-43.6464575126834,-69.1636354921494,
-217.256997787241));
#203510=CARTESIAN_POINT('Ctrl Pts',(-47.0652610833278,-70.8962157902618,
-214.102692345356));
#203511=CARTESIAN_POINT('Ctrl Pts',(-26.3772071408559,-60.6610527709189,
-233.021822686564));
#203512=CARTESIAN_POINT('Ctrl Pts',(-29.8198922647338,-62.3656430824214,
-229.870183157334));
#203513=CARTESIAN_POINT('Ctrl Pts',(-33.2595071470079,-64.0744068681985,
-226.717552132221));
#203514=CARTESIAN_POINT('Ctrl Pts',(-36.6950887844903,-65.7896831337175,
-223.564108323038));
#203515=CARTESIAN_POINT('Ctrl Pts',(-40.1306704219727,-67.5049593992365,
-220.410664513854));
#203516=CARTESIAN_POINT('Ctrl Pts',(-43.5622034605361,-69.2267005231895,
-217.256365654455));
#203517=CARTESIAN_POINT('Ctrl Pts',(-46.9885985225256,-70.9587167786769,
-214.102032318221));
#203518=CARTESIAN_POINT('Ctrl Pts',(-26.2545891898305,-60.7273783411365,
-233.020937743651));
#203519=CARTESIAN_POINT('Ctrl Pts',(-29.704767491125,-62.4315344808983,
-229.869275405273));
#203520=CARTESIAN_POINT('Ctrl Pts',(-33.1518809533354,-64.139871089189,
-226.716620552092));
#203521=CARTESIAN_POINT('Ctrl Pts',(-36.5949698446713,-65.8547248151706,
-223.563151715778));
#203522=CARTESIAN_POINT('Ctrl Pts',(-40.038058736007,-67.5695785411523,
-220.409682879464));
#203523=CARTESIAN_POINT('Ctrl Pts',(-43.4771077064633,-69.2909019608329,
-217.255357871467));
#203524=CARTESIAN_POINT('Ctrl Pts',(-46.911032093483,-71.0224993808136,
-214.10099631368));
#203525=CARTESIAN_POINT('',(-42.5905577899916,-59.5881438265759,-225.000659040692));
#203526=CARTESIAN_POINT('Ctrl Pts',(-48.0699773895611,-67.6025469094357,
-215.850046926336));
#203527=CARTESIAN_POINT('Ctrl Pts',(-47.7935023640231,-67.6024435896897,
-216.017223632964));
#203528=CARTESIAN_POINT('Ctrl Pts',(-47.5226056067636,-67.5828243379733,
-216.193667418601));
#203529=CARTESIAN_POINT('Ctrl Pts',(-46.9774368515139,-67.5066353739982,
-216.5734123135));
#203530=CARTESIAN_POINT('Ctrl Pts',(-46.7040353167265,-67.4475753903814,
-216.777867265658));
#203531=CARTESIAN_POINT('Ctrl Pts',(-45.9194030179567,-67.2207720759118,
-217.40470002861));
#203532=CARTESIAN_POINT('Ctrl Pts',(-45.4358292265386,-67.0029495672062,
-217.845716150046));
#203533=CARTESIAN_POINT('Ctrl Pts',(-44.3014622491111,-66.3069334262107,
-219.018073172344));
#203534=CARTESIAN_POINT('Ctrl Pts',(-43.7134054388051,-65.7467619648911,
-219.774958898609));
#203535=CARTESIAN_POINT('Ctrl Pts',(-42.6715909373129,-64.2628736064779,
-221.493288736712));
#203536=CARTESIAN_POINT('Ctrl Pts',(-42.3167080561632,-63.2947927751177,
-222.434026477107));
#203537=CARTESIAN_POINT('Ctrl Pts',(-42.1771404629454,-61.8708033766699,
-223.580484791686));
#203538=CARTESIAN_POINT('Ctrl Pts',(-42.180006878906,-61.4303388699728,
-223.906345139384));
#203539=CARTESIAN_POINT('Ctrl Pts',(-42.2949054529825,-60.5240489280129,
-224.504112439923));
#203540=CARTESIAN_POINT('Ctrl Pts',(-42.408777306242,-60.0550288947154,
-224.777157735648));
#203541=CARTESIAN_POINT('Ctrl Pts',(-42.5905622784972,-59.5881432109375,
-225.000654103808));
#203542=CARTESIAN_POINT('Ctrl Pts',(-53.9390346875573,-61.9113848028035,
-215.85005));
#203543=CARTESIAN_POINT('Ctrl Pts',(-53.9476622151261,-61.6293619830306,
-216.023587794996));
#203544=CARTESIAN_POINT('Ctrl Pts',(-53.9357969743604,-61.3527628870338,
-216.207117110883));
#203545=CARTESIAN_POINT('Ctrl Pts',(-53.8747173093831,-60.8022834426257,
-216.59757991481));
#203546=CARTESIAN_POINT('Ctrl Pts',(-53.8237963891831,-60.5287413941462,
-216.805449392086));
#203547=CARTESIAN_POINT('Ctrl Pts',(-53.6143973977264,-59.7162941773142,
-217.463133835212));
#203548=CARTESIAN_POINT('Ctrl Pts',(-53.3987000943071,-59.2066382206332,
-217.934268469262));
#203549=CARTESIAN_POINT('Ctrl Pts',(-52.7251467717684,-58.0641624039732,
-219.12859993374));
#203550=CARTESIAN_POINT('Ctrl Pts',(-52.1960061469933,-57.4802041226149,
-219.873917995722));
#203551=CARTESIAN_POINT('Ctrl Pts',(-50.7690642493973,-56.4143480280836,
-221.574539600558));
#203552=CARTESIAN_POINT('Ctrl Pts',(-49.8225109115708,-56.0319094103337,
-222.505508240576));
#203553=CARTESIAN_POINT('Ctrl Pts',(-48.3443436484928,-55.835956780535,
-223.691800920573));
#203554=CARTESIAN_POINT('Ctrl Pts',(-47.8286143703577,-55.8298643113913,
-224.064010045577));
#203555=CARTESIAN_POINT('Ctrl Pts',(-46.8826009388687,-55.9534328528004,
-224.650663983079));
#203556=CARTESIAN_POINT('Ctrl Pts',(-46.4559435829215,-56.0545281652879,
-224.882862691977));
#203557=CARTESIAN_POINT('Ctrl Pts',(-46.030027499011,-56.2113956008523,
-225.073027461904));
#203558=CARTESIAN_POINT('Ctrl Pts',(-41.9650124840222,-58.9506172433346,
-225.850033985948));
#203559=CARTESIAN_POINT('Ctrl Pts',(-42.1763950772714,-59.1660491934041,
-225.5629733364));
#203560=CARTESIAN_POINT('Ctrl Pts',(-42.3849068502055,-59.3785553348708,
-225.279850227117));
#203561=CARTESIAN_POINT('Ctrl Pts',(-42.590551250619,-59.5881391761779,
-225.000663880113));
#203562=CARTESIAN_POINT('Origin',(296.501483394397,-25.4138432731711,-232.85005));
#203563=CARTESIAN_POINT('',(-10.360380424878,38.165365484964,-232.850050038296));
#203564=CARTESIAN_POINT('',(-15.4720288026696,37.8533269327943,-232.85005));
#203565=CARTESIAN_POINT('Origin',(2.61456814389029E-14,-173.57701443073,
-232.85005));
#203566=CARTESIAN_POINT('Ctrl Pts',(-10.3603804210433,38.16536553404,-232.85005));
#203567=CARTESIAN_POINT('Ctrl Pts',(-11.2139414965945,38.2320615098657,
-232.85005));
#203568=CARTESIAN_POINT('Ctrl Pts',(-12.0722256690462,38.2392370527988,
-232.85005));
#203569=CARTESIAN_POINT('Ctrl Pts',(-13.7815229121495,38.1349615420106,
-232.85005));
#203570=CARTESIAN_POINT('Ctrl Pts',(-14.6332355233986,38.0230811620804,
-232.85005));
#203571=CARTESIAN_POINT('Ctrl Pts',(-15.4720288026693,37.853326932793,-232.85005));
#203572=CARTESIAN_POINT('Origin',(296.501483394397,-25.4138432731711,-232.85005));
#203573=CARTESIAN_POINT('Ctrl Pts',(-47.8524635552852,9.39108009191238,
-232.85005));
#203574=CARTESIAN_POINT('Ctrl Pts',(-47.8251207475469,9.27869452829718,
-232.85005));
#203575=CARTESIAN_POINT('Ctrl Pts',(-47.7988578503938,9.16605178669914,
-232.850050000002));
#203576=CARTESIAN_POINT('Ctrl Pts',(-47.7485452399956,8.9404131852861,-232.850050000002));
#203577=CARTESIAN_POINT('Ctrl Pts',(-47.7244950993554,8.82742853781365,
-232.85005));
#203578=CARTESIAN_POINT('Ctrl Pts',(-47.7015450634134,8.71421534318112,
-232.85005));
#203579=CARTESIAN_POINT('',(-23.1986392345853,37.1456077166894,-232.850148165968));
#203580=CARTESIAN_POINT('Origin',(2.61456814389029E-14,-173.57701443073,
-232.85005));
#203581=CARTESIAN_POINT('Ctrl Pts',(-23.1986880090039,37.1456674152139,
-232.85005));
#203582=CARTESIAN_POINT('Ctrl Pts',(-23.3194050754071,37.154620362199,-232.85005));
#203583=CARTESIAN_POINT('Ctrl Pts',(-23.4400518234764,37.164509338947,-232.85005));
#203584=CARTESIAN_POINT('Ctrl Pts',(-23.6811423763216,37.1861531096,-232.85005));
#203585=CARTESIAN_POINT('Ctrl Pts',(-23.8015842986948,37.1979071562942,
-232.85005));
#203586=CARTESIAN_POINT('Ctrl Pts',(-23.9219289938183,37.2105935013701,
-232.85005));
#203587=CARTESIAN_POINT('Origin',(296.501483394397,-25.4138432731711,-232.85005));
#203588=CARTESIAN_POINT('',(-47.8903177140771,0.753846963912779,-232.850053817009));
#203589=CARTESIAN_POINT('',(-47.9312868154534,-1.80167576439668,-232.850051862368));
#203590=CARTESIAN_POINT('Origin',(636.934816028482,-11.5034818258361,-232.85005));
#203591=CARTESIAN_POINT('Ctrl Pts',(-47.8903230579921,0.75384761155794,
-232.85005));
#203592=CARTESIAN_POINT('Ctrl Pts',(-47.9416808738277,0.330078821801721,
-232.85005));
#203593=CARTESIAN_POINT('Ctrl Pts',(-47.9708354565936,-0.095756747675781,
-232.850050000016));
#203594=CARTESIAN_POINT('Ctrl Pts',(-47.9845047846122,-0.949125474243279,
-232.850050000016));
#203595=CARTESIAN_POINT('Ctrl Pts',(-47.9690398565759,-1.37636912129171,
-232.85005));
#203596=CARTESIAN_POINT('Ctrl Pts',(-47.931289209931,-1.80167597693282,
-232.85005));
#203597=CARTESIAN_POINT('Origin',(296.501483394397,-25.4138432731711,-232.85005));
#203598=CARTESIAN_POINT('',(-47.9981322788631,-9.91532742253397,-232.850009339187));
#203599=CARTESIAN_POINT('',(-47.9977289503046,-13.2576712963443,-232.850013209406));
#203600=CARTESIAN_POINT('Origin',(636.934816028482,-11.5034818258361,-232.85005));
#203601=CARTESIAN_POINT('Ctrl Pts',(-47.9981596989451,-9.91572581758163,
-232.85005));
#203602=CARTESIAN_POINT('Ctrl Pts',(-48.0736753643642,-10.4692652745412,
-232.85005));
#203603=CARTESIAN_POINT('Ctrl Pts',(-48.111823774494,-11.0292275871121,
-232.85005));
#203604=CARTESIAN_POINT('Ctrl Pts',(-48.1115279552437,-12.1458824488847,
-232.85005));
#203605=CARTESIAN_POINT('Ctrl Pts',(-48.0732754984808,-12.7047197969431,
-232.85005));
#203606=CARTESIAN_POINT('Ctrl Pts',(-47.9977546165566,-13.2572998177748,
-232.85005));
#203607=CARTESIAN_POINT('Origin',(296.501483394397,-25.4138432731711,-232.85005));
#203608=CARTESIAN_POINT('',(-47.9291893708826,-21.3522304066337,-232.850051757442));
#203609=CARTESIAN_POINT('',(-47.8870567810509,-23.9416215055321,-232.850052596546));
#203610=CARTESIAN_POINT('Origin',(636.934816028482,-11.5034818258361,-232.85005));
#203611=CARTESIAN_POINT('Ctrl Pts',(-47.9291915823105,-21.3522302047528,
-232.85005));
#203612=CARTESIAN_POINT('Ctrl Pts',(-47.9685182384559,-21.783019276162,
-232.85005));
#203613=CARTESIAN_POINT('Ctrl Pts',(-47.9846715385196,-22.2158717780932,
-232.850050000023));
#203614=CARTESIAN_POINT('Ctrl Pts',(-47.9706154668234,-23.0806717086415,
-232.850050000023));
#203615=CARTESIAN_POINT('Ctrl Pts',(-47.9403670434338,-23.5122314437496,
-232.85005));
#203616=CARTESIAN_POINT('Ctrl Pts',(-47.8870605128751,-23.9416219688181,
-232.85005));
#203617=CARTESIAN_POINT('Origin',(296.501483394397,-25.4138432731711,-232.85005));
#203618=CARTESIAN_POINT('',(-10.1856061283707,-61.3499012171703,-232.85005));
#203619=CARTESIAN_POINT('',(-13.6391777675768,-61.2898273935359,-232.85005));
#203620=CARTESIAN_POINT('Ctrl Pts',(-10.1856061283708,-61.3499012171695,
-232.85005));
#203621=CARTESIAN_POINT('Ctrl Pts',(-10.7540331810879,-61.4387873155578,
-232.85005));
#203622=CARTESIAN_POINT('Ctrl Pts',(-11.3321672532956,-61.4795692677295,
-232.85005));
#203623=CARTESIAN_POINT('Ctrl Pts',(-12.4893568184743,-61.4603506900827,
-232.85005));
#203624=CARTESIAN_POINT('Ctrl Pts',(-13.0690230896359,-61.4003891839744,
-232.85005));
#203625=CARTESIAN_POINT('Ctrl Pts',(-13.6391777675768,-61.289827393536,
-232.85005));
#203626=CARTESIAN_POINT('Origin',(-7.14692237356698E-14,623.509175991979,
-232.85005));
#203627=CARTESIAN_POINT('Origin',(-0.128459562639233,-12.6359082483571,
-225.85005));
#203628=CARTESIAN_POINT('',(-46.7347424436738,30.7127197009669,-225.85005));
#203629=CARTESIAN_POINT('Origin',(-48.892180948596,36.2913696007177,-225.85005));
#203630=CARTESIAN_POINT('',(-53.8170476734233,37.8187794096849,-225.85005));
#203631=CARTESIAN_POINT('Origin',(636.934816028482,-11.5034818258361,-234.75005));
#203632=CARTESIAN_POINT('',(-47.9849429580539,-16.0452820755244,-232.250052142049));
#203633=CARTESIAN_POINT('Ctrl Pts',(-47.9849415007718,-16.0452825742631,
-232.250056396759));
#203634=CARTESIAN_POINT('Ctrl Pts',(-47.9880651131553,-15.5742306821108,
-232.306343147704));
#203635=CARTESIAN_POINT('Ctrl Pts',(-47.9906783186251,-15.1065446149179,
-232.390988202572));
#203636=CARTESIAN_POINT('Ctrl Pts',(-47.9942849350928,-14.3203139878749,
-232.579502138114));
#203637=CARTESIAN_POINT('Ctrl Pts',(-47.9949617724383,-14.1407707769958,
-232.636201143858));
#203638=CARTESIAN_POINT('Ctrl Pts',(-47.9965339240235,-13.6931733637722,
-232.756352689979));
#203639=CARTESIAN_POINT('Ctrl Pts',(-47.9971930434488,-13.4765686846904,
-232.80695441365));
#203640=CARTESIAN_POINT('Ctrl Pts',(-47.9977536577298,-13.257674236261,
-232.849976418813));
#203641=CARTESIAN_POINT('',(-47.9866836135147,-7.23226647128753,-232.25005191098));
#203642=CARTESIAN_POINT('Origin',(636.934816028482,-11.5034818258361,-232.25005));
#203643=CARTESIAN_POINT('Ctrl Pts',(-47.9866823371376,-7.23226600773662,
-232.250055704934));
#203644=CARTESIAN_POINT('Ctrl Pts',(-47.9895098141046,-7.68567315063931,
-232.306404893473));
#203645=CARTESIAN_POINT('Ctrl Pts',(-47.9918619737062,-8.13535273752287,
-232.390421945345));
#203646=CARTESIAN_POINT('Ctrl Pts',(-47.9951073324733,-8.89528528197956,
-232.579944924587));
#203647=CARTESIAN_POINT('Ctrl Pts',(-47.9956980243075,-9.06520173831264,
-232.636698278605));
#203648=CARTESIAN_POINT('Ctrl Pts',(-47.9971000734922,-9.4997170477986,
-232.757828881318));
#203649=CARTESIAN_POINT('Ctrl Pts',(-47.9976741114781,-9.70630394983337,
-232.80764645552));
#203650=CARTESIAN_POINT('Ctrl Pts',(-47.9981587676889,-9.91532413904543,
-232.849968678375));
#203651=CARTESIAN_POINT('Origin',(636.934816028482,-11.5034818258361,-234.75005));
#203652=CARTESIAN_POINT('',(-47.8275275119673,3.86645886896237,-232.25005));
#203653=CARTESIAN_POINT('',(-47.9644141218642,-4.51936149851664,-232.250085462751));
#203654=CARTESIAN_POINT('Origin',(636.934816028482,-11.5034818258361,-232.25005));
#203655=CARTESIAN_POINT('Ctrl Pts',(-47.8275275119675,3.86645886896245,
-232.250050000001));
#203656=CARTESIAN_POINT('Ctrl Pts',(-47.8393033810287,3.34181977921662,
-232.308606692494));
#203657=CARTESIAN_POINT('Ctrl Pts',(-47.8504216708136,2.81940125771536,
-232.399682736105));
#203658=CARTESIAN_POINT('Ctrl Pts',(-47.8640428170584,2.14390431815265,
-232.55505864472));
#203659=CARTESIAN_POINT('Ctrl Pts',(-47.8678682595301,1.94983002712662,
-232.604470061216));
#203660=CARTESIAN_POINT('Ctrl Pts',(-47.876573696563,1.50418121394012,-232.71811471315));
#203661=CARTESIAN_POINT('Ctrl Pts',(-47.8835694576846,1.13072531538302,
-232.794863478221));
#203662=CARTESIAN_POINT('Ctrl Pts',(-47.8903149889077,0.753848021453944,
-232.850061370667));
#203663=CARTESIAN_POINT('Ctrl Pts',(-47.9312856139398,-1.8016763710691,
-232.850055542859));
#203664=CARTESIAN_POINT('Ctrl Pts',(-47.9394982187954,-2.38141739948144,
-232.757175193341));
#203665=CARTESIAN_POINT('Ctrl Pts',(-47.9438448367589,-2.72209125824031,
-232.634139478145));
#203666=CARTESIAN_POINT('Ctrl Pts',(-47.954612172792,-3.60581024584066,
-232.397143115374));
#203667=CARTESIAN_POINT('Ctrl Pts',(-47.9597127879937,-4.06055719066972,
-232.308472253544));
#203668=CARTESIAN_POINT('Ctrl Pts',(-47.9643913372016,-4.51935998922945,
-232.250120925502));
#203669=CARTESIAN_POINT('Origin',(636.934816028482,-11.5034818258361,-234.75005));
#203670=CARTESIAN_POINT('',(-47.7599172087244,-29.6370001055566,-232.25005));
#203671=CARTESIAN_POINT('Origin',(636.934816028482,-11.5034818258361,-232.25005));
#203672=CARTESIAN_POINT('Ctrl Pts',(-47.7599172087244,-29.6370001055567,
-232.25005));
#203673=CARTESIAN_POINT('Ctrl Pts',(-47.7492894555136,-30.0382882911887,
-232.296444128103));
#203674=CARTESIAN_POINT('Ctrl Pts',(-47.7383552845378,-30.4376621737927,
-232.368907951216));
#203675=CARTESIAN_POINT('Ctrl Pts',(-47.7170269872741,-31.1933172306936,
-232.569380385358));
#203676=CARTESIAN_POINT('Ctrl Pts',(-47.7066212951508,-31.5515003035446,
-232.693743240766));
#203677=CARTESIAN_POINT('Ctrl Pts',(-47.6963708717086,-31.8956404071764,
-232.849812660495));
#203678=CARTESIAN_POINT('Origin',(636.934816028482,-11.5034818258361,-234.75005));
#203679=CARTESIAN_POINT('',(-47.9620917743623,-18.7116135613516,-232.250083778634));
#203680=CARTESIAN_POINT('',(-47.8203127443142,-27.1915604710334,-232.250049983782));
#203681=CARTESIAN_POINT('Origin',(636.934816028482,-11.5034818258361,-232.25005));
#203682=CARTESIAN_POINT('Ctrl Pts',(-47.9620703904922,-18.7116148410405,
-232.250117557268));
#203683=CARTESIAN_POINT('Ctrl Pts',(-47.9573554138762,-19.1596188938302,
-232.306669892292));
#203684=CARTESIAN_POINT('Ctrl Pts',(-47.952238347251,-19.6037872905696,
-232.393382749887));
#203685=CARTESIAN_POINT('Ctrl Pts',(-47.9411866433023,-20.4904993022867,
-232.635960657362));
#203686=CARTESIAN_POINT('Ctrl Pts',(-47.9372122530391,-20.794255996158,
-232.756243969881));
#203687=CARTESIAN_POINT('Ctrl Pts',(-47.9291882608127,-21.3522298073388,
-232.850055227));
#203688=CARTESIAN_POINT('Ctrl Pts',(-47.8870548777005,-23.9416222224618,
-232.850057734118));
#203689=CARTESIAN_POINT('Ctrl Pts',(-47.8808419217877,-24.283696516233,
-232.800020744851));
#203690=CARTESIAN_POINT('Ctrl Pts',(-47.8744102330401,-24.6236650946472,
-232.733213391971));
#203691=CARTESIAN_POINT('Ctrl Pts',(-47.8666304747006,-25.019568091157,
-232.639069109828));
#203692=CARTESIAN_POINT('Ctrl Pts',(-47.8654339475312,-25.0799470331636,
-232.62410827376));
#203693=CARTESIAN_POINT('Ctrl Pts',(-47.8619240948923,-25.2566749049581,
-232.580479584111));
#203694=CARTESIAN_POINT('Ctrl Pts',(-47.8588236469902,-25.4102068713,-232.54485449108));
#203695=CARTESIAN_POINT('Ctrl Pts',(-47.8446425337259,-26.1008593428905,
-232.395217345888));
#203696=CARTESIAN_POINT('Ctrl Pts',(-47.8328230396433,-26.6455101093022,
-232.305849122883));
#203697=CARTESIAN_POINT('Ctrl Pts',(-47.8203127558795,-27.1915604680009,
-232.250049951514));
#203698=CARTESIAN_POINT('Origin',(-7.14692237356698E-14,623.509175991979,
-234.75005));
#203699=CARTESIAN_POINT('Ctrl Pts',(-13.6391777675768,-61.2898273935359,
-232.85005));
#203700=CARTESIAN_POINT('Ctrl Pts',(-13.7679778538919,-61.2872620754425,
-232.820255967378));
#203701=CARTESIAN_POINT('Ctrl Pts',(-13.8962943913745,-61.2846700045451,
-232.78803439649));
#203702=CARTESIAN_POINT('Ctrl Pts',(-14.0579979559295,-61.2813584495498,
-232.744562636193));
#203703=CARTESIAN_POINT('Ctrl Pts',(-14.0841407462716,-61.2808208278262,
-232.737348171434));
#203704=CARTESIAN_POINT('Ctrl Pts',(-14.1136793535434,-61.280212286192,
-232.729268531082));
#203705=CARTESIAN_POINT('Ctrl Pts',(-14.1196218846364,-61.2800897833729,
-232.727647118086));
#203706=CARTESIAN_POINT('Ctrl Pts',(-14.1382345381682,-61.2797058487589,
-232.722581330731));
#203707=CARTESIAN_POINT('Ctrl Pts',(-14.1509054399916,-61.2794441266336,
-232.719151061211));
#203708=CARTESIAN_POINT('Ctrl Pts',(-14.3680771081964,-61.2749523320009,
-232.660673210664));
#203709=CARTESIAN_POINT('Ctrl Pts',(-14.5738916269567,-61.2706036848072,
-232.610036215289));
#203710=CARTESIAN_POINT('Ctrl Pts',(-15.5130869583053,-61.2503314811182,
-232.401689231682));
#203711=CARTESIAN_POINT('Ctrl Pts',(-16.2652400898949,-61.2328950900326,
-232.297341076771));
#203712=CARTESIAN_POINT('Ctrl Pts',(-17.557415570875,-61.2007887070211,
-232.254652621942));
#203713=CARTESIAN_POINT('Ctrl Pts',(-18.1075672345134,-61.1864563064708,
-232.27870892851));
#203714=CARTESIAN_POINT('Ctrl Pts',(-18.9473592849301,-61.1635855249242,
-232.402122405382));
#203715=CARTESIAN_POINT('Ctrl Pts',(-19.2463100795496,-61.1552436964942,
-232.463744244621));
#203716=CARTESIAN_POINT('Ctrl Pts',(-19.8287142284054,-61.1386226678951,
-232.626250777318));
#203717=CARTESIAN_POINT('Ctrl Pts',(-20.1129420846328,-61.1303255101954,
-232.726867615116));
#203718=CARTESIAN_POINT('Ctrl Pts',(-20.3871350980679,-61.1221605172865,
-232.850025366413));
#203719=CARTESIAN_POINT('',(-8.46314246790651,-61.3733482641917,-232.250044026154));
#203720=CARTESIAN_POINT('Ctrl Pts',(-10.1856061283711,-61.3499012171704,
-232.850049999999));
#203721=CARTESIAN_POINT('Ctrl Pts',(-9.82032687406902,-61.3553338539493,
-232.743373739408));
#203722=CARTESIAN_POINT('Ctrl Pts',(-9.6075193118261,-61.3583117635047,
-232.640308531627));
#203723=CARTESIAN_POINT('Ctrl Pts',(-9.04581817676723,-61.3659623843461,
-232.420098274593));
#203724=CARTESIAN_POINT('Ctrl Pts',(-8.75670787203841,-61.3697245641403,
-232.326864869098));
#203725=CARTESIAN_POINT('Ctrl Pts',(-8.46321410432377,-61.3733513183579,
-232.25005));
#203726=CARTESIAN_POINT('Origin',(-7.14692237356698E-14,623.509175991979,
-232.25005));
#203727=CARTESIAN_POINT('Origin',(-49.9798730220992,-67.1190133783941,-228.35005));
#203728=CARTESIAN_POINT('',(-42.5792116384512,-59.576583500476,-225.85005));
#203729=CARTESIAN_POINT('Origin',(-48.892180948596,36.2913696007177,-218.306418983907));
#203730=CARTESIAN_POINT('',(-46.7347424436738,30.7127197009669,-225.85005));
#203731=CARTESIAN_POINT('Origin',(-53.8170476734233,37.8187794096849,-228.35005));
#203732=CARTESIAN_POINT('Ctrl Pts',(-47.6396641907623,9.56951109638858,
-233.375524009166));
#203733=CARTESIAN_POINT('Ctrl Pts',(-49.8405355389308,11.6556158167396,
-230.003433166063));
#203734=CARTESIAN_POINT('Ctrl Pts',(-52.0418116007037,13.7520462993107,
-226.638133451275));
#203735=CARTESIAN_POINT('Ctrl Pts',(-54.2429855256817,15.8525357612388,
-223.275331821509));
#203736=CARTESIAN_POINT('Ctrl Pts',(-56.4441594506596,17.9530252231669,
-219.912530191744));
#203737=CARTESIAN_POINT('Ctrl Pts',(-58.6452885751193,20.0579121947712,
-216.552478218177));
#203738=CARTESIAN_POINT('Ctrl Pts',(-60.846321628963,22.164968605821,-213.193734192871));
#203739=CARTESIAN_POINT('Ctrl Pts',(-47.1914720210979,7.6140088721643,-233.185323795226));
#203740=CARTESIAN_POINT('Ctrl Pts',(-49.3672203068766,9.52128975296003,
-229.826228944008));
#203741=CARTESIAN_POINT('Ctrl Pts',(-51.5415920964213,11.4345056878504,
-226.469384191172));
#203742=CARTESIAN_POINT('Ctrl Pts',(-53.7154316537813,13.3500108047595,
-223.113404278841));
#203743=CARTESIAN_POINT('Ctrl Pts',(-55.8892712111413,15.2655159216685,
-219.757424366509));
#203744=CARTESIAN_POINT('Ctrl Pts',(-58.0625313135173,17.1835155618891,
-216.402388112408));
#203745=CARTESIAN_POINT('Ctrl Pts',(-60.2355063327765,19.10274141504,-213.047815750158));
#203746=CARTESIAN_POINT('Ctrl Pts',(-47.0946540619524,5.59941768418452,
-233.074415744431));
#203747=CARTESIAN_POINT('Ctrl Pts',(-49.2606104729176,7.3239784675775,-229.720965119143));
#203748=CARTESIAN_POINT('Ctrl Pts',(-51.4258904074922,9.05055026326663,
-226.367922363131));
#203749=CARTESIAN_POINT('Ctrl Pts',(-53.5909200701262,10.7779010963922,
-223.015045172743));
#203750=CARTESIAN_POINT('Ctrl Pts',(-55.7559497327601,12.5052519295177,
-219.662167982355));
#203751=CARTESIAN_POINT('Ctrl Pts',(-57.9207041285279,14.2334502664104,
-216.309468982699));
#203752=CARTESIAN_POINT('Ctrl Pts',(-60.0853267482839,15.9620648827344,
-212.956859706535));
#203753=CARTESIAN_POINT('Ctrl Pts',(-47.3220782931503,3.64213739520988,
-233.009326653747));
#203754=CARTESIAN_POINT('Ctrl Pts',(-49.5001561272747,5.17923014873171,
-229.65822098902));
#203755=CARTESIAN_POINT('Ctrl Pts',(-51.6785800990322,6.71512263630363,
-226.306791304678));
#203756=CARTESIAN_POINT('Ctrl Pts',(-53.8571359353927,8.25054831515734,
-222.955233810924));
#203757=CARTESIAN_POINT('Ctrl Pts',(-56.0356917717532,9.78597399401105,
-219.603676317171));
#203758=CARTESIAN_POINT('Ctrl Pts',(-58.2143916305598,11.3208922926972,
-216.251980359006));
#203759=CARTESIAN_POINT('Ctrl Pts',(-60.3931615898891,12.8555608031383,
-212.900215711346));
#203760=CARTESIAN_POINT('Ctrl Pts',(-47.3789343509497,3.15281732296621,
-232.993054381077));
#203761=CARTESIAN_POINT('Ctrl Pts',(-49.5600425408639,4.64304306902027,
-229.642534956489));
#203762=CARTESIAN_POINT('Ctrl Pts',(-51.7417525219173,6.13126572956288,
-226.291508540064));
#203763=CARTESIAN_POINT('Ctrl Pts',(-53.9236899017093,7.61871011984863,
-222.94028097047));
#203764=CARTESIAN_POINT('Ctrl Pts',(-56.1056272815015,9.10615451013438,
-219.589053400875));
#203765=CARTESIAN_POINT('Ctrl Pts',(-58.2878135060677,10.5927527992689,
-216.237608203082));
#203766=CARTESIAN_POINT('Ctrl Pts',(-60.4701203002903,12.0789347832393,
-212.886054712549));
#203767=CARTESIAN_POINT('Ctrl Pts',(-47.4559590230269,2.66718238323085,
-232.979818118251));
#203768=CARTESIAN_POINT('Ctrl Pts',(-49.6414718351808,4.11022346681344,
-229.629652968461));
#203769=CARTESIAN_POINT('Ctrl Pts',(-51.8278741302197,5.55050627061373,
-226.278876468708));
#203770=CARTESIAN_POINT('Ctrl Pts',(-54.0146079802632,6.98971963348256,
-222.927854342566));
#203771=CARTESIAN_POINT('Ctrl Pts',(-56.2013418303068,8.4289329963514,-219.576832216423));
#203772=CARTESIAN_POINT('Ctrl Pts',(-58.3884396888769,9.86698316181859,
-216.225545116483));
#203773=CARTESIAN_POINT('Ctrl Pts',(-60.5757125562048,11.3044617097837,
-212.874125306097));
#203774=CARTESIAN_POINT('Ctrl Pts',(-47.5526556810106,2.18649568630384,
-232.969248737689));
#203775=CARTESIAN_POINT('Ctrl Pts',(-49.7440252884103,3.58214069800097,
-229.619256142275));
#203776=CARTESIAN_POINT('Ctrl Pts',(-51.9366046755093,4.97428639343047,
-226.268610062602));
#203777=CARTESIAN_POINT('Ctrl Pts',(-54.129628172195,6.36508038888444,-222.917696367826));
#203778=CARTESIAN_POINT('Ctrl Pts',(-56.3226516688807,7.7558743843384,-219.56678267305));
#203779=CARTESIAN_POINT('Ctrl Pts',(-58.5161645712576,9.14519694298261,
-216.215581556974));
#203780=CARTESIAN_POINT('Ctrl Pts',(-60.7099107655409,10.5337979996055,
-212.864235131559));
#203781=CARTESIAN_POINT('Ctrl Pts',(-47.5768298455065,2.06632401207208,
-232.96660639255));
#203782=CARTESIAN_POINT('Ctrl Pts',(-49.7696636517176,3.45012000579785,
-229.616656935729));
#203783=CARTESIAN_POINT('Ctrl Pts',(-51.9637873118318,4.83023142413465,
-226.266043461076));
#203784=CARTESIAN_POINT('Ctrl Pts',(-54.158383220178,6.2089205777349,-222.915156874141));
#203785=CARTESIAN_POINT('Ctrl Pts',(-56.3529791285242,7.58760973133515,
-219.564270287207));
#203786=CARTESIAN_POINT('Ctrl Pts',(-58.5480957918528,8.96475038827362,
-216.213090667097));
#203787=CARTESIAN_POINT('Ctrl Pts',(-60.7434603178749,10.3411320720609,
-212.861762587924));
#203788=CARTESIAN_POINT('Ctrl Pts',(-47.602234241193,1.94646167456563,-232.964131776795));
#203789=CARTESIAN_POINT('Ctrl Pts',(-49.7966228589716,3.3183954301123,-229.614213917398));
#203790=CARTESIAN_POINT('Ctrl Pts',(-51.9923835106293,4.68646023480269,
-226.263625471024));
#203791=CARTESIAN_POINT('Ctrl Pts',(-54.1886450914894,6.05303276847634,
-222.912759842952));
#203792=CARTESIAN_POINT('Ctrl Pts',(-56.3849066723495,7.41960530214998,
-219.561894214879));
#203793=CARTESIAN_POINT('Ctrl Pts',(-58.5817210184137,8.78455283392743,
-216.210731524094));
#203794=CARTESIAN_POINT('Ctrl Pts',(-60.7787980463854,10.1487042615692,
-212.859417974186));
#203795=CARTESIAN_POINT('Ctrl Pts',(-47.628862493758,1.82692857762527,-232.96182118511));
#203796=CARTESIAN_POINT('Ctrl Pts',(-49.8248974717912,3.18698851762863,
-229.611923806209));
#203797=CARTESIAN_POINT('Ctrl Pts',(-52.0223889083793,4.54299549104381,
-226.26135312848));
#203798=CARTESIAN_POINT('Ctrl Pts',(-54.2204105268588,5.89744057105422,
-222.91050257153));
#203799=CARTESIAN_POINT('Ctrl Pts',(-56.4184321453384,7.25188565106463,
-219.559652014579));
#203800=CARTESIAN_POINT('Ctrl Pts',(-58.6170392389817,8.60462958153552,
-216.208501890991));
#203801=CARTESIAN_POINT('Ctrl Pts',(-60.8159240956269,9.95654052871553,
-212.857199226772));
#203802=CARTESIAN_POINT('Ctrl Pts',(-47.6321910253286,1.81198694050772,
-232.961532361149));
#203803=CARTESIAN_POINT('Ctrl Pts',(-49.8284317983937,3.17056265356817,
-229.61163754231));
#203804=CARTESIAN_POINT('Ctrl Pts',(-52.026139583098,4.52506239807395,-226.261069085663));
#203805=CARTESIAN_POINT('Ctrl Pts',(-54.22438120628,5.87799154637645,-222.910220412602));
#203806=CARTESIAN_POINT('Ctrl Pts',(-56.422622829462,7.23092069467897,-219.559371739542));
#203807=CARTESIAN_POINT('Ctrl Pts',(-58.6214540165528,8.58213917498653,
-216.208223186853));
#203808=CARTESIAN_POINT('Ctrl Pts',(-60.8205648517821,9.93252006210882,
-212.856921883345));
#203809=CARTESIAN_POINT('Ctrl Pts',(-47.6355386803079,1.79705044787909,
-232.961246101092));
#203810=CARTESIAN_POINT('Ctrl Pts',(-49.8319866787204,3.15414175308971,
-229.611353668433));
#203811=CARTESIAN_POINT('Ctrl Pts',(-52.0299122769924,4.5071340934001,-226.260787319329));
#203812=CARTESIAN_POINT('Ctrl Pts',(-54.2283753792766,5.85854714070898,
-222.90994043808));
#203813=CARTESIAN_POINT('Ctrl Pts',(-56.4268384815609,7.20996018801785,
-219.55909355683));
#203814=CARTESIAN_POINT('Ctrl Pts',(-58.6258952474512,8.55965305446516,
-216.207946506826));
#203815=CARTESIAN_POINT('Ctrl Pts',(-60.825233550716,9.90850372176869,-212.856646507051));
#203816=CARTESIAN_POINT('Ctrl Pts',(-47.6389054467951,1.78211913870348,
-232.960962398579));
#203817=CARTESIAN_POINT('Ctrl Pts',(-49.8355621025854,3.13772585835723,
-229.611072178893));
#203818=CARTESIAN_POINT('Ctrl Pts',(-52.033706981916,4.48921062136337,-226.260507824327));
#203819=CARTESIAN_POINT('Ctrl Pts',(-54.2323930398121,5.83910740022999,
-222.909662643248));
#203820=CARTESIAN_POINT('Ctrl Pts',(-56.4310790977081,7.18900417909662,
-219.558817462169));
#203821=CARTESIAN_POINT('Ctrl Pts',(-58.6303629299522,8.5371712694402,-216.207671846982));
#203822=CARTESIAN_POINT('Ctrl Pts',(-60.8299301929379,9.88449155844584,
-212.856373094261));
#203823=CARTESIAN_POINT('Ctrl Pts',(-47.6422722132824,1.76718782952786,
-232.960678696067));
#203824=CARTESIAN_POINT('Ctrl Pts',(-49.8391375264504,3.12130996362475,
-229.610790689353));
#203825=CARTESIAN_POINT('Ctrl Pts',(-52.0375016868396,4.47128714932663,
-226.260228329323));
#203826=CARTESIAN_POINT('Ctrl Pts',(-54.2364107003475,5.81966765975101,
-222.909384848415));
#203827=CARTESIAN_POINT('Ctrl Pts',(-56.4353197138554,7.16804817017539,
-219.558541367508));
#203828=CARTESIAN_POINT('Ctrl Pts',(-58.6348306124533,8.51468948441525,
-216.207397187139));
#203829=CARTESIAN_POINT('Ctrl Pts',(-60.8346268351599,9.86047939512299,
-212.856099681471));
#203830=CARTESIAN_POINT('Ctrl Pts',(-47.6439085847953,1.75733843295859,
-232.961288761302));
#203831=CARTESIAN_POINT('Ctrl Pts',(-49.8410717940384,3.10978994722575,
-229.611386840422));
#203832=CARTESIAN_POINT('Ctrl Pts',(-52.0397142106509,4.45813110010028,
-226.26081354148));
#203833=CARTESIAN_POINT('Ctrl Pts',(-54.2388940831247,5.80489015915614,
-222.909960879112));
#203834=CARTESIAN_POINT('Ctrl Pts',(-56.4380739555984,7.151649218212,-219.559108216744));
#203835=CARTESIAN_POINT('Ctrl Pts',(-58.6378476177344,8.49668463701677,
-216.207956614142));
#203836=CARTESIAN_POINT('Ctrl Pts',(-60.8379027023408,9.84087662291507,
-212.856652729236));
#203837=CARTESIAN_POINT('Ctrl Pts',(-47.6460194974834,1.74602297076459,
-232.961641432517));
#203838=CARTESIAN_POINT('Ctrl Pts',(-49.8434528457034,3.09685564489722,
-229.611730184141));
#203839=CARTESIAN_POINT('Ctrl Pts',(-52.042354516691,4.44359608350473,-226.26114964818));
#203840=CARTESIAN_POINT('Ctrl Pts',(-54.2417894607756,5.78876232686925,
-222.91029092321));
#203841=CARTESIAN_POINT('Ctrl Pts',(-56.4412244048602,7.13392857023377,
-219.559432198239));
#203842=CARTESIAN_POINT('Ctrl Pts',(-58.6412485837932,8.47737953915866,
-216.208275719059));
#203843=CARTESIAN_POINT('Ctrl Pts',(-60.8415519676109,9.81999143035988,
-212.856967648949));
#203844=CARTESIAN_POINT('Ctrl Pts',(-47.6502413228594,1.72339204637661,
-232.962346774948));
#203845=CARTESIAN_POINT('Ctrl Pts',(-49.8482149490333,3.07098704024018,
-229.612416871579));
#203846=CARTESIAN_POINT('Ctrl Pts',(-52.0476351287711,4.41452605031363,
-226.261821861581));
#203847=CARTESIAN_POINT('Ctrl Pts',(-54.2475802160774,5.75650666229548,
-222.910951011405));
#203848=CARTESIAN_POINT('Ctrl Pts',(-56.4475253033837,7.09848727427732,
-219.560080161228));
#203849=CARTESIAN_POINT('Ctrl Pts',(-58.6480505159108,8.43876934344246,
-216.208913928891));
#203850=CARTESIAN_POINT('Ctrl Pts',(-60.8488504981511,9.77822104524949,
-212.857597488374));
#203851=CARTESIAN_POINT('Ctrl Pts',(-47.6543975111204,1.70075790412697,
-232.963053249537));
#203852=CARTESIAN_POINT('Ctrl Pts',(-49.8529058064771,3.04510985941153,
-229.613104472738));
#203853=CARTESIAN_POINT('Ctrl Pts',(-52.0528389954907,4.38544246561079,
-226.262494888344));
#203854=CARTESIAN_POINT('Ctrl Pts',(-54.2532887985736,5.72423254074652,
-222.911611841699));
#203855=CARTESIAN_POINT('Ctrl Pts',(-56.4537386016565,7.06302261588225,
-219.560728795054));
#203856=CARTESIAN_POINT('Ctrl Pts',(-58.6547594906971,8.4001309754133,-216.209552773761));
#203857=CARTESIAN_POINT('Ctrl Pts',(-60.8560507563961,9.73641770115673,
-212.858227938596));
#203858=CARTESIAN_POINT('Ctrl Pts',(-47.6584881964675,1.67812063274807,
-232.963760828248));
#203859=CARTESIAN_POINT('Ctrl Pts',(-49.8575254560703,3.01922438781437,
-229.613792971254));
#203860=CARTESIAN_POINT('Ctrl Pts',(-52.0579660735326,4.35634578681776,
-226.263168720394));
#203861=CARTESIAN_POINT('Ctrl Pts',(-54.2589150870478,5.6919405831028,-222.912273412552));
#203862=CARTESIAN_POINT('Ctrl Pts',(-56.459864100563,7.02753537938784,-219.56137810471));
#203863=CARTESIAN_POINT('Ctrl Pts',(-58.6613752354701,8.36146537341484,
-216.210192263444));
#203864=CARTESIAN_POINT('Ctrl Pts',(-60.8631523975563,9.69458248633691,
-212.858859013292));
#203865=CARTESIAN_POINT('Ctrl Pts',(-47.6666695671617,1.63284608999026,
-232.96517598567));
#203866=CARTESIAN_POINT('Ctrl Pts',(-49.8667647552568,2.96745344462007,
-229.615169968288));
#203867=CARTESIAN_POINT('Ctrl Pts',(-52.0682202296165,4.29815242923168,
-226.264516384494));
#203868=CARTESIAN_POINT('Ctrl Pts',(-54.2701676639963,5.62735666781534,
-222.913596554258));
#203869=CARTESIAN_POINT('Ctrl Pts',(-56.4721150983761,6.956560906399,-219.562676724022));
#203870=CARTESIAN_POINT('Ctrl Pts',(-58.6746067250159,8.28413416941793,
-216.211471242811));
#203871=CARTESIAN_POINT('Ctrl Pts',(-60.8773556798765,9.61091205669726,
-212.860121162684));
#203872=CARTESIAN_POINT('Ctrl Pts',(-47.6745889282634,1.58755903151136,
-232.966595558784));
#203873=CARTESIAN_POINT('Ctrl Pts',(-49.8757192238467,2.91564933843912,
-229.616550553645));
#203874=CARTESIAN_POINT('Ctrl Pts',(-52.0781672310342,4.23990669526066,
-226.265867268572));
#203875=CARTESIAN_POINT('Ctrl Pts',(-54.281091064319,5.56270140804211,-222.914922656992));
#203876=CARTESIAN_POINT('Ctrl Pts',(-56.4840148976038,6.88549612082355,
-219.563978045413));
#203877=CARTESIAN_POINT('Ctrl Pts',(-58.6874652929996,8.20669402936436,
-216.212752800202));
#203878=CARTESIAN_POINT('Ctrl Pts',(-60.891164492042,9.52711414398385,-212.861385808758));
#203879=CARTESIAN_POINT('Ctrl Pts',(-47.6822473288034,1.54226015711989,
-232.968019332623));
#203880=CARTESIAN_POINT('Ctrl Pts',(-49.8843891563535,2.86381435135825,
-229.6179346096));
#203881=CARTESIAN_POINT('Ctrl Pts',(-52.0878067306158,4.18161224455118,
-226.267221321995));
#203882=CARTESIAN_POINT('Ctrl Pts',(-54.2916843246343,5.49797977211644,
-222.916251722872));
#203883=CARTESIAN_POINT('Ctrl Pts',(-56.4955619186529,6.81434729968171,
-219.565282123748));
#203884=CARTESIAN_POINT('Ctrl Pts',(-58.6999487759841,8.12915246217079,
-216.214037028638));
#203885=CARTESIAN_POINT('Ctrl Pts',(-60.9045760974657,9.44319745618915,
-212.862653075561));
#203886=CARTESIAN_POINT('Ctrl Pts',(-47.7128809309633,1.36106465955398,
-232.973714427979));
#203887=CARTESIAN_POINT('Ctrl Pts',(-49.9190688863809,2.65647440303478,
-229.623470833417));
#203888=CARTESIAN_POINT('Ctrl Pts',(-52.1263647289421,3.94843444171322,
-226.272637535688));
#203889=CARTESIAN_POINT('Ctrl Pts',(-54.3340573658958,5.23909322841377,
-222.921567986388));
#203890=CARTESIAN_POINT('Ctrl Pts',(-56.5417500028495,6.52975201511432,
-219.570498437088));
#203891=CARTESIAN_POINT('Ctrl Pts',(-58.7498827079224,7.81898619339649,
-216.219173942379));
#203892=CARTESIAN_POINT('Ctrl Pts',(-60.9582225191604,9.10753070501037,
-212.867722142776));
#203893=CARTESIAN_POINT('Ctrl Pts',(-47.7393398420482,1.17968029636359,
-232.979476459983));
#203894=CARTESIAN_POINT('Ctrl Pts',(-49.9491962843832,2.44864037742646,
-229.629062225071));
#203895=CARTESIAN_POINT('Ctrl Pts',(-52.1600026985195,3.71447716168251,
-226.278104081914));
#203896=CARTESIAN_POINT('Ctrl Pts',(-54.3711479805289,4.97914463445542,
-222.926931273635));
#203897=CARTESIAN_POINT('Ctrl Pts',(-56.5822932625382,6.24381210722835,
-219.575758465357));
#203898=CARTESIAN_POINT('Ctrl Pts',(-58.7938147846409,7.50719703392768,
-216.224353199397));
#203899=CARTESIAN_POINT('Ctrl Pts',(-61.0055130419957,8.76996349473516,
-212.872832752187));
#203900=CARTESIAN_POINT('Ctrl Pts',(-47.7616858294571,0.998150138415235,
-232.985293804272));
#203901=CARTESIAN_POINT('Ctrl Pts',(-49.9747881970607,2.24045815861694,
-229.634704119062));
#203902=CARTESIAN_POINT('Ctrl Pts',(-52.1886983731474,3.47997469249725,
-226.283620725365));
#203903=CARTESIAN_POINT('Ctrl Pts',(-54.4028959591866,4.71845222593428,
-222.932344808848));
#203904=CARTESIAN_POINT('Ctrl Pts',(-56.6170935452258,5.95692975937132,
-219.581068892331));
#203905=CARTESIAN_POINT('Ctrl Pts',(-58.8316104681301,7.19426601066472,
-216.229583902017));
#203906=CARTESIAN_POINT('Ctrl Pts',(-61.046277219474,8.43105358570855,-212.877995957148));
#203907=CARTESIAN_POINT('Ctrl Pts',(-47.8510697790929,0.272029506621824,
-233.008563181426));
#203908=CARTESIAN_POINT('Ctrl Pts',(-50.0771558477705,1.40772928337885,
-229.657271695028));
#203909=CARTESIAN_POINT('Ctrl Pts',(-52.3034810716587,2.54196481575621,
-226.305687299172));
#203910=CARTESIAN_POINT('Ctrl Pts',(-54.5298878738176,3.67568259184972,
-222.953998949698));
#203911=CARTESIAN_POINT('Ctrl Pts',(-56.7562946759763,4.80940036794322,
-219.602310600225));
#203912=CARTESIAN_POINT('Ctrl Pts',(-58.9827932020866,5.94254191761289,
-216.250506712501));
#203913=CARTESIAN_POINT('Ctrl Pts',(-61.2093339293867,7.07541394960212,
-212.898648776991));
#203914=CARTESIAN_POINT('Ctrl Pts',(-47.8748620676848,-0.456315238952961,
-233.032739707064));
#203915=CARTESIAN_POINT('Ctrl Pts',(-50.106976448607,0.569429995731811,
-229.68067062904));
#203916=CARTESIAN_POINT('Ctrl Pts',(-52.3389983552511,1.59514136085191,
-226.328577629014));
#203917=CARTESIAN_POINT('Ctrl Pts',(-54.5709908267102,2.62083609058904,
-222.976477458797));
#203918=CARTESIAN_POINT('Ctrl Pts',(-56.8029832981692,3.64653082032617,
-219.624377288579));
#203919=CARTESIAN_POINT('Ctrl Pts',(-59.0349420500259,4.672208415501,-216.272268764454));
#203920=CARTESIAN_POINT('Ctrl Pts',(-61.2668859324121,5.69787672746903,
-212.920156700729));
#203921=CARTESIAN_POINT('Ctrl Pts',(-47.8343566648447,-1.18129562201859,
-233.057735449668));
#203922=CARTESIAN_POINT('Ctrl Pts',(-50.0649792011103,-0.264693413707682,
-229.704700485746));
#203923=CARTESIAN_POINT('Ctrl Pts',(-52.2954559925465,0.653414022650932,
-226.351982116141));
#203924=CARTESIAN_POINT('Ctrl Pts',(-54.525876562459,1.57206651464896,-222.999376095285));
#203925=CARTESIAN_POINT('Ctrl Pts',(-56.7562971323714,2.49071900664698,
-219.646770074429));
#203926=CARTESIAN_POINT('Ctrl Pts',(-58.9866565003629,3.40997442959623,
-216.294288989989));
#203927=CARTESIAN_POINT('Ctrl Pts',(-61.2169859241647,4.32951560431301,
-212.941866493395));
#203928=CARTESIAN_POINT('Ctrl Pts',(-47.8141039634246,-1.54378581355141,
-233.070233320969));
#203929=CARTESIAN_POINT('Ctrl Pts',(-50.043980577362,-0.681755118427429,
-229.716715414099));
#203930=CARTESIAN_POINT('Ctrl Pts',(-52.2736848111942,0.182550353550442,
-226.363684359704));
#203931=CARTESIAN_POINT('Ctrl Pts',(-54.5033194303334,1.04768172667892,
-223.010825413529));
#203932=CARTESIAN_POINT('Ctrl Pts',(-56.7329540494726,1.91281309980739,
-219.657966467354));
#203933=CARTESIAN_POINT('Ctrl Pts',(-58.9625137255313,2.77885743664385,
-216.305299102755));
#203934=CARTESIAN_POINT('Ctrl Pts',(-61.192035920041,3.64533504273501,-212.952721389729));
#203935=CARTESIAN_POINT('Ctrl Pts',(-47.777753685031,-1.90560042502214,
-233.082905053984));
#203936=CARTESIAN_POINT('Ctrl Pts',(-50.0050281763432,-1.0977804796852,
-229.72888694318));
#203937=CARTESIAN_POINT('Ctrl Pts',(-52.2321769379993,-0.286940211741083,
-226.375533132468));
#203938=CARTESIAN_POINT('Ctrl Pts',(-54.4592660843647,0.525003723543879,
-223.022413310737));
#203939=CARTESIAN_POINT('Ctrl Pts',(-56.6863552307302,1.33694765882884,
-219.669293489006));
#203940=CARTESIAN_POINT('Ctrl Pts',(-58.9133824694609,2.15010954210964,
-216.316434370579));
#203941=CARTESIAN_POINT('Ctrl Pts',(-61.140376519071,2.96385127852703,-212.963696992235));
#203942=CARTESIAN_POINT('Ctrl Pts',(-47.725208148176,-2.26586793370592,
-233.095797498554));
#203943=CARTESIAN_POINT('Ctrl Pts',(-49.9481820104395,-1.51156427070571,
-229.741201508812));
#203944=CARTESIAN_POINT('Ctrl Pts',(-52.171153048358,-0.753464571140378,
-226.387470648604));
#203945=CARTESIAN_POINT('Ctrl Pts',(-54.3941000891112,0.00604443117689846,
-223.034045756));
#203946=CARTESIAN_POINT('Ctrl Pts',(-56.6170471298644,0.765553433494175,
-219.680620863394));
#203947=CARTESIAN_POINT('Ctrl Pts',(-58.8399741136204,1.52661141375358,
-216.32753645248));
#203948=CARTESIAN_POINT('Ctrl Pts',(-61.0628850955307,2.28841296751785,
-212.974611260487));
#203949=CARTESIAN_POINT('Ctrl Pts',(-47.6989353797486,-2.4460016880478,
-233.102243720839));
#203950=CARTESIAN_POINT('Ctrl Pts',(-49.9197589274877,-1.71845616621595,
-229.747358791629));
#203951=CARTESIAN_POINT('Ctrl Pts',(-52.1406411035373,-0.986726750840026,
-226.393439406672));
#203952=CARTESIAN_POINT('Ctrl Pts',(-54.3615170914844,-0.253435215006592,
-223.039861978631));
#203953=CARTESIAN_POINT('Ctrl Pts',(-56.5823930794315,0.479856320826842,
-219.686284550589));
#203954=CARTESIAN_POINT('Ctrl Pts',(-58.8032699357002,1.21486234957556,
-216.333087493431));
#203955=CARTESIAN_POINT('Ctrl Pts',(-61.0241393837606,1.95069381201327,
-212.980068394613));
#203956=CARTESIAN_POINT('Ctrl Pts',(-47.6686102280658,-2.62577030498296,
-233.108739309799));
#203957=CARTESIAN_POINT('Ctrl Pts',(-49.8868622268275,-1.92479179417762,
-229.753549805137));
#203958=CARTESIAN_POINT('Ctrl Pts',(-52.1052541434417,-1.21924080077849,
-226.399430730627));
#203959=CARTESIAN_POINT('Ctrl Pts',(-54.3236644404932,-0.511970286406943,
-223.045691665041));
#203960=CARTESIAN_POINT('Ctrl Pts',(-56.5420747375447,0.195300227964602,
-219.691952599455));
#203961=CARTESIAN_POINT('Ctrl Pts',(-58.7605144009039,0.904454604383199,
-216.338635936458));
#203962=CARTESIAN_POINT('Ctrl Pts',(-60.9789586636595,1.61451932982577,
-212.985517079921));
#203963=CARTESIAN_POINT('Ctrl Pts',(-47.6342055660403,-2.80514285302076,
-233.11527543729));
#203964=CARTESIAN_POINT('Ctrl Pts',(-49.8494963118054,-2.13043323572804,
-229.759772872591));
#203965=CARTESIAN_POINT('Ctrl Pts',(-52.0650271669924,-1.4507786685942,
-226.405446498001));
#203966=CARTESIAN_POINT('Ctrl Pts',(-54.2806082192958,-0.769247485060314,
-223.051539438634));
#203967=CARTESIAN_POINT('Ctrl Pts',(-56.4961892715991,-0.0877163015264225,
-219.697632379269));
#203968=CARTESIAN_POINT('Ctrl Pts',(-58.7118360495897,0.595866264290071,
-216.344190859432));
#203969=CARTESIAN_POINT('Ctrl Pts',(-60.9275031739158,1.28044489740776,
-212.990967740646));
#203970=CARTESIAN_POINT('Ctrl Pts',(-47.6299049832871,-2.82756442152549,
-233.116092453226));
#203971=CARTESIAN_POINT('Ctrl Pts',(-49.8448255724277,-2.15613841592184,
-229.760550756022));
#203972=CARTESIAN_POINT('Ctrl Pts',(-52.0599987949363,-1.47972090207117,
-226.406198468922));
#203973=CARTESIAN_POINT('Ctrl Pts',(-54.2752261916461,-0.801407134891986,
-223.052270410334));
#203974=CARTESIAN_POINT('Ctrl Pts',(-56.4904535883559,-0.123093367712802,
-219.698342351745));
#203975=CARTESIAN_POINT('Ctrl Pts',(-58.7057512556755,0.557292721778429,
-216.344885224803));
#203976=CARTESIAN_POINT('Ctrl Pts',(-60.9210712376979,1.23868559335551,
-212.991649073236));
#203977=CARTESIAN_POINT('Ctrl Pts',(-47.6255406457911,-2.84997980588785,
-233.116910107551));
#203978=CARTESIAN_POINT('Ctrl Pts',(-49.8400849976146,-2.18183275209659,
-229.761329146599));
#203979=CARTESIAN_POINT('Ctrl Pts',(-52.0548947978176,-1.50864788311527,
-226.406950828634));
#203980=CARTESIAN_POINT('Ctrl Pts',(-54.2697628615623,-0.83354712920943,
-223.053001671879));
#203981=CARTESIAN_POINT('Ctrl Pts',(-56.4846309253071,-0.158446375303592,
-219.699052515123));
#203982=CARTESIAN_POINT('Ctrl Pts',(-58.699573926166,0.518747611680667,
-216.345579699174));
#203983=CARTESIAN_POINT('Ctrl Pts',(-60.9145412680937,1.1969591078103,-212.992330444524));
#203984=CARTESIAN_POINT('Ctrl Pts',(-47.6211124898449,-2.8723889492326,
-233.117728387381));
#203985=CARTESIAN_POINT('Ctrl Pts',(-49.8352745925261,-2.20751597714286,
-229.762108046517));
#203986=CARTESIAN_POINT('Ctrl Pts',(-52.0497152441705,-1.53755916668926,
-226.407703586764));
#203987=CARTESIAN_POINT('Ctrl Pts',(-54.2642183610334,-0.865666855062723,
-223.053733238581));
#203988=CARTESIAN_POINT('Ctrl Pts',(-56.4787214778963,-0.193774543436184,
-219.699762890398));
#203989=CARTESIAN_POINT('Ctrl Pts',(-58.6933043194368,0.480231871349857,
-216.346274307009));
#203990=CARTESIAN_POINT('Ctrl Pts',(-60.9079135866709,1.15526652998651,
-212.993011881675));
#203991=CARTESIAN_POINT('Ctrl Pts',(-47.6166843338988,-2.89479809257736,
-233.118546667211));
#203992=CARTESIAN_POINT('Ctrl Pts',(-49.8304641874375,-2.23319920218914,
-229.762886946434));
#203993=CARTESIAN_POINT('Ctrl Pts',(-52.0445356905235,-1.56647045026326,
-226.408456344895));
#203994=CARTESIAN_POINT('Ctrl Pts',(-54.2586738605045,-0.897786580916013,
-223.054464805284));
#203995=CARTESIAN_POINT('Ctrl Pts',(-56.4728120304856,-0.229102711568775,
-219.700473265674));
#203996=CARTESIAN_POINT('Ctrl Pts',(-58.6870347127076,0.44171613101905,
-216.346968914843));
#203997=CARTESIAN_POINT('Ctrl Pts',(-60.9012859052481,1.11357395216271,
-212.993693318827));
#203998=CARTESIAN_POINT('Ctrl Pts',(-47.6122821058773,-2.91382681376045,
-233.120123741771));
#203999=CARTESIAN_POINT('Ctrl Pts',(-49.8256462366764,-2.25563426408762,
-229.764381027656));
#204000=CARTESIAN_POINT('Ctrl Pts',(-52.0393253463554,-1.59222179649422,
-226.409896055477));
#204001=CARTESIAN_POINT('Ctrl Pts',(-54.2530784318765,-0.926817341305142,
-223.05586052551));
#204002=CARTESIAN_POINT('Ctrl Pts',(-56.4668315173976,-0.261412886116064,
-219.701824995542));
#204003=CARTESIAN_POINT('Ctrl Pts',(-58.680677501921,0.406166125023995,
-216.348288119608));
#204004=CARTESIAN_POINT('Ctrl Pts',(-60.8945556035063,1.07480407935814,
-212.99498540692));
#204005=CARTESIAN_POINT('Ctrl Pts',(-47.6074726880044,-2.94429670427164,
-233.119124814901));
#204006=CARTESIAN_POINT('Ctrl Pts',(-49.8205052535735,-2.2890391191441,
-229.763446888111));
#204007=CARTESIAN_POINT('Ctrl Pts',(-52.0338426588191,-1.6286224591917,
-226.409003009738));
#204008=CARTESIAN_POINT('Ctrl Pts',(-54.2472513064603,-0.966235601713411,
-223.055000571257));
#204009=CARTESIAN_POINT('Ctrl Pts',(-56.4606599541014,-0.303848744235122,
-219.700998132776));
#204010=CARTESIAN_POINT('Ctrl Pts',(-58.6741582110175,0.36068851501233,
-216.347485336292));
#204011=CARTESIAN_POINT('Ctrl Pts',(-60.8876872878579,1.02627337962685,
-212.994202601728));
#204012=CARTESIAN_POINT('Ctrl Pts',(-47.5978538522586,-3.00523648529404,
-233.117126961161));
#204013=CARTESIAN_POINT('Ctrl Pts',(-49.8102232873676,-2.35584882925707,
-229.761578609019));
#204014=CARTESIAN_POINT('Ctrl Pts',(-52.0228772837467,-1.70142378458667,
-226.407216918259));
#204015=CARTESIAN_POINT('Ctrl Pts',(-54.2355970556278,-1.04507212252995,
-223.053280662751));
#204016=CARTESIAN_POINT('Ctrl Pts',(-56.448316827509,-0.388720460473239,
-219.699344407242));
#204017=CARTESIAN_POINT('Ctrl Pts',(-58.6611196292105,0.269733294988998,
-216.345879769661));
#204018=CARTESIAN_POINT('Ctrl Pts',(-60.873950656561,0.929211980164266,
-212.992636991345));
#204019=CARTESIAN_POINT('Ctrl Pts',(-47.5885508550713,-3.06624038087206,
-233.115176478235));
#204020=CARTESIAN_POINT('Ctrl Pts',(-49.8002794578931,-2.42271445147103,
-229.759753873753));
#204021=CARTESIAN_POINT('Ctrl Pts',(-52.0122734022483,-1.77427184016,-226.405472145231));
#204022=CARTESIAN_POINT('Ctrl Pts',(-54.2243279326664,-1.12394607107203,
-223.051600306617));
#204023=CARTESIAN_POINT('Ctrl Pts',(-56.4363824630845,-0.473620301984068,
-219.697728468003));
#204024=CARTESIAN_POINT('Ctrl Pts',(-58.6485137824127,0.178759449846657,
-216.344310765974));
#204025=CARTESIAN_POINT('Ctrl Pts',(-60.8606708677034,0.832141479427629,
-212.99110694513));
#204026=CARTESIAN_POINT('Ctrl Pts',(-47.5795644264693,-3.1273054400959,
-233.113272591666));
#204027=CARTESIAN_POINT('Ctrl Pts',(-49.7906742268616,-2.48963297721053,
-229.757972064269));
#204028=CARTESIAN_POINT('Ctrl Pts',(-52.0020311559296,-1.84716370589099,
-226.403768144263));
#204029=CARTESIAN_POINT('Ctrl Pts',(-54.2134437517945,-1.20285465735803,
-223.049959011375));
#204030=CARTESIAN_POINT('Ctrl Pts',(-56.4248563476593,-0.558545608825073,
-219.696149878487));
#204031=CARTESIAN_POINT('Ctrl Pts',(-58.6363398184349,0.0877694602078754,
-216.342777920879));
#204032=CARTESIAN_POINT('Ctrl Pts',(-60.8478467270347,0.735064158177848,
-212.989612083611));
#204033=CARTESIAN_POINT('Ctrl Pts',(-47.5615915692654,-3.24943555854357,
-233.109464818529));
#204034=CARTESIAN_POINT('Ctrl Pts',(-49.7714637647986,-2.62347002868952,
-229.7544084453));
#204035=CARTESIAN_POINT('Ctrl Pts',(-51.9815466632923,-1.99294743735296,
-226.40036014233));
#204036=CARTESIAN_POINT('Ctrl Pts',(-54.1916753900507,-1.36067182993002,
-223.046676420892));
#204037=CARTESIAN_POINT('Ctrl Pts',(-56.401804116809,-0.728396222507082,
-219.692992699454));
#204038=CARTESIAN_POINT('Ctrl Pts',(-58.6119918904791,-0.0942105190696879,
-216.339712230689));
#204039=CARTESIAN_POINT('Ctrl Pts',(-60.8221984456974,0.540909515678286,
-212.986622360574));
#204040=CARTESIAN_POINT('Ctrl Pts',(-47.5448849460372,-3.37181033218646,
-233.105843362456));
#204041=CARTESIAN_POINT('Ctrl Pts',(-49.7536076690841,-2.75751868949416,
-229.751016479375));
#204042=CARTESIAN_POINT('Ctrl Pts',(-51.9625086899236,-2.13890640284165,
-226.397115187946));
#204043=CARTESIAN_POINT('Ctrl Pts',(-54.1714467798668,-1.51862754547975,
-223.043550040683));
#204044=CARTESIAN_POINT('Ctrl Pts',(-56.38038486981,-0.898348688117847,
-219.68998489342));
#204045=CARTESIAN_POINT('Ctrl Pts',(-58.5893714844719,-0.276255066290686,
-216.336791153806));
#204046=CARTESIAN_POINT('Ctrl Pts',(-60.798372749993,0.346727601648124,
-212.983773359142));
#204047=CARTESIAN_POINT('Ctrl Pts',(-47.5294508970783,-3.49440615205346,
-233.102402864825));
#204048=CARTESIAN_POINT('Ctrl Pts',(-49.7371099711637,-2.89175495532409,
-229.747791831751));
#204049=CARTESIAN_POINT('Ctrl Pts',(-51.9449186325461,-2.28501732803231,
-226.3940294043));
#204050=CARTESIAN_POINT('Ctrl Pts',(-54.1527566412239,-1.67669958626741,
-223.040576342272));
#204051=CARTESIAN_POINT('Ctrl Pts',(-56.3605946499017,-1.0683818445025,
-219.687123280246));
#204052=CARTESIAN_POINT('Ctrl Pts',(-58.5684718967623,-0.458344461962341,
-216.334011708901));
#204053=CARTESIAN_POINT('Ctrl Pts',(-60.7763601725369,0.15253653159383,
-212.981062249621));
#204054=CARTESIAN_POINT('Ctrl Pts',(-47.4059785054068,-4.47517271098946,
-233.07487888378));
#204055=CARTESIAN_POINT('Ctrl Pts',(-49.6051283878,-3.96564508196357,-229.721994650771));
#204056=CARTESIAN_POINT('Ctrl Pts',(-51.8041981735258,-3.45390472955758,
-226.369343135129));
#204057=CARTESIAN_POINT('Ctrl Pts',(-54.0032355320804,-2.94127591256867,
-223.016786754993));
#204058=CARTESIAN_POINT('Ctrl Pts',(-56.202272890635,-2.42864709557977,
-219.664230374857));
#204059=CARTESIAN_POINT('Ctrl Pts',(-58.4012751950854,-1.91505962733557,
-216.311776149656));
#204060=CARTESIAN_POINT('Ctrl Pts',(-60.6002595528876,-1.40099202884052,
-212.959373373456));
#204061=CARTESIAN_POINT('Ctrl Pts',(-47.3643002300016,-5.47063877596875,
-233.058775431931));
#204062=CARTESIAN_POINT('Ctrl Pts',(-49.5603357959614,-5.05191240085809,
-229.706777484113));
#204063=CARTESIAN_POINT('Ctrl Pts',(-51.7562892676681,-4.63275255105671,
-226.354730416234));
#204064=CARTESIAN_POINT('Ctrl Pts',(-53.9522144422201,-4.21341447341654,
-223.002667034626));
#204065=CARTESIAN_POINT('Ctrl Pts',(-56.148139616772,-3.79407639577637,
-219.650603653018));
#204066=CARTESIAN_POINT('Ctrl Pts',(-58.3440331530531,-3.37454700228228,
-216.298521859654));
#204067=CARTESIAN_POINT('Ctrl Pts',(-60.5399122633319,-2.95492052264675,
-212.94643187892));
#204068=CARTESIAN_POINT('Ctrl Pts',(-47.4064137512828,-6.46376836204135,
-233.053237209745));
#204069=CARTESIAN_POINT('Ctrl Pts',(-49.6038760388037,-6.13507130643716,
-229.701318673814));
#204070=CARTESIAN_POINT('Ctrl Pts',(-51.8014392198341,-5.80767781765755,
-226.34934009846));
#204071=CARTESIAN_POINT('Ctrl Pts',(-53.999040049297,-5.48080969928608,
-222.997335349492));
#204072=CARTESIAN_POINT('Ctrl Pts',(-56.19664087876,-5.15394158091461,-219.645330600522));
#204073=CARTESIAN_POINT('Ctrl Pts',(-58.3942830138637,-4.82763991403419,
-216.293298098971));
#204074=CARTESIAN_POINT('Ctrl Pts',(-60.5919449770341,-4.50162265073271,
-212.941251066378));
#204075=CARTESIAN_POINT('Ctrl Pts',(-47.4274705119234,-6.96033315507766,
-233.050468098652));
#204076=CARTESIAN_POINT('Ctrl Pts',(-49.6256461602249,-6.6766507592267,
-229.698589268665));
#204077=CARTESIAN_POINT('Ctrl Pts',(-51.8240141959171,-6.39514045095797,
-226.346644939574));
#204078=CARTESIAN_POINT('Ctrl Pts',(-54.0224528528355,-6.11450731222085,
-222.994669506924));
#204079=CARTESIAN_POINT('Ctrl Pts',(-56.220891509754,-5.83387417348373,
-219.642694074275));
#204080=CARTESIAN_POINT('Ctrl Pts',(-58.419407944269,-5.55418636991015,
-216.29068621863));
#204081=CARTESIAN_POINT('Ctrl Pts',(-60.6179613338852,-5.27497371477569,
-212.938660660107));
#204082=CARTESIAN_POINT('Ctrl Pts',(-47.4693973645209,-7.45640759953517,
-233.050348887721));
#204083=CARTESIAN_POINT('Ctrl Pts',(-49.6694421105903,-7.21751150761842,
-229.698309141063));
#204084=CARTESIAN_POINT('Ctrl Pts',(-51.8698193135396,-6.98165879246334,
-226.346267078691));
#204085=CARTESIAN_POINT('Ctrl Pts',(-54.0703159902812,-6.74703873870746,
-222.994214128443));
#204086=CARTESIAN_POINT('Ctrl Pts',(-56.2708126670227,-6.51241868495157,
-219.642161178194));
#204087=CARTESIAN_POINT('Ctrl Pts',(-58.4714415769781,-6.27912620426164,
-216.290098836338));
#204088=CARTESIAN_POINT('Ctrl Pts',(-60.6721324487782,-6.0465020347434,
-212.938028751337));
#204089=CARTESIAN_POINT('Ctrl Pts',(-47.5320802669249,-7.94976361170966,
-233.052889623343));
#204090=CARTESIAN_POINT('Ctrl Pts',(-49.7351412982067,-7.7556448112324,
-229.700481632561));
#204091=CARTESIAN_POINT('Ctrl Pts',(-51.9387261626187,-7.5654468780096,
-226.348205936691));
#204092=CARTESIAN_POINT('Ctrl Pts',(-54.1424952790584,-7.37683668146129,
-222.995965483144));
#204093=CARTESIAN_POINT('Ctrl Pts',(-56.3462643954981,-7.18822648491298,
-219.643725029598));
#204094=CARTESIAN_POINT('Ctrl Pts',(-58.5502384998489,-7.00132626939384,
-216.291526839263));
#204095=CARTESIAN_POINT('Ctrl Pts',(-60.7543073371829,-6.81528655387943,
-212.939344378339));
#204096=CARTESIAN_POINT('Ctrl Pts',(-47.563421718127,-8.1964416177969,-233.054159991154));
#204097=CARTESIAN_POINT('Ctrl Pts',(-49.7679908920149,-8.02471146303938,
-229.70156787831));
#204098=CARTESIAN_POINT('Ctrl Pts',(-51.9731795871583,-7.85734092078273,
-226.34917536569));
#204099=CARTESIAN_POINT('Ctrl Pts',(-54.1785849234471,-7.6917356528382,
-222.996841160495));
#204100=CARTESIAN_POINT('Ctrl Pts',(-56.3839902597359,-7.52613038489368,
-219.644506955299));
#204101=CARTESIAN_POINT('Ctrl Pts',(-58.5896369612844,-7.36242630195994,
-216.292240840726));
#204102=CARTESIAN_POINT('Ctrl Pts',(-60.7953947813852,-7.19967881344745,
-212.94000219184));
#204103=CARTESIAN_POINT('Ctrl Pts',(-47.5999371411941,-8.4424144119742,
-233.056093784063));
#204104=CARTESIAN_POINT('Ctrl Pts',(-49.8063055502802,-8.29307945277301,
-229.703266385626));
#204105=CARTESIAN_POINT('Ctrl Pts',(-52.0134014665884,-8.14854160584086,
-226.350723520978));
#204106=CARTESIAN_POINT('Ctrl Pts',(-54.2207502118905,-8.00594532648383,
-222.998268420575));
#204107=CARTESIAN_POINT('Ctrl Pts',(-56.4280989571927,-7.8633490471268,
-219.645813320171));
#204108=CARTESIAN_POINT('Ctrl Pts',(-58.6357298166351,-7.72284397328174,
-216.293459199193));
#204109=CARTESIAN_POINT('Ctrl Pts',(-60.8434900309058,-7.58339072582217,
-212.941147613748));
#204110=CARTESIAN_POINT('Ctrl Pts',(-47.6415907958571,-8.68748728842518,
-233.058700763469));
#204111=CARTESIAN_POINT('Ctrl Pts',(-49.8500528218283,-8.56055336019126,
-229.705584368071));
#204112=CARTESIAN_POINT('Ctrl Pts',(-52.0593649584596,-8.43886161373385,
-226.352856624949));
#204113=CARTESIAN_POINT('Ctrl Pts',(-54.2689704157657,-8.31928937162988,
-223.000252784861));
#204114=CARTESIAN_POINT('Ctrl Pts',(-56.4785758730718,-8.19971712952592,
-219.647648944772));
#204115=CARTESIAN_POINT('Ctrl Pts',(-58.6885092193172,-8.08242819326595,
-216.295186431349));
#204116=CARTESIAN_POINT('Ctrl Pts',(-60.8985922273728,-7.96628687259449,
-212.942784965869));
#204117=CARTESIAN_POINT('Ctrl Pts',(-47.6624176231886,-8.81002372665067,
-233.060004253171));
#204118=CARTESIAN_POINT('Ctrl Pts',(-49.8719264576024,-8.69429031390039,
-229.706743359295));
#204119=CARTESIAN_POINT('Ctrl Pts',(-52.0823467043952,-8.58402161768034,
-226.353923176935));
#204120=CARTESIAN_POINT('Ctrl Pts',(-54.2930805177033,-8.47596139420291,
-223.001244967003));
#204121=CARTESIAN_POINT('Ctrl Pts',(-56.5038143310114,-8.36790117072548,
-219.648566757072));
#204122=CARTESIAN_POINT('Ctrl Pts',(-58.7148989206583,-8.26222030325806,
-216.296050047426));
#204123=CARTESIAN_POINT('Ctrl Pts',(-60.9261433256064,-8.15773494598065,
-212.943603641929));
#204124=CARTESIAN_POINT('Ctrl Pts',(-47.6845291479335,-8.93233516940169,
-233.061476300607));
#204125=CARTESIAN_POINT('Ctrl Pts',(-49.8951583401493,-8.82780373392919,
-229.708057415679));
#204126=CARTESIAN_POINT('Ctrl Pts',(-52.1067639241,-8.72896144063768,-226.355136126385));
#204127=CARTESIAN_POINT('Ctrl Pts',(-54.3187044016857,-8.63241699899096,
-223.002376557269));
#204128=CARTESIAN_POINT('Ctrl Pts',(-56.5306448792714,-8.53587255734424,
-219.649616988152));
#204129=CARTESIAN_POINT('Ctrl Pts',(-58.7429602838421,-8.44180404135816,
-216.297040966938));
#204130=CARTESIAN_POINT('Ctrl Pts',(-60.9554461772338,-8.34897906928816,
-212.944545370418));
#204131=CARTESIAN_POINT('Ctrl Pts',(-47.7079217613744,-9.05439718416747,
-233.063119714194));
#204132=CARTESIAN_POINT('Ctrl Pts',(-49.9197449843438,-8.96106910734242,
-229.709528628916));
#204133=CARTESIAN_POINT('Ctrl Pts',(-52.1326136936507,-8.87365758922025,
-226.356497221309));
#204134=CARTESIAN_POINT('Ctrl Pts',(-54.3458398007892,-8.78863407215474,
-223.003649044211));
#204135=CARTESIAN_POINT('Ctrl Pts',(-56.5590659079277,-8.70361055508924,
-219.650800867113));
#204136=CARTESIAN_POINT('Ctrl Pts',(-58.7726924798428,-8.62116045955843,
-216.298160266832));
#204137=CARTESIAN_POINT('Ctrl Pts',(-60.9865007760101,-8.54000225738003,
-212.945611112248));
#204138=CARTESIAN_POINT('Ctrl Pts',(-47.7108458380545,-9.0696549360132,
-233.063325140892));
#204139=CARTESIAN_POINT('Ctrl Pts',(-49.9228183148681,-8.97772727901907,
-229.709712530571));
#204140=CARTESIAN_POINT('Ctrl Pts',(-52.1358449148446,-8.89174460779308,
-226.356667358174));
#204141=CARTESIAN_POINT('Ctrl Pts',(-54.3492317256771,-8.80816120630022,
-223.003808105078));
#204142=CARTESIAN_POINT('Ctrl Pts',(-56.5626185365097,-8.72457780480736,
-219.650948851983));
#204143=CARTESIAN_POINT('Ctrl Pts',(-58.7764090043429,-8.64358001183346,
-216.29830017932));
#204144=CARTESIAN_POINT('Ctrl Pts',(-60.9903826008572,-8.56388015589151,
-212.945744329977));
#204145=CARTESIAN_POINT('Ctrl Pts',(-47.7137899325008,-9.08490879046653,
-233.063533246565));
#204146=CARTESIAN_POINT('Ctrl Pts',(-49.9259128140418,-8.99438157488791,
-229.709898888829));
#204147=CARTESIAN_POINT('Ctrl Pts',(-52.1390985200058,-8.90982781887923,
-226.356839810649));
#204148=CARTESIAN_POINT('Ctrl Pts',(-54.3526472682709,-8.82768461331957,
-223.003969368145));
#204149=CARTESIAN_POINT('Ctrl Pts',(-56.5661960165361,-8.74554140775991,
-219.65109892564));
#204150=CARTESIAN_POINT('Ctrl Pts',(-58.7801516357373,-8.66599601217575,
-216.29844209819));
#204151=CARTESIAN_POINT('Ctrl Pts',(-60.994291796841,-8.58775460223573,
-212.945879485775));
#204152=CARTESIAN_POINT('Ctrl Pts',(-47.716754038316,-9.10015869973864,
-233.063744037883));
#204153=CARTESIAN_POINT('Ctrl Pts',(-49.9290284754874,-9.01103194700285,
-229.71008770866));
#204154=CARTESIAN_POINT('Ctrl Pts',(-52.1423745037473,-8.92790717652798,
-226.357014582869));
#204155=CARTESIAN_POINT('Ctrl Pts',(-54.3560864243857,-8.84720424996069,
-223.004132836908));
#204156=CARTESIAN_POINT('Ctrl Pts',(-56.5697983450241,-8.7665013233934,
-219.651251090947));
#204157=CARTESIAN_POINT('Ctrl Pts',(-58.78392037252,-8.68840842352587,-216.298586025925));
#204158=CARTESIAN_POINT('Ctrl Pts',(-60.9982283640248,-8.61162556319128,
-212.946016581829));
#204159=CARTESIAN_POINT('Ctrl Pts',(-47.7182360912236,-9.10778365437469,
-233.063849433542));
#204160=CARTESIAN_POINT('Ctrl Pts',(-49.9305863062102,-9.01935713306031,
-229.710182118577));
#204161=CARTESIAN_POINT('Ctrl Pts',(-52.1440124956181,-8.93694685535236,
-226.357101968979));
#204162=CARTESIAN_POINT('Ctrl Pts',(-54.3578060024431,-8.85696406828125,
-223.004214571289));
#204163=CARTESIAN_POINT('Ctrl Pts',(-56.5715995092681,-8.77698128121015,
-219.6513271736));
#204164=CARTESIAN_POINT('Ctrl Pts',(-58.7858047409113,-8.69961462920092,
-216.298657989792));
#204165=CARTESIAN_POINT('Ctrl Pts',(-61.0001966476166,-8.62356104366905,
-212.946085129856));
#204166=CARTESIAN_POINT('Ctrl Pts',(-47.7199389533574,-9.11682055194411,
-233.06406871878));
#204167=CARTESIAN_POINT('Ctrl Pts',(-49.9323460073902,-9.02903001372169,
-229.710378872728));
#204168=CARTESIAN_POINT('Ctrl Pts',(-52.1458407050898,-8.94729076123427,
-226.357284562563));
#204169=CARTESIAN_POINT('Ctrl Pts',(-54.3597065585291,-8.86799272250201,
-223.004385813307));
#204170=CARTESIAN_POINT('Ctrl Pts',(-56.5735724119685,-8.78869468376974,
-219.651487064051));
#204171=CARTESIAN_POINT('Ctrl Pts',(-58.7878543357751,-8.71202766150863,
-216.298809692624));
#204172=CARTESIAN_POINT('Ctrl Pts',(-61.0023248619954,-8.63668103342285,
-212.946230067727));
#204173=CARTESIAN_POINT('Ctrl Pts',(-47.7211311423516,-9.12247799776195,
-233.064017991084));
#204174=CARTESIAN_POINT('Ctrl Pts',(-49.9336413200512,-9.03547708644307,
-229.710333027481));
#204175=CARTESIAN_POINT('Ctrl Pts',(-52.1472334449741,-8.95451285699648,
-226.357241499541));
#204176=CARTESIAN_POINT('Ctrl Pts',(-54.3611948094061,-8.87598426441826,
-223.004344929563));
#204177=CARTESIAN_POINT('Ctrl Pts',(-56.5751561738381,-8.79745567184005,
-219.651448359586));
#204178=CARTESIAN_POINT('Ctrl Pts',(-58.7895314509544,-8.72155201353807,
-216.298772458348));
#204179=CARTESIAN_POINT('Ctrl Pts',(-61.004094357101,-8.64696579840547,
-212.94619401758));
#204180=CARTESIAN_POINT('Ctrl Pts',(-47.7223233313458,-9.1281354435798,
-233.063967263389));
#204181=CARTESIAN_POINT('Ctrl Pts',(-49.9349366327123,-9.04192415916445,
-229.710287182234));
#204182=CARTESIAN_POINT('Ctrl Pts',(-52.1486261848584,-8.96173495275868,
-226.357198436518));
#204183=CARTESIAN_POINT('Ctrl Pts',(-54.362683060283,-8.88397580633452,
-223.004304045819));
#204184=CARTESIAN_POINT('Ctrl Pts',(-56.5767399357077,-8.80621665991036,
-219.651409655121));
#204185=CARTESIAN_POINT('Ctrl Pts',(-58.7912085661337,-8.73107636556752,
-216.298735224073));
#204186=CARTESIAN_POINT('Ctrl Pts',(-61.0058638522065,-8.6572505633881,
-212.946157967432));
#204187=CARTESIAN_POINT('Ctrl Pts',(-47.7235115705647,-9.13379405727712,
-233.063916532445));
#204188=CARTESIAN_POINT('Ctrl Pts',(-49.9362275889306,-9.04837227186877,
-229.710241325062));
#204189=CARTESIAN_POINT('Ctrl Pts',(-52.1500141863611,-8.96895796970056,
-226.357155358521));
#204190=CARTESIAN_POINT('Ctrl Pts',(-54.3641661982611,-8.89196815031558,
-223.004263144959));
#204191=CARTESIAN_POINT('Ctrl Pts',(-56.5783182101612,-8.8149783309306,
-219.651370931397));
#204192=CARTESIAN_POINT('Ctrl Pts',(-58.7928798280227,-8.740601282021,-216.298697969725));
#204193=CARTESIAN_POINT('Ctrl Pts',(-61.0076271318174,-8.66753577332984,
-212.946121896728));
#204194=CARTESIAN_POINT('Ctrl Pts',(-47.724695856798,-9.13945382791814,
-233.06386579822));
#204195=CARTESIAN_POINT('Ctrl Pts',(-49.9375141864838,-9.05482141596443,
-229.710195456012));
#204196=CARTESIAN_POINT('Ctrl Pts',(-52.1513974481024,-8.97618190118969,
-226.357112265619));
#204197=CARTESIAN_POINT('Ctrl Pts',(-54.3656442227822,-8.89996129157268,
-223.00422222707));
#204198=CARTESIAN_POINT('Ctrl Pts',(-56.579890997462,-8.82374068195567,
-219.651332188522));
#204199=CARTESIAN_POINT('Ctrl Pts',(-58.7945452376739,-8.75012676166283,
-216.298660695422));
#204200=CARTESIAN_POINT('Ctrl Pts',(-61.0093841977678,-8.67782142864838,
-212.946085805591));
#204201=CARTESIAN_POINT('Ctrl Pts',(-47.7294330017316,-9.16209291048223,
-233.063662861321));
#204202=CARTESIAN_POINT('Ctrl Pts',(-49.9426605766967,-9.08061799234707,
-229.710011979809));
#204203=CARTESIAN_POINT('Ctrl Pts',(-52.1569304950676,-9.0050776271462,
-226.356939894011));
#204204=CARTESIAN_POINT('Ctrl Pts',(-54.3715563208665,-8.93193385660108,
-223.004058555517));
#204205=CARTESIAN_POINT('Ctrl Pts',(-56.5861821466654,-8.85879008605595,
-219.651177217023));
#204206=CARTESIAN_POINT('Ctrl Pts',(-58.8012068762785,-8.78822868023012,
-216.29851159821));
#204207=CARTESIAN_POINT('Ctrl Pts',(-61.0164124615696,-8.71896404992253,
-212.945941441045));
#204208=CARTESIAN_POINT('Ctrl Pts',(-47.7341068986215,-9.18475050415316,
-233.063459871981));
#204209=CARTESIAN_POINT('Ctrl Pts',(-49.9477372281162,-9.10643107100621,
-229.709828313605));
#204210=CARTESIAN_POINT('Ctrl Pts',(-52.1623877057604,-9.03398798587052,
-226.356767284002));
#204211=CARTESIAN_POINT('Ctrl Pts',(-54.3773866035966,-8.96391917805846,
-223.003894611599));
#204212=CARTESIAN_POINT('Ctrl Pts',(-56.5923855014328,-8.89385037024639,
-219.651021939195));
#204213=CARTESIAN_POINT('Ctrl Pts',(-58.8077748791159,-8.8263396098254,
-216.298362181801));
#204214=CARTESIAN_POINT('Ctrl Pts',(-61.0233413068671,-8.76011379724005,
-212.945796749657));
#204215=CARTESIAN_POINT('Ctrl Pts',(-47.7387173442106,-9.207425908897,-233.06325682779));
#204216=CARTESIAN_POINT('Ctrl Pts',(-49.9527439997195,-9.13226010185821,
-229.709644459743));
#204217=CARTESIAN_POINT('Ctrl Pts',(-52.1677689925887,-9.06291255266274,
-226.356594439508));
#204218=CARTESIAN_POINT('Ctrl Pts',(-54.383135035575,-8.99591694925441,
-223.003730400442));
#204219=CARTESIAN_POINT('Ctrl Pts',(-56.5985010785614,-8.92892134584607,
-219.650866361376));
#204220=CARTESIAN_POINT('Ctrl Pts',(-58.8142493132399,-8.86445947120716,
-216.2982124531));
#204221=CARTESIAN_POINT('Ctrl Pts',(-61.030170850553,-8.80127069719074,
-212.945651738761));
#204222=CARTESIAN_POINT('Ctrl Pts',(-47.7479382353889,-9.25277671838467,
-233.062850739409));
#204223=CARTESIAN_POINT('Ctrl Pts',(-49.9627575429261,-9.18391816356222,
-229.70927675202));
#204224=CARTESIAN_POINT('Ctrl Pts',(-52.1785315662453,-9.12076168624719,
-226.356248750518));
#204225=CARTESIAN_POINT('Ctrl Pts',(-54.394631899532,-9.05991249164631,
-223.003401978127));
#204226=CARTESIAN_POINT('Ctrl Pts',(-56.6107322328186,-8.99906329704543,
-219.650555205738));
#204227=CARTESIAN_POINT('Ctrl Pts',(-58.827198181488,-8.9406991939707,-216.297912995698));
#204228=CARTESIAN_POINT('Ctrl Pts',(-61.0438299379249,-8.88358449709214,
-212.945361716967));
#204229=CARTESIAN_POINT('Ctrl Pts',(-47.7569053178599,-9.29819877221664,
-233.062444432209));
#204230=CARTESIAN_POINT('Ctrl Pts',(-49.9724915649241,-9.23564003421678,
-229.708908294511));
#204231=CARTESIAN_POINT('Ctrl Pts',(-52.1889904432917,-9.1786676522935,
-226.355902124491));
#204232=CARTESIAN_POINT('Ctrl Pts',(-54.4058013599478,-9.12395783319898,
-223.003072487813));
#204233=CARTESIAN_POINT('Ctrl Pts',(-56.6226122766038,-9.06924801410446,
-219.650242851134));
#204234=CARTESIAN_POINT('Ctrl Pts',(-58.8397727753602,-9.01697464410811,
-216.297612290131));
#204235=CARTESIAN_POINT('Ctrl Pts',(-61.0570918196413,-8.96592690776347,
-212.945070418141));
#204236=CARTESIAN_POINT('Ctrl Pts',(-47.7656170077038,-9.34368646884676,
-233.062037879842));
#204237=CARTESIAN_POINT('Ctrl Pts',(-49.9819449608238,-9.2874213104565,
-229.708539095772));
#204238=CARTESIAN_POINT('Ctrl Pts',(-52.1991449367821,-9.23662705053824,
-226.355554581771));
#204239=CARTESIAN_POINT('Ctrl Pts',(-54.4166431400134,-9.18805051768256,
-223.002741959001));
#204240=CARTESIAN_POINT('Ctrl Pts',(-56.6341413432447,-9.13947398482688,
-219.649929336231));
#204241=CARTESIAN_POINT('Ctrl Pts',(-58.8519736255103,-9.09328518499885,
-216.297310379527));
#204242=CARTESIAN_POINT('Ctrl Pts',(-61.069957421301,-9.04829813924799,
-212.94477788882));
#204243=CARTESIAN_POINT('Ctrl Pts',(-47.9050040452069,-10.0714896149287,
-233.055533041971));
#204244=CARTESIAN_POINT('Ctrl Pts',(-50.1331992952188,-10.115921730292,
-229.702631915958));
#204245=CARTESIAN_POINT('Ctrl Pts',(-52.3616168326291,-10.1639774224541,
-226.349993898252));
#204246=CARTESIAN_POINT('Ctrl Pts',(-54.5901116210639,-10.2135334694198,
-222.997453498015));
#204247=CARTESIAN_POINT('Ctrl Pts',(-56.8186064094987,-10.2630895163856,
-219.644913097779));
#204248=CARTESIAN_POINT('Ctrl Pts',(-59.0471872279132,-10.3142538392508,
-216.292479809858));
#204249=CARTESIAN_POINT('Ctrl Pts',(-61.2758070478567,-10.3662378430004,
-212.940097419686));
#204250=CARTESIAN_POINT('Ctrl Pts',(-47.9784204856001,-10.8160623601621,
-233.048965734498));
#204251=CARTESIAN_POINT('Ctrl Pts',(-50.2122149161821,-10.9596359714715,
-229.696533843322));
#204252=CARTESIAN_POINT('Ctrl Pts',(-52.4459513488164,-11.1050325676855,
-226.344195161346));
#204253=CARTESIAN_POINT('Ctrl Pts',(-54.6796638979776,-11.2511741221942,
-222.991894447348));
#204254=CARTESIAN_POINT('Ctrl Pts',(-56.9133764471387,-11.3973156767028,
-219.639593733351));
#204255=CARTESIAN_POINT('Ctrl Pts',(-59.1470633643947,-11.5442580388962,
-216.287333861831));
#204256=CARTESIAN_POINT('Ctrl Pts',(-61.3807372553903,-11.6916056255194,
-212.935094620098));
#204257=CARTESIAN_POINT('Ctrl Pts',(-47.9834035327445,-11.5593373188707,
-233.042545221464));
#204258=CARTESIAN_POINT('Ctrl Pts',(-50.2170610824398,-11.8031522322565,
-229.690412491071));
#204259=CARTESIAN_POINT('Ctrl Pts',(-52.4507177144441,-12.0469951332675,
-226.33828118561));
#204260=CARTESIAN_POINT('Ctrl Pts',(-54.684373970075,-12.2908494697823,
-222.986150461423));
#204261=CARTESIAN_POINT('Ctrl Pts',(-56.9180302257058,-12.5347038062971,
-219.634019737236));
#204262=CARTESIAN_POINT('Ctrl Pts',(-59.1516860770602,-12.7785704359954,
-216.281889638136));
#204263=CARTESIAN_POINT('Ctrl Pts',(-61.3853417234255,-13.0224432858052,
-212.92975985503));
#204264=CARTESIAN_POINT('Ctrl Pts',(-47.9883865798889,-12.3026122775794,
-233.036124708431));
#204265=CARTESIAN_POINT('Ctrl Pts',(-50.2219072486975,-12.6466684930416,
-229.684291138819));
#204266=CARTESIAN_POINT('Ctrl Pts',(-52.4554840800718,-12.9889576988494,
-226.332367209873));
#204267=CARTESIAN_POINT('Ctrl Pts',(-54.6890840421723,-13.3305248173704,
-222.980406475497));
#204268=CARTESIAN_POINT('Ctrl Pts',(-56.9226840042728,-13.6720919358914,
-219.628445741121));
#204269=CARTESIAN_POINT('Ctrl Pts',(-59.1563087897256,-14.0128828330946,
-216.276445414441));
#204270=CARTESIAN_POINT('Ctrl Pts',(-61.3899461914607,-14.353280946091,
-212.924425089962));
#204271=CARTESIAN_POINT('Ctrl Pts',(-47.9249646072757,-13.0488680722298,
-233.029820400472));
#204272=CARTESIAN_POINT('Ctrl Pts',(-50.1526004463906,-13.4919379593521,
-229.678126738255));
#204273=CARTESIAN_POINT('Ctrl Pts',(-52.3806853939039,-13.9314932517732,
-226.326331018504));
#204274=CARTESIAN_POINT('Ctrl Pts',(-54.6089422344929,-14.3695898632513,
-222.974482011522));
#204275=CARTESIAN_POINT('Ctrl Pts',(-56.8371990750819,-14.8076864747294,
-219.622633004539));
#204276=CARTESIAN_POINT('Ctrl Pts',(-59.0656432437958,-15.2442202432178,
-216.270729289381));
#204277=CARTESIAN_POINT('Ctrl Pts',(-61.2941782948235,-15.6799563776017,
-212.918794099076));
#204278=CARTESIAN_POINT('Ctrl Pts',(-47.794905416537,-13.7800486938334,
-233.0237330726));
#204279=CARTESIAN_POINT('Ctrl Pts',(-50.0104931205382,-14.3235088264801,
-229.67202163298));
#204280=CARTESIAN_POINT('Ctrl Pts',(-52.2272657548643,-14.8617096033744,
-226.320268783124));
#204281=CARTESIAN_POINT('Ctrl Pts',(-54.4444686924125,-15.3977680306514,
-222.968464399553));
#204282=CARTESIAN_POINT('Ctrl Pts',(-56.6616716299607,-15.9338264579286,
-219.616660015982));
#204283=CARTESIAN_POINT('Ctrl Pts',(-58.8793495680496,-16.4675807101401,
-216.264808277961));
#204284=CARTESIAN_POINT('Ctrl Pts',(-61.0972513955672,-17.0001720517288,
-212.912922153302));
#204285=CARTESIAN_POINT('Ctrl Pts',(-47.7867767171158,-13.8257474826836,
-233.023352614608));
#204286=CARTESIAN_POINT('Ctrl Pts',(-50.0016114126724,-14.3754820056756,
-229.6716400639));
#204287=CARTESIAN_POINT('Ctrl Pts',(-52.2176770274244,-14.9198481253495,
-226.319889893413));
#204288=CARTESIAN_POINT('Ctrl Pts',(-54.4341890960325,-15.4620291661139,
-222.968088298805));
#204289=CARTESIAN_POINT('Ctrl Pts',(-56.6507011646406,-16.0042102068785,
-219.616286704198));
#204290=CARTESIAN_POINT('Ctrl Pts',(-58.8677062133155,-16.5440407393228,
-216.264438214748));
#204291=CARTESIAN_POINT('Ctrl Pts',(-61.0849434643637,-17.0826855313617,
-212.912555156691));
#204292=CARTESIAN_POINT('Ctrl Pts',(-47.7783900662832,-13.8713871446584,
-233.022972933189));
#204293=CARTESIAN_POINT('Ctrl Pts',(-49.9924469184794,-14.4274016342853,
-229.671258688898));
#204294=CARTESIAN_POINT('Ctrl Pts',(-52.2077820506802,-14.9779386235856,
-226.319510892586));
#204295=CARTESIAN_POINT('Ctrl Pts',(-54.423580209151,-15.5262479876512,
-222.967711846576));
#204296=CARTESIAN_POINT('Ctrl Pts',(-56.6393783676217,-16.0745573517168,
-219.615912800565));
#204297=CARTESIAN_POINT('Ctrl Pts',(-58.8556879728042,-16.6204700248875,
-216.264067401558));
#204298=CARTESIAN_POINT('Ctrl Pts',(-61.0722383017368,-17.1651742681581,
-212.91218728226));
#204299=CARTESIAN_POINT('Ctrl Pts',(-47.7697469949171,-13.9169620127152,
-233.022593985349));
#204300=CARTESIAN_POINT('Ctrl Pts',(-49.983000674726,-14.4792632474105,
-229.670877481921));
#204301=CARTESIAN_POINT('Ctrl Pts',(-52.1975814320602,-15.0359776440825,
-226.319131772858));
#204302=CARTESIAN_POINT('Ctrl Pts',(-54.4126422197256,-15.5904219929251,
-222.967335049774));
#204303=CARTESIAN_POINT('Ctrl Pts',(-56.627703007391,-16.1448663417677,
-219.615538326691));
#204304=CARTESIAN_POINT('Ctrl Pts',(-58.8432942103714,-16.6968678996294,
-216.263695872058));
#204305=CARTESIAN_POINT('Ctrl Pts',(-61.0591348703587,-17.2476384491985,
-212.91181857376));
#204306=CARTESIAN_POINT('Ctrl Pts',(-47.7654254592341,-13.9397494467436,
-233.022404511428));
#204307=CARTESIAN_POINT('Ctrl Pts',(-49.9782775528494,-14.5051940539731,
-229.670686878432));
#204308=CARTESIAN_POINT('Ctrl Pts',(-52.1924811227502,-15.064997154331,
-226.318942212994));
#204309=CARTESIAN_POINT('Ctrl Pts',(-54.4071732250129,-15.6225089955621,
-222.967146651374));
#204310=CARTESIAN_POINT('Ctrl Pts',(-56.6218653272756,-16.1800208367931,
-219.615351089753));
#204311=CARTESIAN_POINT('Ctrl Pts',(-58.8370973291551,-16.7350668370003,
-216.263510107308));
#204312=CARTESIAN_POINT('Ctrl Pts',(-61.0525831546696,-17.2888705397188,
-212.911634219511));
#204313=CARTESIAN_POINT('Ctrl Pts',(-47.7610398192893,-13.962520682369,
-233.022215220766));
#204314=CARTESIAN_POINT('Ctrl Pts',(-49.973483994075,-14.5311103567258,
-229.670496316751));
#204315=CARTESIAN_POINT('Ctrl Pts',(-52.1873044032685,-15.0940037951854,
-226.318752623187));
#204316=CARTESIAN_POINT('Ctrl Pts',(-54.4016219548089,-15.6545847941602,
-222.9669581666));
#204317=CARTESIAN_POINT('Ctrl Pts',(-56.6159395063494,-16.2151657931349,
-219.615163710013));
#204318=CARTESIAN_POINT('Ctrl Pts',(-58.8308065673522,-16.7732579216688,
-216.263324163236));
#204319=CARTESIAN_POINT('Ctrl Pts',(-61.0459318716081,-17.3300964912969,
-212.911449656498));
#204320=CARTESIAN_POINT('Ctrl Pts',(-47.7565902716679,-13.9852750117499,
-233.022026107165));
#204321=CARTESIAN_POINT('Ctrl Pts',(-49.9686201309427,-14.5570115979937,
-229.670305792423));
#204322=CARTESIAN_POINT('Ctrl Pts',(-52.1820513513198,-15.1229971351898,
-226.318563001159));
#204323=CARTESIAN_POINT('Ctrl Pts',(-54.3959884334715,-15.6866490761195,
-222.966769594939));
#204324=CARTESIAN_POINT('Ctrl Pts',(-56.6099255156231,-16.2503010170492,
-219.614976188718));
#204325=CARTESIAN_POINT('Ctrl Pts',(-58.8244218448074,-16.8114410702517,
-216.26313804258));
#204326=CARTESIAN_POINT('Ctrl Pts',(-61.0391808904015,-17.371316327283,
-212.911264888718));
#204327=CARTESIAN_POINT('Ctrl Pts',(-47.7543654978573,-13.9966521764404,
-233.021931550365));
#204328=CARTESIAN_POINT('Ctrl Pts',(-49.9661881993766,-14.5699622186276,
-229.67021053026));
#204329=CARTESIAN_POINT('Ctrl Pts',(-52.1794248253455,-15.137493805192,
-226.318468190145));
#204330=CARTESIAN_POINT('Ctrl Pts',(-54.3931716728027,-15.7026812170992,
-222.966675309108));
#204331=CARTESIAN_POINT('Ctrl Pts',(-56.60691852026,-16.2678686290064,-219.614882428071));
#204332=CARTESIAN_POINT('Ctrl Pts',(-58.821229483535,-16.8305326445432,
-216.263044982252));
#204333=CARTESIAN_POINT('Ctrl Pts',(-61.0358053997983,-17.391926245276,
-212.911172504828));
#204334=CARTESIAN_POINT('Ctrl Pts',(-47.7521247471819,-14.008025114576,
-233.021837037822));
#204335=CARTESIAN_POINT('Ctrl Pts',(-49.9637386917516,-14.5829090738954,
-229.670115277422));
#204336=CARTESIAN_POINT('Ctrl Pts',(-52.1767792162729,-15.1519871499853,
-226.318373371061));
#204337=CARTESIAN_POINT('Ctrl Pts',(-54.3903343493595,-15.7187104789216,
-222.966581001541));
#204338=CARTESIAN_POINT('Ctrl Pts',(-56.6038894824462,-16.2854338078579,
-219.61478863202));
#204339=CARTESIAN_POINT('Ctrl Pts',(-58.8180136320704,-16.8496222348139,
-216.262951877763));
#204340=CARTESIAN_POINT('Ctrl Pts',(-61.0324049846472,-17.4125346343709,
-212.91108006973));
#204341=CARTESIAN_POINT('Ctrl Pts',(-47.7498680445413,-14.0193937377161,
-233.021742568709));
#204342=CARTESIAN_POINT('Ctrl Pts',(-49.9612716248183,-14.5958520941202,
-229.670020033279));
#204343=CARTESIAN_POINT('Ctrl Pts',(-52.1741145339256,-15.1664771156592,
-226.318278543544));
#204344=CARTESIAN_POINT('Ctrl Pts',(-54.3874764662403,-15.7347368225257,
-222.966486672088));
#204345=CARTESIAN_POINT('Ctrl Pts',(-56.600838398555,-16.3029965293923,
-219.614694800631));
#204346=CARTESIAN_POINT('Ctrl Pts',(-58.8147742803545,-16.8687098306404,
-216.262858729364));
#204347=CARTESIAN_POINT('Ctrl Pts',(-61.0289796285328,-17.4331414974815,
-212.910987583833));
#204348=CARTESIAN_POINT('Ctrl Pts',(-47.7476113419008,-14.0307623608562,
-233.021648099596));
#204349=CARTESIAN_POINT('Ctrl Pts',(-49.9588045578851,-14.6087951143449,
-229.669924789137));
#204350=CARTESIAN_POINT('Ctrl Pts',(-52.1714498515783,-15.180967081333,
-226.318183716026));
#204351=CARTESIAN_POINT('Ctrl Pts',(-54.3846185831211,-15.7507631661298,
-222.966392342634));
#204352=CARTESIAN_POINT('Ctrl Pts',(-56.5977873146637,-16.3205592509265,
-219.614600969242));
#204353=CARTESIAN_POINT('Ctrl Pts',(-58.8115349286387,-16.887797426467,
-216.262765580964));
#204354=CARTESIAN_POINT('Ctrl Pts',(-61.0255542724185,-17.4537483605921,
-212.910895097936));
#204355=CARTESIAN_POINT('Ctrl Pts',(-47.7442016228112,-14.0473500394083,
-233.021665980788));
#204356=CARTESIAN_POINT('Ctrl Pts',(-49.9552695851286,-14.62672636609,-229.669960086485));
#204357=CARTESIAN_POINT('Ctrl Pts',(-52.167771235297,-15.2002885297448,
-226.318229365726));
#204358=CARTESIAN_POINT('Ctrl Pts',(-54.3807900271312,-15.7714932773578,
-222.966446178071));
#204359=CARTESIAN_POINT('Ctrl Pts',(-56.5938088189654,-16.3426980249709,
-219.614662990416));
#204360=CARTESIAN_POINT('Ctrl Pts',(-58.8073994401649,-16.9113648377023,
-216.262833288602));
#204361=CARTESIAN_POINT('Ctrl Pts',(-61.0212585846625,-17.4787543086446,
-212.910967436579));
#204362=CARTESIAN_POINT('Ctrl Pts',(-47.7411284099535,-14.0625507697344,
-233.021657357818));
#204363=CARTESIAN_POINT('Ctrl Pts',(-49.9520501521893,-14.6433321699676,
-229.669963755451));
#204364=CARTESIAN_POINT('Ctrl Pts',(-52.164395575698,-15.2183262074345,
-226.318240561216));
#204365=CARTESIAN_POINT('Ctrl Pts',(-54.3772547239517,-15.7909735318649,
-222.966463366842));
#204366=CARTESIAN_POINT('Ctrl Pts',(-56.5901138722054,-16.3636208562953,
-219.614686172468));
#204367=CARTESIAN_POINT('Ctrl Pts',(-58.8035410200603,-16.9337418020372,
-216.262860718253));
#204368=CARTESIAN_POINT('Ctrl Pts',(-61.0172349543283,-17.5025911610169,
-212.910998351897));
#204369=CARTESIAN_POINT('Ctrl Pts',(-47.7165427070916,-14.1841566123428,
-233.021588374054));
#204370=CARTESIAN_POINT('Ctrl Pts',(-49.9262946886754,-14.7761786009886,
-229.669993107177));
#204371=CARTESIAN_POINT('Ctrl Pts',(-52.1373902989064,-15.3626276289524,
-226.318330125135));
#204372=CARTESIAN_POINT('Ctrl Pts',(-54.3489722985157,-15.9468155679217,
-222.966600877007));
#204373=CARTESIAN_POINT('Ctrl Pts',(-56.560554298125,-16.531003506891,-219.614871628879));
#204374=CARTESIAN_POINT('Ctrl Pts',(-58.7726736592232,-17.1127575167165,
-216.263080155467));
#204375=CARTESIAN_POINT('Ctrl Pts',(-60.9850459116547,-17.6932859799952,
-212.911245674445));
#204376=CARTESIAN_POINT('Ctrl Pts',(-47.6932284506644,-14.3060363961889,
-233.021682926744));
#204377=CARTESIAN_POINT('Ctrl Pts',(-49.901885438682,-14.9092956442213,
-229.670173308391));
#204378=CARTESIAN_POINT('Ctrl Pts',(-52.1118097264559,-15.507193974503,
-226.318562347407));
#204379=CARTESIAN_POINT('Ctrl Pts',(-54.3221941272102,-16.1029162862599,
-222.966874425379));
#204380=CARTESIAN_POINT('Ctrl Pts',(-56.5325785279645,-16.6986385980169,
-219.615186503351));
#204381=CARTESIAN_POINT('Ctrl Pts',(-58.7434709011157,-17.2920187463379,
-216.263424143813));
#204382=CARTESIAN_POINT('Ctrl Pts',(-60.9546027715979,-17.8842191820846,
-212.911613494952));
#204383=CARTESIAN_POINT('Ctrl Pts',(-47.6711899624377,-14.4281659124299,
-233.021940707592));
#204384=CARTESIAN_POINT('Ctrl Pts',(-49.8788265984679,-15.0426590253955,
-229.670504307963));
#204385=CARTESIAN_POINT('Ctrl Pts',(-52.0876575029478,-15.6520019918285,
-226.318937245156));
#204386=CARTESIAN_POINT('Ctrl Pts',(-54.296923205648,-16.259253814469,-222.967284070276));
#204387=CARTESIAN_POINT('Ctrl Pts',(-56.5061889083483,-16.8665056371095,
-219.615630895396));
#204388=CARTESIAN_POINT('Ctrl Pts',(-58.7159343195776,-17.4715067819979,
-216.263892782403));
#204389=CARTESIAN_POINT('Ctrl Pts',(-60.9259062922535,-18.0753740181923,
-212.912101903999));
#204390=CARTESIAN_POINT('Ctrl Pts',(-47.6271129859842,-14.672424944912,
-233.022456269286));
#204391=CARTESIAN_POINT('Ctrl Pts',(-49.8327089180398,-15.3093857877439,
-229.671166307109));
#204392=CARTESIAN_POINT('Ctrl Pts',(-52.0393530559316,-15.9416180264796,
-226.319687040658));
#204393=CARTESIAN_POINT('Ctrl Pts',(-54.2463813625237,-16.5719288708872,
-222.968103360071));
#204394=CARTESIAN_POINT('Ctrl Pts',(-56.4534096691157,-17.2022397152948,
-219.616519679485));
#204395=CARTESIAN_POINT('Ctrl Pts',(-58.6608611565012,-17.830482853318,
-216.264830059583));
#204396=CARTESIAN_POINT('Ctrl Pts',(-60.8685133335648,-18.4576836904079,
-212.913078722092));
#204397=CARTESIAN_POINT('Ctrl Pts',(-47.5881385453956,-14.9176828178641,
-233.023623696835));
#204398=CARTESIAN_POINT('Ctrl Pts',(-49.7919925129992,-15.5770978463543,
-229.672430710276));
#204399=CARTESIAN_POINT('Ctrl Pts',(-51.9967617280187,-16.2322007103616,
-226.321006893536));
#204400=CARTESIAN_POINT('Ctrl Pts',(-54.2018683085728,-16.8855511423113,
-222.96946650484));
#204401=CARTESIAN_POINT('Ctrl Pts',(-56.4069748891269,-17.538901574261,
-219.617926116144));
#204402=CARTESIAN_POINT('Ctrl Pts',(-58.6124525981959,-18.1903661459459,
-216.266265596097));
#204403=CARTESIAN_POINT('Ctrl Pts',(-60.8181069486676,-18.8408799020897,
-212.914537613908));
#204404=CARTESIAN_POINT('Ctrl Pts',(-47.554307632397,-15.1637468311187,
-233.025453073475));
#204405=CARTESIAN_POINT('Ctrl Pts',(-49.7567152646595,-15.8456016742832,
-229.674306559616));
#204406=CARTESIAN_POINT('Ctrl Pts',(-51.9599159483462,-16.5235645049904,
-226.322904658655));
#204407=CARTESIAN_POINT('Ctrl Pts',(-54.1634104836589,-17.1999459798668,
-222.971380331423));
#204408=CARTESIAN_POINT('Ctrl Pts',(-56.3669050189717,-17.8763274547433,
-219.619856004191));
#204409=CARTESIAN_POINT('Ctrl Pts',(-58.5707224241369,-18.5510070650469,
-216.268204278443));
#204410=CARTESIAN_POINT('Ctrl Pts',(-60.7746940090617,-19.2248286528632,
-212.916482666117));
#204411=CARTESIAN_POINT('Ctrl Pts',(-47.4866458063998,-15.6558748576279,
-233.029111826755));
#204412=CARTESIAN_POINT('Ctrl Pts',(-49.68616076798,-16.3826093301408,-229.678058258297));
#204413=CARTESIAN_POINT('Ctrl Pts',(-51.8862243890013,-17.1062920942477,
-226.326700188893));
#204414=CARTESIAN_POINT('Ctrl Pts',(-54.0864948338312,-17.8287356549779,
-222.97520798459));
#204415=CARTESIAN_POINT('Ctrl Pts',(-56.2867652786612,-18.551179215708,
-219.623715780286));
#204416=CARTESIAN_POINT('Ctrl Pts',(-58.4872620760191,-19.2722889032489,
-216.272081643134));
#204417=CARTESIAN_POINT('Ctrl Pts',(-60.6878681298499,-19.9927261544104,
-212.920372770536));
#204418=CARTESIAN_POINT('Ctrl Pts',(-47.4396210333615,-16.1511579441859,
-233.035417077088));
#204419=CARTESIAN_POINT('Ctrl Pts',(-49.6374078624443,-16.9227386754765,
-229.684254369749));
#204420=CARTESIAN_POINT('Ctrl Pts',(-51.835544167002,-17.6921151741007,
-226.332805980913));
#204421=CARTESIAN_POINT('Ctrl Pts',(-54.0338142213281,-18.4605999037604,
-222.98123698552));
#204422=CARTESIAN_POINT('Ctrl Pts',(-56.2320842756543,-19.2290846334201,
-219.629667990126));
#204423=CARTESIAN_POINT('Ctrl Pts',(-58.4305002120414,-19.9966086767195,
-216.277970249807));
#204424=CARTESIAN_POINT('Ctrl Pts',(-60.6289872337381,-20.7636493692889,
-212.926206211883));
#204425=CARTESIAN_POINT('Ctrl Pts',(-47.4134504259477,-16.6473487128058,
-233.044455194982));
#204426=CARTESIAN_POINT('Ctrl Pts',(-49.6106642054098,-17.4639704569693,
-229.692980964189));
#204427=CARTESIAN_POINT('Ctrl Pts',(-51.808075938482,-18.2792435060293,
-226.341309714209));
#204428=CARTESIAN_POINT('Ctrl Pts',(-54.0055642141686,-19.0939722550291,
-222.989556757961));
#204429=CARTESIAN_POINT('Ctrl Pts',(-56.2030524898552,-19.9087010040289,
-219.637803801712));
#204430=CARTESIAN_POINT('Ctrl Pts',(-58.4006240585482,-20.7228430676927,
-216.285963294552));
#204431=CARTESIAN_POINT('Ctrl Pts',(-60.5982364662104,-21.5366903458251,
-212.934078132851));
#204432=CARTESIAN_POINT('Ctrl Pts',(-47.3611092111201,-17.6397302500457,
-233.062531430769));
#204433=CARTESIAN_POINT('Ctrl Pts',(-49.5571768913406,-18.5464340199547,
-229.71043415307));
#204434=CARTESIAN_POINT('Ctrl Pts',(-51.753139481442,-19.4535001698865,
-226.358317180801));
#204435=CARTESIAN_POINT('Ctrl Pts',(-53.9490641998496,-20.3607169575665,
-223.006196302843));
#204436=CARTESIAN_POINT('Ctrl Pts',(-56.1449889182572,-21.2679337452465,
-219.654075424885));
#204437=CARTESIAN_POINT('Ctrl Pts',(-58.3408717515618,-22.175311849639,
-216.301949384044));
#204438=CARTESIAN_POINT('Ctrl Pts',(-60.5367349311551,-23.0827722988975,
-212.949821974785));
#204439=CARTESIAN_POINT('Ctrl Pts',(-47.3924301901722,-18.6362326223204,
-233.091564811217));
#204440=CARTESIAN_POINT('Ctrl Pts',(-49.5919089377565,-19.6336206651606,
-229.73800885476));
#204441=CARTESIAN_POINT('Ctrl Pts',(-51.7911544990196,-20.633178776548,
-226.384892671102));
#204442=CARTESIAN_POINT('Ctrl Pts',(-53.9903074147697,-21.6336083947046,
-223.031955741188));
#204443=CARTESIAN_POINT('Ctrl Pts',(-56.1894603305198,-22.6340380128611,
-219.679018811274));
#204444=CARTESIAN_POINT('Ctrl Pts',(-58.3885128958421,-23.6354079399365,
-216.326274549018));
#204445=CARTESIAN_POINT('Ctrl Pts',(-60.5875151336786,-24.637248848966,
-212.973627321642));
#204446=CARTESIAN_POINT('Ctrl Pts',(-47.5062945476757,-19.6195995248629,
-233.133241732319));
#204447=CARTESIAN_POINT('Ctrl Pts',(-49.7144600590333,-20.7098790140667,
-229.777291719128));
#204448=CARTESIAN_POINT('Ctrl Pts',(-51.9225250540634,-21.8042698865183,
-226.422628306549));
#204449=CARTESIAN_POINT('Ctrl Pts',(-54.1305210352282,-22.9002472192685,
-223.06844144768));
#204450=CARTESIAN_POINT('Ctrl Pts',(-56.3385170163929,-23.9962245520186,
-219.714254588812));
#204451=CARTESIAN_POINT('Ctrl Pts',(-58.5464456271153,-25.0939292676188,
-216.360591734734));
#204452=CARTESIAN_POINT('Ctrl Pts',(-60.7543325255676,-26.1924804157199,
-213.007179917814));
#204453=CARTESIAN_POINT('Ctrl Pts',(-47.5205275923637,-19.7425203876807,
-233.138451347457));
#204454=CARTESIAN_POINT('Ctrl Pts',(-49.7297789491929,-20.8444113076799,
-229.782202077174));
#204455=CARTESIAN_POINT('Ctrl Pts',(-51.9389463734439,-21.9506562752646,
-226.42734526098));
#204456=CARTESIAN_POINT('Ctrl Pts',(-54.1480477377855,-23.0585770723389,
-223.073002160992));
#204457=CARTESIAN_POINT('Ctrl Pts',(-56.3571491021271,-24.1664978694133,
-219.718659061004));
#204458=CARTESIAN_POINT('Ctrl Pts',(-58.5661872185244,-25.276244433579,
-216.364881382949));
#204459=CARTESIAN_POINT('Ctrl Pts',(-60.7751846995537,-26.3868843615641,
-213.011373992336));
#204460=CARTESIAN_POINT('Ctrl Pts',(-47.5360446986138,-19.8652437656123,
-233.143861532478));
#204461=CARTESIAN_POINT('Ctrl Pts',(-49.7464660141853,-20.9787779864532,
-229.787297715501));
#204462=CARTESIAN_POINT('Ctrl Pts',(-51.9568241644486,-22.0969116538416,
-226.432238588131));
#204463=CARTESIAN_POINT('Ctrl Pts',(-54.1671204241435,-23.2168106787515,
-223.077732193586));
#204464=CARTESIAN_POINT('Ctrl Pts',(-56.3774166838384,-24.3367097036616,
-219.723225799041));
#204465=CARTESIAN_POINT('Ctrl Pts',(-58.5876552513978,-25.4585332815125,
-216.369328422911));
#204466=CARTESIAN_POINT('Ctrl Pts',(-60.7978548655404,-26.5812970894946,
-213.015721487035));
#204467=CARTESIAN_POINT('Ctrl Pts',(-47.552840900575,-19.9877453892004,
-233.149480158731));
#204468=CARTESIAN_POINT('Ctrl Pts',(-49.764518524335,-21.1129544864435,
-229.792585026173));
#204469=CARTESIAN_POINT('Ctrl Pts',(-51.976158307113,-22.2430122546447,
-226.437313966284));
#204470=CARTESIAN_POINT('Ctrl Pts',(-54.1877416326195,-23.3749253815565,
-223.082636672215));
#204471=CARTESIAN_POINT('Ctrl Pts',(-56.399324958126,-24.5068385084684,
-219.727959378147));
#204472=CARTESIAN_POINT('Ctrl Pts',(-58.6108576613275,-25.6407757471239,
-216.373937091928));
#204473=CARTESIAN_POINT('Ctrl Pts',(-60.8223537175678,-26.7757001729515,
-213.02022637406));
#204474=CARTESIAN_POINT('Ctrl Pts',(-47.5612390015556,-20.0489962009945,
-233.152289471859));
#204475=CARTESIAN_POINT('Ctrl Pts',(-49.7735447794099,-21.1800427364387,
-229.795228681509));
#204476=CARTESIAN_POINT('Ctrl Pts',(-51.9858253784452,-22.3160625550462,
-226.43985165536));
#204477=CARTESIAN_POINT('Ctrl Pts',(-54.1980522368575,-23.453982732959,
-223.08508891153));
#204478=CARTESIAN_POINT('Ctrl Pts',(-56.4102790952697,-24.5919029108718,
-219.730326167701));
#204479=CARTESIAN_POINT('Ctrl Pts',(-58.6224588662923,-25.7318969799296,
-216.376241426438));
#204480=CARTESIAN_POINT('Ctrl Pts',(-60.8346031435815,-26.87290171468,-213.022478817573));
#204481=CARTESIAN_POINT('Ctrl Pts',(-47.5699568885701,-20.1101915733302,
-233.155150913204));
#204482=CARTESIAN_POINT('Ctrl Pts',(-49.7829124042595,-21.2470834394385,
-229.797920267832));
#204483=CARTESIAN_POINT('Ctrl Pts',(-51.9958565445205,-22.3890741581773,
-226.44243486757));
#204484=CARTESIAN_POINT('Ctrl Pts',(-54.2087499771628,-23.5330103552298,
-223.087584770755));
#204485=CARTESIAN_POINT('Ctrl Pts',(-56.421643409805,-24.6769465522823,
-219.732734673941));
#204486=CARTESIAN_POINT('Ctrl Pts',(-58.6344936689916,-25.8230066133188,
-216.378586173355));
#204487=CARTESIAN_POINT('Ctrl Pts',(-60.847309743967,-26.9701008413005,
-213.024770613288));
#204488=CARTESIAN_POINT('Ctrl Pts',(-47.5789940164766,-20.1713284656181,
-233.15806557645));
#204489=CARTESIAN_POINT('Ctrl Pts',(-49.7926211103158,-21.3140735095608,
-229.800660662664));
#204490=CARTESIAN_POINT('Ctrl Pts',(-52.0062518326129,-22.4620440746829,
-226.445064375697));
#204491=CARTESIAN_POINT('Ctrl Pts',(-54.2198352050027,-23.6120053955637,
-223.090124941524));
#204492=CARTESIAN_POINT('Ctrl Pts',(-56.4334185773924,-24.7619667164447,
-219.735185507351));
#204493=CARTESIAN_POINT('Ctrl Pts',(-58.6469630826069,-25.9141021151943,
-216.380971893111));
#204494=CARTESIAN_POINT('Ctrl Pts',(-60.8604748729077,-27.0672952246279,
-213.027102282233));
#204495=CARTESIAN_POINT('Ctrl Pts',(-47.5812532984532,-20.1866126886901,
-233.158794242262));
#204496=CARTESIAN_POINT('Ctrl Pts',(-49.7950482868299,-21.3308210270913,
-229.801345761373));
#204497=CARTESIAN_POINT('Ctrl Pts',(-52.0088506546361,-22.4802865538093,
-226.445721752729));
#204498=CARTESIAN_POINT('Ctrl Pts',(-54.2226065119627,-23.6317541556473,
-223.090759984216));
#204499=CARTESIAN_POINT('Ctrl Pts',(-56.4363623692893,-24.7832217574852,
-219.735798215704));
#204500=CARTESIAN_POINT('Ctrl Pts',(-58.6500804360107,-25.9368759906632,
-216.38156832305));
#204501=CARTESIAN_POINT('Ctrl Pts',(-60.8637661551428,-27.0915938204597,
-213.027685199469));
#204502=CARTESIAN_POINT('Ctrl Pts',(-47.5835325332411,-20.2018932567312,
-233.159526234808));
#204503=CARTESIAN_POINT('Ctrl Pts',(-49.7974967810963,-21.3475653800119,
-229.802033910872));
#204504=CARTESIAN_POINT('Ctrl Pts',(-52.011472234427,-22.4985264274573,
-226.446382023462));
#204505=CARTESIAN_POINT('Ctrl Pts',(-54.2254020370079,-23.6515008792884,
-223.091397796547));
#204506=CARTESIAN_POINT('Ctrl Pts',(-56.4393318395888,-24.8044753311196,
-219.73641356963));
#204507=CARTESIAN_POINT('Ctrl Pts',(-58.6532249526671,-25.9596489828307,
-216.382167313891));
#204508=CARTESIAN_POINT('Ctrl Pts',(-60.8670860954703,-27.1158921197517,
-213.028270608861));
#204509=CARTESIAN_POINT('Ctrl Pts',(-47.5858317128383,-20.2171701221733,
-233.160261571908));
#204510=CARTESIAN_POINT('Ctrl Pts',(-49.7999665889626,-21.3643065199923,
-229.802725125393));
#204511=CARTESIAN_POINT('Ctrl Pts',(-52.0141165726974,-22.5167636487862,
-226.447045200389));
#204512=CARTESIAN_POINT('Ctrl Pts',(-54.22822178586,-23.6712455217665,-223.092038389655));
#204513=CARTESIAN_POINT('Ctrl Pts',(-56.4423269990226,-24.8257273947467,
-219.737031578921));
#204514=CARTESIAN_POINT('Ctrl Pts',(-58.6563966485487,-25.9824210519681,
-216.382768874591));
#204515=CARTESIAN_POINT('Ctrl Pts',(-60.8704347151645,-27.140190085957,
-213.028858518708));
#204516=CARTESIAN_POINT('Ctrl Pts',(-47.5869813026369,-20.2248085548944,
-233.160629240458));
#204517=CARTESIAN_POINT('Ctrl Pts',(-49.8012014928958,-21.3726770899824,
-229.803070732654));
#204518=CARTESIAN_POINT('Ctrl Pts',(-52.0154387418326,-22.5258822594507,
-226.447376788852));
#204519=CARTESIAN_POINT('Ctrl Pts',(-54.2296316602861,-23.6811178430054,
-223.092358686209));
#204520=CARTESIAN_POINT('Ctrl Pts',(-56.4438245787395,-24.8363534265602,
-219.737340583566));
#204521=CARTESIAN_POINT('Ctrl Pts',(-58.6579824964894,-25.9938070865368,
-216.383069654941));
#204522=CARTESIAN_POINT('Ctrl Pts',(-60.8721090250117,-27.1523390690596,
-213.029152473631));
#204523=CARTESIAN_POINT('Ctrl Pts',(-47.5882003780178,-20.2289848114109,
-233.159841710208));
#204524=CARTESIAN_POINT('Ctrl Pts',(-49.8025239788324,-21.3777302901863,
-229.80232330561));
#204525=CARTESIAN_POINT('Ctrl Pts',(-52.016858339954,-22.5317814550976,
-226.446655795734));
#204526=CARTESIAN_POINT('Ctrl Pts',(-54.2311466126926,-23.6878505920434,
-223.091659114758));
#204527=CARTESIAN_POINT('Ctrl Pts',(-56.4454348854312,-24.8439197289892,
-219.736662433782));
#204528=CARTESIAN_POINT('Ctrl Pts',(-58.6596860711528,-26.0021935301855,
-216.382407404553));
#204529=CARTESIAN_POINT('Ctrl Pts',(-60.8739050401878,-27.1615389533073,
-213.028503498334));
#204530=CARTESIAN_POINT('Ctrl Pts',(-47.5893856011509,-20.2345630906963,
-233.159521876246));
#204531=CARTESIAN_POINT('Ctrl Pts',(-49.8038047411002,-21.384127338717,
-229.802018401381));
#204532=CARTESIAN_POINT('Ctrl Pts',(-52.0182317111982,-22.5389852621582,
-226.446360938398));
#204533=CARTESIAN_POINT('Ctrl Pts',(-54.2326117356213,-23.695856045427,
-223.091372426396));
#204534=CARTESIAN_POINT('Ctrl Pts',(-56.4469917600444,-24.8527268286958,
-219.736383914393));
#204535=CARTESIAN_POINT('Ctrl Pts',(-58.661333695373,-26.0117968360436,
-216.38213501004));
#204536=CARTESIAN_POINT('Ctrl Pts',(-60.8756430054541,-27.1719356700459,
-213.028236234081));
#204537=CARTESIAN_POINT('Ctrl Pts',(-47.590570824284,-20.2401413699817,
-233.159202042285));
#204538=CARTESIAN_POINT('Ctrl Pts',(-49.805085503368,-21.3905243872477,
-229.801713497152));
#204539=CARTESIAN_POINT('Ctrl Pts',(-52.0196050824424,-22.5461890692189,
-226.44606608106));
#204540=CARTESIAN_POINT('Ctrl Pts',(-54.23407685855,-23.7038614988106,-223.091085738033));
#204541=CARTESIAN_POINT('Ctrl Pts',(-56.4485486346576,-24.8615339284022,
-219.736105395004));
#204542=CARTESIAN_POINT('Ctrl Pts',(-58.6629813195933,-26.0214001419017,
-216.381862615529));
#204543=CARTESIAN_POINT('Ctrl Pts',(-60.8773809707203,-27.1823323867845,
-213.027968969829));
#204544=CARTESIAN_POINT('Ctrl Pts',(-47.5917520994765,-20.2457201234783,
-233.158882308471));
#204545=CARTESIAN_POINT('Ctrl Pts',(-49.8063619385521,-21.3969222170114,
-229.801408683416));
#204546=CARTESIAN_POINT('Ctrl Pts',(-52.0209737682581,-22.553393946814,
-226.445771304011));
#204547=CARTESIAN_POINT('Ctrl Pts',(-54.235536945469,-23.7118683113933,
-223.090799121214));
#204548=CARTESIAN_POINT('Ctrl Pts',(-56.4501001226798,-24.8703426759725,
-219.735826938416));
#204549=CARTESIAN_POINT('Ctrl Pts',(-58.6646232151106,-26.0310053820113,
-216.38159027621));
#204550=CARTESIAN_POINT('Ctrl Pts',(-60.8791128691258,-27.1927313248522,
-213.027701754131));
#204551=CARTESIAN_POINT('Ctrl Pts',(-47.592929427391,-20.2512993504693,
-233.15856267521));
#204552=CARTESIAN_POINT('Ctrl Pts',(-49.8076340463092,-21.4033208239495,
-229.801103960199));
#204553=CARTESIAN_POINT('Ctrl Pts',(-52.0223377673611,-22.5605998880764,
-226.445476607082));
#204554=CARTESIAN_POINT('Ctrl Pts',(-54.2369919941413,-23.7198764736633,
-223.090512575624));
#204555=CARTESIAN_POINT('Ctrl Pts',(-56.4516462209215,-24.8791530592503,
-219.735548544168));
#204556=CARTESIAN_POINT('Ctrl Pts',(-58.6662593777807,-26.0406125417595,
-216.381317991529));
#204557=CARTESIAN_POINT('Ctrl Pts',(-60.880838695562,-27.2031324672545,
-213.027434586363));
#204558=CARTESIAN_POINT('Ctrl Pts',(-47.5976387390489,-20.2736162584332,
-233.157284142165));
#204559=CARTESIAN_POINT('Ctrl Pts',(-49.8127224773379,-21.4289152517019,
-229.799885067328));
#204560=CARTESIAN_POINT('Ctrl Pts',(-52.0277937637733,-22.5894236531258,
-226.444297819366));
#204561=CARTESIAN_POINT('Ctrl Pts',(-54.2428121888309,-23.7519091227437,
-223.089366393269));
#204562=CARTESIAN_POINT('Ctrl Pts',(-56.4578306138885,-24.9143945923615,
-219.734434967173));
#204563=CARTESIAN_POINT('Ctrl Pts',(-58.6728040284611,-26.079041180752,
-216.380228852809));
#204564=CARTESIAN_POINT('Ctrl Pts',(-60.8877420013067,-27.2447370368634,
-213.02636591529));
#204565=CARTESIAN_POINT('Ctrl Pts',(-47.6022848944595,-20.2959407423872,
-233.156007217897));
#204566=CARTESIAN_POINT('Ctrl Pts',(-49.8177416695991,-21.4545221142991,
-229.798667622657));
#204567=CARTESIAN_POINT('Ctrl Pts',(-52.0331747727777,-22.6182644368655,
-226.443120313462));
#204568=CARTESIAN_POINT('Ctrl Pts',(-54.2485517715197,-23.7839633668058,
-223.088221350469));
#204569=CARTESIAN_POINT('Ctrl Pts',(-56.4639287702618,-24.949662296746,
-219.733322387475));
#204570=CARTESIAN_POINT('Ctrl Pts',(-58.6792569534495,-26.1175005338857,
-216.379140588177));
#204571=CARTESIAN_POINT('Ctrl Pts',(-60.8945481553838,-27.2863768757278,
-213.025298010954));
#204572=CARTESIAN_POINT('Ctrl Pts',(-47.6068679344032,-20.3182727557442,
-233.154731928786));
#204573=CARTESIAN_POINT('Ctrl Pts',(-49.8226916006283,-21.4801411515154,
-229.797451628545));
#204574=CARTESIAN_POINT('Ctrl Pts',(-52.0384807122269,-22.6471217996642,
-226.441944079533));
#204575=CARTESIAN_POINT('Ctrl Pts',(-54.254210599501,-23.8160385972306,
-223.087077428057));
#204576=CARTESIAN_POINT('Ctrl Pts',(-56.4699404867752,-24.984955394797,
-219.732210776581));
#204577=CARTESIAN_POINT('Ctrl Pts',(-58.6856178886063,-26.1559896665116,
-216.378053163374));
#204578=CARTESIAN_POINT('Ctrl Pts',(-60.9012568321316,-27.3280508969457,
-213.024230834597));
#204579=CARTESIAN_POINT('Ctrl Pts',(-47.6435322539531,-20.4969288626005,
-233.144529615889));
#204580=CARTESIAN_POINT('Ctrl Pts',(-49.8622910488621,-21.6850934492459,
-229.78772367565));
#204581=CARTESIAN_POINT('Ctrl Pts',(-52.0809282278205,-22.8779807020543,
-226.432534208105));
#204582=CARTESIAN_POINT('Ctrl Pts',(-54.2994812233516,-24.0726404406297,
-223.077926048768));
#204583=CARTESIAN_POINT('Ctrl Pts',(-56.5180342188827,-25.2673001792052,
-219.723317889431));
#204584=CARTESIAN_POINT('Ctrl Pts',(-58.7365053698609,-26.4639027275198,
-216.369353764958));
#204585=CARTESIAN_POINT('Ctrl Pts',(-60.9549262461142,-27.6614430666891,
-213.015693423744));
#204586=CARTESIAN_POINT('Ctrl Pts',(-47.6761580143262,-20.6760672828885,
-233.134431726961));
#204587=CARTESIAN_POINT('Ctrl Pts',(-49.8974580357697,-21.890825164949,
-229.77808818943));
#204588=CARTESIAN_POINT('Ctrl Pts',(-52.11857127794,-23.1099007208212,-226.423205300924));
#204589=CARTESIAN_POINT('Ctrl Pts',(-54.3395833259005,-24.3305853285644,
-223.068845880567));
#204590=CARTESIAN_POINT('Ctrl Pts',(-56.5605953738609,-25.5512699363075,
-219.714486460211));
#204591=CARTESIAN_POINT('Ctrl Pts',(-58.7815049542864,-26.7737213502237,
-216.36070754227));
#204592=CARTESIAN_POINT('Ctrl Pts',(-61.0023564697282,-27.9970224992499,
-213.007202010553));
#204593=CARTESIAN_POINT('Ctrl Pts',(-47.7047603197491,-20.8556613435138,
-233.124453388251));
#204594=CARTESIAN_POINT('Ctrl Pts',(-49.9281792692869,-22.0972013968281,
-229.768548954079));
#204595=CARTESIAN_POINT('Ctrl Pts',(-52.1513679132233,-23.3426563590316,
-226.413955402434));
#204596=CARTESIAN_POINT('Ctrl Pts',(-54.374445390284,-24.58956219214,-223.059830549548));
#204597=CARTESIAN_POINT('Ctrl Pts',(-56.5975228673448,-25.8364680252484,
-219.705705696663));
#204598=CARTESIAN_POINT('Ctrl Pts',(-58.8204852380101,-27.0849692159872,
-216.352100946617));
#204599=CARTESIAN_POINT('Ctrl Pts',(-61.0433852523227,-28.3342355002131,
-212.998740881412));
#204600=CARTESIAN_POINT('Ctrl Pts',(-47.761964930595,-21.2148494647643,
-233.104496710832));
#204601=CARTESIAN_POINT('Ctrl Pts',(-49.9896217363213,-22.5099538605863,
-229.749470483377));
#204602=CARTESIAN_POINT('Ctrl Pts',(-52.2169611837896,-23.8081676354522,
-226.395455605453));
#204603=CARTESIAN_POINT('Ctrl Pts',(-54.4441695190511,-25.1075159192911,
-223.041799887511));
#204604=CARTESIAN_POINT('Ctrl Pts',(-56.6713778543125,-26.4068642031302,
-219.688144169568));
#204605=CARTESIAN_POINT('Ctrl Pts',(-58.8984458054575,-27.7074649475142,
-216.33488775531));
#204606=CARTESIAN_POINT('Ctrl Pts',(-61.1254428175118,-29.0086615021396,
-212.981818623129));
#204607=CARTESIAN_POINT('Ctrl Pts',(-47.8030826102193,-21.5759569839245,
-233.085053373718));
#204608=CARTESIAN_POINT('Ctrl Pts',(-50.0332812842976,-22.9253020461421,
-229.730786405659));
#204609=CARTESIAN_POINT('Ctrl Pts',(-52.2631570285769,-24.2769902935286,
-226.377264845526));
#204610=CARTESIAN_POINT('Ctrl Pts',(-54.4929077000272,-25.6295283315933,
-223.024008347048));
#204611=CARTESIAN_POINT('Ctrl Pts',(-56.7226583714774,-26.9820663696581,
-219.67075184857));
#204612=CARTESIAN_POINT('Ctrl Pts',(-58.9522730259992,-28.3355440479673,
-216.317789947423));
#204613=CARTESIAN_POINT('Ctrl Pts',(-61.1818210021897,-29.6894673923576,
-212.964966336897));
#204614=CARTESIAN_POINT('Ctrl Pts',(-47.8281547001989,-21.9381226823642,
-233.066054879848));
#204615=CARTESIAN_POINT('Ctrl Pts',(-50.0590295861697,-23.3420565686501,
-229.712518150776));
#204616=CARTESIAN_POINT('Ctrl Pts',(-52.2896542767201,-24.7475525298228,
-226.359471317301));
#204617=CARTESIAN_POINT('Ctrl Pts',(-54.5201844975327,-26.1536136226082,
-223.006599089445));
#204618=CARTESIAN_POINT('Ctrl Pts',(-56.7507147183453,-27.5596747153937,
-219.653726861588));
#204619=CARTESIAN_POINT('Ctrl Pts',(-58.9811415508881,-28.9663610919618,
-216.301048580499));
#204620=CARTESIAN_POINT('Ctrl Pts',(-61.2115183316506,-30.3733436736124,
-212.948461459071));
#204621=CARTESIAN_POINT('Ctrl Pts',(-47.878298880158,-22.6624540792437,
-233.028057892109));
#204622=CARTESIAN_POINT('Ctrl Pts',(-50.1105261899139,-24.1755656136661,
-229.675981641008));
#204623=CARTESIAN_POINT('Ctrl Pts',(-52.3426487730065,-25.6886770024113,
-226.323884260853));
#204624=CARTESIAN_POINT('Ctrl Pts',(-54.5747380925437,-27.201784204638,
-222.971780574238));
#204625=CARTESIAN_POINT('Ctrl Pts',(-56.8068274120809,-28.7148914068648,
-219.619676887624));
#204626=CARTESIAN_POINT('Ctrl Pts',(-59.0388786006661,-30.2279951799507,
-216.267565846653));
#204627=CARTESIAN_POINT('Ctrl Pts',(-61.2709129905723,-31.7410962361218,
-212.915451703421));
#204628=CARTESIAN_POINT('Ctrl Pts',(-47.8643060007033,-23.3916852678342,
-232.992031101241));
#204629=CARTESIAN_POINT('Ctrl Pts',(-50.090369934904,-25.0147380524944,
-229.641119166754));
#204630=CARTESIAN_POINT('Ctrl Pts',(-52.3167608689203,-26.6363742930146,
-226.289781396988));
#204631=CARTESIAN_POINT('Ctrl Pts',(-54.5432642950053,-28.2575096926779,
-222.938292603557));
#204632=CARTESIAN_POINT('Ctrl Pts',(-56.7697677210903,-29.8786450923411,
-219.586803810126));
#204633=CARTESIAN_POINT('Ctrl Pts',(-58.9963973187644,-31.499223086313,
-216.235147117033));
#204634=CARTESIAN_POINT('Ctrl Pts',(-61.2230851874141,-33.1195404004377,
-212.883411876817));
#204635=CARTESIAN_POINT('Ctrl Pts',(-47.7843348584855,-24.1202237497555,
-232.95800139794));
#204636=CARTESIAN_POINT('Ctrl Pts',(-49.99728150262,-25.8497978524297,-229.608138122646));
#204637=CARTESIAN_POINT('Ctrl Pts',(-52.2112045262045,-27.5766829623168,
-226.257539270556));
#204638=CARTESIAN_POINT('Ctrl Pts',(-54.4254782083431,-29.3025655601605,
-222.906657351959));
#204639=CARTESIAN_POINT('Ctrl Pts',(-56.6397518904817,-31.0284481580042,
-219.555775433364));
#204640=CARTESIAN_POINT('Ctrl Pts',(-58.8544142415175,-32.7532300084283,
-216.204585123186));
#204641=CARTESIAN_POINT('Ctrl Pts',(-61.0692598838066,-34.4774822060492,
-212.853243959114));
#204642=CARTESIAN_POINT('Ctrl Pts',(-47.764342072931,-24.3023583702358,
-232.949493972115));
#204643=CARTESIAN_POINT('Ctrl Pts',(-49.974009394549,-26.0585628024136,
-229.599892861619));
#204644=CARTESIAN_POINT('Ctrl Pts',(-52.1848154405255,-27.8117601296424,
-226.249478738948));
#204645=CARTESIAN_POINT('Ctrl Pts',(-54.3960316866775,-29.5638295270311,
-222.898748539061));
#204646=CARTESIAN_POINT('Ctrl Pts',(-56.6072479328295,-31.3158989244199,
-219.548018339173));
#204647=CARTESIAN_POINT('Ctrl Pts',(-58.8189184722057,-33.0667317389572,
-216.196944624725));
#204648=CARTESIAN_POINT('Ctrl Pts',(-61.0308035579046,-34.8169676574521,
-212.845701979688));
#204649=CARTESIAN_POINT('Ctrl Pts',(-47.740213651375,-24.4844399226315,
-232.941108585445));
#204650=CARTESIAN_POINT('Ctrl Pts',(-49.9461781517511,-26.2670695016037,
-229.591763145452));
#204651=CARTESIAN_POINT('Ctrl Pts',(-52.1534586043331,-28.0463810912831,
-226.241533050557));
#204652=CARTESIAN_POINT('Ctrl Pts',(-54.3612152314905,-29.8244384178816,
-222.890954611672));
#204653=CARTESIAN_POINT('Ctrl Pts',(-56.5689718586478,-31.6024957444801,
-219.540376172787));
#204654=CARTESIAN_POINT('Ctrl Pts',(-58.7772552102583,-33.379180627117,
-216.189420287308));
#204655=CARTESIAN_POINT('Ctrl Pts',(-60.9857878512938,-35.1552003357181,
-212.838277543654));
#204656=CARTESIAN_POINT('Ctrl Pts',(-47.7118765658424,-24.6664222949089,
-232.932859181476));
#204657=CARTESIAN_POINT('Ctrl Pts',(-49.9137627052303,-26.4751698404963,
-229.583753063685));
#204658=CARTESIAN_POINT('Ctrl Pts',(-52.1171498878757,-28.280309601158,
-226.233700065929));
#204659=CARTESIAN_POINT('Ctrl Pts',(-54.321084090016,-30.084072222256,-222.883268552734));
#204660=CARTESIAN_POINT('Ctrl Pts',(-56.5250182921564,-31.887834843354,
-219.53283703954));
#204661=CARTESIAN_POINT('Ctrl Pts',(-58.7295564557497,-33.6900941117383,
-216.181996801466));
#204662=CARTESIAN_POINT('Ctrl Pts',(-60.9343814743951,-35.4916209740569,
-212.830952580145));
#204663=CARTESIAN_POINT('Ctrl Pts',(-47.7047922944592,-24.7119178879782,
-232.930796830484));
#204664=CARTESIAN_POINT('Ctrl Pts',(-49.9056588436001,-26.5271949252194,
-229.581750543243));
#204665=CARTESIAN_POINT('Ctrl Pts',(-52.1080727087613,-28.3387917286268,
-226.231741819771));
#204666=CARTESIAN_POINT('Ctrl Pts',(-54.3110513046474,-30.1489806733496,
-222.881347038));
#204667=CARTESIAN_POINT('Ctrl Pts',(-56.5140299005335,-31.9591696180724,
-219.530952256228));
#204668=CARTESIAN_POINT('Ctrl Pts',(-58.7176317671225,-33.7678224828936,
-216.180140930006));
#204669=CARTESIAN_POINT('Ctrl Pts',(-60.9215298801705,-35.5757261336416,
-212.829121339267));
#204670=CARTESIAN_POINT('Ctrl Pts',(-47.6974449417632,-24.7574072627311,
-232.928742990504));
#204671=CARTESIAN_POINT('Ctrl Pts',(-49.8972684550162,-26.5791946079747,
-229.579755520635));
#204672=CARTESIAN_POINT('Ctrl Pts',(-52.0986860379256,-28.3972305774635,
-226.229790640633));
#204673=CARTESIAN_POINT('Ctrl Pts',(-54.3006863636687,-30.2138281843841,
-222.879432289762));
#204674=CARTESIAN_POINT('Ctrl Pts',(-56.5026866894118,-32.0304257913048,
-219.529073938891));
#204675=CARTESIAN_POINT('Ctrl Pts',(-58.705329891559,-33.8454548987401,
-216.178291388644));
#204676=CARTESIAN_POINT('Ctrl Pts',(-60.9082789063849,-35.6597180491639,
-212.827296342558));
#204677=CARTESIAN_POINT('Ctrl Pts',(-47.6898332885707,-24.8028896565292,
-232.926697902178));
#204678=CARTESIAN_POINT('Ctrl Pts',(-49.8885911188174,-26.6311665651389,
-229.577768100455));
#204679=CARTESIAN_POINT('Ctrl Pts',(-52.0889901241519,-28.455622455455,
-226.227846540711));
#204680=CARTESIAN_POINT('Ctrl Pts',(-54.2899901539046,-30.2786097609959,
-222.877524247479));
#204681=CARTESIAN_POINT('Ctrl Pts',(-56.4909901836572,-32.1015970665369,
-219.527201954246));
#204682=CARTESIAN_POINT('Ctrl Pts',(-58.6926529531334,-33.9229838341469,
-216.176447991634));
#204683=CARTESIAN_POINT('Ctrl Pts',(-60.8946312627443,-35.7435879987355,
-212.825477361568));
#204684=CARTESIAN_POINT('Ctrl Pts',(-47.6860274619745,-24.8256308534282,
-232.925675358015));
#204685=CARTESIAN_POINT('Ctrl Pts',(-49.8842524507179,-26.657152543721,
-229.576774390365));
#204686=CARTESIAN_POINT('Ctrl Pts',(-52.0841421672651,-28.4848183944506,
-226.22687449075));
#204687=CARTESIAN_POINT('Ctrl Pts',(-54.2846420490225,-30.3110005493018,
-222.876570226337));
#204688=CARTESIAN_POINT('Ctrl Pts',(-56.4851419307799,-32.1371827041529,
-219.526265961925));
#204689=CARTESIAN_POINT('Ctrl Pts',(-58.6863144839206,-33.9617483018504,
-216.17552629313));
#204690=CARTESIAN_POINT('Ctrl Pts',(-60.887807440924,-35.7855229735214,
-212.824567871073));
#204691=CARTESIAN_POINT('Ctrl Pts',(-47.6821555597811,-24.8483703047961,
-232.924655001894));
#204692=CARTESIAN_POINT('Ctrl Pts',(-49.8798420455288,-26.6831315908415,
-229.575782581129));
#204693=CARTESIAN_POINT('Ctrl Pts',(-52.0792168996413,-28.5140025907287,
-226.225904210874));
#204694=CARTESIAN_POINT('Ctrl Pts',(-54.2792111270821,-30.3433748540391,
-222.875617881988));
#204695=CARTESIAN_POINT('Ctrl Pts',(-56.4792053545228,-32.1727471173495,
-219.525331553101));
#204696=CARTESIAN_POINT('Ctrl Pts',(-58.6798822493665,-34.0004868995374,
-216.174606131045));
#204697=CARTESIAN_POINT('Ctrl Pts',(-60.88088445209,-35.8274274569215,-212.823659884843));
#204698=CARTESIAN_POINT('Ctrl Pts',(-47.6782174267913,-24.8711079134889,
-232.92363686464));
#204699=CARTESIAN_POINT('Ctrl Pts',(-49.8753598495424,-26.7091034156505,
-229.574792687293));
#204700=CARTESIAN_POINT('Ctrl Pts',(-52.0742143523489,-28.5431745827215,
-226.224935704284));
#204701=CARTESIAN_POINT('Ctrl Pts',(-54.2736974997456,-30.3757320511356,
-222.874667208678));
#204702=CARTESIAN_POINT('Ctrl Pts',(-56.4731806471424,-32.2082895195496,
-219.524398713072));
#204703=CARTESIAN_POINT('Ctrl Pts',(-58.6733565172052,-34.0391986871267,
-216.173687484148));
#204704=CARTESIAN_POINT('Ctrl Pts',(-60.8738626376389,-35.8693003593042,
-212.822753376317));
#204705=CARTESIAN_POINT('Ctrl Pts',(-47.6762483602964,-24.8824767178353,
-232.923127796013));
#204706=CARTESIAN_POINT('Ctrl Pts',(-49.8731187515493,-26.722089328055,
-229.574297740375));
#204707=CARTESIAN_POINT('Ctrl Pts',(-52.0717130787027,-28.557760578718,
-226.224451450989));
#204708=CARTESIAN_POINT('Ctrl Pts',(-54.2709406860775,-30.3919106496837,
-222.874191872023));
#204709=CARTESIAN_POINT('Ctrl Pts',(-56.4701682934522,-32.2260607206496,
-219.523932293058));
#204710=CARTESIAN_POINT('Ctrl Pts',(-58.6700936511245,-34.0585545809213,
-216.173228160698));
#204711=CARTESIAN_POINT('Ctrl Pts',(-60.8703517304133,-35.8902368104956,
-212.822300122054));
#204712=CARTESIAN_POINT('Ctrl Pts',(-47.6742627360736,-24.8938450614933,
-232.922619282109));
#204713=CARTESIAN_POINT('Ctrl Pts',(-49.8708597058451,-26.7350734348772,
-229.573803272322));
#204714=CARTESIAN_POINT('Ctrl Pts',(-52.069192485139,-28.5723435236424,
-226.223967641033));
#204715=CARTESIAN_POINT('Ctrl Pts',(-54.2681631960686,-30.4080849713239,
-222.873716953146));
#204716=CARTESIAN_POINT('Ctrl Pts',(-56.4671339069982,-32.2438264190054,
-219.523466265261));
#204717=CARTESIAN_POINT('Ctrl Pts',(-58.666807410665,-34.0779037721973,
-216.172769216067));
#204718=CARTESIAN_POINT('Ctrl Pts',(-60.8668161168113,-35.9111653664389,
-212.821847237238));
#204719=CARTESIAN_POINT('Ctrl Pts',(-47.6722605345507,-24.9052129322023,
-232.922111326828));
#204720=CARTESIAN_POINT('Ctrl Pts',(-49.8685827056453,-26.7480556997355,
-229.573309285042));
#204721=CARTESIAN_POINT('Ctrl Pts',(-52.0666525755381,-28.5869233597964,
-226.223484274919));
#204722=CARTESIAN_POINT('Ctrl Pts',(-54.2653650437259,-30.4242549380612,
-222.873242451443));
#204723=CARTESIAN_POINT('Ctrl Pts',(-56.4640775119137,-32.2615865163259,
-219.523000627968));
#204724=CARTESIAN_POINT('Ctrl Pts',(-58.6634978294311,-34.0972461434794,
-216.172310647723));
#204725=CARTESIAN_POINT('Ctrl Pts',(-60.8632558396737,-35.9320858909674,
-212.821394718674));
#204726=CARTESIAN_POINT('Ctrl Pts',(-47.6712594337893,-24.9108968675569,
-232.921857349187));
#204727=CARTESIAN_POINT('Ctrl Pts',(-49.8674442055454,-26.7545468321646,
-229.573062291402));
#204728=CARTESIAN_POINT('Ctrl Pts',(-52.0653826207377,-28.5942132778735,
-226.223242591862));
#204729=CARTESIAN_POINT('Ctrl Pts',(-54.2639659675545,-30.4323399214299,
-222.873005200592));
#204730=CARTESIAN_POINT('Ctrl Pts',(-56.4625493143714,-32.2704665649863,
-219.522767809321));
#204731=CARTESIAN_POINT('Ctrl Pts',(-58.6618430388141,-34.1069173291204,
-216.172081363551));
#204732=CARTESIAN_POINT('Ctrl Pts',(-60.8614757011049,-35.9425461532316,
-212.821168459392));
#204733=CARTESIAN_POINT('Ctrl Pts',(-47.6708439427048,-24.9151766736244,
-232.921223878144));
#204734=CARTESIAN_POINT('Ctrl Pts',(-49.8668624993017,-26.7596833615473,
-229.572444432014));
#204735=CARTESIAN_POINT('Ctrl Pts',(-52.064650178125,-28.6001828109265,
-226.222636553605));
#204736=CARTESIAN_POINT('Ctrl Pts',(-54.2630886768694,-30.4391324823344,
-222.872409015864));
#204737=CARTESIAN_POINT('Ctrl Pts',(-56.4615271756139,-32.2780821537422,
-219.522181478123));
#204738=CARTESIAN_POINT('Ctrl Pts',(-58.6606824811278,-34.1153452969724,
-216.171502871612));
#204739=CARTESIAN_POINT('Ctrl Pts',(-60.8601798411379,-35.9517810490386,
-212.820596670274));
#204740=CARTESIAN_POINT('Ctrl Pts',(-47.6690974499491,-24.9226147901915,
-232.921444558725));
#204741=CARTESIAN_POINT('Ctrl Pts',(-49.8650134863522,-26.7678656673941,
-229.572661252457));
#204742=CARTESIAN_POINT('Ctrl Pts',(-52.0626926881854,-28.6091201074371,
-226.222850519243));
#204743=CARTESIAN_POINT('Ctrl Pts',(-54.261020613352,-30.4488288829175,
-222.87262061773));
#204744=CARTESIAN_POINT('Ctrl Pts',(-56.4593485385187,-32.2885376583978,
-219.522390716218));
#204745=CARTESIAN_POINT('Ctrl Pts',(-58.65839093571,-34.1265643975113,-216.171710253535));
#204746=CARTESIAN_POINT('Ctrl Pts',(-60.8577743014912,-35.9637659284024,
-212.820802473134));
#204747=CARTESIAN_POINT('Ctrl Pts',(-47.6673509571934,-24.9300529067585,
-232.921665239305));
#204748=CARTESIAN_POINT('Ctrl Pts',(-49.8631644734026,-26.7760479732408,
-229.5728780729));
#204749=CARTESIAN_POINT('Ctrl Pts',(-52.0607351982457,-28.6180574039478,
-226.223064484881));
#204750=CARTESIAN_POINT('Ctrl Pts',(-54.2589525498347,-30.4585252835005,
-222.872832219598));
#204751=CARTESIAN_POINT('Ctrl Pts',(-56.4571699014236,-32.2989931630532,
-219.522599954314));
#204752=CARTESIAN_POINT('Ctrl Pts',(-58.6560993902921,-34.1377834980502,
-216.171917635457));
#204753=CARTESIAN_POINT('Ctrl Pts',(-60.8553687618446,-35.9757508077661,
-212.821008275995));
#204754=CARTESIAN_POINT('Ctrl Pts',(-47.6656092026626,-24.9374924051846,
-232.921886594377));
#204755=CARTESIAN_POINT('Ctrl Pts',(-49.8613205610057,-26.7842316103463,
-229.573095523243));
#204756=CARTESIAN_POINT('Ctrl Pts',(-52.0587831785056,-28.6269959846611,
-226.223279050959));
#204757=CARTESIAN_POINT('Ctrl Pts',(-54.2568903279106,-30.468222923408,
-222.873044397953));
#204758=CARTESIAN_POINT('Ctrl Pts',(-56.4549974773155,-32.3094498621548,
-219.522809744947));
#204759=CARTESIAN_POINT('Ctrl Pts',(-58.6538144314378,-34.1490037503303,
-216.17212555206));
#204760=CARTESIAN_POINT('Ctrl Pts',(-60.8529701831065,-35.987736797489,
-212.821214598585));
#204761=CARTESIAN_POINT('Ctrl Pts',(-47.6638721879803,-24.9449332806664,
-232.922108625287));
#204762=CARTESIAN_POINT('Ctrl Pts',(-49.8594817505659,-26.7924165735007,
-229.57331360468));
#204763=CARTESIAN_POINT('Ctrl Pts',(-52.0568366301129,-28.6359358440905,
-226.223494218563));
#204764=CARTESIAN_POINT('Ctrl Pts',(-54.2548339484627,-30.4779217969194,
-222.873257153795));
#204765=CARTESIAN_POINT('Ctrl Pts',(-56.4528312668125,-32.3199077497483,
-219.523020089027));
#204766=CARTESIAN_POINT('Ctrl Pts',(-58.6515360594894,-34.1602251482123,
-216.172334004182));
#204767=CARTESIAN_POINT('Ctrl Pts',(-60.85057856534,-35.9997238912687,-212.821421441686));
#204768=CARTESIAN_POINT('Ctrl Pts',(-47.6360799530631,-25.0639872883753,
-232.925661119858));
#204769=CARTESIAN_POINT('Ctrl Pts',(-49.8300607835295,-26.9233759839715,
-229.576802907687));
#204770=CARTESIAN_POINT('Ctrl Pts',(-52.0256918558292,-28.7789735949605,
-226.226936900208));
#204771=CARTESIAN_POINT('Ctrl Pts',(-54.2219318772968,-30.6331037731025,
-222.876661247257));
#204772=CARTESIAN_POINT('Ctrl Pts',(-56.4181718987644,-32.4872339512444,
-219.526385594307));
#204773=CARTESIAN_POINT('Ctrl Pts',(-58.6150821083144,-34.339767514325,
-216.175669238136));
#204774=CARTESIAN_POINT('Ctrl Pts',(-60.8123126810755,-36.1915173917436,
-212.824730931321));
#204775=CARTESIAN_POINT('Ctrl Pts',(-47.6095010735459,-25.1833938131447,
-232.929386557426));
#204776=CARTESIAN_POINT('Ctrl Pts',(-49.8019458805959,-27.054674855399,
-229.58045371177));
#204777=CARTESIAN_POINT('Ctrl Pts',(-51.9959477143626,-28.9223386907395,
-226.230533520487));
#204778=CARTESIAN_POINT('Ctrl Pts',(-54.1905254516978,-30.7886015464719,
-222.88021313116));
#204779=CARTESIAN_POINT('Ctrl Pts',(-56.3851031890331,-32.6548644022043,
-219.529892741831));
#204780=CARTESIAN_POINT('Ctrl Pts',(-58.5803143829409,-34.5196031508285,
-216.179141529169));
#204781=CARTESIAN_POINT('Ctrl Pts',(-60.7758287854006,-36.3835935276752,
-212.828173639481));
#204782=CARTESIAN_POINT('Ctrl Pts',(-47.5841424907316,-25.3031332383162,
-232.93329091056));
#204783=CARTESIAN_POINT('Ctrl Pts',(-49.7751430286533,-27.1862918963392,
-229.584271284343));
#204784=CARTESIAN_POINT('Ctrl Pts',(-51.9676091114587,-29.0660086976874,
-226.234288856273));
#204785=CARTESIAN_POINT('Ctrl Pts',(-54.1606184685044,-30.9443917197372,
-222.883917182185));
#204786=CARTESIAN_POINT('Ctrl Pts',(-56.3536278255502,-32.822774741787,
-219.533545508098));
#204787=CARTESIAN_POINT('Ctrl Pts',(-58.5472344262499,-34.6997069346566,
-216.182754549711));
#204788=CARTESIAN_POINT('Ctrl Pts',(-60.7411272633344,-36.5759265044021,
-212.831752983035));
#204789=CARTESIAN_POINT('Ctrl Pts',(-47.4827081594745,-25.7820909390022,
-232.948908323096));
#204790=CARTESIAN_POINT('Ctrl Pts',(-49.667931620883,-27.7127600601,-229.599541574634));
#204791=CARTESIAN_POINT('Ctrl Pts',(-51.854254699843,-29.6406887254791,
-226.249310199414));
#204792=CARTESIAN_POINT('Ctrl Pts',(-54.0409905357308,-31.5675524127984,
-222.898733386289));
#204793=CARTESIAN_POINT('Ctrl Pts',(-56.2277263716187,-33.4944161001178,
-219.548156573164));
#204794=CARTESIAN_POINT('Ctrl Pts',(-58.4149145994856,-35.4201220699693,
-216.197206631876));
#204795=CARTESIAN_POINT('Ctrl Pts',(-60.6023211750695,-37.3452584113098,
-212.84607035725));
#204796=CARTESIAN_POINT('Ctrl Pts',(-47.4007849436546,-26.2663735290611,
-232.967369843972));
#204797=CARTESIAN_POINT('Ctrl Pts',(-49.5817020458226,-28.2443177299668,
-229.617464898372));
#204798=CARTESIAN_POINT('Ctrl Pts',(-51.7633793713291,-30.2202463681864,
-226.266857669841));
#204799=CARTESIAN_POINT('Ctrl Pts',(-53.9453452831587,-32.19539073454,-222.915972481834));
#204800=CARTESIAN_POINT('Ctrl Pts',(-56.1273111949884,-34.1705351008938,
-219.565087293826));
#204801=CARTESIAN_POINT('Ctrl Pts',(-58.3095925631572,-36.1448271352898,
-216.213901211887));
#204802=CARTESIAN_POINT('Ctrl Pts',(-60.4920271624846,-38.1186994663558,
-212.862565596074));
#204803=CARTESIAN_POINT('Ctrl Pts',(-47.338918326904,-26.7547399443242,
-232.989202284253));
#204804=CARTESIAN_POINT('Ctrl Pts',(-49.5169190710851,-28.779613867576,
-229.63849750905));
#204805=CARTESIAN_POINT('Ctrl Pts',(-51.6953679974136,-30.8032553785755,
-226.287341083189));
#204806=CARTESIAN_POINT('Ctrl Pts',(-53.8739882225852,-32.826417079771,
-222.936006744139));
#204807=CARTESIAN_POINT('Ctrl Pts',(-56.0526084477568,-34.8495787809666,
-219.584672405089));
#204808=CARTESIAN_POINT('Ctrl Pts',(-58.2314156201025,-36.8722190976995,
-216.233145260744));
#204809=CARTESIAN_POINT('Ctrl Pts',(-60.4103139494413,-38.8946025877681,
-212.88152253822));
#204810=CARTESIAN_POINT('Ctrl Pts',(-47.0914518599014,-28.7082056053768,
-233.076532045377));
#204811=CARTESIAN_POINT('Ctrl Pts',(-49.2577871721353,-30.9207984180132,
-229.722627951761));
#204812=CARTESIAN_POINT('Ctrl Pts',(-51.4233225017517,-33.1352914201321,
-226.36927473658));
#204813=CARTESIAN_POINT('Ctrl Pts',(-53.588559980291,-35.3505224606949,
-223.016143793358));
#204814=CARTESIAN_POINT('Ctrl Pts',(-55.7537974588302,-37.5657535012578,
-219.663012850137));
#204815=CARTESIAN_POINT('Ctrl Pts',(-57.9187078478837,-39.7817869473385,
-216.310121456173));
#204816=CARTESIAN_POINT('Ctrl Pts',(-60.0834610972678,-41.9982150734171,
-212.9573503068));
#204817=CARTESIAN_POINT('Ctrl Pts',(-47.1654872359782,-30.7268333335968,
-233.215238694904));
#204818=CARTESIAN_POINT('Ctrl Pts',(-49.3424661286879,-33.1216582244425,
-229.854296748355));
#204819=CARTESIAN_POINT('Ctrl Pts',(-51.5175746565146,-35.5225299367126,
-226.496223095384));
#204820=CARTESIAN_POINT('Ctrl Pts',(-53.691970049721,-37.9257105515243,
-223.139241204672));
#204821=CARTESIAN_POINT('Ctrl Pts',(-55.8663654429275,-40.3288911663362,
-219.782259313959));
#204822=CARTESIAN_POINT('Ctrl Pts',(-58.0399820141948,-42.7345941518082,
-216.426471773175));
#204823=CARTESIAN_POINT('Ctrl Pts',(-60.2132186858487,-45.1415311212291,
-213.071269036894));
#204824=CARTESIAN_POINT('Ctrl Pts',(-47.6009947863409,-32.6895605159758,
-233.446187702606));
#204825=CARTESIAN_POINT('Ctrl Pts',(-49.8025157165519,-35.2628848633458,
-230.069700789871));
#204826=CARTESIAN_POINT('Ctrl Pts',(-52.004194845104,-37.8467163541935,
-226.701486649479));
#204827=CARTESIAN_POINT('Ctrl Pts',(-54.2056301169259,-40.4346768564372,
-223.336322656971));
#204828=CARTESIAN_POINT('Ctrl Pts',(-56.4070653887478,-43.0226373586808,
-219.971158664462));
#204829=CARTESIAN_POINT('Ctrl Pts',(-58.6083138625641,-45.6150709680905,
-216.609349785985));
#204830=CARTESIAN_POINT('Ctrl Pts',(-60.8093841578956,-48.2097095522884,
-213.249138279223));
#204831=CARTESIAN_POINT('',(-47.7643893940416,6.45775162350445,-232.249941470498));
#204832=CARTESIAN_POINT('Ctrl Pts',(-47.7643209769699,6.45773201240538,
-232.25005));
#204833=CARTESIAN_POINT('Ctrl Pts',(-47.742487483556,6.0248506060618,-232.25005));
#204834=CARTESIAN_POINT('Ctrl Pts',(-47.7367469535682,5.59139851916973,
-232.250049999992));
#204835=CARTESIAN_POINT('Ctrl Pts',(-47.7578535444487,4.72659631822721,
-232.250049999992));
#204836=CARTESIAN_POINT('Ctrl Pts',(-47.7845553907336,4.29572876651442,
-232.25005));
#204837=CARTESIAN_POINT('Ctrl Pts',(-47.8275275119679,3.86645886896242,
-232.25005));
#204838=CARTESIAN_POINT('Ctrl Pts',(-47.7644582781562,6.45775343049303,
-232.249941470498));
#204839=CARTESIAN_POINT('Ctrl Pts',(-47.7644427531638,6.45834525788562,
-232.249977646999));
#204840=CARTESIAN_POINT('Ctrl Pts',(-47.7644272274041,6.45893708525808,
-232.2500138235));
#204841=CARTESIAN_POINT('Ctrl Pts',(-47.7644117008771,6.45952891261041,
-232.25005));
#204842=CARTESIAN_POINT('',(-47.7598796740376,-29.6330550718714,-232.249824579447));
#204843=CARTESIAN_POINT('Ctrl Pts',(-47.7600215784967,-29.6330588292648,
-232.249824579447));
#204844=CARTESIAN_POINT('Ctrl Pts',(-47.7599867923538,-29.6343725881289,
-232.249899719632));
#204845=CARTESIAN_POINT('Ctrl Pts',(-47.7599520024297,-29.6356863468928,
-232.249974859816));
#204846=CARTESIAN_POINT('Ctrl Pts',(-47.7599172087244,-29.6370001055566,
-232.25005));
#204847=CARTESIAN_POINT('Ctrl Pts',(-47.8203127214913,-27.1915604688604,
-232.25005));
#204848=CARTESIAN_POINT('Ctrl Pts',(-47.7818352998325,-27.5956825746322,
-232.25005));
#204849=CARTESIAN_POINT('Ctrl Pts',(-47.7575670812008,-28.0014343001242,
-232.250050000008));
#204850=CARTESIAN_POINT('Ctrl Pts',(-47.7373322719693,-28.8165134987483,
-232.250050000008));
#204851=CARTESIAN_POINT('Ctrl Pts',(-47.7414965389119,-29.2249682525368,
-232.25005));
#204852=CARTESIAN_POINT('Ctrl Pts',(-47.759738683675,-29.6330167920719,
-232.25005));
#204853=CARTESIAN_POINT('Ctrl Pts',(-47.9849458443842,-16.0452823276962,
-232.25005));
#204854=CARTESIAN_POINT('Ctrl Pts',(-47.9462873275331,-16.4877634160273,
-232.25005));
#204855=CARTESIAN_POINT('Ctrl Pts',(-47.9250450211594,-16.9313786818294,
-232.250050000001));
#204856=CARTESIAN_POINT('Ctrl Pts',(-47.9174315533184,-17.8216219782253,
-232.250050000001));
#204857=CARTESIAN_POINT('Ctrl Pts',(-47.9311272415885,-18.2671771560637,
-232.25005));
#204858=CARTESIAN_POINT('Ctrl Pts',(-47.9621131582323,-18.7116122816628,
-232.25005));
#204859=CARTESIAN_POINT('Ctrl Pts',(-47.9644369065268,-4.51936300780383,
-232.25005));
#204860=CARTESIAN_POINT('Ctrl Pts',(-47.9319477065125,-4.97119967391103,
-232.25005));
#204861=CARTESIAN_POINT('Ctrl Pts',(-47.9174771946989,-5.42425649476983,
-232.25005));
#204862=CARTESIAN_POINT('Ctrl Pts',(-47.9248943561099,-6.33010700446719,
-232.25005));
#204863=CARTESIAN_POINT('Ctrl Pts',(-47.9467635146194,-6.78180681201324,
-232.25005));
#204864=CARTESIAN_POINT('Ctrl Pts',(-47.9866861404267,-7.23226624733626,
-232.25005));
#204865=CARTESIAN_POINT('Origin',(-48.1334350484927,-61.7961505568785,-218.306418983907));
#204866=CARTESIAN_POINT('Origin',(-24.838300653577,28.3971299569735,-229.35005));
#204867=CARTESIAN_POINT('',(-24.960358769668,29.3896529120211,-229.35005));
#204868=CARTESIAN_POINT('',(-24.960358769668,29.3896529120211,-229.35005));
#204869=CARTESIAN_POINT('',(-25.366775135568,29.2460791438418,-229.35005));
#204870=CARTESIAN_POINT('Origin',(-24.838300653577,28.3971299569735,-229.35005));
#204871=CARTESIAN_POINT('',(-25.366775135568,29.2460791438418,-229.35005));
#204872=CARTESIAN_POINT('Origin',(6.29739814579425E-15,-11.5034818258363,
-229.35005));
#204873=CARTESIAN_POINT('',(-39.8203148590359,15.2984308769399,-229.35005));
#204874=CARTESIAN_POINT('Origin',(6.29739814579425E-15,-11.5034818258363,
-229.35005));
#204875=CARTESIAN_POINT('',(-39.8203148590359,15.2984308769399,-229.35005));
#204876=CARTESIAN_POINT('Origin',(-38.9907249661392,14.740057695632,-229.35005));
#204877=CARTESIAN_POINT('',(-39.989972084972,14.7788545447883,-229.35005));
#204878=CARTESIAN_POINT('Origin',(-38.9907249661392,14.740057695632,-229.35005));
#204879=CARTESIAN_POINT('',(-39.989972084972,14.7788545447883,-229.35005));
#204880=CARTESIAN_POINT('Origin',(636.934816028482,-11.5034818258361,-229.35005));
#204881=CARTESIAN_POINT('Origin',(636.934816028482,-11.5034818258361,-229.35005));
#204882=CARTESIAN_POINT('Origin',(-38.9907249661392,-37.7470213473046,-229.35005));
#204883=CARTESIAN_POINT('',(-39.989972084972,-37.7858181964606,-229.35005));
#204884=CARTESIAN_POINT('',(-39.989972084972,-37.7858181964606,-229.35005));
#204885=CARTESIAN_POINT('',(-39.8203148590358,-38.3053945286125,-229.35005));
#204886=CARTESIAN_POINT('Origin',(-38.9907249661392,-37.7470213473046,-229.35005));
#204887=CARTESIAN_POINT('',(-39.8203148590358,-38.3053945286125,-229.35005));
#204888=CARTESIAN_POINT('Origin',(6.29739814579425E-15,-11.5034818258363,
-229.35005));
#204889=CARTESIAN_POINT('Origin',(6.29739814579425E-15,-11.5034818258363,
-229.35005));
#204890=CARTESIAN_POINT('Origin',(-22.9178089794592,-52.5372975341153,-229.35005));
#204891=CARTESIAN_POINT('',(-23.4054219364689,-53.410357442802,-229.35005));
#204892=CARTESIAN_POINT('',(-23.4054219364689,-53.410357442802,-229.35005));
#204893=CARTESIAN_POINT('',(-22.9516892713016,-53.5367234322311,-229.35005));
#204894=CARTESIAN_POINT('Origin',(-22.9178089794592,-52.5372975341153,-229.35005));
#204895=CARTESIAN_POINT('',(-22.9516892713016,-53.5367234322311,-229.35005));
#204896=CARTESIAN_POINT('Origin',(-48.892180948596,36.2913696007177,-218.35005));
#204897=CARTESIAN_POINT('',(-48.892180948596,32.9413696007177,-218.35005));
#204898=CARTESIAN_POINT('Origin',(-48.892180948596,36.2913696007177,-218.35005));
#204899=CARTESIAN_POINT('Origin',(-48.892180948596,36.2913696007177,-218.35005));
#204900=CARTESIAN_POINT('',(-48.892180948596,32.7753941674559,-227.858776203219));
#204901=CARTESIAN_POINT('',(-48.892180948596,32.9413696007177,-218.35005));
#204902=CARTESIAN_POINT('Origin',(-48.892180948596,36.2913696007177,-227.858776203219));
#204903=CARTESIAN_POINT('Origin',(-48.892180948596,36.2913696007177,-227.858776203219));
#204904=CARTESIAN_POINT('Origin',(-48.1334350484927,-61.7961505568785,-218.35005));
#204905=CARTESIAN_POINT('',(-48.1334350484927,-65.1461505568793,-218.35005));
#204906=CARTESIAN_POINT('Origin',(-48.1334350484927,-61.7961505568785,-218.35005));
#204907=CARTESIAN_POINT('Origin',(-48.1334350484927,-61.7961505568785,-218.35005));
#204908=CARTESIAN_POINT('',(-48.1334350484927,-65.1461505568793,-218.35005));
#204909=CARTESIAN_POINT('Origin',(-0.127542579976414,-12.8706479699377,
-228.35005));
#204910=CARTESIAN_POINT('Origin',(-55.2047656166361,-61.9923285455256,-228.35005));
#204911=CARTESIAN_POINT('Origin',(-48.1954151687739,-68.8699303295103,-228.35005));
#204912=CARTESIAN_POINT('Origin',(-0.127542579976414,-12.8706479699377,
-228.35005));
#204913=CARTESIAN_POINT('Origin',(-0.128459562639233,-12.6359082483571,
-228.35005));
#204914=CARTESIAN_POINT('Origin',(-48.892180948596,36.2913696007177,-228.35005));
#204915=CARTESIAN_POINT('Origin',(-48.6323674899383,42.9861279943057,-228.35005));
#204916=CARTESIAN_POINT('Origin',(-55.5877717798047,36.0539745652106,-228.35005));
#204917=CARTESIAN_POINT('Origin',(-0.128459562639233,-12.6359082483571,
-228.35005));
#204918=CARTESIAN_POINT('Origin',(-51.397926952212,-43.6786252257833,-167.906149834141));
#204919=CARTESIAN_POINT('Origin',(-51.7304496786285,-70.1559157828803,-167.906149834141));
#204920=CARTESIAN_POINT('Origin',(0.,-12.9675000200281,-167.906149834141));
#204921=CARTESIAN_POINT('Origin',(-51.3278340104563,17.8606293780317,-167.906149834141));
#204922=CARTESIAN_POINT('Origin',(-51.6000409161409,44.3386087195339,-167.906149834141));
#204923=CARTESIAN_POINT('Origin',(0.,-12.9675000200281,-167.906149834141));
#204924=CARTESIAN_POINT('Ctrl Pts',(-48.9714493645238,-32.4976365372143,
-239.032601429863));
#204925=CARTESIAN_POINT('Ctrl Pts',(-68.1913744168868,-58.588595799019,
-211.730755606268));
#204926=CARTESIAN_POINT('Ctrl Pts',(-47.6504140161628,-30.9809716432943,
-239.032601429841));
#204927=CARTESIAN_POINT('Ctrl Pts',(-66.0438929094031,-54.9590042342752,
-211.730755606272));
#204928=CARTESIAN_POINT('Ctrl Pts',(-46.5919797891444,-28.6187972486599,
-239.032601429843));
#204929=CARTESIAN_POINT('Ctrl Pts',(-64.3781819143446,-49.9473558418611,
-211.730755606271));
#204930=CARTESIAN_POINT('Ctrl Pts',(-46.3023719972087,-25.6595919193811,
-239.032601429843));
#204931=CARTESIAN_POINT('Ctrl Pts',(-63.9692632136205,-43.762285990858,
-211.730755606272));
#204932=CARTESIAN_POINT('Ctrl Pts',(-46.3453291243135,-24.2216224913335,
-239.032601429843));
#204933=CARTESIAN_POINT('Ctrl Pts',(-64.0706036090694,-40.7439486410264,
-211.730755606272));
#204934=CARTESIAN_POINT('Ctrl Pts',(-46.4942182564745,-23.2800468285249,
-239.032601429843));
#204935=CARTESIAN_POINT('Ctrl Pts',(-64.3397924421248,-38.7400276918009,
-211.730755606272));
#204936=CARTESIAN_POINT('Ctrl Pts',(-46.6823308842909,-22.4376754428628,
-239.032601429843));
#204937=CARTESIAN_POINT('Ctrl Pts',(-64.6771567767455,-36.9265599675944,
-211.730755606272));
#204938=CARTESIAN_POINT('Ctrl Pts',(-46.8110566085946,-21.6771313665435,
-239.032601429843));
#204939=CARTESIAN_POINT('Ctrl Pts',(-64.9159602271999,-35.2663729129392,
-211.730755606272));
#204940=CARTESIAN_POINT('Ctrl Pts',(-46.8864232013851,-20.5344885406242,
-239.032601429843));
#204941=CARTESIAN_POINT('Ctrl Pts',(-65.0656320382587,-32.7370789599851,
-211.730755606271));
#204942=CARTESIAN_POINT('Ctrl Pts',(-46.845613352649,-19.389471894004,-239.032601429842));
#204943=CARTESIAN_POINT('Ctrl Pts',(-65.0024851991802,-30.205094760215,
-211.730755606272));
#204944=CARTESIAN_POINT('Ctrl Pts',(-46.739717205202,-18.6241517464968,
-239.032601429843));
#204945=CARTESIAN_POINT('Ctrl Pts',(-64.8208630220631,-28.539554521699,
-211.730755606272));
#204946=CARTESIAN_POINT('Ctrl Pts',(-46.5950583390951,-17.8704826264274,
-239.032601429843));
#204947=CARTESIAN_POINT('Ctrl Pts',(-64.5773028603203,-26.9236650389039,
-211.730755606272));
#204948=CARTESIAN_POINT('Ctrl Pts',(-46.4891834572756,-17.1171663742141,
-239.032601429843));
#204949=CARTESIAN_POINT('Ctrl Pts',(-64.4023778490554,-25.3332388913667,
-211.730755606272));
#204950=CARTESIAN_POINT('Ctrl Pts',(-46.4453565014347,-15.9661997524868,
-239.032601429843));
#204951=CARTESIAN_POINT('Ctrl Pts',(-64.3295185111446,-22.9500603856902,
-211.730755606271));
#204952=CARTESIAN_POINT('Ctrl Pts',(-46.5193900629931,-14.8111705824743,
-239.032601429843));
#204953=CARTESIAN_POINT('Ctrl Pts',(-64.443529180052,-20.5764219053293,
-211.730755606272));
#204954=CARTESIAN_POINT('Ctrl Pts',(-46.6471770799421,-14.0499533302827,
-239.032601429843));
#204955=CARTESIAN_POINT('Ctrl Pts',(-64.6432253119956,-19.0049914961272,
-211.730755606272));
#204956=CARTESIAN_POINT('Ctrl Pts',(-46.7740202606564,-13.4754604930206,
-239.032601429843));
#204957=CARTESIAN_POINT('Ctrl Pts',(-64.8432542225078,-17.8091893041105,
-211.730755606272));
#204958=CARTESIAN_POINT('Ctrl Pts',(-46.8513541209764,-13.0740155121622,
-239.032601429843));
#204959=CARTESIAN_POINT('Ctrl Pts',(-64.9641969010104,-16.980210969671,
-211.730755606271));
#204960=CARTESIAN_POINT('Ctrl Pts',(-46.9348053643729,-12.4640324698742,
-239.032601429843));
#204961=CARTESIAN_POINT('Ctrl Pts',(-65.0935448562552,-15.7339405894364,
-211.730755606272));
#204962=CARTESIAN_POINT('Ctrl Pts',(-46.9850328086675,-11.8494593400854,
-239.032601429843));
#204963=CARTESIAN_POINT('Ctrl Pts',(-65.171164912913,-14.4848476258101,
-211.730755606272));
#204964=CARTESIAN_POINT('Ctrl Pts',(-46.9961709729731,-11.4388750292095,
-239.032601429843));
#204965=CARTESIAN_POINT('Ctrl Pts',(-65.1884659210897,-13.6502250547399,
-211.730755606272));
#204966=CARTESIAN_POINT('Ctrl Pts',(-46.9961709729731,-11.0289590886771,
-239.032601429843));
#204967=CARTESIAN_POINT('Ctrl Pts',(-65.1884659210897,-12.8146289801201,
-211.730755606272));
#204968=CARTESIAN_POINT('Ctrl Pts',(-46.9850328086376,-10.6183760206315,
-239.032601429842));
#204969=CARTESIAN_POINT('Ctrl Pts',(-65.1711648319807,-11.980003483899,
-211.730755606272));
#204970=CARTESIAN_POINT('Ctrl Pts',(-46.9348056898163,-10.0038043022318,
-239.032601429843));
#204971=CARTESIAN_POINT('Ctrl Pts',(-65.093544987819,-10.7309166067835,
-211.730755606272));
#204972=CARTESIAN_POINT('Ctrl Pts',(-46.8513537675148,-9.39381595500219,
-239.032601429843));
#204973=CARTESIAN_POINT('Ctrl Pts',(-64.9641971936048,-9.48464435696854,
-211.730755606272));
#204974=CARTESIAN_POINT('Ctrl Pts',(-46.7740202606564,-8.99237362486574,
-239.032601429843));
#204975=CARTESIAN_POINT('Ctrl Pts',(-64.8432542225078,-8.65566473074882,
-211.730755606272));
#204976=CARTESIAN_POINT('Ctrl Pts',(-46.6471770799421,-8.41788078760364,
-239.032601429843));
#204977=CARTESIAN_POINT('Ctrl Pts',(-64.6432253119957,-7.45986253873205,
-211.730755606272));
#204978=CARTESIAN_POINT('Ctrl Pts',(-46.5193900629931,-7.65666353541205,
-239.032601429843));
#204979=CARTESIAN_POINT('Ctrl Pts',(-64.4435291800518,-5.88843212952995,
-211.730755606271));
#204980=CARTESIAN_POINT('Ctrl Pts',(-46.4453565014347,-6.50163436539958,
-239.032601429843));
#204981=CARTESIAN_POINT('Ctrl Pts',(-64.3295185111447,-3.51479364916907,
-211.730755606272));
#204982=CARTESIAN_POINT('Ctrl Pts',(-46.4891834572756,-5.35066774367227,
-239.032601429843));
#204983=CARTESIAN_POINT('Ctrl Pts',(-64.4023778490553,-1.13161514349255,
-211.730755606272));
#204984=CARTESIAN_POINT('Ctrl Pts',(-46.5950583390951,-4.59735149145896,
-239.032601429843));
#204985=CARTESIAN_POINT('Ctrl Pts',(-64.5773028603203,0.458811004044723,
-211.730755606272));
#204986=CARTESIAN_POINT('Ctrl Pts',(-46.739717205202,-3.84368237138963,
-239.032601429843));
#204987=CARTESIAN_POINT('Ctrl Pts',(-64.8208630220631,2.07470048683978,
-211.730755606272));
#204988=CARTESIAN_POINT('Ctrl Pts',(-46.8456133526491,-3.07836222388228,
-239.032601429843));
#204989=CARTESIAN_POINT('Ctrl Pts',(-65.0024851991801,3.74024072535572,
-211.730755606271));
#204990=CARTESIAN_POINT('Ctrl Pts',(-46.8864232013849,-1.93334557726219,
-239.032601429842));
#204991=CARTESIAN_POINT('Ctrl Pts',(-65.0656320382587,6.27222492512578,
-211.730755606272));
#204992=CARTESIAN_POINT('Ctrl Pts',(-46.8110566085948,-0.790702751342818,
-239.032601429843));
#204993=CARTESIAN_POINT('Ctrl Pts',(-64.9159602271998,8.80151887808002,
-211.730755606272));
#204994=CARTESIAN_POINT('Ctrl Pts',(-46.6823308842909,-0.0301586750235619,
-239.032601429843));
#204995=CARTESIAN_POINT('Ctrl Pts',(-64.6771567767455,10.4617059327352,
-211.730755606272));
#204996=CARTESIAN_POINT('Ctrl Pts',(-46.4942182564745,0.812212710638539,
-239.032601429843));
#204997=CARTESIAN_POINT('Ctrl Pts',(-64.3397924421248,12.2751736569417,
-211.730755606272));
#204998=CARTESIAN_POINT('Ctrl Pts',(-46.3453291243136,1.75378837344716,
-239.032601429843));
#204999=CARTESIAN_POINT('Ctrl Pts',(-64.0706036090695,14.2790946061672,
-211.730755606272));
#205000=CARTESIAN_POINT('Ctrl Pts',(-46.3023719972086,3.1917578014948,-239.032601429843));
#205001=CARTESIAN_POINT('Ctrl Pts',(-63.9692632136205,17.2974319559987,
-211.730755606272));
#205002=CARTESIAN_POINT('Ctrl Pts',(-46.5821989973795,6.05102323992199,
-239.032601429842));
#205003=CARTESIAN_POINT('Ctrl Pts',(-64.3643716897167,23.2736162661097,
-211.730755606271));
#205004=CARTESIAN_POINT('Ctrl Pts',(-47.566430740579,8.32255892669279,-239.032601429843));
#205005=CARTESIAN_POINT('Ctrl Pts',(-65.9117879843948,28.0899407880831,
-211.730755606275));
#205006=CARTESIAN_POINT('Ctrl Pts',(-48.7769866795674,9.7996450480234,-239.032601429843));
#205007=CARTESIAN_POINT('Ctrl Pts',(-67.8755806199084,31.5767606755659,
-211.730755606259));
#205008=CARTESIAN_POINT('Origin',(6.29739814579425E-15,-11.5034818258363,
-234.75005));
#205009=CARTESIAN_POINT('',(-42.9727564520429,17.4202489659096,-234.75005));
#205010=CARTESIAN_POINT('',(-42.9727564520429,17.4202489659097,-234.75005));
#205011=CARTESIAN_POINT('',(-27.3749781671338,32.4720860539414,-234.75005));
#205012=CARTESIAN_POINT('Origin',(6.29739814579425E-15,-11.5034818258363,
-234.75005));
#205013=CARTESIAN_POINT('',(-27.3749781671338,32.4720860539414,-234.75005));
#205014=CARTESIAN_POINT('Origin',(-38.9907249661392,14.740057695632,-234.75005));
#205015=CARTESIAN_POINT('',(-43.7871111365364,14.9262825715819,-234.75005));
#205016=CARTESIAN_POINT('',(-43.7871111365364,14.9262825715819,-234.75005));
#205017=CARTESIAN_POINT('Origin',(-38.9907249661392,14.740057695632,-234.75005));
#205018=CARTESIAN_POINT('Origin',(636.934816028482,-11.5034818258361,-234.75005));
#205019=CARTESIAN_POINT('',(-43.7871111365364,-37.9332462232544,-234.75005));
#205020=CARTESIAN_POINT('',(-43.7871111365364,-37.9332462232544,-234.75005));
#205021=CARTESIAN_POINT('Origin',(636.934816028482,-11.5034818258361,-234.75005));
#205022=CARTESIAN_POINT('Origin',(-38.9907249661392,-37.7470213473046,-234.75005));
#205023=CARTESIAN_POINT('',(-42.9727564520428,-40.4272126175822,-234.75005));
#205024=CARTESIAN_POINT('',(-42.9727564520428,-40.4272126175822,-234.75005));
#205025=CARTESIAN_POINT('Origin',(-38.9907249661392,-37.7470213473046,-234.75005));
#205026=CARTESIAN_POINT('Origin',(6.29739814579425E-15,-11.5034818258363,
-234.75005));
#205027=CARTESIAN_POINT('',(-25.258351173106,-56.7279850958119,-234.75005));
#205028=CARTESIAN_POINT('',(-25.258351173106,-56.7279850958119,-234.75005));
#205029=CARTESIAN_POINT('Origin',(6.29739814579425E-15,-11.5034818258363,
-234.75005));
#205030=CARTESIAN_POINT('Origin',(-22.9178089794592,-52.5372975341153,-234.75005));
#205031=CARTESIAN_POINT('',(-23.0804343803032,-57.3345418450714,-234.75005));
#205032=CARTESIAN_POINT('',(-23.0804343803032,-57.3345418450714,-234.75005));
#205033=CARTESIAN_POINT('Origin',(-22.9178089794592,-52.5372975341153,-234.75005));
#205034=CARTESIAN_POINT('Origin',(-24.838300653577,28.3971299569735,-234.75005));
#205035=CARTESIAN_POINT('',(-25.4241796108136,33.1612401412018,-234.75005));
#205036=CARTESIAN_POINT('Origin',(-24.838300653577,28.3971299569735,-234.75005));
#205037=CARTESIAN_POINT('',(-25.4241796108136,33.1612401412018,-234.75005));
#205038=CARTESIAN_POINT('Origin',(-22.9178089794592,-52.5372975341153,-234.75005));
#205039=CARTESIAN_POINT('',(-25.8434867215177,-57.775656986236,-234.75005));
#205040=CARTESIAN_POINT('',(-25.8434867215177,-57.775656986236,-234.75005));
#205041=CARTESIAN_POINT('',(-23.121090730514,-58.5338529228103,-234.75005));
#205042=CARTESIAN_POINT('Origin',(-22.9178089794592,-52.5372975341153,-234.75005));
#205043=CARTESIAN_POINT('',(-23.121090730514,-58.5338529228103,-234.75005));
#205044=CARTESIAN_POINT('Origin',(-24.838300653577,28.3971299569735,-234.75005));
#205045=CARTESIAN_POINT('',(-25.5706493501227,34.3522676872588,-234.75005));
#205046=CARTESIAN_POINT('',(-25.5706493501227,34.3522676872588,-234.75005));
#205047=CARTESIAN_POINT('',(-28.0091475455229,33.4908250781833,-234.75005));
#205048=CARTESIAN_POINT('Origin',(-24.838300653577,28.3971299569735,-234.75005));
#205049=CARTESIAN_POINT('',(-28.0091475455229,33.4908250781833,-234.75005));
#205050=CARTESIAN_POINT('Origin',(6.29739814579425E-15,-11.5034818258363,
-234.75005));
#205051=CARTESIAN_POINT('',(-43.9682643235187,18.0902967834791,-234.75005));
#205052=CARTESIAN_POINT('Origin',(6.29739814579425E-15,-11.5034818258363,
-234.75005));
#205053=CARTESIAN_POINT('',(-43.9682643235187,18.0902967834791,-234.75005));
#205054=CARTESIAN_POINT('Origin',(-38.9907249661392,14.740057695632,-234.75005));
#205055=CARTESIAN_POINT('',(-44.9862076791357,14.9728387905693,-234.75005));
#205056=CARTESIAN_POINT('Origin',(-38.9907249661392,14.740057695632,-234.75005));
#205057=CARTESIAN_POINT('',(-44.9862076791357,14.9728387905693,-234.75005));
#205058=CARTESIAN_POINT('Origin',(636.934816028482,-11.5034818258361,-234.75005));
#205059=CARTESIAN_POINT('',(-44.9862076791357,-37.9798024422418,-234.75005));
#205060=CARTESIAN_POINT('Origin',(636.934816028482,-11.5034818258361,-234.75005));
#205061=CARTESIAN_POINT('',(-44.9862076791357,-37.9798024422418,-234.75005));
#205062=CARTESIAN_POINT('Origin',(-38.9907249661392,-37.7470213473046,-234.75005));
#205063=CARTESIAN_POINT('',(-43.9682643235187,-41.0972604351516,-234.75005));
#205064=CARTESIAN_POINT('Origin',(-38.9907249661392,-37.7470213473046,-234.75005));
#205065=CARTESIAN_POINT('',(-43.9682643235187,-41.0972604351516,-234.75005));
#205066=CARTESIAN_POINT('Origin',(6.29739814579425E-15,-11.5034818258363,
-234.75005));
#205067=CARTESIAN_POINT('Origin',(6.29739814579425E-15,-11.5034818258363,
-234.75005));
#205068=CARTESIAN_POINT('Ctrl Pts',(-48.1560655127274,-41.999274229607,
-235.35005));
#205069=CARTESIAN_POINT('Ctrl Pts',(-51.9279919200935,-48.6191351285365,
-228.68335));
#205070=CARTESIAN_POINT('Ctrl Pts',(-55.7004001286368,-55.2387363218615,
-222.01665));
#205071=CARTESIAN_POINT('Ctrl Pts',(-59.4732891526772,-61.8580772083615,
-215.34995));
#205072=CARTESIAN_POINT('Ctrl Pts',(-59.5110180429176,-61.9242706172265,
-215.283283));
#205073=CARTESIAN_POINT('Ctrl Pts',(-59.548746933158,-61.9904640260915,
-215.216616));
#205074=CARTESIAN_POINT('Ctrl Pts',(-59.5864758233984,-62.0566574349565,
-215.149949));
#205075=CARTESIAN_POINT('Ctrl Pts',(-48.2756382252007,-41.8104563330539,
-235.35005));
#205076=CARTESIAN_POINT('Ctrl Pts',(-52.0407670149459,-48.4530353242655,
-228.68335));
#205077=CARTESIAN_POINT('Ctrl Pts',(-55.8063647406712,-55.0953754160451,
-222.01665));
#205078=CARTESIAN_POINT('Ctrl Pts',(-59.57243049321,-61.7374760219621,-215.34995));
#205079=CARTESIAN_POINT('Ctrl Pts',(-59.6100911507354,-61.8038970280213,
-215.283283));
#205080=CARTESIAN_POINT('Ctrl Pts',(-59.6477518082608,-61.8703180340805,
-215.216616));
#205081=CARTESIAN_POINT('Ctrl Pts',(-59.6854124657861,-61.9367390401396,
-215.149949));
#205082=CARTESIAN_POINT('Ctrl Pts',(-48.3910626922776,-41.5900298422911,
-235.35005));
#205083=CARTESIAN_POINT('Ctrl Pts',(-52.1903238662186,-48.2138133273298,
-228.68335));
#205084=CARTESIAN_POINT('Ctrl Pts',(-55.9900266043744,-54.8373975226491,
-222.01665));
#205085=CARTESIAN_POINT('Ctrl Pts',(-59.790170143516,-61.4607818737039,
-215.34995));
#205086=CARTESIAN_POINT('Ctrl Pts',(-59.8281715789074,-61.5270157172145,
-215.283283));
#205087=CARTESIAN_POINT('Ctrl Pts',(-59.8661730142988,-61.593249560725,
-215.216616));
#205088=CARTESIAN_POINT('Ctrl Pts',(-59.9041744496902,-61.6594834042356,
-215.149949));
#205089=CARTESIAN_POINT('Ctrl Pts',(-48.5387172079886,-41.2798109487642,
-235.35005));
#205090=CARTESIAN_POINT('Ctrl Pts',(-52.4230972161915,-47.8204177760876,
-228.68335));
#205091=CARTESIAN_POINT('Ctrl Pts',(-56.3078726256209,-54.3608781649969,
-222.01665));
#205092=CARTESIAN_POINT('Ctrl Pts',(-60.1930428686919,-60.9011916159786,
-215.34995));
#205093=CARTESIAN_POINT('Ctrl Pts',(-60.2318945711226,-60.9665947504884,
-215.283283000001));
#205094=CARTESIAN_POINT('Ctrl Pts',(-60.2707462735533,-61.0319978849983,
-215.216616));
#205095=CARTESIAN_POINT('Ctrl Pts',(-60.309597975984,-61.0974010195081,
-215.149949));
#205096=CARTESIAN_POINT('Ctrl Pts',(-48.6371642419829,-41.0193984169334,
-235.35005));
#205097=CARTESIAN_POINT('Ctrl Pts',(-52.6688606290506,-47.3486283864447,
-228.68335));
#205098=CARTESIAN_POINT('Ctrl Pts',(-56.7009009677878,-53.6777576502171,
-222.01665));
#205099=CARTESIAN_POINT('Ctrl Pts',(-60.7332848610003,-60.0067857712577,
-215.34995));
#205100=CARTESIAN_POINT('Ctrl Pts',(-60.7736086999325,-60.0700760524681,
-215.283283));
#205101=CARTESIAN_POINT('Ctrl Pts',(-60.8139325388646,-60.1333663336785,
-215.216616));
#205102=CARTESIAN_POINT('Ctrl Pts',(-60.8542563777967,-60.1966566148889,
-215.149949));
#205103=CARTESIAN_POINT('Ctrl Pts',(-48.7259447515556,-40.7557132274099,
-235.35005));
#205104=CARTESIAN_POINT('Ctrl Pts',(-52.8863489207853,-46.8366038296761,
-228.68335));
#205105=CARTESIAN_POINT('Ctrl Pts',(-57.0470401243311,-52.9174317848832,
-222.016650000001));
#205106=CARTESIAN_POINT('Ctrl Pts',(-61.2080181081436,-58.9981967263321,
-215.349950000001));
#205107=CARTESIAN_POINT('Ctrl Pts',(-61.2496278879817,-59.0590043757466,
-215.283283000001));
#205108=CARTESIAN_POINT('Ctrl Pts',(-61.2912376678198,-59.1198120251611,
-215.216616));
#205109=CARTESIAN_POINT('Ctrl Pts',(-61.332847447658,-59.1806196745756,
-215.149949000001));
#205110=CARTESIAN_POINT('Ctrl Pts',(-48.7945150938174,-40.4960542325497,
-235.35005));
#205111=CARTESIAN_POINT('Ctrl Pts',(-53.0535779259056,-46.3256171279293,
-228.68335));
#205112=CARTESIAN_POINT('Ctrl Pts',(-57.3128652259323,-52.1551472055685,
-222.01665));
#205113=CARTESIAN_POINT('Ctrl Pts',(-61.572376853754,-57.9846441771198,
-215.34995));
#205114=CARTESIAN_POINT('Ctrl Pts',(-61.6149719700322,-58.0429391468354,
-215.283283));
#205115=CARTESIAN_POINT('Ctrl Pts',(-61.6575670863105,-58.1012341165509,
-215.216616));
#205116=CARTESIAN_POINT('Ctrl Pts',(-61.7001622025887,-58.1595290862664,
-215.149949));
#205117=CARTESIAN_POINT('Ctrl Pts',(-48.8537891615446,-40.2227290210882,
-235.35005));
#205118=CARTESIAN_POINT('Ctrl Pts',(-53.184407479365,-45.7839380160283,
-228.68335));
#205119=CARTESIAN_POINT('Ctrl Pts',(-57.5151818684938,-51.3451352378197,
-222.01665));
#205120=CARTESIAN_POINT('Ctrl Pts',(-61.8461122714633,-56.9063204848096,
-215.349950000001));
#205121=CARTESIAN_POINT('Ctrl Pts',(-61.889421575493,-56.9619323372794,
-215.283283000001));
#205122=CARTESIAN_POINT('Ctrl Pts',(-61.9327308795227,-57.0175441897493,
-215.216616));
#205123=CARTESIAN_POINT('Ctrl Pts',(-61.9760401835524,-57.0731560422192,
-215.149949000001));
#205124=CARTESIAN_POINT('Ctrl Pts',(-48.8993219763807,-39.9191637201113,
-235.35005));
#205125=CARTESIAN_POINT('Ctrl Pts',(-53.2653672535676,-45.2450247261708,
-228.68335));
#205126=CARTESIAN_POINT('Ctrl Pts',(-57.631494193953,-50.5708856635808,
-222.01665));
#205127=CARTESIAN_POINT('Ctrl Pts',(-61.9977027895214,-55.8967464260103,
-215.34995));
#205128=CARTESIAN_POINT('Ctrl Pts',(-62.0413648754771,-55.9500050336346,
-215.283283));
#205129=CARTESIAN_POINT('Ctrl Pts',(-62.0850269614327,-56.0032636412589,
-215.216616));
#205130=CARTESIAN_POINT('Ctrl Pts',(-62.1286890473884,-56.0565222488832,
-215.149949));
#205131=CARTESIAN_POINT('Ctrl Pts',(-48.9214109907111,-39.6817730556917,
-235.35005));
#205132=CARTESIAN_POINT('Ctrl Pts',(-53.2924626390134,-44.9053881830262,
-228.68335));
#205133=CARTESIAN_POINT('Ctrl Pts',(-57.6635282520289,-50.1290038777392,
-222.01665));
#205134=CARTESIAN_POINT('Ctrl Pts',(-62.0346078304961,-55.3526201213579,
-215.34995));
#205135=CARTESIAN_POINT('Ctrl Pts',(-62.0783186262807,-55.4048562837941,
-215.283283));
#205136=CARTESIAN_POINT('Ctrl Pts',(-62.1220294220654,-55.4570924462303,
-215.216616));
#205137=CARTESIAN_POINT('Ctrl Pts',(-62.1657402178501,-55.5093286086665,
-215.149949));
#205138=CARTESIAN_POINT('Ctrl Pts',(-48.9276804568491,-39.5283381317121,
-235.35005));
#205139=CARTESIAN_POINT('Ctrl Pts',(-53.2999213760692,-44.7204933330714,
-228.68335));
#205140=CARTESIAN_POINT('Ctrl Pts',(-57.6721622952894,-49.9126485344307,
-222.01665));
#205141=CARTESIAN_POINT('Ctrl Pts',(-62.0444032145095,-55.1048037357899,
-215.34995));
#205142=CARTESIAN_POINT('Ctrl Pts',(-62.0881256237017,-55.1567252878035,
-215.283283));
#205143=CARTESIAN_POINT('Ctrl Pts',(-62.1318480328939,-55.2086468398171,
-215.216616));
#205144=CARTESIAN_POINT('Ctrl Pts',(-62.1755704420861,-55.2605683918307,
-215.149949));
#205145=CARTESIAN_POINT('Ctrl Pts',(-48.4015825627194,-42.4301635567086,
-234.916111528175));
#205146=CARTESIAN_POINT('Ctrl Pts',(-51.8161020106309,-48.4227195017014,
-228.881144730288));
#205147=CARTESIAN_POINT('Ctrl Pts',(-55.2310162579792,-54.4150626175587,
-222.846177932402));
#205148=CARTESIAN_POINT('Ctrl Pts',(-58.6463245735781,-60.4071924582901,
-216.811211134516));
#205149=CARTESIAN_POINT('',(-55.4860418356793,-47.316570933751,-225.35));
#205150=CARTESIAN_POINT('Ctrl Pts',(-24.4127870505286,-62.4913878448826,
-235.35005));
#205151=CARTESIAN_POINT('Ctrl Pts',(-30.252655437952,-66.705065059021,-228.68335));
#205152=CARTESIAN_POINT('Ctrl Pts',(-36.0925246020991,-70.9187639624533,
-222.01665));
#205153=CARTESIAN_POINT('Ctrl Pts',(-41.9323946221365,-75.1324845521997,
-215.34995));
#205154=CARTESIAN_POINT('Ctrl Pts',(-41.990793322337,-75.1746217580972,
-215.283283));
#205155=CARTESIAN_POINT('Ctrl Pts',(-42.0491920225373,-75.2167589639946,
-215.216616));
#205156=CARTESIAN_POINT('Ctrl Pts',(-42.1075907227377,-75.2588961698921,
-215.149949));
#205157=CARTESIAN_POINT('Ctrl Pts',(-24.4238355020022,-62.4909941277675,
-235.35005));
#205158=CARTESIAN_POINT('Ctrl Pts',(-30.2665958673131,-66.7045508406744,
-228.68335));
#205159=CARTESIAN_POINT('Ctrl Pts',(-36.1093567495128,-70.9181220131437,
-222.01665));
#205160=CARTESIAN_POINT('Ctrl Pts',(-41.9521182016317,-75.1317076431822,
-215.34995));
#205161=CARTESIAN_POINT('Ctrl Pts',(-42.0105458161529,-75.1738434994826,
-215.283283));
#205162=CARTESIAN_POINT('Ctrl Pts',(-42.0689734306741,-75.215979355783,
-215.216616));
#205163=CARTESIAN_POINT('Ctrl Pts',(-42.1274010451954,-75.2581152120834,
-215.149949));
#205164=CARTESIAN_POINT('Ctrl Pts',(-24.4348839534758,-62.4906004106524,
-235.35005));
#205165=CARTESIAN_POINT('Ctrl Pts',(-30.2805362966741,-66.7040366223279,
-228.68335));
#205166=CARTESIAN_POINT('Ctrl Pts',(-36.1261888969267,-70.9174800638341,
-222.01665));
#205167=CARTESIAN_POINT('Ctrl Pts',(-41.971841781127,-75.1309307341648,
-215.34995));
#205168=CARTESIAN_POINT('Ctrl Pts',(-42.030298309969,-75.1730652408681,
-215.283283));
#205169=CARTESIAN_POINT('Ctrl Pts',(-42.088754838811,-75.2151997475714,
-215.216616));
#205170=CARTESIAN_POINT('Ctrl Pts',(-42.147211367653,-75.2573342542747,
-215.149949));
#205171=CARTESIAN_POINT('Ctrl Pts',(-24.4459324049493,-62.4902066935372,
-235.35005));
#205172=CARTESIAN_POINT('Ctrl Pts',(-30.2944767260352,-66.7035224039813,
-228.68335));
#205173=CARTESIAN_POINT('Ctrl Pts',(-36.1430210443405,-70.9168381145244,
-222.01665));
#205174=CARTESIAN_POINT('Ctrl Pts',(-41.9915653606222,-75.1301538251473,
-215.34995));
#205175=CARTESIAN_POINT('Ctrl Pts',(-42.050050803785,-75.1722869822535,
-215.283283));
#205176=CARTESIAN_POINT('Ctrl Pts',(-42.1085362469478,-75.2144201393598,
-215.216616));
#205177=CARTESIAN_POINT('Ctrl Pts',(-42.1670216901106,-75.256553296466,
-215.149949));
#205178=CARTESIAN_POINT('Ctrl Pts',(-24.5840380483692,-62.4852852295981,
-235.35005));
#205179=CARTESIAN_POINT('Ctrl Pts',(-30.4687320930486,-66.6970946746494,
-228.68335));
#205180=CARTESIAN_POINT('Ctrl Pts',(-36.3534228870133,-70.9088137481542,
-222.01665));
#205181=CARTESIAN_POINT('Ctrl Pts',(-42.2381101043121,-75.120442462429,
-215.34995));
#205182=CARTESIAN_POINT('Ctrl Pts',(-42.2969569764852,-75.1625587495718,
-215.283283));
#205183=CARTESIAN_POINT('Ctrl Pts',(-42.3558038486582,-75.2046750367146,
-215.216616));
#205184=CARTESIAN_POINT('Ctrl Pts',(-42.4146507208312,-75.2467913238573,
-215.149949));
#205185=CARTESIAN_POINT('Ctrl Pts',(-24.7878826649652,-62.4682791689329,
-235.35005));
#205186=CARTESIAN_POINT('Ctrl Pts',(-30.7858798041607,-66.6737307701245,
-228.68335));
#205187=CARTESIAN_POINT('Ctrl Pts',(-36.7838683264116,-70.8789174633912,
-222.01665));
#205188=CARTESIAN_POINT('Ctrl Pts',(-42.781847274702,-75.0838392837,-215.34995));
#205189=CARTESIAN_POINT('Ctrl Pts',(-42.8418270641849,-75.1258885019031,
-215.283283));
#205190=CARTESIAN_POINT('Ctrl Pts',(-42.9018068536678,-75.1679377201062,
-215.216616));
#205191=CARTESIAN_POINT('Ctrl Pts',(-42.9617866431507,-75.2099869383093,
-215.149949));
#205192=CARTESIAN_POINT('Ctrl Pts',(-25.048207175495,-62.4347017437458,
-235.35005));
#205193=CARTESIAN_POINT('Ctrl Pts',(-31.2985071141138,-66.6007006042259,
-228.68335));
#205194=CARTESIAN_POINT('Ctrl Pts',(-37.5487936188611,-70.7661908933779,
-222.01665));
#205195=CARTESIAN_POINT('Ctrl Pts',(-43.7990648514606,-74.9311726743249,
-215.34995));
#205196=CARTESIAN_POINT('Ctrl Pts',(-43.8615675637866,-74.9728224921344,
-215.283283));
#205197=CARTESIAN_POINT('Ctrl Pts',(-43.9240702761126,-75.0144723099439,
-215.216616));
#205198=CARTESIAN_POINT('Ctrl Pts',(-43.9865729884385,-75.0561221277533,
-215.149949));
#205199=CARTESIAN_POINT('Ctrl Pts',(-25.2812199560259,-62.390732268219,
-235.35005));
#205200=CARTESIAN_POINT('Ctrl Pts',(-31.8143029221326,-66.4798048243852,
-228.68335));
#205201=CARTESIAN_POINT('Ctrl Pts',(-38.3473707133638,-70.5681428074098,
-222.01665));
#205202=CARTESIAN_POINT('Ctrl Pts',(-44.8804206737979,-74.6557463029982,
-215.34995));
#205203=CARTESIAN_POINT('Ctrl Pts',(-44.9457511734022,-74.6966223379541,
-215.283283));
#205204=CARTESIAN_POINT('Ctrl Pts',(-45.0110816730065,-74.73749837291,-215.216616));
#205205=CARTESIAN_POINT('Ctrl Pts',(-45.0764121726109,-74.7783744078659,
-215.149949));
#205206=CARTESIAN_POINT('Ctrl Pts',(-25.5015868365187,-62.3415392578964,
-235.35005));
#205207=CARTESIAN_POINT('Ctrl Pts',(-32.299209143815,-66.325492796133,-228.68335));
#205208=CARTESIAN_POINT('Ctrl Pts',(-39.0968174546589,-70.3085029414293,
-222.01665));
#205209=CARTESIAN_POINT('Ctrl Pts',(-45.8944083573785,-74.2905697967455,
-215.34995));
#205210=CARTESIAN_POINT('Ctrl Pts',(-45.9623842664057,-74.3303904652987,
-215.283283));
#205211=CARTESIAN_POINT('Ctrl Pts',(-46.0303601754329,-74.3702111338518,
-215.216616));
#205212=CARTESIAN_POINT('Ctrl Pts',(-46.0983360844601,-74.410031802405,
-215.149949));
#205213=CARTESIAN_POINT('Ctrl Pts',(-25.7300777644121,-62.275287851211,
-235.35005));
#205214=CARTESIAN_POINT('Ctrl Pts',(-32.7889564583827,-66.1223030781061,
-228.68335));
#205215=CARTESIAN_POINT('Ctrl Pts',(-39.8478250972557,-69.9681827947029,
-222.01665));
#205216=CARTESIAN_POINT('Ctrl Pts',(-46.906679573783,-73.8129271161338,
-215.34995));
#205217=CARTESIAN_POINT('Ctrl Pts',(-46.9772681185483,-73.8513745593482,
-215.283283));
#205218=CARTESIAN_POINT('Ctrl Pts',(-47.0478566633135,-73.8898220025625,
-215.216616));
#205219=CARTESIAN_POINT('Ctrl Pts',(-47.1184452080788,-73.9282694457768,
-215.149949));
#205220=CARTESIAN_POINT('Ctrl Pts',(-25.9496411726737,-62.2064433802863,
-235.35005));
#205221=CARTESIAN_POINT('Ctrl Pts',(-33.2328325215974,-65.8962682476017,
-228.68335));
#205222=CARTESIAN_POINT('Ctrl Pts',(-40.5160203632138,-69.5847817101261,
-222.01665));
#205223=CARTESIAN_POINT('Ctrl Pts',(-47.7991999531534,-73.2719838903286,
-215.34995));
#205224=CARTESIAN_POINT('Ctrl Pts',(-47.8720317490528,-73.3088559121307,
-215.283283));
#205225=CARTESIAN_POINT('Ctrl Pts',(-47.9448635449522,-73.3457279339327,
-215.216616));
#205226=CARTESIAN_POINT('Ctrl Pts',(-48.0176953408516,-73.3825999557347,
-215.149949));
#205227=CARTESIAN_POINT('Ctrl Pts',(-26.2296171960789,-62.0929811520229,
-235.35005));
#205228=CARTESIAN_POINT('Ctrl Pts',(-33.5992240749579,-65.6911775370676,
-228.68335));
#205229=CARTESIAN_POINT('Ctrl Pts',(-40.9688364442604,-69.2879023661194,
-222.01665));
#205230=CARTESIAN_POINT('Ctrl Pts',(-48.3384489792287,-72.8831557643943,
-215.34995));
#205231=CARTESIAN_POINT('Ctrl Pts',(-48.4121451045784,-72.919108298377,
-215.283283));
#205232=CARTESIAN_POINT('Ctrl Pts',(-48.485841229928,-72.9550608323598,
-215.216616));
#205233=CARTESIAN_POINT('Ctrl Pts',(-48.5595373552777,-72.9910133663425,
-215.149949));
#205234=CARTESIAN_POINT('Ctrl Pts',(-26.4137508499222,-62.0144582859218,
-235.35005));
#205235=CARTESIAN_POINT('Ctrl Pts',(-33.8110251833904,-65.5692400768433,
-228.68335));
#205236=CARTESIAN_POINT('Ctrl Pts',(-41.2083125347321,-69.1224537201152,
-222.01665));
#205237=CARTESIAN_POINT('Ctrl Pts',(-48.6056072289401,-72.6740993398878,
-215.34995));
#205238=CARTESIAN_POINT('Ctrl Pts',(-48.6795801758822,-72.7096157960855,
-215.283283));
#205239=CARTESIAN_POINT('Ctrl Pts',(-48.7535531228243,-72.7451322522832,
-215.216616));
#205240=CARTESIAN_POINT('Ctrl Pts',(-48.8275260697664,-72.780648708481,
-215.149949));
#205241=CARTESIAN_POINT('Ctrl Pts',(-26.60131676328,-61.915483833886,-235.35005));
#205242=CARTESIAN_POINT('Ctrl Pts',(-33.9746898504281,-65.4717344596898,
-228.68335));
#205243=CARTESIAN_POINT('Ctrl Pts',(-41.3480800753329,-69.0263711060389,
-222.01665));
#205244=CARTESIAN_POINT('Ctrl Pts',(-48.7214815967444,-72.5793938958684,
-215.34995));
#205245=CARTESIAN_POINT('Ctrl Pts',(-48.7952156119585,-72.6149241237667,
-215.283283));
#205246=CARTESIAN_POINT('Ctrl Pts',(-48.8689496271726,-72.6504543516649,
-215.216616));
#205247=CARTESIAN_POINT('Ctrl Pts',(-48.9426836423867,-72.6859845795632,
-215.149949));
#205248=CARTESIAN_POINT('',(-33.2187488845874,-68.8101802592752,-225.35));
#205249=CARTESIAN_POINT('Ctrl Pts',(-27.0930165135311,-62.1526330725429,
-234.905475377596));
#205250=CARTESIAN_POINT('Ctrl Pts',(-33.75885046978,-65.3675653924474,-228.878503713969));
#205251=CARTESIAN_POINT('Ctrl Pts',(-40.424698326436,-68.5811786244384,
-222.851532050343));
#205252=CARTESIAN_POINT('Ctrl Pts',(-47.0905557676078,-71.7934728593479,
-216.824560386716));
#205253=CARTESIAN_POINT('Ctrl Pts',(-29.0709882823152,37.525873057636,-235.35005));
#205254=CARTESIAN_POINT('Ctrl Pts',(-35.5332604733831,40.6579014073498,
-228.683350000001));
#205255=CARTESIAN_POINT('Ctrl Pts',(-41.9930962102693,43.771133049519,-222.01665));
#205256=CARTESIAN_POINT('Ctrl Pts',(-48.4493862544499,46.8657485296993,
-215.34995));
#205257=CARTESIAN_POINT('Ctrl Pts',(-48.5139491548917,46.8966946845011,
-215.283283));
#205258=CARTESIAN_POINT('Ctrl Pts',(-48.5785120553335,46.9276408393029,
-215.216616));
#205259=CARTESIAN_POINT('Ctrl Pts',(-48.6430749557753,46.9585869941047,
-215.149949));
#205260=CARTESIAN_POINT('Ctrl Pts',(-28.9262831839988,37.6116730896339,
-235.35005));
#205261=CARTESIAN_POINT('Ctrl Pts',(-35.404815368487,40.7403542996618,-228.683350000001));
#205262=CARTESIAN_POINT('Ctrl Pts',(-41.8809828830328,43.8508119821702,
-222.01665));
#205263=CARTESIAN_POINT('Ctrl Pts',(-48.3537103198215,46.9432211795102,
-215.34995));
#205264=CARTESIAN_POINT('Ctrl Pts',(-48.4184375941894,46.9741452714836,
-215.283283));
#205265=CARTESIAN_POINT('Ctrl Pts',(-48.4831648685572,47.005069363457,-215.216616));
#205266=CARTESIAN_POINT('Ctrl Pts',(-48.5478921429251,47.0359934554304,
-215.149949));
#205267=CARTESIAN_POINT('Ctrl Pts',(-28.7510590357854,37.7017381212741,
-235.35005));
#205268=CARTESIAN_POINT('Ctrl Pts',(-35.2153249135404,40.8559840579253,
-228.683350000001));
#205269=CARTESIAN_POINT('Ctrl Pts',(-41.67737658309,43.9932018113665,-222.01665));
#205270=CARTESIAN_POINT('Ctrl Pts',(-48.1362091874323,47.1135549465408,
-215.34995));
#205271=CARTESIAN_POINT('Ctrl Pts',(-48.2007975134757,47.1447584778926,
-215.283283));
#205272=CARTESIAN_POINT('Ctrl Pts',(-48.2653858395191,47.1759620092443,
-215.216616));
#205273=CARTESIAN_POINT('Ctrl Pts',(-48.3299741655626,47.207165540596,-215.149949));
#205274=CARTESIAN_POINT('Ctrl Pts',(-28.5095079111441,37.8154098604791,
-235.350050000001));
#205275=CARTESIAN_POINT('Ctrl Pts',(-34.9092271504532,41.0352703241457,
-228.683350000001));
#205276=CARTESIAN_POINT('Ctrl Pts',(-41.3069791618872,44.2400465335893,
-222.016650000001));
#205277=CARTESIAN_POINT('Ctrl Pts',(-47.7018738162952,47.429883386524,-215.34995));
#205278=CARTESIAN_POINT('Ctrl Pts',(-47.7658227628392,47.4617817550534,
-215.283283));
#205279=CARTESIAN_POINT('Ctrl Pts',(-47.8297717093833,47.4936801235827,
-215.216616));
#205280=CARTESIAN_POINT('Ctrl Pts',(-47.8937206559274,47.525578492112,-215.149949));
#205281=CARTESIAN_POINT('Ctrl Pts',(-28.3066649003232,37.8966208237621,
-235.35005));
#205282=CARTESIAN_POINT('Ctrl Pts',(-34.5530956045189,41.2282169831045,
-228.68335));
#205283=CARTESIAN_POINT('Ctrl Pts',(-40.7978279568429,44.5468276894782,
-222.01665));
#205284=CARTESIAN_POINT('Ctrl Pts',(-47.0400956910773,47.8525776841313,
-215.34995));
#205285=CARTESIAN_POINT('Ctrl Pts',(-47.1025183684196,47.8856351840778,
-215.283283));
#205286=CARTESIAN_POINT('Ctrl Pts',(-47.1649410457619,47.9186926840244,
-215.216616));
#205287=CARTESIAN_POINT('Ctrl Pts',(-47.2273637231043,47.9517501839709,
-215.149949));
#205288=CARTESIAN_POINT('Ctrl Pts',(-28.0997724400839,37.970731452037,-235.35005));
#205289=CARTESIAN_POINT('Ctrl Pts',(-34.1684829306694,41.4070992755122,
-228.683350000001));
#205290=CARTESIAN_POINT('Ctrl Pts',(-40.2357864490083,44.8327392792855,
-222.01665));
#205291=CARTESIAN_POINT('Ctrl Pts',(-46.3010499603476,48.2477545207809,
-215.34995));
#205292=CARTESIAN_POINT('Ctrl Pts',(-46.361702595461,48.2819046731959,-215.283283));
#205293=CARTESIAN_POINT('Ctrl Pts',(-46.4223552305744,48.3160548256108,
-215.216616));
#205294=CARTESIAN_POINT('Ctrl Pts',(-46.4830078656878,48.3502049780258,
-215.149949));
#205295=CARTESIAN_POINT('Ctrl Pts',(-27.9025329741163,38.0324522529201,
-235.35005));
#205296=CARTESIAN_POINT('Ctrl Pts',(-33.7896008939784,41.5559827385479,
-228.683350000001));
#205297=CARTESIAN_POINT('Ctrl Pts',(-39.6755763327887,45.0712058294971,
-222.01665));
#205298=CARTESIAN_POINT('Ctrl Pts',(-45.5599690892415,48.5782013338904,
-215.349950000001));
#205299=CARTESIAN_POINT('Ctrl Pts',(-45.618813016806,48.6132712889344,-215.283283000001));
#205300=CARTESIAN_POINT('Ctrl Pts',(-45.6776569443706,48.6483412439783,
-215.216616));
#205301=CARTESIAN_POINT('Ctrl Pts',(-45.7365008719351,48.6834111990222,
-215.149949000001));
#205302=CARTESIAN_POINT('Ctrl Pts',(-27.6836295517497,38.0888474954169,
-235.35005));
#205303=CARTESIAN_POINT('Ctrl Pts',(-33.3812146101381,41.6857034969331,
-228.68335));
#205304=CARTESIAN_POINT('Ctrl Pts',(-39.0780453981879,45.2768392802963,
-222.01665));
#205305=CARTESIAN_POINT('Ctrl Pts',(-44.773784383473,48.8623098007285,-215.34995));
#205306=CARTESIAN_POINT('Ctrl Pts',(-44.8307417733259,48.8981645059328,
-215.283283));
#205307=CARTESIAN_POINT('Ctrl Pts',(-44.8876991631787,48.9340192111371,
-215.216616));
#205308=CARTESIAN_POINT('Ctrl Pts',(-44.9446565530316,48.9698739163414,
-215.149949));
#205309=CARTESIAN_POINT('Ctrl Pts',(-27.4619512217085,38.1391172889764,
-235.35005));
#205310=CARTESIAN_POINT('Ctrl Pts',(-32.9867338744792,41.7852023290646,
-228.683350000001));
#205311=CARTESIAN_POINT('Ctrl Pts',(-38.511124795091,45.4283250387717,-222.016650000001));
#205312=CARTESIAN_POINT('Ctrl Pts',(-44.0349491888799,49.0685138787004,
-215.349950000001));
#205313=CARTESIAN_POINT('Ctrl Pts',(-44.0901874328179,49.1049157670997,
-215.283283000001));
#205314=CARTESIAN_POINT('Ctrl Pts',(-44.1454256767557,49.141317655499,-215.216616));
#205315=CARTESIAN_POINT('Ctrl Pts',(-44.2006639206936,49.1777195438983,
-215.149949000001));
#205316=CARTESIAN_POINT('Ctrl Pts',(-27.272251770635,38.1696450547512,-235.35005));
#205317=CARTESIAN_POINT('Ctrl Pts',(-32.7234828694691,41.832799228952,-228.68335));
#205318=CARTESIAN_POINT('Ctrl Pts',(-38.1745805518739,45.4949461119472,
-222.01665));
#205319=CARTESIAN_POINT('Ctrl Pts',(-43.625485383249,49.1560953813671,-215.34995));
#205320=CARTESIAN_POINT('Ctrl Pts',(-43.6799944315629,49.1927068740612,
-215.283283));
#205321=CARTESIAN_POINT('Ctrl Pts',(-43.7345034798766,49.2293183667554,
-215.216616));
#205322=CARTESIAN_POINT('Ctrl Pts',(-43.7890125281904,49.2659298594496,
-215.149949));
#205323=CARTESIAN_POINT('Ctrl Pts',(-27.1569075795172,38.1844371310006,
-235.35005));
#205324=CARTESIAN_POINT('Ctrl Pts',(-32.5837764342019,41.8536056393876,
-228.68335));
#205325=CARTESIAN_POINT('Ctrl Pts',(-38.0106452875494,45.5227741479461,
-222.01665));
#205326=CARTESIAN_POINT('Ctrl Pts',(-43.4375141409548,49.1919426564936,
-215.34995));
#205327=CARTESIAN_POINT('Ctrl Pts',(-43.4917828294889,49.2286343415791,
-215.283283));
#205328=CARTESIAN_POINT('Ctrl Pts',(-43.5460515180229,49.2653260266646,
-215.216616));
#205329=CARTESIAN_POINT('Ctrl Pts',(-43.600320206557,49.30201771175,-215.149949));
#205330=CARTESIAN_POINT('Ctrl Pts',(-29.5524353619882,37.7591803693089,
-234.853368133768));
#205331=CARTESIAN_POINT('Ctrl Pts',(-35.3897707041939,40.5875346064766,
-228.831260854445));
#205332=CARTESIAN_POINT('Ctrl Pts',(-41.225095491082,43.4005549188572,-222.809153575121));
#205333=CARTESIAN_POINT('Ctrl Pts',(-47.0575921287078,46.1983743823903,
-216.787046295788));
#205334=CARTESIAN_POINT('',(-35.2972108607157,43.6881898936869,-225.35));
#205335=CARTESIAN_POINT('Ctrl Pts',(-48.9291851287222,16.4845500982845,
-235.35005));
#205336=CARTESIAN_POINT('Ctrl Pts',(-53.3017114728827,20.6931427899333,
-228.68335));
#205337=CARTESIAN_POINT('Ctrl Pts',(-57.6742344655836,24.9017353436595,
-222.01665));
#205338=CARTESIAN_POINT('Ctrl Pts',(-62.0467541066728,29.1103277631972,
-215.34995));
#205339=CARTESIAN_POINT('Ctrl Pts',(-62.0904793030837,29.1524136873926,
-215.283283));
#205340=CARTESIAN_POINT('Ctrl Pts',(-62.1342044994946,29.194499611588,-215.216616));
#205341=CARTESIAN_POINT('Ctrl Pts',(-62.1779296959055,29.2365855357833,
-215.149949));
#205342=CARTESIAN_POINT('Ctrl Pts',(-48.9286835714312,16.4968248922029,
-235.35005));
#205343=CARTESIAN_POINT('Ctrl Pts',(-53.3011147739234,20.7079343778016,
-228.68335));
#205344=CARTESIAN_POINT('Ctrl Pts',(-57.6735437421284,24.9190437709811,
-222.01665));
#205345=CARTESIAN_POINT('Ctrl Pts',(-62.0459704759518,29.1301530740427,
-215.34995));
#205346=CARTESIAN_POINT('Ctrl Pts',(-62.08969474329,29.1722641670733,-215.283283));
#205347=CARTESIAN_POINT('Ctrl Pts',(-62.1334190106282,29.2143752601038,
-215.216616));
#205348=CARTESIAN_POINT('Ctrl Pts',(-62.1771432779665,29.2564863531345,
-215.149949));
#205349=CARTESIAN_POINT('Ctrl Pts',(-48.9281820141402,16.5090996861212,
-235.35005));
#205350=CARTESIAN_POINT('Ctrl Pts',(-53.3005180749641,20.72272596567,-228.68335));
#205351=CARTESIAN_POINT('Ctrl Pts',(-57.6728530186733,24.9363521983027,
-222.01665));
#205352=CARTESIAN_POINT('Ctrl Pts',(-62.0451868452307,29.1499783848881,
-215.34995));
#205353=CARTESIAN_POINT('Ctrl Pts',(-62.0889101834963,29.1921146467539,
-215.283283));
#205354=CARTESIAN_POINT('Ctrl Pts',(-62.1326335217618,29.2342509086198,
-215.216616));
#205355=CARTESIAN_POINT('Ctrl Pts',(-62.1763568600274,29.2763871704856,
-215.149949));
#205356=CARTESIAN_POINT('Ctrl Pts',(-48.9276804568491,16.5213744800396,
-235.35005));
#205357=CARTESIAN_POINT('Ctrl Pts',(-53.2999213760048,20.7375175535383,
-228.68335));
#205358=CARTESIAN_POINT('Ctrl Pts',(-57.6721622952182,24.9536606256242,
-222.01665));
#205359=CARTESIAN_POINT('Ctrl Pts',(-62.0444032145096,29.1698036957335,
-215.34995));
#205360=CARTESIAN_POINT('Ctrl Pts',(-62.0881256237025,29.2119651264346,
-215.283283));
#205361=CARTESIAN_POINT('Ctrl Pts',(-62.1318480328954,29.2541265571357,
-215.216616));
#205362=CARTESIAN_POINT('Ctrl Pts',(-62.1755704420884,29.2962879878368,
-215.149949));
#205363=CARTESIAN_POINT('Ctrl Pts',(-48.9214109907111,16.6748094040191,
-235.35005));
#205364=CARTESIAN_POINT('Ctrl Pts',(-53.2924626390134,20.9224124018924,
-228.68335));
#205365=CARTESIAN_POINT('Ctrl Pts',(-57.663528252029,25.170015967144,-222.01665));
#205366=CARTESIAN_POINT('Ctrl Pts',(-62.0346078304961,29.4176200813015,
-215.34995));
#205367=CARTESIAN_POINT('Ctrl Pts',(-62.0783186262808,29.4600961224431,
-215.283283));
#205368=CARTESIAN_POINT('Ctrl Pts',(-62.1220294220655,29.5025721635847,
-215.216616));
#205369=CARTESIAN_POINT('Ctrl Pts',(-62.1657402178502,29.5450482047262,
-215.149949));
#205370=CARTESIAN_POINT('Ctrl Pts',(-48.8992712925998,16.9131404133547,
-235.35005));
#205371=CARTESIAN_POINT('Ctrl Pts',(-53.2652870417935,21.2619501899207,
-228.68335));
#205372=CARTESIAN_POINT('Ctrl Pts',(-57.6313776897902,25.6107124643303,
-222.01665));
#205373=CARTESIAN_POINT('Ctrl Pts',(-61.9975402416511,29.9594276183431,
-215.34995));
#205374=CARTESIAN_POINT('Ctrl Pts',(-62.0412018671697,30.0029147698833,
-215.283283));
#205375=CARTESIAN_POINT('Ctrl Pts',(-62.0848634926883,30.0464019214233,
-215.216616));
#205376=CARTESIAN_POINT('Ctrl Pts',(-62.1285251182069,30.0898890729635,
-215.149949));
#205377=CARTESIAN_POINT('Ctrl Pts',(-48.8533444192211,17.2181014412188,
-235.35005));
#205378=CARTESIAN_POINT('Ctrl Pts',(-53.1855995667747,21.7941761255924,
-228.68335));
#205379=CARTESIAN_POINT('Ctrl Pts',(-57.5179747573295,26.3699864363254,
-222.01665));
#205380=CARTESIAN_POINT('Ctrl Pts',(-61.8504540244681,30.9455347714532,
-215.34995));
#205381=CARTESIAN_POINT('Ctrl Pts',(-61.8937788171395,30.9912902548045,
-215.283283));
#205382=CARTESIAN_POINT('Ctrl Pts',(-61.9371036098109,31.0370457381558,
-215.216616));
#205383=CARTESIAN_POINT('Ctrl Pts',(-61.9804284024823,31.082801221507,-215.149949));
#205384=CARTESIAN_POINT('Ctrl Pts',(-48.793774157437,17.4925774935122,-235.35005));
#205385=CARTESIAN_POINT('Ctrl Pts',(-53.0569741223029,22.3329163118503,
-228.68335));
#205386=CARTESIAN_POINT('Ctrl Pts',(-57.3203153214379,27.1726388120429,
-222.01665));
#205387=CARTESIAN_POINT('Ctrl Pts',(-61.5837608612094,32.0117507116806,
-215.34995));
#205388=CARTESIAN_POINT('Ctrl Pts',(-61.6263953166071,32.060141830677,-215.283283));
#205389=CARTESIAN_POINT('Ctrl Pts',(-61.6690297720048,32.1085329496734,
-215.216616));
#205390=CARTESIAN_POINT('Ctrl Pts',(-61.7116642274025,32.1569240686698,
-215.149949));
#205391=CARTESIAN_POINT('Ctrl Pts',(-48.7243271460874,17.7538206185435,
-235.35005));
#205392=CARTESIAN_POINT('Ctrl Pts',(-52.8915700395936,22.8426678835018,
-228.68335));
#205393=CARTESIAN_POINT('Ctrl Pts',(-57.0589527628024,27.9304206519508,
-222.01665));
#205394=CARTESIAN_POINT('Ctrl Pts',(-61.2264100602501,33.0170891792215,
-215.34995));
#205395=CARTESIAN_POINT('Ctrl Pts',(-61.2680846332245,33.0679558644942,
-215.283283));
#205396=CARTESIAN_POINT('Ctrl Pts',(-61.309759206199,33.1188225497669,-215.216616));
#205397=CARTESIAN_POINT('Ctrl Pts',(-61.3514337791735,33.1696892350396,
-215.149949));
#205398=CARTESIAN_POINT('Ctrl Pts',(-48.6354732464631,18.0177190827397,
-235.35005));
#205399=CARTESIAN_POINT('Ctrl Pts',(-52.6780922604543,23.3513726702934,
-228.68335));
#205400=CARTESIAN_POINT('Ctrl Pts',(-56.7208284608432,28.6833361882777,
-222.01665));
#205401=CARTESIAN_POINT('Ctrl Pts',(-60.7635813168395,34.0136255628538,
-215.34995));
#205402=CARTESIAN_POINT('Ctrl Pts',(-60.8040088453995,34.0669284565996,
-215.283283));
#205403=CARTESIAN_POINT('Ctrl Pts',(-60.8444363739595,34.1202313503453,
-215.216616));
#205404=CARTESIAN_POINT('Ctrl Pts',(-60.8848639025194,34.1735342440911,
-215.149949));
#205405=CARTESIAN_POINT('Ctrl Pts',(-48.5352774797299,18.2802794424427,
-235.35005));
#205406=CARTESIAN_POINT('Ctrl Pts',(-52.4343101169869,23.8247568642913,
-228.68335));
#205407=CARTESIAN_POINT('Ctrl Pts',(-56.3334174156944,29.3668400879758,
-222.016650000001));
#205408=CARTESIAN_POINT('Ctrl Pts',(-60.2324571773606,34.9065517584836,
-215.349950000001));
#205409=CARTESIAN_POINT('Ctrl Pts',(-60.2714475749772,34.9619488751887,
-215.283283000001));
#205410=CARTESIAN_POINT('Ctrl Pts',(-60.3104379725939,35.0173459918937,
-215.216616));
#205411=CARTESIAN_POINT('Ctrl Pts',(-60.3494283702106,35.0727431085988,
-215.149949000001));
#205412=CARTESIAN_POINT('Ctrl Pts',(-48.3890207412154,18.5878255918932,
-235.35005));
#205413=CARTESIAN_POINT('Ctrl Pts',(-52.1962991404372,24.228375758149,-228.68335));
#205414=CARTESIAN_POINT('Ctrl Pts',(-56.0035911516163,29.8657278812732,
-222.01665));
#205415=CARTESIAN_POINT('Ctrl Pts',(-59.810707037304,35.4999122879811,-215.34995));
#205416=CARTESIAN_POINT('Ctrl Pts',(-59.8487781961609,35.5562541320482,
-215.283283));
#205417=CARTESIAN_POINT('Ctrl Pts',(-59.8868493550178,35.6125959761153,
-215.216616));
#205418=CARTESIAN_POINT('Ctrl Pts',(-59.9249205138747,35.6689378201824,
-215.149949));
#205419=CARTESIAN_POINT('Ctrl Pts',(-48.2711217441656,18.8106246802399,
-235.35005));
#205420=CARTESIAN_POINT('Ctrl Pts',(-52.0406861996216,24.475501377336,-228.68335));
#205421=CARTESIAN_POINT('Ctrl Pts',(-55.8102121224059,30.1365835498488,
-222.01665));
#205422=CARTESIAN_POINT('Ctrl Pts',(-59.5794745156759,35.7939072308497,
-215.34995));
#205423=CARTESIAN_POINT('Ctrl Pts',(-59.6171671396086,35.8504804676597,
-215.283283));
#205424=CARTESIAN_POINT('Ctrl Pts',(-59.6548597635413,35.9070537044696,
-215.216616));
#205425=CARTESIAN_POINT('Ctrl Pts',(-59.692552387474,35.9636269412797,-215.149949));
#205426=CARTESIAN_POINT('Ctrl Pts',(-48.1560655143106,18.9923105754345,
-235.35005));
#205427=CARTESIAN_POINT('Ctrl Pts',(-51.9286217775904,24.6399928719346,
-228.68335));
#205428=CARTESIAN_POINT('Ctrl Pts',(-55.7011108008251,30.2835687301176,
-222.01665));
#205429=CARTESIAN_POINT('Ctrl Pts',(-59.4732891526392,35.9230771683515,
-215.34995));
#205430=CARTESIAN_POINT('Ctrl Pts',(-59.5110109361573,35.9794722527339,
-215.283283));
#205431=CARTESIAN_POINT('Ctrl Pts',(-59.5487327196755,36.0358673371162,
-215.216616));
#205432=CARTESIAN_POINT('Ctrl Pts',(-59.5864545031936,36.0922624214986,
-215.149949));
#205433=CARTESIAN_POINT('Ctrl Pts',(-48.1468610159222,19.00684544705,-235.35005));
#205434=CARTESIAN_POINT('Ctrl Pts',(-51.9196566238279,24.6531521915024,
-228.68335));
#205435=CARTESIAN_POINT('Ctrl Pts',(-55.6923826950986,30.2953275445391,
-222.01665));
#205436=CARTESIAN_POINT('Ctrl Pts',(-59.4647943235962,35.9334107633517,
-215.34995));
#205437=CARTESIAN_POINT('Ctrl Pts',(-59.5025184398812,35.9897915955398,
-215.283283));
#205438=CARTESIAN_POINT('Ctrl Pts',(-59.5402425561662,36.046172427728,-215.216616));
#205439=CARTESIAN_POINT('Ctrl Pts',(-59.5779666724512,36.102553259916,-215.149949));
#205440=CARTESIAN_POINT('Ctrl Pts',(-48.1376565175338,19.0213803186655,
-235.35005));
#205441=CARTESIAN_POINT('Ctrl Pts',(-51.9106914700654,24.6663115110703,
-228.68335));
#205442=CARTESIAN_POINT('Ctrl Pts',(-55.6836545893721,30.3070863589606,
-222.01665));
#205443=CARTESIAN_POINT('Ctrl Pts',(-59.4562994945533,35.9437443583519,
-215.34995));
#205444=CARTESIAN_POINT('Ctrl Pts',(-59.4940259436051,36.0001109383457,
-215.283283));
#205445=CARTESIAN_POINT('Ctrl Pts',(-59.5317523926569,36.0564775183397,
-215.216616));
#205446=CARTESIAN_POINT('Ctrl Pts',(-59.5694788417088,36.1128440983336,
-215.149949));
#205447=CARTESIAN_POINT('Ctrl Pts',(-48.1284520191454,19.0359151902811,
-235.35005));
#205448=CARTESIAN_POINT('Ctrl Pts',(-51.9017263163029,24.6794708306382,
-228.68335));
#205449=CARTESIAN_POINT('Ctrl Pts',(-55.6749264836457,30.3188451733821,
-222.01665));
#205450=CARTESIAN_POINT('Ctrl Pts',(-59.4478046655104,35.9540779533519,
-215.34995));
#205451=CARTESIAN_POINT('Ctrl Pts',(-59.485533447329,36.0104302811517,-215.283283));
#205452=CARTESIAN_POINT('Ctrl Pts',(-59.5232622291477,36.0667826089514,
-215.216616));
#205453=CARTESIAN_POINT('Ctrl Pts',(-59.5609910109663,36.1231349367511,
-215.149949));
#205454=CARTESIAN_POINT('',(-55.4860418356284,22.8455890891576,-225.35));
#205455=CARTESIAN_POINT('Ctrl Pts',(-48.4260896922586,19.3965417854656,
-234.872874618363));
#205456=CARTESIAN_POINT('Ctrl Pts',(-51.8397102119512,24.5067087698627,
-228.840465153427));
#205457=CARTESIAN_POINT('Ctrl Pts',(-55.2532709224339,29.6135143043896,
-222.808055688492));
#205458=CARTESIAN_POINT('Ctrl Pts',(-58.6665914736623,34.7169872964315,
-216.775646223556));
#205459=CARTESIAN_POINT('Origin',(-41.5452362233251,-63.7990866568863,-205.34995));
#205460=CARTESIAN_POINT('',(-48.8319431829163,-72.7145462807723,-205.34995));
#205461=CARTESIAN_POINT('',(-41.9984355604289,-75.3045692187324,-205.34995));
#205462=CARTESIAN_POINT('Origin',(0.,-12.9675000200281,-205.34995));
#205463=CARTESIAN_POINT('',(-59.6081272922882,-61.9689221688742,-205.34995));
#205464=CARTESIAN_POINT('Origin',(-50.7133971693864,-54.6569255427236,-205.34995));
#205465=CARTESIAN_POINT('',(-62.2188176672479,-55.1116977796555,-205.34995));
#205466=CARTESIAN_POINT('Origin',(-50.7133971693864,28.7219255026674,-205.34995));
#205467=CARTESIAN_POINT('',(-59.6081272922883,36.0339221288179,-205.34995));
#205468=CARTESIAN_POINT('',(-62.218817667248,29.176697739599,-205.34995));
#205469=CARTESIAN_POINT('Origin',(0.,-12.9675000200281,-205.34995));
#205470=CARTESIAN_POINT('',(-48.5592309447134,47.0014027710106,-205.34995));
#205471=CARTESIAN_POINT('Origin',(-41.3132181298675,38.0528376956935,-205.34995));
#205472=CARTESIAN_POINT('',(-43.4702127313761,49.3634032389879,-205.34995));
#205473=CARTESIAN_POINT('Origin',(1004.,-12.967500020028,-179.64995));
#205474=CARTESIAN_POINT('',(-65.1651121384123,-55.2281553161325,-179.64995));
#205475=CARTESIAN_POINT('',(-65.1651121384124,-55.2281553161325,-179.64995));
#205476=CARTESIAN_POINT('',(-65.1651121384124,29.2931552760762,-179.64995));
#205477=CARTESIAN_POINT('Origin',(1004.,-12.967500020028,-179.64995));
#205478=CARTESIAN_POINT('',(-65.1651121384125,29.293155276076,-179.64995));
#205479=CARTESIAN_POINT('Origin',(-50.7133971693864,28.7219255026673,-179.64995));
#205480=CARTESIAN_POINT('',(-61.8858792604563,37.9063695753764,-179.64995));
#205481=CARTESIAN_POINT('Origin',(-50.7133971693864,28.7219255026673,-179.64995));
#205482=CARTESIAN_POINT('',(-61.8858792604564,37.9063695753764,-179.64995));
#205483=CARTESIAN_POINT('Origin',(0.,-12.9675000200281,-179.64995));
#205484=CARTESIAN_POINT('',(-50.4147813349261,49.2929407301111,-179.64995));
#205485=CARTESIAN_POINT('Origin',(0.,-12.9675000200281,-179.64995));
#205486=CARTESIAN_POINT('',(-50.4147813349261,49.292940730111,-179.64995));
#205487=CARTESIAN_POINT('Origin',(-41.3132181298675,38.0528376956935,-179.64995));
#205488=CARTESIAN_POINT('',(-44.0225733573905,52.2597994838836,-179.64995));
#205489=CARTESIAN_POINT('Origin',(-41.3132181298675,38.0528376956935,-179.64995));
#205490=CARTESIAN_POINT('',(-44.0225733573905,52.2597994838836,-179.64995));
#205491=CARTESIAN_POINT('Origin',(-41.5452362233251,-63.7990866568863,-179.64995));
#205492=CARTESIAN_POINT('',(-42.1144903105792,-78.2508795831687,-179.64995));
#205493=CARTESIAN_POINT('',(-42.1144903105791,-78.2508795831687,-179.64995));
#205494=CARTESIAN_POINT('',(-50.6979144815776,-74.9976066350312,-179.64995));
#205495=CARTESIAN_POINT('Origin',(-41.5452362233251,-63.7990866568863,-179.64995));
#205496=CARTESIAN_POINT('',(-50.6979144815776,-74.9976066350312,-179.64995));
#205497=CARTESIAN_POINT('Origin',(0.,-12.9675000200281,-179.64995));
#205498=CARTESIAN_POINT('',(-61.8858792604563,-63.8413696154326,-179.64995));
#205499=CARTESIAN_POINT('Origin',(0.,-12.9675000200281,-179.64995));
#205500=CARTESIAN_POINT('',(-61.8858792604563,-63.8413696154326,-179.64995));
#205501=CARTESIAN_POINT('Origin',(-50.7133971693864,-54.6569255427236,-179.64995));
#205502=CARTESIAN_POINT('Origin',(-50.7133971693864,-54.6569255427236,-179.64995));
#205503=CARTESIAN_POINT('Ctrl Pts',(-48.9276804568491,-39.5283381317121,
-235.35005));
#205504=CARTESIAN_POINT('Ctrl Pts',(-53.2999213760692,-44.7204933330714,
-228.68335));
#205505=CARTESIAN_POINT('Ctrl Pts',(-57.6721622952894,-49.9126485344307,
-222.01665));
#205506=CARTESIAN_POINT('Ctrl Pts',(-62.0444032145095,-55.1048037357899,
-215.34995));
#205507=CARTESIAN_POINT('Ctrl Pts',(-49.0194233450359,-37.283081077169,
-235.35005));
#205508=CARTESIAN_POINT('Ctrl Pts',(-53.4090672042376,-42.0148742220589,
-228.683350000001));
#205509=CARTESIAN_POINT('Ctrl Pts',(-57.7985067146479,-46.7466590436653,
-222.016650000001));
#205510=CARTESIAN_POINT('Ctrl Pts',(-62.1877418657617,-51.4784358040522,
-215.34995));
#205511=CARTESIAN_POINT('Ctrl Pts',(-49.1841844420714,-32.7087365060477,
-235.35005));
#205512=CARTESIAN_POINT('Ctrl Pts',(-53.600359505658,-36.5883830285289,
-228.68335));
#205513=CARTESIAN_POINT('Ctrl Pts',(-58.0165345692446,-40.4680295510101,
-222.01665));
#205514=CARTESIAN_POINT('Ctrl Pts',(-62.4327096328312,-44.3476760734913,
-215.34995));
#205515=CARTESIAN_POINT('Ctrl Pts',(-49.3659986639477,-25.6715165814334,
-235.35005));
#205516=CARTESIAN_POINT('Ctrl Pts',(-53.8070961606803,-28.4006856868431,
-228.68335));
#205517=CARTESIAN_POINT('Ctrl Pts',(-58.2481936574129,-31.1298547922528,
-222.01665));
#205518=CARTESIAN_POINT('Ctrl Pts',(-62.6892911541455,-33.8590238976625,
-215.34995));
#205519=CARTESIAN_POINT('Ctrl Pts',(-49.4760453414413,-18.5583238061847,
-235.35005));
#205520=CARTESIAN_POINT('Ctrl Pts',(-53.9314601157808,-20.1883767671888,
-228.68335));
#205521=CARTESIAN_POINT('Ctrl Pts',(-58.3868748901203,-21.8184297281929,
-222.01665));
#205522=CARTESIAN_POINT('Ctrl Pts',(-62.8422896644598,-23.448482689197,
-215.34995));
#205523=CARTESIAN_POINT('Ctrl Pts',(-49.5,-13.8395357876534,-235.35005));
#205524=CARTESIAN_POINT('Ctrl Pts',(-53.9589513940208,-14.7196423822522,
-228.68335));
#205525=CARTESIAN_POINT('Ctrl Pts',(-58.4179027880416,-15.599748976851,
-222.01665));
#205526=CARTESIAN_POINT('Ctrl Pts',(-62.8768541820624,-16.4798555714498,
-215.34995));
#205527=CARTESIAN_POINT('Ctrl Pts',(-49.5,-11.5034818258362,-235.35005));
#205528=CARTESIAN_POINT('Ctrl Pts',(-53.9589513940208,-11.9914878905669,
-228.68335));
#205529=CARTESIAN_POINT('Ctrl Pts',(-58.4179027880416,-12.4794939552975,
-222.01665));
#205530=CARTESIAN_POINT('Ctrl Pts',(-62.8768541820624,-12.9675000200282,
-215.34995));
#205531=CARTESIAN_POINT('Ctrl Pts',(-49.5,-11.5034818258362,-235.35005));
#205532=CARTESIAN_POINT('Ctrl Pts',(-53.9589513940208,-11.9914878905669,
-228.68335));
#205533=CARTESIAN_POINT('Ctrl Pts',(-58.4179027880416,-12.4794939552975,
-222.01665));
#205534=CARTESIAN_POINT('Ctrl Pts',(-62.8768541820624,-12.9675000200282,
-215.34995));
#205535=CARTESIAN_POINT('Ctrl Pts',(-62.9214436960026,-12.9723800806755,
-215.283283));
#205536=CARTESIAN_POINT('Ctrl Pts',(-62.9660332099428,-12.9772601413228,
-215.216616));
#205537=CARTESIAN_POINT('Ctrl Pts',(-63.010622723883,-12.9821402019701,
-215.149949));
#205538=CARTESIAN_POINT('Ctrl Pts',(-49.5,-9.16742786401911,-235.35005));
#205539=CARTESIAN_POINT('Ctrl Pts',(-53.9589513940208,-9.26333339888158,
-228.68335));
#205540=CARTESIAN_POINT('Ctrl Pts',(-58.4179027880416,-9.35923893374405,
-222.01665));
#205541=CARTESIAN_POINT('Ctrl Pts',(-62.8768541820624,-9.45514446860653,
-215.34995));
#205542=CARTESIAN_POINT('Ctrl Pts',(-62.9214436960026,-9.45610352395515,
-215.283283));
#205543=CARTESIAN_POINT('Ctrl Pts',(-62.9660332099428,-9.45706257930377,
-215.216616));
#205544=CARTESIAN_POINT('Ctrl Pts',(-63.010622723883,-9.4580216346524,-215.149949));
#205545=CARTESIAN_POINT('Ctrl Pts',(-49.4760453034623,-4.44863709409477,
-235.35005));
#205546=CARTESIAN_POINT('Ctrl Pts',(-53.9314600904615,-3.79459717968296,
-228.68335));
#205547=CARTESIAN_POINT('Ctrl Pts',(-58.3868748774607,-3.14055726527114,
-222.01665));
#205548=CARTESIAN_POINT('Ctrl Pts',(-62.8422896644599,-2.48651735085932,
-215.34995));
#205549=CARTESIAN_POINT('Ctrl Pts',(-62.8868438123299,-2.47997695171521,
-215.283283));
#205550=CARTESIAN_POINT('Ctrl Pts',(-62.9313979601999,-2.47343655257108,
-215.216616));
#205551=CARTESIAN_POINT('Ctrl Pts',(-62.9759521080699,-2.46689615342696,
-215.149949));
#205552=CARTESIAN_POINT('Ctrl Pts',(-49.3659992921549,2.6645466712911,-235.350050000001));
#205553=CARTESIAN_POINT('Ctrl Pts',(-53.8070965794851,4.41770573339612,
-228.683350000001));
#205554=CARTESIAN_POINT('Ctrl Pts',(-58.2481938668153,6.17086479550113,
-222.016650000001));
#205555=CARTESIAN_POINT('Ctrl Pts',(-62.6892911541455,7.92402385760615,
-215.349950000001));
#205556=CARTESIAN_POINT('Ctrl Pts',(-62.7337021270188,7.9415554482272,-215.283283000001));
#205557=CARTESIAN_POINT('Ctrl Pts',(-62.7781130998921,7.95908703884825,
-215.216616));
#205558=CARTESIAN_POINT('Ctrl Pts',(-62.8225240727654,7.9766186294693,-215.149949000001));
#205559=CARTESIAN_POINT('Ctrl Pts',(-49.1841830823307,9.70178317521733,
-235.35005));
#205560=CARTESIAN_POINT('Ctrl Pts',(-53.6003585991642,12.6054141279565,
-228.68335));
#205561=CARTESIAN_POINT('Ctrl Pts',(-58.0165341159977,15.5090450806958,
-222.01665));
#205562=CARTESIAN_POINT('Ctrl Pts',(-62.4327096328312,18.412676033435,-215.34995));
#205563=CARTESIAN_POINT('Ctrl Pts',(-62.4768713879996,18.4417123429624,
-215.283283));
#205564=CARTESIAN_POINT('Ctrl Pts',(-62.5210331431679,18.4707486524898,
-215.216616));
#205565=CARTESIAN_POINT('Ctrl Pts',(-62.5651948983362,18.4997849620172,
-215.149949));
#205566=CARTESIAN_POINT('Ctrl Pts',(-49.0194233450359,14.2761174254963,
-235.35005));
#205567=CARTESIAN_POINT('Ctrl Pts',(-53.4090672042376,18.031898440925,-228.68335));
#205568=CARTESIAN_POINT('Ctrl Pts',(-57.7985067146477,21.7876711330703,
-222.01665));
#205569=CARTESIAN_POINT('Ctrl Pts',(-62.1877418657617,25.5434357639959,
-215.34995));
#205570=CARTESIAN_POINT('Ctrl Pts',(-62.2316342172729,25.5809934103052,
-215.283283));
#205571=CARTESIAN_POINT('Ctrl Pts',(-62.275526568784,25.6185510566144,-215.216616));
#205572=CARTESIAN_POINT('Ctrl Pts',(-62.3194189202952,25.6561087029237,
-215.149949));
#205573=CARTESIAN_POINT('Ctrl Pts',(-48.9276804568491,16.5213744800396,
-235.35005));
#205574=CARTESIAN_POINT('Ctrl Pts',(-53.2999213760048,20.7375175535383,
-228.68335));
#205575=CARTESIAN_POINT('Ctrl Pts',(-57.6721622952182,24.9536606256242,
-222.01665));
#205576=CARTESIAN_POINT('Ctrl Pts',(-62.0444032145096,29.1698036957335,
-215.34995));
#205577=CARTESIAN_POINT('Ctrl Pts',(-62.0881256237025,29.2119651264346,
-215.283283));
#205578=CARTESIAN_POINT('Ctrl Pts',(-62.1318480328954,29.2541265571357,
-215.216616));
#205579=CARTESIAN_POINT('Ctrl Pts',(-62.1755704420884,29.2962879878368,
-215.149949));
#205580=CARTESIAN_POINT('Origin',(1004.,-12.967500020028,-205.34995));
#205581=CARTESIAN_POINT('Ctrl Pts',(-27.1569075795172,38.1844371310006,
-235.35005));
#205582=CARTESIAN_POINT('Ctrl Pts',(-32.5837764342019,41.8536056393876,
-228.68335));
#205583=CARTESIAN_POINT('Ctrl Pts',(-38.0106452875494,45.5227741479461,
-222.01665));
#205584=CARTESIAN_POINT('Ctrl Pts',(-43.4375141409548,49.1919426564936,
-215.34995));
#205585=CARTESIAN_POINT('Ctrl Pts',(-43.4917828294889,49.2286343415791,
-215.283283));
#205586=CARTESIAN_POINT('Ctrl Pts',(-43.5460515180229,49.2653260266646,
-215.216616));
#205587=CARTESIAN_POINT('Ctrl Pts',(-43.600320206557,49.30201771175,-215.149949));
#205588=CARTESIAN_POINT('Ctrl Pts',(-22.7175376169318,38.7537549124104,
-235.35005));
#205589=CARTESIAN_POINT('Ctrl Pts',(-27.2067518411579,42.6544032575593,
-228.68335));
#205590=CARTESIAN_POINT('Ctrl Pts',(-31.7011009472754,46.5938202572852,
-222.01665));
#205591=CARTESIAN_POINT('Ctrl Pts',(-36.2028725106807,50.5716334315145,
-215.34995));
#205592=CARTESIAN_POINT('Ctrl Pts',(-36.2478902263148,50.6114115632568,
-215.283283));
#205593=CARTESIAN_POINT('Ctrl Pts',(-36.2929079419489,50.6511896949991,
-215.216616));
#205594=CARTESIAN_POINT('Ctrl Pts',(-36.3379256575829,50.6909678267414,
-215.149949));
#205595=CARTESIAN_POINT('Ctrl Pts',(-13.711356444076,39.6240660636921,-235.35005));
#205596=CARTESIAN_POINT('Ctrl Pts',(-16.3741503826813,43.8592570013518,
-228.68335));
#205597=CARTESIAN_POINT('Ctrl Pts',(-19.0446466451262,48.1913695751969,
-222.01665));
#205598=CARTESIAN_POINT('Ctrl Pts',(-21.7262765934597,52.6194725853171,
-215.34995));
#205599=CARTESIAN_POINT('Ctrl Pts',(-21.753092892943,52.6637536154183,-215.283283));
#205600=CARTESIAN_POINT('Ctrl Pts',(-21.7799091924264,52.7080346455195,
-215.216616));
#205601=CARTESIAN_POINT('Ctrl Pts',(-21.8067254919097,52.7523156756207,
-215.149949));
#205602=CARTESIAN_POINT('Ctrl Pts',(5.03069808033274E-14,40.0660654363212,
-235.350050000001));
#205603=CARTESIAN_POINT('Ctrl Pts',(2.50315176572591E-14,44.4636082157172,
-228.683350000001));
#205604=CARTESIAN_POINT('Ctrl Pts',(-3.67646180426256E-14,48.9871491221026,
-222.016650000001));
#205605=CARTESIAN_POINT('Ctrl Pts',(2.42861286636753E-14,53.6354775956494,
-215.34995));
#205606=CARTESIAN_POINT('Ctrl Pts',(2.48966361307383E-14,53.6819608803848,
-215.283283));
#205607=CARTESIAN_POINT('Ctrl Pts',(2.55071435978013E-14,53.7284441651203,
-215.216616));
#205608=CARTESIAN_POINT('Ctrl Pts',(2.61176510648644E-14,53.7749274498558,
-215.149949));
#205609=CARTESIAN_POINT('Ctrl Pts',(13.7113564440761,39.6240660636921,-235.35005));
#205610=CARTESIAN_POINT('Ctrl Pts',(16.3741503826814,43.8592570013518,-228.68335));
#205611=CARTESIAN_POINT('Ctrl Pts',(19.0446466451262,48.1913695751964,-222.01665));
#205612=CARTESIAN_POINT('Ctrl Pts',(21.7262765934598,52.619472585317,-215.34995));
#205613=CARTESIAN_POINT('Ctrl Pts',(21.7530928929431,52.6637536154182,-215.283283));
#205614=CARTESIAN_POINT('Ctrl Pts',(21.7799091924265,52.7080346455194,-215.216616));
#205615=CARTESIAN_POINT('Ctrl Pts',(21.8067254919098,52.7523156756206,-215.149949));
#205616=CARTESIAN_POINT('Ctrl Pts',(22.7175376169319,38.7537549124104,-235.350050000001));
#205617=CARTESIAN_POINT('Ctrl Pts',(27.206751841158,42.6544032575593,-228.68335));
#205618=CARTESIAN_POINT('Ctrl Pts',(31.7011009472754,46.5938202572849,-222.01665));
#205619=CARTESIAN_POINT('Ctrl Pts',(36.2028725106808,50.5716334315145,-215.34995));
#205620=CARTESIAN_POINT('Ctrl Pts',(36.2478902263149,50.6114115632568,-215.283283));
#205621=CARTESIAN_POINT('Ctrl Pts',(36.2929079419489,50.6511896949991,-215.216616));
#205622=CARTESIAN_POINT('Ctrl Pts',(36.337925657583,50.6909678267414,-215.149949));
#205623=CARTESIAN_POINT('Ctrl Pts',(27.1569075795173,38.1844371310006,-235.35005));
#205624=CARTESIAN_POINT('Ctrl Pts',(32.5837764342019,41.8536056393876,-228.68335));
#205625=CARTESIAN_POINT('Ctrl Pts',(38.0106452875494,45.5227741479461,-222.01665));
#205626=CARTESIAN_POINT('Ctrl Pts',(43.4375141409549,49.1919426564936,-215.34995));
#205627=CARTESIAN_POINT('Ctrl Pts',(43.491782829489,49.2286343415791,-215.283283));
#205628=CARTESIAN_POINT('Ctrl Pts',(43.546051518023,49.2653260266646,-215.216616));
#205629=CARTESIAN_POINT('Ctrl Pts',(43.6003202065571,49.30201771175,-215.149949));
#205630=CARTESIAN_POINT('Ctrl Pts',(24.4459324049495,-62.4902066935372,
-235.35005));
#205631=CARTESIAN_POINT('Ctrl Pts',(30.2944767260349,-66.7035224039814,
-228.68335));
#205632=CARTESIAN_POINT('Ctrl Pts',(36.1430210443398,-70.9168381145246,
-222.01665));
#205633=CARTESIAN_POINT('Ctrl Pts',(41.991565360621,-75.1301538251475,-215.34995));
#205634=CARTESIAN_POINT('Ctrl Pts',(42.0500508037838,-75.1722869822537,
-215.283283));
#205635=CARTESIAN_POINT('Ctrl Pts',(42.1085362469466,-75.21442013936,-215.216616));
#205636=CARTESIAN_POINT('Ctrl Pts',(42.1670216901095,-75.2565532964662,
-215.149949));
#205637=CARTESIAN_POINT('Ctrl Pts',(20.4621956228808,-62.6321691537996,
-235.35005));
#205638=CARTESIAN_POINT('Ctrl Pts',(25.267980358079,-66.8889339565476,-228.68335));
#205639=CARTESIAN_POINT('Ctrl Pts',(30.0738587790242,-71.1483055815339,
-222.01665));
#205640=CARTESIAN_POINT('Ctrl Pts',(34.8798403105591,-75.4102836728986,
-215.34995));
#205641=CARTESIAN_POINT('Ctrl Pts',(34.9279001258744,-75.4529034538122,
-215.283283));
#205642=CARTESIAN_POINT('Ctrl Pts',(34.9759599411898,-75.4955232347258,
-215.216616));
#205643=CARTESIAN_POINT('Ctrl Pts',(35.0240197565051,-75.5381430156395,
-215.149949));
#205644=CARTESIAN_POINT('Ctrl Pts',(12.3633338208145,-62.8510026026509,
-235.35005));
#205645=CARTESIAN_POINT('Ctrl Pts',(15.1854795229237,-67.1680657809434,
-228.68335));
#205646=CARTESIAN_POINT('Ctrl Pts',(18.0077657557388,-71.4916460146837,
-222.01665));
#205647=CARTESIAN_POINT('Ctrl Pts',(20.8302066559562,-75.8217424142497,
-215.34995));
#205648=CARTESIAN_POINT('Ctrl Pts',(20.8584310649584,-75.8650433782453,
-215.283283));
#205649=CARTESIAN_POINT('Ctrl Pts',(20.8866554739606,-75.908344342241,-215.216616));
#205650=CARTESIAN_POINT('Ctrl Pts',(20.9148798829627,-75.9516453062367,
-215.149949));
#205651=CARTESIAN_POINT('Ctrl Pts',(1.09287578986539E-13,-62.9629927582852,
-235.35005));
#205652=CARTESIAN_POINT('Ctrl Pts',(-1.49836951995733E-13,-67.3083190291539,
-228.683350000001));
#205653=CARTESIAN_POINT('Ctrl Pts',(-3.24284869790415E-13,-71.6621174720752,
-222.016650000001));
#205654=CARTESIAN_POINT('Ctrl Pts',(-5.36029554076834E-13,-76.0243869305461,
-215.349950000001));
#205655=CARTESIAN_POINT('Ctrl Pts',(-5.38147000919697E-13,-76.0680096251308,
-215.283283000001));
#205656=CARTESIAN_POINT('Ctrl Pts',(-5.40264447762562E-13,-76.1116323197155,
-215.216616000001));
#205657=CARTESIAN_POINT('Ctrl Pts',(-5.42381894605426E-13,-76.1552550143002,
-215.149949000001));
#205658=CARTESIAN_POINT('Ctrl Pts',(-12.3633338208143,-62.8510026026509,
-235.35005));
#205659=CARTESIAN_POINT('Ctrl Pts',(-15.185479522924,-67.1680657809432,
-228.68335));
#205660=CARTESIAN_POINT('Ctrl Pts',(-18.0077657557395,-71.4916460146835,
-222.01665));
#205661=CARTESIAN_POINT('Ctrl Pts',(-20.8302066559573,-75.8217424142497,
-215.34995));
#205662=CARTESIAN_POINT('Ctrl Pts',(-20.8584310649595,-75.8650433782453,
-215.283283));
#205663=CARTESIAN_POINT('Ctrl Pts',(-20.8866554739617,-75.908344342241,
-215.216616));
#205664=CARTESIAN_POINT('Ctrl Pts',(-20.9148798829638,-75.9516453062367,
-215.149949));
#205665=CARTESIAN_POINT('Ctrl Pts',(-20.4621956228805,-62.6321691537997,
-235.35005));
#205666=CARTESIAN_POINT('Ctrl Pts',(-25.2679803580793,-66.8889339565475,
-228.68335));
#205667=CARTESIAN_POINT('Ctrl Pts',(-30.0738587790249,-71.1483055815338,
-222.01665));
#205668=CARTESIAN_POINT('Ctrl Pts',(-34.8798403105602,-75.4102836728983,
-215.34995));
#205669=CARTESIAN_POINT('Ctrl Pts',(-34.9279001258756,-75.4529034538119,
-215.283283));
#205670=CARTESIAN_POINT('Ctrl Pts',(-34.975959941191,-75.4955232347256,
-215.216616));
#205671=CARTESIAN_POINT('Ctrl Pts',(-35.0240197565063,-75.5381430156392,
-215.149949));
#205672=CARTESIAN_POINT('Ctrl Pts',(-24.4459324049493,-62.4902066935372,
-235.35005));
#205673=CARTESIAN_POINT('Ctrl Pts',(-30.2944767260352,-66.7035224039813,
-228.68335));
#205674=CARTESIAN_POINT('Ctrl Pts',(-36.1430210443405,-70.9168381145244,
-222.01665));
#205675=CARTESIAN_POINT('Ctrl Pts',(-41.9915653606222,-75.1301538251473,
-215.34995));
#205676=CARTESIAN_POINT('Ctrl Pts',(-42.050050803785,-75.1722869822535,
-215.283283));
#205677=CARTESIAN_POINT('Ctrl Pts',(-42.1085362469478,-75.2144201393598,
-215.216616));
#205678=CARTESIAN_POINT('Ctrl Pts',(-42.1670216901106,-75.256553296466,
-215.149949));
#205679=CARTESIAN_POINT('Origin',(0.,-12.9675000200281,-218.35005));
#205680=CARTESIAN_POINT('Ctrl Pts',(-7312.83864083626,-22580.9607088348,
-376.75075701007));
#205681=CARTESIAN_POINT('Ctrl Pts',(-6830.77747415825,-19700.0678309805,
-349.81728900813));
#205682=CARTESIAN_POINT('Ctrl Pts',(-6348.71630748024,-16819.1749531262,
-322.88382100619));
#205683=CARTESIAN_POINT('Ctrl Pts',(-5866.65514080223,-13938.2820752719,
-295.95035300425));
#205684=CARTESIAN_POINT('Ctrl Pts',(-5625.62455746322,-12497.8356363448,
-282.483619003281));
#205685=CARTESIAN_POINT('Ctrl Pts',(-5384.59397412422,-11057.3891974177,
-269.01688500231));
#205686=CARTESIAN_POINT('Ctrl Pts',(-5143.56339078521,-9616.94275849054,
-255.55015100134));
#205687=CARTESIAN_POINT('Ctrl Pts',(-5023.0480991157,-8896.71953902697,
-248.816784000855));
#205688=CARTESIAN_POINT('Ctrl Pts',(-4902.5328074462,-8176.49631956341,
-242.083417000367));
#205689=CARTESIAN_POINT('Ctrl Pts',(-4782.0175157767,-7456.27310009984,
-235.350049999879));
#205690=CARTESIAN_POINT('Ctrl Pts',(-4662.69544481679,-6743.18080360126,
-228.683349999394));
#205691=CARTESIAN_POINT('Ctrl Pts',(-4544.55443977813,-6017.25926759624,
-222.01665));
#205692=CARTESIAN_POINT('Ctrl Pts',(-4428.35272571124,-5278.63127980493,
-215.34995));
#205693=CARTESIAN_POINT('Ctrl Pts',(-4427.19070857058,-5271.24499992702,
-215.283283));
#205694=CARTESIAN_POINT('Ctrl Pts',(-4426.02869142993,-5263.85872004911,
-215.216616));
#205695=CARTESIAN_POINT('Ctrl Pts',(-4424.86667428927,-5256.4724401712,
-215.149949));
#205696=CARTESIAN_POINT('Ctrl Pts',(-5678.44144856441,-17578.5062585325,
-376.75075700783));
#205697=CARTESIAN_POINT('Ctrl Pts',(-5307.04370444825,-15333.6138629625,
-349.817289006321));
#205698=CARTESIAN_POINT('Ctrl Pts',(-4935.64596033209,-13088.7214673926,
-322.883821004812));
#205699=CARTESIAN_POINT('Ctrl Pts',(-4564.24821621593,-10843.8290718226,
-295.950353003305));
#205700=CARTESIAN_POINT('Ctrl Pts',(-4378.54934415786,-9721.38287403765,
-282.48361900255));
#205701=CARTESIAN_POINT('Ctrl Pts',(-4192.85047209977,-8598.93667625267,
-269.016885001796));
#205702=CARTESIAN_POINT('Ctrl Pts',(-4007.1516000417,-7476.4904784677,-255.550151001042));
#205703=CARTESIAN_POINT('Ctrl Pts',(-3914.30216401265,-6915.26737957521,
-248.816784000665));
#205704=CARTESIAN_POINT('Ctrl Pts',(-3821.45272798362,-6354.04428068272,
-242.083417000286));
#205705=CARTESIAN_POINT('Ctrl Pts',(-3728.60329195457,-5792.82118179023,
-235.350049999906));
#205706=CARTESIAN_POINT('Ctrl Pts',(-3636.67315727236,-5237.15474724321,
-228.683349999529));
#205707=CARTESIAN_POINT('Ctrl Pts',(-3545.66125393428,-4671.51484522691,
-222.01665));
#205708=CARTESIAN_POINT('Ctrl Pts',(-3456.15702691661,-4095.9969311378,
-215.34995));
#205709=CARTESIAN_POINT('Ctrl Pts',(-3455.26198464644,-4090.24175199691,
-215.283283));
#205710=CARTESIAN_POINT('Ctrl Pts',(-3454.36694237628,-4084.48657285602,
-215.216616));
#205711=CARTESIAN_POINT('Ctrl Pts',(-3453.47190010611,-4078.73139371513,
-215.149949));
#205712=CARTESIAN_POINT('Ctrl Pts',(-4044.04425629255,-12576.0518082303,
-376.750757005589));
#205713=CARTESIAN_POINT('Ctrl Pts',(-3783.30993473824,-10967.1598949446,
-349.817289004512));
#205714=CARTESIAN_POINT('Ctrl Pts',(-3522.57561318394,-9358.26798165898,
-322.883821003436));
#205715=CARTESIAN_POINT('Ctrl Pts',(-3261.84129162964,-7749.37606837333,
-295.950353002358));
#205716=CARTESIAN_POINT('Ctrl Pts',(-3131.47413085249,-6944.9301117305,
-282.483619001821));
#205717=CARTESIAN_POINT('Ctrl Pts',(-3001.10697007533,-6140.48415508768,
-269.016885001282));
#205718=CARTESIAN_POINT('Ctrl Pts',(-2870.73980929818,-5336.03819844486,
-255.550151000744));
#205719=CARTESIAN_POINT('Ctrl Pts',(-2805.5562289096,-4933.81522012345,
-248.816784000475));
#205720=CARTESIAN_POINT('Ctrl Pts',(-2740.37264852102,-4531.59224180204,
-242.083417000204));
#205721=CARTESIAN_POINT('Ctrl Pts',(-2675.18906813245,-4129.36926348062,
-235.350049999933));
#205722=CARTESIAN_POINT('Ctrl Pts',(-2610.65086972792,-3731.12869088517,
-228.683349999664));
#205723=CARTESIAN_POINT('Ctrl Pts',(-2546.76806809043,-3325.77042285759,
-222.01665));
#205724=CARTESIAN_POINT('Ctrl Pts',(-2483.96132812197,-2913.36258247067,
-215.34995));
#205725=CARTESIAN_POINT('Ctrl Pts',(-2483.3332607223,-2909.2385040668,-215.283283));
#205726=CARTESIAN_POINT('Ctrl Pts',(-2482.70519332262,-2905.11442566293,
-215.216616));
#205727=CARTESIAN_POINT('Ctrl Pts',(-2482.07712592294,-2900.99034725906,
-215.149949));
#205728=CARTESIAN_POINT('Ctrl Pts',(-2409.6470640207,-7573.59735792804,
-376.750757003348));
#205729=CARTESIAN_POINT('Ctrl Pts',(-2259.57616502824,-6600.7059269267,
-349.817289002703));
#205730=CARTESIAN_POINT('Ctrl Pts',(-2109.5052660358,-5627.81449592536,
-322.883821002058));
#205731=CARTESIAN_POINT('Ctrl Pts',(-1959.43436704334,-4654.92306492402,
-295.950353001413));
#205732=CARTESIAN_POINT('Ctrl Pts',(-1884.39891754712,-4168.47734942335,
-282.483619001091));
#205733=CARTESIAN_POINT('Ctrl Pts',(-1809.36346805089,-3682.03163392268,
-269.016885000768));
#205734=CARTESIAN_POINT('Ctrl Pts',(-1734.32801855467,-3195.58591842202,
-255.550151000446));
#205735=CARTESIAN_POINT('Ctrl Pts',(-1696.81029380655,-2952.36306067169,
-248.816784000284));
#205736=CARTESIAN_POINT('Ctrl Pts',(-1659.29256905844,-2709.14020292135,
-242.083417000122));
#205737=CARTESIAN_POINT('Ctrl Pts',(-1621.77484431033,-2465.91734517101,
-235.35004999996));
#205738=CARTESIAN_POINT('Ctrl Pts',(-1584.62858218348,-2225.10263452712,
-228.683349999799));
#205739=CARTESIAN_POINT('Ctrl Pts',(-1547.87488224658,-1980.02600048826,
-222.01665));
#205740=CARTESIAN_POINT('Ctrl Pts',(-1511.76562932734,-1730.72823380353,
-215.34995));
#205741=CARTESIAN_POINT('Ctrl Pts',(-1511.40453679815,-1728.23525613669,
-215.283283));
#205742=CARTESIAN_POINT('Ctrl Pts',(-1511.04344426897,-1725.74227846985,
-215.216616));
#205743=CARTESIAN_POINT('Ctrl Pts',(-1510.68235173978,-1723.249300803,-215.149949));
#205744=CARTESIAN_POINT('Ctrl Pts',(-1864.84799993008,-5906.11254116062,
-376.750757002601));
#205745=CARTESIAN_POINT('Ctrl Pts',(-1751.66490845825,-5145.22127092072,
-349.8172890021));
#205746=CARTESIAN_POINT('Ctrl Pts',(-1638.48181698641,-4384.33000068082,
-322.883821001599));
#205747=CARTESIAN_POINT('Ctrl Pts',(-1525.29872551458,-3623.43873044092,
-295.950353001097));
#205748=CARTESIAN_POINT('Ctrl Pts',(-1468.70717977866,-3242.99309532097,
-282.483619000847));
#205749=CARTESIAN_POINT('Ctrl Pts',(-1412.11563404274,-2862.54746020102,
-269.016885000597));
#205750=CARTESIAN_POINT('Ctrl Pts',(-1355.52408830682,-2482.10182508107,
-255.550151000346));
#205751=CARTESIAN_POINT('Ctrl Pts',(-1327.22831543887,-2291.87900752109,
-248.816784000221));
#205752=CARTESIAN_POINT('Ctrl Pts',(-1298.93254257091,-2101.65618996112,
-242.083417000095));
#205753=CARTESIAN_POINT('Ctrl Pts',(-1270.63676970295,-1911.43337240115,
-235.350049999969));
#205754=CARTESIAN_POINT('Ctrl Pts',(-1242.621153002,-1723.09394907444,-228.683349999844));
#205755=CARTESIAN_POINT('Ctrl Pts',(-1214.91048696529,-1531.44452636515,
-222.01665));
#205756=CARTESIAN_POINT('Ctrl Pts',(-1187.70039639579,-1336.51678424783,
-215.34995));
#205757=CARTESIAN_POINT('Ctrl Pts',(-1187.4282954901,-1334.56750682665,
-215.283283));
#205758=CARTESIAN_POINT('Ctrl Pts',(-1187.15619458441,-1332.61822940548,
-215.216616));
#205759=CARTESIAN_POINT('Ctrl Pts',(-1186.88409367872,-1330.66895198431,
-215.149949));
#205760=CARTESIAN_POINT('Ctrl Pts',(-1320.04893583946,-4238.62772439321,
-376.750757001854));
#205761=CARTESIAN_POINT('Ctrl Pts',(-1243.75365188824,-3689.73661491475,
-349.817289001497));
#205762=CARTESIAN_POINT('Ctrl Pts',(-1167.45836793703,-3140.84550543629,
-322.883821001139));
#205763=CARTESIAN_POINT('Ctrl Pts',(-1091.16308398581,-2591.95439595782,
-295.950353000782));
#205764=CARTESIAN_POINT('Ctrl Pts',(-1053.0154420102,-2317.50884121858,
-282.483619000604));
#205765=CARTESIAN_POINT('Ctrl Pts',(-1014.86780003459,-2043.06328647936,
-269.016885000425));
#205766=CARTESIAN_POINT('Ctrl Pts',(-976.720158058986,-1768.61773174013,
-255.550151000247));
#205767=CARTESIAN_POINT('Ctrl Pts',(-957.646337071182,-1631.39495437051,
-248.816784000158));
#205768=CARTESIAN_POINT('Ctrl Pts',(-938.572516083378,-1494.17217700089,
-242.083417000068));
#205769=CARTESIAN_POINT('Ctrl Pts',(-919.498695095574,-1356.94939963128,
-235.350049999978));
#205770=CARTESIAN_POINT('Ctrl Pts',(-900.61372382052,-1221.08526362176,
-228.683349999889));
#205771=CARTESIAN_POINT('Ctrl Pts',(-881.946091684011,-1082.86305224204,
-222.01665));
#205772=CARTESIAN_POINT('Ctrl Pts',(-863.635163464249,-942.305334692116,
-215.34995));
#205773=CARTESIAN_POINT('Ctrl Pts',(-863.452054182054,-940.899757516616,
-215.283283));
#205774=CARTESIAN_POINT('Ctrl Pts',(-863.268944899859,-939.494180341118,
-215.216616));
#205775=CARTESIAN_POINT('Ctrl Pts',(-863.085835617665,-938.088603165619,
-215.149949));
#205776=CARTESIAN_POINT('Ctrl Pts',(-775.24987174884,-2571.1429076258,-376.750757001107));
#205777=CARTESIAN_POINT('Ctrl Pts',(-735.842395318242,-2234.25195890877,
-349.817289000894));
#205778=CARTESIAN_POINT('Ctrl Pts',(-696.434918887644,-1897.36101019174,
-322.883821000681));
#205779=CARTESIAN_POINT('Ctrl Pts',(-657.027442457046,-1560.47006147472,
-295.950353000467));
#205780=CARTESIAN_POINT('Ctrl Pts',(-637.323704241746,-1392.0245871162,
-282.483619000361));
#205781=CARTESIAN_POINT('Ctrl Pts',(-617.619966026447,-1223.57911275769,
-269.016885000254));
#205782=CARTESIAN_POINT('Ctrl Pts',(-597.916227811148,-1055.13363839918,
-255.550151000147));
#205783=CARTESIAN_POINT('Ctrl Pts',(-588.064358703498,-970.910901219922,
-248.816784000094));
#205784=CARTESIAN_POINT('Ctrl Pts',(-578.212489595849,-886.688164040665,
-242.083417000041));
#205785=CARTESIAN_POINT('Ctrl Pts',(-568.360620488199,-802.465426861409,
-235.350049999987));
#205786=CARTESIAN_POINT('Ctrl Pts',(-558.606294639041,-719.076578169076,
-228.683349999934));
#205787=CARTESIAN_POINT('Ctrl Pts',(-548.981696402727,-634.281578118933,
-222.01665));
#205788=CARTESIAN_POINT('Ctrl Pts',(-539.569930532705,-548.093885136405,
-215.34995));
#205789=CARTESIAN_POINT('Ctrl Pts',(-539.475812874006,-547.23200820658,
-215.283283));
#205790=CARTESIAN_POINT('Ctrl Pts',(-539.381695215308,-546.370131276755,
-215.216616));
#205791=CARTESIAN_POINT('Ctrl Pts',(-539.287577556609,-545.50825434693,
-215.149949));
#205792=CARTESIAN_POINT('Ctrl Pts',(-593.650183718634,-2015.31463536999,
-376.750757000858));
#205793=CARTESIAN_POINT('Ctrl Pts',(-566.538643128242,-1749.09040690678,
-349.817289000693));
#205794=CARTESIAN_POINT('Ctrl Pts',(-539.427102537849,-1482.86617844356,
-322.883821000528));
#205795=CARTESIAN_POINT('Ctrl Pts',(-512.315561947457,-1216.64194998035,
-295.950353000362));
#205796=CARTESIAN_POINT('Ctrl Pts',(-498.759791652261,-1083.52983574874,
-282.48361900028));
#205797=CARTESIAN_POINT('Ctrl Pts',(-485.204021357065,-950.417721517136,
-269.016885000197));
#205798=CARTESIAN_POINT('Ctrl Pts',(-471.648251061869,-817.305607285529,
-255.550151000114));
#205799=CARTESIAN_POINT('Ctrl Pts',(-464.87036591427,-750.749550169726,
-248.816784000073));
#205800=CARTESIAN_POINT('Ctrl Pts',(-458.092480766672,-684.193493053923,
-242.083417000031));
#205801=CARTESIAN_POINT('Ctrl Pts',(-451.314595619074,-617.637435938119,
-235.35004999999));
#205802=CARTESIAN_POINT('Ctrl Pts',(-444.603818245215,-551.740349684848,
-228.683349999949));
#205803=CARTESIAN_POINT('Ctrl Pts',(-437.993564642299,-484.754420077896,
-222.01665));
#205804=CARTESIAN_POINT('Ctrl Pts',(-431.54818622219,-416.690068617835,
-215.34995));
#205805=CARTESIAN_POINT('Ctrl Pts',(-431.48373243799,-416.009425103234,
-215.283283));
#205806=CARTESIAN_POINT('Ctrl Pts',(-431.419278653791,-415.328781588633,
-215.216616));
#205807=CARTESIAN_POINT('Ctrl Pts',(-431.354824869591,-414.648138074033,
-215.149949));
#205808=CARTESIAN_POINT('Ctrl Pts',(-412.050495688428,-1459.48636311419,
-376.750757000609));
#205809=CARTESIAN_POINT('Ctrl Pts',(-397.234890938242,-1263.92885490479,
-349.817289000492));
#205810=CARTESIAN_POINT('Ctrl Pts',(-382.419286188055,-1068.37134669538,
-322.883821000374));
#205811=CARTESIAN_POINT('Ctrl Pts',(-367.603681437869,-872.813838485983,
-295.950353000257));
#205812=CARTESIAN_POINT('Ctrl Pts',(-360.195879062775,-775.035084381282,
-282.483619000199));
#205813=CARTESIAN_POINT('Ctrl Pts',(-352.788076687683,-677.256330276581,
-269.016885000139));
#205814=CARTESIAN_POINT('Ctrl Pts',(-345.380274312589,-579.477576171881,
-255.550151000081));
#205815=CARTESIAN_POINT('Ctrl Pts',(-341.676373125042,-530.58819911953,
-248.816784000052));
#205816=CARTESIAN_POINT('Ctrl Pts',(-337.972471937496,-481.69882206718,
-242.083417000022));
#205817=CARTESIAN_POINT('Ctrl Pts',(-334.26857074995,-432.80944501483,-235.350049999993));
#205818=CARTESIAN_POINT('Ctrl Pts',(-330.601341851388,-384.404121200621,
-228.683349999963));
#205819=CARTESIAN_POINT('Ctrl Pts',(-327.005432881871,-335.22726203686,
-222.01665));
#205820=CARTESIAN_POINT('Ctrl Pts',(-323.526441911676,-285.286252099265,
-215.34995));
#205821=CARTESIAN_POINT('Ctrl Pts',(-323.491652001974,-284.786841999889,
-215.283283));
#205822=CARTESIAN_POINT('Ctrl Pts',(-323.456862092273,-284.287431900513,
-215.216616));
#205823=CARTESIAN_POINT('Ctrl Pts',(-323.422072182572,-283.788021801137,
-215.149949));
#205824=CARTESIAN_POINT('Ctrl Pts',(-230.450807658222,-903.658090858384,
-376.75075700036));
#205825=CARTESIAN_POINT('Ctrl Pts',(-227.931138748241,-778.767302902795,
-349.817289000291));
#205826=CARTESIAN_POINT('Ctrl Pts',(-225.411469838261,-653.876514947205,
-322.883821000222));
#205827=CARTESIAN_POINT('Ctrl Pts',(-222.891800928281,-528.985726991616,
-295.950353000152));
#205828=CARTESIAN_POINT('Ctrl Pts',(-221.63196647329,-466.540333013821,
-282.483619000117));
#205829=CARTESIAN_POINT('Ctrl Pts',(-220.3721320183,-404.094939036027,-269.016885000082));
#205830=CARTESIAN_POINT('Ctrl Pts',(-219.11229756331,-341.649545058231,
-255.550151000048));
#205831=CARTESIAN_POINT('Ctrl Pts',(-218.482380335815,-310.426848069334,
-248.816784000031));
#205832=CARTESIAN_POINT('Ctrl Pts',(-217.85246310832,-279.204151080437,
-242.083417000013));
#205833=CARTESIAN_POINT('Ctrl Pts',(-217.222545880824,-247.981454091539,
-235.350049999996));
#205834=CARTESIAN_POINT('Ctrl Pts',(-216.598865457562,-217.067892716394,
-228.683349999979));
#205835=CARTESIAN_POINT('Ctrl Pts',(-216.017301121443,-185.700103995824,
-222.01665));
#205836=CARTESIAN_POINT('Ctrl Pts',(-215.504697601161,-153.882435580695,
-215.34995));
#205837=CARTESIAN_POINT('Ctrl Pts',(-215.499571565958,-153.564258896543,
-215.283283));
#205838=CARTESIAN_POINT('Ctrl Pts',(-215.494445530756,-153.246082212392,
-215.216616));
#205839=CARTESIAN_POINT('Ctrl Pts',(-215.489319495554,-152.92790552824,
-215.149949));
#205840=CARTESIAN_POINT('Ctrl Pts',(-169.91757831482,-718.38200010645,-376.750757000277));
#205841=CARTESIAN_POINT('Ctrl Pts',(-171.496554684908,-617.046785568798,
-349.817289000224));
#205842=CARTESIAN_POINT('Ctrl Pts',(-173.075531054996,-515.711571031146,
-322.883821000171));
#205843=CARTESIAN_POINT('Ctrl Pts',(-174.654507425084,-414.376356493494,
-295.950353000117));
#205844=CARTESIAN_POINT('Ctrl Pts',(-175.443995610129,-363.708749224667,
-282.48361900009));
#205845=CARTESIAN_POINT('Ctrl Pts',(-176.233483795173,-313.041141955842,
-269.016885000063));
#205846=CARTESIAN_POINT('Ctrl Pts',(-177.022971980217,-262.373534687016,
-255.550151000037));
#205847=CARTESIAN_POINT('Ctrl Pts',(-177.417716072739,-237.039731052603,
-248.816784000024));
#205848=CARTESIAN_POINT('Ctrl Pts',(-177.812460165261,-211.70592741819,
-242.08341700001));
#205849=CARTESIAN_POINT('Ctrl Pts',(-178.207204257783,-186.372123783777,
-235.350049999997));
#205850=CARTESIAN_POINT('Ctrl Pts',(-178.598039992953,-161.289149888318,
-228.683349999984));
#205851=CARTESIAN_POINT('Ctrl Pts',(-179.021257201301,-135.857717982145,
-222.01665));
#205852=CARTESIAN_POINT('Ctrl Pts',(-179.497449497656,-110.081163407838,
-215.34995));
#205853=CARTESIAN_POINT('Ctrl Pts',(-179.50221142062,-109.823397862094,
-215.283283));
#205854=CARTESIAN_POINT('Ctrl Pts',(-179.506973343583,-109.565632316351,
-215.216616));
#205855=CARTESIAN_POINT('Ctrl Pts',(-179.511735266547,-109.307866770608,
-215.149949));
#205856=CARTESIAN_POINT('Ctrl Pts',(-109.384348971418,-533.105909354515,
-376.750757000194));
#205857=CARTESIAN_POINT('Ctrl Pts',(-115.061970621574,-455.3262682348,-349.817289000156));
#205858=CARTESIAN_POINT('Ctrl Pts',(-120.739592271731,-377.546627115086,
-322.883821000119));
#205859=CARTESIAN_POINT('Ctrl Pts',(-126.417213921888,-299.766985995371,
-295.950353000081));
#205860=CARTESIAN_POINT('Ctrl Pts',(-129.256024746967,-260.877165435514,
-282.483619000063));
#205861=CARTESIAN_POINT('Ctrl Pts',(-132.094835572045,-221.987344875657,
-269.016885000044));
#205862=CARTESIAN_POINT('Ctrl Pts',(-134.933646397123,-183.097524315799,
-255.550151000025));
#205863=CARTESIAN_POINT('Ctrl Pts',(-136.353051809663,-163.652614035871,
-248.816784000016));
#205864=CARTESIAN_POINT('Ctrl Pts',(-137.772457222202,-144.207703755942,
-242.083417000007));
#205865=CARTESIAN_POINT('Ctrl Pts',(-139.191862634741,-124.762793476013,
-235.350049999998));
#205866=CARTESIAN_POINT('Ctrl Pts',(-140.597214528344,-105.510407060242,
-228.683349999989));
#205867=CARTESIAN_POINT('Ctrl Pts',(-142.025213281158,-86.0153319684663,
-222.01665));
#205868=CARTESIAN_POINT('Ctrl Pts',(-143.490201394151,-66.2798912349809,
-215.34995));
#205869=CARTESIAN_POINT('Ctrl Pts',(-143.504851275281,-66.082536827646,
-215.283283));
#205870=CARTESIAN_POINT('Ctrl Pts',(-143.519501156411,-65.8851824203112,
-215.216616));
#205871=CARTESIAN_POINT('Ctrl Pts',(-143.534151037541,-65.6878280129763,
-215.149949));
#205872=CARTESIAN_POINT('Ctrl Pts',(-48.8511196280154,-347.82981860258,
-376.750757000109));
#205873=CARTESIAN_POINT('Ctrl Pts',(-58.6273865582409,-293.605750900803,
-349.817289000088));
#205874=CARTESIAN_POINT('Ctrl Pts',(-68.4036534884664,-239.381683199026,
-322.883821000067));
#205875=CARTESIAN_POINT('Ctrl Pts',(-78.179920418692,-185.157615497249,
-295.950353000046));
#205876=CARTESIAN_POINT('Ctrl Pts',(-83.0680538838047,-158.04558164636,
-282.483619000036));
#205877=CARTESIAN_POINT('Ctrl Pts',(-87.9561873489175,-130.933547795471,
-269.016885000025));
#205878=CARTESIAN_POINT('Ctrl Pts',(-92.8443208140303,-103.821513944583,
-255.550151000015));
#205879=CARTESIAN_POINT('Ctrl Pts',(-95.2883875465867,-90.2654970191385,
-248.816784000009));
#205880=CARTESIAN_POINT('Ctrl Pts',(-97.7324542791431,-76.7094800936942,
-242.083417000004));
#205881=CARTESIAN_POINT('Ctrl Pts',(-100.176521011699,-63.1534631682499,
-235.350049999999));
#205882=CARTESIAN_POINT('Ctrl Pts',(-102.596389063735,-49.7316642321664,
-228.683349999994));
#205883=CARTESIAN_POINT('Ctrl Pts',(-105.029169361015,-36.1729459547875,
-222.01665));
#205884=CARTESIAN_POINT('Ctrl Pts',(-107.482953290646,-22.4786190621241,
-215.34995));
#205885=CARTESIAN_POINT('Ctrl Pts',(-107.507491129942,-22.3416757931975,
-215.283283));
#205886=CARTESIAN_POINT('Ctrl Pts',(-107.532028969239,-22.2047325242709,
-215.216616));
#205887=CARTESIAN_POINT('Ctrl Pts',(-107.556566808535,-22.0677892553443,
-215.149949));
#205888=CARTESIAN_POINT('Ctrl Pts',(-28.673376513548,-286.071121685269,
-376.750757000082));
#205889=CARTESIAN_POINT('Ctrl Pts',(-39.8158585371298,-239.698911789471,
-349.817289000066));
#205890=CARTESIAN_POINT('Ctrl Pts',(-50.9583405607115,-193.326701893672,
-322.88382100005));
#205891=CARTESIAN_POINT('Ctrl Pts',(-62.1008225842933,-146.954491997874,
-295.950353000034));
#205892=CARTESIAN_POINT('Ctrl Pts',(-67.6720635960841,-123.768387049975,
-282.483619000027));
#205893=CARTESIAN_POINT('Ctrl Pts',(-73.243304607875,-100.582282102076,
-269.016885000018));
#205894=CARTESIAN_POINT('Ctrl Pts',(-78.8145456196659,-77.3961771541774,
-255.550151000011));
#205895=CARTESIAN_POINT('Ctrl Pts',(-81.6001661255613,-65.8031246802278,
-248.816784000007));
#205896=CARTESIAN_POINT('Ctrl Pts',(-84.3857866314568,-54.2100722062783,
-242.083417000003));
#205897=CARTESIAN_POINT('Ctrl Pts',(-87.1714071373522,-42.6170197323288,
-235.350049999999));
#205898=CARTESIAN_POINT('Ctrl Pts',(-89.9294472421992,-31.1387499561412,
-228.683349999995));
#205899=CARTESIAN_POINT('Ctrl Pts',(-92.6971547209677,-19.5588172835613,
-222.01665));
#205900=CARTESIAN_POINT('Ctrl Pts',(-95.4805372561441,-7.8781950045052,
-215.34995));
#205901=CARTESIAN_POINT('Ctrl Pts',(-95.508371081496,-7.76138878171465,
-215.283283));
#205902=CARTESIAN_POINT('Ctrl Pts',(-95.5362049068479,-7.64458255892409,
-215.216616));
#205903=CARTESIAN_POINT('Ctrl Pts',(-95.5640387321998,-7.52777633613354,
-215.149949));
#205904=CARTESIAN_POINT('Ctrl Pts',(-8.49563339908065,-224.312424767957,
-376.750757000054));
#205905=CARTESIAN_POINT('Ctrl Pts',(-21.0043305160186,-185.792072678138,
-349.817289000044));
#205906=CARTESIAN_POINT('Ctrl Pts',(-33.5130276329566,-147.271720588319,
-322.883821000033));
#205907=CARTESIAN_POINT('Ctrl Pts',(-46.0217247498946,-108.7513684985,-295.950353000022));
#205908=CARTESIAN_POINT('Ctrl Pts',(-52.2760733083635,-89.4911924535907,
-282.483619000017));
#205909=CARTESIAN_POINT('Ctrl Pts',(-58.5304218668325,-70.2310164086813,
-269.016885000012));
#205910=CARTESIAN_POINT('Ctrl Pts',(-64.7847704253015,-50.9708403637719,
-255.550151000007));
#205911=CARTESIAN_POINT('Ctrl Pts',(-67.911944704536,-41.3407523413171,
-248.816784000005));
#205912=CARTESIAN_POINT('Ctrl Pts',(-71.0391189837705,-31.7106643188625,
-242.083417000002));
#205913=CARTESIAN_POINT('Ctrl Pts',(-74.166293263005,-22.0805762964077,
-235.35005));
#205914=CARTESIAN_POINT('Ctrl Pts',(-77.2625054206629,-12.5458356801159,
-228.683349999997));
#205915=CARTESIAN_POINT('Ctrl Pts',(-80.3651400809202,-2.94468861233498,
-222.01665));
#205916=CARTESIAN_POINT('Ctrl Pts',(-83.4781212216425,6.72222905311371,
-215.34995));
#205917=CARTESIAN_POINT('Ctrl Pts',(-83.5092510330498,6.81889822976819,
-215.283283));
#205918=CARTESIAN_POINT('Ctrl Pts',(-83.5403808444571,6.91556740642268,
-215.216616));
#205919=CARTESIAN_POINT('Ctrl Pts',(-83.5715106558644,7.01223658307716,
-215.149949));
#205920=CARTESIAN_POINT('Ctrl Pts',(11.6821097153867,-162.553727850645,
-376.750757000025));
#205921=CARTESIAN_POINT('Ctrl Pts',(-2.1928024949075,-131.885233566805,
-349.81728900002));
#205922=CARTESIAN_POINT('Ctrl Pts',(-16.0677147052017,-101.216739282966,
-322.883821000016));
#205923=CARTESIAN_POINT('Ctrl Pts',(-29.9426269154959,-70.548244999126,
-295.95035300001));
#205924=CARTESIAN_POINT('Ctrl Pts',(-36.880083020643,-55.2139978572062,
-282.483619000008));
#205925=CARTESIAN_POINT('Ctrl Pts',(-43.81753912579,-39.8797507152863,-269.016885000005));
#205926=CARTESIAN_POINT('Ctrl Pts',(-50.7549952309371,-24.5455035733664,
-255.550151000003));
#205927=CARTESIAN_POINT('Ctrl Pts',(-54.2237232835107,-16.8783800024065,
-248.816784000002));
#205928=CARTESIAN_POINT('Ctrl Pts',(-57.6924513360842,-9.21125643144658,
-242.083417000001));
#205929=CARTESIAN_POINT('Ctrl Pts',(-61.1611793886578,-1.54413286048666,
-235.35005));
#205930=CARTESIAN_POINT('Ctrl Pts',(-64.5955635991267,6.04707859590932,
-228.683349999999));
#205931=CARTESIAN_POINT('Ctrl Pts',(-68.0331254408726,13.6694400588913,
-222.01665));
#205932=CARTESIAN_POINT('Ctrl Pts',(-71.4757051871408,21.3226531107326,
-215.34995));
#205933=CARTESIAN_POINT('Ctrl Pts',(-71.5101309846035,21.3991852412511,
-215.283283));
#205934=CARTESIAN_POINT('Ctrl Pts',(-71.5445567820663,21.4757173717695,
-215.216616));
#205935=CARTESIAN_POINT('Ctrl Pts',(-71.578982579529,21.5522495022879,-215.149949));
#205936=CARTESIAN_POINT('Ctrl Pts',(18.4080240868758,-141.967495544875,
-376.750757000016));
#205937=CARTESIAN_POINT('Ctrl Pts',(4.07770684546288,-113.916287196361,
-349.817289000013));
#205938=CARTESIAN_POINT('Ctrl Pts',(-10.25261039595,-85.865078847848,-322.88382100001));
#205939=CARTESIAN_POINT('Ctrl Pts',(-24.582927637363,-57.8138704993346,
-295.950353000006));
#205940=CARTESIAN_POINT('Ctrl Pts',(-31.7480862580694,-43.7882663250779,
-282.483619000005));
#205941=CARTESIAN_POINT('Ctrl Pts',(-38.9132448787759,-29.7626621508213,
-269.016885000003));
#205942=CARTESIAN_POINT('Ctrl Pts',(-46.0784034994824,-15.7370579765646,
-255.550151000002));
#205943=CARTESIAN_POINT('Ctrl Pts',(-49.6609828098356,-8.72425588943629,
-248.816784000002));
#205944=CARTESIAN_POINT('Ctrl Pts',(-53.2435621201888,-1.71145380230796,
-242.083417000001));
#205945=CARTESIAN_POINT('Ctrl Pts',(-56.826141430542,5.30134828482038,-235.35005));
#205946=CARTESIAN_POINT('Ctrl Pts',(-60.3732496586146,12.2447166879177,
-228.683349999999));
#205947=CARTESIAN_POINT('Ctrl Pts',(-63.9224538941901,19.2074829493001,
-222.01665));
#205948=CARTESIAN_POINT('Ctrl Pts',(-67.4748998423069,26.1894611299389,
-215.34995));
#205949=CARTESIAN_POINT('Ctrl Pts',(-67.5104243017881,26.2592809117453,
-215.283283));
#205950=CARTESIAN_POINT('Ctrl Pts',(-67.5459487612693,26.3291006935517,
-215.216616));
#205951=CARTESIAN_POINT('Ctrl Pts',(-67.5814732207505,26.3989204753581,
-215.149949));
#205952=CARTESIAN_POINT('Ctrl Pts',(25.1339384583649,-121.381263239104,
-376.750757000007));
#205953=CARTESIAN_POINT('Ctrl Pts',(10.3482161858333,-95.9473408259171,
-349.817289000005));
#205954=CARTESIAN_POINT('Ctrl Pts',(-4.4375060866984,-70.5134184127302,
-322.883821000004));
#205955=CARTESIAN_POINT('Ctrl Pts',(-19.22322835923,-45.0794959995432,-295.950353000003));
#205956=CARTESIAN_POINT('Ctrl Pts',(-26.6160894954959,-32.3625347929498,
-282.483619000002));
#205957=CARTESIAN_POINT('Ctrl Pts',(-34.0089506317617,-19.6455735863562,
-269.016885000001));
#205958=CARTESIAN_POINT('Ctrl Pts',(-41.4018117680275,-6.9286123797628,
-255.550151000001));
#205959=CARTESIAN_POINT('Ctrl Pts',(-45.0982423361605,-0.570131776466063,
-248.816784000001));
#205960=CARTESIAN_POINT('Ctrl Pts',(-48.7946729042934,5.78834882683067,
-242.083417));
#205961=CARTESIAN_POINT('Ctrl Pts',(-52.4911034724263,12.1468294301274,
-235.35005));
#205962=CARTESIAN_POINT('Ctrl Pts',(-56.1509357181025,18.4423547799261,
-228.68335));
#205963=CARTESIAN_POINT('Ctrl Pts',(-59.8117823475076,24.7455258397088,
-222.01665));
#205964=CARTESIAN_POINT('Ctrl Pts',(-63.4740944974731,31.0562691491453,
-215.34995));
#205965=CARTESIAN_POINT('Ctrl Pts',(-63.5107176189727,31.1193765822396,
-215.283283));
#205966=CARTESIAN_POINT('Ctrl Pts',(-63.5473407404724,31.1824840153339,
-215.216616));
#205967=CARTESIAN_POINT('Ctrl Pts',(-63.5839638619721,31.2455914484283,
-215.149949));
#205968=CARTESIAN_POINT('Ctrl Pts',(31.859852829854,-100.795030933333,-376.750756999998));
#205969=CARTESIAN_POINT('Ctrl Pts',(16.6187255262036,-77.9783944554729,
-349.817288999998));
#205970=CARTESIAN_POINT('Ctrl Pts',(1.37759822255324,-55.1617579776124,
-322.883820999999));
#205971=CARTESIAN_POINT('Ctrl Pts',(-13.8635290810972,-32.3451214997519,
-295.950352999999));
#205972=CARTESIAN_POINT('Ctrl Pts',(-21.4840927329223,-20.9368032608216,
-282.483618999999));
#205973=CARTESIAN_POINT('Ctrl Pts',(-29.1046563847475,-9.52848502189127,
-269.016885));
#205974=CARTESIAN_POINT('Ctrl Pts',(-36.7252200365728,1.87983321703902,
-255.550151));
#205975=CARTESIAN_POINT('Ctrl Pts',(-40.5355018624854,7.58399233650416,
-248.816784));
#205976=CARTESIAN_POINT('Ctrl Pts',(-44.345783688398,13.2881514559693,-242.083417));
#205977=CARTESIAN_POINT('Ctrl Pts',(-48.1560655143106,18.9923105754345,
-235.35005));
#205978=CARTESIAN_POINT('Ctrl Pts',(-51.9286217775904,24.6399928719346,
-228.68335));
#205979=CARTESIAN_POINT('Ctrl Pts',(-55.7011108008251,30.2835687301176,
-222.01665));
#205980=CARTESIAN_POINT('Ctrl Pts',(-59.4732891526392,35.9230771683515,
-215.34995));
#205981=CARTESIAN_POINT('Ctrl Pts',(-59.5110109361573,35.9794722527339,
-215.283283));
#205982=CARTESIAN_POINT('Ctrl Pts',(-59.5487327196755,36.0358673371162,
-215.216616));
#205983=CARTESIAN_POINT('Ctrl Pts',(-59.5864545031936,36.0922624214986,
-215.149949));
#205984=CARTESIAN_POINT('Ctrl Pts',(33.5413314227263,-95.6484728568909,
-376.750756999995));
#205985=CARTESIAN_POINT('Ctrl Pts',(18.1863528612963,-73.4861578628619,
-349.817288999997));
#205986=CARTESIAN_POINT('Ctrl Pts',(2.83137429986615,-51.3238428688329,
-322.883820999997));
#205987=CARTESIAN_POINT('Ctrl Pts',(-12.5236042615639,-29.161527874804,
-295.950352999998));
#205988=CARTESIAN_POINT('Ctrl Pts',(-20.201093542279,-18.0803703777895,
-282.483618999998));
#205989=CARTESIAN_POINT('Ctrl Pts',(-27.878582822994,-6.99921288077501,
-269.016884999999));
#205990=CARTESIAN_POINT('Ctrl Pts',(-35.556072103709,4.08194461623947,-255.550151));
#205991=CARTESIAN_POINT('Ctrl Pts',(-39.3948167440666,9.62252336474671,
-248.816784));
#205992=CARTESIAN_POINT('Ctrl Pts',(-43.2335613844241,15.163102113254,-242.083417));
#205993=CARTESIAN_POINT('Ctrl Pts',(-47.0723060247816,20.7036808617612,
-235.35005));
#205994=CARTESIAN_POINT('Ctrl Pts',(-50.8730432924624,26.1894023949367,
-228.683350000001));
#205995=CARTESIAN_POINT('Ctrl Pts',(-54.6734429141545,31.6680794527198,
-222.01665));
#205996=CARTESIAN_POINT('Ctrl Pts',(-58.4730878164307,37.1397791731531,
-215.34995));
#205997=CARTESIAN_POINT('Ctrl Pts',(-58.5110842654535,37.1944961703575,
-215.283283));
#205998=CARTESIAN_POINT('Ctrl Pts',(-58.5490807144762,37.2492131675618,
-215.216616));
#205999=CARTESIAN_POINT('Ctrl Pts',(-58.587077163499,37.3039301647661,-215.149949));
#206000=CARTESIAN_POINT('Ctrl Pts',(41.2301579830855,-81.5182387771612,
-376.750756999989));
#206001=CARTESIAN_POINT('Ctrl Pts',(24.8836555508694,-61.3775485896441,
-349.817288999991));
#206002=CARTESIAN_POINT('Ctrl Pts',(8.53715311865333,-41.2368584021269,
-322.883820999993));
#206003=CARTESIAN_POINT('Ctrl Pts',(-7.80934931356275,-21.0961682146096,
-295.950352999996));
#206004=CARTESIAN_POINT('Ctrl Pts',(-15.9826005296708,-11.025823120851,
-282.483618999996));
#206005=CARTESIAN_POINT('Ctrl Pts',(-24.1558517457789,-0.955478027092413,
-269.016884999998));
#206006=CARTESIAN_POINT('Ctrl Pts',(-32.3291029618869,9.1148670666662,-255.550150999998));
#206007=CARTESIAN_POINT('Ctrl Pts',(-36.4157285699409,14.1500396135455,
-248.816783999999));
#206008=CARTESIAN_POINT('Ctrl Pts',(-40.5023541779949,19.1852121604248,
-242.083416999999));
#206009=CARTESIAN_POINT('Ctrl Pts',(-44.588979786049,24.2203847073041,-235.35005));
#206010=CARTESIAN_POINT('Ctrl Pts',(-48.6351437544193,29.2057040606499,
-228.683350000001));
#206011=CARTESIAN_POINT('Ctrl Pts',(-52.6799616741893,34.1756765917424,
-222.01665));
#206012=CARTESIAN_POINT('Ctrl Pts',(-56.7225263698862,39.1304491224114,
-215.34995));
#206013=CARTESIAN_POINT('Ctrl Pts',(-56.7629520168432,39.1799968477181,
-215.283283));
#206014=CARTESIAN_POINT('Ctrl Pts',(-56.8033776638002,39.2295445730248,
-215.216616));
#206015=CARTESIAN_POINT('Ctrl Pts',(-56.8438033107571,39.2790922983315,
-215.149949));
#206016=CARTESIAN_POINT('Ctrl Pts',(61.5202391452974,-58.1759617860395,
-376.750756999982));
#206017=CARTESIAN_POINT('Ctrl Pts',(42.2054487986876,-41.4892341751692,
-349.817288999985));
#206018=CARTESIAN_POINT('Ctrl Pts',(22.8906584520777,-24.8025065642989,
-322.883820999989));
#206019=CARTESIAN_POINT('Ctrl Pts',(3.5758681054679,-8.11577895342853,-295.950352999993));
#206020=CARTESIAN_POINT('Ctrl Pts',(-6.08152706783702,0.227584852006628,
-282.483618999994));
#206021=CARTESIAN_POINT('Ctrl Pts',(-15.738922241142,8.57094865744179,-269.016884999996));
#206022=CARTESIAN_POINT('Ctrl Pts',(-25.3963174144469,16.9143124628769,
-255.550150999997));
#206023=CARTESIAN_POINT('Ctrl Pts',(-30.2250150010993,21.0859943655945,
-248.816783999999));
#206024=CARTESIAN_POINT('Ctrl Pts',(-35.0537125877518,25.2576762683121,
-242.083416999999));
#206025=CARTESIAN_POINT('Ctrl Pts',(-39.8824101744042,29.4293581710297,
-235.35005));
#206026=CARTESIAN_POINT('Ctrl Pts',(-44.6632988740601,33.5597362925323,
-228.683350000001));
#206027=CARTESIAN_POINT('Ctrl Pts',(-49.4410603210161,37.6624224459266,
-222.01665));
#206028=CARTESIAN_POINT('Ctrl Pts',(-54.214059251162,41.7376821955923,-215.34995));
#206029=CARTESIAN_POINT('Ctrl Pts',(-54.2617892404634,41.778434793089,-215.283283));
#206030=CARTESIAN_POINT('Ctrl Pts',(-54.3095192297649,41.8191873905857,
-215.216616));
#206031=CARTESIAN_POINT('Ctrl Pts',(-54.3572492190663,41.8599399880823,
-215.149949));
#206032=CARTESIAN_POINT('Ctrl Pts',(86.4308715045652,-38.5465561709931,
-376.75075699998));
#206033=CARTESIAN_POINT('Ctrl Pts',(63.394599877538,-24.7210691437011,-349.817288999984));
#206034=CARTESIAN_POINT('Ctrl Pts',(40.3583282505107,-10.8955821164091,
-322.883820999988));
#206035=CARTESIAN_POINT('Ctrl Pts',(17.3220566234834,2.92990491088294,-295.950352999991));
#206036=CARTESIAN_POINT('Ctrl Pts',(5.80392080996978,9.84264842452895,-282.483618999993));
#206037=CARTESIAN_POINT('Ctrl Pts',(-5.71421500354386,16.755391938175,-269.016884999996));
#206038=CARTESIAN_POINT('Ctrl Pts',(-17.2323508170575,23.668135451821,-255.550150999997));
#206039=CARTESIAN_POINT('Ctrl Pts',(-22.9914187238143,27.1245072086439,
-248.816783999998));
#206040=CARTESIAN_POINT('Ctrl Pts',(-28.7504866305711,30.580878965467,-242.083416999999));
#206041=CARTESIAN_POINT('Ctrl Pts',(-34.509554537328,34.03725072229,-235.35005));
#206042=CARTESIAN_POINT('Ctrl Pts',(-40.2116019697604,37.4594009765702,
-228.683350000001));
#206043=CARTESIAN_POINT('Ctrl Pts',(-45.9096065172025,40.8490096838924,
-222.01665));
#206044=CARTESIAN_POINT('Ctrl Pts',(-51.6016474095961,44.2063892516083,
-215.34995));
#206045=CARTESIAN_POINT('Ctrl Pts',(-51.65856781852,44.2399630472854,-215.283283));
#206046=CARTESIAN_POINT('Ctrl Pts',(-51.715488227444,44.2735368429626,-215.216616));
#206047=CARTESIAN_POINT('Ctrl Pts',(-51.7724086363679,44.3071106386397,
-215.149949));
#206048=CARTESIAN_POINT('Ctrl Pts',(101.966904434915,-30.8346247983327,
-376.750756999984));
#206049=CARTESIAN_POINT('Ctrl Pts',(76.6679969066201,-18.0147641121609,
-349.817288999987));
#206050=CARTESIAN_POINT('Ctrl Pts',(51.3690893783256,-5.19490342598898,
-322.88382099999));
#206051=CARTESIAN_POINT('Ctrl Pts',(26.070181850031,7.62495726018286,-295.950352999994));
#206052=CARTESIAN_POINT('Ctrl Pts',(13.4207280858838,14.0348876032688,-282.483618999995));
#206053=CARTESIAN_POINT('Ctrl Pts',(0.771274321736487,20.4448179463547,
-269.016884999996));
#206054=CARTESIAN_POINT('Ctrl Pts',(-11.8781794424108,26.8547482894406,
-255.550150999998));
#206055=CARTESIAN_POINT('Ctrl Pts',(-18.2029063244844,30.0597134609836,
-248.816783999999));
#206056=CARTESIAN_POINT('Ctrl Pts',(-24.5276332065581,33.2646786325266,
-242.083416999999));
#206057=CARTESIAN_POINT('Ctrl Pts',(-30.8523600886317,36.4696438040695,
-235.35005));
#206058=CARTESIAN_POINT('Ctrl Pts',(-37.1144659124669,39.6428766471814,
-228.683350000001));
#206059=CARTESIAN_POINT('Ctrl Pts',(-43.3732515923186,42.7902567304839,
-222.01665));
#206060=CARTESIAN_POINT('Ctrl Pts',(-49.6271914214616,45.9120323459617,
-215.34995));
#206061=CARTESIAN_POINT('Ctrl Pts',(-49.6897308197531,45.9432501021165,
-215.283283));
#206062=CARTESIAN_POINT('Ctrl Pts',(-49.7522702180445,45.9744678582713,
-215.216616));
#206063=CARTESIAN_POINT('Ctrl Pts',(-49.8148096163359,46.005685614426,-215.149949));
#206064=CARTESIAN_POINT('Ctrl Pts',(107.993804890233,-28.9044482397935,
-376.750756999988));
#206065=CARTESIAN_POINT('Ctrl Pts',(81.8862252383193,-16.2510537069498,
-349.81728899999));
#206066=CARTESIAN_POINT('Ctrl Pts',(55.7786455864053,-3.5976591741061,-322.883820999992));
#206067=CARTESIAN_POINT('Ctrl Pts',(29.6710659344913,9.05573535873763,-295.950352999994));
#206068=CARTESIAN_POINT('Ctrl Pts',(16.6172761085343,15.3824326251595,-282.483618999996));
#206069=CARTESIAN_POINT('Ctrl Pts',(3.5634862825773,21.7091298915814,-269.016884999997));
#206070=CARTESIAN_POINT('Ctrl Pts',(-9.49030354337971,28.0358271580032,
-255.550150999998));
#206071=CARTESIAN_POINT('Ctrl Pts',(-16.0171984563582,31.1991757912142,
-248.816783999999));
#206072=CARTESIAN_POINT('Ctrl Pts',(-22.5440933693367,34.3625244244251,
-242.083416999999));
#206073=CARTESIAN_POINT('Ctrl Pts',(-29.0709882823152,37.525873057636,-235.35005));
#206074=CARTESIAN_POINT('Ctrl Pts',(-35.5332604733831,40.6579014073498,
-228.683350000001));
#206075=CARTESIAN_POINT('Ctrl Pts',(-41.9930962102693,43.771133049519,-222.01665));
#206076=CARTESIAN_POINT('Ctrl Pts',(-48.4493862544499,46.8657485296993,
-215.34995));
#206077=CARTESIAN_POINT('Ctrl Pts',(-48.5139491548917,46.8966946845011,
-215.283283));
#206078=CARTESIAN_POINT('Ctrl Pts',(-48.5785120553335,46.9276408393029,
-215.216616));
#206079=CARTESIAN_POINT('Ctrl Pts',(-48.6430749557753,46.9585869941047,
-215.149949));
#206080=CARTESIAN_POINT('Ctrl Pts',(132.101406711508,-21.1837420056372,
-376.750756999997));
#206081=CARTESIAN_POINT('Ctrl Pts',(102.759138565116,-9.1962120861059,-349.817288999997));
#206082=CARTESIAN_POINT('Ctrl Pts',(73.4168704187245,2.79131783342537,-322.883820999998));
#206083=CARTESIAN_POINT('Ctrl Pts',(44.0746022723325,14.7788477529567,-295.950352999998));
#206084=CARTESIAN_POINT('Ctrl Pts',(29.4034681991366,20.7726127127223,-282.483618999999));
#206085=CARTESIAN_POINT('Ctrl Pts',(14.7323341259406,26.766377672488,-269.016884999999));
#206086=CARTESIAN_POINT('Ctrl Pts',(0.0612000527446133,32.7601426322536,
-255.550151));
#206087=CARTESIAN_POINT('Ctrl Pts',(-7.27436698385337,35.7570251121364,
-248.816784));
#206088=CARTESIAN_POINT('Ctrl Pts',(-14.6099340204513,38.7539075920192,
-242.083417));
#206089=CARTESIAN_POINT('Ctrl Pts',(-21.9455010570494,41.7507900719021,
-235.35005));
#206090=CARTESIAN_POINT('Ctrl Pts',(-29.2084387170473,44.7180004480236,
-228.68335));
#206091=CARTESIAN_POINT('Ctrl Pts',(-36.4724746820719,47.694638325659,-222.016650000001));
#206092=CARTESIAN_POINT('Ctrl Pts',(-43.7381655864028,50.6806132646498,
-215.34995));
#206093=CARTESIAN_POINT('Ctrl Pts',(-43.810822495446,50.7104730140397,-215.283283));
#206094=CARTESIAN_POINT('Ctrl Pts',(-43.8834794044894,50.7403327634296,
-215.216616));
#206095=CARTESIAN_POINT('Ctrl Pts',(-43.9561363135327,50.7701925128195,
-215.149949));
#206096=CARTESIAN_POINT('Ctrl Pts',(156.209008532784,-13.4630357714808,
-376.750757000006));
#206097=CARTESIAN_POINT('Ctrl Pts',(123.632051891913,-2.14137046526198,
-349.817289000005));
#206098=CARTESIAN_POINT('Ctrl Pts',(91.0550952510435,9.18029484095685,-322.883821000004));
#206099=CARTESIAN_POINT('Ctrl Pts',(58.4781386101737,20.5019601471757,-295.950353000003));
#206100=CARTESIAN_POINT('Ctrl Pts',(42.1896602897388,26.1627928002851,-282.483619000002));
#206101=CARTESIAN_POINT('Ctrl Pts',(25.9011819693039,31.8236254533946,-269.016885000001));
#206102=CARTESIAN_POINT('Ctrl Pts',(9.61270364886893,37.484458106504,-255.550151000001));
#206103=CARTESIAN_POINT('Ctrl Pts',(1.46846448865147,40.3148744330587,-248.816784000001));
#206104=CARTESIAN_POINT('Ctrl Pts',(-6.67577467156599,43.1452907596133,
-242.083417));
#206105=CARTESIAN_POINT('Ctrl Pts',(-14.8200138317834,45.9757070861681,
-235.35005));
#206106=CARTESIAN_POINT('Ctrl Pts',(-22.8836169607117,48.7780994886975,
-228.68335));
#206107=CARTESIAN_POINT('Ctrl Pts',(-30.9518531538746,51.6181436017991,
-222.016650000001));
#206108=CARTESIAN_POINT('Ctrl Pts',(-39.0269449183556,54.4954779996004,
-215.349950000001));
#206109=CARTESIAN_POINT('Ctrl Pts',(-39.1076958360005,54.5242513435783,
-215.283283000001));
#206110=CARTESIAN_POINT('Ctrl Pts',(-39.1884467536454,54.5530246875563,
-215.216616));
#206111=CARTESIAN_POINT('Ctrl Pts',(-39.2691976712902,54.5817980315343,
-215.149949000001));
#206112=CARTESIAN_POINT('Ctrl Pts',(180.316610354058,-5.74232953732446,
-376.750757000015));
#206113=CARTESIAN_POINT('Ctrl Pts',(144.50496521871,4.91347115558193,-349.817289000013));
#206114=CARTESIAN_POINT('Ctrl Pts',(108.693320083363,15.5692718484884,-322.88382100001));
#206115=CARTESIAN_POINT('Ctrl Pts',(72.8816749480149,26.2250725413947,-295.950353000006));
#206116=CARTESIAN_POINT('Ctrl Pts',(54.975852380341,31.5529728878479,-282.483619000005));
#206117=CARTESIAN_POINT('Ctrl Pts',(37.0700298126672,36.8808732343011,-269.016885000003));
#206118=CARTESIAN_POINT('Ctrl Pts',(19.1642072449932,42.2087735807543,-255.550151000002));
#206119=CARTESIAN_POINT('Ctrl Pts',(10.2112959611563,44.8727237539809,-248.816784000002));
#206120=CARTESIAN_POINT('Ctrl Pts',(1.25838467731937,47.5366739272075,-242.083417000001));
#206121=CARTESIAN_POINT('Ctrl Pts',(-7.69452660651757,50.2006241004341,
-235.35005));
#206122=CARTESIAN_POINT('Ctrl Pts',(-16.558795204376,52.8381985293713,-228.68335));
#206123=CARTESIAN_POINT('Ctrl Pts',(-25.4312316256772,55.5416488779391,
-222.016650000001));
#206124=CARTESIAN_POINT('Ctrl Pts',(-34.3157242503085,58.3103427345509,
-215.349950000001));
#206125=CARTESIAN_POINT('Ctrl Pts',(-34.4045691765549,58.3380296731169,
-215.283283000001));
#206126=CARTESIAN_POINT('Ctrl Pts',(-34.4934141028013,58.365716611683,-215.216616));
#206127=CARTESIAN_POINT('Ctrl Pts',(-34.5822590290476,58.3934035502491,
-215.149949000001));
#206128=CARTESIAN_POINT('Ctrl Pts',(252.639415817883,17.4197891651448,-376.750757000044));
#206129=CARTESIAN_POINT('Ctrl Pts',(207.123705199102,26.0779960181138,-349.817289000036));
#206130=CARTESIAN_POINT('Ctrl Pts',(161.60799458032,34.7362028710828,-322.883821000027));
#206131=CARTESIAN_POINT('Ctrl Pts',(116.092283961538,43.3944097240518,-295.950353000018));
#206132=CARTESIAN_POINT('Ctrl Pts',(93.3344286521477,47.7235131505364,-282.483619000015));
#206133=CARTESIAN_POINT('Ctrl Pts',(70.576573342757,52.0526165770209,-269.01688500001));
#206134=CARTESIAN_POINT('Ctrl Pts',(47.8187180333662,56.3817200035054,-255.550151000006));
#206135=CARTESIAN_POINT('Ctrl Pts',(36.4397903786708,58.5462717167477,-248.816784000004));
#206136=CARTESIAN_POINT('Ctrl Pts',(25.0608627239755,60.7108234299899,-242.083417000002));
#206137=CARTESIAN_POINT('Ctrl Pts',(13.6819350692801,62.8753751432322,-235.35005));
#206138=CARTESIAN_POINT('Ctrl Pts',(2.41567006463117,65.0184956513928,-228.683349999998));
#206139=CARTESIAN_POINT('Ctrl Pts',(-8.86936704108513,67.3121647063593,
-222.016650000002));
#206140=CARTESIAN_POINT('Ctrl Pts',(-20.1820622461672,69.7549369394024,
-215.349950000001));
#206141=CARTESIAN_POINT('Ctrl Pts',(-20.2951891982182,69.7793646617328,
-215.283283000001));
#206142=CARTESIAN_POINT('Ctrl Pts',(-20.4083161502691,69.8037923840631,
-215.216616));
#206143=CARTESIAN_POINT('Ctrl Pts',(-20.5214431023201,69.8282201063935,
-215.149949000001));
#206144=CARTESIAN_POINT('Ctrl Pts',(324.962221281708,40.581907867614,-376.750757000072));
#206145=CARTESIAN_POINT('Ctrl Pts',(269.742445179492,47.2425208806457,-349.817289000059));
#206146=CARTESIAN_POINT('Ctrl Pts',(214.522669077277,53.9031338936774,-322.883821000045));
#206147=CARTESIAN_POINT('Ctrl Pts',(159.302892975062,60.563746906709,-295.950353000031));
#206148=CARTESIAN_POINT('Ctrl Pts',(131.693004923954,63.8940534132249,-282.483619000024));
#206149=CARTESIAN_POINT('Ctrl Pts',(104.083116872847,67.2243599197407,-269.016885000017));
#206150=CARTESIAN_POINT('Ctrl Pts',(76.4732288217392,70.5546664262565,-255.55015100001));
#206151=CARTESIAN_POINT('Ctrl Pts',(62.6682847961853,72.2198196795144,-248.816784000007));
#206152=CARTESIAN_POINT('Ctrl Pts',(48.8633407706315,73.8849729327724,-242.083417000003));
#206153=CARTESIAN_POINT('Ctrl Pts',(35.0583967450777,75.5501261860303,-235.35005));
#206154=CARTESIAN_POINT('Ctrl Pts',(21.3901353336382,77.1987927734144,-228.683349999997));
#206155=CARTESIAN_POINT('Ctrl Pts',(7.69249754350693,79.0826805347794,-222.016650000002));
#206156=CARTESIAN_POINT('Ctrl Pts',(-6.0484002420259,81.199531144254,-215.349950000001));
#206157=CARTESIAN_POINT('Ctrl Pts',(-6.18580921988141,81.2206996503486,
-215.283283000001));
#206158=CARTESIAN_POINT('Ctrl Pts',(-6.32321819773692,81.2418681564432,
-215.216616000001));
#206159=CARTESIAN_POINT('Ctrl Pts',(-6.46062717559243,81.2630366625378,
-215.149949000001));
#206160=CARTESIAN_POINT('Ctrl Pts',(397.285026745533,63.7440265700833,-376.750757000099));
#206161=CARTESIAN_POINT('Ctrl Pts',(332.361185159884,68.4070457431775,-349.81728900008));
#206162=CARTESIAN_POINT('Ctrl Pts',(267.437343574235,73.0700649162719,-322.883821000062));
#206163=CARTESIAN_POINT('Ctrl Pts',(202.513501988586,77.7330840893662,-295.950353000043));
#206164=CARTESIAN_POINT('Ctrl Pts',(170.051581195761,80.0645936759133,-282.483619000033));
#206165=CARTESIAN_POINT('Ctrl Pts',(137.589660402937,82.3961032624605,-269.016885000024));
#206166=CARTESIAN_POINT('Ctrl Pts',(105.127739610112,84.7276128490076,-255.550151000015));
#206167=CARTESIAN_POINT('Ctrl Pts',(88.8967792136999,85.8933676422812,-248.81678400001));
#206168=CARTESIAN_POINT('Ctrl Pts',(72.6658188172876,87.0591224355548,-242.083417000005));
#206169=CARTESIAN_POINT('Ctrl Pts',(56.4348584208753,88.2248772288284,-235.35005));
#206170=CARTESIAN_POINT('Ctrl Pts',(40.3646006026454,89.3790898954359,-228.683349999995));
#206171=CARTESIAN_POINT('Ctrl Pts',(24.254362128099,90.8531963631996,-222.016650000002));
#206172=CARTESIAN_POINT('Ctrl Pts',(8.08526176211542,92.6441253491055,-215.349950000002));
#206173=CARTESIAN_POINT('Ctrl Pts',(7.92357075845534,92.6620346389644,-215.283283000002));
#206174=CARTESIAN_POINT('Ctrl Pts',(7.76187975479526,92.6799439288233,-215.216616000002));
#206175=CARTESIAN_POINT('Ctrl Pts',(7.60018875113518,92.6978532186822,-215.149949000001));
#206176=CARTESIAN_POINT('Ctrl Pts',(614.253443137008,133.230382677491,-376.750757000185));
#206177=CARTESIAN_POINT('Ctrl Pts',(520.217405101058,131.900620330773,-349.81728900015));
#206178=CARTESIAN_POINT('Ctrl Pts',(426.181367065107,130.570857984055,-322.883821000115));
#206179=CARTESIAN_POINT('Ctrl Pts',(332.145329029157,129.241095637338,-295.950353000079));
#206180=CARTESIAN_POINT('Ctrl Pts',(285.127310011182,128.576214463979,-282.483619000062));
#206181=CARTESIAN_POINT('Ctrl Pts',(238.109290993206,127.91133329062,-269.016885000044));
#206182=CARTESIAN_POINT('Ctrl Pts',(191.091271975231,127.246452117261,-255.550151000026));
#206183=CARTESIAN_POINT('Ctrl Pts',(167.582262466243,126.914011530581,-248.816784000018));
#206184=CARTESIAN_POINT('Ctrl Pts',(144.073252957256,126.581570943902,-242.083417000009));
#206185=CARTESIAN_POINT('Ctrl Pts',(120.564243448268,126.249130357223,-235.35005));
#206186=CARTESIAN_POINT('Ctrl Pts',(97.2879964096667,125.9199812615,-228.683349999992));
#206187=CARTESIAN_POINT('Ctrl Pts',(73.9399558818752,126.16474384846,-222.016650000005));
#206188=CARTESIAN_POINT('Ctrl Pts',(50.4862477745394,126.97790796366,-215.349950000003));
#206189=CARTESIAN_POINT('Ctrl Pts',(50.2517106934656,126.986039604812,-215.283283000003));
#206190=CARTESIAN_POINT('Ctrl Pts',(50.0171736123918,126.994171245964,-215.216616000002));
#206191=CARTESIAN_POINT('Ctrl Pts',(49.782636531318,127.002302887115,-215.149949000002));
#206192=CARTESIAN_POINT('Ctrl Pts',(831.221859528483,202.716738784898,-376.75075700027));
#206193=CARTESIAN_POINT('Ctrl Pts',(708.073625042231,195.394194918369,-349.817289000218));
#206194=CARTESIAN_POINT('Ctrl Pts',(584.92539055598,188.071651051839,-322.883821000167));
#206195=CARTESIAN_POINT('Ctrl Pts',(461.777156069728,180.749107185309,-295.950353000116));
#206196=CARTESIAN_POINT('Ctrl Pts',(400.203038826602,177.087835252044,-282.48361900009));
#206197=CARTESIAN_POINT('Ctrl Pts',(338.628921583476,173.426563318779,-269.016885000064));
#206198=CARTESIAN_POINT('Ctrl Pts',(277.05480434035,169.765291385514,-255.550151000039));
#206199=CARTESIAN_POINT('Ctrl Pts',(246.267745718787,167.934655418882,-248.816784000026));
#206200=CARTESIAN_POINT('Ctrl Pts',(215.480687097224,166.10401945225,-242.083417000013));
#206201=CARTESIAN_POINT('Ctrl Pts',(184.693628475661,164.273383485617,-235.35005));
#206202=CARTESIAN_POINT('Ctrl Pts',(154.211392216688,162.460872627565,-228.683349999988));
#206203=CARTESIAN_POINT('Ctrl Pts',(123.625549635651,161.47629133372,-222.016650000007));
#206204=CARTESIAN_POINT('Ctrl Pts',(92.8872337869633,161.311690578215,-215.349950000004));
#206205=CARTESIAN_POINT('Ctrl Pts',(92.5798506284758,161.31004457066,-215.283283000004));
#206206=CARTESIAN_POINT('Ctrl Pts',(92.2724674699883,161.308398563104,-215.216616000004));
#206207=CARTESIAN_POINT('Ctrl Pts',(91.9650843115009,161.306752555549,-215.149949000004));
#206208=CARTESIAN_POINT('Ctrl Pts',(1048.19027591996,272.203094892306,-376.750757000354));
#206209=CARTESIAN_POINT('Ctrl Pts',(895.929844983404,258.887769505964,-349.817289000287));
#206210=CARTESIAN_POINT('Ctrl Pts',(743.669414046851,245.572444119622,-322.883821000219));
#206211=CARTESIAN_POINT('Ctrl Pts',(591.408983110298,232.257118733281,-295.950353000152));
#206212=CARTESIAN_POINT('Ctrl Pts',(515.278767642022,225.59945604011,-282.483619000118));
#206213=CARTESIAN_POINT('Ctrl Pts',(439.148552173745,218.941793346939,-269.016885000084));
#206214=CARTESIAN_POINT('Ctrl Pts',(363.018336705469,212.284130653768,-255.550151000051));
#206215=CARTESIAN_POINT('Ctrl Pts',(324.953228971331,208.955299307182,-248.816784000034));
#206216=CARTESIAN_POINT('Ctrl Pts',(286.888121237192,205.626467960597,-242.083417000017));
#206217=CARTESIAN_POINT('Ctrl Pts',(248.823013503054,202.297636614011,-235.35005));
#206218=CARTESIAN_POINT('Ctrl Pts',(211.134788023709,199.001763993629,-228.683349999984));
#206219=CARTESIAN_POINT('Ctrl Pts',(173.311143389428,196.787838818981,-222.016650000008));
#206220=CARTESIAN_POINT('Ctrl Pts',(135.288219799387,195.64547319277,-215.349950000004));
#206221=CARTESIAN_POINT('Ctrl Pts',(134.907990563486,195.634049536507,-215.283283000005));
#206222=CARTESIAN_POINT('Ctrl Pts',(134.527761327585,195.622625880244,-215.216616000005));
#206223=CARTESIAN_POINT('Ctrl Pts',(134.147532091684,195.611202223982,-215.149949000005));
#206224=CARTESIAN_POINT('Ctrl Pts',(1699.09552509438,480.662163214529,-376.75075700061));
#206225=CARTESIAN_POINT('Ctrl Pts',(1459.49850480692,449.368493268751,-349.817289000493));
#206226=CARTESIAN_POINT('Ctrl Pts',(1219.90148451947,418.074823322972,-322.883821000378));
#206227=CARTESIAN_POINT('Ctrl Pts',(980.30446423201,386.781153377194,-295.950353000261));
#206228=CARTESIAN_POINT('Ctrl Pts',(860.505954088282,371.134318404306,-282.483619000203));
#206229=CARTESIAN_POINT('Ctrl Pts',(740.707443944553,355.487483431416,-269.016885000145));
#206230=CARTESIAN_POINT('Ctrl Pts',(620.908933800825,339.840648458528,-255.550151000087));
#206231=CARTESIAN_POINT('Ctrl Pts',(561.009678728961,332.017230972083,-248.816784000058));
#206232=CARTESIAN_POINT('Ctrl Pts',(501.110423657097,324.193813485639,-242.083417000029));
#206233=CARTESIAN_POINT('Ctrl Pts',(441.211168585233,316.370395999194,-235.35005));
#206234=CARTESIAN_POINT('Ctrl Pts',(381.904975444773,308.624438091823,-228.683349999972));
#206235=CARTESIAN_POINT('Ctrl Pts',(322.367924650756,302.722481274762,-222.016650000015));
#206236=CARTESIAN_POINT('Ctrl Pts',(262.491177836659,298.646821036434,-215.349950000008));
#206237=CARTESIAN_POINT('Ctrl Pts',(261.892410368517,298.60606443405,-215.283283000008));
#206238=CARTESIAN_POINT('Ctrl Pts',(261.293642900374,298.565307831665,-215.216616000008));
#206239=CARTESIAN_POINT('Ctrl Pts',(260.694875432232,298.524551229281,-215.149949000007));
#206240=CARTESIAN_POINT('Ctrl Pts',(2350.0007742688,689.121231536752,-376.750757000865));
#206241=CARTESIAN_POINT('Ctrl Pts',(2023.06716463044,639.849217031537,-349.8172890007));
#206242=CARTESIAN_POINT('Ctrl Pts',(1696.13355499208,590.577202526323,-322.883821000536));
#206243=CARTESIAN_POINT('Ctrl Pts',(1369.19994535372,541.305188021109,-295.95035300037));
#206244=CARTESIAN_POINT('Ctrl Pts',(1205.73314053454,516.669180768502,-282.483619000288));
#206245=CARTESIAN_POINT('Ctrl Pts',(1042.26633571536,492.033173515894,-269.016885000205));
#206246=CARTESIAN_POINT('Ctrl Pts',(878.799530896182,467.397166263287,-255.550151000123));
#206247=CARTESIAN_POINT('Ctrl Pts',(797.066128486591,455.079162636984,-248.816784000082));
#206248=CARTESIAN_POINT('Ctrl Pts',(715.332726077001,442.76115901068,-242.083417000041));
#206249=CARTESIAN_POINT('Ctrl Pts',(633.599323667412,430.443155384376,-235.35005));
#206250=CARTESIAN_POINT('Ctrl Pts',(552.675162865837,418.247112190016,-228.68334999996));
#206251=CARTESIAN_POINT('Ctrl Pts',(471.424705912085,408.657123730544,-222.016650000021));
#206252=CARTESIAN_POINT('Ctrl Pts',(389.694135873931,401.648168880098,-215.34995000001));
#206253=CARTESIAN_POINT('Ctrl Pts',(388.876830173548,401.578079331591,-215.28328300001));
#206254=CARTESIAN_POINT('Ctrl Pts',(388.059524473164,401.507989783086,-215.216616000011));
#206255=CARTESIAN_POINT('Ctrl Pts',(387.242218772781,401.43790023458,-215.149949000011));
#206256=CARTESIAN_POINT('Ctrl Pts',(3000.90602344323,897.580299858975,-376.75075700112));
#206257=CARTESIAN_POINT('Ctrl Pts',(2586.63582445396,830.329940794324,-349.817289000906));
#206258=CARTESIAN_POINT('Ctrl Pts',(2172.36562546469,763.079581729674,-322.883821000693));
#206259=CARTESIAN_POINT('Ctrl Pts',(1758.09542647544,695.829222665023,-295.95035300048));
#206260=CARTESIAN_POINT('Ctrl Pts',(1550.9603269808,662.204043132698,-282.483619000373));
#206261=CARTESIAN_POINT('Ctrl Pts',(1343.82522748617,628.578863600373,-269.016885000266));
#206262=CARTESIAN_POINT('Ctrl Pts',(1136.69012799154,594.953684068047,-255.55015100016));
#206263=CARTESIAN_POINT('Ctrl Pts',(1033.12257824422,578.141094301885,-248.816784000106));
#206264=CARTESIAN_POINT('Ctrl Pts',(929.555028496906,561.328504535722,-242.083417000053));
#206265=CARTESIAN_POINT('Ctrl Pts',(825.98747874959,544.515914769559,-235.35005));
#206266=CARTESIAN_POINT('Ctrl Pts',(723.445350286901,527.86978628821,-228.683349999948));
#206267=CARTESIAN_POINT('Ctrl Pts',(620.481487173413,514.591766186325,-222.016650000027));
#206268=CARTESIAN_POINT('Ctrl Pts',(516.897093911203,504.649516723762,-215.349950000014));
#206269=CARTESIAN_POINT('Ctrl Pts',(515.861249978578,504.550094229134,-215.283283000013));
#206270=CARTESIAN_POINT('Ctrl Pts',(514.825406045954,504.450671734507,-215.216616000014));
#206271=CARTESIAN_POINT('Ctrl Pts',(513.789562113329,504.351249239879,-215.149949000014));
#206272=CARTESIAN_POINT('Ctrl Pts',(4953.62177096649,1522.95750482565,-376.750757001886));
#206273=CARTESIAN_POINT('Ctrl Pts',(4277.34180392452,1401.77211208268,-349.817289001526));
#206274=CARTESIAN_POINT('Ctrl Pts',(3601.06183688254,1280.58671933972,-322.883821001167));
#206275=CARTESIAN_POINT('Ctrl Pts',(2924.78186984057,1159.40132659677,-295.950353000808));
#206276=CARTESIAN_POINT('Ctrl Pts',(2586.64188631958,1098.80863022529,-282.483619000628));
#206277=CARTESIAN_POINT('Ctrl Pts',(2248.50190279859,1038.21593385381,-269.016885000448));
#206278=CARTESIAN_POINT('Ctrl Pts',(1910.36191927761,977.623237482327,-255.550151000268));
#206279=CARTESIAN_POINT('Ctrl Pts',(1741.29192751712,947.326889296587,-248.816784000179));
#206280=CARTESIAN_POINT('Ctrl Pts',(1572.22193575662,917.030541110847,-242.08341700009));
#206281=CARTESIAN_POINT('Ctrl Pts',(1403.15194399613,886.734192925108,-235.35005));
#206282=CARTESIAN_POINT('Ctrl Pts',(1235.75591255009,856.737808582791,-228.683349999911));
#206283=CARTESIAN_POINT('Ctrl Pts',(1067.6518309574,832.395693553669,-222.016650000045));
#206284=CARTESIAN_POINT('Ctrl Pts',(898.505968023019,813.653560254753,-215.349950000023));
#206285=CARTESIAN_POINT('Ctrl Pts',(896.814509393671,813.466138921761,-215.283283000022));
#206286=CARTESIAN_POINT('Ctrl Pts',(895.123050764323,813.278717588769,-215.216616000022));
#206287=CARTESIAN_POINT('Ctrl Pts',(893.431592134975,813.091296255777,-215.149949000023));
#206288=CARTESIAN_POINT('Ctrl Pts',(6906.33751848976,2148.33470979231,-376.750757002651));
#206289=CARTESIAN_POINT('Ctrl Pts',(5968.04778339507,1973.21428337105,-349.817289002145));
#206290=CARTESIAN_POINT('Ctrl Pts',(5029.75804830038,1798.09385694977,-322.883821001641));
#206291=CARTESIAN_POINT('Ctrl Pts',(4091.4683132057,1622.97343052851,-295.950353001135));
#206292=CARTESIAN_POINT('Ctrl Pts',(3622.32344565836,1535.41321731788,-282.483619000883));
#206293=CARTESIAN_POINT('Ctrl Pts',(3153.17857811102,1447.85300410724,-269.01688500063));
#206294=CARTESIAN_POINT('Ctrl Pts',(2684.03371056368,1360.29279089661,-255.550151000377));
#206295=CARTESIAN_POINT('Ctrl Pts',(2449.46127679,1316.51268429129,-248.816784000251));
#206296=CARTESIAN_POINT('Ctrl Pts',(2214.88884301634,1272.73257768597,-242.083417000126));
#206297=CARTESIAN_POINT('Ctrl Pts',(1980.31640924266,1228.95247108066,-235.35005));
#206298=CARTESIAN_POINT('Ctrl Pts',(1748.06647481329,1185.60583087737,-228.683349999876));
#206299=CARTESIAN_POINT('Ctrl Pts',(1514.82217474138,1150.19962092101,-222.016650000063));
#206300=CARTESIAN_POINT('Ctrl Pts',(1280.11484213483,1122.65760378574,-215.349950000032));
#206301=CARTESIAN_POINT('Ctrl Pts',(1277.76776880876,1122.38218361439,-215.283283000032));
#206302=CARTESIAN_POINT('Ctrl Pts',(1275.42069548269,1122.10676344303,-215.216616000032));
#206303=CARTESIAN_POINT('Ctrl Pts',(1273.07362215662,1121.83134327167,-215.149949000032));
#206304=CARTESIAN_POINT('Ctrl Pts',(8859.05326601302,2773.71191475898,-376.750757003417));
#206305=CARTESIAN_POINT('Ctrl Pts',(7658.75376286563,2544.6564546594,-349.817289002765));
#206306=CARTESIAN_POINT('Ctrl Pts',(6458.45425971823,2315.60099455983,-322.883821002114));
#206307=CARTESIAN_POINT('Ctrl Pts',(5258.15475657084,2086.54553446025,-295.950353001463));
#206308=CARTESIAN_POINT('Ctrl Pts',(4658.00500499714,1972.01780441047,-282.483619001138));
#206309=CARTESIAN_POINT('Ctrl Pts',(4057.85525342344,1857.49007436067,-269.016885000812));
#206310=CARTESIAN_POINT('Ctrl Pts',(3457.70550184975,1742.96234431089,-255.550151000486));
#206311=CARTESIAN_POINT('Ctrl Pts',(3157.6306260629,1685.69847928599,-248.816784000324));
#206312=CARTESIAN_POINT('Ctrl Pts',(2857.55575027604,1628.4346142611,-242.083417000162));
#206313=CARTESIAN_POINT('Ctrl Pts',(2557.4808744892,1571.17074923621,-235.35005));
#206314=CARTESIAN_POINT('Ctrl Pts',(2260.37703707648,1514.47385317195,-228.683349999839));
#206315=CARTESIAN_POINT('Ctrl Pts',(1961.99251852537,1468.00354828836,-222.01665000008));
#206316=CARTESIAN_POINT('Ctrl Pts',(1661.72371624665,1431.66164731674,-215.349950000041));
#206317=CARTESIAN_POINT('Ctrl Pts',(1658.72102822386,1431.29822830702,-215.28328300004));
#206318=CARTESIAN_POINT('Ctrl Pts',(1655.71834020106,1430.93480929729,-215.216616000041));
#206319=CARTESIAN_POINT('Ctrl Pts',(1652.71565217826,1430.57139028757,-215.149949000041));
#206320=CARTESIAN_POINT('Ctrl Pts',(14717.2005085828,4649.84352965899,-376.750757005713));
#206321=CARTESIAN_POINT('Ctrl Pts',(12730.8717012773,4258.98296852449,-349.817289004623));
#206322=CARTESIAN_POINT('Ctrl Pts',(10744.5428939718,3868.12240738999,-322.883821003535));
#206323=CARTESIAN_POINT('Ctrl Pts',(8758.21408666624,3477.26184625548,-295.950353002446));
#206324=CARTESIAN_POINT('Ctrl Pts',(7765.04968301347,3281.83156568823,-282.483619001902));
#206325=CARTESIAN_POINT('Ctrl Pts',(6771.88527936071,3086.40128512098,-269.016885001358));
#206326=CARTESIAN_POINT('Ctrl Pts',(5778.72087570795,2890.97100455373,-255.550151000813));
#206327=CARTESIAN_POINT('Ctrl Pts',(5282.13867388157,2793.2558642701,-248.816784000541));
#206328=CARTESIAN_POINT('Ctrl Pts',(4785.55647205519,2695.54072398648,-242.083417000271));
#206329=CARTESIAN_POINT('Ctrl Pts',(4288.9742702288,2597.82558370285,-235.35005));
#206330=CARTESIAN_POINT('Ctrl Pts',(3797.30872386605,2501.0779200557,-228.683349999731));
#206331=CARTESIAN_POINT('Ctrl Pts',(3303.50354987733,2421.41533039039,-222.016650000135));
#206332=CARTESIAN_POINT('Ctrl Pts',(2806.55033858209,2358.67377790971,-215.349950000068));
#206333=CARTESIAN_POINT('Ctrl Pts',(2801.58080646913,2358.0463623849,-215.283283000067));
#206334=CARTESIAN_POINT('Ctrl Pts',(2796.61127435617,2357.41894686008,-215.216616000068));
#206335=CARTESIAN_POINT('Ctrl Pts',(2791.64174224321,2356.79153133527,-215.149949000068));
#206336=CARTESIAN_POINT('Ctrl Pts',(20575.3477511526,6525.97514455899,-376.750757008008));
#206337=CARTESIAN_POINT('Ctrl Pts',(17802.9896396889,5973.30948238956,-349.817289006482));
#206338=CARTESIAN_POINT('Ctrl Pts',(15030.6315282253,5420.64382022014,-322.883821004956));
#206339=CARTESIAN_POINT('Ctrl Pts',(12258.2734167616,4867.97815805071,-295.950353003429));
#206340=CARTESIAN_POINT('Ctrl Pts',(10872.0943610298,4591.645326966,-282.483619002666));
#206341=CARTESIAN_POINT('Ctrl Pts',(9485.91530529798,4315.31249588128,-269.016885001903));
#206342=CARTESIAN_POINT('Ctrl Pts',(8099.73624956616,4038.97966479657,-255.55015100114));
#206343=CARTESIAN_POINT('Ctrl Pts',(7406.64672170025,3900.81324925421,-248.816784000758));
#206344=CARTESIAN_POINT('Ctrl Pts',(6713.55719383433,3762.64683371185,-242.083417000379));
#206345=CARTESIAN_POINT('Ctrl Pts',(6020.46766596842,3624.4804181695,-235.35005));
#206346=CARTESIAN_POINT('Ctrl Pts',(5334.24041065563,3487.68198693944,-228.683349999624));
#206347=CARTESIAN_POINT('Ctrl Pts',(4645.01458122929,3374.82711249242,-222.016650000188));
#206348=CARTESIAN_POINT('Ctrl Pts',(3951.37696091755,3285.68590850268,-215.349950000095));
#206349=CARTESIAN_POINT('Ctrl Pts',(3944.44058471441,3284.79449646278,-215.283283000095));
#206350=CARTESIAN_POINT('Ctrl Pts',(3937.50420851128,3283.90308442287,-215.216616000095));
#206351=CARTESIAN_POINT('Ctrl Pts',(3930.56783230814,3283.01167238296,-215.149949000095));
#206352=CARTESIAN_POINT('Ctrl Pts',(26433.4949937224,8402.106759459,-376.750757010304));
#206353=CARTESIAN_POINT('Ctrl Pts',(22875.1075781007,7687.63599625465,-349.81728900834));
#206354=CARTESIAN_POINT('Ctrl Pts',(19316.7201624788,6973.16523305029,-322.883821006377));
#206355=CARTESIAN_POINT('Ctrl Pts',(15758.332746857,6258.69446984594,-295.950353004413));
#206356=CARTESIAN_POINT('Ctrl Pts',(13979.1390390461,5901.45908824376,-282.48361900343));
#206357=CARTESIAN_POINT('Ctrl Pts',(12199.9453312353,5544.22370664158,-269.016885002448));
#206358=CARTESIAN_POINT('Ctrl Pts',(10420.7516234244,5186.98832503941,-255.550151001467));
#206359=CARTESIAN_POINT('Ctrl Pts',(9531.15476951892,5008.37063423832,-248.816784000976));
#206360=CARTESIAN_POINT('Ctrl Pts',(8641.55791561347,4829.75294343723,-242.083417000487));
#206361=CARTESIAN_POINT('Ctrl Pts',(7751.96106170802,4651.13525263614,-235.35005));
#206362=CARTESIAN_POINT('Ctrl Pts',(6871.1720974452,4474.28605382318,-228.683349999516));
#206363=CARTESIAN_POINT('Ctrl Pts',(5986.52561258124,4328.23889459445,-222.016650000243));
#206364=CARTESIAN_POINT('Ctrl Pts',(5096.20358325299,4212.69803909567,-215.349950000122));
#206365=CARTESIAN_POINT('Ctrl Pts',(5087.30036295968,4211.54263054066,-215.283283000121));
#206366=CARTESIAN_POINT('Ctrl Pts',(5078.39714266638,4210.38722198566,-215.216616000122));
#206367=CARTESIAN_POINT('Ctrl Pts',(5069.49392237307,4209.23181343066,-215.149949000122));
#206368=CARTESIAN_POINT('Origin',(0.,-12.9675000200281,-218.35005));
#206369=CARTESIAN_POINT('Ctrl Pts',(10765.646428189,-1979.29526939781,-376.750757000846));
#206370=CARTESIAN_POINT('Ctrl Pts',(9257.10677574949,-1902.78686830728,
-349.817289000686));
#206371=CARTESIAN_POINT('Ctrl Pts',(7748.56712330994,-1826.27846721676,
-322.883821000524));
#206372=CARTESIAN_POINT('Ctrl Pts',(6240.0274708704,-1749.77006612623,-295.950353000363));
#206373=CARTESIAN_POINT('Ctrl Pts',(5485.75764465062,-1711.51586558096,
-282.483619000282));
#206374=CARTESIAN_POINT('Ctrl Pts',(4731.48781843085,-1673.2616650357,-269.016885000202));
#206375=CARTESIAN_POINT('Ctrl Pts',(3977.21799221108,-1635.00746449044,
-255.550151000121));
#206376=CARTESIAN_POINT('Ctrl Pts',(3600.08307910119,-1615.8803642178,-248.816784000081));
#206377=CARTESIAN_POINT('Ctrl Pts',(3222.9481659913,-1596.75326394517,-242.083417000041));
#206378=CARTESIAN_POINT('Ctrl Pts',(2845.81325288141,-1577.62616367254,
-235.35005));
#206379=CARTESIAN_POINT('Ctrl Pts',(2472.41234881222,-1558.68844063033,
-228.68334999996));
#206380=CARTESIAN_POINT('Ctrl Pts',(2099.07452015968,-1540.45097924114,
-222.01665));
#206381=CARTESIAN_POINT('Ctrl Pts',(1725.79722689738,-1522.91379824522,
-215.34994999996));
#206382=CARTESIAN_POINT('Ctrl Pts',(1722.06445396475,-1522.73842643524,
-215.28328299996));
#206383=CARTESIAN_POINT('Ctrl Pts',(1718.33168103213,-1522.56305462527,
-215.21661599996));
#206384=CARTESIAN_POINT('Ctrl Pts',(1714.5989080995,-1522.3876828153,-215.14994899996));
#206385=CARTESIAN_POINT('Ctrl Pts',(8392.35568812379,-1534.61913504983,
-376.750757000658));
#206386=CARTESIAN_POINT('Ctrl Pts',(7213.78531733318,-1478.38877237011,
-349.817289000532));
#206387=CARTESIAN_POINT('Ctrl Pts',(6035.21494654257,-1422.15840969038,
-322.883821000408));
#206388=CARTESIAN_POINT('Ctrl Pts',(4856.64457575196,-1365.92804701065,
-295.950353000282));
#206389=CARTESIAN_POINT('Ctrl Pts',(4267.35939035666,-1337.81286567079,
-282.48361900022));
#206390=CARTESIAN_POINT('Ctrl Pts',(3678.07420496136,-1309.69768433093,
-269.016885000157));
#206391=CARTESIAN_POINT('Ctrl Pts',(3088.78901956605,-1281.58250299106,
-255.550151000094));
#206392=CARTESIAN_POINT('Ctrl Pts',(2794.1464268684,-1267.52491232113,-248.816784000063));
#206393=CARTESIAN_POINT('Ctrl Pts',(2499.50383417074,-1253.4673216512,-242.083417000031));
#206394=CARTESIAN_POINT('Ctrl Pts',(2204.8612414731,-1239.40973098127,-235.35005));
#206395=CARTESIAN_POINT('Ctrl Pts',(1913.13590216849,-1225.49132437738,
-228.683349999968));
#206396=CARTESIAN_POINT('Ctrl Pts',(1621.45955977666,-1212.11656254984,
-222.01665));
#206397=CARTESIAN_POINT('Ctrl Pts',(1329.83024235737,-1199.28546008462,
-215.349949999969));
#206398=CARTESIAN_POINT('Ctrl Pts',(1326.91394918317,-1199.15714905996,
-215.283282999969));
#206399=CARTESIAN_POINT('Ctrl Pts',(1323.99765600898,-1199.02883803529,
-215.216615999969));
#206400=CARTESIAN_POINT('Ctrl Pts',(1321.08136283478,-1198.90052701063,
-215.149948999969));
#206401=CARTESIAN_POINT('Ctrl Pts',(6019.06494805854,-1089.94300070186,
-376.750757000469));
#206402=CARTESIAN_POINT('Ctrl Pts',(5170.46385891687,-1053.99067643293,
-349.817289000379));
#206403=CARTESIAN_POINT('Ctrl Pts',(4321.8627697752,-1018.03835216401,-322.88382100029));
#206404=CARTESIAN_POINT('Ctrl Pts',(3473.26168063352,-982.086027895082,
-295.950353000201));
#206405=CARTESIAN_POINT('Ctrl Pts',(3048.96113606269,-964.10986576062,-282.483619000157));
#206406=CARTESIAN_POINT('Ctrl Pts',(2624.66059149186,-946.133703626157,
-269.016885000112));
#206407=CARTESIAN_POINT('Ctrl Pts',(2200.36004692103,-928.157541491694,
-255.550151000067));
#206408=CARTESIAN_POINT('Ctrl Pts',(1988.2097746356,-919.169460424462,-248.816784000044));
#206409=CARTESIAN_POINT('Ctrl Pts',(1776.05950235019,-910.181379357231,
-242.083417000023));
#206410=CARTESIAN_POINT('Ctrl Pts',(1563.90923006478,-901.19329829,-235.35005));
#206411=CARTESIAN_POINT('Ctrl Pts',(1353.85945552476,-892.294208124424,
-228.683349999978));
#206412=CARTESIAN_POINT('Ctrl Pts',(1143.84459939364,-883.782145858533,
-222.01665));
#206413=CARTESIAN_POINT('Ctrl Pts',(933.863257817356,-875.657121924021,
-215.349949999977));
#206414=CARTESIAN_POINT('Ctrl Pts',(931.763444401592,-875.575871684668,
-215.283282999978));
#206415=CARTESIAN_POINT('Ctrl Pts',(929.663630985828,-875.494621445315,
-215.216615999977));
#206416=CARTESIAN_POINT('Ctrl Pts',(927.563817570064,-875.413371205962,
-215.149948999978));
#206417=CARTESIAN_POINT('Ctrl Pts',(3645.77420799329,-645.266866353884,
-376.75075700028));
#206418=CARTESIAN_POINT('Ctrl Pts',(3127.14240050056,-629.592580495759,
-349.817289000227));
#206419=CARTESIAN_POINT('Ctrl Pts',(2608.51059300782,-613.918294637635,
-322.883821000173));
#206420=CARTESIAN_POINT('Ctrl Pts',(2089.87878551509,-598.24400877951,-295.95035300012));
#206421=CARTESIAN_POINT('Ctrl Pts',(1830.56288176873,-590.406865850448,
-282.483619000093));
#206422=CARTESIAN_POINT('Ctrl Pts',(1571.24697802237,-582.569722921386,
-269.016885000067));
#206423=CARTESIAN_POINT('Ctrl Pts',(1311.931074276,-574.732579992324,-255.55015100004));
#206424=CARTESIAN_POINT('Ctrl Pts',(1182.27312240282,-570.814008527792,
-248.816784000027));
#206425=CARTESIAN_POINT('Ctrl Pts',(1052.61517052964,-566.895437063261,
-242.083417000014));
#206426=CARTESIAN_POINT('Ctrl Pts',(922.957218656454,-562.97686559873,-235.35005));
#206427=CARTESIAN_POINT('Ctrl Pts',(794.583008881026,-559.097091871471,
-228.683349999987));
#206428=CARTESIAN_POINT('Ctrl Pts',(666.229639010622,-555.447729167229,
-222.01665));
#206429=CARTESIAN_POINT('Ctrl Pts',(537.896273277345,-552.028783763422,
-215.349949999987));
#206430=CARTESIAN_POINT('Ctrl Pts',(536.612939620012,-551.994594309379,
-215.283282999987));
#206431=CARTESIAN_POINT('Ctrl Pts',(535.329605962679,-551.960404855337,
-215.216615999987));
#206432=CARTESIAN_POINT('Ctrl Pts',(534.046272305346,-551.926215401294,
-215.149948999987));
#206433=CARTESIAN_POINT('Ctrl Pts',(2854.6772946382,-497.041488237892,-376.750757000217));
#206434=CARTESIAN_POINT('Ctrl Pts',(2446.03524769512,-488.126548516702,
-349.817289000176));
#206435=CARTESIAN_POINT('Ctrl Pts',(2037.39320075203,-479.211608795511,
-322.883821000135));
#206436=CARTESIAN_POINT('Ctrl Pts',(1628.75115380895,-470.29666907432,-295.950353000093));
#206437=CARTESIAN_POINT('Ctrl Pts',(1424.43013033741,-465.839199213724,
-282.483619000073));
#206438=CARTESIAN_POINT('Ctrl Pts',(1220.10910686587,-461.381729353129,
-269.016885000052));
#206439=CARTESIAN_POINT('Ctrl Pts',(1015.78808339432,-456.924259492534,
-255.550151000031));
#206440=CARTESIAN_POINT('Ctrl Pts',(913.627571658554,-454.695524562236,
-248.816784000021));
#206441=CARTESIAN_POINT('Ctrl Pts',(811.467059922784,-452.466789631938,
-242.083417000011));
#206442=CARTESIAN_POINT('Ctrl Pts',(709.306548187014,-450.23805470164,-235.35005));
#206443=CARTESIAN_POINT('Ctrl Pts',(608.157526666449,-448.03138645382,-228.68334999999));
#206444=CARTESIAN_POINT('Ctrl Pts',(507.024652216282,-446.002923603462,
-222.01665));
#206445=CARTESIAN_POINT('Ctrl Pts',(405.907278430675,-444.152671043223,
-215.34994999999));
#206446=CARTESIAN_POINT('Ctrl Pts',(404.896104692818,-444.134168517617,
-215.283282999989));
#206447=CARTESIAN_POINT('Ctrl Pts',(403.884930954962,-444.115665992011,
-215.21661599999));
#206448=CARTESIAN_POINT('Ctrl Pts',(402.873757217106,-444.097163466405,
-215.14994899999));
#206449=CARTESIAN_POINT('Ctrl Pts',(2063.58038128312,-348.816110121901,
-376.750757000154));
#206450=CARTESIAN_POINT('Ctrl Pts',(1764.92809488968,-346.660516537644,
-349.817289000125));
#206451=CARTESIAN_POINT('Ctrl Pts',(1466.27580849624,-344.504922953386,
-322.883821000096));
#206452=CARTESIAN_POINT('Ctrl Pts',(1167.6235221028,-342.349329369129,-295.950353000066));
#206453=CARTESIAN_POINT('Ctrl Pts',(1018.29737890609,-341.271532577001,
-282.483619000052));
#206454=CARTESIAN_POINT('Ctrl Pts',(868.971235709368,-340.193735784872,
-269.016885000037));
#206455=CARTESIAN_POINT('Ctrl Pts',(719.64509251265,-339.115938992743,-255.550151000022));
#206456=CARTESIAN_POINT('Ctrl Pts',(644.982020914291,-338.577040596679,
-248.816784000015));
#206457=CARTESIAN_POINT('Ctrl Pts',(570.318949315933,-338.038142200615,
-242.083417000008));
#206458=CARTESIAN_POINT('Ctrl Pts',(495.655877717574,-337.49924380455,-235.35005));
#206459=CARTESIAN_POINT('Ctrl Pts',(421.732044451872,-336.96568103617,-228.683349999993));
#206460=CARTESIAN_POINT('Ctrl Pts',(347.819665421942,-336.558118039694,
-222.01665));
#206461=CARTESIAN_POINT('Ctrl Pts',(273.918283584005,-336.276558323023,
-215.349949999993));
#206462=CARTESIAN_POINT('Ctrl Pts',(273.179269765626,-336.273742725853,
-215.283282999993));
#206463=CARTESIAN_POINT('Ctrl Pts',(272.440255947246,-336.270927128685,
-215.216615999993));
#206464=CARTESIAN_POINT('Ctrl Pts',(271.701242128866,-336.268111531515,
-215.149948999993));
#206465=CARTESIAN_POINT('Ctrl Pts',(1272.48346792803,-200.59073200591,-376.750757000092));
#206466=CARTESIAN_POINT('Ctrl Pts',(1083.82094208424,-205.194484558586,
-349.817289000074));
#206467=CARTESIAN_POINT('Ctrl Pts',(895.15841624045,-209.798237111262,-322.883821000057));
#206468=CARTESIAN_POINT('Ctrl Pts',(706.49589039666,-214.401989663939,-295.950353000039));
#206469=CARTESIAN_POINT('Ctrl Pts',(612.164627474765,-216.703865940277,
-282.483619000031));
#206470=CARTESIAN_POINT('Ctrl Pts',(517.83336455287,-219.005742216615,-269.016885000022));
#206471=CARTESIAN_POINT('Ctrl Pts',(423.502101630976,-221.307618492953,
-255.550151000013));
#206472=CARTESIAN_POINT('Ctrl Pts',(376.336470170028,-222.458556631122,
-248.816784000009));
#206473=CARTESIAN_POINT('Ctrl Pts',(329.170838709081,-223.609494769291,
-242.083417000004));
#206474=CARTESIAN_POINT('Ctrl Pts',(282.005207248134,-224.760432907461,
-235.35005));
#206475=CARTESIAN_POINT('Ctrl Pts',(235.306562237295,-225.899975618519,
-228.683349999995));
#206476=CARTESIAN_POINT('Ctrl Pts',(188.614678627603,-227.113312475926,
-222.01665));
#206477=CARTESIAN_POINT('Ctrl Pts',(141.929288737335,-228.400445602824,
-215.349949999996));
#206478=CARTESIAN_POINT('Ctrl Pts',(141.462434838432,-228.413316934091,
-215.283282999995));
#206479=CARTESIAN_POINT('Ctrl Pts',(140.995580939529,-228.426188265358,
-215.216615999995));
#206480=CARTESIAN_POINT('Ctrl Pts',(140.528727040626,-228.439059596626,
-215.149948999996));
#206481=CARTESIAN_POINT('Ctrl Pts',(1008.78449680967,-151.182272633913,
-376.750757000071));
#206482=CARTESIAN_POINT('Ctrl Pts',(856.785224482427,-158.039140565566,
-349.817289000057));
#206483=CARTESIAN_POINT('Ctrl Pts',(704.785952155186,-164.896008497221,
-322.883821000044));
#206484=CARTESIAN_POINT('Ctrl Pts',(552.786679827945,-171.752876428875,
-295.95035300003));
#206485=CARTESIAN_POINT('Ctrl Pts',(476.787043664325,-175.181310394702,
-282.483619000024));
#206486=CARTESIAN_POINT('Ctrl Pts',(400.787407500704,-178.609744360529,
-269.016885000016));
#206487=CARTESIAN_POINT('Ctrl Pts',(324.787771337084,-182.038178326357,
-255.55015100001));
#206488=CARTESIAN_POINT('Ctrl Pts',(286.787953255274,-183.75239530927,-248.816784000007));
#206489=CARTESIAN_POINT('Ctrl Pts',(248.788135173463,-185.466612292184,
-242.083417000003));
#206490=CARTESIAN_POINT('Ctrl Pts',(210.788317091653,-187.180829275097,
-235.35005));
#206491=CARTESIAN_POINT('Ctrl Pts',(173.164734832436,-188.878073812635,
-228.683349999997));
#206492=CARTESIAN_POINT('Ctrl Pts',(135.546349696156,-190.631710621336,
-222.01665));
#206493=CARTESIAN_POINT('Ctrl Pts',(97.932957121778,-192.441741362757,-215.349949999997));
#206494=CARTESIAN_POINT('Ctrl Pts',(97.5568231960341,-192.45984167017,-215.283282999997));
#206495=CARTESIAN_POINT('Ctrl Pts',(97.1806892702902,-192.477941977583,
-215.216615999996));
#206496=CARTESIAN_POINT('Ctrl Pts',(96.8045553445463,-192.496042284996,
-215.149948999996));
#206497=CARTESIAN_POINT('Ctrl Pts',(745.085525691306,-101.773813261915,
-376.75075700005));
#206498=CARTESIAN_POINT('Ctrl Pts',(629.749506880614,-110.883796572547,
-349.81728900004));
#206499=CARTESIAN_POINT('Ctrl Pts',(514.413488069922,-119.993779883179,
-322.88382100003));
#206500=CARTESIAN_POINT('Ctrl Pts',(399.07746925923,-129.103763193811,-295.950353000021));
#206501=CARTESIAN_POINT('Ctrl Pts',(341.409459853884,-133.658754849127,
-282.483619000017));
#206502=CARTESIAN_POINT('Ctrl Pts',(283.741450448538,-138.213746504444,
-269.016885000012));
#206503=CARTESIAN_POINT('Ctrl Pts',(226.073441043192,-142.76873815976,-255.550151000007));
#206504=CARTESIAN_POINT('Ctrl Pts',(197.239436340519,-145.046233987418,
-248.816784000005));
#206505=CARTESIAN_POINT('Ctrl Pts',(168.405431637847,-147.323729815076,
-242.083417000002));
#206506=CARTESIAN_POINT('Ctrl Pts',(139.571426935173,-149.601225642734,
-235.35005));
#206507=CARTESIAN_POINT('Ctrl Pts',(111.022907427576,-151.856172006752,
-228.683349999998));
#206508=CARTESIAN_POINT('Ctrl Pts',(82.4780207647092,-154.150108766748,
-222.01665));
#206509=CARTESIAN_POINT('Ctrl Pts',(53.9366255062213,-156.48303712269,-215.349949999998));
#206510=CARTESIAN_POINT('Ctrl Pts',(53.6512115536363,-156.506366406249,
-215.283282999997));
#206511=CARTESIAN_POINT('Ctrl Pts',(53.3657976010514,-156.529695689807,
-215.216615999998));
#206512=CARTESIAN_POINT('Ctrl Pts',(53.0803836484664,-156.553024973366,
-215.149948999998));
#206513=CARTESIAN_POINT('Ctrl Pts',(481.386554572944,-52.3653538899179,
-376.750757000028));
#206514=CARTESIAN_POINT('Ctrl Pts',(402.713789278801,-63.7284525795279,
-349.817289000023));
#206515=CARTESIAN_POINT('Ctrl Pts',(324.041023984658,-75.0915512691379,
-322.883821000018));
#206516=CARTESIAN_POINT('Ctrl Pts',(245.368258690515,-86.4546499587479,
-295.950353000012));
#206517=CARTESIAN_POINT('Ctrl Pts',(206.031876043444,-92.1361993035529,
-282.48361900001));
#206518=CARTESIAN_POINT('Ctrl Pts',(166.695493396372,-97.8177486483579,
-269.016885000007));
#206519=CARTESIAN_POINT('Ctrl Pts',(127.359110749301,-103.499297993163,
-255.550151000004));
#206520=CARTESIAN_POINT('Ctrl Pts',(107.690919425765,-106.340072665565,
-248.816784000003));
#206521=CARTESIAN_POINT('Ctrl Pts',(88.0227281022291,-109.180847337968,
-242.083417000002));
#206522=CARTESIAN_POINT('Ctrl Pts',(68.3545367786933,-112.02162201037,-235.35005));
#206523=CARTESIAN_POINT('Ctrl Pts',(48.8810800227174,-114.834270200868,
-228.683349999999));
#206524=CARTESIAN_POINT('Ctrl Pts',(29.4096918332626,-117.668506912158,
-222.01665));
#206525=CARTESIAN_POINT('Ctrl Pts',(9.94029389066457,-120.524332882624,
-215.349949999999));
#206526=CARTESIAN_POINT('Ctrl Pts',(9.74559991123855,-120.552891142328,
-215.283282999999));
#206527=CARTESIAN_POINT('Ctrl Pts',(9.55090593181253,-120.581449402032,
-215.216615999999));
#206528=CARTESIAN_POINT('Ctrl Pts',(9.3562119523865,-120.610007661736,-215.149948999999));
#206529=CARTESIAN_POINT('Ctrl Pts',(393.48689753349,-35.8958674325856,-376.750757000021));
#206530=CARTESIAN_POINT('Ctrl Pts',(327.035216744864,-48.0100045818548,
-349.817289000017));
#206531=CARTESIAN_POINT('Ctrl Pts',(260.583535956237,-60.1241417311241,
-322.883821000013));
#206532=CARTESIAN_POINT('Ctrl Pts',(194.13185516761,-72.2382788803934,-295.950353000009));
#206533=CARTESIAN_POINT('Ctrl Pts',(160.906014773297,-78.2953474550281,
-282.483619000007));
#206534=CARTESIAN_POINT('Ctrl Pts',(127.680174378983,-84.3524160296627,
-269.016885000005));
#206535=CARTESIAN_POINT('Ctrl Pts',(94.45433398467,-90.4094846042973,-255.550151000003));
#206536=CARTESIAN_POINT('Ctrl Pts',(77.8414137875133,-93.4380188916147,
-248.816784000002));
#206537=CARTESIAN_POINT('Ctrl Pts',(61.2284935903567,-96.466553178932,-242.083417000001));
#206538=CARTESIAN_POINT('Ctrl Pts',(44.6155733932,-99.4950874662493,-235.35005));
#206539=CARTESIAN_POINT('Ctrl Pts',(28.167137554431,-102.493636265573,-228.683349999999));
#206540=CARTESIAN_POINT('Ctrl Pts',(11.7202488561137,-105.507972960628,
-222.01665));
#206541=CARTESIAN_POINT('Ctrl Pts',(-4.72514998118767,-108.538098135935,
-215.349949999999));
#206542=CARTESIAN_POINT('Ctrl Pts',(-4.88960396956071,-108.568399387688,
-215.283282999999));
#206543=CARTESIAN_POINT('Ctrl Pts',(-5.05405795793375,-108.59870063944,
-215.216615999999));
#206544=CARTESIAN_POINT('Ctrl Pts',(-5.2185119463068,-108.629001891193,
-215.149948999999));
#206545=CARTESIAN_POINT('Ctrl Pts',(305.587240494037,-19.4263809752531,
-376.750757000014));
#206546=CARTESIAN_POINT('Ctrl Pts',(251.356644210927,-32.2915565841817,
-349.817289000011));
#206547=CARTESIAN_POINT('Ctrl Pts',(197.126047927816,-45.1567321931103,
-322.883821000009));
#206548=CARTESIAN_POINT('Ctrl Pts',(142.895451644705,-58.0219078020389,
-295.950353000006));
#206549=CARTESIAN_POINT('Ctrl Pts',(115.78015350315,-64.4544956065032,-282.483619000005));
#206550=CARTESIAN_POINT('Ctrl Pts',(88.6648553615948,-70.8870834109675,
-269.016885000003));
#206551=CARTESIAN_POINT('Ctrl Pts',(61.5495572200395,-77.3196712154318,
-255.550151000002));
#206552=CARTESIAN_POINT('Ctrl Pts',(47.9919081492619,-80.5359651176639,
-248.816784000002));
#206553=CARTESIAN_POINT('Ctrl Pts',(34.4342590784842,-83.7522590198961,
-242.083417000001));
#206554=CARTESIAN_POINT('Ctrl Pts',(20.8766100077067,-86.9685529221282,
-235.35005));
#206555=CARTESIAN_POINT('Ctrl Pts',(7.45319508614462,-90.1530023302789,
-228.68335));
#206556=CARTESIAN_POINT('Ctrl Pts',(-5.96919412103514,-93.3474390090985,
-222.01665));
#206557=CARTESIAN_POINT('Ctrl Pts',(-19.3905938530399,-96.5518633892461,
-215.34995));
#206558=CARTESIAN_POINT('Ctrl Pts',(-19.52480785036,-96.5839076330473,-215.283283));
#206559=CARTESIAN_POINT('Ctrl Pts',(-19.6590218476801,-96.6159518768485,
-215.216616));
#206560=CARTESIAN_POINT('Ctrl Pts',(-19.7932358450001,-96.6479961206498,
-215.149949));
#206561=CARTESIAN_POINT('Ctrl Pts',(217.687583454584,-2.9568945179205,-376.750757000007));
#206562=CARTESIAN_POINT('Ctrl Pts',(175.67807167699,-16.5731085865084,-349.817289000006));
#206563=CARTESIAN_POINT('Ctrl Pts',(133.668559899395,-30.1893226550964,
-322.883821000005));
#206564=CARTESIAN_POINT('Ctrl Pts',(91.6590481218006,-43.8055367236842,
-295.950353000003));
#206565=CARTESIAN_POINT('Ctrl Pts',(70.6542922330034,-50.6136437579782,
-282.483619000003));
#206566=CARTESIAN_POINT('Ctrl Pts',(49.6495363442062,-57.4217507922722,
-269.016885000001));
#206567=CARTESIAN_POINT('Ctrl Pts',(28.644780455409,-64.2298578265662,-255.550151000001));
#206568=CARTESIAN_POINT('Ctrl Pts',(18.1424025110104,-67.6339113437132,
-248.816784000001));
#206569=CARTESIAN_POINT('Ctrl Pts',(7.64002456661188,-71.0379648608601,
-242.083417000001));
#206570=CARTESIAN_POINT('Ctrl Pts',(-2.8623533777867,-74.4420183780071,
-235.35005));
#206571=CARTESIAN_POINT('Ctrl Pts',(-13.2607473821417,-77.8123683949843,
-228.68335));
#206572=CARTESIAN_POINT('Ctrl Pts',(-23.658637098184,-81.1869050575687,
-222.01665));
#206573=CARTESIAN_POINT('Ctrl Pts',(-34.0560377248921,-84.5656286425572,
-215.34995));
#206574=CARTESIAN_POINT('Ctrl Pts',(-34.1600117311593,-84.599415878407,
-215.283283));
#206575=CARTESIAN_POINT('Ctrl Pts',(-34.2639857374263,-84.6332031142567,
-215.216616));
#206576=CARTESIAN_POINT('Ctrl Pts',(-34.3679597436934,-84.6669903501065,
-215.149949));
#206577=CARTESIAN_POINT('Ctrl Pts',(188.387697774766,2.53293430119023,-376.750757000005));
#206578=CARTESIAN_POINT('Ctrl Pts',(150.451880832343,-11.3336259206174,
-349.817289000004));
#206579=CARTESIAN_POINT('Ctrl Pts',(112.516063889921,-25.2001861424251,
-322.883821000003));
#206580=CARTESIAN_POINT('Ctrl Pts',(74.580246947499,-39.0667463642328,-295.950353000002));
#206581=CARTESIAN_POINT('Ctrl Pts',(55.6123384762878,-46.0000264751366,
-282.483619000002));
#206582=CARTESIAN_POINT('Ctrl Pts',(36.6444300050767,-52.9333065860405,
-269.016885000001));
#206583=CARTESIAN_POINT('Ctrl Pts',(17.6765215338656,-59.8665866969443,
-255.550151000001));
#206584=CARTESIAN_POINT('Ctrl Pts',(8.19256729825999,-63.3332267523963,
-248.816784000001));
#206585=CARTESIAN_POINT('Ctrl Pts',(-1.29138693734558,-66.7998668078482,
-242.083417));
#206586=CARTESIAN_POINT('Ctrl Pts',(-10.7753411729511,-70.2665068633001,
-235.35005));
#206587=CARTESIAN_POINT('Ctrl Pts',(-20.1653948715705,-73.6988237498861,
-228.68335));
#206588=CARTESIAN_POINT('Ctrl Pts',(-29.5551180905669,-77.1333937403921,
-222.01665));
#206589=CARTESIAN_POINT('Ctrl Pts',(-38.9445190155095,-80.5702170603276,
-215.34995));
#206590=CARTESIAN_POINT('Ctrl Pts',(-39.038413024759,-80.6045852935269,
-215.283283));
#206591=CARTESIAN_POINT('Ctrl Pts',(-39.1323070340084,-80.6389535267262,
-215.216616));
#206592=CARTESIAN_POINT('Ctrl Pts',(-39.2262010432579,-80.6733217599254,
-215.149949));
#206593=CARTESIAN_POINT('Ctrl Pts',(159.087812094948,8.022763120301,-376.750757000003));
#206594=CARTESIAN_POINT('Ctrl Pts',(125.225689987698,-6.09414325472644,
-349.817289000002));
#206595=CARTESIAN_POINT('Ctrl Pts',(91.3635678804476,-20.2110496297539,
-322.883821000001));
#206596=CARTESIAN_POINT('Ctrl Pts',(57.5014457731974,-34.3279560047813,
-295.950353000001));
#206597=CARTESIAN_POINT('Ctrl Pts',(40.5703847195723,-41.386409192295,-282.483619000001));
#206598=CARTESIAN_POINT('Ctrl Pts',(23.6393236659472,-48.4448623798088,
-269.016885));
#206599=CARTESIAN_POINT('Ctrl Pts',(6.70826261232206,-55.5033155673225,
-255.550151000001));
#206600=CARTESIAN_POINT('Ctrl Pts',(-1.75726791449049,-59.0325421610793,
-248.816784));
#206601=CARTESIAN_POINT('Ctrl Pts',(-10.222798441303,-62.5617687548362,
-242.083417));
#206602=CARTESIAN_POINT('Ctrl Pts',(-18.6883289681156,-66.090995348593,
-235.35005));
#206603=CARTESIAN_POINT('Ctrl Pts',(-27.0700423609993,-69.585279104788,
-228.68335));
#206604=CARTESIAN_POINT('Ctrl Pts',(-35.4515990829499,-73.0798824232155,
-222.01665));
#206605=CARTESIAN_POINT('Ctrl Pts',(-43.833000306127,-76.574805478098,-215.34995));
#206606=CARTESIAN_POINT('Ctrl Pts',(-43.9168143183588,-76.6097547086468,
-215.283283));
#206607=CARTESIAN_POINT('Ctrl Pts',(-44.0006283305905,-76.6447039391955,
-215.216616));
#206608=CARTESIAN_POINT('Ctrl Pts',(-44.0844423428223,-76.6796531697443,
-215.149949));
#206609=CARTESIAN_POINT('Ctrl Pts',(129.78792641513,13.512591939412,-376.750757));
#206610=CARTESIAN_POINT('Ctrl Pts',(99.9994991430521,-0.854660588835203,
-349.817289000001));
#206611=CARTESIAN_POINT('Ctrl Pts',(70.211071870974,-15.2219131170825,-322.883821));
#206612=CARTESIAN_POINT('Ctrl Pts',(40.4226445988958,-29.5891656453297,
-295.950353));
#206613=CARTESIAN_POINT('Ctrl Pts',(25.5284309628568,-36.7727919094533,
-282.483619));
#206614=CARTESIAN_POINT('Ctrl Pts',(10.6342173268177,-43.9564181735769,
-269.016885));
#206615=CARTESIAN_POINT('Ctrl Pts',(-4.25999630922143,-51.1400444377006,
-255.550151));
#206616=CARTESIAN_POINT('Ctrl Pts',(-11.707103127241,-54.7318575697624,
-248.816784));
#206617=CARTESIAN_POINT('Ctrl Pts',(-19.1542099452605,-58.3236707018242,
-242.083417));
#206618=CARTESIAN_POINT('Ctrl Pts',(-26.60131676328,-61.915483833886,-235.35005));
#206619=CARTESIAN_POINT('Ctrl Pts',(-33.9746898504281,-65.4717344596898,
-228.68335));
#206620=CARTESIAN_POINT('Ctrl Pts',(-41.3480800753329,-69.0263711060389,
-222.01665));
#206621=CARTESIAN_POINT('Ctrl Pts',(-48.7214815967444,-72.5793938958684,
-215.34995));
#206622=CARTESIAN_POINT('Ctrl Pts',(-48.7952156119585,-72.6149241237667,
-215.283283));
#206623=CARTESIAN_POINT('Ctrl Pts',(-48.8689496271726,-72.6504543516649,
-215.216616));
#206624=CARTESIAN_POINT('Ctrl Pts',(-48.9426836423867,-72.6859845795632,
-215.149949));
#206625=CARTESIAN_POINT('Ctrl Pts',(122.462954995176,14.8850491441897,-376.750756999999));
#206626=CARTESIAN_POINT('Ctrl Pts',(93.6929514318907,0.455210077637512,
-349.817289));
#206627=CARTESIAN_POINT('Ctrl Pts',(64.9229478686056,-13.9746289889147,
-322.883821));
#206628=CARTESIAN_POINT('Ctrl Pts',(36.1529443053205,-28.4044680554669,
-295.950353));
#206629=CARTESIAN_POINT('Ctrl Pts',(21.7679425236779,-35.619387588743,-282.483619));
#206630=CARTESIAN_POINT('Ctrl Pts',(7.38294074203528,-42.834307122019,-269.016885));
#206631=CARTESIAN_POINT('Ctrl Pts',(-7.00206103960729,-50.0492266552951,
-255.550151));
#206632=CARTESIAN_POINT('Ctrl Pts',(-14.1945619304286,-53.6566864219332,
-248.816784));
#206633=CARTESIAN_POINT('Ctrl Pts',(-21.3870628212499,-57.2641461885712,
-242.083417));
#206634=CARTESIAN_POINT('Ctrl Pts',(-28.5795637120712,-60.8716059552093,
-235.35005));
#206635=CARTESIAN_POINT('Ctrl Pts',(-35.7008517227853,-64.4433482984152,
-228.68335));
#206636=CARTESIAN_POINT('Ctrl Pts',(-42.8222003234286,-68.0129932767448,
-222.01665));
#206637=CARTESIAN_POINT('Ctrl Pts',(-49.9436019193987,-71.5805410003109,
-215.34995));
#206638=CARTESIAN_POINT('Ctrl Pts',(-50.0148159353584,-71.6162164775466,
-215.283283));
#206639=CARTESIAN_POINT('Ctrl Pts',(-50.0860299513181,-71.6518919547823,
-215.216616));
#206640=CARTESIAN_POINT('Ctrl Pts',(-50.1572439672778,-71.687567432018,
-215.149949));
#206641=CARTESIAN_POINT('Ctrl Pts',(103.0219124536,22.8222305961756,-376.750757000007));
#206642=CARTESIAN_POINT('Ctrl Pts',(77.174697282254,7.34909250165779,-349.817289000007));
#206643=CARTESIAN_POINT('Ctrl Pts',(51.3274821109085,-8.12404559286004,
-322.883821000005));
#206644=CARTESIAN_POINT('Ctrl Pts',(25.480266939563,-23.5971836873778,-295.950353000003));
#206645=CARTESIAN_POINT('Ctrl Pts',(12.5566593538902,-31.3337527346368,
-282.483619000003));
#206646=CARTESIAN_POINT('Ctrl Pts',(-0.366948231782582,-39.0703217818957,
-269.016885000003));
#206647=CARTESIAN_POINT('Ctrl Pts',(-13.2905558174553,-46.8068908291546,
-255.550151000002));
#206648=CARTESIAN_POINT('Ctrl Pts',(-19.7523596102917,-50.6751753527841,
-248.816784000002));
#206649=CARTESIAN_POINT('Ctrl Pts',(-26.2141634031281,-54.5434598764135,
-242.083417000001));
#206650=CARTESIAN_POINT('Ctrl Pts',(-32.6759671959645,-58.411744400043,
-235.350050000001));
#206651=CARTESIAN_POINT('Ctrl Pts',(-39.0737927334262,-62.2417290769038,
-228.683350000001));
#206652=CARTESIAN_POINT('Ctrl Pts',(-45.4718450018044,-66.0691978041651,
-222.01665));
#206653=CARTESIAN_POINT('Ctrl Pts',(-51.8701148758579,-69.894150514329,
-215.34995));
#206654=CARTESIAN_POINT('Ctrl Pts',(-51.9340975745985,-69.9324000414307,
-215.283283));
#206655=CARTESIAN_POINT('Ctrl Pts',(-51.998080273339,-69.9706495685323,
-215.216616));
#206656=CARTESIAN_POINT('Ctrl Pts',(-52.0620629720796,-70.0088990956339,
-215.149949));
#206657=CARTESIAN_POINT('Ctrl Pts',(71.4332298554826,45.3676034181815,-376.750756999996));
#206658=CARTESIAN_POINT('Ctrl Pts',(50.4371334176971,26.5324811107851,-349.817288999997));
#206659=CARTESIAN_POINT('Ctrl Pts',(29.4410369799117,7.69735880338874,-322.883820999997));
#206660=CARTESIAN_POINT('Ctrl Pts',(8.44494054212614,-11.1377635040076,
-295.950352999998));
#206661=CARTESIAN_POINT('Ctrl Pts',(-2.05310767676661,-20.5553246577058,
-282.483618999998));
#206662=CARTESIAN_POINT('Ctrl Pts',(-12.5511558956594,-29.972885811404,
-269.016884999999));
#206663=CARTESIAN_POINT('Ctrl Pts',(-23.0492041145521,-39.3904469651022,
-255.550150999999));
#206664=CARTESIAN_POINT('Ctrl Pts',(-28.2982282239985,-44.0992275419513,
-248.816783999999));
#206665=CARTESIAN_POINT('Ctrl Pts',(-33.5472523334448,-48.8080081188004,
-242.083416999999));
#206666=CARTESIAN_POINT('Ctrl Pts',(-38.7962764428913,-53.5167886956495,
-235.35005));
#206667=CARTESIAN_POINT('Ctrl Pts',(-43.9933300166005,-58.1789476826288,
-228.68335));
#206668=CARTESIAN_POINT('Ctrl Pts',(-49.1909136386903,-62.839044754287,
-222.01665));
#206669=CARTESIAN_POINT('Ctrl Pts',(-54.3890197977427,-67.4970794092701,
-215.34995));
#206670=CARTESIAN_POINT('Ctrl Pts',(-54.4410008593333,-67.5436597558199,
-215.283283));
#206671=CARTESIAN_POINT('Ctrl Pts',(-54.4929819209238,-67.5902401023698,
-215.216616));
#206672=CARTESIAN_POINT('Ctrl Pts',(-54.5449629825143,-67.6368204489196,
-215.149949));
#206673=CARTESIAN_POINT('Ctrl Pts',(45.0390725903934,73.7599134480721,-376.750757000003));
#206674=CARTESIAN_POINT('Ctrl Pts',(28.0469137085574,50.6061693294573,-349.817289000002));
#206675=CARTESIAN_POINT('Ctrl Pts',(11.0547548267215,27.4524252108426,-322.883821000002));
#206676=CARTESIAN_POINT('Ctrl Pts',(-5.93740405511448,4.29868109222778,
-295.950353000001));
#206677=CARTESIAN_POINT('Ctrl Pts',(-14.4334834960324,-7.2781909670796,
-282.483619000001));
#206678=CARTESIAN_POINT('Ctrl Pts',(-22.9295629369504,-18.855063026387,
-269.016885000001));
#206679=CARTESIAN_POINT('Ctrl Pts',(-31.4256423778684,-30.4319350856944,
-255.550151000001));
#206680=CARTESIAN_POINT('Ctrl Pts',(-35.6736820983274,-36.2203711153481,
-248.816784000001));
#206681=CARTESIAN_POINT('Ctrl Pts',(-39.9217218187864,-42.0088071450018,
-242.083417000001));
#206682=CARTESIAN_POINT('Ctrl Pts',(-44.1697615392454,-47.7972431746554,
-235.35005));
#206683=CARTESIAN_POINT('Ctrl Pts',(-48.3757414604919,-53.5283679564908,
-228.68335));
#206684=CARTESIAN_POINT('Ctrl Pts',(-52.582425249623,-59.2584041216488,
-222.01665));
#206685=CARTESIAN_POINT('Ctrl Pts',(-56.7898089004066,-64.9873508559399,
-215.34995));
#206686=CARTESIAN_POINT('Ctrl Pts',(-56.8318827369145,-65.0446403232828,
-215.283283));
#206687=CARTESIAN_POINT('Ctrl Pts',(-56.8739565734223,-65.1019297906258,
-215.216616));
#206688=CARTESIAN_POINT('Ctrl Pts',(-56.9160304099302,-65.1592192579687,
-215.149949));
#206689=CARTESIAN_POINT('Ctrl Pts',(34.4954719600033,91.6721063226136,-376.750757));
#206690=CARTESIAN_POINT('Ctrl Pts',(18.9810705532065,65.8496728858911,-349.817289000001));
#206691=CARTESIAN_POINT('Ctrl Pts',(3.46666914640964,40.0272394491684,-322.883821));
#206692=CARTESIAN_POINT('Ctrl Pts',(-12.0477322603872,14.2048060124459,
-295.950353));
#206693=CARTESIAN_POINT('Ctrl Pts',(-19.8049329637856,1.2935892940846,-282.483619));
#206694=CARTESIAN_POINT('Ctrl Pts',(-27.562133667184,-11.6176274242767,
-269.016885));
#206695=CARTESIAN_POINT('Ctrl Pts',(-35.3193343705824,-24.528844142638,
-255.550151));
#206696=CARTESIAN_POINT('Ctrl Pts',(-39.1979347222817,-30.9844525018186,
-248.816784));
#206697=CARTESIAN_POINT('Ctrl Pts',(-43.0765350739809,-37.4400608609993,
-242.083417));
#206698=CARTESIAN_POINT('Ctrl Pts',(-46.9551354256801,-43.8956692201799,
-235.35005));
#206699=CARTESIAN_POINT('Ctrl Pts',(-50.7953337936991,-50.2873606649132,
-228.68335));
#206700=CARTESIAN_POINT('Ctrl Pts',(-54.6361431746697,-56.6785834369767,
-222.01665));
#206701=CARTESIAN_POINT('Ctrl Pts',(-58.477561814447,-63.069336786611,-215.34995));
#206702=CARTESIAN_POINT('Ctrl Pts',(-58.5159760008448,-63.1332443201074,
-215.283283));
#206703=CARTESIAN_POINT('Ctrl Pts',(-58.5543901872426,-63.1971518536037,
-215.216616));
#206704=CARTESIAN_POINT('Ctrl Pts',(-58.5928043736403,-63.2610593871,-215.149949));
#206705=CARTESIAN_POINT('Ctrl Pts',(31.8464935875069,98.4079754366887,-376.750756999999));
#206706=CARTESIAN_POINT('Ctrl Pts',(16.6079109017479,71.6637374050134,-349.817289));
#206707=CARTESIAN_POINT('Ctrl Pts',(1.36932821598904,44.919499373338,-322.883821));
#206708=CARTESIAN_POINT('Ctrl Pts',(-13.8692544697699,18.1752613416626,
-295.950353));
#206709=CARTESIAN_POINT('Ctrl Pts',(-21.4885458126493,4.80314232582491,
-282.483619));
#206710=CARTESIAN_POINT('Ctrl Pts',(-29.1078371555287,-8.56897669001278,
-269.016885));
#206711=CARTESIAN_POINT('Ctrl Pts',(-36.7271284984082,-21.9410957058504,
-255.550151));
#206712=CARTESIAN_POINT('Ctrl Pts',(-40.5367741698479,-28.6271552137693,
-248.816784));
#206713=CARTESIAN_POINT('Ctrl Pts',(-44.3464198412877,-35.3132147216881,
-242.083417));
#206714=CARTESIAN_POINT('Ctrl Pts',(-48.1560655127274,-41.999274229607,
-235.35005));
#206715=CARTESIAN_POINT('Ctrl Pts',(-51.9279919200935,-48.6191351285365,
-228.68335));
#206716=CARTESIAN_POINT('Ctrl Pts',(-55.7004001286368,-55.2387363218615,
-222.01665));
#206717=CARTESIAN_POINT('Ctrl Pts',(-59.4732891526772,-61.8580772083615,
-215.34995));
#206718=CARTESIAN_POINT('Ctrl Pts',(-59.5110180429176,-61.9242706172265,
-215.283283));
#206719=CARTESIAN_POINT('Ctrl Pts',(-59.548746933158,-61.9904640260915,
-215.216616));
#206720=CARTESIAN_POINT('Ctrl Pts',(-59.5864758233984,-62.0566574349565,
-215.149949));
#206721=CARTESIAN_POINT('Ctrl Pts',(21.2505800975213,125.351451892989,-376.750756999997));
#206722=CARTESIAN_POINT('Ctrl Pts',(7.11527229591406,94.9199954815027,-349.817288999997));
#206723=CARTESIAN_POINT('Ctrl Pts',(-7.02003550569317,64.4885390700161,
-322.883820999998));
#206724=CARTESIAN_POINT('Ctrl Pts',(-21.1553433073004,34.0570826585295,
-295.950352999998));
#206725=CARTESIAN_POINT('Ctrl Pts',(-28.222997208104,18.8413544527863,-282.483618999999));
#206726=CARTESIAN_POINT('Ctrl Pts',(-35.2906511089077,3.62562624704296,
-269.016884999999));
#206727=CARTESIAN_POINT('Ctrl Pts',(-42.3583050097113,-11.5901019587003,
-255.550151));
#206728=CARTESIAN_POINT('Ctrl Pts',(-45.8921319601131,-19.197966061572,
-248.816784));
#206729=CARTESIAN_POINT('Ctrl Pts',(-49.4259589105149,-26.8058301644436,
-242.083417));
#206730=CARTESIAN_POINT('Ctrl Pts',(-52.9597858609167,-34.4136942673153,
-235.35005));
#206731=CARTESIAN_POINT('Ctrl Pts',(-56.458624425671,-41.9462329830297,
-228.68335));
#206732=CARTESIAN_POINT('Ctrl Pts',(-59.957427944505,-49.4793478614006,
-222.01665));
#206733=CARTESIAN_POINT('Ctrl Pts',(-63.4561985055979,-57.0130388953633,
-215.34995));
#206734=CARTESIAN_POINT('Ctrl Pts',(-63.4911862112088,-57.0883758057029,
-215.283283));
#206735=CARTESIAN_POINT('Ctrl Pts',(-63.5261739168198,-57.1637127160426,
-215.216616));
#206736=CARTESIAN_POINT('Ctrl Pts',(-63.5611616224307,-57.2390496263822,
-215.149949));
#206737=CARTESIAN_POINT('Ctrl Pts',(10.6546666075359,152.29492834929,-376.750756999995));
#206738=CARTESIAN_POINT('Ctrl Pts',(-2.37736630991967,118.176253557992,
-349.817288999995));
#206739=CARTESIAN_POINT('Ctrl Pts',(-15.4093992273753,84.0575787666943,
-322.883820999996));
#206740=CARTESIAN_POINT('Ctrl Pts',(-28.4414321448309,49.9389039753965,
-295.950352999998));
#206741=CARTESIAN_POINT('Ctrl Pts',(-34.9574486035587,32.8795665797476,
-282.483618999998));
#206742=CARTESIAN_POINT('Ctrl Pts',(-41.4734650622865,15.8202291840987,
-269.016884999999));
#206743=CARTESIAN_POINT('Ctrl Pts',(-47.9894815210143,-1.2391082115502,
-255.550151));
#206744=CARTESIAN_POINT('Ctrl Pts',(-51.2474897503782,-9.76877690937465,
-248.816784));
#206745=CARTESIAN_POINT('Ctrl Pts',(-54.5054979797421,-18.2984456071991,
-242.083417));
#206746=CARTESIAN_POINT('Ctrl Pts',(-57.763506209106,-26.8281143050236,
-235.35005));
#206747=CARTESIAN_POINT('Ctrl Pts',(-60.9892569312485,-35.273330837523,
-228.683350000001));
#206748=CARTESIAN_POINT('Ctrl Pts',(-64.2144557603733,-43.7199594009398,
-222.016650000001));
#206749=CARTESIAN_POINT('Ctrl Pts',(-67.4391078585187,-52.1680005823651,
-215.349950000001));
#206750=CARTESIAN_POINT('Ctrl Pts',(-67.4713543795001,-52.2524809941794,
-215.283283000001));
#206751=CARTESIAN_POINT('Ctrl Pts',(-67.5036009004816,-52.3369614059937,
-215.216616));
#206752=CARTESIAN_POINT('Ctrl Pts',(-67.535847421463,-52.4214418178079,
-215.149949000001));
#206753=CARTESIAN_POINT('Ctrl Pts',(0.0587531175507312,179.238404805591,
-376.750756999993));
#206754=CARTESIAN_POINT('Ctrl Pts',(-11.8700049157533,141.432511634481,
-349.817288999993));
#206755=CARTESIAN_POINT('Ctrl Pts',(-23.7987629490573,103.626618463372,
-322.883820999995));
#206756=CARTESIAN_POINT('Ctrl Pts',(-35.7275209823613,65.8207252922634,
-295.950352999997));
#206757=CARTESIAN_POINT('Ctrl Pts',(-41.6918999990133,46.9177787067089,
-282.483618999997));
#206758=CARTESIAN_POINT('Ctrl Pts',(-47.6562790156653,28.0148321211544,
-269.016884999998));
#206759=CARTESIAN_POINT('Ctrl Pts',(-53.6206580323173,9.11188553559992,
-255.550150999999));
#206760=CARTESIAN_POINT('Ctrl Pts',(-56.6028475406433,-0.339587757177323,
-248.816784));
#206761=CARTESIAN_POINT('Ctrl Pts',(-59.5850370489693,-9.79106104995457,
-242.083416999999));
#206762=CARTESIAN_POINT('Ctrl Pts',(-62.5672265572953,-19.2425343427318,
-235.35005));
#206763=CARTESIAN_POINT('Ctrl Pts',(-65.519889436826,-28.6004286920162,
-228.683350000001));
#206764=CARTESIAN_POINT('Ctrl Pts',(-68.4714835762416,-37.9605709404789,
-222.016650000001));
#206765=CARTESIAN_POINT('Ctrl Pts',(-71.4220172114394,-47.322962269367,
-215.349950000001));
#206766=CARTESIAN_POINT('Ctrl Pts',(-71.4515225477914,-47.4165861826559,
-215.283283000001));
#206767=CARTESIAN_POINT('Ctrl Pts',(-71.4810278841433,-47.5102100959448,
-215.216616));
#206768=CARTESIAN_POINT('Ctrl Pts',(-71.5105332204953,-47.6038340092336,
-215.149949000001));
#206769=CARTESIAN_POINT('Ctrl Pts',(-31.728987352405,260.068834174492,-376.750756999986));
#206770=CARTESIAN_POINT('Ctrl Pts',(-40.3479207332542,211.20128586395,-349.817288999988));
#206771=CARTESIAN_POINT('Ctrl Pts',(-48.9668541141034,162.333737553407,
-322.883820999991));
#206772=CARTESIAN_POINT('Ctrl Pts',(-57.5857874949526,113.466189242864,
-295.950352999994));
#206773=CARTESIAN_POINT('Ctrl Pts',(-61.8952541853772,89.0324150875929,
-282.483618999995));
#206774=CARTESIAN_POINT('Ctrl Pts',(-66.2047208758018,64.5986409323216,
-269.016884999996));
#206775=CARTESIAN_POINT('Ctrl Pts',(-70.5141875662264,40.1648667770503,
-255.550150999998));
#206776=CARTESIAN_POINT('Ctrl Pts',(-72.6689209114386,27.9479796994146,
-248.816783999999));
#206777=CARTESIAN_POINT('Ctrl Pts',(-74.8236542566509,15.731092621779,-242.083416999999));
#206778=CARTESIAN_POINT('Ctrl Pts',(-76.9783876018632,3.51420554414337,
-235.35005));
#206779=CARTESIAN_POINT('Ctrl Pts',(-79.1117869535586,-8.58172225549588,
-228.683350000001));
#206780=CARTESIAN_POINT('Ctrl Pts',(-81.2425670238464,-20.6824055590965,
-222.016650000001));
#206781=CARTESIAN_POINT('Ctrl Pts',(-83.3707452702016,-32.7878473303725,
-215.349950000001));
#206782=CARTESIAN_POINT('Ctrl Pts',(-83.3920270526652,-32.9089017480852,
-215.283283000001));
#206783=CARTESIAN_POINT('Ctrl Pts',(-83.4133088351287,-33.0299561657981,
-215.216616));
#206784=CARTESIAN_POINT('Ctrl Pts',(-83.4345906175922,-33.1510105835108,
-215.149949000001));
#206785=CARTESIAN_POINT('Ctrl Pts',(-63.5167278223608,340.899263543393,
-376.750756999979));
#206786=CARTESIAN_POINT('Ctrl Pts',(-68.8258365507552,280.970060093418,
-349.817288999983));
#206787=CARTESIAN_POINT('Ctrl Pts',(-74.1349452791495,221.040856643441,
-322.883820999986));
#206788=CARTESIAN_POINT('Ctrl Pts',(-79.4440540075439,161.111653193465,
-295.950352999991));
#206789=CARTESIAN_POINT('Ctrl Pts',(-82.098608371741,131.147051468477,-282.483618999993));
#206790=CARTESIAN_POINT('Ctrl Pts',(-84.7531627359382,101.182449743489,
-269.016884999995));
#206791=CARTESIAN_POINT('Ctrl Pts',(-87.4077171001354,71.2178480185007,
-255.550150999997));
#206792=CARTESIAN_POINT('Ctrl Pts',(-88.734994282234,56.2355471560066,-248.816783999998));
#206793=CARTESIAN_POINT('Ctrl Pts',(-90.0622714643326,41.2532462935126,
-242.083416999999));
#206794=CARTESIAN_POINT('Ctrl Pts',(-91.3895486464312,26.2709454310185,
-235.35005));
#206795=CARTESIAN_POINT('Ctrl Pts',(-92.7036844702911,11.4369841810244,
-228.683350000001));
#206796=CARTESIAN_POINT('Ctrl Pts',(-94.0136504714512,-3.40424017771396,
-222.016650000001));
#206797=CARTESIAN_POINT('Ctrl Pts',(-95.3194733289638,-18.252732391378,
-215.349950000001));
#206798=CARTESIAN_POINT('Ctrl Pts',(-95.3325315575389,-18.4012173135146,
-215.283283000001));
#206799=CARTESIAN_POINT('Ctrl Pts',(-95.345589786114,-18.5497022356513,
-215.216616000001));
#206800=CARTESIAN_POINT('Ctrl Pts',(-95.3586480146891,-18.698187157788,
-215.149949000001));
#206801=CARTESIAN_POINT('Ctrl Pts',(-95.3044682923166,421.729692912295,
-376.750756999971));
#206802=CARTESIAN_POINT('Ctrl Pts',(-97.3037523682561,350.738834322885,
-349.817288999976));
#206803=CARTESIAN_POINT('Ctrl Pts',(-99.3030364441956,279.747975733475,
-322.883820999982));
#206804=CARTESIAN_POINT('Ctrl Pts',(-101.302320520135,208.757117144065,
-295.950352999988));
#206805=CARTESIAN_POINT('Ctrl Pts',(-102.301962558105,173.261687849361,
-282.48361899999));
#206806=CARTESIAN_POINT('Ctrl Pts',(-103.301604596075,137.766258554656,
-269.016884999993));
#206807=CARTESIAN_POINT('Ctrl Pts',(-104.301246634044,102.270829259951,
-255.550150999996));
#206808=CARTESIAN_POINT('Ctrl Pts',(-104.801067653029,84.5231146125986,
-248.816783999998));
#206809=CARTESIAN_POINT('Ctrl Pts',(-105.300888672014,66.7753999652462,
-242.083416999998));
#206810=CARTESIAN_POINT('Ctrl Pts',(-105.800709690999,49.0276853178937,
-235.35005));
#206811=CARTESIAN_POINT('Ctrl Pts',(-106.295581987024,31.4556906175448,
-228.683350000001));
#206812=CARTESIAN_POINT('Ctrl Pts',(-106.784733919056,13.8739252036685,
-222.016650000002));
#206813=CARTESIAN_POINT('Ctrl Pts',(-107.268201387726,-3.71761745238349,
-215.349950000002));
#206814=CARTESIAN_POINT('Ctrl Pts',(-107.273036062413,-3.89353287894403,
-215.283283000002));
#206815=CARTESIAN_POINT('Ctrl Pts',(-107.277870737099,-4.06944830550458,
-215.216616000002));
#206816=CARTESIAN_POINT('Ctrl Pts',(-107.282705411786,-4.24536373206513,
-215.149949000001));
#206817=CARTESIAN_POINT('Ctrl Pts',(-190.667689702184,664.220981018999,
-376.750756999951));
#206818=CARTESIAN_POINT('Ctrl Pts',(-182.737499820759,560.045157011288,
-349.81728899996));
#206819=CARTESIAN_POINT('Ctrl Pts',(-174.807309939334,455.869333003578,
-322.883820999969));
#206820=CARTESIAN_POINT('Ctrl Pts',(-166.877120057909,351.693508995868,
-295.950352999979));
#206821=CARTESIAN_POINT('Ctrl Pts',(-162.912025117196,299.605596992013,
-282.483618999983));
#206822=CARTESIAN_POINT('Ctrl Pts',(-158.946930176484,247.517684988157,
-269.016884999988));
#206823=CARTESIAN_POINT('Ctrl Pts',(-154.981835235771,195.429772984302,
-255.550150999993));
#206824=CARTESIAN_POINT('Ctrl Pts',(-152.999287765415,169.385816982375,
-248.816783999995));
#206825=CARTESIAN_POINT('Ctrl Pts',(-151.016740295059,143.341860980447,
-242.083416999997));
#206826=CARTESIAN_POINT('Ctrl Pts',(-149.034192824703,117.297904978519,
-235.35005));
#206827=CARTESIAN_POINT('Ctrl Pts',(-147.071274537221,91.5118099271058,
-228.683350000003));
#206828=CARTESIAN_POINT('Ctrl Pts',(-145.09798426187,65.708421347816,-222.016650000002));
#206829=CARTESIAN_POINT('Ctrl Pts',(-143.114385564013,39.8877273646,-215.349950000003));
#206830=CARTESIAN_POINT('Ctrl Pts',(-143.094549577034,39.6295204247678,
-215.283283000003));
#206831=CARTESIAN_POINT('Ctrl Pts',(-143.074713590055,39.3713134849356,
-215.216616000002));
#206832=CARTESIAN_POINT('Ctrl Pts',(-143.054877603077,39.1131065451034,
-215.149949000002));
#206833=CARTESIAN_POINT('Ctrl Pts',(-286.030911112051,906.712269125702,
-376.750756999929));
#206834=CARTESIAN_POINT('Ctrl Pts',(-268.171247273262,769.351479699691,
-349.817288999943));
#206835=CARTESIAN_POINT('Ctrl Pts',(-250.311583434473,631.990690273681,
-322.883820999956));
#206836=CARTESIAN_POINT('Ctrl Pts',(-232.451919595683,494.62990084767,-295.95035299997));
#206837=CARTESIAN_POINT('Ctrl Pts',(-223.522087676288,425.949506134664,
-282.483618999976));
#206838=CARTESIAN_POINT('Ctrl Pts',(-214.592255756894,357.269111421658,
-269.016884999983));
#206839=CARTESIAN_POINT('Ctrl Pts',(-205.662423837499,288.588716708654,
-255.55015099999));
#206840=CARTESIAN_POINT('Ctrl Pts',(-201.197507877801,254.24851935215,-248.816783999994));
#206841=CARTESIAN_POINT('Ctrl Pts',(-196.732591918104,219.908321995647,
-242.083416999997));
#206842=CARTESIAN_POINT('Ctrl Pts',(-192.267675958407,185.568124639145,
-235.35005));
#206843=CARTESIAN_POINT('Ctrl Pts',(-187.846967087419,151.567929236667,
-228.683350000004));
#206844=CARTESIAN_POINT('Ctrl Pts',(-183.411234604685,117.542917491964,
-222.016650000003));
#206845=CARTESIAN_POINT('Ctrl Pts',(-178.960569740299,83.4930721815835,
-215.349950000004));
#206846=CARTESIAN_POINT('Ctrl Pts',(-178.916063091656,83.1525737284796,
-215.283283000004));
#206847=CARTESIAN_POINT('Ctrl Pts',(-178.871556443012,82.8120752753758,
-215.216616000004));
#206848=CARTESIAN_POINT('Ctrl Pts',(-178.827049794367,82.4715768222719,
-215.149949000004));
#206849=CARTESIAN_POINT('Ctrl Pts',(-381.394132521918,1149.20355723241,
-376.750756999909));
#206850=CARTESIAN_POINT('Ctrl Pts',(-353.604994725765,978.657802388094,
-349.817288999926));
#206851=CARTESIAN_POINT('Ctrl Pts',(-325.815856929611,808.112047543783,
-322.883820999944));
#206852=CARTESIAN_POINT('Ctrl Pts',(-298.026719133457,637.566292699472,
-295.950352999961));
#206853=CARTESIAN_POINT('Ctrl Pts',(-284.13215023538,552.293415277316,-282.48361899997));
#206854=CARTESIAN_POINT('Ctrl Pts',(-270.237581337303,467.02053785516,-269.016884999978));
#206855=CARTESIAN_POINT('Ctrl Pts',(-256.343012439226,381.747660433005,
-255.550150999987));
#206856=CARTESIAN_POINT('Ctrl Pts',(-249.395727990188,339.111221721927,
-248.816783999992));
#206857=CARTESIAN_POINT('Ctrl Pts',(-242.448443541149,296.474783010849,
-242.083416999996));
#206858=CARTESIAN_POINT('Ctrl Pts',(-235.501159092111,253.83834429977,-235.35005));
#206859=CARTESIAN_POINT('Ctrl Pts',(-228.622659637617,211.624048546228,
-228.683350000005));
#206860=CARTESIAN_POINT('Ctrl Pts',(-221.724484947499,169.377413636111,
-222.016650000005));
#206861=CARTESIAN_POINT('Ctrl Pts',(-214.806753916586,127.098416998567,
-215.349950000004));
#206862=CARTESIAN_POINT('Ctrl Pts',(-214.737576606277,126.675627032191,
-215.283283000005));
#206863=CARTESIAN_POINT('Ctrl Pts',(-214.668399295968,126.252837065816,
-215.216616000005));
#206864=CARTESIAN_POINT('Ctrl Pts',(-214.599221985659,125.83004709944,-215.149949000005));
#206865=CARTESIAN_POINT('Ctrl Pts',(-667.483796751521,1876.67742155251,
-376.750756999846));
#206866=CARTESIAN_POINT('Ctrl Pts',(-609.906237083273,1606.57677045331,
-349.817288999875));
#206867=CARTESIAN_POINT('Ctrl Pts',(-552.328677415026,1336.47611935409,
-322.883820999905));
#206868=CARTESIAN_POINT('Ctrl Pts',(-494.751117746779,1066.37546825488,
-295.950352999934));
#206869=CARTESIAN_POINT('Ctrl Pts',(-465.962337912655,931.325142705271,
-282.483618999949));
#206870=CARTESIAN_POINT('Ctrl Pts',(-437.173558078531,796.274817155664,
-269.016884999963));
#206871=CARTESIAN_POINT('Ctrl Pts',(-408.384778244408,661.224491606058,
-255.550150999978));
#206872=CARTESIAN_POINT('Ctrl Pts',(-393.990388327346,593.699328831254,
-248.816783999986));
#206873=CARTESIAN_POINT('Ctrl Pts',(-379.595998410284,526.174166056451,
-242.083416999993));
#206874=CARTESIAN_POINT('Ctrl Pts',(-365.201608493222,458.649003281647,
-235.35005));
#206875=CARTESIAN_POINT('Ctrl Pts',(-350.94973728821,391.792406474911,-228.683350000008));
#206876=CARTESIAN_POINT('Ctrl Pts',(-336.664235975943,324.880902068554,
-222.016650000008));
#206877=CARTESIAN_POINT('Ctrl Pts',(-322.345306445446,257.914451449517,
-215.349950000008));
#206878=CARTESIAN_POINT('Ctrl Pts',(-322.202117150141,257.244786943327,
-215.283283000008));
#206879=CARTESIAN_POINT('Ctrl Pts',(-322.058927854835,256.575122437136,
-215.216616000008));
#206880=CARTESIAN_POINT('Ctrl Pts',(-321.91573855953,255.905457930946,-215.149949000007));
#206881=CARTESIAN_POINT('Ctrl Pts',(-953.573460981123,2604.15128587263,
-376.750756999783));
#206882=CARTESIAN_POINT('Ctrl Pts',(-866.207479440782,2234.49573851851,
-349.817288999824));
#206883=CARTESIAN_POINT('Ctrl Pts',(-778.841497900441,1864.8401911644,-322.883820999866));
#206884=CARTESIAN_POINT('Ctrl Pts',(-691.4755163601,1495.18464381028,-295.950352999906));
#206885=CARTESIAN_POINT('Ctrl Pts',(-647.79252558993,1310.35687013323,-282.483618999927));
#206886=CARTESIAN_POINT('Ctrl Pts',(-604.109534819759,1125.52909645617,
-269.016884999948));
#206887=CARTESIAN_POINT('Ctrl Pts',(-560.426544049589,940.701322779111,
-255.550150999969));
#206888=CARTESIAN_POINT('Ctrl Pts',(-538.585048664503,848.287435940582,
-248.81678399998));
#206889=CARTESIAN_POINT('Ctrl Pts',(-516.743553279418,755.873549102053,
-242.08341699999));
#206890=CARTESIAN_POINT('Ctrl Pts',(-494.902057894333,663.459662263524,
-235.35005));
#206891=CARTESIAN_POINT('Ctrl Pts',(-473.276814938803,571.960764403594,
-228.683350000011));
#206892=CARTESIAN_POINT('Ctrl Pts',(-451.603987004386,480.384390500996,
-222.016650000011));
#206893=CARTESIAN_POINT('Ctrl Pts',(-429.883858974306,388.730485900468,
-215.34995000001));
#206894=CARTESIAN_POINT('Ctrl Pts',(-429.666657694005,387.813946854463,
-215.28328300001));
#206895=CARTESIAN_POINT('Ctrl Pts',(-429.449456413704,386.897407808457,
-215.216616000011));
#206896=CARTESIAN_POINT('Ctrl Pts',(-429.232255133403,385.980868762451,
-215.149949000011));
#206897=CARTESIAN_POINT('Ctrl Pts',(-1239.66312521072,3331.62515019274,
-376.750756999719));
#206898=CARTESIAN_POINT('Ctrl Pts',(-1122.50872179829,2862.41470658373,
-349.817288999773));
#206899=CARTESIAN_POINT('Ctrl Pts',(-1005.35431838586,2393.20426297471,
-322.883820999826));
#206900=CARTESIAN_POINT('Ctrl Pts',(-888.199914973422,1923.99381936569,
-295.95035299988));
#206901=CARTESIAN_POINT('Ctrl Pts',(-829.622713267204,1689.38859756118,
-282.483618999906));
#206902=CARTESIAN_POINT('Ctrl Pts',(-771.045511560987,1454.78337575667,
-269.016884999933));
#206903=CARTESIAN_POINT('Ctrl Pts',(-712.46830985477,1220.17815395216,-255.55015099996));
#206904=CARTESIAN_POINT('Ctrl Pts',(-683.179709001661,1102.87554304991,
-248.816783999974));
#206905=CARTESIAN_POINT('Ctrl Pts',(-653.891108148553,985.572932147655,
-242.083416999987));
#206906=CARTESIAN_POINT('Ctrl Pts',(-624.602507295445,868.2703212454,-235.35005));
#206907=CARTESIAN_POINT('Ctrl Pts',(-595.603892589396,752.129122332277,
-228.683350000014));
#206908=CARTESIAN_POINT('Ctrl Pts',(-566.54373803283,635.887878933439,-222.016650000014));
#206909=CARTESIAN_POINT('Ctrl Pts',(-537.422411503166,519.546520351418,
-215.349950000014));
#206910=CARTESIAN_POINT('Ctrl Pts',(-537.131198237869,518.383106765598,
-215.283283000013));
#206911=CARTESIAN_POINT('Ctrl Pts',(-536.839984972572,517.219693179777,
-215.216616000014));
#206912=CARTESIAN_POINT('Ctrl Pts',(-536.548771707275,516.056279593957,
-215.149949000014));
#206913=CARTESIAN_POINT('Ctrl Pts',(-2097.93211789953,5514.04674315307,
-376.750756999531));
#206914=CARTESIAN_POINT('Ctrl Pts',(-1891.41244887082,4746.17161077935,
-349.81728899962));
#206915=CARTESIAN_POINT('Ctrl Pts',(-1684.8927798421,3978.29647840563,-322.88382099971));
#206916=CARTESIAN_POINT('Ctrl Pts',(-1478.37311081339,3210.42134603191,
-295.950352999799));
#206917=CARTESIAN_POINT('Ctrl Pts',(-1375.11327629903,2826.48377984504,
-282.483618999843));
#206918=CARTESIAN_POINT('Ctrl Pts',(-1271.85344178467,2442.54621365819,
-269.016884999889));
#206919=CARTESIAN_POINT('Ctrl Pts',(-1168.59360727031,2058.60864747133,
-255.550150999933));
#206920=CARTESIAN_POINT('Ctrl Pts',(-1116.96369001313,1866.6398643779,-248.816783999956));
#206921=CARTESIAN_POINT('Ctrl Pts',(-1065.33377275596,1674.67108128446,
-242.083416999977));
#206922=CARTESIAN_POINT('Ctrl Pts',(-1013.70385549878,1482.70229819103,
-235.35005));
#206923=CARTESIAN_POINT('Ctrl Pts',(-962.585125541175,1292.63419611833,
-228.683350000023));
#206924=CARTESIAN_POINT('Ctrl Pts',(-911.362991118159,1102.39834423077,
-222.016650000023));
#206925=CARTESIAN_POINT('Ctrl Pts',(-860.038069089746,911.99462370427,-215.349950000023));
#206926=CARTESIAN_POINT('Ctrl Pts',(-859.524819869462,910.090586499004,
-215.283283000022));
#206927=CARTESIAN_POINT('Ctrl Pts',(-859.011570649176,908.186549293739,
-215.216616000022));
#206928=CARTESIAN_POINT('Ctrl Pts',(-858.498321428892,906.282512088474,
-215.149949000023));
#206929=CARTESIAN_POINT('Ctrl Pts',(-2956.20111058834,7696.4683361134,-376.750756999341));
#206930=CARTESIAN_POINT('Ctrl Pts',(-2660.31617594335,6629.92851497498,
-349.817288999467));
#206931=CARTESIAN_POINT('Ctrl Pts',(-2364.43124129834,5563.38869383655,
-322.883820999593));
#206932=CARTESIAN_POINT('Ctrl Pts',(-2068.54630665335,4496.84887269812,
-295.950352999718));
#206933=CARTESIAN_POINT('Ctrl Pts',(-1920.60383933086,3963.57896212891,
-282.48361899978));
#206934=CARTESIAN_POINT('Ctrl Pts',(-1772.66137200836,3430.3090515597,-269.016884999844));
#206935=CARTESIAN_POINT('Ctrl Pts',(-1624.71890468586,2897.03914099049,
-255.550150999906));
#206936=CARTESIAN_POINT('Ctrl Pts',(-1550.74767102461,2630.40418570588,
-248.816783999938));
#206937=CARTESIAN_POINT('Ctrl Pts',(-1476.77643736336,2363.76923042127,
-242.083416999969));
#206938=CARTESIAN_POINT('Ctrl Pts',(-1402.80520370211,2097.13427513666,
-235.35005));
#206939=CARTESIAN_POINT('Ctrl Pts',(-1329.56635849295,1833.13926990437,
-228.683350000032));
#206940=CARTESIAN_POINT('Ctrl Pts',(-1256.18224420349,1568.9088095281,-222.016650000032));
#206941=CARTESIAN_POINT('Ctrl Pts',(-1182.65372667633,1304.44272705712,
-215.349950000032));
#206942=CARTESIAN_POINT('Ctrl Pts',(-1181.91844150105,1301.79806623241,
-215.283283000032));
#206943=CARTESIAN_POINT('Ctrl Pts',(-1181.18315632578,1299.1534054077,-215.216616000032));
#206944=CARTESIAN_POINT('Ctrl Pts',(-1180.44787115051,1296.50874458299,
-215.149949000032));
#206945=CARTESIAN_POINT('Ctrl Pts',(-3814.47010327714,9878.88992907374,
-376.750756999153));
#206946=CARTESIAN_POINT('Ctrl Pts',(-3429.21990301587,8513.68541917061,
-349.817288999315));
#206947=CARTESIAN_POINT('Ctrl Pts',(-3043.96970275459,7148.48090926748,
-322.883820999476));
#206948=CARTESIAN_POINT('Ctrl Pts',(-2658.71950249332,5783.27639936434,
-295.950352999637));
#206949=CARTESIAN_POINT('Ctrl Pts',(-2466.09440236268,5100.67414441278,
-282.483618999717));
#206950=CARTESIAN_POINT('Ctrl Pts',(-2273.46930223204,4418.07188946121,
-269.016884999799));
#206951=CARTESIAN_POINT('Ctrl Pts',(-2080.84420210141,3735.46963450965,
-255.550150999879));
#206952=CARTESIAN_POINT('Ctrl Pts',(-1984.53165203609,3394.16850703386,
-248.81678399992));
#206953=CARTESIAN_POINT('Ctrl Pts',(-1888.21910197076,3052.86737955808,
-242.08341699996));
#206954=CARTESIAN_POINT('Ctrl Pts',(-1791.90655190545,2711.56625208229,
-235.35005));
#206955=CARTESIAN_POINT('Ctrl Pts',(-1696.54759144473,2373.64434369042,
-228.683350000041));
#206956=CARTESIAN_POINT('Ctrl Pts',(-1601.00149728882,2035.41927482542,
-222.016650000041));
#206957=CARTESIAN_POINT('Ctrl Pts',(-1505.26938426291,1696.89083040998,
-215.349950000041));
#206958=CARTESIAN_POINT('Ctrl Pts',(-1504.31206313264,1693.50554596582,
-215.28328300004));
#206959=CARTESIAN_POINT('Ctrl Pts',(-1503.35474200239,1690.12026152166,
-215.216616000041));
#206960=CARTESIAN_POINT('Ctrl Pts',(-1502.39742087213,1686.7349770775,-215.149949000041));
#206961=CARTESIAN_POINT('Origin',(636.934816028482,-11.5034818258361,-229.35005));
#206962=CARTESIAN_POINT('Origin',(636.934816028482,-11.5034818258361,-229.35005));
#206963=CARTESIAN_POINT('Origin',(636.934816028482,-11.5034818258361,-229.35005));
#206964=CARTESIAN_POINT('Origin',(636.934816028482,-11.5034818258361,-229.35005));
#206965=CARTESIAN_POINT('Origin',(636.934816028482,-11.5034818258361,-229.35005));
#206966=CARTESIAN_POINT('Origin',(636.934816028482,-11.5034818258361,-229.35005));
#206967=CARTESIAN_POINT('Origin',(636.934816028482,-11.5034818258361,-229.35005));
#206968=CARTESIAN_POINT('Origin',(636.934816028482,-11.5034818258361,-229.35005));
#206969=CARTESIAN_POINT('Origin',(636.934816028482,-11.5034818258361,-229.35005));
#206970=CARTESIAN_POINT('Origin',(636.934816028482,-11.5034818258361,-229.35005));
#206971=CARTESIAN_POINT('Origin',(0.,-32.21456093117,-229.35005));
#206972=CARTESIAN_POINT('',(0.,-32.21456093117,-229.35005));
#206973=CARTESIAN_POINT('Origin',(0.,-33.21456093117,-229.35005));
#206974=CARTESIAN_POINT('',(0.,-33.21456093117,-229.35005));
#206975=CARTESIAN_POINT('Origin',(2.22174260618994E-13,-11.0034818258363,
-229.35005));
#206976=CARTESIAN_POINT('',(2.22174260618994E-13,-11.0034818258363,-229.35005));
#206977=CARTESIAN_POINT('Origin',(2.22174260618994E-13,-12.0034818258363,
-229.35005));
#206978=CARTESIAN_POINT('',(2.22174260618994E-13,-12.0034818258363,-229.35005));
#206979=CARTESIAN_POINT('Origin',(1.54373336646987E-15,-42.8201004838369,
-229.35005));
#206980=CARTESIAN_POINT('',(1.54373336646987E-15,-42.8201004838369,-229.35005));
#206981=CARTESIAN_POINT('Origin',(1.23757166668304E-15,-43.8201004838368,
-229.35005));
#206982=CARTESIAN_POINT('',(1.23757166668304E-15,-43.8201004838368,-229.35005));
#206983=CARTESIAN_POINT('Origin',(2.8425373731103E-15,9.20759727949731,
-229.35005));
#206984=CARTESIAN_POINT('',(2.8425373731103E-15,9.20759727949731,-229.35005));
#206985=CARTESIAN_POINT('Origin',(2.53637567332344E-15,10.2075972794973,
-229.35005));
#206986=CARTESIAN_POINT('',(2.53637567332344E-15,10.2075972794973,-229.35005));
#206987=CARTESIAN_POINT('Origin',(1.54373336646988E-15,19.8131368321642,
-229.35005));
#206988=CARTESIAN_POINT('',(1.54373336646988E-15,19.8131368321642,-229.35005));
#206989=CARTESIAN_POINT('Origin',(1.23757166668304E-15,20.8131368321642,
-229.35005));
#206990=CARTESIAN_POINT('',(1.23757166668304E-15,20.8131368321642,-229.35005));
#206991=CARTESIAN_POINT('Origin',(2.61456814389029E-14,-173.57701443073,
-229.35005));
#206992=CARTESIAN_POINT('Origin',(2.61456814389029E-14,-173.57701443073,
-229.35005));
#206993=CARTESIAN_POINT('Origin',(-7.14692237356698E-14,623.509175991979,
-229.35005));
#206994=CARTESIAN_POINT('Origin',(-7.14692237356698E-14,623.509175991979,
-229.35005));
#206995=CARTESIAN_POINT('Origin',(2.61456814389029E-14,-173.57701443073,
-229.35005));
#206996=CARTESIAN_POINT('Origin',(2.61456814389029E-14,-173.57701443073,
-232.25005));
#206997=CARTESIAN_POINT('Origin',(2.61456814389029E-14,-173.57701443073,
-229.35005));
#206998=CARTESIAN_POINT('Origin',(0.,-32.21456093117,-229.35005));
#206999=CARTESIAN_POINT('',(0.,-32.21456093117,-229.35005));
#207000=CARTESIAN_POINT('Origin',(0.,-33.21456093117,-229.35005));
#207001=CARTESIAN_POINT('',(0.,-33.21456093117,-229.35005));
#207002=CARTESIAN_POINT('Origin',(3.33261390928491E-13,-21.6090213785032,
-229.35005));
#207003=CARTESIAN_POINT('',(3.33261390928491E-13,-21.6090213785032,-229.35005));
#207004=CARTESIAN_POINT('Origin',(3.33261390928491E-13,-22.6090213785032,
-229.35005));
#207005=CARTESIAN_POINT('',(3.33261390928491E-13,-22.6090213785032,-229.35005));
#207006=CARTESIAN_POINT('Origin',(2.22174260618994E-13,-11.0034818258363,
-229.35005));
#207007=CARTESIAN_POINT('',(2.22174260618994E-13,-11.0034818258363,-229.35005));
#207008=CARTESIAN_POINT('Origin',(2.22174260618994E-13,-12.0034818258363,
-229.35005));
#207009=CARTESIAN_POINT('',(2.22174260618994E-13,-12.0034818258363,-229.35005));
#207010=CARTESIAN_POINT('Origin',(1.11087130309497E-13,-0.397942273169518,
-229.35005));
#207011=CARTESIAN_POINT('',(1.11087130309497E-13,-0.397942273169518,-229.35005));
#207012=CARTESIAN_POINT('Origin',(1.11087130309497E-13,-1.3979422731695,
-229.35005));
#207013=CARTESIAN_POINT('',(1.11087130309497E-13,-1.3979422731695,-229.35005));
#207014=CARTESIAN_POINT('Origin',(1.54373336646987E-15,-42.8201004838369,
-229.35005));
#207015=CARTESIAN_POINT('',(1.54373336646987E-15,-42.8201004838369,-229.35005));
#207016=CARTESIAN_POINT('Origin',(1.23757166668304E-15,-43.8201004838368,
-229.35005));
#207017=CARTESIAN_POINT('',(1.23757166668304E-15,-43.8201004838368,-229.35005));
#207018=CARTESIAN_POINT('Origin',(2.8425373731103E-15,9.20759727949731,
-229.35005));
#207019=CARTESIAN_POINT('',(2.8425373731103E-15,9.20759727949731,-229.35005));
#207020=CARTESIAN_POINT('Origin',(2.53637567332344E-15,10.2075972794973,
-229.35005));
#207021=CARTESIAN_POINT('',(2.53637567332344E-15,10.2075972794973,-229.35005));
#207022=CARTESIAN_POINT('Origin',(1.54373336646988E-15,19.8131368321642,
-229.35005));
#207023=CARTESIAN_POINT('',(1.54373336646988E-15,19.8131368321642,-229.35005));
#207024=CARTESIAN_POINT('Origin',(1.23757166668304E-15,20.8131368321642,
-229.35005));
#207025=CARTESIAN_POINT('',(1.23757166668304E-15,20.8131368321642,-229.35005));
#207026=CARTESIAN_POINT('Origin',(2.61456814389029E-14,-173.57701443073,
-229.35005));
#207027=CARTESIAN_POINT('Origin',(2.61456814389029E-14,-173.57701443073,
-229.35005));
#207028=CARTESIAN_POINT('Origin',(2.61456814389029E-14,-173.57701443073,
-229.35005));
#207029=CARTESIAN_POINT('Origin',(2.61456814389029E-14,-173.57701443073,
-229.35005));
#207030=CARTESIAN_POINT('Origin',(-7.14692237356698E-14,623.509175991979,
-229.35005));
#207031=CARTESIAN_POINT('Origin',(-7.14692237356698E-14,623.509175991979,
-229.35005));
#207032=CARTESIAN_POINT('Origin',(-7.14692237356698E-14,623.509175991979,
-229.35005));
#207033=CARTESIAN_POINT('Origin',(-7.14692237356698E-14,623.509175991979,
-229.35005));
#207034=CARTESIAN_POINT('Origin',(6.29739814579425E-15,-11.5034818258363,
-229.35005));
#207035=CARTESIAN_POINT('Origin',(6.29739814579425E-15,-11.5034818258363,
-229.35005));
#207036=CARTESIAN_POINT('Origin',(6.29739814579425E-15,-11.5034818258363,
-229.35005));
#207037=CARTESIAN_POINT('Origin',(6.29739814579425E-15,-11.5034818258363,
-229.35005));
#207038=CARTESIAN_POINT('Origin',(6.29739814579425E-15,-11.5034818258363,
-229.35005));
#207039=CARTESIAN_POINT('Origin',(6.29739814579425E-15,-11.5034818258363,
-229.35005));
#207040=CARTESIAN_POINT('Origin',(6.29739814579425E-15,-11.5034818258363,
-229.35005));
#207041=CARTESIAN_POINT('Origin',(6.29739814579425E-15,-11.5034818258363,
-229.35005));
#207042=CARTESIAN_POINT('Origin',(0.,-32.21456093117,-229.35005));
#207043=CARTESIAN_POINT('',(0.,-32.21456093117,-229.35005));
#207044=CARTESIAN_POINT('Origin',(0.,-32.21456093117,-229.35005));
#207045=CARTESIAN_POINT('',(0.,-32.21456093117,-229.35005));
#207046=CARTESIAN_POINT('Origin',(0.,-33.21456093117,-229.35005));
#207047=CARTESIAN_POINT('',(0.,-33.21456093117,-229.35005));
#207048=CARTESIAN_POINT('Origin',(0.,-33.21456093117,-229.35005));
#207049=CARTESIAN_POINT('',(0.,-33.21456093117,-229.35005));
#207050=CARTESIAN_POINT('Origin',(3.33261390928491E-13,-21.6090213785032,
-229.35005));
#207051=CARTESIAN_POINT('',(3.33261390928491E-13,-21.6090213785032,-229.35005));
#207052=CARTESIAN_POINT('Origin',(3.33261390928491E-13,-21.6090213785032,
-229.35005));
#207053=CARTESIAN_POINT('',(3.33261390928491E-13,-21.6090213785032,-229.35005));
#207054=CARTESIAN_POINT('Origin',(3.33261390928491E-13,-22.6090213785032,
-229.35005));
#207055=CARTESIAN_POINT('',(3.33261390928491E-13,-22.6090213785032,-229.35005));
#207056=CARTESIAN_POINT('Origin',(3.33261390928491E-13,-22.6090213785032,
-229.35005));
#207057=CARTESIAN_POINT('',(3.33261390928491E-13,-22.6090213785032,-229.35005));
#207058=CARTESIAN_POINT('Origin',(2.22174260618994E-13,-11.0034818258363,
-229.35005));
#207059=CARTESIAN_POINT('',(2.22174260618994E-13,-11.0034818258363,-229.35005));
#207060=CARTESIAN_POINT('Origin',(2.22174260618994E-13,-11.0034818258363,
-229.35005));
#207061=CARTESIAN_POINT('',(2.22174260618994E-13,-11.0034818258363,-229.35005));
#207062=CARTESIAN_POINT('Origin',(2.22174260618994E-13,-12.0034818258363,
-229.35005));
#207063=CARTESIAN_POINT('',(2.22174260618994E-13,-12.0034818258363,-229.35005));
#207064=CARTESIAN_POINT('Origin',(2.22174260618994E-13,-12.0034818258363,
-229.35005));
#207065=CARTESIAN_POINT('',(2.22174260618994E-13,-12.0034818258363,-229.35005));
#207066=CARTESIAN_POINT('Origin',(1.11087130309497E-13,-0.397942273169518,
-229.35005));
#207067=CARTESIAN_POINT('',(1.11087130309497E-13,-0.397942273169518,-229.35005));
#207068=CARTESIAN_POINT('Origin',(1.11087130309497E-13,-0.397942273169518,
-229.35005));
#207069=CARTESIAN_POINT('',(1.11087130309497E-13,-0.397942273169518,-229.35005));
#207070=CARTESIAN_POINT('Origin',(1.11087130309497E-13,-1.3979422731695,
-229.35005));
#207071=CARTESIAN_POINT('',(1.11087130309497E-13,-1.3979422731695,-229.35005));
#207072=CARTESIAN_POINT('Origin',(1.11087130309497E-13,-1.3979422731695,
-229.35005));
#207073=CARTESIAN_POINT('',(1.11087130309497E-13,-1.3979422731695,-229.35005));
#207074=CARTESIAN_POINT('Origin',(1.54373336646987E-15,-42.8201004838369,
-229.35005));
#207075=CARTESIAN_POINT('',(1.54373336646987E-15,-42.8201004838369,-229.35005));
#207076=CARTESIAN_POINT('Origin',(1.54373336646987E-15,-42.8201004838369,
-229.35005));
#207077=CARTESIAN_POINT('',(1.54373336646987E-15,-42.8201004838369,-229.35005));
#207078=CARTESIAN_POINT('Origin',(1.23757166668304E-15,-43.8201004838368,
-229.35005));
#207079=CARTESIAN_POINT('',(1.23757166668304E-15,-43.8201004838368,-229.35005));
#207080=CARTESIAN_POINT('Origin',(1.23757166668304E-15,-43.8201004838368,
-229.35005));
#207081=CARTESIAN_POINT('',(1.23757166668304E-15,-43.8201004838368,-229.35005));
#207082=CARTESIAN_POINT('Origin',(2.8425373731103E-15,9.20759727949731,
-229.35005));
#207083=CARTESIAN_POINT('',(2.8425373731103E-15,9.20759727949731,-229.35005));
#207084=CARTESIAN_POINT('Origin',(2.8425373731103E-15,9.20759727949731,
-229.35005));
#207085=CARTESIAN_POINT('',(2.8425373731103E-15,9.20759727949731,-229.35005));
#207086=CARTESIAN_POINT('Origin',(2.53637567332344E-15,10.2075972794973,
-229.35005));
#207087=CARTESIAN_POINT('',(2.53637567332344E-15,10.2075972794973,-229.35005));
#207088=CARTESIAN_POINT('Origin',(2.53637567332344E-15,10.2075972794973,
-229.35005));
#207089=CARTESIAN_POINT('',(2.53637567332344E-15,10.2075972794973,-229.35005));
#207090=CARTESIAN_POINT('Origin',(1.54373336646988E-15,19.8131368321642,
-229.35005));
#207091=CARTESIAN_POINT('',(1.54373336646988E-15,19.8131368321642,-229.35005));
#207092=CARTESIAN_POINT('Origin',(1.54373336646988E-15,19.8131368321642,
-229.35005));
#207093=CARTESIAN_POINT('',(1.54373336646988E-15,19.8131368321642,-229.35005));
#207094=CARTESIAN_POINT('Origin',(1.23757166668304E-15,20.8131368321642,
-229.35005));
#207095=CARTESIAN_POINT('',(1.23757166668304E-15,20.8131368321642,-229.35005));
#207096=CARTESIAN_POINT('Origin',(1.23757166668304E-15,20.8131368321642,
-229.35005));
#207097=CARTESIAN_POINT('',(1.23757166668304E-15,20.8131368321642,-229.35005));
#207098=CARTESIAN_POINT('Ctrl Pts',(51.7233397168138,38.3762252975093,-227.858776203219));
#207099=CARTESIAN_POINT('Ctrl Pts',(51.7302447133037,38.3813101134616,-228.35005));
#207100=CARTESIAN_POINT('Ctrl Pts',(52.1258919562643,38.67266339879,-228.35005));
#207101=CARTESIAN_POINT('Ctrl Pts',(51.6174495896917,38.5200202664566,-227.858776175692));
#207102=CARTESIAN_POINT('Ctrl Pts',(51.6128088111955,38.5425689461205,-228.410692739194));
#207103=CARTESIAN_POINT('Ctrl Pts',(52.0466039743291,38.878041220954,-228.35005));
#207104=CARTESIAN_POINT('Ctrl Pts',(51.5002798258237,38.6559630716119,-227.854887707304));
#207105=CARTESIAN_POINT('Ctrl Pts',(51.5043449566927,38.6663650434491,-228.441452922891));
#207106=CARTESIAN_POINT('Ctrl Pts',(51.9333069568917,39.0542288907298,-228.338384512236));
#207107=CARTESIAN_POINT('Ctrl Pts',(51.247332174135,38.9079983209904,-227.854896823446));
#207108=CARTESIAN_POINT('Ctrl Pts',(51.2577525408945,38.9120667908531,-228.441337182113));
#207109=CARTESIAN_POINT('Ctrl Pts',(51.6439737530735,39.342374196026,-228.3384118607));
#207110=CARTESIAN_POINT('Ctrl Pts',(51.1119650116918,39.023887086559,-227.858776175352));
#207111=CARTESIAN_POINT('Ctrl Pts',(51.1344983277446,39.0193462915006,-228.410782960183));
#207112=CARTESIAN_POINT('Ctrl Pts',(51.4685984426326,39.4543128793957,-228.35005));
#207113=CARTESIAN_POINT('Ctrl Pts',(50.9675450051224,39.1294935022024,-227.858776203219));
#207114=CARTESIAN_POINT('Ctrl Pts',(50.9726066716339,39.136415486161,-228.35005));
#207115=CARTESIAN_POINT('Ctrl Pts',(51.2626335243565,39.533036088795,-228.35005));
#207116=CARTESIAN_POINT('',(52.1258919562641,38.6726633987897,-228.35005));
#207117=CARTESIAN_POINT('',(51.7233397168138,38.3762252975093,-227.858776203219));
#207118=CARTESIAN_POINT('Origin',(52.1258919562641,38.6726633987897,-227.85005));
#207119=CARTESIAN_POINT('',(50.9675450051224,39.1294935022024,-227.858776203219));
#207120=CARTESIAN_POINT('Ctrl Pts',(50.9675450051224,39.1294935022024,-227.858776203219));
#207121=CARTESIAN_POINT('Ctrl Pts',(50.9830880714985,39.1181277118405,-227.858776203219));
#207122=CARTESIAN_POINT('Ctrl Pts',(51.0010148380594,39.1048281103116,-227.858730357654));
#207123=CARTESIAN_POINT('Ctrl Pts',(51.0212177237975,39.0894556321685,-227.85860987035));
#207124=CARTESIAN_POINT('Ctrl Pts',(51.0407951016109,39.0745591061753,-227.858493113492));
#207125=CARTESIAN_POINT('Ctrl Pts',(51.0625096818472,39.0577159016543,-227.858305190088));
#207126=CARTESIAN_POINT('Ctrl Pts',(51.0862346209097,39.0387664781746,-227.858039584716));
#207127=CARTESIAN_POINT('Ctrl Pts',(51.108501017397,39.0209820119935,-227.857790308017));
#207128=CARTESIAN_POINT('Ctrl Pts',(51.1325379340948,39.0013420490696,-227.857471813149));
#207129=CARTESIAN_POINT('Ctrl Pts',(51.1582177288737,38.9796886779462,-227.857109298627));
#207130=CARTESIAN_POINT('Ctrl Pts',(51.164515737183,38.9743781560967,-227.857020391395));
#207131=CARTESIAN_POINT('Ctrl Pts',(51.1709124581292,38.968946412574,-227.8569290201));
#207132=CARTESIAN_POINT('Ctrl Pts',(51.1774058068761,38.9633908868785,-227.85683594779));
#207133=CARTESIAN_POINT('Ctrl Pts',(51.2041328930996,38.9405239471736,-227.856452855527));
#207134=CARTESIAN_POINT('Ctrl Pts',(51.2285321441227,38.9189559026779,-227.856101868042));
#207135=CARTESIAN_POINT('Ctrl Pts',(51.2507490067655,38.8988503544204,-227.85581896922));
#207136=CARTESIAN_POINT('Ctrl Pts',(51.2739503915884,38.8778538451608,-227.855523533967));
#207137=CARTESIAN_POINT('Ctrl Pts',(51.2947718475604,38.8584525160497,-227.855301345718));
#207138=CARTESIAN_POINT('Ctrl Pts',(51.3133513197527,38.8408013282161,-227.855152877392));
#207139=CARTESIAN_POINT('Ctrl Pts',(51.3327688896871,38.8223539164361,-227.854997711837));
#207140=CARTESIAN_POINT('Ctrl Pts',(51.3497378512431,38.8058183365427,-227.854921938072));
#207141=CARTESIAN_POINT('Ctrl Pts',(51.3643831288794,38.7913345616423,-227.854899769182));
#207142=CARTESIAN_POINT('Ctrl Pts',(51.3676380035395,38.788115580543,-227.854894842204));
#207143=CARTESIAN_POINT('Ctrl Pts',(51.370777973267,38.7849977994569,-227.854892502014));
#207144=CARTESIAN_POINT('Ctrl Pts',(51.3738041885888,38.7819825040676,-227.854892383582));
#207145=CARTESIAN_POINT('Ctrl Pts',(51.3738047928673,38.7819819019696,-227.854892383558));
#207146=CARTESIAN_POINT('Ctrl Pts',(51.37380539715,38.7819812998671,-227.854892383534));
#207147=CARTESIAN_POINT('Ctrl Pts',(51.3738060014367,38.78198069776,-227.854892383511));
#207148=CARTESIAN_POINT('Ctrl Pts',(51.3873290404909,38.7685064364501,-227.854891858251));
#207149=CARTESIAN_POINT('Ctrl Pts',(51.4029131555694,38.7527647227732,-227.854936775985));
#207150=CARTESIAN_POINT('Ctrl Pts',(51.4204379639646,38.734631047722,-227.855055719537));
#207151=CARTESIAN_POINT('Ctrl Pts',(51.4373488622628,38.7171326119248,-227.855170496387));
#207152=CARTESIAN_POINT('Ctrl Pts',(51.4560669428818,38.6974064333121,-227.855355226822));
#207153=CARTESIAN_POINT('Ctrl Pts',(51.4764468776254,38.6753178021015,-227.855616531962));
#207154=CARTESIAN_POINT('Ctrl Pts',(51.4954944831492,38.6546732053866,-227.855860754393));
#207155=CARTESIAN_POINT('Ctrl Pts',(51.515993657152,38.6319645100545,-227.856172586645));
#207156=CARTESIAN_POINT('Ctrl Pts',(51.5377932005687,38.6070676878515,-227.856528479526));
#207157=CARTESIAN_POINT('Ctrl Pts',(51.5438321409979,38.600170734861,-227.856627069477));
#207158=CARTESIAN_POINT('Ctrl Pts',(51.5499706739712,38.593105796085,-227.856728824965));
#207159=CARTESIAN_POINT('Ctrl Pts',(51.556205114735,38.58587009375,-227.856832699314));
#207160=CARTESIAN_POINT('Ctrl Pts',(51.5791743717403,38.5592119358101,-227.857215398697));
#207161=CARTESIAN_POINT('Ctrl Pts',(51.6000534221824,38.5341766143175,-227.857566058089));
#207162=CARTESIAN_POINT('Ctrl Pts',(51.6189965727127,38.5109146691511,-227.857848834773));
#207163=CARTESIAN_POINT('Ctrl Pts',(51.6388353321281,38.486552927795,-227.858144980791));
#207164=CARTESIAN_POINT('Ctrl Pts',(51.6565512897508,38.4641361492409,-227.858367658238));
#207165=CARTESIAN_POINT('Ctrl Pts',(51.6723014335466,38.4438000309361,-227.858516309415));
#207166=CARTESIAN_POINT('Ctrl Pts',(51.6888025129355,38.4224943268766,-227.858672047985));
#207167=CARTESIAN_POINT('Ctrl Pts',(51.703146422698,38.4034723566256,-227.858747661482));
#207168=CARTESIAN_POINT('Ctrl Pts',(51.7154836737872,38.3868512424513,-227.858769253939));
#207169=CARTESIAN_POINT('Ctrl Pts',(51.7181992444909,38.3831927442666,-227.858774006687));
#207170=CARTESIAN_POINT('Ctrl Pts',(51.7208174652636,38.3796504240554,-227.858776203219));
#207171=CARTESIAN_POINT('Ctrl Pts',(51.7233397168138,38.3762252975093,-227.858776203219));
#207172=CARTESIAN_POINT('',(51.2626335243563,39.5330360887948,-228.35005));
#207173=CARTESIAN_POINT('Origin',(51.2626335243564,39.5330360887949,-227.85005));
#207174=CARTESIAN_POINT('Ctrl Pts',(52.1258919562641,38.6726633987898,-228.35005));
#207175=CARTESIAN_POINT('Ctrl Pts',(52.101394940538,38.7361174509243,-228.35005));
#207176=CARTESIAN_POINT('Ctrl Pts',(52.0737422806294,38.7965600493266,-228.348939269426));
#207177=CARTESIAN_POINT('Ctrl Pts',(52.04303112011,38.8540344509297,-228.347412323243));
#207178=CARTESIAN_POINT('Ctrl Pts',(52.0113965235525,38.9132370169139,-228.345839464202));
#207179=CARTESIAN_POINT('Ctrl Pts',(51.9765167444005,38.9692904956714,-228.343823772569));
#207180=CARTESIAN_POINT('Ctrl Pts',(51.938458912692,39.0222114372786,-228.342098890823));
#207181=CARTESIAN_POINT('Ctrl Pts',(51.9116888594152,39.0594362701891,-228.340885601097));
#207182=CARTESIAN_POINT('Ctrl Pts',(51.8833455488624,39.0951105484446,-228.339815631152));
#207183=CARTESIAN_POINT('Ctrl Pts',(51.8534413111295,39.1292301746532,-228.339142200799));
#207184=CARTESIAN_POINT('Ctrl Pts',(51.8340942469303,39.1513044573889,-228.338706513376));
#207185=CARTESIAN_POINT('Ctrl Pts',(51.8140936482124,39.1727278475187,-228.338436787019));
#207186=CARTESIAN_POINT('Ctrl Pts',(51.7934409172728,39.1934973238057,-228.338402007334));
#207187=CARTESIAN_POINT('Ctrl Pts',(51.7918446266259,39.1951026379326,-228.338399319143));
#207188=CARTESIAN_POINT('Ctrl Pts',(51.7902444453824,39.1967040387988,-228.338398034845));
#207189=CARTESIAN_POINT('Ctrl Pts',(51.7886403549826,39.1983015433779,-228.338398186468));
#207190=CARTESIAN_POINT('Ctrl Pts',(51.724379729213,39.2622983380304,-228.338404260535));
#207191=CARTESIAN_POINT('Ctrl Pts',(51.6539261706324,39.3200860120821,-228.340708253783));
#207192=CARTESIAN_POINT('Ctrl Pts',(51.5772375424492,39.3714801303097,-228.343273660827));
#207193=CARTESIAN_POINT('Ctrl Pts',(51.4964326560892,39.425632825192,-228.345976765962));
#207194=CARTESIAN_POINT('Ctrl Pts',(51.4087052720494,39.4726870394319,-228.348969753843));
#207195=CARTESIAN_POINT('Ctrl Pts',(51.3140209355321,39.512440028451,-228.349816254427));
#207196=CARTESIAN_POINT('Ctrl Pts',(51.2971136329727,39.5195385184199,-228.34996740975));
#207197=CARTESIAN_POINT('Ctrl Pts',(51.2799845442189,39.5264042410929,-228.35005));
#207198=CARTESIAN_POINT('Ctrl Pts',(51.2626335243564,39.5330360887947,-228.35005));
#207199=CARTESIAN_POINT('Origin',(48.892180948596,36.2913696007177,-227.85005));
#207200=CARTESIAN_POINT('Origin',(48.892180948596,36.2913696007177,-228.35005));
#207201=CARTESIAN_POINT('',(48.892180948596,32.7753941674559,-227.858776203219));
#207202=CARTESIAN_POINT('Origin',(48.892180948596,36.2913696007177,-227.858776203219));
#207203=CARTESIAN_POINT('Origin',(48.892180948596,36.2913696007177,-227.858776203219));
#207204=CARTESIAN_POINT('Origin',(48.1334350484927,-61.7961505568785,-227.85005));
#207205=CARTESIAN_POINT('',(48.1334350484927,-57.7802512760377,-228.35005));
#207206=CARTESIAN_POINT('Origin',(48.1334350484927,-61.7961505568785,-228.35005));
#207207=CARTESIAN_POINT('',(48.1334350484927,-58.2801751236159,-227.858776203219));
#207208=CARTESIAN_POINT('Origin',(48.1334350484927,-57.7802512760377,-227.85005));
#207209=CARTESIAN_POINT('',(48.1334350484927,-65.3121259901411,-227.858776203219));
#207210=CARTESIAN_POINT('Origin',(48.1334350484927,-61.7961505568785,-227.858776203219));
#207211=CARTESIAN_POINT('Origin',(48.1334350484927,-61.7961505568785,-227.858776203219));
#207212=CARTESIAN_POINT('Ctrl Pts',(54.2123842387114,-60.9809369188682,
-220.34872120014));
#207213=CARTESIAN_POINT('Ctrl Pts',(53.9849086976504,-60.7491038125482,
-220.006959754302));
#207214=CARTESIAN_POINT('Ctrl Pts',(54.3075179287798,-60.4058635314347,
-219.986910060041));
#207215=CARTESIAN_POINT('Ctrl Pts',(54.2905773520916,-61.0606279145824,
-220.207250076519));
#207216=CARTESIAN_POINT('Ctrl Pts',(54.0902539551932,-60.8227589927709,
-219.884871134182));
#207217=CARTESIAN_POINT('Ctrl Pts',(54.4118428785764,-60.5120824447637,
-219.845412347007));
#207218=CARTESIAN_POINT('Ctrl Pts',(54.359483942211,-61.1484321661822,-220.068048613768));
#207219=CARTESIAN_POINT('Ctrl Pts',(54.1883692315684,-60.9105945733191,
-219.759116870628));
#207220=CARTESIAN_POINT('Ctrl Pts',(54.5038491541938,-60.6290451815934,
-219.706184350974));
#207221=CARTESIAN_POINT('Ctrl Pts',(54.4780017311477,-61.3407746536632,
-219.794316977736));
#207222=CARTESIAN_POINT('Ctrl Pts',(54.3601921871582,-61.1113013655168,
-219.509518223974));
#207223=CARTESIAN_POINT('Ctrl Pts',(54.6622597796057,-60.8851359437949,
-219.432400986523));
#207224=CARTESIAN_POINT('Ctrl Pts',(54.527958659632,-61.4464128888113,-219.65854206581));
#207225=CARTESIAN_POINT('Ctrl Pts',(54.4358335264181,-61.2248747082977,
-219.383842189249));
#207226=CARTESIAN_POINT('Ctrl Pts',(54.7291280292789,-61.0257268060029,
-219.29660115324));
#207227=CARTESIAN_POINT('Ctrl Pts',(54.602542940236,-61.6709815877632,-219.399995666978));
#207228=CARTESIAN_POINT('Ctrl Pts',(54.5543689314799,-61.4719546649753,
-219.143398711153));
#207229=CARTESIAN_POINT('Ctrl Pts',(54.8292130354721,-61.324481551372,-219.038012931781));
#207230=CARTESIAN_POINT('Ctrl Pts',(54.6275380455227,-61.7897249373771,
-219.277032330241));
#207231=CARTESIAN_POINT('Ctrl Pts',(54.5990060222776,-61.6050459038175,
-219.027646728975));
#207232=CARTESIAN_POINT('Ctrl Pts',(54.8629184699323,-61.4823979173559,
-218.915032638408));
#207233=CARTESIAN_POINT('Ctrl Pts',(54.647034139304,-62.043025557965,-219.046408327258));
#207234=CARTESIAN_POINT('Ctrl Pts',(54.6493563799739,-61.8922244718436,
-218.810400243037));
#207235=CARTESIAN_POINT('Ctrl Pts',(54.8898067560441,-61.8191471195123,
-218.684386523562));
#207236=CARTESIAN_POINT('Ctrl Pts',(54.641064245613,-62.1766218791842,-218.939992225721));
#207237=CARTESIAN_POINT('Ctrl Pts',(54.6555291975715,-62.0456431176211,
-218.709001772433));
#207238=CARTESIAN_POINT('Ctrl Pts',(54.8823609599701,-61.9966926518151,
-218.577969748941));
#207239=CARTESIAN_POINT('Ctrl Pts',(54.6151554910244,-62.3124799546862,
-218.850050000001));
#207240=CARTESIAN_POINT('Ctrl Pts',(54.6359260398381,-62.2035651560494,
-218.622717457036));
#207241=CARTESIAN_POINT('Ctrl Pts',(54.848380895554,-62.1772035872432,-218.488025452359));
#207242=CARTESIAN_POINT('',(54.8483808955536,-62.1772035872456,-218.488025452358));
#207243=CARTESIAN_POINT('',(54.615155491024,-62.3124799546881,-218.85005));
#207244=CARTESIAN_POINT('Origin',(55.1063041457817,-62.4061442430845,-218.85005));
#207245=CARTESIAN_POINT('',(54.2123842387114,-60.9809369188682,-220.34872120014));
#207246=CARTESIAN_POINT('Ctrl Pts',(54.2123842387114,-60.9809369188682,
-220.34872120014));
#207247=CARTESIAN_POINT('Ctrl Pts',(54.2537240469357,-61.0230686404178,
-220.273927028716));
#207248=CARTESIAN_POINT('Ctrl Pts',(54.2896597958659,-61.0646008231263,
-220.204851872225));
#207249=CARTESIAN_POINT('Ctrl Pts',(54.3210095713433,-61.1044816969448,
-220.141567685847));
#207250=CARTESIAN_POINT('Ctrl Pts',(54.3238457271854,-61.1080896453766,
-220.135842483284));
#207251=CARTESIAN_POINT('Ctrl Pts',(54.3266443240743,-61.1116841049447,
-220.130164684514));
#207252=CARTESIAN_POINT('Ctrl Pts',(54.3294059505124,-61.115264314403,-220.124534347917));
#207253=CARTESIAN_POINT('Ctrl Pts',(54.3510792439722,-61.1433618619816,
-220.080347366046));
#207254=CARTESIAN_POINT('Ctrl Pts',(54.370479895722,-61.1705828148596,-220.039078356947));
#207255=CARTESIAN_POINT('Ctrl Pts',(54.3879023892055,-61.1966031534464,
-220.00071034299));
#207256=CARTESIAN_POINT('Ctrl Pts',(54.3955663297739,-61.2080491803131,
-219.983832725617));
#207257=CARTESIAN_POINT('Ctrl Pts',(54.4028473735161,-61.2192634874255,
-219.967516092357));
#207258=CARTESIAN_POINT('Ctrl Pts',(54.4097697233646,-61.2302215008038,
-219.951757419607));
#207259=CARTESIAN_POINT('Ctrl Pts',(54.4111288373526,-61.2323729652038,
-219.948663407742));
#207260=CARTESIAN_POINT('Ctrl Pts',(54.4120182448729,-61.2337858808344,
-219.946634534833));
#207261=CARTESIAN_POINT('Ctrl Pts',(54.4136687028363,-61.2364267554626,
-219.942853784503));
#207262=CARTESIAN_POINT('Ctrl Pts',(54.4138526602173,-61.2367211030867,
-219.942432388173));
#207263=CARTESIAN_POINT('Ctrl Pts',(54.4140460332135,-61.2370307393494,
-219.941989237738));
#207264=CARTESIAN_POINT('Ctrl Pts',(54.4142504910173,-61.2373584174968,
-219.9415204411));
#207265=CARTESIAN_POINT('Ctrl Pts',(54.4157577062355,-61.2397739843335,
-219.938064581681));
#207266=CARTESIAN_POINT('Ctrl Pts',(54.4172550982855,-61.2421889601547,
-219.934618672845));
#207267=CARTESIAN_POINT('Ctrl Pts',(54.4187427686362,-61.2446032994954,
-219.931182653013));
#207268=CARTESIAN_POINT('Ctrl Pts',(54.4361365177009,-61.2728316046632,
-219.891008923185));
#207269=CARTESIAN_POINT('Ctrl Pts',(54.4522303236627,-61.3010643287227,
-219.852083180668));
#207270=CARTESIAN_POINT('Ctrl Pts',(54.4671094261737,-61.3291558492811,
-219.814439928106));
#207271=CARTESIAN_POINT('Ctrl Pts',(54.4785012271342,-61.3506633972424,
-219.785619342968));
#207272=CARTESIAN_POINT('Ctrl Pts',(54.4891812458271,-61.3720890889861,
-219.757549559389));
#207273=CARTESIAN_POINT('Ctrl Pts',(54.4991903161083,-61.3933821403281,
-219.730231992184));
#207274=CARTESIAN_POINT('Ctrl Pts',(54.5158763994284,-61.4288797059211,
-219.684690978917));
#207275=CARTESIAN_POINT('Ctrl Pts',(54.5307001536245,-61.4640120265341,
-219.641236079515));
#207276=CARTESIAN_POINT('Ctrl Pts',(54.5438437305745,-61.4985738453453,
-219.599859124708));
#207277=CARTESIAN_POINT('Ctrl Pts',(54.5449970207671,-61.5016064906308,
-219.596228481667));
#207278=CARTESIAN_POINT('Ctrl Pts',(54.5461373724362,-61.5046347625141,
-219.592613825135));
#207279=CARTESIAN_POINT('Ctrl Pts',(54.5472649091519,-61.5076585370498,
-219.589015137637));
#207280=CARTESIAN_POINT('Ctrl Pts',(54.5495945111213,-61.5139059532228,
-219.581579894628));
#207281=CARTESIAN_POINT('Ctrl Pts',(54.5518694025075,-61.5201341524938,
-219.574212841306));
#207282=CARTESIAN_POINT('Ctrl Pts',(54.554090649916,-61.5263419968953,-219.566913836884));
#207283=CARTESIAN_POINT('Ctrl Pts',(54.5555526235454,-61.5304278563884,
-219.562109801122));
#207284=CARTESIAN_POINT('Ctrl Pts',(54.5567753187678,-61.5338904711071,
-219.558053827738));
#207285=CARTESIAN_POINT('Ctrl Pts',(54.5581873646019,-61.5379417398871,
-219.553326108062));
#207286=CARTESIAN_POINT('Ctrl Pts',(54.5589207084565,-61.5400457601614,
-219.550870774044));
#207287=CARTESIAN_POINT('Ctrl Pts',(54.5597045823261,-61.5423088586908,
-219.548234516646));
#207288=CARTESIAN_POINT('Ctrl Pts',(54.5605944954227,-61.5449032557025,
-219.545220712212));
#207289=CARTESIAN_POINT('Ctrl Pts',(54.5621719558726,-61.549502085288,-219.539878440797));
#207290=CARTESIAN_POINT('Ctrl Pts',(54.5637240141203,-61.5541001818136,
-219.534560962645));
#207291=CARTESIAN_POINT('Ctrl Pts',(54.5652507364924,-61.5586970472681,
-219.529268620771));
#207292=CARTESIAN_POINT('Ctrl Pts',(54.5780112412408,-61.5971181279658,
-219.485034675651));
#207293=CARTESIAN_POINT('Ctrl Pts',(54.5890413035181,-61.6354331544369,
-219.442535875386));
#207294=CARTESIAN_POINT('Ctrl Pts',(54.5984153252178,-61.6735157296616,
-219.401798240125));
#207295=CARTESIAN_POINT('Ctrl Pts',(54.6027277343643,-61.6910351733947,
-219.383057367046));
#207296=CARTESIAN_POINT('Ctrl Pts',(54.6066902752954,-61.7085051178258,
-219.364688932253));
#207297=CARTESIAN_POINT('Ctrl Pts',(54.6103132286145,-61.7259117389287,
-219.346694043013));
#207298=CARTESIAN_POINT('Ctrl Pts',(54.6183417653991,-61.7644851583222,
-219.306817009699));
#207299=CARTESIAN_POINT('Ctrl Pts',(54.6246998913435,-61.8027476831842,
-219.268776760042));
#207300=CARTESIAN_POINT('Ctrl Pts',(54.6295318825711,-61.8405436932965,
-219.232560832877));
#207301=CARTESIAN_POINT('Ctrl Pts',(54.6312513254441,-61.8539932376264,
-219.21967355413));
#207302=CARTESIAN_POINT('Ctrl Pts',(54.6327779097984,-61.8673837179251,
-219.20701693033));
#207303=CARTESIAN_POINT('Ctrl Pts',(54.6341193240819,-61.8807082423834,
-219.194589255187));
#207304=CARTESIAN_POINT('Ctrl Pts',(54.6345726244288,-61.8852109613671,
-219.190389605964));
#207305=CARTESIAN_POINT('Ctrl Pts',(54.6349450981342,-61.8890796851728,
-219.186797222501));
#207306=CARTESIAN_POINT('Ctrl Pts',(54.6353505020694,-61.8934796155092,
-219.182728343179));
#207307=CARTESIAN_POINT('Ctrl Pts',(54.6355981015012,-61.8961668618742,
-219.180243285387));
#207308=CARTESIAN_POINT('Ctrl Pts',(54.6358573830125,-61.8990525672118,
-219.177580791167));
#207309=CARTESIAN_POINT('Ctrl Pts',(54.6361464827514,-61.9024062219641,
-219.174497870032));
#207310=CARTESIAN_POINT('Ctrl Pts',(54.6365480120771,-61.9070640979499,
-219.170216014747));
#207311=CARTESIAN_POINT('Ctrl Pts',(54.6369277824627,-61.9117200028051,
-219.1659562532));
#207312=CARTESIAN_POINT('Ctrl Pts',(54.6372859911519,-61.9163739319722,
-219.161718390579));
#207313=CARTESIAN_POINT('Ctrl Pts',(54.6402489447282,-61.9548693020932,
-219.126664550208));
#207314=CARTESIAN_POINT('Ctrl Pts',(54.6416927844994,-61.9931370662252,
-219.093227206538));
#207315=CARTESIAN_POINT('Ctrl Pts',(54.6417016572482,-62.0310368381492,
-219.061436133771));
#207316=CARTESIAN_POINT('Ctrl Pts',(54.6417109462764,-62.0707147391475,
-219.028153531427));
#207317=CARTESIAN_POINT('Ctrl Pts',(54.6401477866251,-62.1099895493046,
-218.996674810712));
#207318=CARTESIAN_POINT('Ctrl Pts',(54.6371107038755,-62.1487460190625,
-218.966996442013));
#207319=CARTESIAN_POINT('Ctrl Pts',(54.6338463359794,-62.1904028937909,
-218.935097043157));
#207320=CARTESIAN_POINT('Ctrl Pts',(54.6288796078067,-62.231461062838,-218.905277062178));
#207321=CARTESIAN_POINT('Ctrl Pts',(54.6223290653762,-62.2718265419444,
-218.87749714131));
#207322=CARTESIAN_POINT('Ctrl Pts',(54.6201170830798,-62.2854571269101,
-218.868116438291));
#207323=CARTESIAN_POINT('Ctrl Pts',(54.6177244432035,-62.2990091065251,
-218.858968114652));
#207324=CARTESIAN_POINT('Ctrl Pts',(54.6151554910244,-62.3124799546862,
-218.850050000001));
#207325=CARTESIAN_POINT('',(54.3075179287798,-60.4058635314347,-219.986910060041));
#207326=CARTESIAN_POINT('Origin',(54.5692758093764,-60.630753528645,-220.34872120014));
#207327=CARTESIAN_POINT('Ctrl Pts',(54.848380895554,-62.1772035872432,-218.488025452359));
#207328=CARTESIAN_POINT('Ctrl Pts',(54.8595780951736,-62.1177211521084,
-218.517664132001));
#207329=CARTESIAN_POINT('Ctrl Pts',(54.8678564354363,-62.0587810759542,
-218.548979038982));
#207330=CARTESIAN_POINT('Ctrl Pts',(54.8734777099421,-62.0004951204819,
-218.581727253286));
#207331=CARTESIAN_POINT('Ctrl Pts',(54.8794967639772,-61.9380846626563,
-218.616792836944));
#207332=CARTESIAN_POINT('Ctrl Pts',(54.8824693653225,-61.8764235092185,
-218.653502177699));
#207333=CARTESIAN_POINT('Ctrl Pts',(54.8826645527079,-61.8156518061647,
-218.691591283606));
#207334=CARTESIAN_POINT('Ctrl Pts',(54.8828436018189,-61.7599047640072,
-218.726531146832));
#207335=CARTESIAN_POINT('Ctrl Pts',(54.8806845561729,-61.7049057977467,
-218.762632937219));
#207336=CARTESIAN_POINT('Ctrl Pts',(54.8763620068724,-61.6507727587228,
-218.799709864555));
#207337=CARTESIAN_POINT('Ctrl Pts',(54.8763424593426,-61.6505279570742,
-218.799877534671));
#207338=CARTESIAN_POINT('Ctrl Pts',(54.8763228688496,-61.6502831758785,
-218.800045222107));
#207339=CARTESIAN_POINT('Ctrl Pts',(54.8763032354031,-61.6500384151223,
-218.800212926867));
#207340=CARTESIAN_POINT('Ctrl Pts',(54.8628119724682,-61.4818493143656,
-218.915452449409));
#207341=CARTESIAN_POINT('Ctrl Pts',(54.8291146403181,-61.3241894585149,
-219.038266143607));
#207342=CARTESIAN_POINT('Ctrl Pts',(54.7791703042592,-61.175104320049,-219.167307118481));
#207343=CARTESIAN_POINT('Ctrl Pts',(54.7790856375891,-61.174851587843,-219.167525871407));
#207344=CARTESIAN_POINT('Ctrl Pts',(54.7790009228209,-61.1745988809922,
-219.167744642781));
#207345=CARTESIAN_POINT('Ctrl Pts',(54.7789161599765,-61.1743461995148,
-219.167963432577));
#207346=CARTESIAN_POINT('Ctrl Pts',(54.7321821205352,-61.0350301322992,
-219.288593303123));
#207347=CARTESIAN_POINT('Ctrl Pts',(54.6708383586244,-60.9034276348827,
-219.414819509759));
#207348=CARTESIAN_POINT('Ctrl Pts',(54.5985281980209,-60.7825291610854,
-219.542285535957));
#207349=CARTESIAN_POINT('Ctrl Pts',(54.5934244554191,-60.7739959938782,
-219.55128224932));
#207350=CARTESIAN_POINT('Ctrl Pts',(54.58826606349,-60.7655161570842,-219.560285148006));
#207351=CARTESIAN_POINT('Ctrl Pts',(54.5830542956885,-60.757090705388,-219.569292703597));
#207352=CARTESIAN_POINT('Ctrl Pts',(54.5829701683847,-60.7569547034476,
-219.569438101741));
#207353=CARTESIAN_POINT('Ctrl Pts',(54.5828860266501,-60.7568187140274,
-219.569583502503));
#207354=CARTESIAN_POINT('Ctrl Pts',(54.5828018704853,-60.7566827371269,
-219.569728905881));
#207355=CARTESIAN_POINT('Ctrl Pts',(54.5036381576416,-60.6287724845599,
-219.706506423312));
#207356=CARTESIAN_POINT('Ctrl Pts',(54.4117181269148,-60.5119554283026,
-219.845581549818));
#207357=CARTESIAN_POINT('Ctrl Pts',(54.3075179287798,-60.4058635314347,
-219.986910060041));
#207358=CARTESIAN_POINT('Ctrl Pts',(54.3075179287798,-60.4058635314347,
-219.986910060041));
#207359=CARTESIAN_POINT('Ctrl Pts',(53.9849086976503,-60.7491038125481,
-220.006959754301));
#207360=CARTESIAN_POINT('Ctrl Pts',(54.2123842387114,-60.9809369188682,
-220.34872120014));
#207361=CARTESIAN_POINT('Ctrl Pts',(52.5270340116508,-58.593055911284,-222.401810820094));
#207362=CARTESIAN_POINT('Ctrl Pts',(52.2079291156962,-58.9380840675622,
-222.419842682816));
#207363=CARTESIAN_POINT('Ctrl Pts',(52.433041068884,-59.1675083087135,-222.763182656182));
#207364=CARTESIAN_POINT('Ctrl Pts',(50.7503363279055,-56.7819842883116,
-224.820210504335));
#207365=CARTESIAN_POINT('Ctrl Pts',(50.428037288823,-57.124096290766,-224.842059161051));
#207366=CARTESIAN_POINT('Ctrl Pts',(50.6562579911382,-57.3566888322572,
-225.181485677498));
#207367=CARTESIAN_POINT('Ctrl Pts',(48.9740484537045,-54.9709070690089,
-227.238815650979));
#207368=CARTESIAN_POINT('Ctrl Pts',(48.6520074870279,-55.3140445196239,
-227.259140997287));
#207369=CARTESIAN_POINT('Ctrl Pts',(48.8796513269547,-55.5460491487752,
-227.60005));
#207370=CARTESIAN_POINT('',(48.8796513269546,-55.5460491487752,-227.60005));
#207371=CARTESIAN_POINT('',(48.9740484537045,-54.9709070690089,-227.238815650979));
#207372=CARTESIAN_POINT('Origin',(49.2365428976196,-55.195865758552,-227.60005));
#207373=CARTESIAN_POINT('Ctrl Pts',(54.3075179287798,-60.4058635314347,
-219.986910060041));
#207374=CARTESIAN_POINT('Ctrl Pts',(53.8875633330448,-59.9782848917578,
-220.556501654024));
#207375=CARTESIAN_POINT('Ctrl Pts',(53.4552664659625,-59.5380214346079,
-221.143316453006));
#207376=CARTESIAN_POINT('Ctrl Pts',(53.0105815049601,-59.0850311267164,
-221.747382788392));
#207377=CARTESIAN_POINT('Ctrl Pts',(52.6770677842083,-58.7452883957977,
-222.200432539931));
#207378=CARTESIAN_POINT('Ctrl Pts',(52.3365853899896,-58.3983865617056,
-222.663186174999));
#207379=CARTESIAN_POINT('Ctrl Pts',(51.9891084328353,-58.044304097751,-223.135650875041));
#207380=CARTESIAN_POINT('Ctrl Pts',(51.9239565033689,-57.9779136357595,
-223.224238006299));
#207381=CARTESIAN_POINT('Ctrl Pts',(51.8585586551558,-57.9112707208977,
-223.313166528186));
#207382=CARTESIAN_POINT('Ctrl Pts',(51.7929146954598,-57.8443751995069,
-223.402436467273));
#207383=CARTESIAN_POINT('Ctrl Pts',(51.7621440893522,-57.8130179238549,
-223.44428175122));
#207384=CARTESIAN_POINT('Ctrl Pts',(51.731319405913,-57.7816051437855,-223.486202053495));
#207385=CARTESIAN_POINT('Ctrl Pts',(51.7004406247366,-57.7501368431761,
-223.528197376319));
#207386=CARTESIAN_POINT('Ctrl Pts',(51.6929621699204,-57.7425156141222,
-223.538368118565));
#207387=CARTESIAN_POINT('Ctrl Pts',(51.6854805420115,-57.7348911285222,
-223.548543261124));
#207388=CARTESIAN_POINT('Ctrl Pts',(51.6779957407168,-57.7272633861453,
-223.558722804025));
#207389=CARTESIAN_POINT('Ctrl Pts',(51.6741238780136,-57.7233175804979,
-223.563988647557));
#207390=CARTESIAN_POINT('Ctrl Pts',(51.6702511661257,-57.7193709033506,
-223.569255668603));
#207391=CARTESIAN_POINT('Ctrl Pts',(51.6663776050122,-57.7154233546713,
-223.574523867165));
#207392=CARTESIAN_POINT('Ctrl Pts',(51.6653057221808,-57.7143309981726,
-223.575981670831));
#207393=CARTESIAN_POINT('Ctrl Pts',(51.664233774322,-57.7132385749384,-223.577439564662));
#207394=CARTESIAN_POINT('Ctrl Pts',(51.6631617614348,-57.712146084968,-223.57889754866));
#207395=CARTESIAN_POINT('Ctrl Pts',(51.6625551133699,-57.7115278489986,
-223.579722616325));
#207396=CARTESIAN_POINT('Ctrl Pts',(51.6619484444804,-57.7109095916577,
-223.580547712866));
#207397=CARTESIAN_POINT('Ctrl Pts',(51.6613417547661,-57.7102913129452,
-223.581372838281));
#207398=CARTESIAN_POINT('Ctrl Pts',(51.660743488977,-57.7096816190717,-223.582186506777));
#207399=CARTESIAN_POINT('Ctrl Pts',(51.6601403769267,-57.7090669862187,
-223.583006766944));
#207400=CARTESIAN_POINT('Ctrl Pts',(51.6595329670214,-57.7084479732613,
-223.58383287295));
#207401=CARTESIAN_POINT('Ctrl Pts',(51.6557850761697,-57.704628488298,-223.588930180572));
#207402=CARTESIAN_POINT('Ctrl Pts',(51.6518829388499,-57.7006518043736,
-223.594237292841));
#207403=CARTESIAN_POINT('Ctrl Pts',(51.6481312278776,-57.6968284147854,
-223.599339838672));
#207404=CARTESIAN_POINT('Ctrl Pts',(51.646262699952,-57.6949241875491,-223.601881145677));
#207405=CARTESIAN_POINT('Ctrl Pts',(51.6444314852871,-57.693057985038,-223.604371709749));
#207406=CARTESIAN_POINT('Ctrl Pts',(51.6426752228762,-57.6912681656368,
-223.606760338636));
#207407=CARTESIAN_POINT('Ctrl Pts',(51.6416597675426,-57.6902333079493,
-223.608141422652));
#207408=CARTESIAN_POINT('Ctrl Pts',(51.6406693691138,-57.6892239855127,
-223.609488429222));
#207409=CARTESIAN_POINT('Ctrl Pts',(51.6397113028646,-57.6882476126825,
-223.610791463244));
#207410=CARTESIAN_POINT('Ctrl Pts',(51.6393123131538,-57.6878409991384,
-223.611334115872));
#207411=CARTESIAN_POINT('Ctrl Pts',(51.6389191572805,-57.6874403308405,
-223.611868834326));
#207412=CARTESIAN_POINT('Ctrl Pts',(51.6385241006106,-57.6870377253632,
-223.612406138221));
#207413=CARTESIAN_POINT('Ctrl Pts',(51.1416290490366,-57.1806479219664,
-224.2882171474));
#207414=CARTESIAN_POINT('Ctrl Pts',(50.6267656464817,-56.6558456527314,
-224.988840225086));
#207415=CARTESIAN_POINT('Ctrl Pts',(50.0938544585926,-56.1125730789731,
-225.714254827363));
#207416=CARTESIAN_POINT('Ctrl Pts',(49.7290551815088,-55.7406810138965,
-226.210830482952));
#207417=CARTESIAN_POINT('Ctrl Pts',(49.3557981786686,-55.3601335228959,
-226.719022737376));
#207418=CARTESIAN_POINT('Ctrl Pts',(48.9740484537045,-54.9709070690089,
-227.238815650979));
#207419=CARTESIAN_POINT('Ctrl Pts',(48.8796513269547,-55.5460491487752,
-227.60005));
#207420=CARTESIAN_POINT('Ctrl Pts',(50.6562583519279,-57.3566891999582,
-225.181485185797));
#207421=CARTESIAN_POINT('Ctrl Pts',(52.4330406746144,-59.1675079068912,
-222.763183190988));
#207422=CARTESIAN_POINT('Ctrl Pts',(54.2123842387114,-60.9809369188682,
-220.34872120014));
#207423=CARTESIAN_POINT('Origin',(55.1063041457817,-62.4061442430845,-218.85005));
#207424=CARTESIAN_POINT('',(55.1063041458243,-62.4061442430364,-218.35005));
#207425=CARTESIAN_POINT('Origin',(55.1063041458054,-62.4061442430575,-218.85005));
#207426=CARTESIAN_POINT('Origin',(55.1063041457932,-62.4061442430715,-218.85005));
#207427=CARTESIAN_POINT('Ctrl Pts',(47.4613130320155,-55.2424342950265,
-228.348304885641));
#207428=CARTESIAN_POINT('Ctrl Pts',(47.3021046372418,-55.1176952304439,
-228.346450927386));
#207429=CARTESIAN_POINT('Ctrl Pts',(47.1811427047561,-55.0343199344272,
-228.485631153611));
#207430=CARTESIAN_POINT('Ctrl Pts',(47.5376722342335,-55.1241814098811,
-228.358006905805));
#207431=CARTESIAN_POINT('Ctrl Pts',(47.406151448781,-54.9745809391036,-228.36408944129));
#207432=CARTESIAN_POINT('Ctrl Pts',(47.3217648821301,-54.8530430703057,
-228.501869875666));
#207433=CARTESIAN_POINT('Ctrl Pts',(47.6631621977863,-55.0560571955665,
-228.326632472374));
#207434=CARTESIAN_POINT('Ctrl Pts',(47.5601436638269,-54.8771403537813,
-228.316192700349));
#207435=CARTESIAN_POINT('Ctrl Pts',(47.5116824699239,-54.7217215905284,
-228.449649225183));
#207436=CARTESIAN_POINT('Ctrl Pts',(47.9275209649132,-55.0225868309807,
-228.21963517134));
#207437=CARTESIAN_POINT('Ctrl Pts',(47.850416577859,-54.802837775062,-228.155623333054));
#207438=CARTESIAN_POINT('Ctrl Pts',(47.8754805878992,-54.5907583268247,
-228.271417688637));
#207439=CARTESIAN_POINT('Ctrl Pts',(48.0593323270884,-55.0436861910913,
-228.152274449338));
#207440=CARTESIAN_POINT('Ctrl Pts',(47.9863428228055,-54.8113544609062,
-228.052661933177));
#207441=CARTESIAN_POINT('Ctrl Pts',(48.0444656792804,-54.5754212470967,
-228.159184370623));
#207442=CARTESIAN_POINT('Ctrl Pts',(48.3135352870045,-55.1294371299156,
-228.006090181985));
#207443=CARTESIAN_POINT('Ctrl Pts',(48.2286493510528,-54.8812191556274,
-227.834617170415));
#207444=CARTESIAN_POINT('Ctrl Pts',(48.3555740327057,-54.6054209473356,
-227.915582350477));
#207445=CARTESIAN_POINT('Ctrl Pts',(48.4368943091309,-55.1940478275634,
-227.92683964474));
#207446=CARTESIAN_POINT('Ctrl Pts',(48.3369447816902,-54.944944352671,-227.716654532444));
#207447=CARTESIAN_POINT('Ctrl Pts',(48.49900012063,-54.6503832012681,-227.783505557683));
#207448=CARTESIAN_POINT('Ctrl Pts',(48.6860658100372,-55.3621740854522,
-227.753484899464));
#207449=CARTESIAN_POINT('Ctrl Pts',(48.5353337959282,-55.1181513278107,
-227.465234070536));
#207450=CARTESIAN_POINT('Ctrl Pts',(48.7763611981979,-54.7909405035185,
-227.49457033784));
#207451=CARTESIAN_POINT('Ctrl Pts',(48.808149438057,-55.468371606431,-227.660133432125));
#207452=CARTESIAN_POINT('Ctrl Pts',(48.6175640550392,-55.2345767175589,
-227.333089928053));
#207453=CARTESIAN_POINT('Ctrl Pts',(48.9044383729524,-54.8912970631231,
-227.33896894949));
#207454=CARTESIAN_POINT('Ctrl Pts',(48.9209614213312,-55.5892183382082,
-227.56593431681));
#207455=CARTESIAN_POINT('Ctrl Pts',(48.6743407164146,-55.3608255688747,
-227.213117273111));
#207456=CARTESIAN_POINT('Ctrl Pts',(49.0153493238984,-55.0140778973635,
-227.181921047664));
#207457=CARTESIAN_POINT('',(47.4910910659473,-55.2017568268661,-228.35005));
#207458=CARTESIAN_POINT('',(47.2343490658922,-54.9709330687352,-228.488381729218));
#207459=CARTESIAN_POINT('Origin',(47.4910910659474,-55.2017568268662,-228.85005));
#207460=CARTESIAN_POINT('Ctrl Pts',(48.9740484537045,-54.9709070690089,
-227.238815650979));
#207461=CARTESIAN_POINT('Ctrl Pts',(48.9229565323117,-54.9188144908534,
-227.30838274414));
#207462=CARTESIAN_POINT('Ctrl Pts',(48.8416414398881,-54.8479207863561,
-227.411623042946));
#207463=CARTESIAN_POINT('Ctrl Pts',(48.738379705309,-54.7781024203753,-227.530126961583));
#207464=CARTESIAN_POINT('Ctrl Pts',(48.6923014503903,-54.7509634238684,
-227.580497977433));
#207465=CARTESIAN_POINT('Ctrl Pts',(48.6611746664914,-54.7334914992703,
-227.613986126256));
#207466=CARTESIAN_POINT('Ctrl Pts',(48.6464955257704,-54.7256187239374,
-227.629549471375));
#207467=CARTESIAN_POINT('Ctrl Pts',(48.5611906556844,-54.6822841007737,
-227.718479526806));
#207468=CARTESIAN_POINT('Ctrl Pts',(48.4914725151753,-54.6544212751007,
-227.786430965697));
#207469=CARTESIAN_POINT('Ctrl Pts',(48.3845686321144,-54.6228948487552,
-227.883569215853));
#207470=CARTESIAN_POINT('Ctrl Pts',(48.3305350506504,-54.6096981433835,
-227.930941113887));
#207471=CARTESIAN_POINT('Ctrl Pts',(48.2664530938673,-54.5988018476774,
-227.98411318093));
#207472=CARTESIAN_POINT('Ctrl Pts',(48.2387632988875,-54.5950968611026,
-228.006452249522));
#207473=CARTESIAN_POINT('Ctrl Pts',(48.2202528979549,-54.5928413400655,
-228.021245192995));
#207474=CARTESIAN_POINT('Ctrl Pts',(48.212327822807,-54.5919538315903,-228.027529021694));
#207475=CARTESIAN_POINT('Ctrl Pts',(48.1163763146568,-54.582537302858,-228.10276417424));
#207476=CARTESIAN_POINT('Ctrl Pts',(48.0325110079193,-54.5834648765834,
-228.162697419324));
#207477=CARTESIAN_POINT('Ctrl Pts',(47.9088313425645,-54.5986997083007,
-228.242183617849));
#207478=CARTESIAN_POINT('Ctrl Pts',(47.8475214607299,-54.6097772709699,
-228.279323299837));
#207479=CARTESIAN_POINT('Ctrl Pts',(47.7870065001217,-54.6260191079529,
-228.312557855911));
#207480=CARTESIAN_POINT('Ctrl Pts',(47.7468401025145,-54.6379912724447,
-228.333846420869));
#207481=CARTESIAN_POINT('Ctrl Pts',(47.7287456377893,-54.6438689926409,
-228.34312351292));
#207482=CARTESIAN_POINT('Ctrl Pts',(47.6633263561034,-54.6672964949944,
-228.375252805728));
#207483=CARTESIAN_POINT('Ctrl Pts',(47.6206907845702,-54.6856607265798,
-228.394188721727));
#207484=CARTESIAN_POINT('Ctrl Pts',(47.5373966142101,-54.7278310248293,
-228.427093328645));
#207485=CARTESIAN_POINT('Ctrl Pts',(47.4983789032494,-54.7505406095228,
-228.440586801717));
#207486=CARTESIAN_POINT('Ctrl Pts',(47.3744847769716,-54.8333295171273,
-228.476467690392));
#207487=CARTESIAN_POINT('Ctrl Pts',(47.3001594386793,-54.8976848030761,
-228.488412567484));
#207488=CARTESIAN_POINT('Ctrl Pts',(47.2343490658922,-54.9709330687352,
-228.488381729218));
#207489=CARTESIAN_POINT('Ctrl Pts',(47.4910910659473,-55.2017568268661,
-228.35005));
#207490=CARTESIAN_POINT('Ctrl Pts',(47.5339427387703,-55.1499211321669,
-228.35005));
#207491=CARTESIAN_POINT('Ctrl Pts',(47.5881950341781,-55.1087905244168,
-228.341044977978));
#207492=CARTESIAN_POINT('Ctrl Pts',(47.6839946527033,-55.0657816325896,
-228.31377766011));
#207493=CARTESIAN_POINT('Ctrl Pts',(47.7183291272714,-55.054562056961,-228.302405862635));
#207494=CARTESIAN_POINT('Ctrl Pts',(47.7730862638229,-55.0427477414354,
-228.281993305555));
#207495=CARTESIAN_POINT('Ctrl Pts',(47.801278640751,-55.0380943922812,-228.270949402552));
#207496=CARTESIAN_POINT('Ctrl Pts',(47.8355181611567,-55.0349339773232,
-228.256625838884));
#207497=CARTESIAN_POINT('Ctrl Pts',(47.8504731154847,-55.0340735392657,
-228.250182443202));
#207498=CARTESIAN_POINT('Ctrl Pts',(47.8605046077288,-55.0336105743244,
-228.245819553912));
#207499=CARTESIAN_POINT('Ctrl Pts',(47.8671616032058,-55.0333962334904,
-228.242891178549));
#207500=CARTESIAN_POINT('Ctrl Pts',(47.9260892897782,-55.0319989091495,
-228.216792199271));
#207501=CARTESIAN_POINT('Ctrl Pts',(47.9863251637679,-55.0372942416347,
-228.187704506116));
#207502=CARTESIAN_POINT('Ctrl Pts',(48.0825738653862,-55.0563960118545,
-228.137219522214));
#207503=CARTESIAN_POINT('Ctrl Pts',(48.1156375092139,-55.0646247696504,
-228.119253305707));
#207504=CARTESIAN_POINT('Ctrl Pts',(48.1665329703472,-55.0799280610835,
-228.090632666823));
#207505=CARTESIAN_POINT('Ctrl Pts',(48.1923055907121,-55.0883198524848,
-228.075905015572));
#207506=CARTESIAN_POINT('Ctrl Pts',(48.2229038264921,-55.0994431878277,
-228.058005688231));
#207507=CARTESIAN_POINT('Ctrl Pts',(48.2361268097716,-55.1045000334963,
-228.050182680758));
#207508=CARTESIAN_POINT('Ctrl Pts',(48.244965992782,-55.1079360956767,-228.044933803818));
#207509=CARTESIAN_POINT('Ctrl Pts',(48.2506824272076,-55.1102021852281,
-228.041523979641));
#207510=CARTESIAN_POINT('Ctrl Pts',(48.3043736715184,-55.1317487878865,
-228.009406678981));
#207511=CARTESIAN_POINT('Ctrl Pts',(48.3580533109924,-55.1569140229942,
-227.976053422806));
#207512=CARTESIAN_POINT('Ctrl Pts',(48.4422450190772,-55.2030191070475,
-227.921281485012));
#207513=CARTESIAN_POINT('Ctrl Pts',(48.470919305374,-55.2197819670126,-227.902237232472));
#207514=CARTESIAN_POINT('Ctrl Pts',(48.5147023734957,-55.2471592361541,
-227.872519388519));
#207515=CARTESIAN_POINT('Ctrl Pts',(48.5367866985082,-55.2614062320095,
-227.857373013928));
#207516=CARTESIAN_POINT('Ctrl Pts',(48.5628565451969,-55.279036830306,-227.839210184702));
#207517=CARTESIAN_POINT('Ctrl Pts',(48.5740911026579,-55.286812519136,-227.83132216892));
#207518=CARTESIAN_POINT('Ctrl Pts',(48.5815941382064,-55.2920455257207,
-227.826040568224));
#207519=CARTESIAN_POINT('Ctrl Pts',(48.586626808195,-55.2955891551262,-227.822486557596));
#207520=CARTESIAN_POINT('Ctrl Pts',(48.668802202713,-55.3537811062054,-227.764344353453));
#207521=CARTESIAN_POINT('Ctrl Pts',(48.7690559004533,-55.4333351349916,
-227.690384734712));
#207522=CARTESIAN_POINT('Ctrl Pts',(48.8796513269546,-55.5460491487752,
-227.60005));
#207523=CARTESIAN_POINT('Origin',(53.1417095267163,-62.031487089538,-218.85005));
#207524=CARTESIAN_POINT('',(54.6082148364463,-63.3913996516292,-218.35005));
#207525=CARTESIAN_POINT('',(54.2415885090138,-63.0514215111064,-218.85005));
#207526=CARTESIAN_POINT('Origin',(54.6082148364463,-63.3913996516292,-218.85005));
#207527=CARTESIAN_POINT('Origin',(53.1417095267163,-62.031487089538,-218.85005));
#207528=CARTESIAN_POINT('Origin',(53.1417095267163,-62.031487089538,-218.35005));
#207529=CARTESIAN_POINT('Ctrl Pts',(47.2343490658922,-54.9709330687353,
-228.488381729218));
#207530=CARTESIAN_POINT('Ctrl Pts',(47.3421114593162,-55.0678167910323,
-228.35005));
#207531=CARTESIAN_POINT('Ctrl Pts',(47.4910910659474,-55.2017568268662,
-228.35005));
#207532=CARTESIAN_POINT('Ctrl Pts',(46.3105395613661,-55.9991515869664,
-228.487948838892));
#207533=CARTESIAN_POINT('Ctrl Pts',(46.4160092042075,-56.0984512122452,
-228.350050000212));
#207534=CARTESIAN_POINT('Ctrl Pts',(46.5610878289829,-56.2361862677858,
-228.35005));
#207535=CARTESIAN_POINT('Ctrl Pts',(45.350506384691,-56.9893433179289,-228.48772415168));
#207536=CARTESIAN_POINT('Ctrl Pts',(45.4531166269507,-57.091545569762,-228.350050000038));
#207537=CARTESIAN_POINT('Ctrl Pts',(45.5947854895852,-57.2325158021754,
-228.35005));
#207538=CARTESIAN_POINT('Ctrl Pts',(43.3550620161755,-58.8891661040005,
-228.487824007409));
#207539=CARTESIAN_POINT('Ctrl Pts',(43.4520711334389,-58.9967304277239,
-228.350049999962));
#207540=CARTESIAN_POINT('Ctrl Pts',(43.5860475125547,-59.145141081541,-228.35005));
#207541=CARTESIAN_POINT('Ctrl Pts',(42.3185849747264,-59.7984761650306,
-228.488134585451));
#207542=CARTESIAN_POINT('Ctrl Pts',(42.4124726432155,-59.9088386926303,
-228.35005000027));
#207543=CARTESIAN_POINT('Ctrl Pts',(42.5429028274419,-60.0607223439083,
-228.35005));
#207544=CARTESIAN_POINT('Ctrl Pts',(41.2456587371609,-60.6702615191614,
-228.488620962447));
#207545=CARTESIAN_POINT('Ctrl Pts',(41.3371131727634,-60.7827319875555,
-228.35005));
#207546=CARTESIAN_POINT('Ctrl Pts',(41.4636310035132,-60.9383233439605,
-228.35005));
#207547=CARTESIAN_POINT('',(41.4636310035131,-60.9383233439604,-228.35005));
#207548=CARTESIAN_POINT('',(41.2456587371609,-60.6702615191614,-228.488620962447));
#207549=CARTESIAN_POINT('Origin',(41.4636310035131,-60.9383233439605,-228.85005));
#207550=CARTESIAN_POINT('Ctrl Pts',(47.2343490658922,-54.9709330687353,
-228.488381729218));
#207551=CARTESIAN_POINT('Ctrl Pts',(46.9328032818251,-55.3065595781188,
-228.48824042704));
#207552=CARTESIAN_POINT('Ctrl Pts',(46.6244555698817,-55.6414031174716,
-228.488119930198));
#207553=CARTESIAN_POINT('Ctrl Pts',(46.3094873419398,-55.9746757314993,
-228.48802406009));
#207554=CARTESIAN_POINT('Ctrl Pts',(46.0030015393239,-56.2989729638508,
-228.487930771864));
#207555=CARTESIAN_POINT('Ctrl Pts',(45.6902469778881,-56.6217826575224,
-228.48786080601));
#207556=CARTESIAN_POINT('Ctrl Pts',(45.3714253331597,-56.9424129887812,
-228.487817653494));
#207557=CARTESIAN_POINT('Ctrl Pts',(45.0526036884314,-57.2630433200401,
-228.487774500978));
#207558=CARTESIAN_POINT('Ctrl Pts',(44.7277147844279,-57.5814940621824,
-228.487758166213));
#207559=CARTESIAN_POINT('Ctrl Pts',(44.3969971042378,-57.8971105887381,
-228.487772045555));
#207560=CARTESIAN_POINT('Ctrl Pts',(44.3822709262308,-57.9111643434371,
-228.487772663573));
#207561=CARTESIAN_POINT('Ctrl Pts',(44.3675332810124,-57.9252124055014,
-228.487773341473));
#207562=CARTESIAN_POINT('Ctrl Pts',(44.3527842004334,-57.9392547109648,
-228.487774079544));
#207563=CARTESIAN_POINT('Ctrl Pts',(44.0592830129135,-58.2186913380103,
-228.487788766885));
#207564=CARTESIAN_POINT('Ctrl Pts',(43.7611582389086,-58.4958173950288,
-228.487826099836));
#207565=CARTESIAN_POINT('Ctrl Pts',(43.458773346099,-58.7702839246494,-228.487884322887));
#207566=CARTESIAN_POINT('Ctrl Pts',(43.1544170933402,-59.0465398039921,
-228.487942925516));
#207567=CARTESIAN_POINT('Ctrl Pts',(42.8457450210993,-59.3201014229422,
-228.488022688327));
#207568=CARTESIAN_POINT('Ctrl Pts',(42.5331641521048,-59.5906515496429,
-228.488121528093));
#207569=CARTESIAN_POINT('Ctrl Pts',(42.2168635114787,-59.8644212741694,
-228.48822154407));
#207570=CARTESIAN_POINT('Ctrl Pts',(41.8965605056513,-60.1351074534593,
-228.488341090339));
#207571=CARTESIAN_POINT('Ctrl Pts',(41.5727137355554,-60.4024200399638,
-228.488477758894));
#207572=CARTESIAN_POINT('Ctrl Pts',(41.464087735809,-60.4920831140937,-228.488523600816));
#207573=CARTESIAN_POINT('Ctrl Pts',(41.3550633321572,-60.5813669426097,
-228.488571367329));
#207574=CARTESIAN_POINT('Ctrl Pts',(41.2456587371609,-60.6702615191614,
-228.488620962447));
#207575=CARTESIAN_POINT('Ctrl Pts',(41.4636310035131,-60.9383233439604,
-228.35005));
#207576=CARTESIAN_POINT('Ctrl Pts',(42.5429085052274,-60.0607177270638,
-228.35005));
#207577=CARTESIAN_POINT('Ctrl Pts',(43.5860475125577,-59.1451410815382,
-228.35005));
#207578=CARTESIAN_POINT('Ctrl Pts',(44.5904165010271,-58.1888284418133,
-228.35005));
#207579=CARTESIAN_POINT('Ctrl Pts',(45.5947854894966,-57.2325158020884,
-228.35005));
#207580=CARTESIAN_POINT('Ctrl Pts',(46.5610786115705,-56.2361965201832,
-228.35005));
#207581=CARTESIAN_POINT('Ctrl Pts',(47.4910910659473,-55.2017568268661,
-228.35005));
#207582=CARTESIAN_POINT('Origin',(0.127542579976414,-12.8706479699377,-218.85005));
#207583=CARTESIAN_POINT('',(49.6055526500885,-68.3000311480131,-218.35005));
#207584=CARTESIAN_POINT('',(49.2725916132775,-67.9270204940557,-218.85005));
#207585=CARTESIAN_POINT('Origin',(49.6055526500885,-68.3000311480131,-218.85005));
#207586=CARTESIAN_POINT('Origin',(0.127542579976414,-12.8706479699377,-218.85005));
#207587=CARTESIAN_POINT('Origin',(0.127542579976414,-12.8706479699377,-218.35005));
#207588=CARTESIAN_POINT('Ctrl Pts',(41.8829757794224,-62.4277604346488,
-227.501386391297));
#207589=CARTESIAN_POINT('Ctrl Pts',(41.6736215736677,-62.1444346782205,
-227.135070658787));
#207590=CARTESIAN_POINT('Ctrl Pts',(41.3169485390188,-62.5017525488842,
-227.074161006169));
#207591=CARTESIAN_POINT('Ctrl Pts',(41.7287883985619,-62.2910497761554,
-227.617062287714));
#207592=CARTESIAN_POINT('Ctrl Pts',(41.5115567796579,-62.083269453487,-227.276647215301));
#207593=CARTESIAN_POINT('Ctrl Pts',(41.1560049633125,-62.3716221357762,
-227.267023357385));
#207594=CARTESIAN_POINT('Ctrl Pts',(41.5970941915982,-62.142277885216,-227.731465467726));
#207595=CARTESIAN_POINT('Ctrl Pts',(41.3631012191682,-61.9849776212493,
-227.438037521325));
#207596=CARTESIAN_POINT('Ctrl Pts',(41.029038944944,-62.2181773292512,-227.457737962389));
#207597=CARTESIAN_POINT('Ctrl Pts',(41.4165235670895,-61.863351898693,-227.924583312038));
#207598=CARTESIAN_POINT('Ctrl Pts',(41.1742388084123,-61.7588443268157,
-227.719355887922));
#207599=CARTESIAN_POINT('Ctrl Pts',(40.8795052413903,-61.9086867290362,
-227.779669319348));
#207600=CARTESIAN_POINT('Ctrl Pts',(41.3544951862324,-61.7387982044088,
-228.004831636089));
#207601=CARTESIAN_POINT('Ctrl Pts',(41.1128065542583,-61.64889903365,-227.838230834733));
#207602=CARTESIAN_POINT('Ctrl Pts',(40.83755717967,-61.7643747830512,-227.9134383294));
#207603=CARTESIAN_POINT('Ctrl Pts',(41.2769460700564,-61.4864549806276,
-228.15152387739));
#207604=CARTESIAN_POINT('Ctrl Pts',(41.0509213652705,-61.4074771774304,
-228.055852077472));
#207605=CARTESIAN_POINT('Ctrl Pts',(40.8167874720303,-61.4561982274081,
-228.157939415417));
#207606=CARTESIAN_POINT('Ctrl Pts',(41.26069413732,-61.3563209527895,-228.219337533727));
#207607=CARTESIAN_POINT('Ctrl Pts',(41.047419886702,-61.2728349773798,-228.158786517575));
#207608=CARTESIAN_POINT('Ctrl Pts',(40.8377574579081,-61.2894729474476,
-228.270955921442));
#207609=CARTESIAN_POINT('Ctrl Pts',(41.3125718827386,-61.0669017530136,
-228.340235822512));
#207610=CARTESIAN_POINT('Ctrl Pts',(41.1455858541625,-60.9545637033621,
-228.337710180632));
#207611=CARTESIAN_POINT('Ctrl Pts',(41.001859551751,-60.8897708053934,-228.472378638455));
#207612=CARTESIAN_POINT('Ctrl Pts',(41.4201040030741,-60.9266188466363,
-228.370752133428));
#207613=CARTESIAN_POINT('Ctrl Pts',(41.2921211277785,-60.7745213841431,
-228.383736779337));
#207614=CARTESIAN_POINT('Ctrl Pts',(41.1915219835725,-60.6688302795368,
-228.523150593268));
#207615=CARTESIAN_POINT('Ctrl Pts',(41.6001886489201,-60.8718793597729,
-228.335060161219));
#207616=CARTESIAN_POINT('Ctrl Pts',(41.5006043490813,-60.6869018002498,
-228.322259765032));
#207617=CARTESIAN_POINT('Ctrl Pts',(41.4493760764998,-60.5376437416971,
-228.463541011146));
#207618=CARTESIAN_POINT('',(41.7563078823353,-62.3074742642099,-227.60005));
#207619=CARTESIAN_POINT('',(41.1874522920715,-62.3844144545142,-227.238927571877));
#207620=CARTESIAN_POINT('Origin',(41.3994163116703,-62.6576576544332,-227.60005));
#207621=CARTESIAN_POINT('Ctrl Pts',(41.2456587371608,-60.6702615191613,
-228.488620962446));
#207622=CARTESIAN_POINT('Ctrl Pts',(41.2197244417364,-60.6913339308266,
-228.488632715863));
#207623=CARTESIAN_POINT('Ctrl Pts',(41.1947961167656,-60.7134311818696,
-228.48724613514));
#207624=CARTESIAN_POINT('Ctrl Pts',(41.1708632827344,-60.7365186965675,
-228.484495167239));
#207625=CARTESIAN_POINT('Ctrl Pts',(41.1596112218472,-60.7473733291938,
-228.483201795201));
#207626=CARTESIAN_POINT('Ctrl Pts',(41.1485791592349,-60.7584475828374,
-228.481606311605));
#207627=CARTESIAN_POINT('Ctrl Pts',(41.1377675402693,-60.7697403512738,
-228.479709419403));
#207628=CARTESIAN_POINT('Ctrl Pts',(41.1258039235476,-60.7822363848215,
-228.477610409871));
#207629=CARTESIAN_POINT('Ctrl Pts',(41.1139760163711,-60.7951667696545,
-228.475098941214));
#207630=CARTESIAN_POINT('Ctrl Pts',(41.1024394739555,-60.8083607221593,
-228.472208416089));
#207631=CARTESIAN_POINT('Ctrl Pts',(41.0976756225717,-60.8138089775059,
-228.471014814781));
#207632=CARTESIAN_POINT('Ctrl Pts',(41.0929610512213,-60.8193019557174,
-228.469756992603));
#207633=CARTESIAN_POINT('Ctrl Pts',(41.0883049776624,-60.8248267792451,
-228.468439019492));
#207634=CARTESIAN_POINT('Ctrl Pts',(41.0803391715892,-60.8342788792288,
-228.466184175773));
#207635=CARTESIAN_POINT('Ctrl Pts',(41.0725424991094,-60.8438221898664,
-228.463756003074));
#207636=CARTESIAN_POINT('Ctrl Pts',(41.0649629951811,-60.8533924384031,
-228.461173742144));
#207637=CARTESIAN_POINT('Ctrl Pts',(41.0573834912528,-60.8629626869397,
-228.458591481213));
#207638=CARTESIAN_POINT('Ctrl Pts',(41.0500211562498,-60.8725598738205,
-228.45585513266));
#207639=CARTESIAN_POINT('Ctrl Pts',(41.0429240799344,-60.8821197945625,
-228.452984028281));
#207640=CARTESIAN_POINT('Ctrl Pts',(41.0247366592379,-60.9066186575638,
-228.445626352967));
#207641=CARTESIAN_POINT('Ctrl Pts',(41.0076807313764,-60.9315713204337,
-228.437229166001));
#207642=CARTESIAN_POINT('Ctrl Pts',(40.9917410517639,-60.9569680117623,
-228.427810778945));
#207643=CARTESIAN_POINT('Ctrl Pts',(40.9828008708308,-60.9712124019319,
-228.422528233347));
#207644=CARTESIAN_POINT('Ctrl Pts',(40.9742125859198,-60.9855966398325,
-228.41692385506));
#207645=CARTESIAN_POINT('Ctrl Pts',(40.965979388266,-61.0001195637171,-228.410996850065));
#207646=CARTESIAN_POINT('Ctrl Pts',(40.9545231990119,-61.0203276738028,
-228.402749642383));
#207647=CARTESIAN_POINT('Ctrl Pts',(40.9437436672703,-61.0408032710641,
-228.393885042642));
#207648=CARTESIAN_POINT('Ctrl Pts',(40.9336502467295,-61.0615476677132,
-228.384396871472));
#207649=CARTESIAN_POINT('Ctrl Pts',(40.929608662109,-61.0698540920934,-228.380597639436));
#207650=CARTESIAN_POINT('Ctrl Pts',(40.92553780094,-61.0784981103401,-228.3765612754));
#207651=CARTESIAN_POINT('Ctrl Pts',(40.9216159438804,-61.0871276381461,
-228.372444588586));
#207652=CARTESIAN_POINT('Ctrl Pts',(40.9176158482466,-61.0959293195877,
-228.368245776466));
#207653=CARTESIAN_POINT('Ctrl Pts',(40.9137709112863,-61.1047157126402,
-228.363963477019));
#207654=CARTESIAN_POINT('Ctrl Pts',(40.9102260118624,-61.1131057492398,
-228.359796853342));
#207655=CARTESIAN_POINT('Ctrl Pts',(40.908812233677,-61.1164518669433,-228.358135118844));
#207656=CARTESIAN_POINT('Ctrl Pts',(40.907445684125,-61.1197348779016,-228.35649213395));
#207657=CARTESIAN_POINT('Ctrl Pts',(40.9061336970849,-61.1229304187023,
-228.354881812122));
#207658=CARTESIAN_POINT('Ctrl Pts',(40.9059057765971,-61.1234855531631,
-228.354602064437));
#207659=CARTESIAN_POINT('Ctrl Pts',(40.9056794946264,-61.1240379804454,
-228.354323359087));
#207660=CARTESIAN_POINT('Ctrl Pts',(40.9054548859916,-61.1245875752137,
-228.354045769407));
#207661=CARTESIAN_POINT('Ctrl Pts',(40.8895791691886,-61.163433859588,-228.334425263015));
#207662=CARTESIAN_POINT('Ctrl Pts',(40.8760959108351,-61.202729232473,-228.313004683474));
#207663=CARTESIAN_POINT('Ctrl Pts',(40.864938821336,-61.2424592911638,-228.289840584947));
#207664=CARTESIAN_POINT('Ctrl Pts',(40.8551443466649,-61.2773371196117,
-228.269505516709));
#207665=CARTESIAN_POINT('Ctrl Pts',(40.8471421184351,-61.3125510851886,
-228.247826182382));
#207666=CARTESIAN_POINT('Ctrl Pts',(40.8409152666239,-61.348111079235,-228.224809686116));
#207667=CARTESIAN_POINT('Ctrl Pts',(40.8348327040824,-61.3828470733333,
-228.202326530539));
#207668=CARTESIAN_POINT('Ctrl Pts',(40.8304445378103,-61.4179102691019,
-228.178569468885));
#207669=CARTESIAN_POINT('Ctrl Pts',(40.8277690023158,-61.4533105529692,
-228.153524940798));
#207670=CARTESIAN_POINT('Ctrl Pts',(40.8249932163602,-61.4900372609432,
-228.127542011598));
#207671=CARTESIAN_POINT('Ctrl Pts',(40.8240607946239,-61.5271238425471,
-228.100175491165));
#207672=CARTESIAN_POINT('Ctrl Pts',(40.8250357033287,-61.5645566624456,
-228.071404099149));
#207673=CARTESIAN_POINT('Ctrl Pts',(40.8251726188277,-61.5698137015823,
-228.067363464908));
#207674=CARTESIAN_POINT('Ctrl Pts',(40.8253472277531,-61.5750775224125,
-228.063295116071));
#207675=CARTESIAN_POINT('Ctrl Pts',(40.8255597807069,-61.5803480206386,
-228.059199003225));
#207676=CARTESIAN_POINT('Ctrl Pts',(40.825799634981,-61.5862954869228,-228.054576766009));
#207677=CARTESIAN_POINT('Ctrl Pts',(40.8261100272156,-61.5926975688732,
-228.049569932398));
#207678=CARTESIAN_POINT('Ctrl Pts',(40.8264578487316,-61.5987977399614,
-228.044768050139));
#207679=CARTESIAN_POINT('Ctrl Pts',(40.8266877729433,-61.6028302019118,
-228.041593810069));
#207680=CARTESIAN_POINT('Ctrl Pts',(40.8269329257887,-61.6067311348939,
-228.038509504216));
#207681=CARTESIAN_POINT('Ctrl Pts',(40.8271725319483,-61.6102864365788,
-228.035688802337));
#207682=CARTESIAN_POINT('Ctrl Pts',(40.8272131709247,-61.6108894420335,
-228.035210390441));
#207683=CARTESIAN_POINT('Ctrl Pts',(40.8272536360648,-61.6114825561387,
-228.034739531352));
#207684=CARTESIAN_POINT('Ctrl Pts',(40.8272938061133,-61.6120647388012,
-228.034277080873));
#207685=CARTESIAN_POINT('Ctrl Pts',(40.8298349940696,-61.6488940587812,
-228.00502211024));
#207686=CARTESIAN_POINT('Ctrl Pts',(40.8341898410855,-61.6853715561985,
-227.974947206424));
#207687=CARTESIAN_POINT('Ctrl Pts',(40.840294556687,-61.7215236844399,-227.944074086286));
#207688=CARTESIAN_POINT('Ctrl Pts',(40.8466081307678,-61.7589126726802,
-227.912144714988));
#207689=CARTESIAN_POINT('Ctrl Pts',(40.854793122881,-61.7959550152558,-227.879360657465));
#207690=CARTESIAN_POINT('Ctrl Pts',(40.86482559579,-61.8326735860296,-227.845723429335));
#207691=CARTESIAN_POINT('Ctrl Pts',(40.8745653337792,-61.8683207551688,
-227.813067693144));
#207692=CARTESIAN_POINT('Ctrl Pts',(40.8860468086191,-61.9036640700498,
-227.779606546507));
#207693=CARTESIAN_POINT('Ctrl Pts',(40.8992893740948,-61.9387038113221,
-227.745333169578));
#207694=CARTESIAN_POINT('Ctrl Pts',(40.9053795738278,-61.9548184398155,
-227.729570988798));
#207695=CARTESIAN_POINT('Ctrl Pts',(40.9118428318196,-61.9708685867213,
-227.713636893048));
#207696=CARTESIAN_POINT('Ctrl Pts',(40.9186838005535,-61.9868520978782,
-227.697530300764));
#207697=CARTESIAN_POINT('Ctrl Pts',(40.9224514188616,-61.9956549109891,
-227.688659701537));
#207698=CARTESIAN_POINT('Ctrl Pts',(40.9264807276567,-62.0047698498522,
-227.679399004713));
#207699=CARTESIAN_POINT('Ctrl Pts',(40.9305535053323,-62.013685526149,-227.67026325364));
#207700=CARTESIAN_POINT('Ctrl Pts',(40.9343385705297,-62.0219713739782,
-227.661772877737));
#207701=CARTESIAN_POINT('Ctrl Pts',(40.9381604199117,-62.0300854268991,
-227.653390637984));
#207702=CARTESIAN_POINT('Ctrl Pts',(40.9418110223868,-62.0376411022744,
-227.645531244992));
#207703=CARTESIAN_POINT('Ctrl Pts',(40.9419554686057,-62.0379400635409,
-227.645220266295));
#207704=CARTESIAN_POINT('Ctrl Pts',(40.9420996426571,-62.038238161741,-227.644910100089));
#207705=CARTESIAN_POINT('Ctrl Pts',(40.9422435309139,-62.0385353735754,
-227.644600772006));
#207706=CARTESIAN_POINT('Ctrl Pts',(41.0037900116267,-62.1656641806455,
-227.512289384515));
#207707=CARTESIAN_POINT('Ctrl Pts',(41.0857394019224,-62.2807520250138,
-227.377065009777));
#207708=CARTESIAN_POINT('Ctrl Pts',(41.1874522920715,-62.3844144545142,
-227.238927571877));
#207709=CARTESIAN_POINT('Ctrl Pts',(41.7563078823353,-62.3074742642099,
-227.60005));
#207710=CARTESIAN_POINT('Ctrl Pts',(41.7026267238965,-62.2527647791652,
-227.643792731266));
#207711=CARTESIAN_POINT('Ctrl Pts',(41.6565415403856,-62.200359156799,-227.684086045573));
#207712=CARTESIAN_POINT('Ctrl Pts',(41.5970055355346,-62.1269748350088,
-227.738766339681));
#207713=CARTESIAN_POINT('Ctrl Pts',(41.5787613895645,-62.1033815672565,
-227.756041513266));
#207714=CARTESIAN_POINT('Ctrl Pts',(41.5535989156551,-62.0694882409635,
-227.780515268765));
#207715=CARTESIAN_POINT('Ctrl Pts',(41.5415689308369,-62.0529154117129,
-227.792392926535));
#207716=CARTESIAN_POINT('Ctrl Pts',(41.5284587659491,-62.0342737779368,
-227.805623935743));
#207717=CARTESIAN_POINT('Ctrl Pts',(41.5230342538352,-62.0264370469646,
-227.811160687378));
#207718=CARTESIAN_POINT('Ctrl Pts',(41.5194606092816,-62.0212468923819,
-227.814822210717));
#207719=CARTESIAN_POINT('Ctrl Pts',(41.5185130669224,-62.0198696273061,
-227.815793580791));
#207720=CARTESIAN_POINT('Ctrl Pts',(41.4749543623288,-61.955929657224,-227.860770813693));
#207721=CARTESIAN_POINT('Ctrl Pts',(41.4402071580976,-61.8974857906177,
-227.900311593228));
#207722=CARTESIAN_POINT('Ctrl Pts',(41.3963536552126,-61.8135081173075,
-227.95506194786));
#207723=CARTESIAN_POINT('Ctrl Pts',(41.3831145126627,-61.7861294546533,
-227.97255652996));
#207724=CARTESIAN_POINT('Ctrl Pts',(41.3651951560785,-61.7461085650297,
-227.997655201073));
#207725=CARTESIAN_POINT('Ctrl Pts',(41.3567204361325,-61.7263597795088,
-228.009919084671));
#207726=CARTESIAN_POINT('Ctrl Pts',(41.3476551381641,-61.7038037315272,
-228.023728678121));
#207727=CARTESIAN_POINT('Ctrl Pts',(41.343943347233,-61.6942433384729,-228.029540639883));
#207728=CARTESIAN_POINT('Ctrl Pts',(41.3415070331292,-61.6878937067045,
-228.033391670802));
#207729=CARTESIAN_POINT('Ctrl Pts',(41.3407858071833,-61.6860066029679,
-228.034535283631));
#207730=CARTESIAN_POINT('Ctrl Pts',(41.3126011552024,-61.6107572390613,
-228.079959711279));
#207731=CARTESIAN_POINT('Ctrl Pts',(41.2945210437306,-61.5431299204009,
-228.118474409734));
#207732=CARTESIAN_POINT('Ctrl Pts',(41.2787043693704,-61.4478231136571,
-228.169410280855));
#207733=CARTESIAN_POINT('Ctrl Pts',(41.2753166770858,-61.4170759345204,
-228.185255180313));
#207734=CARTESIAN_POINT('Ctrl Pts',(41.2729000846091,-61.372646611079,-228.207308552331));
#207735=CARTESIAN_POINT('Ctrl Pts',(41.2723581451704,-61.3508546926235,
-228.2179071948));
#207736=CARTESIAN_POINT('Ctrl Pts',(41.2728580181042,-61.3262039384022,
-228.229524784819));
#207737=CARTESIAN_POINT('Ctrl Pts',(41.27331130909,-61.3158084787955,-228.234344013731));
#207738=CARTESIAN_POINT('Ctrl Pts',(41.2736662371782,-61.308916144085,-228.237521390818));
#207739=CARTESIAN_POINT('Ctrl Pts',(41.2737659913982,-61.307031081556,-228.238389501627));
#207740=CARTESIAN_POINT('Ctrl Pts',(41.2847906540784,-61.1436769906793,
-228.312841875131));
#207741=CARTESIAN_POINT('Ctrl Pts',(41.3528351981069,-61.0176483773379,
-228.35005));
#207742=CARTESIAN_POINT('Ctrl Pts',(41.4636310035131,-60.9383233439604,
-228.35005));
#207743=CARTESIAN_POINT('Origin',(48.2737085028446,-66.8079885321834,-218.85005));
#207744=CARTESIAN_POINT('',(49.0417551583074,-68.6546353135231,-218.35005));
#207745=CARTESIAN_POINT('',(48.8497434944417,-68.1929736181882,-218.85005));
#207746=CARTESIAN_POINT('Origin',(49.0417551583074,-68.6546353135231,-218.85005));
#207747=CARTESIAN_POINT('Origin',(48.2737085028446,-66.8079885321834,-218.85005));
#207748=CARTESIAN_POINT('Origin',(48.2737085028446,-66.8079885321834,-218.35005));
#207749=CARTESIAN_POINT('Ctrl Pts',(41.1874522920715,-62.3844144545142,
-227.238927571877));
#207750=CARTESIAN_POINT('Ctrl Pts',(41.533590072875,-62.0804900295131,-227.265723268608));
#207751=CARTESIAN_POINT('Ctrl Pts',(41.7563078823354,-62.3074742642099,
-227.60005));
#207752=CARTESIAN_POINT('Ctrl Pts',(42.9977586927641,-64.2294190860942,
-224.780329817623));
#207753=CARTESIAN_POINT('Ctrl Pts',(43.3439332486946,-63.9255124877361,
-224.807072796208));
#207754=CARTESIAN_POINT('Ctrl Pts',(43.5663090949841,-64.1521482085568,
-225.141881592783));
#207755=CARTESIAN_POINT('Ctrl Pts',(44.8096404055398,-66.0773673148437,
-222.324535970207));
#207756=CARTESIAN_POINT('Ctrl Pts',(45.1633560000594,-65.7797884513162,
-222.341036594742));
#207757=CARTESIAN_POINT('Ctrl Pts',(45.3784193710744,-65.9989716179707,
-222.686835360681));
#207758=CARTESIAN_POINT('Ctrl Pts',(46.6323854374629,-67.9411854921914,
-219.886423382228));
#207759=CARTESIAN_POINT('Ctrl Pts',(46.9799636370447,-67.6311953742356,
-219.91012892279));
#207760=CARTESIAN_POINT('Ctrl Pts',(47.2030337908495,-67.8585387028531,
-220.250747695207));
#207761=CARTESIAN_POINT('',(47.2030337908494,-67.858538702853,-220.250747695207));
#207762=CARTESIAN_POINT('',(46.6323854374629,-67.9411854921913,-219.886423382228));
#207763=CARTESIAN_POINT('Origin',(46.8461422201844,-68.2087220930763,-220.250747695207));
#207764=CARTESIAN_POINT('Ctrl Pts',(41.1874522920715,-62.3844144545142,
-227.238927571877));
#207765=CARTESIAN_POINT('Ctrl Pts',(41.6650043735109,-62.8711197999119,
-226.59035864759));
#207766=CARTESIAN_POINT('Ctrl Pts',(42.1301866064175,-63.3454119978617,
-225.959062309233));
#207767=CARTESIAN_POINT('Ctrl Pts',(42.8097176035461,-64.0383310888314,
-225.038026680594));
#207768=CARTESIAN_POINT('Ctrl Pts',(43.1449188366604,-64.3801644733344,
-224.583986085998));
#207769=CARTESIAN_POINT('Ctrl Pts',(43.528027568592,-64.7709351764863,-224.065607193486));
#207770=CARTESIAN_POINT('Ctrl Pts',(43.717592476361,-64.9643223419007,-223.809251530859));
#207771=CARTESIAN_POINT('Ctrl Pts',(43.8118775094903,-65.0605177877102,
-223.681782145453));
#207772=CARTESIAN_POINT('Ctrl Pts',(43.8588955882238,-65.1084912135109,
-223.618224564227));
#207773=CARTESIAN_POINT('Ctrl Pts',(43.8790195202237,-65.1290246426943,
-223.591023553304));
#207774=CARTESIAN_POINT('Ctrl Pts',(43.8924295465235,-65.1427076848833,
-223.572897979902));
#207775=CARTESIAN_POINT('Ctrl Pts',(43.8984888898217,-65.1488904466342,
-223.564708078702));
#207776=CARTESIAN_POINT('Ctrl Pts',(44.8455797929338,-66.1152831054553,
-222.284638320274));
#207777=CARTESIAN_POINT('Ctrl Pts',(45.753629864441,-67.0426283261149,-221.061851095243));
#207778=CARTESIAN_POINT('Ctrl Pts',(46.6323854374629,-67.9411854921913,
-219.886423382228));
#207779=CARTESIAN_POINT('Ctrl Pts',(47.2030337908494,-67.858538702853,-220.250747695207));
#207780=CARTESIAN_POINT('Ctrl Pts',(45.378411470404,-65.9989635659536,-222.68684590906));
#207781=CARTESIAN_POINT('Ctrl Pts',(43.5663164045416,-64.1521556581376,
-225.14187166565));
#207782=CARTESIAN_POINT('Ctrl Pts',(41.7563078823354,-62.3074742642099,
-227.60005));
#207783=CARTESIAN_POINT('Ctrl Pts',(48.8497434944417,-68.1929736181882,
-218.85005));
#207784=CARTESIAN_POINT('Ctrl Pts',(48.8497434944417,-68.1929736181882,
-218.35005));
#207785=CARTESIAN_POINT('Ctrl Pts',(49.0417551583074,-68.6546353135231,
-218.35005));
#207786=CARTESIAN_POINT('Ctrl Pts',(48.7287312757308,-68.2433043207298,
-218.85004996112));
#207787=CARTESIAN_POINT('Ctrl Pts',(48.7557592223196,-68.232063046543,-218.382837715704));
#207788=CARTESIAN_POINT('Ctrl Pts',(48.8914370751605,-68.6805168842225,
-218.35005));
#207789=CARTESIAN_POINT('Ctrl Pts',(48.6040131804169,-68.2768832027127,
-218.836912439222));
#207790=CARTESIAN_POINT('Ctrl Pts',(48.6402644556944,-68.2689304282727,
-218.402170544444));
#207791=CARTESIAN_POINT('Ctrl Pts',(48.7342750095003,-68.6918682705249,
-218.342169793108));
#207792=CARTESIAN_POINT('Ctrl Pts',(48.4757604447939,-68.2943179077776,
-218.82266550408));
#207793=CARTESIAN_POINT('Ctrl Pts',(48.5093251395215,-68.2897551158004,
-218.412348259396));
#207794=CARTESIAN_POINT('Ctrl Pts',(48.5701931618903,-68.6892604152372,
-218.333619302448));
#207795=CARTESIAN_POINT('',(48.5701931618903,-68.6892604152372,-218.333619302448));
#207796=CARTESIAN_POINT('',(48.4757604447939,-68.2943179077777,-218.82266550408));
#207797=CARTESIAN_POINT('Origin',(48.5431110921104,-68.7897610329756,-218.82266550408));
#207798=CARTESIAN_POINT('Ctrl Pts',(48.8497434944417,-68.1929736181882,
-218.85005));
#207799=CARTESIAN_POINT('Ctrl Pts',(48.8253786724137,-68.2031072941346,
-218.850049992172));
#207800=CARTESIAN_POINT('Ctrl Pts',(48.7996420667697,-68.213071276654,-218.849493836655));
#207801=CARTESIAN_POINT('Ctrl Pts',(48.7724981693848,-68.2226546374388,
-218.848378544969));
#207802=CARTESIAN_POINT('Ctrl Pts',(48.7693432105752,-68.2237685198008,
-218.848248913646));
#207803=CARTESIAN_POINT('Ctrl Pts',(48.7661692323878,-68.2248772454103,
-218.848111784651));
#207804=CARTESIAN_POINT('Ctrl Pts',(48.7629761734588,-68.225980471413,-218.84796719926));
#207805=CARTESIAN_POINT('Ctrl Pts',(48.7476437968494,-68.2312779234595,
-218.847272931563));
#207806=CARTESIAN_POINT('Ctrl Pts',(48.7318720892122,-68.2364484273792,
-218.846405096242));
#207807=CARTESIAN_POINT('Ctrl Pts',(48.7156578079315,-68.2414522477113,
-218.845363694404));
#207808=CARTESIAN_POINT('Ctrl Pts',(48.7075506672912,-68.2439541578774,
-218.844842993486));
#207809=CARTESIAN_POINT('Ctrl Pts',(48.6993328825448,-68.2464143815189,
-218.844278900983));
#207810=CARTESIAN_POINT('Ctrl Pts',(48.6910043184336,-68.2488278002158,
-218.843671417198));
#207811=CARTESIAN_POINT('Ctrl Pts',(48.686840036378,-68.2500345095643,-218.843367675305));
#207812=CARTESIAN_POINT('Ctrl Pts',(48.6826480594132,-68.2512295172066,
-218.843053085484));
#207813=CARTESIAN_POINT('Ctrl Pts',(48.6784283853964,-68.252412176893,-218.842727562152));
#207814=CARTESIAN_POINT('Ctrl Pts',(48.6751994187233,-68.2533171682971,
-218.842478466135));
#207815=CARTESIAN_POINT('Ctrl Pts',(48.6711530911778,-68.2544347700194,
-218.842158889697));
#207816=CARTESIAN_POINT('Ctrl Pts',(48.6681283537951,-68.2552591312216,
-218.841915521378));
#207817=CARTESIAN_POINT('Ctrl Pts',(48.6672003078158,-68.2555120606506,
-218.841840851427));
#207818=CARTESIAN_POINT('Ctrl Pts',(48.666368517125,-68.2557377718834,-218.841773526889));
#207819=CARTESIAN_POINT('Ctrl Pts',(48.6656862746315,-68.255922463752,-218.841718135008));
#207820=CARTESIAN_POINT('Ctrl Pts',(48.649737121747,-68.2602401057584,-218.840423208958));
#207821=CARTESIAN_POINT('Ctrl Pts',(48.6318323557602,-68.2648053884177,
-218.838855344496));
#207822=CARTESIAN_POINT('Ctrl Pts',(48.6119507030164,-68.2694009179544,
-218.836970612394));
#207823=CARTESIAN_POINT('Ctrl Pts',(48.5929129470642,-68.2738013856076,
-218.835165879645));
#207824=CARTESIAN_POINT('Ctrl Pts',(48.5720624686907,-68.2782291657522,
-218.833069427729));
#207825=CARTESIAN_POINT('Ctrl Pts',(48.5493736675765,-68.2824612289884,
-218.830677796369));
#207826=CARTESIAN_POINT('Ctrl Pts',(48.5285405771963,-68.2863471529494,
-218.828481775872));
#207827=CARTESIAN_POINT('Ctrl Pts',(48.5061574779594,-68.2900676146866,
-218.826036371646));
#207828=CARTESIAN_POINT('Ctrl Pts',(48.4821999960562,-68.2934285274618,
-218.82338018019));
#207829=CARTESIAN_POINT('Ctrl Pts',(48.4800659796662,-68.2937279012849,
-218.823143579527));
#207830=CARTESIAN_POINT('Ctrl Pts',(48.4779194688382,-68.2940244095746,
-218.822905338518));
#207831=CARTESIAN_POINT('Ctrl Pts',(48.4757604447939,-68.2943179077776,
-218.82266550408));
#207832=CARTESIAN_POINT('Ctrl Pts',(48.5701931618903,-68.6892604152372,
-218.333619302448));
#207833=CARTESIAN_POINT('Ctrl Pts',(48.7359603200225,-68.6918950616687,
-218.342257615425));
#207834=CARTESIAN_POINT('Ctrl Pts',(48.8931846693406,-68.6802159916351,
-218.35005));
#207835=CARTESIAN_POINT('Ctrl Pts',(49.0417551583074,-68.6546353135231,
-218.35005));
#207836=CARTESIAN_POINT('Ctrl Pts',(48.4757604447937,-68.2943179077776,
-218.82266550408));
#207837=CARTESIAN_POINT('Ctrl Pts',(48.3620909039911,-68.309770170134,-218.591540694519));
#207838=CARTESIAN_POINT('Ctrl Pts',(48.3245605310988,-68.5271120961852,
-218.457629631481));
#207839=CARTESIAN_POINT('Ctrl Pts',(48.2145031263758,-68.3298332850564,
-218.997150144364));
#207840=CARTESIAN_POINT('Ctrl Pts',(48.0565790003986,-68.3305373905487,
-218.760296345904));
#207841=CARTESIAN_POINT('Ctrl Pts',(47.9776226084149,-68.5733796207043,
-218.632054575151));
#207842=CARTESIAN_POINT('Ctrl Pts',(47.9672522644602,-68.2939398715798,
-219.226769248345));
#207843=CARTESIAN_POINT('Ctrl Pts',(47.7753561891483,-68.2571865053622,
-218.980775448776));
#207844=CARTESIAN_POINT('Ctrl Pts',(47.6490670814862,-68.5245197011494,
-218.861741583456));
#207845=CARTESIAN_POINT('Ctrl Pts',(47.539630313305,-68.1358047923417,-219.716553805522));
#207846=CARTESIAN_POINT('Ctrl Pts',(47.3075378575116,-68.013479625276,-219.436238572541));
#207847=CARTESIAN_POINT('Ctrl Pts',(47.0804817541883,-68.3120180317949,
-219.351800153131));
#207848=CARTESIAN_POINT('Ctrl Pts',(47.354847997338,-68.013261091513,-219.980493179131));
#207849=CARTESIAN_POINT('Ctrl Pts',(47.1165089694488,-67.8332337800358,
-219.681063518939));
#207850=CARTESIAN_POINT('Ctrl Pts',(46.8345979831258,-68.1479546277615,
-219.615942902681));
#207851=CARTESIAN_POINT('Ctrl Pts',(47.2030337908474,-67.858538702855,-220.250747695207));
#207852=CARTESIAN_POINT('Ctrl Pts',(46.9799636370427,-67.6311953742376,
-219.91012892279));
#207853=CARTESIAN_POINT('Ctrl Pts',(46.6323854374609,-67.9411854921933,
-219.886423382227));
#207854=CARTESIAN_POINT('',(48.3245605310987,-68.5271120961857,-218.45762963148));
#207855=CARTESIAN_POINT('Origin',(48.5431110921103,-68.7897610329758,-218.82266550408));
#207856=CARTESIAN_POINT('Ctrl Pts',(46.632385437463,-67.9411854921914,-219.886423382228));
#207857=CARTESIAN_POINT('Ctrl Pts',(46.6789349826013,-67.9887839692199,
-219.824158485406));
#207858=CARTESIAN_POINT('Ctrl Pts',(46.7272112617812,-68.0335239722974,
-219.763011130579));
#207859=CARTESIAN_POINT('Ctrl Pts',(46.7770922567545,-68.0754781330116,
-219.702981480643));
#207860=CARTESIAN_POINT('Ctrl Pts',(46.8296502730403,-68.1196838964142,
-219.639730149737));
#207861=CARTESIAN_POINT('Ctrl Pts',(46.8839897850005,-68.160797451316,-219.577719302768));
#207862=CARTESIAN_POINT('Ctrl Pts',(46.9400226203996,-68.1988812889257,
-219.516936401576));
#207863=CARTESIAN_POINT('Ctrl Pts',(46.9985251342596,-68.2386436929114,
-219.453474460125));
#207864=CARTESIAN_POINT('Ctrl Pts',(47.0588761815705,-68.2751048341591,
-219.391348551543));
#207865=CARTESIAN_POINT('Ctrl Pts',(47.1210077877848,-68.3082886731283,
-219.330562267133));
#207866=CARTESIAN_POINT('Ctrl Pts',(47.1831393939991,-68.3414725120975,
-219.269775982722));
#207867=CARTESIAN_POINT('Ctrl Pts',(47.2470552838015,-68.3713804372138,
-219.210326169212));
#207868=CARTESIAN_POINT('Ctrl Pts',(47.3127122895345,-68.3979939965537,
-219.152234411495));
#207869=CARTESIAN_POINT('Ctrl Pts',(47.3221962661813,-68.4018382531178,
-219.143843214434));
#207870=CARTESIAN_POINT('Ctrl Pts',(47.3312777219034,-68.4054398649159,
-219.135865758659));
#207871=CARTESIAN_POINT('Ctrl Pts',(47.3406919758767,-68.409094347228,-219.127653243753));
#207872=CARTESIAN_POINT('Ctrl Pts',(47.3480787307764,-68.4119617826299,
-219.121209415608));
#207873=CARTESIAN_POINT('Ctrl Pts',(47.3556708314958,-68.4148611232482,
-219.114621070859));
#207874=CARTESIAN_POINT('Ctrl Pts',(47.3638354720275,-68.4179171786934,
-219.107580695432));
#207875=CARTESIAN_POINT('Ctrl Pts',(47.364148530177,-68.418034357528,-219.107310745163));
#207876=CARTESIAN_POINT('Ctrl Pts',(47.3644616002814,-68.4181514532561,
-219.107040847959));
#207877=CARTESIAN_POINT('Ctrl Pts',(47.3647746823481,-68.4182684659211,
-219.10677100378));
#207878=CARTESIAN_POINT('Ctrl Pts',(47.4110307172631,-68.4355563993204,
-219.066903112672));
#207879=CARTESIAN_POINT('Ctrl Pts',(47.4576985949707,-68.4510436336742,
-219.028094295378));
#207880=CARTESIAN_POINT('Ctrl Pts',(47.5047241972111,-68.4647642254001,
-218.990341332514));
#207881=CARTESIAN_POINT('Ctrl Pts',(47.5329030678403,-68.4729859335927,
-218.967718850169));
#207882=CARTESIAN_POINT('Ctrl Pts',(47.5612113910329,-68.4805730273755,
-218.945475130944));
#207883=CARTESIAN_POINT('Ctrl Pts',(47.5896454632259,-68.4875294857434,
-218.923607470301));
#207884=CARTESIAN_POINT('Ctrl Pts',(47.6277488305346,-68.4968515584511,
-218.894303489499));
#207885=CARTESIAN_POINT('Ctrl Pts',(47.6660759138159,-68.5050408980252,
-218.865676249708));
#207886=CARTESIAN_POINT('Ctrl Pts',(47.7046218854028,-68.5120873419134,
-218.837731470339));
#207887=CARTESIAN_POINT('Ctrl Pts',(47.7238948711963,-68.5156105638575,
-218.823759080654));
#207888=CARTESIAN_POINT('Ctrl Pts',(47.7432236774575,-68.5188456333958,
-218.809958418662));
#207889=CARTESIAN_POINT('Ctrl Pts',(47.7626047403424,-68.5217969580725,
-218.796327863849));
#207890=CARTESIAN_POINT('Ctrl Pts',(47.7729855113983,-68.5233777292595,
-218.789027146147));
#207891=CARTESIAN_POINT('Ctrl Pts',(47.7829426565521,-68.524813935548,-218.782081134656));
#207892=CARTESIAN_POINT('Ctrl Pts',(47.7931789075124,-68.5262114580297,
-218.774996323705));
#207893=CARTESIAN_POINT('Ctrl Pts',(47.8020538981449,-68.527423132009,-218.768853681144));
#207894=CARTESIAN_POINT('Ctrl Pts',(47.8111389551874,-68.5286052992481,
-218.762606853945));
#207895=CARTESIAN_POINT('Ctrl Pts',(47.8209032985487,-68.5298001944143,
-218.755946475681));
#207896=CARTESIAN_POINT('Ctrl Pts',(47.8790078311355,-68.5369106392807,
-218.716312661959));
#207897=CARTESIAN_POINT('Ctrl Pts',(47.9371237250222,-68.5414328500945,
-218.678502918883));
#207898=CARTESIAN_POINT('Ctrl Pts',(47.9951858050162,-68.5434012407283,
-218.642520231142));
#207899=CARTESIAN_POINT('Ctrl Pts',(48.0542593885108,-68.5454039228311,
-218.605910686516));
#207900=CARTESIAN_POINT('Ctrl Pts',(48.1132779188672,-68.5447637771468,
-218.571191543065));
#207901=CARTESIAN_POINT('Ctrl Pts',(48.1722176288345,-68.5414882566244,
-218.538361397313));
#207902=CARTESIAN_POINT('Ctrl Pts',(48.2230544566548,-68.538663046373,-218.510044656906));
#207903=CARTESIAN_POINT('Ctrl Pts',(48.2738336083459,-68.5338770215185,
-218.483132870144));
#207904=CARTESIAN_POINT('Ctrl Pts',(48.3245605310988,-68.5271120961852,
-218.457629631481));
#207905=CARTESIAN_POINT('',(48.2736913638528,-68.3080354249668,-218.970411512989));
#207906=CARTESIAN_POINT('Ctrl Pts',(48.2736913638528,-68.3080354249668,
-218.970411512989));
#207907=CARTESIAN_POINT('Ctrl Pts',(48.2352706160841,-68.3080419600251,
-219.000929763438));
#207908=CARTESIAN_POINT('Ctrl Pts',(48.1961538364747,-68.3065666156675,
-219.033386630441));
#207909=CARTESIAN_POINT('Ctrl Pts',(48.1564716235175,-68.3034518671295,
-219.067833966359));
#207910=CARTESIAN_POINT('Ctrl Pts',(48.1190450812612,-68.3005141713942,
-219.100323199627));
#207911=CARTESIAN_POINT('Ctrl Pts',(48.0811155483893,-68.2961179360676,
-219.134583250583));
#207912=CARTESIAN_POINT('Ctrl Pts',(48.0428230551683,-68.2901435429112,
-219.170624127822));
#207913=CARTESIAN_POINT('Ctrl Pts',(48.0120582244176,-68.2853436153318,
-219.199579972561));
#207914=CARTESIAN_POINT('Ctrl Pts',(47.9810624393644,-68.2795258339341,
-219.229681930507));
#207915=CARTESIAN_POINT('Ctrl Pts',(47.9499142999773,-68.2726338250037,
-219.260926465793));
#207916=CARTESIAN_POINT('Ctrl Pts',(47.9173884187917,-68.2654369693324,
-219.293553006651));
#207917=CARTESIAN_POINT('Ctrl Pts',(47.884690621732,-68.2570677822824,-219.327430912405));
#207918=CARTESIAN_POINT('Ctrl Pts',(47.8519122600643,-68.2474620614157,
-219.362556430075));
#207919=CARTESIAN_POINT('Ctrl Pts',(47.831598938395,-68.2415092288792,-219.384324325203));
#207920=CARTESIAN_POINT('Ctrl Pts',(47.811255962524,-68.2350819225415,-219.406569983772));
#207921=CARTESIAN_POINT('Ctrl Pts',(47.7909033810425,-68.2281634706586,
-219.429295593734));
#207922=CARTESIAN_POINT('Ctrl Pts',(47.7784142497046,-68.2239180409426,
-219.443240907147));
#207923=CARTESIAN_POINT('Ctrl Pts',(47.7659232461178,-68.2194881738068,
-219.457365090839));
#207924=CARTESIAN_POINT('Ctrl Pts',(47.7534412888826,-68.2148723319607,
-219.471661526933));
#207925=CARTESIAN_POINT('Ctrl Pts',(47.7408887066471,-68.21023037291,-219.486038854652));
#207926=CARTESIAN_POINT('Ctrl Pts',(47.7283302837597,-68.2053993054349,
-219.500603213225));
#207927=CARTESIAN_POINT('Ctrl Pts',(47.7157811377292,-68.2003778392676,
-219.515344195403));
#207928=CARTESIAN_POINT('Ctrl Pts',(47.7069924423551,-68.1968610950709,
-219.525667925922));
#207929=CARTESIAN_POINT('Ctrl Pts',(47.6982072159195,-68.1932505778963,
-219.536079512527));
#207930=CARTESIAN_POINT('Ctrl Pts',(47.6894276522935,-68.1895447985078,
-219.546578761834));
#207931=CARTESIAN_POINT('Ctrl Pts',(47.6850378704804,-68.1876919088135,
-219.551828386488));
#207932=CARTESIAN_POINT('Ctrl Pts',(47.6806495046123,-68.1858152041822,
-219.557099926126));
#207933=CARTESIAN_POINT('Ctrl Pts',(47.6762628309838,-68.1839145024519,
-219.562393351676));
#207934=CARTESIAN_POINT('Ctrl Pts',(47.6751661625767,-68.1834393270193,
-219.563716708063));
#207935=CARTESIAN_POINT('Ctrl Pts',(47.6740695999485,-68.1829626517843,
-219.565041432296));
#207936=CARTESIAN_POINT('Ctrl Pts',(47.6729731474406,-68.1824844739318,
-219.566367523873));
#207937=CARTESIAN_POINT('Ctrl Pts',(47.6727519650219,-68.1823880132704,
-219.566635030345));
#207938=CARTESIAN_POINT('Ctrl Pts',(47.6725293350301,-68.1822908590618,
-219.566904347797));
#207939=CARTESIAN_POINT('Ctrl Pts',(47.6723008586559,-68.182191085278,-219.567180803719));
#207940=CARTESIAN_POINT('Ctrl Pts',(47.6694450526422,-68.1809439779004,
-219.570636322859));
#207941=CARTESIAN_POINT('Ctrl Pts',(47.6659219370643,-68.1793899298261,
-219.574914316411));
#207942=CARTESIAN_POINT('Ctrl Pts',(47.6637661869299,-68.1784326234025,
-219.577538166137));
#207943=CARTESIAN_POINT('Ctrl Pts',(47.663529499819,-68.1783275174869,-219.577826247488));
#207944=CARTESIAN_POINT('Ctrl Pts',(47.6633092672032,-68.1782296454147,
-219.5780943722));
#207945=CARTESIAN_POINT('Ctrl Pts',(47.6631081652735,-68.1781402268487,
-219.578339252732));
#207946=CARTESIAN_POINT('Ctrl Pts',(47.6312267100201,-68.1639643608312,
-219.617161096537));
#207947=CARTESIAN_POINT('Ctrl Pts',(47.5979339811122,-68.1478376530234,
-219.65898213675));
#207948=CARTESIAN_POINT('Ctrl Pts',(47.5635841092145,-68.1294106324221,
-219.703868909107));
#207949=CARTESIAN_POINT('Ctrl Pts',(47.5312117306429,-68.1120444399476,
-219.746171587613));
#207950=CARTESIAN_POINT('Ctrl Pts',(47.4979006949716,-68.092634432448,-219.791197643804));
#207951=CARTESIAN_POINT('Ctrl Pts',(47.4639844702321,-68.07088947511,-219.838976427383));
#207952=CARTESIAN_POINT('Ctrl Pts',(47.4313133363501,-68.0499427919839,
-219.885001214842));
#207953=CARTESIAN_POINT('Ctrl Pts',(47.398080746371,-68.0268288922644,-219.933580747127));
#207954=CARTESIAN_POINT('Ctrl Pts',(47.3646176674441,-68.0012979457342,
-219.984709699179));
#207955=CARTESIAN_POINT('Ctrl Pts',(47.3328901754178,-67.9770911802948,
-220.033186810986));
#207956=CARTESIAN_POINT('Ctrl Pts',(47.3009556582199,-67.9507112332735,
-220.083955944682));
#207957=CARTESIAN_POINT('Ctrl Pts',(47.269124158351,-67.9219610284792,-220.136979491753));
#207958=CARTESIAN_POINT('Ctrl Pts',(47.2470063865729,-67.9019842610999,
-220.173822327241));
#207959=CARTESIAN_POINT('Ctrl Pts',(47.2249389168298,-67.8808634476479,
-220.211752930696));
#207960=CARTESIAN_POINT('Ctrl Pts',(47.2030337908474,-67.858538702855,-220.250747695207));
#207961=CARTESIAN_POINT('Origin',(48.3024486247851,-65.8934766456585,-221.196305192212));
#207962=CARTESIAN_POINT('Origin',(48.5431110921103,-68.7897610329758,-218.82266550408));
#207963=CARTESIAN_POINT('Origin',(48.5431110921103,-68.7897610329758,-218.82266550408));
#207964=CARTESIAN_POINT('Ctrl Pts',(49.9129432931154,30.3691563923977,-227.499480149477));
#207965=CARTESIAN_POINT('Ctrl Pts',(49.6184756168536,30.1420169376964,-227.148453859162));
#207966=CARTESIAN_POINT('Ctrl Pts',(49.9837284343871,29.7888486466285,-227.087470733639));
#207967=CARTESIAN_POINT('Ctrl Pts',(49.7890584560673,30.2238721235565,-227.617517102611));
#207968=CARTESIAN_POINT('Ctrl Pts',(49.5695507897331,29.9909534013765,-227.289688948551));
#207969=CARTESIAN_POINT('Ctrl Pts',(49.8665188865492,29.6366170163525,-227.284491638227));
#207970=CARTESIAN_POINT('Ctrl Pts',(49.6516701724817,30.1008771252358,-227.734473228363));
#207971=CARTESIAN_POINT('Ctrl Pts',(49.4836503780786,29.8530854215471,-227.451963630924));
#207972=CARTESIAN_POINT('Ctrl Pts',(49.7240534002376,29.5185044777796,-227.479632631849));
#207973=CARTESIAN_POINT('Ctrl Pts',(49.3886607896581,29.9360305472667,-227.932360963694));
#207974=CARTESIAN_POINT('Ctrl Pts',(49.2742353859129,29.682693950235,-227.736609390718));
#207975=CARTESIAN_POINT('Ctrl Pts',(49.4281098110363,29.3861258524904,-227.809829648684));
#207976=CARTESIAN_POINT('Ctrl Pts',(49.2735716953388,29.882741984255,-228.012019018908));
#207977=CARTESIAN_POINT('Ctrl Pts',(49.1732865590743,29.6308954154206,-227.853520161143));
#207978=CARTESIAN_POINT('Ctrl Pts',(49.2924069787687,29.3532300095823,-227.942750035685));
#207979=CARTESIAN_POINT('Ctrl Pts',(49.0943862810714,29.8358745178422,-228.122462272144));
#207980=CARTESIAN_POINT('Ctrl Pts',(49.0001873355215,29.5964093801985,-228.017396499293));
#207981=CARTESIAN_POINT('Ctrl Pts',(49.0692583324707,29.3499433053121,-228.127035773479));
#207982=CARTESIAN_POINT('Ctrl Pts',(49.0341585258203,29.8261040960875,-228.157331139179));
#207983=CARTESIAN_POINT('Ctrl Pts',(48.9401951728418,29.592107178363,-228.069035448677));
#207984=CARTESIAN_POINT('Ctrl Pts',(48.9922826040891,29.356783950037,-228.185219179292));
#207985=CARTESIAN_POINT('Ctrl Pts',(48.9155060353659,29.8208605820001,-228.220674964975));
#207986=CARTESIAN_POINT('Ctrl Pts',(48.8177391420467,29.6007095174117,-228.162636460521));
#207987=CARTESIAN_POINT('Ctrl Pts',(48.8360255565098,29.3888574699875,-228.290916415101));
#207988=CARTESIAN_POINT('Ctrl Pts',(48.8558606667612,29.8254987747837,-228.249737935875));
#207989=CARTESIAN_POINT('Ctrl Pts',(48.7537342504269,29.6136686499989,-228.205811972947));
#207990=CARTESIAN_POINT('Ctrl Pts',(48.7550839596696,29.4146403264887,-228.339409706525));
#207991=CARTESIAN_POINT('Ctrl Pts',(48.6420919128915,29.8753757465965,-228.341028197144));
#207992=CARTESIAN_POINT('Ctrl Pts',(48.5186265173263,29.6983851148206,-228.339000179185));
#207993=CARTESIAN_POINT('Ctrl Pts',(48.4540259802448,29.5512136888258,-228.491735739523));
#207994=CARTESIAN_POINT('Ctrl Pts',(48.5064500994514,29.983068024979,-228.369467059033));
#207995=CARTESIAN_POINT('Ctrl Pts',(48.3448350811457,29.8430513441803,-228.381209650087));
#207996=CARTESIAN_POINT('Ctrl Pts',(48.2378026611094,29.7390715475708,-228.539159295418));
#207997=CARTESIAN_POINT('Ctrl Pts',(48.4475474979323,30.1465475641224,-228.335963042699));
#207998=CARTESIAN_POINT('Ctrl Pts',(48.2552013856293,30.0316164665649,-228.324119572824));
#207999=CARTESIAN_POINT('Ctrl Pts',(48.1059399365173,29.9750822258506,-228.483236405913));
#208000=CARTESIAN_POINT('',(48.2384287873563,29.7860380279371,-228.505869818703));
#208001=CARTESIAN_POINT('',(48.515339402069,30.020261242545,-228.35005));
#208002=CARTESIAN_POINT('Origin',(48.515339402069,30.020261242545,-228.85005));
#208003=CARTESIAN_POINT('',(49.8031531494471,30.2499539750197,-227.60005));
#208004=CARTESIAN_POINT('Ctrl Pts',(49.8031531494471,30.2499539750197,-227.60005));
#208005=CARTESIAN_POINT('Ctrl Pts',(49.7527362723413,30.1993679966667,-227.644974522657));
#208006=CARTESIAN_POINT('Ctrl Pts',(49.7041257946578,30.1562841819435,-227.686309984401));
#208007=CARTESIAN_POINT('Ctrl Pts',(49.6358287764031,30.1010089879944,-227.742300319835));
#208008=CARTESIAN_POINT('Ctrl Pts',(49.6138301469231,30.0841450753157,-227.759970768332));
#208009=CARTESIAN_POINT('Ctrl Pts',(49.5821921102083,30.0609822914565,-227.784975491548));
#208010=CARTESIAN_POINT('Ctrl Pts',(49.566712728017,30.0499345103878,-227.797103193557));
#208011=CARTESIAN_POINT('Ctrl Pts',(49.549289886841,30.0379373173742,-227.810599354216));
#208012=CARTESIAN_POINT('Ctrl Pts',(49.5419635975734,30.0329825325858,-227.816244118858));
#208013=CARTESIAN_POINT('Ctrl Pts',(49.5371111255115,30.0297204039543,-227.819976409313));
#208014=CARTESIAN_POINT('Ctrl Pts',(49.5358192723333,30.0288527682603,-227.820969727432));
#208015=CARTESIAN_POINT('Ctrl Pts',(49.4761015676757,29.9891895263879,-227.866745295705));
#208016=CARTESIAN_POINT('Ctrl Pts',(49.4212428073257,29.9579805853916,-227.906937128057));
#208017=CARTESIAN_POINT('Ctrl Pts',(49.3421216382348,29.919204999993,-227.962493464653));
#208018=CARTESIAN_POINT('Ctrl Pts',(49.3162749091124,29.9076202744173,-227.980228558398));
#208019=CARTESIAN_POINT('Ctrl Pts',(49.2784287290678,29.8921209136238,-228.005645523579));
#208020=CARTESIAN_POINT('Ctrl Pts',(49.2597364927902,29.8848407893681,-228.018057957077));
#208021=CARTESIAN_POINT('Ctrl Pts',(49.2383606512453,29.8771413537661,-228.0320224667));
#208022=CARTESIAN_POINT('Ctrl Pts',(49.2292949767161,29.8740088784577,-228.03789690835));
#208023=CARTESIAN_POINT('Ctrl Pts',(49.2232727107977,29.8719574195942,-228.041788726452));
#208024=CARTESIAN_POINT('Ctrl Pts',(49.2214396993231,29.8713363276065,-228.042972081044));
#208025=CARTESIAN_POINT('Ctrl Pts',(49.1507737414336,29.8479572973245,-228.088392226472));
#208026=CARTESIAN_POINT('Ctrl Pts',(49.0869264206795,29.8340568928808,-228.126800162686));
#208027=CARTESIAN_POINT('Ctrl Pts',(48.9965302726213,29.8239838805917,-228.17740626585));
#208028=CARTESIAN_POINT('Ctrl Pts',(48.9672934413079,29.8224230610671,-228.193113085777));
#208029=CARTESIAN_POINT('Ctrl Pts',(48.924945017721,29.8226136605282,-228.214916183171));
#208030=CARTESIAN_POINT('Ctrl Pts',(48.9041473927209,29.8233420361004,-228.225378910074));
#208031=CARTESIAN_POINT('Ctrl Pts',(48.8805769903507,29.8252653389655,-228.236818978745));
#208032=CARTESIAN_POINT('Ctrl Pts',(48.8706275872652,29.8263160738771,-228.241558062775));
#208033=CARTESIAN_POINT('Ctrl Pts',(48.8640288696302,29.8270664940945,-228.244681106617));
#208034=CARTESIAN_POINT('Ctrl Pts',(48.8619974565436,29.8273038682259,-228.245640131405));
#208035=CARTESIAN_POINT('Ctrl Pts',(48.7129766922957,29.8466994525346,-228.315254631247));
#208036=CARTESIAN_POINT('Ctrl Pts',(48.5945826105962,29.9151547892192,-228.35005));
#208037=CARTESIAN_POINT('Ctrl Pts',(48.515339402069,30.020261242545,-228.35005));
#208038=CARTESIAN_POINT('',(49.8755750290351,29.6684593880862,-227.255950349386));
#208039=CARTESIAN_POINT('Origin',(50.1572979707234,29.8969930061248,-227.60005));
#208040=CARTESIAN_POINT('Ctrl Pts',(48.2384287873563,29.7860380279371,-228.505869818703));
#208041=CARTESIAN_POINT('Ctrl Pts',(48.3005627733003,29.7125636424197,-228.505880994607));
#208042=CARTESIAN_POINT('Ctrl Pts',(48.3682975812994,29.6477646817255,-228.495224421534));
#208043=CARTESIAN_POINT('Ctrl Pts',(48.4781251048924,29.5638843894103,-228.463237938458));
#208044=CARTESIAN_POINT('Ctrl Pts',(48.5350955562029,29.5252734538315,-228.443244291053));
#208045=CARTESIAN_POINT('Ctrl Pts',(48.6051255375809,29.4861167483495,-228.412917658814));
#208046=CARTESIAN_POINT('Ctrl Pts',(48.6358987065498,29.4706038724335,-228.398420378511));
#208047=CARTESIAN_POINT('Ctrl Pts',(48.6565827304486,29.4605445821547,-228.38842215782));
#208048=CARTESIAN_POINT('Ctrl Pts',(48.6680836436967,29.4551709393352,-228.382711156425));
#208049=CARTESIAN_POINT('Ctrl Pts',(48.7530057377613,29.4168188138147,-228.339625726171));
#208050=CARTESIAN_POINT('Ctrl Pts',(48.8296829433926,29.3915172223634,-228.294286688015));
#208051=CARTESIAN_POINT('Ctrl Pts',(48.9465146046185,29.3668671949067,-228.215716813884));
#208052=CARTESIAN_POINT('Ctrl Pts',(49.0053847104949,29.3578670652606,-228.173791547594));
#208053=CARTESIAN_POINT('Ctrl Pts',(49.0748703494029,29.3532047319551,-228.120258160781));
#208054=CARTESIAN_POINT('Ctrl Pts',(49.1048232381759,29.3524592107239,-228.096325157259));
#208055=CARTESIAN_POINT('Ctrl Pts',(49.1248304708793,29.3522407306626,-228.080149794142));
#208056=CARTESIAN_POINT('Ctrl Pts',(49.1360275453979,29.3522905620935,-228.070980769437));
#208057=CARTESIAN_POINT('Ctrl Pts',(49.2158411714096,29.353636723251,-228.004953353353));
#208058=CARTESIAN_POINT('Ctrl Pts',(49.2851376328763,29.3618147939751,-227.942889930398));
#208059=CARTESIAN_POINT('Ctrl Pts',(49.3867128239049,29.3845233081293,-227.844736216309));
#208060=CARTESIAN_POINT('Ctrl Pts',(49.4369079545403,29.3984875351963,-227.794394714351));
#208061=CARTESIAN_POINT('Ctrl Pts',(49.4862331273773,29.4163574712173,-227.742156245023));
#208062=CARTESIAN_POINT('Ctrl Pts',(49.5189252866697,29.4291374288087,-227.706909050499));
#208063=CARTESIAN_POINT('Ctrl Pts',(49.5362231832806,29.4364311931001,-227.687904724522));
#208064=CARTESIAN_POINT('Ctrl Pts',(49.6721982976717,29.4975011599834,-227.53602800549));
#208065=CARTESIAN_POINT('Ctrl Pts',(49.7801088316737,29.572761994563,-227.397668277446));
#208066=CARTESIAN_POINT('Ctrl Pts',(49.8755750290351,29.6684593880862,-227.255950349386));
#208067=CARTESIAN_POINT('Ctrl Pts',(49.8755750290351,29.6684593880862,-227.255950349386));
#208068=CARTESIAN_POINT('Ctrl Pts',(49.566578371721,30.0125857112181,-227.280382264872));
#208069=CARTESIAN_POINT('Ctrl Pts',(49.8031531494471,30.2499539750196,-227.60005));
#208070=CARTESIAN_POINT('Ctrl Pts',(51.4695961402316,31.2663408349186,-224.889653425376));
#208071=CARTESIAN_POINT('Ctrl Pts',(51.160952124674,31.6123070902132,-224.911157102841));
#208072=CARTESIAN_POINT('Ctrl Pts',(51.3963758794861,31.8485204702035,-225.233951755693));
#208073=CARTESIAN_POINT('Ctrl Pts',(53.0649609053862,32.864644901729,-222.524371622939));
#208074=CARTESIAN_POINT('Ctrl Pts',(52.757248450643,33.2139574900831,-222.540616273922));
#208075=CARTESIAN_POINT('Ctrl Pts',(52.9904440332794,33.4479352247441,-222.868995945589));
#208076=CARTESIAN_POINT('Ctrl Pts',(54.6643562096698,34.4651804296883,-220.162900223157));
#208077=CARTESIAN_POINT('Ctrl Pts',(54.3487296401403,34.8107766034666,-220.183958003048));
#208078=CARTESIAN_POINT('Ctrl Pts',(54.5875190481085,35.0503669255136,-220.508112862707));
#208079=CARTESIAN_POINT('',(54.5875190481084,35.0503669255136,-220.508112862707));
#208080=CARTESIAN_POINT('',(54.6643562096698,34.4651804296884,-220.162900223157));
#208081=CARTESIAN_POINT('Origin',(54.9416638693848,34.6974059566189,-220.508112862707));
#208082=CARTESIAN_POINT('Ctrl Pts',(49.8755750290351,29.6684593880862,-227.255950349386));
#208083=CARTESIAN_POINT('Ctrl Pts',(51.5864044294278,31.383432005677,-224.716253529058));
#208084=CARTESIAN_POINT('Ctrl Pts',(53.1817714358015,32.9815387074691,-222.351903486981));
#208085=CARTESIAN_POINT('Ctrl Pts',(54.6643562096698,34.4651804296884,-220.162900223157));
#208086=CARTESIAN_POINT('Ctrl Pts',(54.5875190481084,35.0503669255136,-220.508112862707));
#208087=CARTESIAN_POINT('Ctrl Pts',(52.990443779671,33.4479349702851,-222.86899632084));
#208088=CARTESIAN_POINT('Ctrl Pts',(51.3963761190905,31.8485207106117,-225.233951400128));
#208089=CARTESIAN_POINT('Ctrl Pts',(49.8031531494471,30.2499539750197,-227.60005));
#208090=CARTESIAN_POINT('Ctrl Pts',(42.4431629103415,35.679860391633,-228.507034483728));
#208091=CARTESIAN_POINT('Ctrl Pts',(42.5405392130025,35.7913421132894,-228.35005));
#208092=CARTESIAN_POINT('Ctrl Pts',(42.6824807550636,35.9538445605081,-228.35005));
#208093=CARTESIAN_POINT('Ctrl Pts',(43.4842614434386,34.7712285271383,-228.506443516651));
#208094=CARTESIAN_POINT('Ctrl Pts',(43.5839578161182,34.8805832623425,-228.350049999846));
#208095=CARTESIAN_POINT('Ctrl Pts',(43.7299304472252,35.0389252651105,-228.35005));
#208096=CARTESIAN_POINT('Ctrl Pts',(44.4876418177359,33.826550002353,-228.506035020985));
#208097=CARTESIAN_POINT('Ctrl Pts',(44.590423195572,33.9329609873047,-228.350049999904));
#208098=CARTESIAN_POINT('Ctrl Pts',(44.7400658047431,34.0873590008399,-228.35005));
#208099=CARTESIAN_POINT('Ctrl Pts',(46.4180861418825,31.8610058543969,-228.505671567324));
#208100=CARTESIAN_POINT('Ctrl Pts',(46.5261142282933,31.9620046547715,-228.350050000096));
#208101=CARTESIAN_POINT('Ctrl Pts',(46.6832166107726,32.108381759188,-228.35005));
#208102=CARTESIAN_POINT('Ctrl Pts',(47.3461759565219,30.8411406013281,-228.505709331207));
#208103=CARTESIAN_POINT('Ctrl Pts',(47.4568224915956,30.9392657163356,-228.350050000173));
#208104=CARTESIAN_POINT('Ctrl Pts',(47.617275666974,31.0819979338032,-228.35005));
#208105=CARTESIAN_POINT('Ctrl Pts',(48.2384287873563,29.7860380279371,-228.505869818703));
#208106=CARTESIAN_POINT('Ctrl Pts',(48.3513278433713,29.8815330303712,-228.35005));
#208107=CARTESIAN_POINT('Ctrl Pts',(48.515339402069,30.020261242545,-228.35005));
#208108=CARTESIAN_POINT('',(42.4431629103415,35.679860391633,-228.507034483728));
#208109=CARTESIAN_POINT('',(42.6824807550636,35.9538445605081,-228.35005));
#208110=CARTESIAN_POINT('Origin',(42.6824807550636,35.9538445605081,-228.85005));
#208111=CARTESIAN_POINT('Ctrl Pts',(48.515339402069,30.020261242545,-228.35005));
#208112=CARTESIAN_POINT('Ctrl Pts',(47.6172684110892,31.0820065120798,-228.35005));
#208113=CARTESIAN_POINT('Ctrl Pts',(46.6832166107701,32.1083817591879,-228.35005));
#208114=CARTESIAN_POINT('Ctrl Pts',(45.7116412077571,33.0978703800133,-228.35005));
#208115=CARTESIAN_POINT('Ctrl Pts',(44.7400658047442,34.0873590008387,-228.35005));
#208116=CARTESIAN_POINT('Ctrl Pts',(43.7299213057923,35.0389332497409,-228.35005));
#208117=CARTESIAN_POINT('Ctrl Pts',(42.6824807550636,35.9538445605081,-228.35005));
#208118=CARTESIAN_POINT('Ctrl Pts',(42.4431629103415,35.679860391633,-228.507034483728));
#208119=CARTESIAN_POINT('Ctrl Pts',(42.783732660266,35.3826238505884,-228.5068411634));
#208120=CARTESIAN_POINT('Ctrl Pts',(43.1251178195728,35.0772901594386,-228.506664609947));
#208121=CARTESIAN_POINT('Ctrl Pts',(43.4664349615021,34.7639460185337,-228.506508376881));
#208122=CARTESIAN_POINT('Ctrl Pts',(43.7986630315905,34.4589460451426,-228.506356304208));
#208123=CARTESIAN_POINT('Ctrl Pts',(44.1308266151257,34.1463564072806,-228.506223487408));
#208124=CARTESIAN_POINT('Ctrl Pts',(44.4621498940903,33.8262865256091,-228.506113215303));
#208125=CARTESIAN_POINT('Ctrl Pts',(44.7934731730549,33.5062166439377,-228.506002943198));
#208126=CARTESIAN_POINT('Ctrl Pts',(45.1239551433519,33.1786670679477,-228.50591521934));
#208127=CARTESIAN_POINT('Ctrl Pts',(45.4528639798093,32.8437779283751,-228.505853294154));
#208128=CARTESIAN_POINT('Ctrl Pts',(45.7418215590338,32.5495664498336,-228.505798890776));
#208129=CARTESIAN_POINT('Ctrl Pts',(46.0296572151249,32.2497783732728,-228.505763776886));
#208130=CARTESIAN_POINT('Ctrl Pts',(46.3158895995213,31.9447181809263,-228.505746122221));
#208131=CARTESIAN_POINT('Ctrl Pts',(46.6021152411152,31.6396651749107,-228.505728467972));
#208132=CARTESIAN_POINT('Ctrl Pts',(46.8867376705897,31.3293403107133,-228.505728268231));
#208133=CARTESIAN_POINT('Ctrl Pts',(47.1693119506508,31.0140854067816,-228.505743316248));
#208134=CARTESIAN_POINT('Ctrl Pts',(47.4524717478086,30.6981772688189,-228.505758395446));
#208135=CARTESIAN_POINT('Ctrl Pts',(47.7335748895764,30.3773186565972,-228.505788781456));
#208136=CARTESIAN_POINT('Ctrl Pts',(48.0122104039763,30.0518908485059,-228.505831936305));
#208137=CARTESIAN_POINT('Ctrl Pts',(48.0878005118504,29.9636066139142,-228.505843643641));
#208138=CARTESIAN_POINT('Ctrl Pts',(48.1632092196792,29.8749863133239,-228.505856289123));
#208139=CARTESIAN_POINT('Ctrl Pts',(48.2384287873563,29.7860380279371,-228.505869818703));
#208140=CARTESIAN_POINT('Ctrl Pts',(54.9968660030027,36.3988348033229,-218.849954951747));
#208141=CARTESIAN_POINT('Ctrl Pts',(55.018269151756,36.2900558272771,-218.637811171833));
#208142=CARTESIAN_POINT('Ctrl Pts',(55.2146353748417,36.257836765148,-218.504776656654));
#208143=CARTESIAN_POINT('Ctrl Pts',(55.052102137237,36.1181036738987,-219.049315831028));
#208144=CARTESIAN_POINT('Ctrl Pts',(55.0614326261139,35.9588010119692,-218.832425369541));
#208145=CARTESIAN_POINT('Ctrl Pts',(55.2870795674735,35.8851781565784,-218.70395400533));
#208146=CARTESIAN_POINT('Ctrl Pts',(55.0225064544189,35.8553343499292,-219.318743015247));
#208147=CARTESIAN_POINT('Ctrl Pts',(54.9920018852822,35.6566773356544,-219.093930954085));
#208148=CARTESIAN_POINT('Ctrl Pts',(55.2466620625239,35.5359310914396,-218.973388048174));
#208149=CARTESIAN_POINT('Ctrl Pts',(54.8701701172632,35.4039199531589,-219.888552047874));
#208150=CARTESIAN_POINT('Ctrl Pts',(54.7478058041725,35.1574653296587,-219.629072060686));
#208151=CARTESIAN_POINT('Ctrl Pts',(55.04206217923,34.9357811050907,-219.543206859615));
#208152=CARTESIAN_POINT('Ctrl Pts',(54.745550854066,35.2089287796815,-220.196631257494));
#208153=CARTESIAN_POINT('Ctrl Pts',(54.5592271140423,34.9538518370357,-219.918109540734));
#208154=CARTESIAN_POINT('Ctrl Pts',(54.8753705653342,34.6763452196017,-219.851342245783));
#208155=CARTESIAN_POINT('Ctrl Pts',(54.5875190481085,35.0503669255137,-220.508112862707));
#208156=CARTESIAN_POINT('Ctrl Pts',(54.3487296401403,34.8107766034666,-220.183958003048));
#208157=CARTESIAN_POINT('Ctrl Pts',(54.6643562096698,34.4651804296883,-220.162900223157));
#208158=CARTESIAN_POINT('',(54.9968660030035,36.3988348033192,-218.84995495175));
#208159=CARTESIAN_POINT('',(55.2146353748417,36.257836765148,-218.504776656654));
#208160=CARTESIAN_POINT('Origin',(55.4874598092474,36.4953631270242,-218.849954951747));
#208161=CARTESIAN_POINT('Ctrl Pts',(54.6643562096698,34.4651804296883,-220.162900223157));
#208162=CARTESIAN_POINT('Ctrl Pts',(54.7074039308287,34.508258839999,-220.099341225512));
#208163=CARTESIAN_POINT('Ctrl Pts',(54.7480314614451,34.5527651846987,-220.036777704785));
#208164=CARTESIAN_POINT('Ctrl Pts',(54.7863060742582,34.5985925935165,-219.975215224127));
#208165=CARTESIAN_POINT('Ctrl Pts',(54.8273110867564,34.6476891965443,-219.909261054947));
#208166=CARTESIAN_POINT('Ctrl Pts',(54.8656162789774,34.69830187121,-219.844455384552));
#208167=CARTESIAN_POINT('Ctrl Pts',(54.9012839494488,34.7503560715278,-219.780785198212));
#208168=CARTESIAN_POINT('Ctrl Pts',(54.9313207276235,34.7941924210102,-219.727166690522));
#208169=CARTESIAN_POINT('Ctrl Pts',(54.959488169708,34.8390547171882,-219.674350124633));
#208170=CARTESIAN_POINT('Ctrl Pts',(54.9858017155598,34.8849169151779,-219.622333509997));
#208171=CARTESIAN_POINT('Ctrl Pts',(55.0178834325347,34.9408325285293,-219.558914375301));
#208172=CARTESIAN_POINT('Ctrl Pts',(55.0472095907453,34.998232325381,-219.496685631604));
#208173=CARTESIAN_POINT('Ctrl Pts',(55.0737733419852,35.0570995269978,-219.435651937387));
#208174=CARTESIAN_POINT('Ctrl Pts',(55.0959985739645,35.1063522549011,-219.384586558846));
#208175=CARTESIAN_POINT('Ctrl Pts',(55.1162888777561,35.1566323285765,-219.334358625518));
#208176=CARTESIAN_POINT('Ctrl Pts',(55.1346165986468,35.2079360988119,-219.284985901448));
#208177=CARTESIAN_POINT('Ctrl Pts',(55.1370365296852,35.2147100772414,-219.278466891903));
#208178=CARTESIAN_POINT('Ctrl Pts',(55.1392598915153,35.221036410009,-219.272407652944));
#208179=CARTESIAN_POINT('Ctrl Pts',(55.1416546709122,35.2279680296668,-219.265801317888));
#208180=CARTESIAN_POINT('Ctrl Pts',(55.1424346005327,35.2302255133815,-219.263649772573));
#208181=CARTESIAN_POINT('Ctrl Pts',(55.1432323949011,35.2325473997641,-219.261440311746));
#208182=CARTESIAN_POINT('Ctrl Pts',(55.1440597796072,35.2349706839286,-219.259138509777));
#208183=CARTESIAN_POINT('Ctrl Pts',(55.1441605630477,35.2352658633217,-219.258858128087));
#208184=CARTESIAN_POINT('Ctrl Pts',(55.1442612725152,35.2355610486931,-219.25857780077));
#208185=CARTESIAN_POINT('Ctrl Pts',(55.1443619080441,35.2358562400493,-219.258297527793));
#208186=CARTESIAN_POINT('Ctrl Pts',(55.1603383653164,35.2827195311766,-219.213802613465));
#208187=CARTESIAN_POINT('Ctrl Pts',(55.1745132525297,35.3299375330594,-219.170490352343));
#208188=CARTESIAN_POINT('Ctrl Pts',(55.1868961950868,35.377471738341,-219.128368907279));
#208189=CARTESIAN_POINT('Ctrl Pts',(55.1952874349737,35.4096830578649,-219.099825517992));
#208190=CARTESIAN_POINT('Ctrl Pts',(55.2028557096548,35.4420407056901,-219.071828315238));
#208191=CARTESIAN_POINT('Ctrl Pts',(55.2096002183572,35.4745446654207,-219.044375123623));
#208192=CARTESIAN_POINT('Ctrl Pts',(55.2179802508663,35.5149307411503,-219.010264612634));
#208193=CARTESIAN_POINT('Ctrl Pts',(55.2250915055409,35.5555371343618,-218.976995360291));
#208194=CARTESIAN_POINT('Ctrl Pts',(55.2309378807329,35.5963523838428,-218.944567088419));
#208195=CARTESIAN_POINT('Ctrl Pts',(55.233861068329,35.6167600085833,-218.928352952483));
#208196=CARTESIAN_POINT('Ctrl Pts',(55.2364680386656,35.6372198496141,-218.91234906497));
#208197=CARTESIAN_POINT('Ctrl Pts',(55.2387592664335,35.6577305151278,-218.896555409356));
#208198=CARTESIAN_POINT('Ctrl Pts',(55.2399048803175,35.6679858478847,-218.888658581548));
#208199=CARTESIAN_POINT('Ctrl Pts',(55.2409715586851,35.678253886869,-218.880814311874));
#208200=CARTESIAN_POINT('Ctrl Pts',(55.241959358827,35.688534461645,-218.873022599437));
#208201=CARTESIAN_POINT('Ctrl Pts',(55.2426458899188,35.6956795651188,-218.867607280467));
#208202=CARTESIAN_POINT('Ctrl Pts',(55.2432514894495,35.7023487309182,-218.862579958581));
#208203=CARTESIAN_POINT('Ctrl Pts',(55.2438669137039,35.7095462696188,-218.8571838814));
#208204=CARTESIAN_POINT('Ctrl Pts',(55.2441369790844,35.7127047509656,-218.854815931767));
#208205=CARTESIAN_POINT('Ctrl Pts',(55.2444084132222,35.7159652044752,-218.852377223766));
#208206=CARTESIAN_POINT('Ctrl Pts',(55.2446861814473,35.7194136243086,-218.849805133612));
#208207=CARTESIAN_POINT('Ctrl Pts',(55.2483291642508,35.7646403025828,-218.816071684817));
#208208=CARTESIAN_POINT('Ctrl Pts',(55.2504339246697,35.8097873894187,-218.783583104913));
#208209=CARTESIAN_POINT('Ctrl Pts',(55.2510014461176,35.8548473662421,-218.752339591324));
#208210=CARTESIAN_POINT('Ctrl Pts',(55.251799183524,35.9181859927769,-218.708422097834));
#208211=CARTESIAN_POINT('Ctrl Pts',(55.2495512973704,35.9813642859329,-218.666963136053));
#208212=CARTESIAN_POINT('Ctrl Pts',(55.2442764911647,36.0443389392307,-218.627967205458));
#208213=CARTESIAN_POINT('Ctrl Pts',(55.2389089241922,36.1084210412002,-218.588285507031));
#208214=CARTESIAN_POINT('Ctrl Pts',(55.2304080556554,36.1722930120072,-218.551152986505));
#208215=CARTESIAN_POINT('Ctrl Pts',(55.2187640677965,36.2359515925339,-218.516569914905));
#208216=CARTESIAN_POINT('Ctrl Pts',(55.2174292017159,36.2432494084467,-218.512605313619));
#208217=CARTESIAN_POINT('Ctrl Pts',(55.2160529867808,36.2505444581524,-218.508674224936));
#208218=CARTESIAN_POINT('Ctrl Pts',(55.2146353748417,36.257836765148,-218.504776656654));
#208219=CARTESIAN_POINT('Ctrl Pts',(54.9968660030034,36.3988348033192,-218.84995495175));
#208220=CARTESIAN_POINT('Ctrl Pts',(55.0040920464924,36.362109290608,-218.876035526304));
#208221=CARTESIAN_POINT('Ctrl Pts',(55.0100902040703,36.3245420184541,-218.904133384402));
#208222=CARTESIAN_POINT('Ctrl Pts',(55.0146816372595,36.2862590986273,-218.934320638599));
#208223=CARTESIAN_POINT('Ctrl Pts',(55.0175341077067,36.26247547967,-218.953074750208));
#208224=CARTESIAN_POINT('Ctrl Pts',(55.0198440529379,36.2384160209788,-218.972634555083));
#208225=CARTESIAN_POINT('Ctrl Pts',(55.0215733928243,36.2141149072774,-218.99300918415));
#208226=CARTESIAN_POINT('Ctrl Pts',(55.0248772919048,36.1676876966138,-219.031934856756));
#208227=CARTESIAN_POINT('Ctrl Pts',(55.0260595476318,36.1203762301498,-219.073838887151));
#208228=CARTESIAN_POINT('Ctrl Pts',(55.0248935219138,36.0724066660917,-219.118759345035));
#208229=CARTESIAN_POINT('Ctrl Pts',(55.0240041749923,36.0358194935617,-219.153020914324));
#208230=CARTESIAN_POINT('Ctrl Pts',(55.0217494012894,35.9988459801408,-219.189039842437));
#208231=CARTESIAN_POINT('Ctrl Pts',(55.0180465606492,35.961603893522,-219.226800636546));
#208232=CARTESIAN_POINT('Ctrl Pts',(55.0143234843304,35.9241582823743,-219.264767789873));
#208233=CARTESIAN_POINT('Ctrl Pts',(55.0091362504138,35.8864343633192,-219.304502287204));
#208234=CARTESIAN_POINT('Ctrl Pts',(55.0024125558477,35.8485468343893,-219.345982968744));
#208235=CARTESIAN_POINT('Ctrl Pts',(54.9959666612172,35.8122246878533,-219.385749811182));
#208236=CARTESIAN_POINT('Ctrl Pts',(54.9881101007026,35.7757565885262,-219.427115973757));
#208237=CARTESIAN_POINT('Ctrl Pts',(54.978783579186,35.7392359043793,-219.47006753094));
#208238=CARTESIAN_POINT('Ctrl Pts',(54.9737864840352,35.7196683374868,-219.493080721627));
#208239=CARTESIAN_POINT('Ctrl Pts',(54.9683676566711,35.700086635794,-219.516547938461));
#208240=CARTESIAN_POINT('Ctrl Pts',(54.962518087953,35.6805061616403,-219.540466343658));
#208241=CARTESIAN_POINT('Ctrl Pts',(54.9584722404756,35.6669633492073,-219.557009481108));
#208242=CARTESIAN_POINT('Ctrl Pts',(54.9542204118081,35.6534213830759,-219.573768146966));
#208243=CARTESIAN_POINT('Ctrl Pts',(54.9497594430271,35.6398852506478,-219.590741752706));
#208244=CARTESIAN_POINT('Ctrl Pts',(54.9486324135337,35.6364654507742,-219.595030003806));
#208245=CARTESIAN_POINT('Ctrl Pts',(54.9474919474504,35.6330457676747,-219.599332298452));
#208246=CARTESIAN_POINT('Ctrl Pts',(54.9463382858411,35.629627151544,-219.60364753156));
#208247=CARTESIAN_POINT('Ctrl Pts',(54.9461922858206,35.6291945133935,-219.60419363981));
#208248=CARTESIAN_POINT('Ctrl Pts',(54.9460460675899,35.6287618689978,-219.604739983546));
#208249=CARTESIAN_POINT('Ctrl Pts',(54.9458996314877,35.6283292201355,-219.605286560807));
#208250=CARTESIAN_POINT('Ctrl Pts',(54.9457655873106,35.6279331835038,-219.605786884826));
#208251=CARTESIAN_POINT('Ctrl Pts',(54.945631966464,35.6275389212305,-219.606285153914));
#208252=CARTESIAN_POINT('Ctrl Pts',(54.9454942839764,35.6271332403158,-219.606798055818));
#208253=CARTESIAN_POINT('Ctrl Pts',(54.9447134539827,35.6248325277747,-219.609706843985));
#208254=CARTESIAN_POINT('Ctrl Pts',(54.9438343666549,35.6222630584633,-219.612962841538));
#208255=CARTESIAN_POINT('Ctrl Pts',(54.9430286280765,35.6199273297219,-219.615929620851));
#208256=CARTESIAN_POINT('Ctrl Pts',(54.9426383484526,35.6187959611129,-219.617366654581));
#208257=CARTESIAN_POINT('Ctrl Pts',(54.9422654235513,35.6177193398141,-219.618735762759));
#208258=CARTESIAN_POINT('Ctrl Pts',(54.9419300749024,35.6167541113451,-219.619964278477));
#208259=CARTESIAN_POINT('Ctrl Pts',(54.941747008926,35.6162271955734,-219.62063492209));
#208260=CARTESIAN_POINT('Ctrl Pts',(54.941575148176,35.6157334705899,-219.621263665118));
#208261=CARTESIAN_POINT('Ctrl Pts',(54.9414178205515,35.6152821267846,-219.621838668181));
#208262=CARTESIAN_POINT('Ctrl Pts',(54.9413537204437,35.6150982354517,-219.622072942094));
#208263=CARTESIAN_POINT('Ctrl Pts',(54.9412924648862,35.6149226137709,-219.622296720729));
#208264=CARTESIAN_POINT('Ctrl Pts',(54.9412304034246,35.6147447846829,-219.622523349969));
#208265=CARTESIAN_POINT('Ctrl Pts',(54.9281435230044,35.5772460221848,-219.670312584787));
#208266=CARTESIAN_POINT('Ctrl Pts',(54.9131804711756,35.5390861037303,-219.720677924238));
#208267=CARTESIAN_POINT('Ctrl Pts',(54.8960963824159,35.500529589748,-219.773644865139));
#208268=CARTESIAN_POINT('Ctrl Pts',(54.8905118862791,35.4879261254128,-219.790958851328));
#208269=CARTESIAN_POINT('Ctrl Pts',(54.8847008768019,35.4752805096263,-219.808550513932));
#208270=CARTESIAN_POINT('Ctrl Pts',(54.8786552093599,35.4626026527875,-219.826419782291));
#208271=CARTESIAN_POINT('Ctrl Pts',(54.8663596694719,35.4368187181017,-219.862761890748));
#208272=CARTESIAN_POINT('Ctrl Pts',(54.8530933057166,35.410900869322,-219.900253099045));
#208273=CARTESIAN_POINT('Ctrl Pts',(54.8387867552026,35.3849304106352,-219.938883517151));
#208274=CARTESIAN_POINT('Ctrl Pts',(54.8316334799456,35.3719451812918,-219.958198726204));
#208275=CARTESIAN_POINT('Ctrl Pts',(54.8242199501464,35.3589465132715,-219.977798384425));
#208276=CARTESIAN_POINT('Ctrl Pts',(54.8165395696195,35.3459480790558,-219.997684076851));
#208277=CARTESIAN_POINT('Ctrl Pts',(54.8126993793561,35.339448861948,-220.007626923063));
#208278=CARTESIAN_POINT('Ctrl Pts',(54.8087924839424,35.3329497025708,-220.01764127887));
#208279=CARTESIAN_POINT('Ctrl Pts',(54.8048180095845,35.3264521669541,-220.027727144102));
#208280=CARTESIAN_POINT('Ctrl Pts',(54.8028307724055,35.3232033991458,-220.032770076718));
#208281=CARTESIAN_POINT('Ctrl Pts',(54.800826640669,35.3199550371977,-220.037830886689));
#208282=CARTESIAN_POINT('Ctrl Pts',(54.7988055087113,35.3167072803064,-220.042909573995));
#208283=CARTESIAN_POINT('Ctrl Pts',(54.797056869173,35.3138973914768,-220.047303544113));
#208284=CARTESIAN_POINT('Ctrl Pts',(54.7948825822304,35.310433149772,-220.052740770874));
#208285=CARTESIAN_POINT('Ctrl Pts',(54.7933541298033,35.3080144248348,-220.056548243653));
#208286=CARTESIAN_POINT('Ctrl Pts',(54.7931159493833,35.3076375122719,-220.057141566317));
#208287=CARTESIAN_POINT('Ctrl Pts',(54.7928935324271,35.307285921985,-220.0576952873));
#208288=CARTESIAN_POINT('Ctrl Pts',(54.7926910080452,35.3069660248027,-220.058199267894));
#208289=CARTESIAN_POINT('Ctrl Pts',(54.7778673199726,35.2835512833232,-220.095087918257));
#208290=CARTESIAN_POINT('Ctrl Pts',(54.761373636425,35.2589411193526,-220.134834364075));
#208291=CARTESIAN_POINT('Ctrl Pts',(54.7429690732774,35.2333793116411,-220.177477225497));
#208292=CARTESIAN_POINT('Ctrl Pts',(54.7251831383047,35.2086767068525,-220.218686742626));
#208293=CARTESIAN_POINT('Ctrl Pts',(54.7056120315136,35.1830853552272,-220.262601832834));
#208294=CARTESIAN_POINT('Ctrl Pts',(54.6840331800314,35.1568641348512,-220.30923021939));
#208295=CARTESIAN_POINT('Ctrl Pts',(54.6636061794762,35.1320425689946,-220.353369643532));
#208296=CARTESIAN_POINT('Ctrl Pts',(54.6413795825545,35.1066567034407,-220.399940802683));
#208297=CARTESIAN_POINT('Ctrl Pts',(54.6171673998294,35.0809605126591,-220.448918846524));
#208298=CARTESIAN_POINT('Ctrl Pts',(54.6075983865104,35.0708049973705,-220.468275695065));
#208299=CARTESIAN_POINT('Ctrl Pts',(54.5977193044027,35.0606013940828,-220.48800809843));
#208300=CARTESIAN_POINT('Ctrl Pts',(54.5875190481085,35.0503669255137,-220.508112862707));
#208301=CARTESIAN_POINT('Ctrl Pts',(42.6824807550636,35.9538445605081,-228.35005));
#208302=CARTESIAN_POINT('Ctrl Pts',(42.5404167002247,35.791201853955,-228.35005));
#208303=CARTESIAN_POINT('Ctrl Pts',(42.443021269923,35.6796982339285,-228.50726297195));
#208304=CARTESIAN_POINT('Ctrl Pts',(42.5913145600393,36.0267272443623,-228.35005));
#208305=CARTESIAN_POINT('Ctrl Pts',(42.4282834326699,35.8863211720346,-228.352241313908));
#208306=CARTESIAN_POINT('Ctrl Pts',(42.2979928747684,35.806276985376,-228.507342686565));
#208307=CARTESIAN_POINT('Ctrl Pts',(42.5313139073579,36.1299188273931,-228.321794566394));
#208308=CARTESIAN_POINT('Ctrl Pts',(42.3443085102026,36.0112714706978,-228.310299465652));
#208309=CARTESIAN_POINT('Ctrl Pts',(42.1843277826865,35.9629604673028,-228.460330590341));
#208310=CARTESIAN_POINT('Ctrl Pts',(42.4814079540288,36.3579978037835,-228.225751005231));
#208311=CARTESIAN_POINT('Ctrl Pts',(42.2569704879925,36.2630116503163,-228.16819510465));
#208312=CARTESIAN_POINT('Ctrl Pts',(42.0432088071097,36.2819979616018,-228.300386998121));
#208313=CARTESIAN_POINT('Ctrl Pts',(42.4898483164371,36.4810484712422,-228.159605024773));
#208314=CARTESIAN_POINT('Ctrl Pts',(42.2522549527837,36.3904916192652,-228.068484337662));
#208315=CARTESIAN_POINT('Ctrl Pts',(42.0140892672452,36.4425131983365,-228.190195527837));
#208316=CARTESIAN_POINT('Ctrl Pts',(42.5520089174244,36.7203516154467,-228.012906367619));
#208317=CARTESIAN_POINT('Ctrl Pts',(42.2976224084343,36.6185146335635,-227.852954061751));
#208318=CARTESIAN_POINT('Ctrl Pts',(42.0182756482514,36.7396699246603,-227.945762342978));
#208319=CARTESIAN_POINT('Ctrl Pts',(42.6046949644287,36.835724973434,-227.933213206321));
#208320=CARTESIAN_POINT('Ctrl Pts',(42.3488315361518,36.7193728341531,-227.736107069137));
#208321=CARTESIAN_POINT('Ctrl Pts',(42.0504918440331,36.8754822200752,-227.812957113271));
#208322=CARTESIAN_POINT('Ctrl Pts',(42.7406007705538,37.0550530398967,-227.767956190477));
#208323=CARTESIAN_POINT('Ctrl Pts',(42.4877694298107,36.8912905811231,-227.501601704626));
#208324=CARTESIAN_POINT('Ctrl Pts',(42.1592600405123,37.1219402239383,-227.537528223444));
#208325=CARTESIAN_POINT('Ctrl Pts',(42.8221296650751,37.1564022812852,-227.68437936815));
#208326=CARTESIAN_POINT('Ctrl Pts',(42.5766199121254,36.9595585654922,-227.385429649693));
#208327=CARTESIAN_POINT('Ctrl Pts',(42.2344115671227,37.22968036859,-227.398223401081));
#208328=CARTESIAN_POINT('Ctrl Pts',(42.9157357330403,37.2503223096489,-227.60005));
#208329=CARTESIAN_POINT('Ctrl Pts',(42.6749497694503,37.0087287354121,-227.278243940858));
#208330=CARTESIAN_POINT('Ctrl Pts',(42.3280651351011,37.3236108350448,-227.257633534302));
#208331=CARTESIAN_POINT('',(42.3284659498332,37.323247286775,-227.257657541791));
#208332=CARTESIAN_POINT('',(42.9157357330403,37.2503223096489,-227.60005));
#208333=CARTESIAN_POINT('Origin',(42.561590911764,37.6032832785437,-227.60005));
#208334=CARTESIAN_POINT('Ctrl Pts',(42.6824807550636,35.9538445605081,-228.35005));
#208335=CARTESIAN_POINT('Ctrl Pts',(42.6316328790924,35.9944948069838,-228.35005));
#208336=CARTESIAN_POINT('Ctrl Pts',(42.5896593585113,36.0448083850312,-228.34162603267));
#208337=CARTESIAN_POINT('Ctrl Pts',(42.5424025219209,36.1323898340594,-228.316179318494));
#208338=CARTESIAN_POINT('Ctrl Pts',(42.5292691936361,36.1636004599124,-228.305571179723));
#208339=CARTESIAN_POINT('Ctrl Pts',(42.5138046839852,36.2131355824937,-228.286535124351));
#208340=CARTESIAN_POINT('Ctrl Pts',(42.5071313240516,36.2385829156178,-228.276237069799));
#208341=CARTESIAN_POINT('Ctrl Pts',(42.5012657853535,36.2693943137178,-228.262881841837));
#208342=CARTESIAN_POINT('Ctrl Pts',(42.4991705525361,36.2828327009754,-228.256874092392));
#208343=CARTESIAN_POINT('Ctrl Pts',(42.4978675356399,36.2918427283243,-228.252806174876));
#208344=CARTESIAN_POINT('Ctrl Pts',(42.4971073002351,36.2976454866849,-228.250155383563));
#208345=CARTESIAN_POINT('Ctrl Pts',(42.4902787436054,36.3534654942239,-228.224467376528));
#208346=CARTESIAN_POINT('Ctrl Pts',(42.4900043444909,36.4104109333233,-228.195635420535));
#208347=CARTESIAN_POINT('Ctrl Pts',(42.500106112153,36.5011621787222,-228.145358810264));
#208348=CARTESIAN_POINT('Ctrl Pts',(42.5052272864443,36.5322997566167,-228.127432972543));
#208349=CARTESIAN_POINT('Ctrl Pts',(42.5157127222045,36.5801646485169,-228.098833017281));
#208350=CARTESIAN_POINT('Ctrl Pts',(42.5216564611549,36.6043866235847,-228.08410574718));
#208351=CARTESIAN_POINT('Ctrl Pts',(42.5298562807234,36.6331137291362,-228.066190354362));
#208352=CARTESIAN_POINT('Ctrl Pts',(42.5336458407521,36.6455214921606,-228.058357028594));
#208353=CARTESIAN_POINT('Ctrl Pts',(42.5362338683169,36.6538142366302,-228.053100521665));
#208354=CARTESIAN_POINT('Ctrl Pts',(42.537938728552,36.6591389606888,-228.049708921276));
#208355=CARTESIAN_POINT('Ctrl Pts',(42.5545287108761,36.7101243781582,-228.017133053639));
#208356=CARTESIAN_POINT('Ctrl Pts',(42.5747596787098,36.7609669156392,-227.98326264424));
#208357=CARTESIAN_POINT('Ctrl Pts',(42.6131000308354,36.8404500872112,-227.927602813803));
#208358=CARTESIAN_POINT('Ctrl Pts',(42.6272141217683,36.8674793873369,-227.908244075784));
#208359=CARTESIAN_POINT('Ctrl Pts',(42.6505325971428,36.9086798126113,-227.878030386003));
#208360=CARTESIAN_POINT('Ctrl Pts',(42.6627287854389,36.929444028542,-227.862630076912));
#208361=CARTESIAN_POINT('Ctrl Pts',(42.6779304132337,36.9539229855824,-227.844161463063));
#208362=CARTESIAN_POINT('Ctrl Pts',(42.6846574393355,36.9644648178459,-227.836140473796));
#208363=CARTESIAN_POINT('Ctrl Pts',(42.6891896446285,36.9715036068993,-227.830769810322));
#208364=CARTESIAN_POINT('Ctrl Pts',(42.6922398709184,36.9761885029208,-227.827182725376));
#208365=CARTESIAN_POINT('Ctrl Pts',(42.7435040992353,37.0543999679727,-227.767172645826));
#208366=CARTESIAN_POINT('Ctrl Pts',(42.8141078943411,37.1483536050482,-227.691606152183));
#208367=CARTESIAN_POINT('Ctrl Pts',(42.9157357330403,37.2503223096489,-227.60005));
#208368=CARTESIAN_POINT('Ctrl Pts',(42.3284659498332,37.323247286775,-227.257657541791));
#208369=CARTESIAN_POINT('Ctrl Pts',(42.2811180628148,37.2757753423908,-227.328721687048));
#208370=CARTESIAN_POINT('Ctrl Pts',(42.2176885536698,37.1997647460476,-227.434077804087));
#208371=CARTESIAN_POINT('Ctrl Pts',(42.1571641943227,37.102490126336,-227.554823097481));
#208372=CARTESIAN_POINT('Ctrl Pts',(42.1341311988921,37.0589366221338,-227.606106042546));
#208373=CARTESIAN_POINT('Ctrl Pts',(42.1194236021323,37.0294840880552,-227.640191330852));
#208374=CARTESIAN_POINT('Ctrl Pts',(42.1128271528602,37.015528461262,-227.656087200987));
#208375=CARTESIAN_POINT('Ctrl Pts',(42.0771342094186,36.9349109661749,-227.746259228812));
#208376=CARTESIAN_POINT('Ctrl Pts',(42.0554154181983,36.8688204128193,-227.815014008253));
#208377=CARTESIAN_POINT('Ctrl Pts',(42.0331267124034,36.767193592861,-227.913071913187));
#208378=CARTESIAN_POINT('Ctrl Pts',(42.0245542841569,36.7157574583335,-227.960832299597));
#208379=CARTESIAN_POINT('Ctrl Pts',(42.0190571196657,36.6546381121702,-228.01433275981));
#208380=CARTESIAN_POINT('Ctrl Pts',(42.0176663611937,36.6282039350124,-228.036785816201));
#208381=CARTESIAN_POINT('Ctrl Pts',(42.0169536651772,36.6105275347935,-228.051648806624));
#208382=CARTESIAN_POINT('Ctrl Pts',(42.0167229576871,36.6028158122403,-228.058077290188));
#208383=CARTESIAN_POINT('Ctrl Pts',(42.0152804436434,36.5124088085728,-228.132560715103));
#208384=CARTESIAN_POINT('Ctrl Pts',(42.0227620917502,36.4331676079849,-228.191748775822));
#208385=CARTESIAN_POINT('Ctrl Pts',(42.0470046923612,36.3159899802422,-228.270001724761));
#208386=CARTESIAN_POINT('Ctrl Pts',(42.0623804322714,36.2578224973236,-228.306495913695));
#208387=CARTESIAN_POINT('Ctrl Pts',(42.0826088707734,36.2002903559472,-228.339041674326));
#208388=CARTESIAN_POINT('Ctrl Pts',(42.0971692804965,36.1620773525,-228.359861419569));
#208389=CARTESIAN_POINT('Ctrl Pts',(42.1043788617509,36.1444221549774,-228.369138705036));
#208390=CARTESIAN_POINT('Ctrl Pts',(42.1312624500863,36.0833875270383,-228.399817656059));
#208391=CARTESIAN_POINT('Ctrl Pts',(42.1516074709484,36.0435243978327,-228.41787768135));
#208392=CARTESIAN_POINT('Ctrl Pts',(42.1970961458717,35.9654732242671,-228.449212514483));
#208393=CARTESIAN_POINT('Ctrl Pts',(42.2213297257763,35.9285200210562,-228.46212743063));
#208394=CARTESIAN_POINT('Ctrl Pts',(42.3066148061692,35.8127999962566,-228.495853703076));
#208395=CARTESIAN_POINT('Ctrl Pts',(42.3711567239947,35.7427046981823,-228.50707535717));
#208396=CARTESIAN_POINT('Ctrl Pts',(42.4431629103415,35.679860391633,-228.507034483728));
#208397=CARTESIAN_POINT('Origin',(55.4874598092496,36.4953631270247,-218.849954951747));
#208398=CARTESIAN_POINT('',(55.4814981831708,36.4969369346298,-218.349992971048));
#208399=CARTESIAN_POINT('Origin',(55.4874598092437,36.4953631270311,-218.849954951747));
#208400=CARTESIAN_POINT('Origin',(55.4874598092496,36.4953631270247,-218.849954951747));
#208401=CARTESIAN_POINT('Ctrl Pts',(47.045128487469,42.0562187287015,-220.184138377616));
#208402=CARTESIAN_POINT('Ctrl Pts',(47.3919300806126,41.7415300830818,-220.204915325333));
#208403=CARTESIAN_POINT('Ctrl Pts',(47.632114758242,41.9825203546087,-220.52735443572));
#208404=CARTESIAN_POINT('Ctrl Pts',(45.4710211549778,40.4746337203406,-222.538908637374));
#208405=CARTESIAN_POINT('Ctrl Pts',(45.8197306764781,40.1640574272761,-222.557165671255));
#208406=CARTESIAN_POINT('Ctrl Pts',(46.0573262334548,40.4024498941129,-222.881354490551));
#208407=CARTESIAN_POINT('Ctrl Pts',(43.9001479472544,38.8990472866343,-224.898729936232));
#208408=CARTESIAN_POINT('Ctrl Pts',(44.2455143968232,38.5845611308926,-224.921907632466));
#208409=CARTESIAN_POINT('Ctrl Pts',(44.4868142732993,38.8266703421046,-225.241085046204));
#208410=CARTESIAN_POINT('Ctrl Pts',(42.3284659498332,37.3232472867751,-227.257657541791));
#208411=CARTESIAN_POINT('Ctrl Pts',(42.6752110219232,37.0089908641416,-227.278593100034));
#208412=CARTESIAN_POINT('Ctrl Pts',(42.9157357330403,37.2503223096489,-227.60005));
#208413=CARTESIAN_POINT('',(47.045128487469,42.0562187287015,-220.184138377616));
#208414=CARTESIAN_POINT('',(47.632114758242,41.9825203546087,-220.52735443572));
#208415=CARTESIAN_POINT('Origin',(47.2779699369656,42.3354813235036,-220.52735443572));
#208416=CARTESIAN_POINT('Ctrl Pts',(42.9157357330403,37.2503223096489,-227.60005));
#208417=CARTESIAN_POINT('Ctrl Pts',(44.486815106976,38.8266711785776,-225.241083793951));
#208418=CARTESIAN_POINT('Ctrl Pts',(46.0573252848254,40.4024489423018,-222.881355908373));
#208419=CARTESIAN_POINT('Ctrl Pts',(47.632114758242,41.9825203546087,-220.52735443572));
#208420=CARTESIAN_POINT('Ctrl Pts',(47.045128487469,42.0562187287015,-220.184138377616));
#208421=CARTESIAN_POINT('Ctrl Pts',(46.6671603770723,41.6764551098387,-220.74955602554));
#208422=CARTESIAN_POINT('Ctrl Pts',(46.2816417972639,41.2893651286945,-221.326854599969));
#208423=CARTESIAN_POINT('Ctrl Pts',(45.6919698908576,40.6973563649584,-222.210623851371));
#208424=CARTESIAN_POINT('Ctrl Pts',(45.4935115980833,40.4981264890257,-222.508183833464));
#208425=CARTESIAN_POINT('Ctrl Pts',(45.1929349926702,40.1964208373708,-222.958979154044));
#208426=CARTESIAN_POINT('Ctrl Pts',(45.0419240224792,40.0448531632896,-223.185490651193));
#208427=CARTESIAN_POINT('Ctrl Pts',(44.8644692412467,39.8667714265379,-223.451703279039));
#208428=CARTESIAN_POINT('Ctrl Pts',(44.775421562876,39.7774172976856,-223.585296896588));
#208429=CARTESIAN_POINT('Ctrl Pts',(44.7371894799003,39.7390555405282,-223.642655726315));
#208430=CARTESIAN_POINT('Ctrl Pts',(44.7116861193944,39.713466117932,-223.680918151067));
#208431=CARTESIAN_POINT('Ctrl Pts',(44.6978670848006,39.6996007071365,-223.701650844387));
#208432=CARTESIAN_POINT('Ctrl Pts',(43.9368930555956,38.9360854584715,-224.843345868572));
#208433=CARTESIAN_POINT('Ctrl Pts',(43.1511964037071,38.1481333969899,-226.022826588096));
#208434=CARTESIAN_POINT('Ctrl Pts',(42.3284659498332,37.323247286775,-227.257657541791));
#208435=CARTESIAN_POINT('Ctrl Pts',(54.9916284043978,36.4242882801268,-218.85005));
#208436=CARTESIAN_POINT('Ctrl Pts',(54.9916284043978,36.4242882801267,-218.35005));
#208437=CARTESIAN_POINT('Ctrl Pts',(55.4804763444372,36.5293010961029,-218.35005));
#208438=CARTESIAN_POINT('Ctrl Pts',(54.9934502776071,36.4158072299129,-218.850049997976));
#208439=CARTESIAN_POINT('Ctrl Pts',(54.9932481939215,36.4167479617736,-218.351913756624));
#208440=CARTESIAN_POINT('Ctrl Pts',(55.4808808567138,36.5185275155889,-218.35005));
#208441=CARTESIAN_POINT('Ctrl Pts',(54.9951959309483,36.4073227473215,-218.85001713104));
#208442=CARTESIAN_POINT('Ctrl Pts',(54.9948238206649,36.4091341749127,-218.353722457588));
#208443=CARTESIAN_POINT('Ctrl Pts',(55.4812212937741,36.5077394466269,-218.350030277458));
#208444=CARTESIAN_POINT('Ctrl Pts',(54.9968660030035,36.3988348033192,-218.849954951747));
#208445=CARTESIAN_POINT('Ctrl Pts',(54.9963513974766,36.4014502251401,-218.35547736011));
#208446=CARTESIAN_POINT('Ctrl Pts',(55.4814981831709,36.4969369346252,-218.349992971048));
#208447=CARTESIAN_POINT('',(54.9916284043978,36.4242882801268,-218.85005));
#208448=CARTESIAN_POINT('',(55.4804763444372,36.529301096103,-218.35005));
#208449=CARTESIAN_POINT('Origin',(55.4804763444372,36.529301096103,-218.85005));
#208450=CARTESIAN_POINT('Ctrl Pts',(55.4814981831708,36.4969369346298,-218.349992971048));
#208451=CARTESIAN_POINT('Ctrl Pts',(55.4812216183662,36.507726772777,-218.350030233692));
#208452=CARTESIAN_POINT('Ctrl Pts',(55.4808813172563,36.5185152497272,-218.35005));
#208453=CARTESIAN_POINT('Ctrl Pts',(55.4804763444372,36.5293010961029,-218.35005));
#208454=CARTESIAN_POINT('Ctrl Pts',(54.9916284043978,36.4242882801268,-218.85005));
#208455=CARTESIAN_POINT('Ctrl Pts',(54.9934477121007,36.4158191726697,-218.850049997978));
#208456=CARTESIAN_POINT('Ctrl Pts',(54.9951937291456,36.4073339377235,-218.850017211078));
#208457=CARTESIAN_POINT('Ctrl Pts',(54.9968660030035,36.3988348033193,-218.849954951747));
#208458=CARTESIAN_POINT('Ctrl Pts',(47.6321147582419,41.9825203546088,-220.52735443572));
#208459=CARTESIAN_POINT('Ctrl Pts',(47.3919300806125,41.7415300830818,-220.204915325333));
#208460=CARTESIAN_POINT('Ctrl Pts',(47.0451284874689,42.0562187287016,-220.184138377616));
#208461=CARTESIAN_POINT('Ctrl Pts',(47.7902484566451,42.1411844429755,-220.212182607147));
#208462=CARTESIAN_POINT('Ctrl Pts',(47.5344785649843,41.9530961111727,-219.935794482803));
#208463=CARTESIAN_POINT('Ctrl Pts',(47.255889523814,42.2679809657455,-219.868852497358));
#208464=CARTESIAN_POINT('Ctrl Pts',(47.979916006804,42.2643583982894,-219.907394043497));
#208465=CARTESIAN_POINT('Ctrl Pts',(47.7321494909123,42.1394451765273,-219.649704637013));
#208466=CARTESIAN_POINT('Ctrl Pts',(47.5083824724237,42.4326649364373,-219.563965012339));
#208467=CARTESIAN_POINT('Ctrl Pts',(48.3223344522033,42.3817233472697,-219.469720269686));
#208468=CARTESIAN_POINT('Ctrl Pts',(48.1175959253334,42.3304889669946,-219.231029546912));
#208469=CARTESIAN_POINT('Ctrl Pts',(47.9638307571195,42.5902413709234,-219.126165729975));
#208470=CARTESIAN_POINT('Ctrl Pts',(48.4441285568109,42.4082510978142,-219.330335434312));
#208471=CARTESIAN_POINT('Ctrl Pts',(48.2547747023757,42.3779588184084,-219.098571457423));
#208472=CARTESIAN_POINT('Ctrl Pts',(48.1257697081393,42.6260372470741,-218.986746587154));
#208473=CARTESIAN_POINT('Ctrl Pts',(48.7024187673651,42.4292025475747,-219.071888450679));
#208474=CARTESIAN_POINT('Ctrl Pts',(48.5489925463845,42.4312682822061,-218.853050886544));
#208475=CARTESIAN_POINT('Ctrl Pts',(48.4690711499939,42.6549505391914,-218.728256059428));
#208476=CARTESIAN_POINT('Ctrl Pts',(48.8408569866003,42.4234942721779,-218.951187879954));
#208477=CARTESIAN_POINT('Ctrl Pts',(48.7086549671031,42.4384217702358,-218.737132750757));
#208478=CARTESIAN_POINT('Ctrl Pts',(48.653008232647,42.6479010052335,-218.607549287092));
#208479=CARTESIAN_POINT('Ctrl Pts',(48.9829866058019,42.3956441991541,-218.850009606915));
#208480=CARTESIAN_POINT('Ctrl Pts',(48.874649979175,42.4168725889835,-218.639304842979));
#208481=CARTESIAN_POINT('Ctrl Pts',(48.841793010828,42.6113834075459,-218.506376562157));
#208482=CARTESIAN_POINT('',(48.8417930108281,42.6113834075459,-218.506376562157));
#208483=CARTESIAN_POINT('',(48.9829866058019,42.3956441991541,-218.850009606915));
#208484=CARTESIAN_POINT('Origin',(49.0791324003789,42.8863131162308,-218.850009606915));
#208485=CARTESIAN_POINT('Ctrl Pts',(47.6321147582419,41.9825203546088,-220.527354435719));
#208486=CARTESIAN_POINT('Ctrl Pts',(47.6671476766846,42.0176707755733,-220.45753131079));
#208487=CARTESIAN_POINT('Ctrl Pts',(47.702587917472,42.0499288628698,-220.390497026025));
#208488=CARTESIAN_POINT('Ctrl Pts',(47.7381227903546,42.0794845162404,-220.326313799903));
#208489=CARTESIAN_POINT('Ctrl Pts',(47.7765285867267,42.1114280216736,-220.256945100567));
#208490=CARTESIAN_POINT('Ctrl Pts',(47.8150447748923,42.1402149076497,-220.190906713326));
#208491=CARTESIAN_POINT('Ctrl Pts',(47.8532392505425,42.1661345339121,-220.128263389041));
#208492=CARTESIAN_POINT('Ctrl Pts',(47.8771525096411,42.1823626068991,-220.089042899195));
#208493=CARTESIAN_POINT('Ctrl Pts',(47.9009389144252,42.1974677336501,-220.051152968164));
#208494=CARTESIAN_POINT('Ctrl Pts',(47.9244865778018,42.2115289122536,-220.014607284998));
#208495=CARTESIAN_POINT('Ctrl Pts',(47.9717155479152,42.2397310728417,-219.941308505817));
#208496=CARTESIAN_POINT('Ctrl Pts',(48.0179957113527,42.2637421484083,-219.873396984484));
#208497=CARTESIAN_POINT('Ctrl Pts',(48.0625242392206,42.2842897519008,-219.810804136404));
#208498=CARTESIAN_POINT('Ctrl Pts',(48.0965454910983,42.2999887931083,-219.762981152977));
#208499=CARTESIAN_POINT('Ctrl Pts',(48.1295446337251,42.3136683515992,-219.718260357638));
#208500=CARTESIAN_POINT('Ctrl Pts',(48.161211549205,42.3256611217467,-219.67656254218));
#208501=CARTESIAN_POINT('Ctrl Pts',(48.1709917013847,42.3293650226578,-219.663684401869));
#208502=CARTESIAN_POINT('Ctrl Pts',(48.1806451362829,42.3329079837966,-219.651094352271));
#208503=CARTESIAN_POINT('Ctrl Pts',(48.1901636764875,42.3362995838709,-219.638789476176));
#208504=CARTESIAN_POINT('Ctrl Pts',(48.1914442602548,42.3367558752671,-219.637134030673));
#208505=CARTESIAN_POINT('Ctrl Pts',(48.1918676801253,42.3369073614638,-219.636586003471));
#208506=CARTESIAN_POINT('Ctrl Pts',(48.1939977635784,42.337660147459,-219.633838241004));
#208507=CARTESIAN_POINT('Ctrl Pts',(48.1987254711478,42.3393309515031,-219.627739598532));
#208508=CARTESIAN_POINT('Ctrl Pts',(48.2034571415651,42.3409777836824,-219.621663132572));
#208509=CARTESIAN_POINT('Ctrl Pts',(48.2081925863628,42.3426008804874,-219.615608748564));
#208510=CARTESIAN_POINT('Ctrl Pts',(48.2505195271242,42.357108645914,-219.561492701556));
#208511=CARTESIAN_POINT('Ctrl Pts',(48.2928719490673,42.3695301859433,-219.509592142788));
#208512=CARTESIAN_POINT('Ctrl Pts',(48.3351019107294,42.3799619787972,-219.459922348728));
#208513=CARTESIAN_POINT('Ctrl Pts',(48.3798530128249,42.3910165525801,-219.407287254176));
#208514=CARTESIAN_POINT('Ctrl Pts',(48.4244665059068,42.3998369007734,-219.357157107164));
#208515=CARTESIAN_POINT('Ctrl Pts',(48.4687832982745,42.4065723067832,-219.30950325958));
#208516=CARTESIAN_POINT('Ctrl Pts',(48.5038177012274,42.4118969459458,-219.271830765491));
#208517=CARTESIAN_POINT('Ctrl Pts',(48.5386670314813,42.4159193551787,-219.235704827783));
#208518=CARTESIAN_POINT('Ctrl Pts',(48.5732599550489,42.4187257113642,-219.201093557407));
#208519=CARTESIAN_POINT('Ctrl Pts',(48.6064110596672,42.4214150997681,-219.167924870669));
#208520=CARTESIAN_POINT('Ctrl Pts',(48.6394527787534,42.4229783080772,-219.136041680009));
#208521=CARTESIAN_POINT('Ctrl Pts',(48.6722329973828,42.4234626745377,-219.105527001474));
#208522=CARTESIAN_POINT('Ctrl Pts',(48.7065599782558,42.4239698962379,-219.073572462115));
#208523=CARTESIAN_POINT('Ctrl Pts',(48.740600205348,42.4232941558778,-219.043118528264));
#208524=CARTESIAN_POINT('Ctrl Pts',(48.7742098510797,42.4215075438899,-219.014215586192));
#208525=CARTESIAN_POINT('Ctrl Pts',(48.8101746554899,42.4195957370468,-218.983287302483));
#208526=CARTESIAN_POINT('Ctrl Pts',(48.8456463337473,42.416411997341,-218.954134987967));
#208527=CARTESIAN_POINT('Ctrl Pts',(48.8804839718521,42.4120632042333,-218.926770715568));
#208528=CARTESIAN_POINT('Ctrl Pts',(48.9153216099568,42.4077144111257,-218.899406443168));
#208529=CARTESIAN_POINT('Ctrl Pts',(48.9495255120609,42.4022008472995,-218.873829660666));
#208530=CARTESIAN_POINT('Ctrl Pts',(48.9829866058019,42.3956441991541,-218.850009606915));
#208531=CARTESIAN_POINT('Ctrl Pts',(48.841793010828,42.6113834075459,-218.506376562157));
#208532=CARTESIAN_POINT('Ctrl Pts',(48.7921389548229,42.6209882435831,-218.532986949914));
#208533=CARTESIAN_POINT('Ctrl Pts',(48.7423679185265,42.6286450457463,-218.561188681117));
#208534=CARTESIAN_POINT('Ctrl Pts',(48.6924667173058,42.634401307697,-218.59095945731));
#208535=CARTESIAN_POINT('Ctrl Pts',(48.6430231770834,42.640104776999,-218.620457195524));
#208536=CARTESIAN_POINT('Ctrl Pts',(48.5934540403996,42.6439416775049,-218.651494363475));
#208537=CARTESIAN_POINT('Ctrl Pts',(48.543772185369,42.6459227720059,-218.6840600903));
#208538=CARTESIAN_POINT('Ctrl Pts',(48.4932286959486,42.6479382247078,-218.717190605821));
#208539=CARTESIAN_POINT('Ctrl Pts',(48.4425606545126,42.6480337331324,-218.751907906809));
#208540=CARTESIAN_POINT('Ctrl Pts',(48.3917898255881,42.6461829344346,-218.788225803387));
#208541=CARTESIAN_POINT('Ctrl Pts',(48.3715210860928,42.6454440582441,-218.80272464062));
#208542=CARTESIAN_POINT('Ctrl Pts',(48.3512361589158,42.6443945431748,-218.817478808531));
#208543=CARTESIAN_POINT('Ctrl Pts',(48.3309376355839,42.6430308843516,-218.832489881455));
#208544=CARTESIAN_POINT('Ctrl Pts',(48.3233495728856,42.6425211167946,-218.838101371544));
#208545=CARTESIAN_POINT('Ctrl Pts',(48.3152632055342,42.6419301470072,-218.844118980124));
#208546=CARTESIAN_POINT('Ctrl Pts',(48.3076677770069,42.6413300633137,-218.849806740241));
#208547=CARTESIAN_POINT('Ctrl Pts',(48.3041115100809,42.6410490972321,-218.852469814894));
#208548=CARTESIAN_POINT('Ctrl Pts',(48.3006625067958,42.6407667959799,-218.85506030479));
#208549=CARTESIAN_POINT('Ctrl Pts',(48.2974204929156,42.6404937520387,-218.857501393121));
#208550=CARTESIAN_POINT('Ctrl Pts',(48.2971497386314,42.6404709489849,-218.857705258727));
#208551=CARTESIAN_POINT('Ctrl Pts',(48.296880421018,42.6404482119113,-218.857908086002));
#208552=CARTESIAN_POINT('Ctrl Pts',(48.2966125980265,42.6404255474864,-218.858109829903));
#208553=CARTESIAN_POINT('Ctrl Pts',(48.2228468677989,42.6341831489165,-218.913675582879));
#208554=CARTESIAN_POINT('Ctrl Pts',(48.1497074685359,42.6239015850986,-218.971998779091));
#208555=CARTESIAN_POINT('Ctrl Pts',(48.0772565138272,42.609556511184,-219.033078804808));
#208556=CARTESIAN_POINT('Ctrl Pts',(48.0685873731365,42.6078400470672,-219.040387353584));
#208557=CARTESIAN_POINT('Ctrl Pts',(48.0599281431717,42.6060654018618,-219.047735343152));
#208558=CARTESIAN_POINT('Ctrl Pts',(48.0512789750459,42.6042325345101,-219.05512274593));
#208559=CARTESIAN_POINT('Ctrl Pts',(48.0108123723846,42.5956571531817,-219.089685965027));
#208560=CARTESIAN_POINT('Ctrl Pts',(47.9705646754492,42.5858071104717,-219.1251129597));
#208561=CARTESIAN_POINT('Ctrl Pts',(47.9305490404132,42.5746767894346,-219.161403956555));
#208562=CARTESIAN_POINT('Ctrl Pts',(47.9105412228952,42.5691116289161,-219.179549454982));
#208563=CARTESIAN_POINT('Ctrl Pts',(47.8905914347185,42.5632263822981,-219.197910966478));
#208564=CARTESIAN_POINT('Ctrl Pts',(47.8707014981217,42.5570201524988,-219.216488612424));
#208565=CARTESIAN_POINT('Ctrl Pts',(47.8607565298232,42.5539170375991,-219.225777435397));
#208566=CARTESIAN_POINT('Ctrl Pts',(47.8508265142323,42.5507336940937,-219.235120285671));
#208567=CARTESIAN_POINT('Ctrl Pts',(47.8409116461696,42.5474700662204,-219.244517159201));
#208568=CARTESIAN_POINT('Ctrl Pts',(47.8337212795827,42.5451032489654,-219.251331870706));
#208569=CARTESIAN_POINT('Ctrl Pts',(47.8260625557433,42.5425331118276,-219.258629887513));
#208570=CARTESIAN_POINT('Ctrl Pts',(47.8189725322148,42.5401089729406,-219.265421986316));
#208571=CARTESIAN_POINT('Ctrl Pts',(47.8165753157007,42.5392893443809,-219.267718471138));
#208572=CARTESIAN_POINT('Ctrl Pts',(47.8142428881523,42.5384867810019,-219.269956972505));
#208573=CARTESIAN_POINT('Ctrl Pts',(47.8120146859391,42.5377158576958,-219.272098836301));
#208574=CARTESIAN_POINT('Ctrl Pts',(47.8117458163428,42.5376228329978,-219.272357287733));
#208575=CARTESIAN_POINT('Ctrl Pts',(47.8114784723229,42.5375302752592,-219.272614321647));
#208576=CARTESIAN_POINT('Ctrl Pts',(47.8112127226038,42.537438210317,-219.272869870324));
#208577=CARTESIAN_POINT('Ctrl Pts',(47.731812238609,42.5099311220856,-219.349222495541));
#208578=CARTESIAN_POINT('Ctrl Pts',(47.6546767982,42.4779131198223,-219.427655041056));
#208579=CARTESIAN_POINT('Ctrl Pts',(47.5799714073587,42.4412550793883,-219.508179149439));
#208580=CARTESIAN_POINT('Ctrl Pts',(47.5061288943132,42.4050204543033,-219.587773171461));
#208581=CARTESIAN_POINT('Ctrl Pts',(47.4346606908892,42.3642522713035,-219.669410737826));
#208582=CARTESIAN_POINT('Ctrl Pts',(47.3656965554581,42.3188657023054,-219.753094765277));
#208583=CARTESIAN_POINT('Ctrl Pts',(47.2978184355232,42.2741938601279,-219.835460975139));
#208584=CARTESIAN_POINT('Ctrl Pts',(47.2323661737487,42.2250479023035,-219.919809709308));
#208585=CARTESIAN_POINT('Ctrl Pts',(47.169433903332,42.1713867096496,-220.006135435357));
#208586=CARTESIAN_POINT('Ctrl Pts',(47.1268378225816,42.1350658129092,-220.064565515398));
#208587=CARTESIAN_POINT('Ctrl Pts',(47.0853956260421,42.0966771525707,-220.123901151368));
#208588=CARTESIAN_POINT('Ctrl Pts',(47.0451284874691,42.0562187287014,-220.184138377616));
#208589=CARTESIAN_POINT('Origin',(53.5250845842796,36.1092498321983,-218.85005));
#208590=CARTESIAN_POINT('',(54.6328983814091,37.1205601658197,-218.85005));
#208591=CARTESIAN_POINT('',(55.0021696471189,37.4576636103602,-218.35005));
#208592=CARTESIAN_POINT('Origin',(55.0021696471189,37.4576636103602,-218.85005));
#208593=CARTESIAN_POINT('Origin',(53.5250845842796,36.1092498321983,-218.35005));
#208594=CARTESIAN_POINT('Origin',(53.5250845842796,36.1092498321983,-218.85005));
#208595=CARTESIAN_POINT('Origin',(49.0791324003789,42.8863131162308,-218.850009606915));
#208596=CARTESIAN_POINT('',(49.0801870931398,42.8824343798319,-218.350025764149));
#208597=CARTESIAN_POINT('Origin',(49.0791324003789,42.8863131162308,-218.850009606915));
#208598=CARTESIAN_POINT('Origin',(49.0791324003789,42.8863131162308,-218.850009606915));
#208599=CARTESIAN_POINT('Origin',(0.128459562639233,-12.6359082483571,-218.85005));
#208600=CARTESIAN_POINT('',(49.7021444432209,42.0348313420379,-218.85005));
#208601=CARTESIAN_POINT('',(50.0380095169376,42.4052293067426,-218.35005));
#208602=CARTESIAN_POINT('Origin',(50.0380095169376,42.4052293067426,-218.85005));
#208603=CARTESIAN_POINT('Origin',(0.128459562639233,-12.6359082483571,-218.35005));
#208604=CARTESIAN_POINT('Origin',(0.128459562639233,-12.6359082483571,-218.85005));
#208605=CARTESIAN_POINT('Ctrl Pts',(49.1011166787324,42.8818771940186,-218.35005));
#208606=CARTESIAN_POINT('Ctrl Pts',(48.9994748145671,42.3923172574951,-218.35005));
#208607=CARTESIAN_POINT('Ctrl Pts',(48.999474814567,42.392317257495,-218.85005));
#208608=CARTESIAN_POINT('Ctrl Pts',(49.09414603136,42.8820897398471,-218.35005));
#208609=CARTESIAN_POINT('Ctrl Pts',(48.994587444257,42.3933319685669,-218.351257450515));
#208610=CARTESIAN_POINT('Ctrl Pts',(48.9939799633645,42.3934580921056,-218.85004999869));
#208611=CARTESIAN_POINT('Ctrl Pts',(49.0871694989175,42.882275419924,-218.350041726378));
#208612=CARTESIAN_POINT('Ctrl Pts',(48.9896694475663,42.3943279693454,-218.352441808199));
#208613=CARTESIAN_POINT('Ctrl Pts',(48.9884838968603,42.394567013707,-218.850036211906));
#208614=CARTESIAN_POINT('Ctrl Pts',(49.0801870931398,42.8824343798319,-218.350025764149));
#208615=CARTESIAN_POINT('Ctrl Pts',(48.9847217242793,42.3953042054457,-218.353603405568));
#208616=CARTESIAN_POINT('Ctrl Pts',(48.9829866058019,42.3956441991541,-218.850009606915));
#208617=CARTESIAN_POINT('',(49.1011166787325,42.8818771940186,-218.35005));
#208618=CARTESIAN_POINT('',(48.999474814567,42.392317257495,-218.85005));
#208619=CARTESIAN_POINT('Origin',(49.1011166787325,42.8818771940186,-218.85005));
#208620=CARTESIAN_POINT('Ctrl Pts',(48.9829866058019,42.3956441991541,-218.850009606915));
#208621=CARTESIAN_POINT('Ctrl Pts',(48.9884887606911,42.3945660606471,-218.85003623417));
#208622=CARTESIAN_POINT('Ctrl Pts',(48.993985033412,42.3934570394682,-218.850049998691));
#208623=CARTESIAN_POINT('Ctrl Pts',(48.999474814567,42.392317257495,-218.85005));
#208624=CARTESIAN_POINT('Ctrl Pts',(49.1011166787325,42.8818771940186,-218.35005));
#208625=CARTESIAN_POINT('Ctrl Pts',(49.0941409157939,42.8820898960309,-218.35005));
#208626=CARTESIAN_POINT('Ctrl Pts',(49.0871642720694,42.8822755387356,-218.35004171443));
#208627=CARTESIAN_POINT('Ctrl Pts',(49.0801870931398,42.8824343798319,-218.350025764149));
#208628=CARTESIAN_POINT('Origin',(48.6945492220708,40.9236374479242,-218.85005));
#208629=CARTESIAN_POINT('Origin',(48.6945492220708,40.9236374479242,-218.85005));
#208630=CARTESIAN_POINT('Origin',(48.6945492220708,40.9236374479242,-218.35005));
#208631=CARTESIAN_POINT('Origin',(0.,-178.58000002,-205.84995));
#208632=CARTESIAN_POINT('',(43.4686063353067,49.3549798298524,-205.841223796781));
#208633=CARTESIAN_POINT('Origin',(0.,-178.58000002,-205.841223796781));
#208634=CARTESIAN_POINT('',(43.5622571193626,49.8460535351382,-205.34995));
#208635=CARTESIAN_POINT('Origin',(0.,-178.58000002,-205.34995));
#208636=CARTESIAN_POINT('Origin',(43.5622571193626,49.8460535351382,-205.84995));
#208637=CARTESIAN_POINT('Origin',(41.3132181298675,38.0528376956935,-205.84995));
#208638=CARTESIAN_POINT('',(48.8684365469981,47.38326056293,-205.34995));
#208639=CARTESIAN_POINT('',(48.5538345628697,46.9947384336248,-205.841223796781));
#208640=CARTESIAN_POINT('Origin',(48.8684365469981,47.38326056293,-205.84995));
#208641=CARTESIAN_POINT('Origin',(41.3132181298675,38.0528376956935,-205.841223796781));
#208642=CARTESIAN_POINT('Origin',(41.3132181298675,38.0528376956935,-205.34995));
#208643=CARTESIAN_POINT('Origin',(0.,-12.9675000200281,-205.84995));
#208644=CARTESIAN_POINT('',(59.9876878113059,36.3459434263872,-205.34995));
#208645=CARTESIAN_POINT('',(59.6015030478428,36.0284766063157,-205.841223796781));
#208646=CARTESIAN_POINT('Origin',(59.9876878113059,36.3459434263873,-205.84995));
#208647=CARTESIAN_POINT('Origin',(0.,-12.9675000200281,-205.841223796781));
#208648=CARTESIAN_POINT('Origin',(0.,-12.9675000200281,-205.34995));
#208649=CARTESIAN_POINT('Origin',(50.7133971693864,28.7219255026674,-205.84995));
#208650=CARTESIAN_POINT('',(62.7097829146859,29.1961040154388,-205.34995));
#208651=CARTESIAN_POINT('',(62.2102491422031,29.1763590533857,-205.841223796781));
#208652=CARTESIAN_POINT('Origin',(62.709782914686,29.1961040154388,-205.84995));
#208653=CARTESIAN_POINT('Origin',(50.7133971693864,28.7219255026674,-205.841223796781));
#208654=CARTESIAN_POINT('Origin',(50.7133971693864,28.7219255026674,-205.34995));
#208655=CARTESIAN_POINT('Origin',(-1004.,-12.967500020028,-205.84995));
#208656=CARTESIAN_POINT('',(62.7097829146858,-55.1311040554952,-205.34995));
#208657=CARTESIAN_POINT('',(62.210249142203,-55.1113590934421,-205.841223796781));
#208658=CARTESIAN_POINT('Origin',(62.7097829146858,-55.1311040554952,-205.84995));
#208659=CARTESIAN_POINT('Origin',(-1004.,-12.967500020028,-205.841223796781));
#208660=CARTESIAN_POINT('Origin',(-1004.,-12.967500020028,-205.34995));
#208661=CARTESIAN_POINT('Origin',(50.7133971693864,-54.6569255427236,-205.84995));
#208662=CARTESIAN_POINT('',(59.9876878113058,-62.2809434664435,-205.34995));
#208663=CARTESIAN_POINT('',(59.6015030478428,-61.963476646372,-205.841223796781));
#208664=CARTESIAN_POINT('Origin',(59.9876878113059,-62.2809434664436,-205.84995));
#208665=CARTESIAN_POINT('Origin',(50.7133971693864,-54.6569255427236,-205.841223796781));
#208666=CARTESIAN_POINT('Origin',(50.7133971693864,-54.6569255427236,-205.34995));
#208667=CARTESIAN_POINT('Origin',(0.,-12.9675000200281,-205.84995));
#208668=CARTESIAN_POINT('',(49.142885306769,-73.0949913797652,-205.34995));
#208669=CARTESIAN_POINT('',(48.8265164945923,-72.7079065982776,-205.841223796781));
#208670=CARTESIAN_POINT('Origin',(49.142885306769,-73.0949913797652,-205.84995));
#208671=CARTESIAN_POINT('Origin',(0.,-12.9675000200281,-205.841223796781));
#208672=CARTESIAN_POINT('Origin',(0.,-12.9675000200281,-205.34995));
#208673=CARTESIAN_POINT('Origin',(41.5452362233251,-63.7990866568863,-205.84995));
#208674=CARTESIAN_POINT('',(42.0177747166746,-75.7955371145968,-205.34995));
#208675=CARTESIAN_POINT('',(41.998098045614,-75.2960006474661,-205.841223796781));
#208676=CARTESIAN_POINT('Origin',(42.0177747166746,-75.7955371145968,-205.84995));
#208677=CARTESIAN_POINT('Origin',(41.5452362233251,-63.7990866568863,-205.841223796781));
#208678=CARTESIAN_POINT('Origin',(41.5452362233251,-63.7990866568863,-205.34995));
#208679=CARTESIAN_POINT('Origin',(0.,990.91999998,-205.84995));
#208680=CARTESIAN_POINT('Origin',(0.,990.91999998,-205.34995));
#208681=CARTESIAN_POINT('Origin',(0.,990.91999998,-205.841223796781));
#208682=CARTESIAN_POINT('Ctrl Pts',(55.1063041457933,-62.4061442430715,
-218.35005));
#208683=CARTESIAN_POINT('Ctrl Pts',(54.9567009523894,-62.2733518205981,
-218.35005));
#208684=CARTESIAN_POINT('Ctrl Pts',(54.8483808955536,-62.1772035872457,
-218.488025452358));
#208685=CARTESIAN_POINT('Ctrl Pts',(55.189518743021,-62.3123951476979,-218.35005));
#208686=CARTESIAN_POINT('Ctrl Pts',(55.0396688463657,-62.1798977449584,
-218.35005000001));
#208687=CARTESIAN_POINT('Ctrl Pts',(54.9311672479814,-62.0839582776323,
-218.48801196499));
#208688=CARTESIAN_POINT('Ctrl Pts',(55.2724546450001,-62.2184167144346,
-218.35005));
#208689=CARTESIAN_POINT('Ctrl Pts',(55.1223583736958,-62.0862177900441,
-218.350049999979));
#208690=CARTESIAN_POINT('Ctrl Pts',(55.0136740740194,-61.9904901268701,
-218.487996778695));
#208691=CARTESIAN_POINT('Ctrl Pts',(55.3551085347194,-62.1242062049499,
-218.35005));
#208692=CARTESIAN_POINT('Ctrl Pts',(55.204767621478,-61.9923073188158,-218.35005));
#208693=CARTESIAN_POINT('Ctrl Pts',(55.0958998011493,-61.8967941020366,
-218.487980161586));
#208694=CARTESIAN_POINT('',(55.3551085347089,-62.1242062049619,-218.35005));
#208695=CARTESIAN_POINT('Origin',(6.53661563613523,-19.2936643109222,-218.35005));
#208696=CARTESIAN_POINT('',(55.0958998011388,-61.8967941020485,-218.487980161586));
#208697=CARTESIAN_POINT('Origin',(6.32111438748812,-19.0925318432536,-218.204998012194));
#208698=CARTESIAN_POINT('Origin',(55.3551085347089,-62.1242062049619,-218.85005));
#208699=CARTESIAN_POINT('Ctrl Pts',(55.2339673727997,-61.7389489519143,
-218.487950878256));
#208700=CARTESIAN_POINT('Ctrl Pts',(55.3431423575669,-61.8341015991581,
-218.35005));
#208701=CARTESIAN_POINT('Ctrl Pts',(55.4938952567199,-61.9654919306031,
-218.35005));
#208702=CARTESIAN_POINT('Ctrl Pts',(55.1880309233148,-61.7916386130721,
-218.487961072495));
#208703=CARTESIAN_POINT('Ctrl Pts',(55.2971033694472,-61.8869121544979,
-218.350049999996));
#208704=CARTESIAN_POINT('Ctrl Pts',(55.4477195716702,-62.0184723768345,
-218.35005));
#208705=CARTESIAN_POINT('Ctrl Pts',(55.14200840849,-61.8442534512036,-218.487970843436));
#208706=CARTESIAN_POINT('Ctrl Pts',(55.2509784443238,-61.9396472076622,
-218.350050000013));
#208707=CARTESIAN_POINT('Ctrl Pts',(55.4014572374666,-62.0713770530022,
-218.35005));
#208708=CARTESIAN_POINT('Ctrl Pts',(55.0958998011388,-61.8967941020486,
-218.487980161586));
#208709=CARTESIAN_POINT('Ctrl Pts',(55.2047676214677,-61.9923073188278,
-218.35005));
#208710=CARTESIAN_POINT('Ctrl Pts',(55.3551085347089,-62.1242062049619,
-218.35005));
#208711=CARTESIAN_POINT('',(55.2339673727996,-61.7389489519143,-218.487950878256));
#208712=CARTESIAN_POINT('',(55.4938952567199,-61.9654919306031,-218.35005));
#208713=CARTESIAN_POINT('Origin',(55.4938952567198,-61.9654919306031,-218.85005));
#208714=CARTESIAN_POINT('Ctrl Pts',(55.3551085347089,-62.1242062049619,
-218.35005));
#208715=CARTESIAN_POINT('Ctrl Pts',(55.4014571755248,-62.0713771235952,
-218.35005));
#208716=CARTESIAN_POINT('Ctrl Pts',(55.4477196335097,-62.0184723058819,
-218.35005));
#208717=CARTESIAN_POINT('Ctrl Pts',(55.4938952567199,-61.9654919306031,
-218.35005));
#208718=CARTESIAN_POINT('Origin',(7.62393634648824,-43.3515330069781,-218.305892816451));
#208719=CARTESIAN_POINT('Ctrl Pts',(49.4570218871579,-69.5396831399799,
-217.525618242158));
#208720=CARTESIAN_POINT('Ctrl Pts',(49.2592415957564,-69.455430883311,-217.233755494175));
#208721=CARTESIAN_POINT('Ctrl Pts',(49.1082596796586,-69.7601043330141,
-217.107989577217));
#208722=CARTESIAN_POINT('Ctrl Pts',(49.2622754448157,-69.4954973356379,
-217.612334261911));
#208723=CARTESIAN_POINT('Ctrl Pts',(49.0757606270564,-69.4511605712625,
-217.34710501445));
#208724=CARTESIAN_POINT('Ctrl Pts',(48.912676519449,-69.7205296868298,-217.252740911407));
#208725=CARTESIAN_POINT('Ctrl Pts',(49.0788953913437,-69.440810795047,-217.70194766018));
#208726=CARTESIAN_POINT('Ctrl Pts',(48.8940785173341,-69.4269663422441,
-217.47286760646));
#208727=CARTESIAN_POINT('Ctrl Pts',(48.7307698712856,-69.6620794550121,
-217.402284510414));
#208728=CARTESIAN_POINT('Ctrl Pts',(48.7966565591402,-69.3194187518267,
-217.863510508004));
#208729=CARTESIAN_POINT('Ctrl Pts',(48.6179833119651,-69.3347292882382,
-217.703261160372));
#208730=CARTESIAN_POINT('Ctrl Pts',(48.4568130848015,-69.5116847789954,
-217.67207172234));
#208731=CARTESIAN_POINT('Ctrl Pts',(48.6861912261675,-69.2595360633236,
-217.934600613269));
#208732=CARTESIAN_POINT('Ctrl Pts',(48.5105553232489,-69.2816866454383,
-217.805049640232));
#208733=CARTESIAN_POINT('Ctrl Pts',(48.3516107950449,-69.4327456757647,
-217.790813441481));
#208734=CARTESIAN_POINT('Ctrl Pts',(48.5120925091425,-69.1176128201212,
-218.077169784276));
#208735=CARTESIAN_POINT('Ctrl Pts',(48.346506115558,-69.1351464133951,-218.00756927047));
#208736=CARTESIAN_POINT('Ctrl Pts',(48.1935846999847,-69.2311811089996,
-218.029011852183));
#208737=CARTESIAN_POINT('Ctrl Pts',(48.44853190302,-69.0341658346798,-218.149562838542));
#208738=CARTESIAN_POINT('Ctrl Pts',(48.2881462840732,-69.0394916099964,
-218.110930665774));
#208739=CARTESIAN_POINT('Ctrl Pts',(48.141063563618,-69.1062596209728,-218.149999563001));
#208740=CARTESIAN_POINT('Ctrl Pts',(48.4345085199297,-68.8996986141391,
-218.239932923561));
#208741=CARTESIAN_POINT('Ctrl Pts',(48.2846281886007,-68.8713617818855,
-218.233863811861));
#208742=CARTESIAN_POINT('Ctrl Pts',(48.1484532516179,-68.8904009633176,
-218.301080288388));
#208743=CARTESIAN_POINT('Ctrl Pts',(48.4438278731385,-68.8541286362714,
-218.266363445181));
#208744=CARTESIAN_POINT('Ctrl Pts',(48.2975896440283,-68.8120721221255,
-218.268779191712));
#208745=CARTESIAN_POINT('Ctrl Pts',(48.1656057057525,-68.8149306500085,
-218.345277024483));
#208746=CARTESIAN_POINT('Ctrl Pts',(48.507784321035,-68.732929092821,-218.324806358094));
#208747=CARTESIAN_POINT('Ctrl Pts',(48.3709960733748,-68.6498345611464,
-218.341572514799));
#208748=CARTESIAN_POINT('Ctrl Pts',(48.2519986346533,-68.6077656957913,
-218.443032871038));
#208749=CARTESIAN_POINT('Ctrl Pts',(48.5915006514379,-68.6628850039255,
-218.344419445302));
#208750=CARTESIAN_POINT('Ctrl Pts',(48.4608840740975,-68.5494670324552,
-218.359917285752));
#208751=CARTESIAN_POINT('Ctrl Pts',(48.3506511305266,-68.4802802531201,
-218.475898114176));
#208752=CARTESIAN_POINT('Ctrl Pts',(48.6940335790739,-68.6081147401982,
-218.348150004632));
#208753=CARTESIAN_POINT('Ctrl Pts',(48.5650271218342,-68.4711538784475,
-218.353348100088));
#208754=CARTESIAN_POINT('Ctrl Pts',(48.4661517708994,-68.3748018054678,
-218.482144505478));
#208755=CARTESIAN_POINT('',(48.9443109379934,-69.7210624363875,-217.233400031701));
#208756=CARTESIAN_POINT('Ctrl Pts',(48.3245605310987,-68.5271120961857,
-218.45762963148));
#208757=CARTESIAN_POINT('Ctrl Pts',(48.2969090264087,-68.5624400955583,
-218.448765818759));
#208758=CARTESIAN_POINT('Ctrl Pts',(48.272373979724,-68.5979809825957,-218.437849245981));
#208759=CARTESIAN_POINT('Ctrl Pts',(48.2296118037038,-68.6694696560977,
-218.411910580311));
#208760=CARTESIAN_POINT('Ctrl Pts',(48.2118419283057,-68.7043185904572,
-218.39740761229));
#208761=CARTESIAN_POINT('Ctrl Pts',(48.1808487368591,-68.7788024321227,
-218.362219656654));
#208762=CARTESIAN_POINT('Ctrl Pts',(48.1629168738174,-68.8344186687614,
-218.332820537156));
#208763=CARTESIAN_POINT('Ctrl Pts',(48.1530254853042,-68.8896516378129,
-218.2989091885));
#208764=CARTESIAN_POINT('Ctrl Pts',(48.1482245464656,-68.9263872954923,
-218.275298905138));
#208765=CARTESIAN_POINT('Ctrl Pts',(48.1466843549373,-68.9458148942746,
-218.262219668185));
#208766=CARTESIAN_POINT('Ctrl Pts',(48.1449816941239,-68.997348945024,-218.226114299801));
#208767=CARTESIAN_POINT('Ctrl Pts',(48.1481130692551,-69.0481950185523,
-218.18764191845));
#208768=CARTESIAN_POINT('Ctrl Pts',(48.1585276426128,-69.0980066943639,
-218.145619017648));
#208769=CARTESIAN_POINT('Ctrl Pts',(48.1670914404119,-69.1309846393012,
-218.116814746125));
#208770=CARTESIAN_POINT('Ctrl Pts',(48.172730617193,-69.1488647385631,-218.100610979771));
#208771=CARTESIAN_POINT('Ctrl Pts',(48.1888010654547,-69.1931241036076,
-218.059258944812));
#208772=CARTESIAN_POINT('Ctrl Pts',(48.2086778269923,-69.2362855894174,
-218.016459214628));
#208773=CARTESIAN_POINT('Ctrl Pts',(48.2385256773599,-69.2847267297988,
-217.963992729438));
#208774=CARTESIAN_POINT('Ctrl Pts',(48.252743015283,-69.3050781343457,-217.940964207218));
#208775=CARTESIAN_POINT('Ctrl Pts',(48.2625378116414,-69.3185549550489,
-217.925491217803));
#208776=CARTESIAN_POINT('Ctrl Pts',(48.2682837752384,-69.3261280787323,
-217.916654176065));
#208777=CARTESIAN_POINT('Ctrl Pts',(48.3089960702895,-69.378036374536,-217.855301989849));
#208778=CARTESIAN_POINT('Ctrl Pts',(48.3519830933143,-69.4212627364945,
-217.798872847759));
#208779=CARTESIAN_POINT('Ctrl Pts',(48.426557326924,-69.4817802610263,-217.711388336444));
#208780=CARTESIAN_POINT('Ctrl Pts',(48.4663669961376,-69.5109587572413,
-217.666935881241));
#208781=CARTESIAN_POINT('Ctrl Pts',(48.5171938223511,-69.5431236077837,
-217.613831834301));
#208782=CARTESIAN_POINT('Ctrl Pts',(48.5399117039659,-69.5565080736488,
-217.590806632211));
#208783=CARTESIAN_POINT('Ctrl Pts',(48.5552642540727,-69.5653422517974,
-217.575397314189));
#208784=CARTESIAN_POINT('Ctrl Pts',(48.5641005162855,-69.5702949293905,
-217.566622736532));
#208785=CARTESIAN_POINT('Ctrl Pts',(48.6801593526136,-69.6340177431732,
-217.452322976306));
#208786=CARTESIAN_POINT('Ctrl Pts',(48.8048901567373,-69.6829147138422,
-217.343489913132));
#208787=CARTESIAN_POINT('Ctrl Pts',(48.9443109379934,-69.7210624363875,
-217.233400031701));
#208788=CARTESIAN_POINT('',(49.2925903552098,-69.4989817480832,-217.60005));
#208789=CARTESIAN_POINT('Ctrl Pts',(49.2925903552098,-69.4989817480832,
-217.60005));
#208790=CARTESIAN_POINT('Ctrl Pts',(49.1484673907459,-69.4601446914727,
-217.668076900971));
#208791=CARTESIAN_POINT('Ctrl Pts',(49.0242599947267,-69.4170675539365,
-217.732996299125));
#208792=CARTESIAN_POINT('Ctrl Pts',(48.8668072751,-69.3498582752364,-217.822902511881));
#208793=CARTESIAN_POINT('Ctrl Pts',(48.8191318230071,-69.3270264133442,
-217.851645777573));
#208794=CARTESIAN_POINT('Ctrl Pts',(48.7547036967668,-69.2926109521484,
-217.892735727221));
#208795=CARTESIAN_POINT('Ctrl Pts',(48.7242609407847,-69.2753611405731,
-217.91277605223));
#208796=CARTESIAN_POINT('Ctrl Pts',(48.6918169106576,-69.2552639129,-217.935248183673));
#208797=CARTESIAN_POINT('Ctrl Pts',(48.6763596974272,-69.2452345365248,
-217.946255129638));
#208798=CARTESIAN_POINT('Ctrl Pts',(48.669898709807,-69.2409416675107,-217.950923096411));
#208799=CARTESIAN_POINT('Ctrl Pts',(48.6656276861863,-69.2380811075938,
-217.954024100342));
#208800=CARTESIAN_POINT('Ctrl Pts',(48.6650074713428,-69.2376705467468,
-217.954471148243));
#208801=CARTESIAN_POINT('Ctrl Pts',(48.6038690780288,-69.1960562874253,
-217.999308408621));
#208802=CARTESIAN_POINT('Ctrl Pts',(48.5576057289715,-69.1560179545467,
-218.03878501502));
#208803=CARTESIAN_POINT('Ctrl Pts',(48.5048358437187,-69.0957393063493,
-218.093132674187));
#208804=CARTESIAN_POINT('Ctrl Pts',(48.4826068126659,-69.0655460792566,
-218.119094170054));
#208805=CARTESIAN_POINT('Ctrl Pts',(48.4638790662549,-69.0304739208104,
-218.147136413011));
#208806=CARTESIAN_POINT('Ctrl Pts',(48.4573898341797,-69.0155026490939,
-218.158662749366));
#208807=CARTESIAN_POINT('Ctrl Pts',(48.4534044218793,-69.0055380297188,
-218.166236605228));
#208808=CARTESIAN_POINT('Ctrl Pts',(48.4521313177971,-69.002214019677,-218.168746457979));
#208809=CARTESIAN_POINT('Ctrl Pts',(48.4147042004739,-68.8897627549664,
-218.252011243573));
#208810=CARTESIAN_POINT('Ctrl Pts',(48.4558803503785,-68.7836110335151,
-218.307899599653));
#208811=CARTESIAN_POINT('Ctrl Pts',(48.5701931618903,-68.6892604152372,
-218.333619302448));
#208812=CARTESIAN_POINT('Origin',(49.1624951782473,-69.9817604188332,-217.60005));
#208813=CARTESIAN_POINT('Ctrl Pts',(55.4237479323138,-62.1328188643259,
-218.341144661975));
#208814=CARTESIAN_POINT('Ctrl Pts',(55.2405234564513,-62.0021381064316,
-218.318170442032));
#208815=CARTESIAN_POINT('Ctrl Pts',(55.0928795124925,-61.9237973298156,
-218.473054790165));
#208816=CARTESIAN_POINT('Ctrl Pts',(55.494632995213,-61.9315980237713,-218.361192001577));
#208817=CARTESIAN_POINT('Ctrl Pts',(55.3400279587498,-61.8078970750489,
-218.369232738601));
#208818=CARTESIAN_POINT('Ctrl Pts',(55.2399321713626,-61.7035864993853,
-218.506552167714));
#208819=CARTESIAN_POINT('Ctrl Pts',(55.6064180550928,-61.7413047615639,
-218.350163543339));
#208820=CARTESIAN_POINT('Ctrl Pts',(55.5091017198289,-61.6043114926627,
-218.374336100872));
#208821=CARTESIAN_POINT('Ctrl Pts',(55.4522604695358,-61.4873000226074,
-218.488185460704));
#208822=CARTESIAN_POINT('Ctrl Pts',(55.7967381055322,-61.6583804609248,
-218.254186826194));
#208823=CARTESIAN_POINT('Ctrl Pts',(55.7613184164348,-61.5067436997404,
-218.252944363189));
#208824=CARTESIAN_POINT('Ctrl Pts',(55.774129320809,-61.3703224231151,-218.328019869095));
#208825=CARTESIAN_POINT('Ctrl Pts',(55.8477306234162,-61.6541946099495,
-218.22271673907));
#208826=CARTESIAN_POINT('Ctrl Pts',(55.8266978017486,-61.4985748755131,
-218.210789756319));
#208827=CARTESIAN_POINT('Ctrl Pts',(55.8574329037833,-61.3577410974567,
-218.275498156808));
#208828=CARTESIAN_POINT('Ctrl Pts',(55.9478060913509,-61.6785900219245,
-218.1506974888));
#208829=CARTESIAN_POINT('Ctrl Pts',(55.9489905260305,-61.5152696674129,
-218.112160517346));
#208830=CARTESIAN_POINT('Ctrl Pts',(56.0156028250703,-61.3669778003364,
-218.155301834069));
#208831=CARTESIAN_POINT('Ctrl Pts',(55.9954662711786,-61.7067706426262,
-218.111190879857));
#208832=CARTESIAN_POINT('Ctrl Pts',(56.0045190211886,-61.5400305154986,
-218.056751473387));
#208833=CARTESIAN_POINT('Ctrl Pts',(56.0882300869458,-61.3886089876927,
-218.089366319566));
#208834=CARTESIAN_POINT('Ctrl Pts',(56.1267636112953,-61.8218463607312,
-217.990670505791));
#208835=CARTESIAN_POINT('Ctrl Pts',(56.1502648139586,-61.6460669288342,
-217.886016299921));
#208836=CARTESIAN_POINT('Ctrl Pts',(56.2821971389062,-61.4871566064044,
-217.888227119225));
#208837=CARTESIAN_POINT('Ctrl Pts',(56.1994729047277,-61.9375893837876,
-217.907702178034));
#208838=CARTESIAN_POINT('Ctrl Pts',(56.2191388000639,-61.7583243798369,
-217.767022200493));
#208839=CARTESIAN_POINT('Ctrl Pts',(56.3811156518498,-61.5958538338606,
-217.749769988996));
#208840=CARTESIAN_POINT('Ctrl Pts',(56.3439578714798,-62.2446096393604,
-217.718697327292));
#208841=CARTESIAN_POINT('Ctrl Pts',(56.3359782479612,-62.0576869907416,
-217.49766835849));
#208842=CARTESIAN_POINT('Ctrl Pts',(56.5650907006514,-61.8919890523586,
-217.43440812177));
#208843=CARTESIAN_POINT('Ctrl Pts',(56.4064091508865,-62.4540207436425,
-217.612944268375));
#208844=CARTESIAN_POINT('Ctrl Pts',(56.3631474716341,-62.2659851591403,
-217.349074894179));
#208845=CARTESIAN_POINT('Ctrl Pts',(56.6320495252993,-62.09974891787,-217.258041794045));
#208846=CARTESIAN_POINT('Ctrl Pts',(56.4532198574233,-62.6711239243471,
-217.514416680063));
#208847=CARTESIAN_POINT('Ctrl Pts',(56.363816920114,-62.4684902652751,-217.222377953599));
#208848=CARTESIAN_POINT('Ctrl Pts',(56.6724481617213,-62.3181880639774,
-217.093652670756));
#208849=CARTESIAN_POINT('',(56.6309943627598,-62.1341374253209,-217.237388612086));
#208850=CARTESIAN_POINT('',(56.4090189474477,-62.4870630585556,-217.60005));
#208851=CARTESIAN_POINT('Origin',(56.8921651292037,-62.3583394513399,-217.60005));
#208852=CARTESIAN_POINT('Ctrl Pts',(55.4938952567199,-61.9654919306031,
-218.35005));
#208853=CARTESIAN_POINT('Ctrl Pts',(55.57896365653,-61.7965571013242,-218.35005));
#208854=CARTESIAN_POINT('Ctrl Pts',(55.6778758905696,-61.6964283653063,
-218.318350028606));
#208855=CARTESIAN_POINT('Ctrl Pts',(55.8312897454811,-61.6535904959217,
-218.233316266271));
#208856=CARTESIAN_POINT('Ctrl Pts',(55.8841740643655,-61.6572520033479,
-218.198283210441));
#208857=CARTESIAN_POINT('Ctrl Pts',(55.9636629054506,-61.6903101237091,
-218.136750461095));
#208858=CARTESIAN_POINT('Ctrl Pts',(55.990187345622,-61.7059235141358,-218.114749592215));
#208859=CARTESIAN_POINT('Ctrl Pts',(56.0297268316923,-61.7363117331637,
-218.079709596312));
#208860=CARTESIAN_POINT('Ctrl Pts',(56.0494350297545,-61.7532478097978,
-218.061680601021));
#208861=CARTESIAN_POINT('Ctrl Pts',(56.0722599880634,-61.7760710568074,
-218.039806012764));
#208862=CARTESIAN_POINT('Ctrl Pts',(56.0836232219663,-61.7882507374176,
-218.028665294619));
#208863=CARTESIAN_POINT('Ctrl Pts',(56.0884818569286,-61.7936353893167,
-218.023847847065));
#208864=CARTESIAN_POINT('Ctrl Pts',(56.0917183460573,-61.7972617995588,
-218.020626775486));
#208865=CARTESIAN_POINT('Ctrl Pts',(56.0940933660921,-61.7999613204208,
-218.018251410963));
#208866=CARTESIAN_POINT('Ctrl Pts',(56.2047141650995,-61.9266217894036,
-217.90733398084));
#208867=CARTESIAN_POINT('Ctrl Pts',(56.319891141774,-62.1525342185782,-217.762647327886));
#208868=CARTESIAN_POINT('Ctrl Pts',(56.4090189474477,-62.4870630585556,
-217.60005));
#208869=CARTESIAN_POINT('Ctrl Pts',(56.6309943627598,-62.1341374253209,
-217.237388612085));
#208870=CARTESIAN_POINT('Ctrl Pts',(56.6169100679614,-62.0818886112393,
-217.279832325573));
#208871=CARTESIAN_POINT('Ctrl Pts',(56.6012339430048,-62.0318061452899,
-217.32206232518));
#208872=CARTESIAN_POINT('Ctrl Pts',(56.5839430146363,-61.983949822002,-217.364070353647));
#208873=CARTESIAN_POINT('Ctrl Pts',(56.5749805387295,-61.9591442629644,
-217.385844542691));
#208874=CARTESIAN_POINT('Ctrl Pts',(56.565584111166,-61.9349359769846,-217.407559629734));
#208875=CARTESIAN_POINT('Ctrl Pts',(56.555749303194,-61.9113292073645,-217.429217603718));
#208876=CARTESIAN_POINT('Ctrl Pts',(56.5413449582148,-61.8767540479494,
-217.460938500528));
#208877=CARTESIAN_POINT('Ctrl Pts',(56.5260014871927,-61.8434724446632,
-217.492534008143));
#208878=CARTESIAN_POINT('Ctrl Pts',(56.5097077166323,-61.8115034765981,
-217.524004303589));
#208879=CARTESIAN_POINT('Ctrl Pts',(56.5015608313522,-61.7955189925656,
-217.539739451313));
#208880=CARTESIAN_POINT('Ctrl Pts',(56.4931762425887,-61.7798627597669,
-217.555443322554));
#208881=CARTESIAN_POINT('Ctrl Pts',(56.484552572944,-61.7645370401173,-217.571115950688));
#208882=CARTESIAN_POINT('Ctrl Pts',(56.4802407381216,-61.7568741802925,
-217.578952264755));
#208883=CARTESIAN_POINT('Ctrl Pts',(56.4758692047043,-61.7492938920849,
-217.586780750714));
#208884=CARTESIAN_POINT('Ctrl Pts',(56.4714378241961,-61.7417964317611,
-217.594601409107));
#208885=CARTESIAN_POINT('Ctrl Pts',(56.4688298172435,-61.7373839403005,
-217.599204112807));
#208886=CARTESIAN_POINT('Ctrl Pts',(56.4664773451866,-61.7334599236759,
-217.603321244088));
#208887=CARTESIAN_POINT('Ctrl Pts',(56.4638952029632,-61.7292104003187,
-217.607804843996));
#208888=CARTESIAN_POINT('Ctrl Pts',(56.4620899125892,-61.7262393696988,
-217.610939527935));
#208889=CARTESIAN_POINT('Ctrl Pts',(56.4601717903347,-61.7231097076094,
-217.614253458791));
#208890=CARTESIAN_POINT('Ctrl Pts',(56.4579637271793,-61.719553010382,-217.618039957184));
#208891=CARTESIAN_POINT('Ctrl Pts',(56.4578997107073,-61.7194498941248,
-217.618149735869));
#208892=CARTESIAN_POINT('Ctrl Pts',(56.4578356866977,-61.7193468013413,
-217.61825950554));
#208893=CARTESIAN_POINT('Ctrl Pts',(56.4577716551528,-61.7192437320224,
-217.618369266201));
#208894=CARTESIAN_POINT('Ctrl Pts',(56.4421392669783,-61.6940808282613,
-217.64516576577));
#208895=CARTESIAN_POINT('Ctrl Pts',(56.4259894997883,-61.6701881268128,
-217.671554538388));
#208896=CARTESIAN_POINT('Ctrl Pts',(56.4093342638972,-61.6475961080088,
-217.697509113608));
#208897=CARTESIAN_POINT('Ctrl Pts',(56.3906581150786,-61.6222628189425,
-217.726612964943));
#208898=CARTESIAN_POINT('Ctrl Pts',(56.371347168254,-61.5985638219521,-217.755171020173));
#208899=CARTESIAN_POINT('Ctrl Pts',(56.3513931964498,-61.5764978346059,
-217.783190968782));
#208900=CARTESIAN_POINT('Ctrl Pts',(56.3403344621818,-61.5642685955942,
-217.798719965661));
#208901=CARTESIAN_POINT('Ctrl Pts',(56.3290777206293,-61.5525403034329,
-217.814084430147));
#208902=CARTESIAN_POINT('Ctrl Pts',(56.317617496657,-61.5413100898162,-217.829290220593));
#208903=CARTESIAN_POINT('Ctrl Pts',(56.2843115039728,-61.5086725590434,
-217.873481673272));
#208904=CARTESIAN_POINT('Ctrl Pts',(56.2493216160993,-61.4802753388256,
-217.916287262279));
#208905=CARTESIAN_POINT('Ctrl Pts',(56.2126168425407,-61.4561551423685,
-217.957709313443));
#208906=CARTESIAN_POINT('Ctrl Pts',(56.2074534717953,-61.4527620818838,
-217.963536277798));
#208907=CARTESIAN_POINT('Ctrl Pts',(56.2022561580052,-61.4494536957759,
-217.969335844824));
#208908=CARTESIAN_POINT('Ctrl Pts',(56.1970247680347,-61.4462301002552,
-217.975108045127));
#208909=CARTESIAN_POINT('Ctrl Pts',(56.189954819578,-61.4418735804193,-217.982908870311));
#208910=CARTESIAN_POINT('Ctrl Pts',(56.1828226665242,-61.4376719457195,
-217.990659675144));
#208911=CARTESIAN_POINT('Ctrl Pts',(56.1756278034111,-61.4336259639,-217.998360366589));
#208912=CARTESIAN_POINT('Ctrl Pts',(56.1719130982625,-61.4315370249918,
-218.002336230718));
#208913=CARTESIAN_POINT('Ctrl Pts',(56.1685141252281,-61.4296717765924,
-218.005945833167));
#208914=CARTESIAN_POINT('Ctrl Pts',(56.164919310722,-61.427743320513,-218.009736234828));
#208915=CARTESIAN_POINT('Ctrl Pts',(56.1615514734821,-61.4259366275144,
-218.013287309813));
#208916=CARTESIAN_POINT('Ctrl Pts',(56.1580118462168,-61.4240742515902,
-218.0169971257));
#208917=CARTESIAN_POINT('Ctrl Pts',(56.1538562118344,-61.4219533837318,
-218.021312277383));
#208918=CARTESIAN_POINT('Ctrl Pts',(56.1535326322412,-61.4217882417833,
-218.021648277834));
#208919=CARTESIAN_POINT('Ctrl Pts',(56.1532089858838,-61.4216234325919,
-218.021984122385));
#208920=CARTESIAN_POINT('Ctrl Pts',(56.152885272635,-61.4214589557602,-218.022319811373));
#208921=CARTESIAN_POINT('Ctrl Pts',(56.1326266942832,-61.4111656891305,
-218.04332785384));
#208922=CARTESIAN_POINT('Ctrl Pts',(56.1120734784841,-61.4022192130818,
-218.063722287668));
#208923=CARTESIAN_POINT('Ctrl Pts',(56.0912527901401,-61.3945894700681,
-218.083499993318));
#208924=CARTESIAN_POINT('Ctrl Pts',(56.0770726973867,-61.3893931738732,
-218.096969754544));
#208925=CARTESIAN_POINT('Ctrl Pts',(56.0627674817464,-61.3848077257068,
-218.110154174073));
#208926=CARTESIAN_POINT('Ctrl Pts',(56.0483341812414,-61.3808286563396,
-218.123057646765));
#208927=CARTESIAN_POINT('Ctrl Pts',(56.0303519758079,-61.3758712009903,
-218.139133865552));
#208928=CARTESIAN_POINT('Ctrl Pts',(56.0121738273229,-61.3718554913409,
-218.15477159619));
#208929=CARTESIAN_POINT('Ctrl Pts',(55.9937942323692,-61.3687879496844,
-218.169970023791));
#208930=CARTESIAN_POINT('Ctrl Pts',(55.9862609286416,-61.3675306465146,
-218.176199452219));
#208931=CARTESIAN_POINT('Ctrl Pts',(55.9789241937587,-61.3664673725087,
-218.182166842088));
#208932=CARTESIAN_POINT('Ctrl Pts',(55.9715043320131,-61.3655468829179,
-218.188106246611));
#208933=CARTESIAN_POINT('Ctrl Pts',(55.9643409032318,-61.3646582057628,
-218.193840383278));
#208934=CARTESIAN_POINT('Ctrl Pts',(55.9570998422772,-61.3639025843755,
-218.199548566063));
#208935=CARTESIAN_POINT('Ctrl Pts',(55.9495121619786,-61.3632758832898,
-218.205428014337));
#208936=CARTESIAN_POINT('Ctrl Pts',(55.9457841879237,-61.3629679729278,
-218.208316700966));
#208937=CARTESIAN_POINT('Ctrl Pts',(55.9419722879021,-61.362691833393,-218.211246512342));
#208938=CARTESIAN_POINT('Ctrl Pts',(55.9380430218637,-61.3624511630172,
-218.214239363226));
#208939=CARTESIAN_POINT('Ctrl Pts',(55.9375347347342,-61.3624200300643,
-218.214626516341));
#208940=CARTESIAN_POINT('Ctrl Pts',(55.9370262986849,-61.3623896074125,
-218.215013338391));
#208941=CARTESIAN_POINT('Ctrl Pts',(55.9365177134434,-61.3623598955499,
-218.21539982926));
#208942=CARTESIAN_POINT('Ctrl Pts',(55.9168041387,-61.3612082163902,-218.230380831454));
#208943=CARTESIAN_POINT('Ctrl Pts',(55.8970064047387,-61.3611339147912,
-218.244756879731));
#208944=CARTESIAN_POINT('Ctrl Pts',(55.8771158279607,-61.3621037947684,
-218.258552765903));
#208945=CARTESIAN_POINT('Ctrl Pts',(55.8615464471865,-61.3628629698712,
-218.26935151786));
#208946=CARTESIAN_POINT('Ctrl Pts',(55.8459239121599,-61.3642624475839,
-218.27979178035));
#208947=CARTESIAN_POINT('Ctrl Pts',(55.8302484900842,-61.366294962689,-218.289876937764));
#208948=CARTESIAN_POINT('Ctrl Pts',(55.8257068705157,-61.3668838406363,
-218.292798897252));
#208949=CARTESIAN_POINT('Ctrl Pts',(55.8211607962849,-61.3675259035511,
-218.29569103093));
#208950=CARTESIAN_POINT('Ctrl Pts',(55.8166102389797,-61.3682210877797,
-218.298553376832));
#208951=CARTESIAN_POINT('Ctrl Pts',(55.8128092045475,-61.3688017681255,
-218.300944265376));
#208952=CARTESIAN_POINT('Ctrl Pts',(55.8089983934449,-61.3694205155333,
-218.303318560299));
#208953=CARTESIAN_POINT('Ctrl Pts',(55.8051757780505,-61.3700780867166,
-218.30567724614));
#208954=CARTESIAN_POINT('Ctrl Pts',(55.7983202521378,-61.3712573830416,
-218.309907342614));
#208955=CARTESIAN_POINT('Ctrl Pts',(55.7914313802385,-61.3725609532495,
-218.314084260537));
#208956=CARTESIAN_POINT('Ctrl Pts',(55.7845238850248,-61.3739877414227,
-218.318197921959));
#208957=CARTESIAN_POINT('Ctrl Pts',(55.7688812052958,-61.3772188389109,
-218.327513699409));
#208958=CARTESIAN_POINT('Ctrl Pts',(55.7531422004866,-61.3810931503088,
-218.336498652793));
#208959=CARTESIAN_POINT('Ctrl Pts',(55.7374922209247,-61.3855480998269,
-218.345056637219));
#208960=CARTESIAN_POINT('Ctrl Pts',(55.7335797260343,-61.3866618372065,
-218.347196133325));
#208961=CARTESIAN_POINT('Ctrl Pts',(55.7296728414405,-61.3878108496662,
-218.349309539776));
#208962=CARTESIAN_POINT('Ctrl Pts',(55.7257744241213,-61.3889940773438,
-218.351395437214));
#208963=CARTESIAN_POINT('Ctrl Pts',(55.7140791721637,-61.3925437603767,
-218.357653129527));
#208964=CARTESIAN_POINT('Ctrl Pts',(55.7024601151168,-61.396401379636,-218.3636632402));
#208965=CARTESIAN_POINT('Ctrl Pts',(55.6909944590457,-61.4005387214182,
-218.369387227857));
#208966=CARTESIAN_POINT('Ctrl Pts',(55.6904721203629,-61.4007272055,-218.369647994459));
#208967=CARTESIAN_POINT('Ctrl Pts',(55.6899496363347,-61.400916414908,-218.369908412714));
#208968=CARTESIAN_POINT('Ctrl Pts',(55.6894270067505,-61.4011063509032,
-218.370168481955));
#208969=CARTESIAN_POINT('Ctrl Pts',(55.6619133365653,-61.4111054716716,
-218.383859745449));
#208970=CARTESIAN_POINT('Ctrl Pts',(55.6344763347929,-61.4229456905876,
-218.396340222171));
#208971=CARTESIAN_POINT('Ctrl Pts',(55.6070891104916,-61.4365888112143,
-218.407649991647));
#208972=CARTESIAN_POINT('Ctrl Pts',(55.5943945396522,-61.4429126927205,
-218.412892314425));
#208973=CARTESIAN_POINT('Ctrl Pts',(55.5817109693076,-61.4496244068266,
-218.417882581383));
#208974=CARTESIAN_POINT('Ctrl Pts',(55.5690375149754,-61.456722141651,-218.422622187911));
#208975=CARTESIAN_POINT('Ctrl Pts',(55.5487702728249,-61.4680727574056,
-218.430201712062));
#208976=CARTESIAN_POINT('Ctrl Pts',(55.5285322537927,-61.4804082518478,
-218.437139243937));
#208977=CARTESIAN_POINT('Ctrl Pts',(55.5083252248452,-61.4937253997328,
-218.443433751089));
#208978=CARTESIAN_POINT('Ctrl Pts',(55.5005249296046,-61.498866070612,-218.445863549864));
#208979=CARTESIAN_POINT('Ctrl Pts',(55.4924700861797,-61.5043278139308,
-218.448275734037));
#208980=CARTESIAN_POINT('Ctrl Pts',(55.4844646831107,-61.5099172845121,
-218.450571066518));
#208981=CARTESIAN_POINT('Ctrl Pts',(55.4761777049345,-61.5157033542859,
-218.452947133034));
#208982=CARTESIAN_POINT('Ctrl Pts',(55.4679439040137,-61.5216261860161,
-218.455197900852));
#208983=CARTESIAN_POINT('Ctrl Pts',(55.460084220559,-61.5274306880095,-218.457250847136));
#208984=CARTESIAN_POINT('Ctrl Pts',(55.4558674763759,-61.5305448210606,
-218.458352259089));
#208985=CARTESIAN_POINT('Ctrl Pts',(55.4517581179666,-61.5336242111068,
-218.45939738176));
#208986=CARTESIAN_POINT('Ctrl Pts',(55.447803718,-61.5366253992586,-218.46037904842));
#208987=CARTESIAN_POINT('Ctrl Pts',(55.4234882934493,-61.555079567953,-218.466415271821));
#208988=CARTESIAN_POINT('Ctrl Pts',(55.3994642092221,-61.5747880095429,
-218.471443614322));
#208989=CARTESIAN_POINT('Ctrl Pts',(55.3756994679743,-61.5957362573536,
-218.475492346442));
#208990=CARTESIAN_POINT('Ctrl Pts',(55.3515266265266,-61.6170442391092,
-218.479610605446));
#208991=CARTESIAN_POINT('Ctrl Pts',(55.3276213481284,-61.6396363978418,
-218.482715013696));
#208992=CARTESIAN_POINT('Ctrl Pts',(55.3039893611285,-61.6635080810643,
-218.48479891848));
#208993=CARTESIAN_POINT('Ctrl Pts',(55.2819264708097,-61.6857947524588,
-218.486744457917));
#208994=CARTESIAN_POINT('Ctrl Pts',(55.2601016111223,-61.7091979209098,
-218.487799869925));
#208995=CARTESIAN_POINT('Ctrl Pts',(55.2385592394913,-61.7337037475461,
-218.487935855327));
#208996=CARTESIAN_POINT('Ctrl Pts',(55.23702716172,-61.7354465840777,-218.487945526509));
#208997=CARTESIAN_POINT('Ctrl Pts',(55.2354965312477,-61.737194988746,-218.487950538905));
#208998=CARTESIAN_POINT('Ctrl Pts',(55.2339673727997,-61.7389489519143,
-218.487950878257));
#208999=CARTESIAN_POINT('Ctrl Pts',(48.9443109379934,-69.7210624363875,
-217.233400031701));
#209000=CARTESIAN_POINT('Ctrl Pts',(49.0991171386076,-69.4468461963775,
-217.336253844649));
#209001=CARTESIAN_POINT('Ctrl Pts',(49.2925903552098,-69.4989817480832,
-217.60005));
#209002=CARTESIAN_POINT('Ctrl Pts',(49.130620489061,-69.7720396651474,-217.086285690494));
#209003=CARTESIAN_POINT('Ctrl Pts',(49.2856293770243,-69.4971059616069,
-217.188797196021));
#209004=CARTESIAN_POINT('Ctrl Pts',(49.479508186842,-69.5493508092223,-217.453006109745));
#209005=CARTESIAN_POINT('Ctrl Pts',(49.3167847015304,-69.8229858522605,
-216.938985563531));
#209006=CARTESIAN_POINT('Ctrl Pts',(49.4718979894171,-69.5473000765824,
-217.041226996676));
#209007=CARTESIAN_POINT('Ctrl Pts',(49.6662875276291,-69.5996825510014,
-217.305773775928));
#209008=CARTESIAN_POINT('Ctrl Pts',(49.502798597092,-69.8738997057058,-216.791493525167));
#209009=CARTESIAN_POINT('Ctrl Pts',(49.6579114178628,-69.5974254266744,
-216.893543128263));
#209010=CARTESIAN_POINT('Ctrl Pts',(49.8529236261983,-69.6499756930601,
-217.158346534073));
#209011=CARTESIAN_POINT('',(49.8529236261983,-69.6499756930601,-217.158346534073));
#209012=CARTESIAN_POINT('',(49.5029673643273,-69.8740806799455,-216.790758026401));
#209013=CARTESIAN_POINT('Origin',(49.7228284492359,-70.13275436381,-217.158346534073));
#209014=CARTESIAN_POINT('Origin',(-167.970418940429,-23.6135530814242,73.4534718919959));
#209015=CARTESIAN_POINT('Origin',(-165.63543440526,-11.5819668880935,75.4526175248521));
#209016=CARTESIAN_POINT('Ctrl Pts',(56.7788252534563,-62.6825329319095,
-216.79113809033));
#209017=CARTESIAN_POINT('Ctrl Pts',(56.5025836743465,-62.8382452661243,
-216.892152466627));
#209018=CARTESIAN_POINT('Ctrl Pts',(56.5555093174817,-63.0368943169927,
-217.153871927429));
#209019=CARTESIAN_POINT('Ctrl Pts',(56.7295803718938,-62.4998572980931,
-216.940045714159));
#209020=CARTESIAN_POINT('Ctrl Pts',(56.4539126170321,-62.6555652121921,
-217.041204177849));
#209021=CARTESIAN_POINT('Ctrl Pts',(56.5067115045409,-62.8537385034605,
-217.302758005793));
#209022=CARTESIAN_POINT('Ctrl Pts',(56.680302877991,-62.3170582944071,-217.088794981881));
#209023=CARTESIAN_POINT('Ctrl Pts',(56.4051889499832,-62.4726876949562,
-217.190156301151));
#209024=CARTESIAN_POINT('Ctrl Pts',(56.4578811804683,-62.6704606639105,
-217.451483035533));
#209025=CARTESIAN_POINT('Ctrl Pts',(56.6309943627598,-62.1341374253209,
-217.237388612086));
#209026=CARTESIAN_POINT('Ctrl Pts',(56.3564132949791,-62.2896150482124,
-217.339009989763));
#209027=CARTESIAN_POINT('Ctrl Pts',(56.4090189474476,-62.4870630585555,
-217.60005));
#209028=CARTESIAN_POINT('',(56.7789323645482,-62.6826309921534,-216.790388211429));
#209029=CARTESIAN_POINT('',(56.5555093174817,-63.0368943169928,-217.153871927429));
#209030=CARTESIAN_POINT('Origin',(57.0386554992377,-62.9081707097771,-217.153871927429));
#209031=CARTESIAN_POINT('Origin',(-11.7909588194732,193.492081547376,120.824020637011));
#209032=CARTESIAN_POINT('Origin',(-10.1481943050527,195.398995247496,121.950798030302));
#209033=CARTESIAN_POINT('Ctrl Pts',(49.502798597092,-69.8738997057057,-216.791493525167));
#209034=CARTESIAN_POINT('Ctrl Pts',(49.6579114178629,-69.5974254266743,
-216.893543128263));
#209035=CARTESIAN_POINT('Ctrl Pts',(49.8529236261983,-69.6499756930601,
-217.158346534073));
#209036=CARTESIAN_POINT('Ctrl Pts',(49.8904699761689,-69.961109459285,-216.497441344741));
#209037=CARTESIAN_POINT('Ctrl Pts',(50.0485994592274,-69.7027047875172,
-216.601129210477));
#209038=CARTESIAN_POINT('Ctrl Pts',(50.2627282054337,-69.7604064193654,
-216.834634459542));
#209039=CARTESIAN_POINT('Ctrl Pts',(50.234208458361,-70.0386649773616,-216.158971875201));
#209040=CARTESIAN_POINT('Ctrl Pts',(50.4024671800086,-69.798062114882,-216.256560731386));
#209041=CARTESIAN_POINT('Ctrl Pts',(50.6264190422318,-69.8584107982651,
-216.462106475915));
#209042=CARTESIAN_POINT('Ctrl Pts',(50.5261810352842,-70.1046957156775,
-215.770277860521));
#209043=CARTESIAN_POINT('Ctrl Pts',(50.704122433655,-69.8793496612891,-215.854989245265));
#209044=CARTESIAN_POINT('Ctrl Pts',(50.9355365677156,-69.9417092155658,
-216.034373717099));
#209045=CARTESIAN_POINT('',(50.9355365677156,-69.9417092155658,-216.034373717099));
#209046=CARTESIAN_POINT('',(50.5260891840881,-70.1045902648202,-215.770190216137));
#209047=CARTESIAN_POINT('Origin',(50.8054413907531,-70.4244878863158,-216.034373717099));
#209048=CARTESIAN_POINT('Ctrl Pts',(49.503005485031,-69.8741215579355,-216.790591893854));
#209049=CARTESIAN_POINT('Ctrl Pts',(49.5036598824408,-69.8736705791977,
-216.790517784408));
#209050=CARTESIAN_POINT('Ctrl Pts',(49.507504324357,-69.8740966385711,-216.787917197217));
#209051=CARTESIAN_POINT('Ctrl Pts',(49.5145301680683,-69.8753873628897,
-216.7827677998));
#209052=CARTESIAN_POINT('Ctrl Pts',(49.5215382096988,-69.8766748167714,
-216.777631449924));
#209053=CARTESIAN_POINT('Ctrl Pts',(49.5317116207978,-69.8788226274945,
-216.769959125464));
#209054=CARTESIAN_POINT('Ctrl Pts',(49.5450246500239,-69.8817948135687,
-216.759685963983));
#209055=CARTESIAN_POINT('Ctrl Pts',(49.5540742065074,-69.8838151626043,
-216.752702763277));
#209056=CARTESIAN_POINT('Ctrl Pts',(49.5645741163918,-69.8862159430578,
-216.744516923557));
#209057=CARTESIAN_POINT('Ctrl Pts',(49.5765113792548,-69.888979213311,-216.735097065284));
#209058=CARTESIAN_POINT('Ctrl Pts',(49.5939391216258,-69.8930134347759,
-216.721344594134));
#209059=CARTESIAN_POINT('Ctrl Pts',(49.6144315139314,-69.8978215885242,
-216.704963518013));
#209060=CARTESIAN_POINT('Ctrl Pts',(49.6379310279013,-69.9033253866201,
-216.685823358771));
#209061=CARTESIAN_POINT('Ctrl Pts',(49.6461891503198,-69.9052595133642,
-216.679097186548));
#209062=CARTESIAN_POINT('Ctrl Pts',(49.6548184385922,-69.907279295187,-216.672029942124));
#209063=CARTESIAN_POINT('Ctrl Pts',(49.6638157326524,-69.9093804828061,
-216.664614872801));
#209064=CARTESIAN_POINT('Ctrl Pts',(49.6811158390666,-69.9134206719079,
-216.650357087349));
#209065=CARTESIAN_POINT('Ctrl Pts',(49.699776875429,-69.9177622530644,-216.634813749881));
#209066=CARTESIAN_POINT('Ctrl Pts',(49.7197723867992,-69.9223700050012,
-216.617931309463));
#209067=CARTESIAN_POINT('Ctrl Pts',(49.7297701424842,-69.9246738809696,
-216.609490089255));
#209068=CARTESIAN_POINT('Ctrl Pts',(49.7401014354786,-69.9270442043552,
-216.600713971417));
#209069=CARTESIAN_POINT('Ctrl Pts',(49.750762420894,-69.9294759003914,-216.59159562903));
#209070=CARTESIAN_POINT('Ctrl Pts',(49.7560929136017,-69.9306917484095,
-216.587036457837));
#209071=CARTESIAN_POINT('Ctrl Pts',(49.7615058242863,-69.9319229335857,
-216.582391722711));
#209072=CARTESIAN_POINT('Ctrl Pts',(49.7670006367179,-69.9331687794098,
-216.577660468699));
#209073=CARTESIAN_POINT('Ctrl Pts',(49.7697480429336,-69.9337917023218,
-216.575294841692));
#209074=CARTESIAN_POINT('Ctrl Pts',(49.772515924257,-69.9344182900113,-216.572907584482));
#209075=CARTESIAN_POINT('Ctrl Pts',(49.7753042138934,-69.9350484551439,
-216.570498575359));
#209076=CARTESIAN_POINT('Ctrl Pts',(49.7780925035297,-69.9356786202765,
-216.568089566236));
#209077=CARTESIAN_POINT('Ctrl Pts',(49.7822817015456,-69.9366233157115,
-216.564461979738));
#209078=CARTESIAN_POINT('Ctrl Pts',(49.7837302395077,-69.9369495938251,
-216.563206168813));
#209079=CARTESIAN_POINT('Ctrl Pts',(49.8300834542953,-69.9473904934593,
-216.523020219228));
#209080=CARTESIAN_POINT('Ctrl Pts',(49.8753773599085,-69.9575976012502,
-216.482374323618));
#209081=CARTESIAN_POINT('Ctrl Pts',(49.9195996591217,-69.9675665793152,
-216.441323275821));
#209082=CARTESIAN_POINT('Ctrl Pts',(49.9417108087283,-69.9725510683477,
-216.420797751923));
#209083=CARTESIAN_POINT('Ctrl Pts',(49.9635540819862,-69.9774760543192,
-216.400170973799));
#209084=CARTESIAN_POINT('Ctrl Pts',(49.9851282539123,-69.98234128434,-216.379449755809));
#209085=CARTESIAN_POINT('Ctrl Pts',(49.9994083221236,-69.9855616080122,
-216.365734262703));
#209086=CARTESIAN_POINT('Ctrl Pts',(50.0131165140574,-69.9886508257923,
-216.352422200884));
#209087=CARTESIAN_POINT('Ctrl Pts',(50.0271549209438,-69.9918184673918,
-216.33863391884));
#209088=CARTESIAN_POINT('Ctrl Pts',(50.0343255866789,-69.9934364643101,
-216.331591014157));
#209089=CARTESIAN_POINT('Ctrl Pts',(50.0415820727045,-69.9950744894472,
-216.324423275089));
#209090=CARTESIAN_POINT('Ctrl Pts',(50.0490423476813,-69.99675757341,-216.317009695042));
#209091=CARTESIAN_POINT('Ctrl Pts',(50.1373050109276,-70.0166701736136,
-216.229299480458));
#209092=CARTESIAN_POINT('Ctrl Pts',(50.221254127075,-70.0356392133376,-216.139590511556));
#209093=CARTESIAN_POINT('Ctrl Pts',(50.3007842172754,-70.0536146832101,
-216.048306803414));
#209094=CARTESIAN_POINT('Ctrl Pts',(50.3803143074759,-70.0715901530826,
-215.957023095271));
#209095=CARTESIAN_POINT('Ctrl Pts',(50.4554254383405,-70.0885721436241,
-215.864165404149));
#209096=CARTESIAN_POINT('Ctrl Pts',(50.5260568509089,-70.1045534073734,
-215.770160360609));
#209097=CARTESIAN_POINT('Ctrl Pts',(50.9355365677156,-69.9417092155658,
-216.034373717099));
#209098=CARTESIAN_POINT('Ctrl Pts',(50.8116343558521,-69.9083210790241,
-216.205819948822));
#209099=CARTESIAN_POINT('Ctrl Pts',(50.679045627584,-69.8725921723587,-216.368291840782));
#209100=CARTESIAN_POINT('Ctrl Pts',(50.5382668565233,-69.8346562811454,
-216.522302092548));
#209101=CARTESIAN_POINT('Ctrl Pts',(50.3916404967015,-69.7951446303951,
-216.682709534817));
#209102=CARTESIAN_POINT('Ctrl Pts',(50.2361294127338,-69.7532387981491,
-216.833937733262));
#209103=CARTESIAN_POINT('Ctrl Pts',(50.0722553986623,-69.7090793931218,
-216.976525935758));
#209104=CARTESIAN_POINT('Ctrl Pts',(50.0007248884674,-69.6898039467406,
-217.03876525375));
#209105=CARTESIAN_POINT('Ctrl Pts',(49.9276005183839,-69.6700990002659,
-217.099357901494));
#209106=CARTESIAN_POINT('Ctrl Pts',(49.8529236261983,-69.6499756930601,
-217.158346534073));
#209107=CARTESIAN_POINT('Ctrl Pts',(56.9946437140725,-63.654341638523,-215.806005173342));
#209108=CARTESIAN_POINT('Ctrl Pts',(56.7673159108321,-63.8318809481279,
-215.890327243741));
#209109=CARTESIAN_POINT('Ctrl Pts',(56.8293274051384,-64.0646324794683,
-216.070020447202));
#209110=CARTESIAN_POINT('Ctrl Pts',(56.932619322676,-63.3755293978699,-216.178019997802));
#209111=CARTESIAN_POINT('Ctrl Pts',(56.6905874263868,-63.5438912383415,
-216.274438039323));
#209112=CARTESIAN_POINT('Ctrl Pts',(56.7507244929534,-63.769607365439,-216.47928372567));
#209113=CARTESIAN_POINT('Ctrl Pts',(56.860146560067,-63.0493377881462,-216.504716595751));
#209114=CARTESIAN_POINT('Ctrl Pts',(56.6011588045338,-63.2082333266141,
-216.606979895655));
#209115=CARTESIAN_POINT('Ctrl Pts',(56.6588023342389,-63.4245903094199,
-216.83871657078));
#209116=CARTESIAN_POINT('Ctrl Pts',(56.7788252534563,-62.6825329319096,
-216.79113809033));
#209117=CARTESIAN_POINT('Ctrl Pts',(56.5025836743465,-62.8382452661242,
-216.892152466627));
#209118=CARTESIAN_POINT('Ctrl Pts',(56.5555093174817,-63.0368943169927,
-217.153871927429));
#209119=CARTESIAN_POINT('',(56.9945465422419,-63.6542557031434,-215.80592400831));
#209120=CARTESIAN_POINT('',(56.8293274051384,-64.0646324794683,-216.070020447202));
#209121=CARTESIAN_POINT('Origin',(57.3124735868944,-63.9359088722526,-216.070020447202));
#209122=CARTESIAN_POINT('Ctrl Pts',(56.5555093174817,-63.0368943169928,
-217.153871927428));
#209123=CARTESIAN_POINT('Ctrl Pts',(56.6017653589551,-63.2105099443389,
-217.012740999606));
#209124=CARTESIAN_POINT('Ctrl Pts',(56.6457145720425,-63.3754672117248,
-216.862817131852));
#209125=CARTESIAN_POINT('Ctrl Pts',(56.6872100613026,-63.5312147675134,
-216.70354056544));
#209126=CARTESIAN_POINT('Ctrl Pts',(56.7270307212971,-63.6806760842641,
-216.550692675001));
#209127=CARTESIAN_POINT('Ctrl Pts',(56.7645917777123,-63.8216562928075,
-216.389231897198));
#209128=CARTESIAN_POINT('Ctrl Pts',(56.7997545451807,-63.953634856878,-216.218629552566));
#209129=CARTESIAN_POINT('Ctrl Pts',(56.8098094620337,-63.9913745907972,
-216.169845212944));
#209130=CARTESIAN_POINT('Ctrl Pts',(56.8196682125205,-64.0283780415051,
-216.120313149194));
#209131=CARTESIAN_POINT('Ctrl Pts',(56.8293274051384,-64.0646324794683,
-216.070020447202));
#209132=CARTESIAN_POINT('Ctrl Pts',(56.9944699555807,-63.6541878226818,
-215.805860862997));
#209133=CARTESIAN_POINT('Ctrl Pts',(56.9794459967772,-63.5866902802209,
-215.895894129132));
#209134=CARTESIAN_POINT('Ctrl Pts',(56.9635084836788,-63.5150703368537,
-215.984953436998));
#209135=CARTESIAN_POINT('Ctrl Pts',(56.9466685708699,-63.4393805477762,
-216.072641385784));
#209136=CARTESIAN_POINT('Ctrl Pts',(56.9382486144655,-63.4015356532375,
-216.116485360177));
#209137=CARTESIAN_POINT('Ctrl Pts',(56.9296030730276,-63.3626733585993,
-216.159987654482));
#209138=CARTESIAN_POINT('Ctrl Pts',(56.9207359629282,-63.3228030795314,
-216.20310039353));
#209139=CARTESIAN_POINT('Ctrl Pts',(56.9163024078785,-63.3028679399975,
-216.224656763054));
#209140=CARTESIAN_POINT('Ctrl Pts',(56.91181348634,-63.2826808269247,-216.246115770319));
#209141=CARTESIAN_POINT('Ctrl Pts',(56.9072699345539,-63.2622431718491,
-216.267471425441));
#209142=CARTESIAN_POINT('Ctrl Pts',(56.9042193408906,-63.2485210918547,
-216.281809861373));
#209143=CARTESIAN_POINT('Ctrl Pts',(56.9010480846113,-63.2342431449902,
-216.296555148204));
#209144=CARTESIAN_POINT('Ctrl Pts',(56.897948704089,-63.2203010182936,-216.310790655394));
#209145=CARTESIAN_POINT('Ctrl Pts',(56.8964318697161,-63.2134777525306,
-216.317757501337));
#209146=CARTESIAN_POINT('Ctrl Pts',(56.8949327040015,-63.2067352855026,
-216.324602831575));
#209147=CARTESIAN_POINT('Ctrl Pts',(56.8934762334649,-63.2001801107107,
-216.331222459184));
#209148=CARTESIAN_POINT('Ctrl Pts',(56.8846112168146,-63.1602810999074,
-216.371513771297));
#209149=CARTESIAN_POINT('Ctrl Pts',(56.8755237821599,-63.1193619943915,
-216.411526369275));
#209150=CARTESIAN_POINT('Ctrl Pts',(56.8662137807326,-63.077429139806,-216.45120864926));
#209151=CARTESIAN_POINT('Ctrl Pts',(56.861558780019,-63.0564627125132,-216.471049789252));
#209152=CARTESIAN_POINT('Ctrl Pts',(56.8568481595931,-63.0352428671797,
-216.490808375499));
#209153=CARTESIAN_POINT('Ctrl Pts',(56.8520821602383,-63.0137706793198,
-216.510477896976));
#209154=CARTESIAN_POINT('Ctrl Pts',(56.8496991605609,-63.0030345853899,
-216.520312657714));
#209155=CARTESIAN_POINT('Ctrl Pts',(56.8473023177016,-62.9922354071859,
-216.530125154026));
#209156=CARTESIAN_POINT('Ctrl Pts',(56.8448916738711,-62.9813732913107,
-216.539914577476));
#209157=CARTESIAN_POINT('Ctrl Pts',(56.8436863519558,-62.9759422333731,
-216.5448092892));
#209158=CARTESIAN_POINT('Ctrl Pts',(56.8424775798923,-62.9704954411003,
-216.549698232825));
#209159=CARTESIAN_POINT('Ctrl Pts',(56.8412653639348,-62.9650329338615,
-216.55458130727));
#209160=CARTESIAN_POINT('Ctrl Pts',(56.8403562019666,-62.9609360534324,
-216.558243613104));
#209161=CARTESIAN_POINT('Ctrl Pts',(56.839445102816,-62.9568303333417,-216.561902617535));
#209162=CARTESIAN_POINT('Ctrl Pts',(56.8385320693501,-62.9527157820021,
-216.56555827794));
#209163=CARTESIAN_POINT('Ctrl Pts',(56.8382277248615,-62.9513442648889,
-216.566776831409));
#209164=CARTESIAN_POINT('Ctrl Pts',(56.8382152206193,-62.9512879268144,
-216.566828027));
#209165=CARTESIAN_POINT('Ctrl Pts',(56.8376183912324,-62.94859828724,-216.569212822087));
#209166=CARTESIAN_POINT('Ctrl Pts',(56.8305025760161,-62.9165305328181,
-216.597646008419));
#209167=CARTESIAN_POINT('Ctrl Pts',(56.8238616028387,-62.8872265401915,
-216.623070944351));
#209168=CARTESIAN_POINT('Ctrl Pts',(56.8178173128131,-62.8607818805868,
-216.645667973915));
#209169=CARTESIAN_POINT('Ctrl Pts',(56.8117204483761,-62.8341072001847,
-216.668461556843));
#209170=CARTESIAN_POINT('Ctrl Pts',(56.8062304512243,-62.8103415608514,
-216.688378132289));
#209171=CARTESIAN_POINT('Ctrl Pts',(56.8014409140339,-62.7895571321941,
-216.705568966566));
#209172=CARTESIAN_POINT('Ctrl Pts',(56.7966107261207,-62.7685962977551,
-216.722905706347));
#209173=CARTESIAN_POINT('Ctrl Pts',(56.7924927406286,-62.750667289575,-216.737470473255));
#209174=CARTESIAN_POINT('Ctrl Pts',(56.7891544483765,-62.7358213501912,
-216.749380072365));
#209175=CARTESIAN_POINT('Ctrl Pts',(56.7858060768922,-62.7209305867902,
-216.761325629864));
#209176=CARTESIAN_POINT('Ctrl Pts',(56.7832419532595,-62.709141376279,-216.770600095729));
#209177=CARTESIAN_POINT('Ctrl Pts',(56.7815043823577,-62.7004854065422,
-216.777280214984));
#209178=CARTESIAN_POINT('Ctrl Pts',(56.7797629254889,-62.6918100782785,
-216.783975273901));
#209179=CARTESIAN_POINT('Ctrl Pts',(56.7788516311555,-62.6862819290349,
-216.788064444018));
#209180=CARTESIAN_POINT('Ctrl Pts',(56.7787891208614,-62.6839146946666,
-216.789582191217));
#209181=CARTESIAN_POINT('Ctrl Pts',(56.7787708428251,-62.6832225143423,
-216.790025981136));
#209182=CARTESIAN_POINT('Ctrl Pts',(56.7788249825049,-62.6828004720904,
-216.79024963763));
#209183=CARTESIAN_POINT('Ctrl Pts',(56.7789516318532,-62.6826486313781,
-216.79025332208));
#209184=CARTESIAN_POINT('Ctrl Pts',(51.9620199839905,-69.8524482833038,
-212.903250403248));
#209185=CARTESIAN_POINT('Ctrl Pts',(51.8928715700308,-69.8849735800753,
-212.914037308895));
#209186=CARTESIAN_POINT('Ctrl Pts',(51.8371967923162,-69.9365578441711,
-212.924798774573));
#209187=CARTESIAN_POINT('Ctrl Pts',(52.0023737441193,-69.8310690362166,
-213.304505435696));
#209188=CARTESIAN_POINT('Ctrl Pts',(51.941700685795,-69.8615494218525,-213.296380663458));
#209189=CARTESIAN_POINT('Ctrl Pts',(51.8900804694045,-69.9070006930946,
-213.289619354923));
#209190=CARTESIAN_POINT('Ctrl Pts',(51.9342823138335,-69.8685686407292,
-213.657783042067));
#209191=CARTESIAN_POINT('Ctrl Pts',(51.8593850051349,-69.9028934810734,
-213.636762861553));
#209192=CARTESIAN_POINT('Ctrl Pts',(51.8014625992089,-69.9580400304186,
-213.610486438733));
#209193=CARTESIAN_POINT('Ctrl Pts',(51.7621689112058,-69.9305269210584,
-214.242088767328));
#209194=CARTESIAN_POINT('Ctrl Pts',(51.6558225747516,-69.9634677621137,
-214.190398126914));
#209195=CARTESIAN_POINT('Ctrl Pts',(51.5789777052583,-70.0457813460658,
-214.141301452941));
#209196=CARTESIAN_POINT('Ctrl Pts',(51.6732637051828,-69.9557792147167,
-214.478511967556));
#209197=CARTESIAN_POINT('Ctrl Pts',(51.5497057881375,-69.985967309418,-214.415265918991));
#209198=CARTESIAN_POINT('Ctrl Pts',(51.4643785947433,-70.0826136343188,
-214.356059518454));
#209199=CARTESIAN_POINT('Ctrl Pts',(51.3492289962179,-70.0110328842746,
-215.2590218875));
#209200=CARTESIAN_POINT('Ctrl Pts',(51.1618526758825,-70.0201965830603,
-215.162496083505));
#209201=CARTESIAN_POINT('Ctrl Pts',(51.0486202117362,-70.1704592965568,
-215.065022277779));
#209202=CARTESIAN_POINT('Ctrl Pts',(51.0782728947073,-70.0027462486926,
-215.78151451348));
#209203=CARTESIAN_POINT('Ctrl Pts',(50.8352661021995,-69.9666501783504,
-215.659256381595));
#209204=CARTESIAN_POINT('Ctrl Pts',(50.7036055976657,-70.1752051070453,
-215.539933768453));
#209205=CARTESIAN_POINT('Ctrl Pts',(50.79511229761,-69.8965255868172,-216.289741858889));
#209206=CARTESIAN_POINT('Ctrl Pts',(50.5508501997346,-69.8033231077245,
-216.081892433387));
#209207=CARTESIAN_POINT('Ctrl Pts',(50.3485321404655,-70.0571221488448,
-216.001649432013));
#209208=CARTESIAN_POINT('',(51.9718267086745,-69.8471376007524,-213.236262748316));
#209209=CARTESIAN_POINT('',(51.8506357968709,-69.9286975784453,-213.227536544931));
#209210=CARTESIAN_POINT('Origin',(52.1871615786983,-70.2983923998978,-213.236262748316));
#209211=CARTESIAN_POINT('Ctrl Pts',(50.526181157749,-70.1046957431703,-215.770277696984));
#209212=CARTESIAN_POINT('Ctrl Pts',(50.5900491822617,-70.1190337938543,
-215.684989847738));
#209213=CARTESIAN_POINT('Ctrl Pts',(50.6579835771245,-70.130651334725,-215.593317406618));
#209214=CARTESIAN_POINT('Ctrl Pts',(50.7646990473915,-70.1424896494519,
-215.44560740904));
#209215=CARTESIAN_POINT('Ctrl Pts',(50.8192571781922,-70.1470086832376,
-215.36920511009));
#209216=CARTESIAN_POINT('Ctrl Pts',(50.8847365884144,-70.149516553765,-215.275553310463));
#209217=CARTESIAN_POINT('Ctrl Pts',(50.9178970323605,-70.1500380291522,
-215.227594876075));
#209218=CARTESIAN_POINT('Ctrl Pts',(50.9357693297152,-70.1501156065902,
-215.201599164668));
#209219=CARTESIAN_POINT('Ctrl Pts',(50.9441383948169,-70.1500961107514,
-215.189385131094));
#209220=CARTESIAN_POINT('Ctrl Pts',(50.9489276109694,-70.1500711879545,
-215.182385426043));
#209221=CARTESIAN_POINT('Ctrl Pts',(50.9507973949068,-70.150059025442,-215.179650830219));
#209222=CARTESIAN_POINT('Ctrl Pts',(50.9850227491289,-70.1498153761691,
-215.129579963741));
#209223=CARTESIAN_POINT('Ctrl Pts',(51.0361537920302,-70.1483467098581,
-215.05498416666));
#209224=CARTESIAN_POINT('Ctrl Pts',(51.1351942660711,-70.1398574995953,
-214.903171554453));
#209225=CARTESIAN_POINT('Ctrl Pts',(51.1719033536906,-70.135947513949,-214.84590539025));
#209226=CARTESIAN_POINT('Ctrl Pts',(51.2317676039139,-70.1276087918756,
-214.749763328443));
#209227=CARTESIAN_POINT('Ctrl Pts',(51.2628970020121,-70.1228178480742,
-214.699132199145));
#209228=CARTESIAN_POINT('Ctrl Pts',(51.3011167631323,-70.1159211083316,
-214.635539753149));
#209229=CARTESIAN_POINT('Ctrl Pts',(51.3178816154838,-70.1126596506502,
-214.607313326825));
#209230=CARTESIAN_POINT('Ctrl Pts',(51.3291411614471,-70.1104145156853,
-214.588279274963));
#209231=CARTESIAN_POINT('Ctrl Pts',(51.3354355945575,-70.1091261688492,
-214.577592011259));
#209232=CARTESIAN_POINT('Ctrl Pts',(51.4219363715995,-70.0910297574046,
-214.430175036717));
#209233=CARTESIAN_POINT('Ctrl Pts',(51.4883839419626,-70.0723789788218,
-214.306593959656));
#209234=CARTESIAN_POINT('Ctrl Pts',(51.569496385825,-70.0464887061108,-214.145707845131));
#209235=CARTESIAN_POINT('Ctrl Pts',(51.5934318573064,-70.038194487785,-214.096142505444));
#209236=CARTESIAN_POINT('Ctrl Pts',(51.6250789004642,-70.0267088171666,
-214.027984609541));
#209237=CARTESIAN_POINT('Ctrl Pts',(51.6398373799156,-70.0212036779678,
-213.995452202307));
#209238=CARTESIAN_POINT('Ctrl Pts',(51.6552677865945,-70.0152828821744,
-213.960216179522));
#209239=CARTESIAN_POINT('Ctrl Pts',(51.6625447127538,-70.012457719356,-213.943278765729));
#209240=CARTESIAN_POINT('Ctrl Pts',(51.6655703886093,-70.0112769379038,
-213.936165814877));
#209241=CARTESIAN_POINT('Ctrl Pts',(51.667566936517,-70.0104965286416,-213.931456288653));
#209242=CARTESIAN_POINT('Ctrl Pts',(51.6678426662331,-70.0103889860098,
-213.930809474077));
#209243=CARTESIAN_POINT('Ctrl Pts',(51.7236131045389,-69.9885217372769,
-213.798345974757));
#209244=CARTESIAN_POINT('Ctrl Pts',(51.7641862310625,-69.9702533041814,
-213.680412346262));
#209245=CARTESIAN_POINT('Ctrl Pts',(51.8000752575117,-69.9534191577125,
-213.546566643314));
#209246=CARTESIAN_POINT('Ctrl Pts',(51.8065101620132,-69.9503504498528,
-213.520473763259));
#209247=CARTESIAN_POINT('Ctrl Pts',(51.815081994581,-69.9462323856597,-213.482350651028));
#209248=CARTESIAN_POINT('Ctrl Pts',(51.8177782617349,-69.9449337383462,
-213.469834026062));
#209249=CARTESIAN_POINT('Ctrl Pts',(51.8240538444693,-69.9418920320008,
-213.438561955842));
#209250=CARTESIAN_POINT('Ctrl Pts',(51.8385687686859,-69.934807758839,-213.360902677902));
#209251=CARTESIAN_POINT('Ctrl Pts',(51.8472684687624,-69.9303859558978,
-213.285865302574));
#209252=CARTESIAN_POINT('Ctrl Pts',(51.8506358032439,-69.9286975854465,
-213.227536545096));
#209253=CARTESIAN_POINT('Ctrl Pts',(51.9718267086745,-69.8471376007524,
-213.236262748316));
#209254=CARTESIAN_POINT('Ctrl Pts',(51.9712180886111,-69.8474280289595,
-213.25115219161));
#209255=CARTESIAN_POINT('Ctrl Pts',(51.9704619947239,-69.8477893139844,
-213.266128674664));
#209256=CARTESIAN_POINT('Ctrl Pts',(51.9695578201616,-69.8482201770776,
-213.281192197065));
#209257=CARTESIAN_POINT('Ctrl Pts',(51.9668452964747,-69.849512766357,-213.326382764268));
#209258=CARTESIAN_POINT('Ctrl Pts',(51.9628004574897,-69.8514324567245,
-213.372356687621));
#209259=CARTESIAN_POINT('Ctrl Pts',(51.957403416313,-69.8539366328684,-213.419113967205));
#209260=CARTESIAN_POINT('Ctrl Pts',(51.953805388862,-69.8556060836309,-213.450285486928));
#209261=CARTESIAN_POINT('Ctrl Pts',(51.9496063062332,-69.857535073295,-213.481805164329));
#209262=CARTESIAN_POINT('Ctrl Pts',(51.9447991135993,-69.859707575833,-213.513672998779));
#209263=CARTESIAN_POINT('Ctrl Pts',(51.9423955172823,-69.8607938271019,
-213.529606916005));
#209264=CARTESIAN_POINT('Ctrl Pts',(51.9398398741415,-69.8619409124089,
-213.545627872515));
#209265=CARTESIAN_POINT('Ctrl Pts',(51.9371312039438,-69.8631465120197,
-213.561735868497));
#209266=CARTESIAN_POINT('Ctrl Pts',(51.9357768688449,-69.863749311825,-213.569789866489));
#209267=CARTESIAN_POINT('Ctrl Pts',(51.9343842753551,-69.8643667368211,
-213.577865624349));
#209268=CARTESIAN_POINT('Ctrl Pts',(51.9329532930758,-69.8649984740466,
-213.585963142108));
#209269=CARTESIAN_POINT('Ctrl Pts',(51.9318040898334,-69.8655058139895,
-213.59246615322));
#209270=CARTESIAN_POINT('Ctrl Pts',(51.9304882819738,-69.8660846575816,
-213.599761180333));
#209271=CARTESIAN_POINT('Ctrl Pts',(51.9293469843985,-69.8665849976042,
-213.605973625865));
#209272=CARTESIAN_POINT('Ctrl Pts',(51.9290671437927,-69.8667076785404,
-213.607496887247));
#209273=CARTESIAN_POINT('Ctrl Pts',(51.9287980217135,-69.8668255599709,
-213.608955159132));
#209274=CARTESIAN_POINT('Ctrl Pts',(51.9285450430171,-69.8669362930855,
-213.6103209751));
#209275=CARTESIAN_POINT('Ctrl Pts',(51.9259755968611,-69.8680609837394,
-213.624193252248));
#209276=CARTESIAN_POINT('Ctrl Pts',(51.9232746503919,-69.8692348882112,
-213.638224440989));
#209277=CARTESIAN_POINT('Ctrl Pts',(51.9204413918511,-69.8704558726239,
-213.652414541545));
#209278=CARTESIAN_POINT('Ctrl Pts',(51.9130092672967,-69.8736587247825,
-213.689637616408));
#209279=CARTESIAN_POINT('Ctrl Pts',(51.9046682050277,-69.8771859654199,
-213.727954683684));
#209280=CARTESIAN_POINT('Ctrl Pts',(51.8953968498963,-69.8809927158852,
-213.767364302023));
#209281=CARTESIAN_POINT('Ctrl Pts',(51.8940649868285,-69.8815395690993,
-213.773025633558));
#209282=CARTESIAN_POINT('Ctrl Pts',(51.8927139885145,-69.8820921380719,
-213.778709544735));
#209283=CARTESIAN_POINT('Ctrl Pts',(51.8913438570338,-69.8826502356811,
-213.784416065952));
#209284=CARTESIAN_POINT('Ctrl Pts',(51.8840719367677,-69.8856123173298,
-213.81470320837));
#209285=CARTESIAN_POINT('Ctrl Pts',(51.8762586474763,-69.8887317234872,
-213.845625996737));
#209286=CARTESIAN_POINT('Ctrl Pts',(51.8678939860897,-69.8919803770025,
-213.877184429624));
#209287=CARTESIAN_POINT('Ctrl Pts',(51.8637116553965,-69.8936047037601,
-213.892963646068));
#209288=CARTESIAN_POINT('Ctrl Pts',(51.8593914425586,-69.8952612418583,
-213.908901773702));
#209289=CARTESIAN_POINT('Ctrl Pts',(51.8549319444312,-69.8969457262148,
-213.924998812825));
#209290=CARTESIAN_POINT('Ctrl Pts',(51.8527021953674,-69.897787968393,-213.933047332387));
#209291=CARTESIAN_POINT('Ctrl Pts',(51.8504376220739,-69.898637188788,-213.941135579829));
#209292=CARTESIAN_POINT('Ctrl Pts',(51.8481380362862,-69.8994927979795,
-213.949263555208));
#209293=CARTESIAN_POINT('Ctrl Pts',(51.8461958706252,-69.9002154215058,
-213.956128215252));
#209294=CARTESIAN_POINT('Ctrl Pts',(51.8438732407178,-69.9010733451928,
-213.964258553209));
#209295=CARTESIAN_POINT('Ctrl Pts',(51.842070356574,-69.9017349392692,-213.970519352044));
#209296=CARTESIAN_POINT('Ctrl Pts',(51.8417385686673,-69.9018566935785,
-213.97167153775));
#209297=CARTESIAN_POINT('Ctrl Pts',(51.841424522012,-69.9019717967303,-213.972760460356));
#209298=CARTESIAN_POINT('Ctrl Pts',(51.8411339883627,-69.9020781818389,
-213.973766641235));
#209299=CARTESIAN_POINT('Ctrl Pts',(51.8387541055504,-69.902949626824,-213.982008690256));
#209300=CARTESIAN_POINT('Ctrl Pts',(51.8363363641231,-69.903827736172,-213.990295341577));
#209301=CARTESIAN_POINT('Ctrl Pts',(51.8338819984518,-69.9047112698955,
-213.998627680016));
#209302=CARTESIAN_POINT('Ctrl Pts',(51.8324808638191,-69.9052156567168,
-214.003384399072));
#209303=CARTESIAN_POINT('Ctrl Pts',(51.8310675260514,-69.9057218589305,
-214.008155744382));
#209304=CARTESIAN_POINT('Ctrl Pts',(51.8296420981419,-69.9062297402504,
-214.012941827738));
#209305=CARTESIAN_POINT('Ctrl Pts',(51.8153492654977,-69.9113222901152,
-214.060932110502));
#209306=CARTESIAN_POINT('Ctrl Pts',(51.7998409444251,-69.916585345507,-214.11040028011));
#209307=CARTESIAN_POINT('Ctrl Pts',(51.7830759342136,-69.9219270924958,
-214.161345223105));
#209308=CARTESIAN_POINT('Ctrl Pts',(51.7676354711688,-69.9268468059905,
-214.208265177207));
#209309=CARTESIAN_POINT('Ctrl Pts',(51.7511288569624,-69.9318331635702,
-214.256437733182));
#209310=CARTESIAN_POINT('Ctrl Pts',(51.7335529865694,-69.9367881584781,
-214.305864031718));
#209311=CARTESIAN_POINT('Ctrl Pts',(51.715411255478,-69.941902681012,-214.356881625546));
#209312=CARTESIAN_POINT('Ctrl Pts',(51.6961231833034,-69.9469868554723,
-214.409234130947));
#209313=CARTESIAN_POINT('Ctrl Pts',(51.6756673953278,-69.9519113844906,
-214.462922288982));
#209314=CARTESIAN_POINT('Ctrl Pts',(51.6725028704175,-69.952673212623,-214.471227885115));
#209315=CARTESIAN_POINT('Ctrl Pts',(51.6693104576324,-69.9534311389829,
-214.479565427316));
#209316=CARTESIAN_POINT('Ctrl Pts',(51.666090144668,-69.9541845926543,-214.487934896969));
#209317=CARTESIAN_POINT('Ctrl Pts',(51.6540717845718,-69.9569965173456,
-214.519170153049));
#209318=CARTESIAN_POINT('Ctrl Pts',(51.6416637393713,-69.9597467973301,
-214.550850462129));
#209319=CARTESIAN_POINT('Ctrl Pts',(51.6288629772096,-69.9624031668261,
-214.582975828909));
#209320=CARTESIAN_POINT('Ctrl Pts',(51.6224625961287,-69.9637313515741,
-214.599038512299));
#209321=CARTESIAN_POINT('Ctrl Pts',(51.6159640247811,-69.9650359813243,
-214.615212460306));
#209322=CARTESIAN_POINT('Ctrl Pts',(51.6093669926804,-69.9663124743072,
-214.631497673968));
#209323=CARTESIAN_POINT('Ctrl Pts',(51.6060684766301,-69.9669507207987,
-214.639640280798));
#209324=CARTESIAN_POINT('Ctrl Pts',(51.6027453449678,-69.967581927318,-214.647810704043));
#209325=CARTESIAN_POINT('Ctrl Pts',(51.5993975681366,-69.9682054833559,
-214.656008943773));
#209326=CARTESIAN_POINT('Ctrl Pts',(51.5960497913055,-69.9688290393938,
-214.664207183504));
#209327=CARTESIAN_POINT('Ctrl Pts',(51.5922089524539,-69.9695287310569,
-214.673571360434));
#209328=CARTESIAN_POINT('Ctrl Pts',(51.5892787609849,-69.97005283305,-214.680686254955));
#209329=CARTESIAN_POINT('Ctrl Pts',(51.5855178612913,-69.9707255177692,
-214.689818219507));
#209330=CARTESIAN_POINT('Ctrl Pts',(51.5817432158244,-69.9713850932742,
-214.698946551937));
#209331=CARTESIAN_POINT('Ctrl Pts',(51.577955362358,-69.9720309789322,-214.70807142067));
#209332=CARTESIAN_POINT('Ctrl Pts',(51.5407516159422,-69.9783747740254,
-214.797694555628));
#209333=CARTESIAN_POINT('Ctrl Pts',(51.5021322457915,-69.983522563863,-214.887276965874));
#209334=CARTESIAN_POINT('Ctrl Pts',(51.4620858828276,-69.9871863037332,
-214.977038137691));
#209335=CARTESIAN_POINT('Ctrl Pts',(51.4553825953226,-69.987799570454,-214.992063096188));
#209336=CARTESIAN_POINT('Ctrl Pts',(51.4486393137466,-69.9883711391208,
-215.007093047948));
#209337=CARTESIAN_POINT('Ctrl Pts',(51.4418559736239,-69.9888995124673,
-215.022129004877));
#209338=CARTESIAN_POINT('Ctrl Pts',(51.4054244374199,-69.9917372667819,
-215.102883176025));
#209339=CARTESIAN_POINT('Ctrl Pts',(51.3678140905141,-69.9933348295019,
-215.183840248426));
#209340=CARTESIAN_POINT('Ctrl Pts',(51.3289922766921,-69.9934293097912,
-215.265239689279));
#209341=CARTESIAN_POINT('Ctrl Pts',(51.3130055938261,-69.9934682164335,
-215.29875968534));
#209342=CARTESIAN_POINT('Ctrl Pts',(51.2968134974982,-69.9932516514847,
-215.332354687047));
#209343=CARTESIAN_POINT('Ctrl Pts',(51.2804138736011,-69.9927586351109,
-215.366041430998));
#209344=CARTESIAN_POINT('Ctrl Pts',(51.2322113007033,-69.991309537385,-215.465055148702));
#209345=CARTESIAN_POINT('Ctrl Pts',(51.1833271215805,-69.9875001826157,
-215.562558563164));
#209346=CARTESIAN_POINT('Ctrl Pts',(51.1340474348521,-69.9811339312681,
-215.658556370273));
#209347=CARTESIAN_POINT('Ctrl Pts',(51.0857566979389,-69.9748954385065,
-215.752627683529));
#209348=CARTESIAN_POINT('Ctrl Pts',(51.0370862445689,-69.9662015861898,
-215.845253336452));
#209349=CARTESIAN_POINT('Ctrl Pts',(50.988291150118,-69.9549150808236,-215.936431165693));
#209350=CARTESIAN_POINT('Ctrl Pts',(50.9707187829144,-69.9508505202571,
-215.969266644634));
#209351=CARTESIAN_POINT('Ctrl Pts',(50.9531301111087,-69.9464501771695,
-216.001914282774));
#209352=CARTESIAN_POINT('Ctrl Pts',(50.9355365677156,-69.9417092155658,
-216.034373717099));
#209353=CARTESIAN_POINT('Ctrl Pts',(56.7848125695504,-63.9246781901443,
-216.32517479574));
#209354=CARTESIAN_POINT('Ctrl Pts',(56.6914248998238,-63.6774027044323,
-216.115752570451));
#209355=CARTESIAN_POINT('Ctrl Pts',(56.9501445726978,-63.4755122787923,
-216.036568692573));
#209356=CARTESIAN_POINT('Ctrl Pts',(56.8894862224836,-64.207100718668,-215.816976621421));
#209357=CARTESIAN_POINT('Ctrl Pts',(56.8535591097954,-63.9616332231967,
-215.693685144435));
#209358=CARTESIAN_POINT('Ctrl Pts',(57.0658653622442,-63.8303542975169,
-215.574406016486));
#209359=CARTESIAN_POINT('Ctrl Pts',(56.8975641679252,-64.4758958672083,
-215.297354439506));
#209360=CARTESIAN_POINT('Ctrl Pts',(56.9070622928758,-64.2861767382064,
-215.200133915087));
#209361=CARTESIAN_POINT('Ctrl Pts',(57.0603127501189,-64.1729106578878,
-215.102057245562));
#209362=CARTESIAN_POINT('Ctrl Pts',(56.8418253372028,-64.8002473979207,
-214.513441216471));
#209363=CARTESIAN_POINT('Ctrl Pts',(56.8725452070173,-64.6752546110846,
-214.449672310422));
#209364=CARTESIAN_POINT('Ctrl Pts',(56.9710064262051,-64.589603741335,-214.390090855151));
#209365=CARTESIAN_POINT('Ctrl Pts',(56.8164834138299,-64.8889909543264,
-214.276550655991));
#209366=CARTESIAN_POINT('Ctrl Pts',(56.8499614295511,-64.7813997862752,
-214.224386280783));
#209367=CARTESIAN_POINT('Ctrl Pts',(56.9338189208405,-64.7041705810812,
-214.174927340598));
#209368=CARTESIAN_POINT('Ctrl Pts',(56.7542865190199,-65.0610681985444,
-213.691334443373));
#209369=CARTESIAN_POINT('Ctrl Pts',(56.7891152509752,-64.9853348405543,
-213.67002187732));
#209370=CARTESIAN_POINT('Ctrl Pts',(56.845223212725,-64.9270476219534,-213.643352384884));
#209371=CARTESIAN_POINT('Ctrl Pts',(56.715855751278,-65.1308968640445,-213.329423714843));
#209372=CARTESIAN_POINT('Ctrl Pts',(56.7467138871531,-65.0699208185081,
-213.321468010001));
#209373=CARTESIAN_POINT('Ctrl Pts',(56.7926294083244,-65.0181571456724,
-213.314757534777));
#209374=CARTESIAN_POINT('Ctrl Pts',(56.7379487726703,-65.0891150537523,
-212.933426638013));
#209375=CARTESIAN_POINT('Ctrl Pts',(56.7708234918149,-65.0194823467915,
-212.944141985026));
#209376=CARTESIAN_POINT('Ctrl Pts',(56.8230504447964,-64.9635917011068,
-212.954964540018));
#209377=CARTESIAN_POINT('',(56.8144552895507,-64.9781463989707,-213.256094899005));
#209378=CARTESIAN_POINT('',(56.7323722878851,-65.0994854859682,-213.264821102391));
#209379=CARTESIAN_POINT('Origin',(57.1832000972235,-65.315712880919,-213.264821102391));
#209380=CARTESIAN_POINT('Ctrl Pts',(56.8293274051384,-64.0646324794683,
-216.070020447203));
#209381=CARTESIAN_POINT('Ctrl Pts',(56.84326082334,-64.1169296295291,-215.973290586946));
#209382=CARTESIAN_POINT('Ctrl Pts',(56.8540807904868,-64.1687301223484,
-215.875753618678));
#209383=CARTESIAN_POINT('Ctrl Pts',(56.8620665015112,-64.2197520230989,
-215.777434450787));
#209384=CARTESIAN_POINT('Ctrl Pts',(56.8704637792726,-64.2734034852173,
-215.674048119936));
#209385=CARTESIAN_POINT('Ctrl Pts',(56.8757276601601,-64.3261933988336,
-215.569796347129));
#209386=CARTESIAN_POINT('Ctrl Pts',(56.8782372726827,-64.3778064713355,
-215.464718636094));
#209387=CARTESIAN_POINT('Ctrl Pts',(56.8787179510732,-64.3876921761587,
-215.444592586928));
#209388=CARTESIAN_POINT('Ctrl Pts',(56.8790977254115,-64.3975347599611,
-215.424436281727));
#209389=CARTESIAN_POINT('Ctrl Pts',(56.8793794439324,-64.4073320876536,
-215.404250065956));
#209390=CARTESIAN_POINT('Ctrl Pts',(56.8809734983155,-64.462768532161,-215.290029937206));
#209391=CARTESIAN_POINT('Ctrl Pts',(56.8794264385425,-64.516761707439,-215.174834553312));
#209392=CARTESIAN_POINT('Ctrl Pts',(56.8752707176649,-64.5689845407945,
-215.058643815246));
#209393=CARTESIAN_POINT('Ctrl Pts',(56.8717243682961,-64.6135497119317,
-214.959490632745));
#209394=CARTESIAN_POINT('Ctrl Pts',(56.8662794381607,-64.6568268726743,
-214.859611308838));
#209395=CARTESIAN_POINT('Ctrl Pts',(56.8592726682421,-64.6986417564396,
-214.758976432767));
#209396=CARTESIAN_POINT('Ctrl Pts',(56.8589144900082,-64.7007792864842,
-214.753832090567));
#209397=CARTESIAN_POINT('Ctrl Pts',(56.858569077902,-64.7028133839436,-214.748925881222));
#209398=CARTESIAN_POINT('Ctrl Pts',(56.858219143076,-64.7048497019118,-214.744003822932));
#209399=CARTESIAN_POINT('Ctrl Pts',(56.857577925288,-64.708581034737,-214.734984682525));
#209400=CARTESIAN_POINT('Ctrl Pts',(56.8569216476466,-64.7123212263355,
-214.725912519824));
#209401=CARTESIAN_POINT('Ctrl Pts',(56.856129531978,-64.7167079167791,-214.715214173572));
#209402=CARTESIAN_POINT('Ctrl Pts',(56.8521198803907,-64.7389131337681,
-214.661059657083));
#209403=CARTESIAN_POINT('Ctrl Pts',(56.8477627871993,-64.7600622131556,
-214.608091953219));
#209404=CARTESIAN_POINT('Ctrl Pts',(56.8432140576396,-64.780169866364,-214.556312554883));
#209405=CARTESIAN_POINT('Ctrl Pts',(56.8422067256955,-64.784622775936,-214.544845827459));
#209406=CARTESIAN_POINT('Ctrl Pts',(56.8411898176111,-64.7890246987895,
-214.533437326435));
#209407=CARTESIAN_POINT('Ctrl Pts',(56.8401647355452,-64.7933759337862,
-214.522086984327));
#209408=CARTESIAN_POINT('Ctrl Pts',(56.8352240963379,-64.8143477983232,
-214.467381173837));
#209409=CARTESIAN_POINT('Ctrl Pts',(56.8300966765821,-64.8341405916693,
-214.414027988426));
#209410=CARTESIAN_POINT('Ctrl Pts',(56.8249223102875,-64.8527646839859,
-214.362027845373));
#209411=CARTESIAN_POINT('Ctrl Pts',(56.8241752397253,-64.8554536144417,
-214.354520109372));
#209412=CARTESIAN_POINT('Ctrl Pts',(56.8234271210218,-64.8581182365231,
-214.347040568721));
#209413=CARTESIAN_POINT('Ctrl Pts',(56.8226783067622,-64.8607586336227,
-214.339589215315));
#209414=CARTESIAN_POINT('Ctrl Pts',(56.8172799740449,-64.8797937172462,
-214.28587110783));
#209415=CARTESIAN_POINT('Ctrl Pts',(56.8118472574457,-64.8975712685443,
-214.233618613337));
#209416=CARTESIAN_POINT('Ctrl Pts',(56.8064985328116,-64.9141125012779,
-214.182831658659));
#209417=CARTESIAN_POINT('Ctrl Pts',(56.8059665418472,-64.9157577133529,
-214.177780323463));
#209418=CARTESIAN_POINT('Ctrl Pts',(56.8054353518806,-64.9173907247201,
-214.172743487259));
#209419=CARTESIAN_POINT('Ctrl Pts',(56.8049050600144,-64.9190115751451,
-214.167721150608));
#209420=CARTESIAN_POINT('Ctrl Pts',(56.8019740932707,-64.9279701487072,
-214.139962283016));
#209421=CARTESIAN_POINT('Ctrl Pts',(56.7990710543229,-64.9365561442558,
-214.112646317844));
#209422=CARTESIAN_POINT('Ctrl Pts',(56.7962122881473,-64.9447733636485,
-214.085773252415));
#209423=CARTESIAN_POINT('Ctrl Pts',(56.7947829050594,-64.9488819733448,
-214.0723367197));
#209424=CARTESIAN_POINT('Ctrl Pts',(56.793364567285,-64.9528983769426,-214.059010911378));
#209425=CARTESIAN_POINT('Ctrl Pts',(56.7919591967795,-64.9568229761714,
-214.04579579105));
#209426=CARTESIAN_POINT('Ctrl Pts',(56.7914940574196,-64.9581219116236,
-214.041421946155));
#209427=CARTESIAN_POINT('Ctrl Pts',(56.7910303191845,-64.9594108420278,
-214.0370598135));
#209428=CARTESIAN_POINT('Ctrl Pts',(56.7905681137647,-64.9606896047482,
-214.032710478153));
#209429=CARTESIAN_POINT('Ctrl Pts',(56.7903320662302,-64.9613426667301,
-214.030489279869));
#209430=CARTESIAN_POINT('Ctrl Pts',(56.7900963750574,-64.9619931979646,
-214.028271126613));
#209431=CARTESIAN_POINT('Ctrl Pts',(56.7898610688874,-64.9626411620832,
-214.026056163046));
#209432=CARTESIAN_POINT('Ctrl Pts',(56.7892594651863,-64.9642978020765,
-214.02039319943));
#209433=CARTESIAN_POINT('Ctrl Pts',(56.7887964162145,-64.9655667092386,
-214.016032247683));
#209434=CARTESIAN_POINT('Ctrl Pts',(56.7881197951723,-64.9674090172119,
-214.009650980091));
#209435=CARTESIAN_POINT('Ctrl Pts',(56.7880135606757,-64.9676982731583,
-214.00864907399));
#209436=CARTESIAN_POINT('Ctrl Pts',(56.7879020590799,-64.9680015799114,
-214.007597310036));
#209437=CARTESIAN_POINT('Ctrl Pts',(56.7877839260599,-64.9683225474116,
-214.006482759224));
#209438=CARTESIAN_POINT('Ctrl Pts',(56.7831823982202,-64.9808249018571,
-213.963068677471));
#209439=CARTESIAN_POINT('Ctrl Pts',(56.7787367570231,-64.9923644894355,
-213.920682639109));
#209440=CARTESIAN_POINT('Ctrl Pts',(56.7745322143122,-65.0029589631916,
-213.879327038137));
#209441=CARTESIAN_POINT('Ctrl Pts',(56.7723732859695,-65.0083989625544,
-213.858091963313));
#209442=CARTESIAN_POINT('Ctrl Pts',(56.7702771925501,-65.0135903115608,
-213.837128418878));
#209443=CARTESIAN_POINT('Ctrl Pts',(56.7682513586567,-65.0185384446053,
-213.81643577243));
#209444=CARTESIAN_POINT('Ctrl Pts',(56.7652657719922,-65.0258307897876,
-213.785939842091));
#209445=CARTESIAN_POINT('Ctrl Pts',(56.7624343578982,-65.0325914981013,
-213.756033196312));
#209446=CARTESIAN_POINT('Ctrl Pts',(56.7597790035186,-65.0388290000784,
-213.726715837373));
#209447=CARTESIAN_POINT('Ctrl Pts',(56.7584513263288,-65.0419477510669,
-213.712057157904));
#209448=CARTESIAN_POINT('Ctrl Pts',(56.7571675863838,-65.0449356659555,
-213.697545800093));
#209449=CARTESIAN_POINT('Ctrl Pts',(56.7559300838455,-65.0477936839908,
-213.683181763961));
#209450=CARTESIAN_POINT('Ctrl Pts',(56.7553113325763,-65.0492226930084,
-213.675999745895));
#209451=CARTESIAN_POINT('Ctrl Pts',(56.7547041368897,-65.0506192261019,
-213.668854558246));
#209452=CARTESIAN_POINT('Ctrl Pts',(56.7541087628032,-65.0519833917363,
-213.661746201));
#209453=CARTESIAN_POINT('Ctrl Pts',(56.7536173495646,-65.0531093545007,
-213.655879064802));
#209454=CARTESIAN_POINT('Ctrl Pts',(56.7532003342218,-65.054062025313,-213.650845260365));
#209455=CARTESIAN_POINT('Ctrl Pts',(56.7526934344304,-65.0552163784068,
-213.644643633688));
#209456=CARTESIAN_POINT('Ctrl Pts',(56.7525861973272,-65.0554605873883,
-213.643331649562));
#209457=CARTESIAN_POINT('Ctrl Pts',(56.7524749911325,-65.0557136672505,
-213.641967333306));
#209458=CARTESIAN_POINT('Ctrl Pts',(56.7523583579841,-65.0559788895194,
-213.640531620456));
#209459=CARTESIAN_POINT('Ctrl Pts',(56.7484892101348,-65.0647772816159,
-213.592903777379));
#209460=CARTESIAN_POINT('Ctrl Pts',(56.7450977176229,-65.0722727884523,
-213.546104049185));
#209461=CARTESIAN_POINT('Ctrl Pts',(56.7422442798078,-65.0784822788702,
-213.500132498924));
#209462=CARTESIAN_POINT('Ctrl Pts',(56.7411569104229,-65.0808485507898,
-213.482613961788));
#209463=CARTESIAN_POINT('Ctrl Pts',(56.7401472913062,-65.0830284776309,
-213.465215688936));
#209464=CARTESIAN_POINT('Ctrl Pts',(56.739217431577,-65.0850244019591,-213.447937667528));
#209465=CARTESIAN_POINT('Ctrl Pts',(56.7375324485498,-65.0886411825456,
-213.416628458296));
#209466=CARTESIAN_POINT('Ctrl Pts',(56.7361109105069,-65.0916508059742,
-213.385714140014));
#209467=CARTESIAN_POINT('Ctrl Pts',(56.7349660432972,-65.0940592063371,
-213.355194712262));
#209468=CARTESIAN_POINT('Ctrl Pts',(56.7343936096924,-65.0952634065186,
-213.339934998386));
#209469=CARTESIAN_POINT('Ctrl Pts',(56.7338903052853,-65.0963172819309,
-213.324774007188));
#209470=CARTESIAN_POINT('Ctrl Pts',(56.7334575601726,-65.0972214635079,
-213.309711738833));
#209471=CARTESIAN_POINT('Ctrl Pts',(56.7330248150599,-65.0981256450848,
-213.294649470477));
#209472=CARTESIAN_POINT('Ctrl Pts',(56.7326626297635,-65.0988801316234,
-213.279685924923));
#209473=CARTESIAN_POINT('Ctrl Pts',(56.7323722878852,-65.0994854859681,
-213.264821102391));
#209474=CARTESIAN_POINT('Ctrl Pts',(56.8144552965909,-64.9781464054155,
-213.256094899172));
#209475=CARTESIAN_POINT('Ctrl Pts',(56.8173698192824,-64.9724082471664,
-213.354908067617));
#209476=CARTESIAN_POINT('Ctrl Pts',(56.826589953151,-64.9552496135495,-213.462936231746));
#209477=CARTESIAN_POINT('Ctrl Pts',(56.8478208203418,-64.9105102551182,
-213.638651304624));
#209478=CARTESIAN_POINT('Ctrl Pts',(56.8561265977695,-64.8924262632227,
-213.699497248996));
#209479=CARTESIAN_POINT('Ctrl Pts',(56.8701310542426,-64.8602769803466,
-213.794107197711));
#209480=CARTESIAN_POINT('Ctrl Pts',(56.877519322744,-64.8429461914106,-213.842246804829));
#209481=CARTESIAN_POINT('Ctrl Pts',(56.8867453394759,-64.8204671022411,
-213.899847655935));
#209482=CARTESIAN_POINT('Ctrl Pts',(56.891500998712,-64.8086546888112,-213.929004149363));
#209483=CARTESIAN_POINT('Ctrl Pts',(56.8935687422973,-64.8034686168898,
-213.941575706016));
#209484=CARTESIAN_POINT('Ctrl Pts',(56.894953708788,-64.7999836718063,-213.94997356981));
#209485=CARTESIAN_POINT('Ctrl Pts',(56.8959660672666,-64.7974254727206,
-213.956090873043));
#209486=CARTESIAN_POINT('Ctrl Pts',(56.9085806509794,-64.7654768744261,
-214.032181519627));
#209487=CARTESIAN_POINT('Ctrl Pts',(56.9245208634359,-64.7239387163797,
-214.123129670428));
#209488=CARTESIAN_POINT('Ctrl Pts',(56.9506552785366,-64.6428094702132,
-214.284669744791));
#209489=CARTESIAN_POINT('Ctrl Pts',(56.9597238315858,-64.6126176262786,
-214.342694808236));
#209490=CARTESIAN_POINT('Ctrl Pts',(56.9733270105072,-64.5621346734833,
-214.435816572145));
#209491=CARTESIAN_POINT('Ctrl Pts',(56.9801274940962,-64.5355934286946,
-214.483897125758));
#209492=CARTESIAN_POINT('Ctrl Pts',(56.9868156677765,-64.5070058705281,
-214.534208560028));
#209493=CARTESIAN_POINT('Ctrl Pts',(56.9912365333911,-64.4874815157085,
-214.568238727438));
#209494=CARTESIAN_POINT('Ctrl Pts',(56.9932850709852,-64.4781618507159,
-214.584343321439));
#209495=CARTESIAN_POINT('Ctrl Pts',(57.0140657811359,-64.3799782829966,
-214.752247756963));
#209496=CARTESIAN_POINT('Ctrl Pts',(57.0241767490285,-64.3015299352387,
-214.877176173881));
#209497=CARTESIAN_POINT('Ctrl Pts',(57.0331607991196,-64.2027589295951,
-215.029558796027));
#209498=CARTESIAN_POINT('Ctrl Pts',(57.0351000718181,-64.1729616787377,
-215.07453124402));
#209499=CARTESIAN_POINT('Ctrl Pts',(57.0369954878965,-64.1334541081786,
-215.13349269937));
#209500=CARTESIAN_POINT('Ctrl Pts',(57.0376874847421,-64.1149952719801,
-215.160849123836));
#209501=CARTESIAN_POINT('Ctrl Pts',(57.03814759071,-64.0958133018828,-215.189096154017));
#209502=CARTESIAN_POINT('Ctrl Pts',(57.0383015913884,-64.0868199657608,
-215.202308125432));
#209503=CARTESIAN_POINT('Ctrl Pts',(57.038352406177,-64.0830947089198,-215.207775655625));
#209504=CARTESIAN_POINT('Ctrl Pts',(57.0383830268799,-64.0806399804401,
-215.211377463292));
#209505=CARTESIAN_POINT('Ctrl Pts',(57.0383846983023,-64.080615480532,-215.211413793855));
#209506=CARTESIAN_POINT('Ctrl Pts',(57.0399527711531,-63.9254596265941,
-215.438958594151));
#209507=CARTESIAN_POINT('Ctrl Pts',(57.022928908771,-63.7820296637233,-215.635331946852));
#209508=CARTESIAN_POINT('Ctrl Pts',(56.9946437346772,-63.6543417315389,
-215.806005049013));
#209509=CARTESIAN_POINT('Ctrl Pts',(51.822850344383,-69.9419965866856,-213.735470748631));
#209510=CARTESIAN_POINT('Ctrl Pts',(51.8804433982798,-69.889324596863,-213.7397430898));
#209511=CARTESIAN_POINT('Ctrl Pts',(51.9513667677563,-69.856765622058,-213.744232219612));
#209512=CARTESIAN_POINT('Ctrl Pts',(51.8765276514687,-69.9171366797839,
-212.719415019637));
#209513=CARTESIAN_POINT('Ctrl Pts',(51.9284789001597,-69.8695011096846,
-212.726011510236));
#209514=CARTESIAN_POINT('Ctrl Pts',(51.991780071228,-69.8379778346573,-212.728235356937));
#209515=CARTESIAN_POINT('Ctrl Pts',(51.9334544096015,-69.8892734758678,
-211.703692143478));
#209516=CARTESIAN_POINT('Ctrl Pts',(51.9794687356772,-69.8470038946564,
-211.710263762613));
#209517=CARTESIAN_POINT('Ctrl Pts',(52.0346456619607,-69.816925009228,-211.71249177384));
#209518=CARTESIAN_POINT('Ctrl Pts',(52.0385712075059,-69.8271258445134,
-210.267504272468));
#209519=CARTESIAN_POINT('Ctrl Pts',(52.0734597321493,-69.7950116391773,
-210.272241986443));
#209520=CARTESIAN_POINT('Ctrl Pts',(52.1138191538044,-69.7700067918124,
-210.276283653453));
#209521=CARTESIAN_POINT('Ctrl Pts',(52.072185388712,-69.806348038251,-209.845388043713));
#209522=CARTESIAN_POINT('Ctrl Pts',(52.1034382988763,-69.7775433560357,
-209.850130119974));
#209523=CARTESIAN_POINT('Ctrl Pts',(52.1391384959575,-69.7543237267294,
-209.854167521602));
#209524=CARTESIAN_POINT('Ctrl Pts',(52.1354652353079,-69.763262836332,-209.213638050098));
#209525=CARTESIAN_POINT('Ctrl Pts',(52.1597481032177,-69.7408313624291,
-209.21810272547));
#209526=CARTESIAN_POINT('Ctrl Pts',(52.1868109938527,-69.7218145199576,
-209.222414495584));
#209527=CARTESIAN_POINT('Ctrl Pts',(52.1584910060187,-69.747112810802,-209.003150816985));
#209528=CARTESIAN_POINT('Ctrl Pts',(52.1802056110658,-69.7270298301124,
-209.007617928732));
#209529=CARTESIAN_POINT('Ctrl Pts',(52.2041584674497,-69.7096301545639,
-209.011927312326));
#209530=CARTESIAN_POINT('Ctrl Pts',(52.2022638893192,-69.7142992552832,
-208.689605786204));
#209531=CARTESIAN_POINT('Ctrl Pts',(52.2190101918288,-69.6987724358089,
-208.694007820048));
#209532=CARTESIAN_POINT('Ctrl Pts',(52.2371408246248,-69.6848794419398,
-208.698381586053));
#209533=CARTESIAN_POINT('Ctrl Pts',(52.2182336078506,-69.7020812266945,
-208.585328566142));
#209534=CARTESIAN_POINT('Ctrl Pts',(52.2331514504351,-69.6882319207143,
-208.589731796556));
#209535=CARTESIAN_POINT('Ctrl Pts',(52.249174245292,-69.6756642254024,-208.594104390417));
#209536=CARTESIAN_POINT('Ctrl Pts',(52.2489412320905,-69.6774578274061,
-208.431136608511));
#209537=CARTESIAN_POINT('Ctrl Pts',(52.2602903339986,-69.6668890135686,
-208.435525620945));
#209538=CARTESIAN_POINT('Ctrl Pts',(52.2723150773139,-69.6570951860835,
-208.439912289689));
#209539=CARTESIAN_POINT('Ctrl Pts',(52.2601800097299,-69.6683161240625,
-208.380021453291));
#209540=CARTESIAN_POINT('Ctrl Pts',(52.270214924355,-69.658955894537,-208.384411029018));
#209541=CARTESIAN_POINT('Ctrl Pts',(52.2807846875617,-69.6502015352889,
-208.388797146169));
#209542=CARTESIAN_POINT('Ctrl Pts',(52.281999678196,-69.6499593019998,-208.305729941084));
#209543=CARTESIAN_POINT('Ctrl Pts',(52.2894520983595,-69.6429772988716,
-208.310116951883));
#209544=CARTESIAN_POINT('Ctrl Pts',(52.2972292893049,-69.6363602565428,
-208.314505613017));
#209545=CARTESIAN_POINT('Ctrl Pts',(52.2900513245554,-69.6431141725604,
-208.281238728998));
#209546=CARTESIAN_POINT('Ctrl Pts',(52.2965464863421,-69.6370140514492,
-208.285625985819));
#209547=CARTESIAN_POINT('Ctrl Pts',(52.3032976103578,-69.6311990926332,
-208.290014406272));
#209548=CARTESIAN_POINT('Ctrl Pts',(52.3055109262683,-69.6296515882696,
-208.24731365204));
#209549=CARTESIAN_POINT('Ctrl Pts',(52.3101508205055,-69.6252622995574,
-208.251700725001));
#209550=CARTESIAN_POINT('Ctrl Pts',(52.3149497431651,-69.6210491476294,
-208.256089330814));
#209551=CARTESIAN_POINT('Ctrl Pts',(52.3112700002316,-69.624596121335,-208.236328897454));
#209552=CARTESIAN_POINT('Ctrl Pts',(52.31521638535,-69.6208465529984,-208.24071608881));
#209553=CARTESIAN_POINT('Ctrl Pts',(52.3192905030199,-69.6172377131638,
-208.245104578722));
#209554=CARTESIAN_POINT('Ctrl Pts',(52.4157911999455,-69.5313285632376,
-208.09911365756));
#209555=CARTESIAN_POINT('Ctrl Pts',(52.4070413724992,-69.5392973207822,
-208.103538654047));
#209556=CARTESIAN_POINT('Ctrl Pts',(52.3980737175552,-69.546924914442,-208.107889777235));
#209557=CARTESIAN_POINT('Ctrl Pts',(52.8039539674273,-69.1685749088719,
-208.261113958564));
#209558=CARTESIAN_POINT('Ctrl Pts',(52.7473775130206,-69.2207759621712,
-208.265385690945));
#209559=CARTESIAN_POINT('Ctrl Pts',(52.6906841717837,-69.273483049227,-208.269888341076));
#209560=CARTESIAN_POINT('Ctrl Pts',(53.3726051882046,-68.2329805102008,
-225.06502763524));
#209561=CARTESIAN_POINT('Ctrl Pts',(53.252682904108,-68.3309162879933,-225.681318331171));
#209562=CARTESIAN_POINT('Ctrl Pts',(53.1203834433686,-68.5685596498648,
-225.080427005024));
#209563=CARTESIAN_POINT('',(52.3440043138885,-69.594874440935,-208.218811515427));
#209564=CARTESIAN_POINT('',(52.3440560052495,-69.5949303622595,-208.210085312208));
#209565=CARTESIAN_POINT('Origin',(52.6833983856504,-69.9620415201413,-208.218811515427));
#209566=CARTESIAN_POINT('Ctrl Pts',(51.8506358032439,-69.9286975854465,
-213.227536545096));
#209567=CARTESIAN_POINT('Ctrl Pts',(51.8965359306666,-69.9068955059224,
-212.381067577369));
#209568=CARTESIAN_POINT('Ctrl Pts',(51.9463091177219,-69.8815088904097,
-211.535021517202));
#209569=CARTESIAN_POINT('Ctrl Pts',(52.0389353307874,-69.8267824525318,
-210.267914982609));
#209570=CARTESIAN_POINT('Ctrl Pts',(52.0725035102325,-69.806045505995,-209.8458402758));
#209571=CARTESIAN_POINT('Ctrl Pts',(52.1356910661391,-69.7630436587203,
-209.214130441658));
#209572=CARTESIAN_POINT('Ctrl Pts',(52.1586824184498,-69.7469248062077,
-209.003656181328));
#209573=CARTESIAN_POINT('Ctrl Pts',(52.2023855392512,-69.7141755312691,
-208.690099641439));
#209574=CARTESIAN_POINT('Ctrl Pts',(52.2183291852341,-69.7019815954277,
-208.585816112664));
#209575=CARTESIAN_POINT('Ctrl Pts',(52.2489833267826,-69.6774084341258,
-208.431581516949));
#209576=CARTESIAN_POINT('Ctrl Pts',(52.2602021616247,-69.6682855321809,
-208.380448072074));
#209577=CARTESIAN_POINT('Ctrl Pts',(52.2819812944307,-69.6499675527577,
-208.306095531171));
#209578=CARTESIAN_POINT('Ctrl Pts',(52.2900177211888,-69.6431370963428,
-208.281577994998));
#209579=CARTESIAN_POINT('Ctrl Pts',(52.3054538148208,-69.6296980513237,
-208.247576563664));
#209580=CARTESIAN_POINT('Ctrl Pts',(52.3112042959167,-69.6246512725098,
-208.236560595082));
#209581=CARTESIAN_POINT('Ctrl Pts',(52.3253253083163,-69.6120530454534,
-208.217923065672));
#209582=CARTESIAN_POINT('Ctrl Pts',(52.3341567138414,-69.6040808580668,
-208.210085312176));
#209583=CARTESIAN_POINT('Ctrl Pts',(52.3440560052495,-69.5949303622595,
-208.210085312208));
#209584=CARTESIAN_POINT('Ctrl Pts',(52.3440043138833,-69.5948744409406,
-208.218811515393));
#209585=CARTESIAN_POINT('Ctrl Pts',(52.3424820359817,-69.5962815717119,
-208.218811515395));
#209586=CARTESIAN_POINT('Ctrl Pts',(52.3408547147374,-69.5977800490423,
-208.219125748933));
#209587=CARTESIAN_POINT('Ctrl Pts',(52.3391512870202,-69.5993409672496,
-208.21987200544));
#209588=CARTESIAN_POINT('Ctrl Pts',(52.3376186249417,-69.6007454061464,
-208.220543451042));
#209589=CARTESIAN_POINT('Ctrl Pts',(52.3360244145561,-69.6022003180093,
-208.221565577745));
#209590=CARTESIAN_POINT('Ctrl Pts',(52.3343938226836,-69.6036815434254,
-208.222987281035));
#209591=CARTESIAN_POINT('Ctrl Pts',(52.3328814720798,-69.6050553587805,
-208.224305890471));
#209592=CARTESIAN_POINT('Ctrl Pts',(52.3313378567263,-69.6064517683912,
-208.225968890555));
#209593=CARTESIAN_POINT('Ctrl Pts',(52.3297861601934,-69.6078494379871,
-208.227971012618));
#209594=CARTESIAN_POINT('Ctrl Pts',(52.3283529596706,-69.6091403739099,
-208.229820241721));
#209595=CARTESIAN_POINT('Ctrl Pts',(52.3269128910609,-69.6104323547897,
-208.2319590992));
#209596=CARTESIAN_POINT('Ctrl Pts',(52.3254865791142,-69.6117072283637,
-208.234337728021));
#209597=CARTESIAN_POINT('Ctrl Pts',(52.3251941318254,-69.6119686251227,
-208.234825435883));
#209598=CARTESIAN_POINT('Ctrl Pts',(52.3249022706465,-69.6122292986765,
-208.23532305026));
#209599=CARTESIAN_POINT('Ctrl Pts',(52.3246111854786,-69.612489086511,-208.235829859775));
#209600=CARTESIAN_POINT('Ctrl Pts',(52.3226799130822,-69.6142127094541,
-208.239192405634));
#209601=CARTESIAN_POINT('Ctrl Pts',(52.3207618818214,-69.6159161659265,
-208.242988126939));
#209602=CARTESIAN_POINT('Ctrl Pts',(52.3188715230813,-69.6175861945551,
-208.247212540653));
#209603=CARTESIAN_POINT('Ctrl Pts',(52.3171376894694,-69.6191179417879,
-208.25108716526));
#209604=CARTESIAN_POINT('Ctrl Pts',(52.3154272482004,-69.6206214591213,
-208.25532266912));
#209605=CARTESIAN_POINT('Ctrl Pts',(52.313737915979,-69.6220996391995,-208.259876064165));
#209606=CARTESIAN_POINT('Ctrl Pts',(52.312839974451,-69.6228853456825,-208.26229635927));
#209607=CARTESIAN_POINT('Ctrl Pts',(52.3119477536723,-69.6236641313598,
-208.264805759652));
#209608=CARTESIAN_POINT('Ctrl Pts',(52.3110589927009,-69.6244383044097,
-208.267392287932));
#209609=CARTESIAN_POINT('Ctrl Pts',(52.3085864708634,-69.6265920440916,
-208.274587977059));
#209610=CARTESIAN_POINT('Ctrl Pts',(52.3061287484059,-69.6287200926668,
-208.282439487147));
#209611=CARTESIAN_POINT('Ctrl Pts',(52.3037047421696,-69.6308048212131,
-208.290954531357));
#209612=CARTESIAN_POINT('Ctrl Pts',(52.3015089296444,-69.6326932953372,
-208.29866797716));
#209613=CARTESIAN_POINT('Ctrl Pts',(52.2993409311851,-69.634546082569,-208.3069260843));
#209614=CARTESIAN_POINT('Ctrl Pts',(52.2971949154258,-69.6363690309351,
-208.315703747231));
#209615=CARTESIAN_POINT('Ctrl Pts',(52.295364326622,-69.637924037628,-208.323191246527));
#209616=CARTESIAN_POINT('Ctrl Pts',(52.2935495863094,-69.6394574727516,
-208.331056549212));
#209617=CARTESIAN_POINT('Ctrl Pts',(52.2917323870528,-69.6409869521274,
-208.339261708216));
#209618=CARTESIAN_POINT('Ctrl Pts',(52.2884850180848,-69.6437201603016,
-208.353924480407));
#209619=CARTESIAN_POINT('Ctrl Pts',(52.2852408400929,-69.6464298179871,
-208.369711727464));
#209620=CARTESIAN_POINT('Ctrl Pts',(52.2820272057473,-69.6490902832157,
-208.38664308245));
#209621=CARTESIAN_POINT('Ctrl Pts',(52.2790795380118,-69.6515305631829,
-208.402173165666));
#209622=CARTESIAN_POINT('Ctrl Pts',(52.2761578716336,-69.6539291711863,
-208.418666029657));
#209623=CARTESIAN_POINT('Ctrl Pts',(52.2732561995377,-69.6562917771648,
-208.436115348614));
#209624=CARTESIAN_POINT('Ctrl Pts',(52.2705180528767,-69.658521237096,-208.452581300955));
#209625=CARTESIAN_POINT('Ctrl Pts',(52.2677979993281,-69.6607183676128,
-208.469899152139));
#209626=CARTESIAN_POINT('Ctrl Pts',(52.2650615521283,-69.6629155667661,
-208.488040589413));
#209627=CARTESIAN_POINT('Ctrl Pts',(52.2648981281873,-69.6630467861606,
-208.489124018019));
#209628=CARTESIAN_POINT('Ctrl Pts',(52.2647346358121,-69.6631780151523,
-208.490210376304));
#209629=CARTESIAN_POINT('Ctrl Pts',(52.2645710637428,-69.6633092643157,
-208.491299655199));
#209630=CARTESIAN_POINT('Ctrl Pts',(52.260313528908,-69.6667254825471,-208.519651945799));
#209631=CARTESIAN_POINT('Ctrl Pts',(52.2560326046515,-69.6701265640873,
-208.550011208226));
#209632=CARTESIAN_POINT('Ctrl Pts',(52.2517649403206,-69.6734780506684,
-208.582409808769));
#209633=CARTESIAN_POINT('Ctrl Pts',(52.2477984711022,-69.6765930023912,
-208.61252184238));
#209634=CARTESIAN_POINT('Ctrl Pts',(52.2438438954802,-69.6796647025151,
-208.644395735144));
#209635=CARTESIAN_POINT('Ctrl Pts',(52.2399006765453,-69.6826934930627,
-208.678040517083));
#209636=CARTESIAN_POINT('Ctrl Pts',(52.2362593492553,-69.685490400325,-208.709109464727));
#209637=CARTESIAN_POINT('Ctrl Pts',(52.2326279198868,-69.688250517501,-208.741688626789));
#209638=CARTESIAN_POINT('Ctrl Pts',(52.2289751792274,-69.6910028859806,
-208.775768002304));
#209639=CARTESIAN_POINT('Ctrl Pts',(52.2280173563656,-69.6917246129522,
-208.784704307404));
#209640=CARTESIAN_POINT('Ctrl Pts',(52.2270578831674,-69.6924459799922,
-208.793743664294));
#209641=CARTESIAN_POINT('Ctrl Pts',(52.2260957795316,-69.6931679007633,
-208.802885662675));
#209642=CARTESIAN_POINT('Ctrl Pts',(52.2204632758245,-69.6973942868489,
-208.856406237649));
#209643=CARTESIAN_POINT('Ctrl Pts',(52.2147742585669,-69.7016079333847,
-208.913478699865));
#209644=CARTESIAN_POINT('Ctrl Pts',(52.2090738657013,-69.705766109449,-208.9741602494));
#209645=CARTESIAN_POINT('Ctrl Pts',(52.2037779171684,-69.7096292618573,
-209.030536427466));
#209646=CARTESIAN_POINT('Ctrl Pts',(52.1984726040311,-69.7134441130084,
-209.090027907352));
#209647=CARTESIAN_POINT('Ctrl Pts',(52.1931642068981,-69.7172043138646,
-209.152666203404));
#209648=CARTESIAN_POINT('Ctrl Pts',(52.1882858395736,-69.7206599032885,
-209.210230211722));
#209649=CARTESIAN_POINT('Ctrl Pts',(52.1834050653669,-69.7240691542093,
-209.270451914207));
#209650=CARTESIAN_POINT('Ctrl Pts',(52.1784963359389,-69.7274555197984,
-209.333341603547));
#209651=CARTESIAN_POINT('Ctrl Pts',(52.1759593382091,-69.7292057083019,
-209.365845126387));
#209652=CARTESIAN_POINT('Ctrl Pts',(52.1734143426905,-69.730950278557,-209.39906106946));
#209653=CARTESIAN_POINT('Ctrl Pts',(52.1708539451181,-69.7326960847145,
-209.432989076637));
#209654=CARTESIAN_POINT('Ctrl Pts',(52.1632697473111,-69.7378673672427,
-209.533487811832));
#209655=CARTESIAN_POINT('Ctrl Pts',(52.1555870040426,-69.7430150975709,
-209.640265501971));
#209656=CARTESIAN_POINT('Ctrl Pts',(52.1478593423169,-69.7480875585307,
-209.75344383926));
#209657=CARTESIAN_POINT('Ctrl Pts',(52.1406857719123,-69.7527963122406,
-209.858507026501));
#209658=CARTESIAN_POINT('Ctrl Pts',(52.1334739691835,-69.7574397630151,
-209.969085955311));
#209659=CARTESIAN_POINT('Ctrl Pts',(52.1262360091054,-69.762005099994,-210.085273463446));
#209660=CARTESIAN_POINT('Ctrl Pts',(52.1196204051817,-69.7661778863737,
-210.191470586172));
#209661=CARTESIAN_POINT('Ctrl Pts',(52.1129831293641,-69.7702852473543,
-210.302353273817));
#209662=CARTESIAN_POINT('Ctrl Pts',(52.1063025138116,-69.7743460201426,
-210.417987894064));
#209663=CARTESIAN_POINT('Ctrl Pts',(52.1010659831097,-69.7775290144658,
-210.508626882994));
#209664=CARTESIAN_POINT('Ctrl Pts',(52.0958023524557,-69.7806838219579,
-210.602185411385));
#209665=CARTESIAN_POINT('Ctrl Pts',(52.0904846874294,-69.7838348020659,
-210.698693024827));
#209666=CARTESIAN_POINT('Ctrl Pts',(52.080225495559,-69.7899138817652,-210.884881910058));
#209667=CARTESIAN_POINT('Ctrl Pts',(52.0698067521628,-69.7959401628047,
-211.082055011306));
#209668=CARTESIAN_POINT('Ctrl Pts',(52.0592899423143,-69.8018521875684,
-211.290461140744));
#209669=CARTESIAN_POINT('Ctrl Pts',(52.0495256953229,-69.8073411591142,
-211.483954124991));
#209670=CARTESIAN_POINT('Ctrl Pts',(52.0396773891904,-69.8127312015491,
-211.687130103457));
#209671=CARTESIAN_POINT('Ctrl Pts',(52.0297642950147,-69.81800077633,-211.900183231084));
#209672=CARTESIAN_POINT('Ctrl Pts',(52.0202586260742,-69.8230537731479,
-212.104479938256));
#209673=CARTESIAN_POINT('Ctrl Pts',(52.0106939094361,-69.8279955156581,
-212.317858666779));
#209674=CARTESIAN_POINT('Ctrl Pts',(52.0010513321796,-69.832840099181,-212.540484705824));
#209675=CARTESIAN_POINT('Ctrl Pts',(51.9922011668754,-69.8372865623895,
-212.744815684374));
#209676=CARTESIAN_POINT('Ctrl Pts',(51.9832855225751,-69.8416510762705,
-212.956936580511));
#209677=CARTESIAN_POINT('Ctrl Pts',(51.9742552168064,-69.8459765591321,
-213.176969516857));
#209678=CARTESIAN_POINT('Ctrl Pts',(51.9734466757251,-69.8463638473015,
-213.196670474147));
#209679=CARTESIAN_POINT('Ctrl Pts',(51.9726371899477,-69.8467508461296,
-213.216434856257));
#209680=CARTESIAN_POINT('Ctrl Pts',(51.9718267086745,-69.8471376007524,
-213.236262748315));
#209681=CARTESIAN_POINT('Ctrl Pts',(56.4785498900846,-65.4721614184049,
-208.210085312209));
#209682=CARTESIAN_POINT('Ctrl Pts',(56.4784941157842,-65.4721095684412,
-208.214448081532));
#209683=CARTESIAN_POINT('Ctrl Pts',(56.478494115784,-65.4721095684411,-208.218811515427));
#209684=CARTESIAN_POINT('Ctrl Pts',(56.4880093612199,-65.4619859436241,
-208.210087277606));
#209685=CARTESIAN_POINT('Ctrl Pts',(56.4867940706151,-65.4631813685704,
-208.214450046893));
#209686=CARTESIAN_POINT('Ctrl Pts',(56.4856347339016,-65.464428502687,-208.218813480809));
#209687=CARTESIAN_POINT('Ctrl Pts',(56.4960155064695,-65.4531598633657,
-208.218220200296));
#209688=CARTESIAN_POINT('Ctrl Pts',(56.4938064756652,-65.455425583918,-208.222583010898));
#209689=CARTESIAN_POINT('Ctrl Pts',(56.4916787645948,-65.4577664915776,
-208.226946403507));
#209690=CARTESIAN_POINT('Ctrl Pts',(56.5087297972239,-65.4389829337676,
-208.237237256758));
#209691=CARTESIAN_POINT('Ctrl Pts',(56.5049328760549,-65.4429598777431,
-208.241599714584));
#209692=CARTESIAN_POINT('Ctrl Pts',(56.5012774655679,-65.4470659442998,
-208.245963459985));
#209693=CARTESIAN_POINT('Ctrl Pts',(56.5138509238801,-65.4331773923495,
-208.248518783163));
#209694=CARTESIAN_POINT('Ctrl Pts',(56.5094087292744,-65.4378503136699,
-208.25288112094));
#209695=CARTESIAN_POINT('Ctrl Pts',(56.5051439252244,-65.4426842233343,
-208.257244986379));
#209696=CARTESIAN_POINT('Ctrl Pts',(56.5273807159321,-65.4177153790657,
-208.283038207423));
#209697=CARTESIAN_POINT('Ctrl Pts',(56.5212265334526,-65.4242355589788,
-208.287400749103));
#209698=CARTESIAN_POINT('Ctrl Pts',(56.5153591918106,-65.4310145177164,
-208.291764410647));
#209699=CARTESIAN_POINT('Ctrl Pts',(56.5341593626729,-65.4097792264604,
-208.307533252362));
#209700=CARTESIAN_POINT('Ctrl Pts',(56.5271357114541,-65.4172387338904,
-208.311895535072));
#209701=CARTESIAN_POINT('Ctrl Pts',(56.5204776688227,-65.4250252363654,
-208.316259455579));
#209702=CARTESIAN_POINT('Ctrl Pts',(56.5525209588637,-65.3880602085305,
-208.38232400629));
#209703=CARTESIAN_POINT('Ctrl Pts',(56.5431294167638,-65.3980791094533,
-208.386688866059));
#209704=CARTESIAN_POINT('Ctrl Pts',(56.5343427956335,-65.4086346803882,
-208.391050209511));
#209705=CARTESIAN_POINT('Ctrl Pts',(56.5617269524415,-65.3767978707557,
-208.434001333226));
#209706=CARTESIAN_POINT('Ctrl Pts',(56.5511242891442,-65.3881281081246,
-208.438365624418));
#209707=CARTESIAN_POINT('Ctrl Pts',(56.5412952751588,-65.4001361493426,
-208.442727536444));
#209708=CARTESIAN_POINT('Ctrl Pts',(56.5863764886281,-65.3462052619613,
-208.588987026056));
#209709=CARTESIAN_POINT('Ctrl Pts',(56.5725061054701,-65.3610757695375,
-208.59336548035));
#209710=CARTESIAN_POINT('Ctrl Pts',(56.5599119337509,-65.3770518735271,
-208.597713229276));
#209711=CARTESIAN_POINT('Ctrl Pts',(56.5986098697023,-65.3302929526477,
-208.693634753733));
#209712=CARTESIAN_POINT('Ctrl Pts',(56.5830688742296,-65.3469778303877,
-208.698012046015));
#209713=CARTESIAN_POINT('Ctrl Pts',(56.5691529780988,-65.365046299052,-208.702360956951));
#209714=CARTESIAN_POINT('Ctrl Pts',(56.6315194173109,-65.2866023733443,
-209.008772950752));
#209715=CARTESIAN_POINT('Ctrl Pts',(56.6114339742289,-65.3082260137793,
-209.013214961635));
#209716=CARTESIAN_POINT('Ctrl Pts',(56.594014810857,-65.3320840644752,-209.017499153971));
#209717=CARTESIAN_POINT('Ctrl Pts',(56.6477298291647,-65.2635998038976,
-209.220340888184));
#209718=CARTESIAN_POINT('Ctrl Pts',(56.6253012100655,-65.2877789793426,
-209.224780476847));
#209719=CARTESIAN_POINT('Ctrl Pts',(56.6062646503943,-65.3147324550994,
-209.229067091402));
#209720=CARTESIAN_POINT('Ctrl Pts',(56.6909645146964,-65.2003964473429,
-209.855114420997));
#209721=CARTESIAN_POINT('Ctrl Pts',(56.6621798760702,-65.2315103701136,
-209.859829541482));
#209722=CARTESIAN_POINT('Ctrl Pts',(56.6389405444651,-65.2670590859439,
-209.863840624216));
#209723=CARTESIAN_POINT('Ctrl Pts',(56.7118396592687,-65.1667799745591,
-210.279514012908));
#209724=CARTESIAN_POINT('Ctrl Pts',(56.6797528213393,-65.2015162456806,
-210.284225552072));
#209725=CARTESIAN_POINT('Ctrl Pts',(56.6547249564177,-65.2417076178786,
-210.288240216126));
#209726=CARTESIAN_POINT('Ctrl Pts',(56.7669337250065,-65.0740063908786,
-211.553866504694));
#209727=CARTESIAN_POINT('Ctrl Pts',(56.7258904584642,-65.1185576981398,
-211.559720606721));
#209728=CARTESIAN_POINT('Ctrl Pts',(56.6963931899382,-65.1717493422662,
-211.562592707913));
#209729=CARTESIAN_POINT('Ctrl Pts',(56.7925037337705,-65.0241267882654,
-212.404990365038));
#209730=CARTESIAN_POINT('Ctrl Pts',(56.7467526277092,-65.0738827156515,
-212.410853939053));
#209731=CARTESIAN_POINT('Ctrl Pts',(56.7157486990471,-65.1341451836486,
-212.413730817787));
#209732=CARTESIAN_POINT('Ctrl Pts',(56.8144552965912,-64.9781464054152,
-213.256094899172));
#209733=CARTESIAN_POINT('Ctrl Pts',(56.7643939904929,-65.0327211703679,
-213.2603619646));
#209734=CARTESIAN_POINT('Ctrl Pts',(56.7323722878852,-65.0994854859681,
-213.264821102391));
#209735=CARTESIAN_POINT('',(56.4785498900846,-65.4721614184049,-208.210085312208));
#209736=CARTESIAN_POINT('',(56.478494115784,-65.4721095684411,-208.218811515426));
#209737=CARTESIAN_POINT('Origin',(56.8446958677552,-65.8125449908831,-208.218811515427));
#209738=CARTESIAN_POINT('Ctrl Pts',(56.7323722878852,-65.0994854859681,
-213.264821102391));
#209739=CARTESIAN_POINT('Ctrl Pts',(56.7280331299638,-65.1085325036252,
-213.0426659958));
#209740=CARTESIAN_POINT('Ctrl Pts',(56.7236600161187,-65.1174598023183,
-212.828408289229));
#209741=CARTESIAN_POINT('Ctrl Pts',(56.7192071520268,-65.1263191176805,
-212.621942418159));
#209742=CARTESIAN_POINT('Ctrl Pts',(56.7143712859647,-65.1359404449006,
-212.397717901465));
#209743=CARTESIAN_POINT('Ctrl Pts',(56.7094414942533,-65.1454814483888,
-212.182683232543));
#209744=CARTESIAN_POINT('Ctrl Pts',(56.7044007704901,-65.1549636966398,
-211.976689932902));
#209745=CARTESIAN_POINT('Ctrl Pts',(56.6990509914586,-65.16502731751,-211.758066836935));
#209746=CARTESIAN_POINT('Ctrl Pts',(56.6935766980629,-65.1750242887845,
-211.549627667317));
#209747=CARTESIAN_POINT('Ctrl Pts',(56.6879977785627,-65.1849372191661,
-211.351181755465));
#209748=CARTESIAN_POINT('Ctrl Pts',(56.6816574551575,-65.1962030537977,
-211.125652195569));
#209749=CARTESIAN_POINT('Ctrl Pts',(56.6751822988107,-65.207360021443,-210.913029724019));
#209750=CARTESIAN_POINT('Ctrl Pts',(56.6686464737588,-65.2183342962373,
-210.713019035319));
#209751=CARTESIAN_POINT('Ctrl Pts',(56.6645436973053,-65.2252232499444,
-210.587465009999));
#209752=CARTESIAN_POINT('Ctrl Pts',(56.6604331251529,-65.2320228858102,
-210.466880293573));
#209753=CARTESIAN_POINT('Ctrl Pts',(56.6562668550037,-65.2387859569443,
-210.351202386143));
#209754=CARTESIAN_POINT('Ctrl Pts',(56.6519002114437,-65.2458742925433,
-210.229961042825));
#209755=CARTESIAN_POINT('Ctrl Pts',(56.6474728117744,-65.2529220025824,
-210.114109749179));
#209756=CARTESIAN_POINT('Ctrl Pts',(56.6429718362471,-65.2599444300887,
-210.003567964623));
#209757=CARTESIAN_POINT('Ctrl Pts',(56.6379688409285,-65.2677501094857,
-209.880696816514));
#209758=CARTESIAN_POINT('Ctrl Pts',(56.6328751836196,-65.2755242926631,
-209.764385579971));
#209759=CARTESIAN_POINT('Ctrl Pts',(56.6277194341623,-65.2832385350797,
-209.654514291435));
#209760=CARTESIAN_POINT('Ctrl Pts',(56.624236911128,-65.2884492279441,-209.580300193892));
#209761=CARTESIAN_POINT('Ctrl Pts',(56.6207270390862,-65.2936315211658,
-209.509024134166));
#209762=CARTESIAN_POINT('Ctrl Pts',(56.617207440978,-65.2987671927539,-209.440647356452));
#209763=CARTESIAN_POINT('Ctrl Pts',(56.613775609728,-65.303774798084,-209.373975664024));
#209764=CARTESIAN_POINT('Ctrl Pts',(56.6103458753721,-65.3087263946004,
-209.310034156505));
#209765=CARTESIAN_POINT('Ctrl Pts',(56.6068764958621,-65.313666809265,-209.2488250452));
#209766=CARTESIAN_POINT('Ctrl Pts',(56.6032170825836,-65.3188778330151,
-209.184263231186));
#209767=CARTESIAN_POINT('Ctrl Pts',(56.5995139374616,-65.3240760159455,
-209.122741170297));
#209768=CARTESIAN_POINT('Ctrl Pts',(56.5957575695313,-65.329271895427,-209.064240357975));
#209769=CARTESIAN_POINT('Ctrl Pts',(56.5915999777325,-65.3350227553855,
-208.999490977178));
#209770=CARTESIAN_POINT('Ctrl Pts',(56.587377473491,-65.3407704865255,-208.938442616069));
#209771=CARTESIAN_POINT('Ctrl Pts',(56.5831193370057,-65.3464844948962,
-208.881047056792));
#209772=CARTESIAN_POINT('Ctrl Pts',(56.581245602093,-65.3489988663853,-208.855790923359));
#209773=CARTESIAN_POINT('Ctrl Pts',(56.5793654496022,-65.3515061949731,
-208.831241819825));
#209774=CARTESIAN_POINT('Ctrl Pts',(56.5774833115673,-65.3540018120632,
-208.807394533789));
#209775=CARTESIAN_POINT('Ctrl Pts',(56.5746535978651,-65.3577538651775,
-208.771541163416));
#209776=CARTESIAN_POINT('Ctrl Pts',(56.5718312042982,-65.3614666511509,
-208.737278831632));
#209777=CARTESIAN_POINT('Ctrl Pts',(56.5689753515512,-65.3651839879222,
-208.704609317259));
#209778=CARTESIAN_POINT('Ctrl Pts',(56.5659574293187,-65.3691122833498,
-208.670085809751));
#209779=CARTESIAN_POINT('Ctrl Pts',(56.5629025346554,-65.3730452421391,
-208.637340870275));
#209780=CARTESIAN_POINT('Ctrl Pts',(56.5598023265609,-65.3769921095606,
-208.606359994172));
#209781=CARTESIAN_POINT('Ctrl Pts',(56.5563780436769,-65.3813515558121,
-208.572140586786));
#209782=CARTESIAN_POINT('Ctrl Pts',(56.5528988257772,-65.3857275999304,
-208.540073180714));
#209783=CARTESIAN_POINT('Ctrl Pts',(56.5493950389307,-65.390088291123,-208.510120866391));
#209784=CARTESIAN_POINT('Ctrl Pts',(56.5487734136095,-65.3908619443679,
-208.504806868186));
#209785=CARTESIAN_POINT('Ctrl Pts',(56.5481511020616,-65.3916350213848,
-208.499559408636));
#209786=CARTESIAN_POINT('Ctrl Pts',(56.5475283779876,-65.3924072326121,
-208.494378238166));
#209787=CARTESIAN_POINT('Ctrl Pts',(56.5453287383415,-65.3951349036653,
-208.476076861271));
#209788=CARTESIAN_POINT('Ctrl Pts',(56.5431272051926,-65.3978490668695,
-208.45856228272));
#209789=CARTESIAN_POINT('Ctrl Pts',(56.5408939522005,-65.4005806848653,
-208.441891167501));
#209790=CARTESIAN_POINT('Ctrl Pts',(56.5385406282808,-65.4034591684012,
-208.424323729171));
#209791=CARTESIAN_POINT('Ctrl Pts',(56.5361523910466,-65.4063567084215,
-208.407692546603));
#209792=CARTESIAN_POINT('Ctrl Pts',(56.5337249489466,-65.4092773915755,
-208.392024350581));
#209793=CARTESIAN_POINT('Ctrl Pts',(56.5310690780669,-65.4124729188087,
-208.374881735499));
#209794=CARTESIAN_POINT('Ctrl Pts',(56.5283665728401,-65.4156958368807,
-208.358891580038));
#209795=CARTESIAN_POINT('Ctrl Pts',(56.5256428710774,-65.4189189062079,
-208.344047558516));
#209796=CARTESIAN_POINT('Ctrl Pts',(56.5254666684109,-65.4191274141355,
-208.343087263886));
#209797=CARTESIAN_POINT('Ctrl Pts',(56.5252903858615,-65.4193359134402,
-208.342131753863));
#209798=CARTESIAN_POINT('Ctrl Pts',(56.5251140337793,-65.4195443931164,
-208.341181021962));
#209799=CARTESIAN_POINT('Ctrl Pts',(56.5232954613085,-65.4216942707653,
-208.331376913944));
#209800=CARTESIAN_POINT('Ctrl Pts',(56.5214784629796,-65.4238324204977,
-208.322080413569));
#209801=CARTESIAN_POINT('Ctrl Pts',(56.5196276349714,-65.4259963733911,
-208.313319636639));
#209802=CARTESIAN_POINT('Ctrl Pts',(56.5175968875829,-65.4283706846008,
-208.303707222741));
#209803=CARTESIAN_POINT('Ctrl Pts',(56.5155255808571,-65.4307758824906,
-208.294739604155));
#209804=CARTESIAN_POINT('Ctrl Pts',(56.5134060791767,-65.4332201265201,
-208.286419651956));
#209805=CARTESIAN_POINT('Ctrl Pts',(56.5118129578226,-65.4350573401415,
-208.280165968067));
#209806=CARTESIAN_POINT('Ctrl Pts',(56.5101935109831,-65.4369156575986,
-208.274277409077));
#209807=CARTESIAN_POINT('Ctrl Pts',(56.5085556806693,-65.438786705909,-208.268745398167));
#209808=CARTESIAN_POINT('Ctrl Pts',(56.507131055958,-65.4404141893159,-208.263933520294));
#209809=CARTESIAN_POINT('Ctrl Pts',(56.5056850988358,-65.442059709221,-208.259369841015));
#209810=CARTESIAN_POINT('Ctrl Pts',(56.504210950984,-65.4437291528628,-208.255130145768));
#209811=CARTESIAN_POINT('Ctrl Pts',(56.5026151415113,-65.4455363759132,
-208.250540547902));
#209812=CARTESIAN_POINT('Ctrl Pts',(56.5009863989148,-65.4473715290094,
-208.246330361089));
#209813=CARTESIAN_POINT('Ctrl Pts',(56.4993319052539,-65.4492261566959,
-208.242536805959));
#209814=CARTESIAN_POINT('Ctrl Pts',(56.4983885522403,-65.4502836213804,
-208.240373810869));
#209815=CARTESIAN_POINT('Ctrl Pts',(56.4974371021737,-65.4513471421316,
-208.238345233095));
#209816=CARTESIAN_POINT('Ctrl Pts',(56.4964806846606,-65.4524133534391,
-208.236451053781));
#209817=CARTESIAN_POINT('Ctrl Pts',(56.4952333113097,-65.4538039214214,
-208.233980638125));
#209818=CARTESIAN_POINT('Ctrl Pts',(56.493956861388,-65.4552217028158,-208.231715946767));
#209819=CARTESIAN_POINT('Ctrl Pts',(56.4926742013412,-65.4566408027887,
-208.229722706621));
#209820=CARTESIAN_POINT('Ctrl Pts',(56.4912629399021,-65.4582021838225,
-208.227529621271));
#209821=CARTESIAN_POINT('Ctrl Pts',(56.4898441983158,-65.4597651242878,
-208.225664960423));
#209822=CARTESIAN_POINT('Ctrl Pts',(56.4884441179479,-65.4613010606549,
-208.224151229051));
#209823=CARTESIAN_POINT('Ctrl Pts',(56.4869391839692,-65.4629520250432,
-208.222524132615));
#209824=CARTESIAN_POINT('Ctrl Pts',(56.4854558349875,-65.4645717792676,
-208.221301691147));
#209825=CARTESIAN_POINT('Ctrl Pts',(56.4840212932626,-65.4661317407865,
-208.220448513651));
#209826=CARTESIAN_POINT('Ctrl Pts',(56.4823555603527,-65.4679431061828,
-208.219457837807));
#209827=CARTESIAN_POINT('Ctrl Pts',(56.4807557628038,-65.469673732465,-208.218964148661));
#209828=CARTESIAN_POINT('Ctrl Pts',(56.4792563268586,-65.4712890580059,
-208.218842434544));
#209829=CARTESIAN_POINT('Ctrl Pts',(56.4789992766148,-65.4715659753529,
-208.218821568935));
#209830=CARTESIAN_POINT('Ctrl Pts',(56.4787451563535,-65.4718395275162,
-208.218811515426));
#209831=CARTESIAN_POINT('Ctrl Pts',(56.478494115784,-65.4721095684411,-208.218811515426));
#209832=CARTESIAN_POINT('Ctrl Pts',(56.4785498900846,-65.4721614184049,
-208.210085312209));
#209833=CARTESIAN_POINT('Ctrl Pts',(56.4880134607985,-65.4619815336005,
-208.210087283952));
#209834=CARTESIAN_POINT('Ctrl Pts',(56.4960210114868,-65.4531537245717,
-208.218228453105));
#209835=CARTESIAN_POINT('Ctrl Pts',(56.5023726430475,-65.4460714077127,
-208.227728741309));
#209836=CARTESIAN_POINT('Ctrl Pts',(56.5087366507261,-65.4389752909997,
-208.23724754077));
#209837=CARTESIAN_POINT('Ctrl Pts',(56.513854727351,-65.433173044492,-208.248528534057));
#209838=CARTESIAN_POINT('Ctrl Pts',(56.5183608448225,-65.4280233981992,
-208.260025266392));
#209839=CARTESIAN_POINT('Ctrl Pts',(56.527384064744,-65.4177115518456,-208.283046757708));
#209840=CARTESIAN_POINT('Ctrl Pts',(56.5341620389057,-65.4097760673606,
-208.307543894395));
#209841=CARTESIAN_POINT('Ctrl Pts',(56.5402792876314,-65.4025401997578,
-208.332463842479));
#209842=CARTESIAN_POINT('Ctrl Pts',(56.5525225633485,-65.3880580810659,
-208.382339498829));
#209843=CARTESIAN_POINT('Ctrl Pts',(56.5617281325892,-65.3767964110653,
-208.434008552021));
#209844=CARTESIAN_POINT('Ctrl Pts',(56.5699429720804,-65.3666008613971,
-208.485663414341));
#209845=CARTESIAN_POINT('Ctrl Pts',(56.5863768923929,-65.346204498088,-208.588999808438));
#209846=CARTESIAN_POINT('Ctrl Pts',(56.5986107835984,-65.3302917454577,
-208.693643261059));
#209847=CARTESIAN_POINT('Ctrl Pts',(56.6095793668545,-65.3157298046138,
-208.79868090921));
#209848=CARTESIAN_POINT('Ctrl Pts',(56.6315196526886,-65.2866017817001,
-209.008786076848));
#209849=CARTESIAN_POINT('Ctrl Pts',(56.6477302855814,-65.2635991432574,
-209.220347327344));
#209850=CARTESIAN_POINT('Ctrl Pts',(56.6621411615825,-65.2425322660162,
-209.431932106333));
#209851=CARTESIAN_POINT('Ctrl Pts',(56.6909646006573,-65.200396045247,-209.855126434415));
#209852=CARTESIAN_POINT('Ctrl Pts',(56.7118400320305,-65.1667793523224,
-210.279522418803));
#209853=CARTESIAN_POINT('Ctrl Pts',(56.7302042319515,-65.1358555723291,
-210.704298191088));
#209854=CARTESIAN_POINT('Ctrl Pts',(56.7669339286709,-65.0740058285095,
-211.553879733265));
#209855=CARTESIAN_POINT('Ctrl Pts',(56.7925011773325,-65.0241321427268,
-212.404891259688));
#209856=CARTESIAN_POINT('Ctrl Pts',(56.8144552965909,-64.9781464054155,
-213.256094899172));
#209857=CARTESIAN_POINT('Origin',(0.,-12.9675000200281,-208.218811515427));
#209858=CARTESIAN_POINT('Origin',(0.,-12.9675000200281,-208.218811515427));
#209859=CARTESIAN_POINT('Origin',(0.,-12.9675000200281,-208.210085312208));
#209860=CARTESIAN_POINT('Ctrl Pts',(56.7131249770401,39.136390603742,-213.924107582134));
#209861=CARTESIAN_POINT('Ctrl Pts',(56.6591708158967,39.1947585157316,-213.928380187744));
#209862=CARTESIAN_POINT('Ctrl Pts',(56.6260312186758,39.26699791474,-213.932877779247));
#209863=CARTESIAN_POINT('Ctrl Pts',(56.6878438485494,39.1909973438446,-212.873680972192));
#209864=CARTESIAN_POINT('Ctrl Pts',(56.6390541381501,39.2436411705138,-212.880445101553));
#209865=CARTESIAN_POINT('Ctrl Pts',(56.6069323298669,39.308101280162,-212.882516880404));
#209866=CARTESIAN_POINT('Ctrl Pts',(56.6594850052376,39.248900569515,-211.823591080281));
#209867=CARTESIAN_POINT('Ctrl Pts',(56.6161967667701,39.2955248737877,-211.830328584023));
#209868=CARTESIAN_POINT('Ctrl Pts',(56.5855128843193,39.3516918804354,-211.83240628728));
#209869=CARTESIAN_POINT('Ctrl Pts',(56.5961170971406,39.3557075607436,-210.338665903179));
#209870=CARTESIAN_POINT('Ctrl Pts',(56.5632284029528,39.3910644172893,-210.343434951173));
#209871=CARTESIAN_POINT('Ctrl Pts',(56.5376887518409,39.4321195627096,-210.347455422068));
#209872=CARTESIAN_POINT('Ctrl Pts',(56.5749226987295,39.3898533622913,-209.90220762928));
#209873=CARTESIAN_POINT('Ctrl Pts',(56.5454235880735,39.4215267027753,-209.906981158345));
#209874=CARTESIAN_POINT('Ctrl Pts',(56.5216963051399,39.4578331766847,-209.910997266658));
#209875=CARTESIAN_POINT('Ctrl Pts',(56.5309467959293,39.4540847109595,-209.24891615073));
#209876=CARTESIAN_POINT('Ctrl Pts',(56.5079716151444,39.4786993973283,-209.253391637796));
#209877=CARTESIAN_POINT('Ctrl Pts',(56.4885248990568,39.506210827646,-209.257701934938));
#209878=CARTESIAN_POINT('Ctrl Pts',(56.5144681134185,39.4774389991119,-209.031360415952));
#209879=CARTESIAN_POINT('Ctrl Pts',(56.4938957981811,39.4994537797928,-209.035838362477));
#209880=CARTESIAN_POINT('Ctrl Pts',(56.4760962345234,39.5238015154724,-209.040146260381));
#209881=CARTESIAN_POINT('Ctrl Pts',(56.4809774462897,39.5218092152179,-208.707139552256));
#209882=CARTESIAN_POINT('Ctrl Pts',(56.4650653119284,39.5387956857416,-208.711547487502));
#209883=CARTESIAN_POINT('Ctrl Pts',(56.4508419233835,39.557225742165,-208.715924510879));
#209884=CARTESIAN_POINT('Ctrl Pts',(56.4685043569935,39.5379957558533,-208.599289345334));
#209885=CARTESIAN_POINT('Ctrl Pts',(56.4543082678724,39.5531313413699,-208.603698519052));
#209886=CARTESIAN_POINT('Ctrl Pts',(56.4414369686318,39.5694195255203,-208.60807433386));
#209887=CARTESIAN_POINT('Ctrl Pts',(56.4433791076362,39.5690861270511,-208.439774659198));
#209888=CARTESIAN_POINT('Ctrl Pts',(56.4325361263003,39.5806119265652,-208.444168467643));
#209889=CARTESIAN_POINT('Ctrl Pts',(56.4224946430317,39.5928429539091,-208.448559464111));
#209890=CARTESIAN_POINT('Ctrl Pts',(56.434042377723,39.5804730986549,-208.386840352034));
#209891=CARTESIAN_POINT('Ctrl Pts',(56.4244358024192,39.5906684103489,-208.391234746251));
#209892=CARTESIAN_POINT('Ctrl Pts',(56.4154558353936,39.6014220979252,-208.395625171312));
#209893=CARTESIAN_POINT('Ctrl Pts',(56.4153197235611,39.602540640524,-208.309894071191));
#209894=CARTESIAN_POINT('Ctrl Pts',(56.4081423174308,39.6101253887744,-208.314285655015));
#209895=CARTESIAN_POINT('Ctrl Pts',(56.4013424744876,39.6180493256973,-208.318678862813));
#209896=CARTESIAN_POINT('Ctrl Pts',(56.4083623316493,39.6106555249509,-208.284557461711));
#209897=CARTESIAN_POINT('Ctrl Pts',(56.4020826208256,39.6172758938669,-208.288949312307));
#209898=CARTESIAN_POINT('Ctrl Pts',(56.3960980548982,39.6241637622927,-208.293342260033));
#209899=CARTESIAN_POINT('Ctrl Pts',(56.3945592936364,39.6263652686867,-208.249138326507));
#209900=CARTESIAN_POINT('Ctrl Pts',(56.3900359410543,39.6311005791763,-208.253529947332));
#209901=CARTESIAN_POINT('Ctrl Pts',(56.3856941549037,39.6360014284045,-208.257923126188));
#209902=CARTESIAN_POINT('Ctrl Pts',(56.3894732411015,39.6321076620074,-208.237848616086));
#209903=CARTESIAN_POINT('Ctrl Pts',(56.3855943263936,39.6361515194816,-208.24224035659));
#209904=CARTESIAN_POINT('Ctrl Pts',(56.3818606603298,39.6403285142035,-208.246633418771));
#209905=CARTESIAN_POINT('Ctrl Pts',(56.2937742808158,39.7383680155035,-208.093554903205));
#209906=CARTESIAN_POINT('Ctrl Pts',(56.3019347808255,39.7295012949887,-208.097988441706));
#209907=CARTESIAN_POINT('Ctrl Pts',(56.3097336024218,39.7204021456198,-208.102340277927));
#209908=CARTESIAN_POINT('Ctrl Pts',(55.901541357958,40.1547597432569,-208.230910731216));
#209909=CARTESIAN_POINT('Ctrl Pts',(55.957654116832,40.0945682331347,-208.235168290733));
#209910=CARTESIAN_POINT('Ctrl Pts',(56.0141418475234,40.0342093581467,-208.239693755738));
#209911=CARTESIAN_POINT('Ctrl Pts',(55.1111144719458,40.5151527971883,-226.746035420514));
#209912=CARTESIAN_POINT('Ctrl Pts',(55.1914520133701,40.4117219444719,-227.50020914733));
#209913=CARTESIAN_POINT('Ctrl Pts',(55.4188282852024,40.3069503931471,-226.764375983926));
#209914=CARTESIAN_POINT('',(56.699489854167,39.164766900886,-213.398999668926));
#209915=CARTESIAN_POINT('',(56.6162420139465,39.2878063792742,-213.407725872324));
#209916=CARTESIAN_POINT('Origin',(57.0675004159511,39.5031336989999,-213.407725872324));
#209917=CARTESIAN_POINT('',(56.3587426896623,39.6656306474361,-208.218811515434));
#209918=CARTESIAN_POINT('Ctrl Pts',(56.3587426896624,39.665630647436,-208.218811515434));
#209919=CARTESIAN_POINT('Ctrl Pts',(56.3601495832745,39.6641241675047,-208.218811515434));
#209920=CARTESIAN_POINT('Ctrl Pts',(56.3616493238422,39.6625121262006,-208.219123491817));
#209921=CARTESIAN_POINT('Ctrl Pts',(56.3632133291857,39.6608228164564,-208.219864826396));
#209922=CARTESIAN_POINT('Ctrl Pts',(56.3646224181208,39.6593008346561,-208.22053273099));
#209923=CARTESIAN_POINT('Ctrl Pts',(56.3660836031149,39.6577161880681,-208.221550081639));
#209924=CARTESIAN_POINT('Ctrl Pts',(56.3675724084783,39.6560941073193,-208.222966468907));
#209925=CARTESIAN_POINT('Ctrl Pts',(56.3689541239424,39.6545887029798,-208.224280975315));
#209926=CARTESIAN_POINT('Ctrl Pts',(56.3703595934114,39.6530510813804,-208.225939838963));
#209927=CARTESIAN_POINT('Ctrl Pts',(56.3717666744691,39.6515050309337,-208.227939015451));
#209928=CARTESIAN_POINT('Ctrl Pts',(56.3730638621233,39.6500797274366,-208.229782055725));
#209929=CARTESIAN_POINT('Ctrl Pts',(56.3743623913668,39.6486472843762,-208.231914630948));
#209930=CARTESIAN_POINT('Ctrl Pts',(56.3756430732668,39.6472291934253,-208.234288738312));
#209931=CARTESIAN_POINT('Ctrl Pts',(56.376094096522,39.6467297782334,-208.235124837918));
#209932=CARTESIAN_POINT('Ctrl Pts',(56.3765428903921,39.6462321689465,-208.235990441946));
#209933=CARTESIAN_POINT('Ctrl Pts',(56.3769885653368,39.6457373905793,-208.236881866521));
#209934=CARTESIAN_POINT('Ctrl Pts',(56.37881285369,39.6437121064042,-208.24053074894));
#209935=CARTESIAN_POINT('Ctrl Pts',(56.3806052038614,39.6417121634959,-208.244629681269));
#209936=CARTESIAN_POINT('Ctrl Pts',(56.3823572094279,39.6397463121279,-208.249191218014));
#209937=CARTESIAN_POINT('Ctrl Pts',(56.3839571735553,39.6379510600302,-208.253356898361));
#209938=CARTESIAN_POINT('Ctrl Pts',(56.3855233415072,39.6361843954567,-208.257908600676));
#209939=CARTESIAN_POINT('Ctrl Pts',(56.3870701495925,39.6344312926996,-208.262824066145));
#209940=CARTESIAN_POINT('Ctrl Pts',(56.3877712828556,39.6336366507085,-208.265052135921));
#209941=CARTESIAN_POINT('Ctrl Pts',(56.388468749925,39.6328444709097,-208.267354469389));
#209942=CARTESIAN_POINT('Ctrl Pts',(56.3891656252778,39.6320515532012,-208.269726355525));
#209943=CARTESIAN_POINT('Ctrl Pts',(56.3913816577841,39.6295301102924,-208.277268847532));
#209944=CARTESIAN_POINT('Ctrl Pts',(56.3935673157433,39.6270280076159,-208.285480742852));
#209945=CARTESIAN_POINT('Ctrl Pts',(56.3957051192765,39.6245637499415,-208.294372756304));
#209946=CARTESIAN_POINT('Ctrl Pts',(56.3976391821956,39.6223343451728,-208.302417327858));
#209947=CARTESIAN_POINT('Ctrl Pts',(56.3995339263727,39.6201360741756,-208.311018721799));
#209948=CARTESIAN_POINT('Ctrl Pts',(56.4013976801705,39.6179604017859,-208.320157411357));
#209949=CARTESIAN_POINT('Ctrl Pts',(56.4029651061584,39.6161306507486,-208.327843093621));
#209950=CARTESIAN_POINT('Ctrl Pts',(56.4045108040343,39.6143166839342,-208.335908542756));
#209951=CARTESIAN_POINT('Ctrl Pts',(56.4060546455774,39.6124978246064,-208.344323125453));
#209952=CARTESIAN_POINT('Ctrl Pts',(56.4088227595351,39.6092366026791,-208.35941050532));
#209953=CARTESIAN_POINT('Ctrl Pts',(56.4115687404984,39.6059763732055,-208.375650545353));
#209954=CARTESIAN_POINT('Ctrl Pts',(56.414266332437,39.6027448960211,-208.393061304987));
#209955=CARTESIAN_POINT('Ctrl Pts',(56.4167639475216,39.5997529734676,-208.409181376846));
#209956=CARTESIAN_POINT('Ctrl Pts',(56.4192197492829,39.5967860493275,-208.426305292677));
#209957=CARTESIAN_POINT('Ctrl Pts',(56.4216387710761,39.5938389153697,-208.444423890791));
#209958=CARTESIAN_POINT('Ctrl Pts',(56.4239005683569,39.5910833306161,-208.461364869191));
#209959=CARTESIAN_POINT('Ctrl Pts',(56.4261299837435,39.5883452872419,-208.479175614652));
#209960=CARTESIAN_POINT('Ctrl Pts',(56.4283584828494,39.5855917216612,-208.49782421793));
#209961=CARTESIAN_POINT('Ctrl Pts',(56.4285133927028,39.585400312816,-208.499120539922));
#209962=CARTESIAN_POINT('Ctrl Pts',(56.428668310598,39.5852088158322,-208.500420899441));
#209963=CARTESIAN_POINT('Ctrl Pts',(56.4288232528699,39.5850172135307,-208.501725280663));
#209964=CARTESIAN_POINT('Ctrl Pts',(56.432293438562,39.580725966494,-208.530939032316));
#209965=CARTESIAN_POINT('Ctrl Pts',(56.4357490676031,39.5764097172179,-208.562213621881));
#209966=CARTESIAN_POINT('Ctrl Pts',(56.4391551317323,39.5721053282918,-208.595581146484));
#209967=CARTESIAN_POINT('Ctrl Pts',(56.4423216937235,39.5681036084618,-208.626602387169));
#209968=CARTESIAN_POINT('Ctrl Pts',(56.4454450058205,39.5641125747319,-208.659432798495));
#209969=CARTESIAN_POINT('Ctrl Pts',(56.4485249814543,39.5601321607569,-208.694080862067));
#209970=CARTESIAN_POINT('Ctrl Pts',(56.451369297175,39.5564563024417,-208.726077878807));
#209971=CARTESIAN_POINT('Ctrl Pts',(56.4541764558065,39.5527897115675,-208.759625141864));
#209972=CARTESIAN_POINT('Ctrl Pts',(56.4569751886937,39.5491018419698,-208.794711891478));
#209973=CARTESIAN_POINT('Ctrl Pts',(56.4577444522914,39.5480881890244,-208.804355884073));
#209974=CARTESIAN_POINT('Ctrl Pts',(56.4585132677862,39.5470727289412,-208.814116069679));
#209975=CARTESIAN_POINT('Ctrl Pts',(56.4592826862095,39.5460543462138,-208.823991952248));
#209976=CARTESIAN_POINT('Ctrl Pts',(56.4635914453566,39.5403513817942,-208.879297099709));
#209977=CARTESIAN_POINT('Ctrl Pts',(56.4678871861578,39.5345902747531,-208.938264807565));
#209978=CARTESIAN_POINT('Ctrl Pts',(56.4721263985457,39.5288164538003,-209.000955538769));
#209979=CARTESIAN_POINT('Ctrl Pts',(56.4760642649888,39.523453066997,-209.059189876687));
#209980=CARTESIAN_POINT('Ctrl Pts',(56.4799529250891,39.5180791658712,-209.120636905201));
#209981=CARTESIAN_POINT('Ctrl Pts',(56.4837859987149,39.5127008938574,-209.185332844094));
#209982=CARTESIAN_POINT('Ctrl Pts',(56.4873081739301,39.5077588504122,-209.244781332365));
#209983=CARTESIAN_POINT('Ctrl Pts',(56.4907832286359,39.5028133138086,-209.306973134386));
#209984=CARTESIAN_POINT('Ctrl Pts',(56.4942351443273,39.4978383106628,-209.37192419101));
#209985=CARTESIAN_POINT('Ctrl Pts',(56.4960297197263,39.4952519154396,-209.405690823447));
#209986=CARTESIAN_POINT('Ctrl Pts',(56.4978185487061,39.4926570170179,-209.440202996464));
#209987=CARTESIAN_POINT('Ctrl Pts',(56.4996087590354,39.4900459724346,-209.475461388355));
#209988=CARTESIAN_POINT('Ctrl Pts',(56.5048651761802,39.4823794210307,-209.578987109661));
#209989=CARTESIAN_POINT('Ctrl Pts',(56.5100972729331,39.4746123732906,-209.688950789672));
#209990=CARTESIAN_POINT('Ctrl Pts',(56.5152526591312,39.4667985899322,-209.805474420592));
#209991=CARTESIAN_POINT('Ctrl Pts',(56.5200402606557,39.4595422410028,-209.913685268741));
#209992=CARTESIAN_POINT('Ctrl Pts',(56.5247612649405,39.4522460582652,-210.02755354853));
#209993=CARTESIAN_POINT('Ctrl Pts',(56.5294024349243,39.4449224211257,-210.147172612983));
#209994=CARTESIAN_POINT('Ctrl Pts',(56.5336452006572,39.4382274548126,-210.256523416644));
#209995=CARTESIAN_POINT('Ctrl Pts',(56.5378210834422,39.431509723132,-210.370680096185));
#209996=CARTESIAN_POINT('Ctrl Pts',(56.5419487316549,39.4247479639329,-210.489709612087));
#209997=CARTESIAN_POINT('Ctrl Pts',(56.5452447224076,39.4193485949355,-210.584756516158));
#209998=CARTESIAN_POINT('Ctrl Pts',(56.5485103637142,39.4139207189296,-210.682910410159));
#209999=CARTESIAN_POINT('Ctrl Pts',(56.5517715302822,39.4084360149103,-210.784202905567));
#210000=CARTESIAN_POINT('Ctrl Pts',(56.5579467539937,39.398050383387,-210.97600660722));
#210001=CARTESIAN_POINT('Ctrl Pts',(56.5640670191006,39.3875025211926,-211.179071278287));
#210002=CARTESIAN_POINT('Ctrl Pts',(56.5700699283836,39.3768543172624,-211.393646924193));
#210003=CARTESIAN_POINT('Ctrl Pts',(56.5756452528862,39.3669645805561,-211.592938434341));
#210004=CARTESIAN_POINT('Ctrl Pts',(56.5811189037804,39.3569887584367,-211.802159549538));
#210005=CARTESIAN_POINT('Ctrl Pts',(56.5864687201405,39.3469466599906,-212.021505773689));
#210006=CARTESIAN_POINT('Ctrl Pts',(56.5916371677434,39.3372450074199,-212.233415751551));
#210007=CARTESIAN_POINT('Ctrl Pts',(56.5966894928584,39.3274820752966,-212.454776044889));
#210008=CARTESIAN_POINT('Ctrl Pts',(56.6016398763514,39.3176391858333,-212.685757113719));
#210009=CARTESIAN_POINT('Ctrl Pts',(56.6061501516399,39.3086713672439,-212.896203073781));
#210010=CARTESIAN_POINT('Ctrl Pts',(56.6105757435957,39.2996372422124,-213.114635211445));
#210011=CARTESIAN_POINT('Ctrl Pts',(56.614959710428,39.290488109814,-213.341176963337));
#210012=CARTESIAN_POINT('Ctrl Pts',(56.6153874935782,39.289595346518,-213.363282683563));
#210013=CARTESIAN_POINT('Ctrl Pts',(56.6158149084831,39.2887014581205,-213.385465616055));
#210014=CARTESIAN_POINT('Ctrl Pts',(56.6162420139465,39.2878063792742,-213.407725872324));
#210015=CARTESIAN_POINT('',(56.3587983457046,39.6656826243185,-208.210085312216));
#210016=CARTESIAN_POINT('Origin',(56.7241679835722,40.0068993898824,-208.218811515434));
#210017=CARTESIAN_POINT('Ctrl Pts',(56.6994898617306,39.1647669078403,-213.398999669105));
#210018=CARTESIAN_POINT('Ctrl Pts',(56.6773193211235,39.2114480278548,-212.523894235562));
#210019=CARTESIAN_POINT('Ctrl Pts',(56.651479770637,39.2620537363991,-211.649203631226));
#210020=CARTESIAN_POINT('Ctrl Pts',(56.5956975036787,39.3561498317412,-210.339090933364));
#210021=CARTESIAN_POINT('Ctrl Pts',(56.5745517354038,39.3902416134919,-209.902674994602));
#210022=CARTESIAN_POINT('Ctrl Pts',(56.5306742644768,39.4543652326716,-209.24942443662));
#210023=CARTESIAN_POINT('Ctrl Pts',(56.5142321837007,39.4776795989311,-209.03188052566));
#210024=CARTESIAN_POINT('Ctrl Pts',(56.480816494081,39.5219692158454,-208.70764780547));
#210025=CARTESIAN_POINT('Ctrl Pts',(56.4683713984661,39.5381257486172,-208.599790912822));
#210026=CARTESIAN_POINT('Ctrl Pts',(56.4433041343981,39.569154837062,-208.440233728844));
#210027=CARTESIAN_POINT('Ctrl Pts',(56.4339894177057,39.5805185781009,-208.387282545977));
#210028=CARTESIAN_POINT('Ctrl Pts',(56.4153107858428,39.6025404853857,-208.310273287259));
#210029=CARTESIAN_POINT('Ctrl Pts',(56.4083698728123,39.6106383616431,-208.284910555051));
#210030=CARTESIAN_POINT('Ctrl Pts',(56.394596442102,39.6263182576719,-208.249418094709));
#210031=CARTESIAN_POINT('Ctrl Pts',(56.3895186643059,39.6320526747255,-208.238093899573));
#210032=CARTESIAN_POINT('Ctrl Pts',(56.3765990499463,39.6464010040802,-208.218501926116));
#210033=CARTESIAN_POINT('Ctrl Pts',(56.3682899804801,39.6555191285273,-208.210085312216));
#210034=CARTESIAN_POINT('Ctrl Pts',(56.3587983457046,39.6656826243185,-208.210085312216));
#210035=CARTESIAN_POINT('Origin',(0.,-12.9675000200281,-208.218811515434));
#210036=CARTESIAN_POINT('',(52.2148720050704,43.7789665035542,-208.218811515434));
#210037=CARTESIAN_POINT('',(52.2149235689092,43.779022542486,-208.210085312216));
#210038=CARTESIAN_POINT('Origin',(52.5534287939255,44.1469057658247,-208.218811515435));
#210039=CARTESIAN_POINT('Origin',(0.,-12.9675000200281,-208.210085312216));
#210040=CARTESIAN_POINT('Origin',(0.,-12.9675000200281,-208.218811515434));
#210041=CARTESIAN_POINT('Ctrl Pts',(56.6214560695998,39.2782015364689,-213.075568750364));
#210042=CARTESIAN_POINT('Ctrl Pts',(56.654483236613,39.2080032797481,-213.086332264511));
#210043=CARTESIAN_POINT('Ctrl Pts',(56.7071198771834,39.1517102271814,-213.09704916438));
#210044=CARTESIAN_POINT('Ctrl Pts',(56.6004809601567,39.3177369985946,-213.475440414112));
#210045=CARTESIAN_POINT('Ctrl Pts',(56.6315613449632,39.2557964829605,-213.467329046301));
#210046=CARTESIAN_POINT('Ctrl Pts',(56.6782189205445,39.2033836493307,-213.460581076327));
#210047=CARTESIAN_POINT('Ctrl Pts',(56.6372034409747,39.2511121778754,-213.828824822694));
#210048=CARTESIAN_POINT('Ctrl Pts',(56.6720387769172,39.1751400320608,-213.807827408045));
#210049=CARTESIAN_POINT('Ctrl Pts',(56.7283118338796,39.116606690349,-213.781595977465));
#210050=CARTESIAN_POINT('Ctrl Pts',(56.6987085996655,39.0810160666721,-214.413338469428));
#210051=CARTESIAN_POINT('Ctrl Pts',(56.7321412993442,38.9737779499193,-214.361684674043));
#210052=CARTESIAN_POINT('Ctrl Pts',(56.8155652495982,38.8966330687837,-214.312698211001));
#210053=CARTESIAN_POINT('Ctrl Pts',(56.7239630070022,38.9928957520747,-214.64988909805));
#210054=CARTESIAN_POINT('Ctrl Pts',(56.7546676004383,38.8685060470322,-214.586687956946));
#210055=CARTESIAN_POINT('Ctrl Pts',(56.8524370552797,38.7830099878374,-214.527620279871));
#210056=CARTESIAN_POINT('Ctrl Pts',(56.7797859812607,38.6711930024679,-215.430608964657));
#210057=CARTESIAN_POINT('Ctrl Pts',(56.7896319635179,38.4831137119568,-215.334185599672));
#210058=CARTESIAN_POINT('Ctrl Pts',(56.9411099182686,38.3701449194622,-215.236934347207));
#210059=CARTESIAN_POINT('Ctrl Pts',(56.7727925783854,38.4015216091642,-215.952884479091));
#210060=CARTESIAN_POINT('Ctrl Pts',(56.7377496633354,38.1576856081976,-215.83078434059));
#210061=CARTESIAN_POINT('Ctrl Pts',(56.9475441086433,38.0266995615636,-215.711762130513));
#210062=CARTESIAN_POINT('Ctrl Pts',(56.6685131435906,38.118834322735,-216.461270781929));
#210063=CARTESIAN_POINT('Ctrl Pts',(56.576365951004,37.8732757014601,-216.253572790495));
#210064=CARTESIAN_POINT('Ctrl Pts',(56.8319648105423,37.6721636895405,-216.173673746282));
#210065=CARTESIAN_POINT('',(56.8784089882814,37.8494074227593,-215.942195856527));
#210066=CARTESIAN_POINT('',(56.7127812850717,38.2589564044561,-216.205851068199));
#210067=CARTESIAN_POINT('Origin',(57.1962194441171,38.1313337325768,-216.205851068199));
#210068=CARTESIAN_POINT('Ctrl Pts',(56.6162420139465,39.2878063792742,-213.407725872324));
#210069=CARTESIAN_POINT('Ctrl Pts',(56.6165277343106,39.2872075991701,-213.422617255017));
#210070=CARTESIAN_POINT('Ctrl Pts',(56.6168832113971,39.2864637908029,-213.437594243781));
#210071=CARTESIAN_POINT('Ctrl Pts',(56.6173071902525,39.2855743587294,-213.452656838247));
#210072=CARTESIAN_POINT('Ctrl Pts',(56.6185791268188,39.282906062509,-213.497844621643));
#210073=CARTESIAN_POINT('Ctrl Pts',(56.6204684474054,39.2789275478084,-213.543802858157));
#210074=CARTESIAN_POINT('Ctrl Pts',(56.6229334705114,39.2736193407654,-213.590531548545));
#210075=CARTESIAN_POINT('Ctrl Pts',(56.6245768192488,39.27008053607,-213.621684008803));
#210076=CARTESIAN_POINT('Ctrl Pts',(56.626475810809,39.2659506824126,-213.653178892369));
#210077=CARTESIAN_POINT('Ctrl Pts',(56.6286148188683,39.2612228888315,-213.68501619841));
#210078=CARTESIAN_POINT('Ctrl Pts',(56.6296843228979,39.258858992041,-213.700934851431));
#210079=CARTESIAN_POINT('Ctrl Pts',(56.6308137885021,39.2563455917412,-213.716939110088));
#210080=CARTESIAN_POINT('Ctrl Pts',(56.6320009587241,39.2536817324465,-213.733028974519));
#210081=CARTESIAN_POINT('Ctrl Pts',(56.6325945438351,39.2523498027992,-213.741073906734));
#210082=CARTESIAN_POINT('Ctrl Pts',(56.6332025518579,39.2509802568528,-213.749140240395));
#210083=CARTESIAN_POINT('Ctrl Pts',(56.6338246786909,39.2495729676807,-213.757227975525));
#210084=CARTESIAN_POINT('Ctrl Pts',(56.6343290486238,39.2484320518617,-213.763784854618));
#210085=CARTESIAN_POINT('Ctrl Pts',(56.6349037212799,39.2471275146199,-213.771128572755));
#210086=CARTESIAN_POINT('Ctrl Pts',(56.6354002884089,39.2459963926713,-213.777379412664));
#210087=CARTESIAN_POINT('Ctrl Pts',(56.6355162235629,39.2457323059252,-213.778838816731));
#210088=CARTESIAN_POINT('Ctrl Pts',(56.6356278283714,39.2454778780714,-213.780238734505));
#210089=CARTESIAN_POINT('Ctrl Pts',(56.6357330959044,39.2452377374264,-213.781555385346));
#210090=CARTESIAN_POINT('Ctrl Pts',(56.636845383284,39.2427003415081,-213.795467501181));
#210091=CARTESIAN_POINT('Ctrl Pts',(56.6380061653357,39.2400336252933,-213.809533615601));
#210092=CARTESIAN_POINT('Ctrl Pts',(56.6392133653724,39.2372367967664,-213.823753728813));
#210093=CARTESIAN_POINT('Ctrl Pts',(56.6424287823681,39.2297873520133,-213.861629467972));
#210094=CARTESIAN_POINT('Ctrl Pts',(56.6459740125889,39.2214162094164,-213.900598182719));
#210095=CARTESIAN_POINT('Ctrl Pts',(56.6498032020704,39.2121020323048,-213.940658617166));
#210096=CARTESIAN_POINT('Ctrl Pts',(56.6502869191469,39.2109254317358,-213.945719196259));
#210097=CARTESIAN_POINT('Ctrl Pts',(56.6507751265893,39.2097338312328,-213.950797222392));
#210098=CARTESIAN_POINT('Ctrl Pts',(56.6512676955233,39.2085272315157,-213.955892716039));
#210099=CARTESIAN_POINT('Ctrl Pts',(56.6541955830412,39.2013550612736,-213.986180927933));
#210100=CARTESIAN_POINT('Ctrl Pts',(56.6572790751068,39.1936506663972,-214.017085134124));
#210101=CARTESIAN_POINT('Ctrl Pts',(56.6604911051498,39.1854043760091,-214.048605333297));
#210102=CARTESIAN_POINT('Ctrl Pts',(56.6620971201713,39.181281230815,-214.064365432883));
#210103=CARTESIAN_POINT('Ctrl Pts',(56.6637351748836,39.1770225746252,-214.08027953076));
#210104=CARTESIAN_POINT('Ctrl Pts',(56.6654011751468,39.1726270545194,-214.096347627154));
#210105=CARTESIAN_POINT('Ctrl Pts',(56.6662341752783,39.1704292944666,-214.104381675351));
#210106=CARTESIAN_POINT('Ctrl Pts',(56.6670741539691,39.1681973156772,-214.112454223184));
#210107=CARTESIAN_POINT('Ctrl Pts',(56.6679205467032,39.1659309368603,-214.120565270699));
#210108=CARTESIAN_POINT('Ctrl Pts',(56.6686382008055,39.1640092804117,-214.127442605876));
#210109=CARTESIAN_POINT('Ctrl Pts',(56.6694887205913,39.1617155181499,-214.135571608633));
#210110=CARTESIAN_POINT('Ctrl Pts',(56.6701455208158,39.1599327774048,-214.141838684002));
#210111=CARTESIAN_POINT('Ctrl Pts',(56.6702633429838,39.1596129748655,-214.142962922971));
#210112=CARTESIAN_POINT('Ctrl Pts',(56.6703749277195,39.1593097487773,-214.14402729556));
#210113=CARTESIAN_POINT('Ctrl Pts',(56.6704783877725,39.159028345972,-214.145013884847));
#210114=CARTESIAN_POINT('Ctrl Pts',(56.6713398659602,39.156685196402,-214.153228892734));
#210115=CARTESIAN_POINT('Ctrl Pts',(56.6722080330432,39.1543049369045,-214.161487512375));
#210116=CARTESIAN_POINT('Ctrl Pts',(56.6730817428456,39.1518886370445,-214.169790761554));
#210117=CARTESIAN_POINT('Ctrl Pts',(56.6735877457118,39.1504892540327,-214.17459952972));
#210118=CARTESIAN_POINT('Ctrl Pts',(56.6740956287835,39.1490775454481,-214.179423011065));
#210119=CARTESIAN_POINT('Ctrl Pts',(56.6746052615809,39.1476536047955,-214.18426131276));
#210120=CARTESIAN_POINT('Ctrl Pts',(56.6796915033885,39.1334423795473,-214.232548574649));
#210121=CARTESIAN_POINT('Ctrl Pts',(56.684953508893,39.1180134548084,-214.282308281078));
#210122=CARTESIAN_POINT('Ctrl Pts',(56.6902997298246,39.1013256022754,-214.333539572759));
#210123=CARTESIAN_POINT('Ctrl Pts',(56.6951779830848,39.0860984779072,-214.380286465352));
#210124=CARTESIAN_POINT('Ctrl Pts',(56.7001262124787,39.0698230353042,-214.428258560292));
#210125=CARTESIAN_POINT('Ctrl Pts',(56.7050492608573,39.052496006805,-214.477456751543));
#210126=CARTESIAN_POINT('Ctrl Pts',(56.7101720338601,39.0344660328969,-214.52865087895));
#210127=CARTESIAN_POINT('Ctrl Pts',(56.7152706315545,39.0152903364839,-214.581171861781));
#210128=CARTESIAN_POINT('Ctrl Pts',(56.7202164165074,38.9949472473483,-214.635020459656));
#210129=CARTESIAN_POINT('Ctrl Pts',(56.720963128566,38.9918758582537,-214.643150493161));
#210130=CARTESIAN_POINT('Ctrl Pts',(56.7217062798833,38.9887779139132,-214.651310770207));
#210131=CARTESIAN_POINT('Ctrl Pts',(56.7224453422406,38.9856534013085,-214.659501272636));
#210132=CARTESIAN_POINT('Ctrl Pts',(56.7252624323166,38.9737436708722,-214.690721078222));
#210133=CARTESIAN_POINT('Ctrl Pts',(56.7280207596582,38.9614468560358,-214.722380406985));
#210134=CARTESIAN_POINT('Ctrl Pts',(56.7306885429869,38.9487598472382,-214.75447926351));
#210135=CARTESIAN_POINT('Ctrl Pts',(56.7320224346512,38.9424163428394,-214.770528691772));
#210136=CARTESIAN_POINT('Ctrl Pts',(56.7333336141141,38.9359752788485,-214.786688002162));
#210137=CARTESIAN_POINT('Ctrl Pts',(56.7346175684232,38.9294363703326,-214.802957195691));
#210138=CARTESIAN_POINT('Ctrl Pts',(56.7352595455777,38.9261669160747,-214.811091792455));
#210139=CARTESIAN_POINT('Ctrl Pts',(56.7358947107526,38.9228730002466,-214.819253860003));
#210140=CARTESIAN_POINT('Ctrl Pts',(56.7365224626186,38.919554591232,-214.827443398408));
#210141=CARTESIAN_POINT('Ctrl Pts',(56.7371502144845,38.9162361822173,-214.835632936812));
#210142=CARTESIAN_POINT('Ctrl Pts',(56.7378546750073,38.9124306555081,-214.844982606075));
#210143=CARTESIAN_POINT('Ctrl Pts',(56.7383831203994,38.9095243687999,-214.852093589858));
#210144=CARTESIAN_POINT('Ctrl Pts',(56.7390624730686,38.9057881386,-214.861235245527));
#210145=CARTESIAN_POINT('Ctrl Pts',(56.7397290362713,38.9020376117849,-214.870374141699));
#210146=CARTESIAN_POINT('Ctrl Pts',(56.7403822137486,38.8982733493814,-214.879510354443));
#210147=CARTESIAN_POINT('Ctrl Pts',(56.7470703821133,38.8597294289335,-214.973060011575));
#210148=CARTESIAN_POINT('Ctrl Pts',(56.7524888154197,38.8195967151214,-215.066647774888));
#210149=CARTESIAN_POINT('Ctrl Pts',(56.75629923383,38.7778906329865,-215.160439317411));
#210150=CARTESIAN_POINT('Ctrl Pts',(56.7567481817338,38.7729767741574,-215.171489945418));
#210151=CARTESIAN_POINT('Ctrl Pts',(56.7571747476926,38.7680410765947,-215.18254339977));
#210152=CARTESIAN_POINT('Ctrl Pts',(56.757578329166,38.7630835681807,-215.193599949725));
#210153=CARTESIAN_POINT('Ctrl Pts',(56.7606513461903,38.7253352849747,-215.277788567095));
#210154=CARTESIAN_POINT('Ctrl Pts',(56.7623974702021,38.686301527375,-215.362190731822));
#210155=CARTESIAN_POINT('Ctrl Pts',(56.762521509791,38.6459704543063,-215.447017807587));
#210156=CARTESIAN_POINT('Ctrl Pts',(56.7625655254613,38.6316589008054,-215.477118847326));
#210157=CARTESIAN_POINT('Ctrl Pts',(56.7624048272067,38.6171840356244,-215.507273405936));
#210158=CARTESIAN_POINT('Ctrl Pts',(56.7620246220546,38.6025455154463,-215.537491003004));
#210159=CARTESIAN_POINT('Ctrl Pts',(56.7607704964948,38.5542596302855,-215.637165246309));
#210160=CARTESIAN_POINT('Ctrl Pts',(56.7571502586175,38.5052402567317,-215.735351647595));
#210161=CARTESIAN_POINT('Ctrl Pts',(56.7509534925747,38.4557760674619,-215.832054892088));
#210162=CARTESIAN_POINT('Ctrl Pts',(56.7448960684165,38.4074241411545,-215.926583645525));
#210163=CARTESIAN_POINT('Ctrl Pts',(56.7363766210372,38.3586472645085,-216.019695331112));
#210164=CARTESIAN_POINT('Ctrl Pts',(56.7252464812199,38.3097021723518,-216.11138771604));
#210165=CARTESIAN_POINT('Ctrl Pts',(56.7214037584742,38.2928036947039,-216.143044857724));
#210166=CARTESIAN_POINT('Ctrl Pts',(56.7172502712356,38.2758850458335,-216.174532750333));
#210167=CARTESIAN_POINT('Ctrl Pts',(56.7127812850717,38.2589564044561,-216.205851068199));
#210168=CARTESIAN_POINT('Ctrl Pts',(56.8784089882814,37.8494074227593,-215.942195856527));
#210169=CARTESIAN_POINT('Ctrl Pts',(56.8923194163109,37.9131111636755,-215.85684824432));
#210170=CARTESIAN_POINT('Ctrl Pts',(56.9035288072913,37.9808416687619,-215.765163207208));
#210171=CARTESIAN_POINT('Ctrl Pts',(56.914779818816,38.0871684291001,-215.617449341681));
#210172=CARTESIAN_POINT('Ctrl Pts',(56.9190114191349,38.1415114743169,-215.541048698008));
#210173=CARTESIAN_POINT('Ctrl Pts',(56.9212013859612,38.2067058130031,-215.447397971083));
#210174=CARTESIAN_POINT('Ctrl Pts',(56.9215690259601,38.2397154101224,-215.399438830714));
#210175=CARTESIAN_POINT('Ctrl Pts',(56.9215656600791,38.257504698105,-215.373442266851));
#210176=CARTESIAN_POINT('Ctrl Pts',(56.9215088034732,38.265834430532,-215.361227686592));
#210177=CARTESIAN_POINT('Ctrl Pts',(56.9214626351149,38.2706010257896,-215.354227629012));
#210178=CARTESIAN_POINT('Ctrl Pts',(56.9214422193595,38.272460437043,-215.351495124754));
#210179=CARTESIAN_POINT('Ctrl Pts',(56.9210462352772,38.3066224801052,-215.301276190226));
#210180=CARTESIAN_POINT('Ctrl Pts',(56.9193511735892,38.3575254740986,-215.226640355385));
#210181=CARTESIAN_POINT('Ctrl Pts',(56.910501986457,38.4560022236843,-215.074830340481));
#210182=CARTESIAN_POINT('Ctrl Pts',(56.9064692885258,38.4924866873854,-215.017574749515));
#210183=CARTESIAN_POINT('Ctrl Pts',(56.897957870777,38.5519627451836,-214.921443048506));
#210184=CARTESIAN_POINT('Ctrl Pts',(56.8930834404498,38.5828852244691,-214.870815628649));
#210185=CARTESIAN_POINT('Ctrl Pts',(56.8860976844991,38.6208417602848,-214.807219480818));
#210186=CARTESIAN_POINT('Ctrl Pts',(56.8828002197628,38.6374891685479,-214.77898909186));
#210187=CARTESIAN_POINT('Ctrl Pts',(56.8805315935286,38.6486693924329,-214.759951795426));
#210188=CARTESIAN_POINT('Ctrl Pts',(56.8792297676071,38.6549228173467,-214.74925617217));
#210189=CARTESIAN_POINT('Ctrl Pts',(56.8609765545196,38.7407461211646,-214.601910135731));
#210190=CARTESIAN_POINT('Ctrl Pts',(56.8422826729904,38.806650416647,-214.478282783532));
#210191=CARTESIAN_POINT('Ctrl Pts',(56.816389824676,38.8870611879215,-214.317263299172));
#210192=CARTESIAN_POINT('Ctrl Pts',(56.8081057773634,38.9107819956799,-214.267642766951));
#210193=CARTESIAN_POINT('Ctrl Pts',(56.7966451030072,38.9421347884435,-214.199397507333));
#210194=CARTESIAN_POINT('Ctrl Pts',(56.7911549400794,38.956753098342,-214.166820249596));
#210195=CARTESIAN_POINT('Ctrl Pts',(56.7852548655275,38.9720320741206,-214.131532088428));
#210196=CARTESIAN_POINT('Ctrl Pts',(56.7824407647108,38.9792363102246,-214.114568907703));
#210197=CARTESIAN_POINT('Ctrl Pts',(56.7812648629523,38.9822314816374,-214.107445005404));
#210198=CARTESIAN_POINT('Ctrl Pts',(56.78048773646,38.9842078373838,-214.10272820146));
#210199=CARTESIAN_POINT('Ctrl Pts',(56.7804066536062,38.9844148179716,-214.102238950507));
#210200=CARTESIAN_POINT('Ctrl Pts',(56.7358311456287,39.0974359385773,-213.830613670394));
#210201=CARTESIAN_POINT('Ctrl Pts',(56.7051832112126,39.1534726566657,-213.596834029539));
#210202=CARTESIAN_POINT('Ctrl Pts',(56.6994898617306,39.1647669078403,-213.398999669105));
#210203=CARTESIAN_POINT('Ctrl Pts',(52.2149235689092,43.779022542486,-208.210085312216));
#210204=CARTESIAN_POINT('Ctrl Pts',(52.2148720050705,43.7789665035542,-208.214448081539));
#210205=CARTESIAN_POINT('Ctrl Pts',(52.2148720050704,43.7789665035542,-208.218811515435));
#210206=CARTESIAN_POINT('Ctrl Pts',(52.2043847769924,43.7887196915372,-208.210087338187));
#210207=CARTESIAN_POINT('Ctrl Pts',(52.2056250202409,43.7874750042174,-208.214450107462));
#210208=CARTESIAN_POINT('Ctrl Pts',(52.2069166839655,43.7862865377113,-208.21881354139));
#210209=CARTESIAN_POINT('Ctrl Pts',(52.195333723769,43.7968389605576,-208.218672616477));
#210210=CARTESIAN_POINT('Ctrl Pts',(52.1976712649932,43.7945859134348,-208.223035434656));
#210211=CARTESIAN_POINT('Ctrl Pts',(52.2000848734438,43.7924159898367,-208.227398819688));
#210212=CARTESIAN_POINT('Ctrl Pts',(52.1808472399183,43.8096868118422,-208.238463951946));
#210213=CARTESIAN_POINT('Ctrl Pts',(52.1849330344943,43.8058281558383,-208.242826402981));
#210214=CARTESIAN_POINT('Ctrl Pts',(52.1891506941446,43.8021155648562,-208.247190155172));
#210215=CARTESIAN_POINT('Ctrl Pts',(52.1749286143212,43.8148481482676,-208.250157029773));
#210216=CARTESIAN_POINT('Ctrl Pts',(52.1797237791601,43.8103385591305,-208.254519356384));
#210217=CARTESIAN_POINT('Ctrl Pts',(52.1846836299068,43.8060124062017,-208.258883232989));
#210218=CARTESIAN_POINT('Ctrl Pts',(52.1591833603872,43.828467493664,-208.285836176959));
#210219=CARTESIAN_POINT('Ctrl Pts',(52.1658591933782,43.8222328676652,-208.290198743649));
#210220=CARTESIAN_POINT('Ctrl Pts',(52.1728001724479,43.8162953562062,-208.294562380182));
#210221=CARTESIAN_POINT('Ctrl Pts',(52.1510964156406,43.8352931366209,-208.311120909483));
#210222=CARTESIAN_POINT('Ctrl Pts',(52.1587292093287,43.8281818395797,-208.315483211337));
#210223=CARTESIAN_POINT('Ctrl Pts',(52.1666971009815,43.8214493653102,-208.3198471127));
#210224=CARTESIAN_POINT('Ctrl Pts',(52.1289643871997,43.8537790486242,-208.388298939608));
#210225=CARTESIAN_POINT('Ctrl Pts',(52.1392045981911,43.8442802812313,-208.392664031458));
#210226=CARTESIAN_POINT('Ctrl Pts',(52.1499948920096,43.8354085050508,-208.397025142829));
#210227=CARTESIAN_POINT('Ctrl Pts',(52.1174992362576,43.8630330920583,-208.441520592514));
#210228=CARTESIAN_POINT('Ctrl Pts',(52.1290740876191,43.852314411835,-208.445885091517));
#210229=CARTESIAN_POINT('Ctrl Pts',(52.141343336723,43.8423973674724,-208.450246795732));
#210230=CARTESIAN_POINT('Ctrl Pts',(52.0863347270061,43.8878226116337,-208.601175288826));
#210231=CARTESIAN_POINT('Ctrl Pts',(52.1015151102266,43.8738103589885,-208.605554907233));
#210232=CARTESIAN_POINT('Ctrl Pts',(52.1178275724807,43.8611200325978,-208.609901492046));
#210233=CARTESIAN_POINT('Ctrl Pts',(52.0701168476483,43.9001220002185,-208.708951634353));
#210234=CARTESIAN_POINT('Ctrl Pts',(52.0871460895594,43.884425032588,-208.713330067135));
#210235=CARTESIAN_POINT('Ctrl Pts',(52.1055914799472,43.8704111305645,-208.717677837571));
#210236=CARTESIAN_POINT('Ctrl Pts',(52.0255864626054,43.9331969723227,-209.0334926008));
#210237=CARTESIAN_POINT('Ctrl Pts',(52.0476481597434,43.9129173610403,-209.037939859074));
#210238=CARTESIAN_POINT('Ctrl Pts',(52.071995743712,43.8953985191085,-209.042218804019));
#210239=CARTESIAN_POINT('Ctrl Pts',(52.0021445297993,43.949466653783,-209.251266491716));
#210240=CARTESIAN_POINT('Ctrl Pts',(52.0268103251713,43.9268242456044,-209.255711234979));
#210241=CARTESIAN_POINT('Ctrl Pts',(52.0543127614129,43.9076935513658,-209.259992694935));
#210242=CARTESIAN_POINT('Ctrl Pts',(51.937720029348,43.9928431481926,-209.90473928415));
#210243=CARTESIAN_POINT('Ctrl Pts',(51.9694532568106,43.9637905045621,-209.909476451697));
#210244=CARTESIAN_POINT('Ctrl Pts',(52.0057184578615,43.940477854794,-209.913465487369));
#210245=CARTESIAN_POINT('Ctrl Pts',(51.9034482509577,44.0137474304281,-210.34162185738));
#210246=CARTESIAN_POINT('Ctrl Pts',(51.9388750336111,43.9813630646936,-210.346355470779));
#210247=CARTESIAN_POINT('Ctrl Pts',(51.9798728970522,43.9562851731636,-210.350348060599));
#210248=CARTESIAN_POINT('Ctrl Pts',(51.8088683580654,44.0688586918087,-211.653440509504));
#210249=CARTESIAN_POINT('Ctrl Pts',(51.8543012271538,44.0274385666118,-211.659386088869));
#210250=CARTESIAN_POINT('Ctrl Pts',(51.9085528218201,43.9979691256788,-211.662166712722));
#210251=CARTESIAN_POINT('Ctrl Pts',(51.7580215322863,44.0943375071556,-212.529490943221));
#210252=CARTESIAN_POINT('Ctrl Pts',(51.8087639397327,44.0481656078252,-212.535446734955));
#210253=CARTESIAN_POINT('Ctrl Pts',(51.870219684202,44.0172576131423,-212.538231376868));
#210254=CARTESIAN_POINT('Ctrl Pts',(51.7111509881033,44.1161634878026,-213.405556127478));
#210255=CARTESIAN_POINT('Ctrl Pts',(51.7668122505506,44.0656404359961,-213.409820292477));
#210256=CARTESIAN_POINT('Ctrl Pts',(51.8348891643276,44.0337882456516,-213.414282330697));
#210257=CARTESIAN_POINT('',(51.8348891643276,44.0337882456516,-213.414282330697));
#210258=CARTESIAN_POINT('',(51.7111509810702,44.1161634800382,-213.405556127296));
#210259=CARTESIAN_POINT('Origin',(52.0467850062684,44.4866680886213,-213.414282330697));
#210260=CARTESIAN_POINT('Ctrl Pts',(52.2149235689092,43.779022542486,-208.210085312216));
#210261=CARTESIAN_POINT('Ctrl Pts',(52.2043801934833,43.7887239088728,-208.210087344463));
#210262=CARTESIAN_POINT('Ctrl Pts',(52.1953274288659,43.796844542981,-208.218681234754));
#210263=CARTESIAN_POINT('Ctrl Pts',(52.1880904910527,43.8032628774376,-208.228568296719));
#210264=CARTESIAN_POINT('Ctrl Pts',(52.1808394389761,43.8096937296283,-208.238474641509));
#210265=CARTESIAN_POINT('Ctrl Pts',(52.1749242234792,43.8148519452172,-208.250167023561));
#210266=CARTESIAN_POINT('Ctrl Pts',(52.1696802065441,43.8193879205004,-208.262050087041));
#210267=CARTESIAN_POINT('Ctrl Pts',(52.1591795680454,43.8284707738317,-208.28584477638));
#210268=CARTESIAN_POINT('Ctrl Pts',(52.1510932946611,43.8352957489707,-208.311131552955));
#210269=CARTESIAN_POINT('Ctrl Pts',(52.1437197227052,43.8414545028842,-208.336847252802));
#210270=CARTESIAN_POINT('Ctrl Pts',(52.1289623042575,43.8537805924866,-208.38831448545));
#210271=CARTESIAN_POINT('Ctrl Pts',(52.117497806034,43.8630342337481,-208.441527742187));
#210272=CARTESIAN_POINT('Ctrl Pts',(52.1071115904079,43.871295780733,-208.494739003265));
#210273=CARTESIAN_POINT('Ctrl Pts',(52.0863339472228,43.8878230204506,-208.601188227497));
#210274=CARTESIAN_POINT('Ctrl Pts',(52.0701156440688,43.9001228988017,-208.708960203697));
#210275=CARTESIAN_POINT('Ctrl Pts',(52.0552737632954,43.9111466435138,-208.817132044246));
#210276=CARTESIAN_POINT('Ctrl Pts',(52.0255859242023,43.9331971615186,-209.033505443658));
#210277=CARTESIAN_POINT('Ctrl Pts',(52.0021438786448,43.9494670967064,-209.251272899507));
#210278=CARTESIAN_POINT('Ctrl Pts',(51.980669942658,43.9639252593981,-209.469090795394));
#210279=CARTESIAN_POINT('Ctrl Pts',(51.9377196179987,43.9928432361475,-209.904751465645));
#210280=CARTESIAN_POINT('Ctrl Pts',(51.9034476265843,44.0137477974947,-210.34163037533));
#210281=CARTESIAN_POINT('Ctrl Pts',(51.8719217450993,44.032117736709,-210.778894755328));
#210282=CARTESIAN_POINT('Ctrl Pts',(51.8088678222893,44.0688588736632,-211.653453472328));
#210283=CARTESIAN_POINT('Ctrl Pts',(51.7580264403492,44.0943352215171,-212.529399211082));
#210284=CARTESIAN_POINT('Ctrl Pts',(51.7111509881036,44.1161634878024,-213.405556127478));
#210285=CARTESIAN_POINT('Ctrl Pts',(51.8348891643276,44.0337882456516,-213.414282330697));
#210286=CARTESIAN_POINT('Ctrl Pts',(51.8440852954194,44.0294855106755,-213.18625626589));
#210287=CARTESIAN_POINT('Ctrl Pts',(51.8531604919734,44.0251462166332,-212.96630637642));
#210288=CARTESIAN_POINT('Ctrl Pts',(51.8621671183822,44.0207245304424,-212.754324487476));
#210289=CARTESIAN_POINT('Ctrl Pts',(51.871945121168,44.0159241470436,-212.524187318841));
#210290=CARTESIAN_POINT('Ctrl Pts',(51.8816421638536,44.0110267854007,-212.303441420756));
#210291=CARTESIAN_POINT('Ctrl Pts',(51.8912802016416,44.0060153259421,-212.091936017557));
#210292=CARTESIAN_POINT('Ctrl Pts',(51.9015055904708,44.0006984634549,-211.867541277181));
#210293=CARTESIAN_POINT('Ctrl Pts',(51.9116640949647,43.9952536058705,-211.653547491765));
#210294=CARTESIAN_POINT('Ctrl Pts',(51.9217383966445,43.9897004291075,-211.449762344375));
#210295=CARTESIAN_POINT('Ctrl Pts',(51.933310516654,43.9833216219229,-211.215679004733));
#210296=CARTESIAN_POINT('Ctrl Pts',(51.9447712866266,43.976800121988,-210.995065528174));
#210297=CARTESIAN_POINT('Ctrl Pts',(51.9560438134912,43.9702123981561,-210.787615525048));
#210298=CARTESIAN_POINT('Ctrl Pts',(51.9630659686827,43.9661086138261,-210.658385749514));
#210299=CARTESIAN_POINT('Ctrl Pts',(51.9699973687366,43.9619953951688,-210.534265420326));
#210300=CARTESIAN_POINT('Ctrl Pts',(51.9768916294888,43.9578245559274,-210.415191219797));
#210301=CARTESIAN_POINT('Ctrl Pts',(51.9840937110015,43.953467493543,-210.290800494079));
#210302=CARTESIAN_POINT('Ctrl Pts',(51.9912547789145,43.9490479969219,-210.171916472859));
#210303=CARTESIAN_POINT('Ctrl Pts',(51.9983902835959,43.944553289385,-210.058458378852));
#210304=CARTESIAN_POINT('Ctrl Pts',(52.0063183623385,43.9395593335446,-209.932397960781));
#210305=CARTESIAN_POINT('Ctrl Pts',(52.0142146268005,43.9344727678281,-209.81303573055));
#210306=CARTESIAN_POINT('Ctrl Pts',(52.0220505221564,43.9293219842294,-209.700251538583));
#210307=CARTESIAN_POINT('Ctrl Pts',(52.0274154131935,43.9257954704734,-209.6230331898));
#210308=CARTESIAN_POINT('Ctrl Pts',(52.0327509345153,43.9222398433349,-209.548898118242));
#210309=CARTESIAN_POINT('Ctrl Pts',(52.0380379633556,43.9186734067761,-209.477805892547));
#210310=CARTESIAN_POINT('Ctrl Pts',(52.0431331684242,43.9152363675277,-209.40929303218));
#210311=CARTESIAN_POINT('Ctrl Pts',(52.0481711845886,43.9118009093687,-209.343582163061));
#210312=CARTESIAN_POINT('Ctrl Pts',(52.053197688286,43.9083249915534,-209.280672317176));
#210313=CARTESIAN_POINT('Ctrl Pts',(52.0584989082176,43.9046591025156,-209.214324225347));
#210314=CARTESIAN_POINT('Ctrl Pts',(52.0637869189831,43.9009485849322,-209.151091534621));
#210315=CARTESIAN_POINT('Ctrl Pts',(52.0690726236707,43.8971837489602,-209.090953530795));
#210316=CARTESIAN_POINT('Ctrl Pts',(52.0749226987908,43.8930169302381,-209.024394413184));
#210317=CARTESIAN_POINT('Ctrl Pts',(52.080769641772,43.8887838588144,-208.96162602192));
#210318=CARTESIAN_POINT('Ctrl Pts',(52.0865826447208,43.8845137395771,-208.902598818566));
#210319=CARTESIAN_POINT('Ctrl Pts',(52.0891752874545,43.8826092345029,-208.876272244984));
#210320=CARTESIAN_POINT('Ctrl Pts',(52.0917606452554,43.8806978553632,-208.850689622922));
#210321=CARTESIAN_POINT('Ctrl Pts',(52.0943337930903,43.8787842296859,-208.825845487606));
#210322=CARTESIAN_POINT('Ctrl Pts',(52.0981470647389,43.8759483356722,-208.789027767476));
#210323=CARTESIAN_POINT('Ctrl Pts',(52.1019204343215,43.8731194191416,-208.753839003036));
#210324=CARTESIAN_POINT('Ctrl Pts',(52.1056979659228,43.8702568909374,-208.720280928359));
#210325=CARTESIAN_POINT('Ctrl Pts',(52.1096891458759,43.8672324648333,-208.684824887469));
#210326=CARTESIAN_POINT('Ctrl Pts',(52.1136845529443,43.8641709060281,-208.651189045429));
#210327=CARTESIAN_POINT('Ctrl Pts',(52.1176934819693,43.8610639150675,-208.619358840089));
#210328=CARTESIAN_POINT('Ctrl Pts',(52.1221209898717,43.8576325180672,-208.584205190623));
#210329=CARTESIAN_POINT('Ctrl Pts',(52.1265646218548,43.8541460483929,-208.551253778001));
#210330=CARTESIAN_POINT('Ctrl Pts',(52.1309922302586,43.8506347478063,-208.520467603443));
#210331=CARTESIAN_POINT('Ctrl Pts',(52.1318186983157,43.849979319975,-208.514720981893));
#210332=CARTESIAN_POINT('Ctrl Pts',(52.1326445047111,43.8493231228087,-208.509049763197));
#210333=CARTESIAN_POINT('Ctrl Pts',(52.1334693091333,43.8486664746894,-208.50345365565));
#210334=CARTESIAN_POINT('Ctrl Pts',(52.1362477509627,43.8464544853346,-208.484602569417));
#210335=CARTESIAN_POINT('Ctrl Pts',(52.1390115559275,43.8442411033876,-208.466564424385));
#210336=CARTESIAN_POINT('Ctrl Pts',(52.141792873597,43.8419957546331,-208.449393395525));
#210337=CARTESIAN_POINT('Ctrl Pts',(52.1447241951854,43.8396293082002,-208.431296287042));
#210338=CARTESIAN_POINT('Ctrl Pts',(52.1476746346871,43.8372276679482,-208.414162016015));
#210339=CARTESIAN_POINT('Ctrl Pts',(52.1506486851097,43.834786239038,-208.398015691187));
#210340=CARTESIAN_POINT('Ctrl Pts',(52.1539039947587,43.8321139215049,-208.380342390623));
#210341=CARTESIAN_POINT('Ctrl Pts',(52.1571872713604,43.82939423425,-208.36385244999));
#210342=CARTESIAN_POINT('Ctrl Pts',(52.1604707470427,43.8266528564292,-208.34853874569));
#210343=CARTESIAN_POINT('Ctrl Pts',(52.1606844005896,43.8264744768242,-208.347542293285));
#210344=CARTESIAN_POINT('Ctrl Pts',(52.1608980453075,43.8262960144973,-208.346550809251));
#210345=CARTESIAN_POINT('Ctrl Pts',(52.1611116697293,43.8261174801212,-208.345564286924));
#210346=CARTESIAN_POINT('Ctrl Pts',(52.1632956867302,43.8242922107564,-208.33547844787));
#210347=CARTESIAN_POINT('Ctrl Pts',(52.1654674542167,43.822468685508,-208.325913484142));
#210348=CARTESIAN_POINT('Ctrl Pts',(52.1676645419426,43.8206118261382,-208.316897375615));
#210349=CARTESIAN_POINT('Ctrl Pts',(52.1700759527451,43.8185738325294,-208.30700175732));
#210350=CARTESIAN_POINT('Ctrl Pts',(52.1725176882122,43.8164958491871,-208.297767152186));
#210351=CARTESIAN_POINT('Ctrl Pts',(52.1749977315457,43.8143704840783,-208.289196225522));
#210352=CARTESIAN_POINT('Ctrl Pts',(52.1768850775668,43.812753052912,-208.28267363613));
#210353=CARTESIAN_POINT('Ctrl Pts',(52.1787936398816,43.8111090875315,-208.276534612158));
#210354=CARTESIAN_POINT('Ctrl Pts',(52.1807145176352,43.8094469441326,-208.270770100534));
#210355=CARTESIAN_POINT('Ctrl Pts',(52.1823557293411,43.8080267969119,-208.26584486053));
#210356=CARTESIAN_POINT('Ctrl Pts',(52.1840153685614,43.8065851661576,-208.261166956059));
#210357=CARTESIAN_POINT('Ctrl Pts',(52.1856993914338,43.80511516462,-208.256813689259));
#210358=CARTESIAN_POINT('Ctrl Pts',(52.187522563892,43.8035236979238,-208.252100715187));
#210359=CARTESIAN_POINT('Ctrl Pts',(52.1893742116152,43.8018990789262,-208.247767994534));
#210360=CARTESIAN_POINT('Ctrl Pts',(52.1912458864848,43.8002483732425,-208.243854523133));
#210361=CARTESIAN_POINT('Ctrl Pts',(52.1923633055812,43.7992628761973,-208.241518119654));
#210362=CARTESIAN_POINT('Ctrl Pts',(52.1934875690653,43.798268371482,-208.239330052569));
#210363=CARTESIAN_POINT('Ctrl Pts',(52.1946147722137,43.7972684489249,-208.237290523636));
#210364=CARTESIAN_POINT('Ctrl Pts',(52.1960055218434,43.7960347388096,-208.234774141286));
#210365=CARTESIAN_POINT('Ctrl Pts',(52.1974238413554,43.7947720316984,-208.23245629745));
#210366=CARTESIAN_POINT('Ctrl Pts',(52.1988449817247,43.7935018380268,-208.230406082707));
#210367=CARTESIAN_POINT('Ctrl Pts',(52.200408453943,43.7921044303109,-208.228150532263));
#210368=CARTESIAN_POINT('Ctrl Pts',(52.2019753026815,43.7906979991141,-208.226218733228));
#210369=CARTESIAN_POINT('Ctrl Pts',(52.2035177395458,43.7893076301571,-208.22463719045));
#210370=CARTESIAN_POINT('Ctrl Pts',(52.2051740594693,43.7878146058021,-208.222938877298));
#210371=CARTESIAN_POINT('Ctrl Pts',(52.2068022133339,43.7863401325541,-208.221643660656));
#210372=CARTESIAN_POINT('Ctrl Pts',(52.2083738943961,43.7849108267,-208.220720401459));
#210373=CARTESIAN_POINT('Ctrl Pts',(52.2102017346834,43.7832485665343,-208.219646665573));
#210374=CARTESIAN_POINT('Ctrl Pts',(52.2119530649539,43.7816475301323,-208.219075197685));
#210375=CARTESIAN_POINT('Ctrl Pts',(52.2135926537553,43.7801423382395,-208.218885518605));
#210376=CARTESIAN_POINT('Ctrl Pts',(52.2140270829265,43.7797435191783,-208.218835260806));
#210377=CARTESIAN_POINT('Ctrl Pts',(52.2144537171266,43.7793513883371,-208.218811515434));
#210378=CARTESIAN_POINT('Ctrl Pts',(52.2148720050704,43.7789665035542,-208.218811515434));
#210379=CARTESIAN_POINT('Ctrl Pts',(56.7089132278424,37.0787382657864,-216.762440352386));
#210380=CARTESIAN_POINT('Ctrl Pts',(56.4432500919345,37.2379648996087,-216.862162585544));
#210381=CARTESIAN_POINT('Ctrl Pts',(56.4975419847624,37.4436240691992,-217.108396707512));
#210382=CARTESIAN_POINT('Ctrl Pts',(56.7718148744283,37.3652096903236,-216.516505964954));
#210383=CARTESIAN_POINT('Ctrl Pts',(56.5198175013863,37.5280043332472,-216.615579405895));
#210384=CARTESIAN_POINT('Ctrl Pts',(56.5775101129868,37.7465455181985,-216.837759178115));
#210385=CARTESIAN_POINT('Ctrl Pts',(56.8285940470758,37.6233003639439,-216.244019387511));
#210386=CARTESIAN_POINT('Ctrl Pts',(56.5898249632591,37.7931945066467,-216.337771859736));
#210387=CARTESIAN_POINT('Ctrl Pts',(56.6495991956979,38.0196209280746,-216.537932548464));
#210388=CARTESIAN_POINT('Ctrl Pts',(56.8784089512595,37.8494072532151,-215.942196083675));
#210389=CARTESIAN_POINT('Ctrl Pts',(56.6513917750255,38.0264112674188,-216.026572725176));
#210390=CARTESIAN_POINT('Ctrl Pts',(56.7127812850717,38.2589564044561,-216.205851068199));
#210391=CARTESIAN_POINT('',(56.7089758625812,37.0787996208419,-216.761769944484));
#210392=CARTESIAN_POINT('',(56.4975419847624,37.4436240691992,-217.108396707512));
#210393=CARTESIAN_POINT('Origin',(56.9809801438088,37.3160013973188,-217.108396707512));
#210394=CARTESIAN_POINT('Ctrl Pts',(56.7127812850717,38.2589564044561,-216.205851068199));
#210395=CARTESIAN_POINT('Ctrl Pts',(56.675820350007,38.1189473751743,-216.400115647765));
#210396=CARTESIAN_POINT('Ctrl Pts',(56.6358255784857,37.9674460907173,-216.583274967065));
#210397=CARTESIAN_POINT('Ctrl Pts',(56.5929883959844,37.8051776760066,-216.756029715358));
#210398=CARTESIAN_POINT('Ctrl Pts',(56.5625833082106,37.6900023749221,-216.878648033801));
#210399=CARTESIAN_POINT('Ctrl Pts',(56.5307460013724,37.5694017889912,-216.996023775216));
#210400=CARTESIAN_POINT('Ctrl Pts',(56.4975419847624,37.4436240691992,-217.108396707512));
#210401=CARTESIAN_POINT('Ctrl Pts',(56.7089871854281,37.0788107123531,-216.761648750938));
#210402=CARTESIAN_POINT('Ctrl Pts',(56.708661470963,37.0793030031369,-216.761567481551));
#210403=CARTESIAN_POINT('Ctrl Pts',(56.7091315247285,37.0828254646993,-216.758788759137));
#210404=CARTESIAN_POINT('Ctrl Pts',(56.7103842705187,37.0893682154781,-216.753291228247));
#210405=CARTESIAN_POINT('Ctrl Pts',(56.7116344616361,37.0958976238959,-216.747804908245));
#210406=CARTESIAN_POINT('Ctrl Pts',(56.7136642224785,37.1054350836466,-216.739610788918));
#210407=CARTESIAN_POINT('Ctrl Pts',(56.7164352191511,37.1179511891652,-216.728646837421));
#210408=CARTESIAN_POINT('Ctrl Pts',(56.7174682169894,37.1226170590566,-216.724559593901));
#210409=CARTESIAN_POINT('Ctrl Pts',(56.7186039669403,37.1276966754221,-216.720087019819));
#210410=CARTESIAN_POINT('Ctrl Pts',(56.7198395388826,37.1331877755253,-216.715224484388));
#210411=CARTESIAN_POINT('Ctrl Pts',(56.7231360303223,37.14783796615,-216.702251296932));
#210412=CARTESIAN_POINT('Ctrl Pts',(56.7271451237326,37.1654188113094,-216.686504936086));
#210413=CARTESIAN_POINT('Ctrl Pts',(56.7317921133979,37.1858721625638,-216.667871599096));
#210414=CARTESIAN_POINT('Ctrl Pts',(56.7326930081959,37.1898373785583,-216.664259222574));
#210415=CARTESIAN_POINT('Ctrl Pts',(56.7336177907719,37.1939104852922,-216.660538231029));
#210416=CARTESIAN_POINT('Ctrl Pts',(56.7345657887601,37.1980909556426,-216.656707638063));
#210417=CARTESIAN_POINT('Ctrl Pts',(56.737484766271,37.2109630282513,-216.644912871764));
#210418=CARTESIAN_POINT('Ctrl Pts',(56.7406241476852,37.2248532466774,-216.6320793121));
#210419=CARTESIAN_POINT('Ctrl Pts',(56.7439616646172,37.2397440600632,-216.618175276465));
#210420=CARTESIAN_POINT('Ctrl Pts',(56.7456304230831,37.2471894667561,-216.611223258648));
#210421=CARTESIAN_POINT('Ctrl Pts',(56.7473486557363,37.2548849699725,-216.604003551846));
#210422=CARTESIAN_POINT('Ctrl Pts',(56.749113183206,37.2628280516737,-216.596511808696));
#210423=CARTESIAN_POINT('Ctrl Pts',(56.7499954469408,37.2667995925243,-216.592765937121));
#210424=CARTESIAN_POINT('Ctrl Pts',(56.7508892806168,37.2708330247062,-216.588952051994));
#210425=CARTESIAN_POINT('Ctrl Pts',(56.7517942616762,37.2749280118441,-216.585069586494));
#210426=CARTESIAN_POINT('Ctrl Pts',(56.7522467522059,37.2769755054131,-216.583128353743));
#210427=CARTESIAN_POINT('Ctrl Pts',(56.7527020293418,37.2790383875113,-216.581169975623));
#210428=CARTESIAN_POINT('Ctrl Pts',(56.7531600386458,37.2811166147432,-216.579194379838));
#210429=CARTESIAN_POINT('Ctrl Pts',(56.7536180479497,37.2831948419751,-216.577218784053));
#210430=CARTESIAN_POINT('Ctrl Pts',(56.7543059888436,37.286322328817,-216.574240479364));
#210431=CARTESIAN_POINT('Ctrl Pts',(56.7545422075944,37.2873972875617,-216.573215866174));
#210432=CARTESIAN_POINT('Ctrl Pts',(56.7621012076203,37.3217959673925,-216.540428244085));
#210433=CARTESIAN_POINT('Ctrl Pts',(56.7695178549811,37.355535319443,-216.507387750391));
#210434=CARTESIAN_POINT('Ctrl Pts',(56.7767905876617,37.3886103535824,-216.474120942766));
#210435=CARTESIAN_POINT('Ctrl Pts',(56.7809009568357,37.4073035472863,-216.455319363418));
#210436=CARTESIAN_POINT('Ctrl Pts',(56.7848762867467,37.4253986755092,-216.436844242353));
#210437=CARTESIAN_POINT('Ctrl Pts',(56.78886986911,37.4435511814868,-216.418027355469));
#210438=CARTESIAN_POINT('Ctrl Pts',(56.7919423812352,37.4575170371138,-216.40355035015));
#210439=CARTESIAN_POINT('Ctrl Pts',(56.795025195344,37.4715164619458,-216.388870306284));
#210440=CARTESIAN_POINT('Ctrl Pts',(56.7981765486193,37.4858386382505,-216.373668133342));
#210441=CARTESIAN_POINT('Ctrl Pts',(56.8159359101986,37.5665508546774,-216.287996720946));
#210442=CARTESIAN_POINT('Ctrl Pts',(56.832854077496,37.6433264560983,-216.200613606556));
#210443=CARTESIAN_POINT('Ctrl Pts',(56.8488877595288,37.7160793736129,-216.111889150275));
#210444=CARTESIAN_POINT('Ctrl Pts',(56.8590267960587,37.7620853058016,-216.055783478384));
#210445=CARTESIAN_POINT('Ctrl Pts',(56.8688128764962,37.8064834155413,-215.999141637438));
#210446=CARTESIAN_POINT('Ctrl Pts',(56.8782424684847,37.8492596800295,-215.942057996927));
#210447=CARTESIAN_POINT('Ctrl Pts',(50.6668571239968,44.0777189530043,-216.468046015339));
#210448=CARTESIAN_POINT('Ctrl Pts',(50.4202954871045,43.9828326938916,-216.258996421318));
#210449=CARTESIAN_POINT('Ctrl Pts',(50.2169391861068,44.2398739469141,-216.179548839231));
#210450=CARTESIAN_POINT('Ctrl Pts',(50.9477024065591,44.1832652290949,-215.960963622776));
#210451=CARTESIAN_POINT('Ctrl Pts',(50.702607269904,44.1457324009489,-215.837685287199));
#210452=CARTESIAN_POINT('Ctrl Pts',(50.5697429859293,44.3569399972268,-215.718609917522));
#210453=CARTESIAN_POINT('Ctrl Pts',(51.2153988083273,44.192734708103,-215.442665058708));
#210454=CARTESIAN_POINT('Ctrl Pts',(51.0255093994164,44.2008217405635,-215.345450727964));
#210455=CARTESIAN_POINT('Ctrl Pts',(50.9110336349312,44.3534119066666,-215.247525543514));
#210456=CARTESIAN_POINT('Ctrl Pts',(51.5381992078581,44.1395055735188,-214.660447877432));
#210457=CARTESIAN_POINT('Ctrl Pts',(51.4124712437483,44.1693327463343,-214.59669191525));
#210458=CARTESIAN_POINT('Ctrl Pts',(51.3258123082479,44.2676079799153,-214.537190176925));
#210459=CARTESIAN_POINT('Ctrl Pts',(51.6264957021156,44.1149795137312,-214.423951342294));
#210460=CARTESIAN_POINT('Ctrl Pts',(51.5180263342635,44.1477293653001,-214.371802696835));
#210461=CARTESIAN_POINT('Ctrl Pts',(51.4398111504988,44.2315500222654,-214.322416627157));
#210462=CARTESIAN_POINT('Ctrl Pts',(51.7972884149161,44.0548047396562,-213.839739291795));
#210463=CARTESIAN_POINT('Ctrl Pts',(51.7203476126764,44.089286352992,-213.818433091759));
#210464=CARTESIAN_POINT('Ctrl Pts',(51.6610101464785,44.1457350486596,-213.79183067467));
#210465=CARTESIAN_POINT('Ctrl Pts',(51.8659565316503,44.0178105340169,-213.478656833619));
#210466=CARTESIAN_POINT('Ctrl Pts',(51.8035205704321,44.0485969165887,-213.470699334602));
#210467=CARTESIAN_POINT('Ctrl Pts',(51.7505801429124,44.0950938200302,-213.464005878851));
#210468=CARTESIAN_POINT('Ctrl Pts',(51.8248396661196,44.0390948051906,-213.083798271317));
#210469=CARTESIAN_POINT('Ctrl Pts',(51.753836136243,44.0717738930276,-213.094488712702));
#210470=CARTESIAN_POINT('Ctrl Pts',(51.6968104056281,44.1244887290081,-213.105265698142));
#210471=CARTESIAN_POINT('',(50.8056178277775,44.122591905242,-216.213154850206));
#210472=CARTESIAN_POINT('',(50.3946587200443,44.285292057478,-215.949493832057));
#210473=CARTESIAN_POINT('Origin',(50.6744232242015,44.605072968075,-216.213154850206));
#210474=CARTESIAN_POINT('Ctrl Pts',(51.7111509881036,44.1161634878024,-213.405556127478));
#210475=CARTESIAN_POINT('Ctrl Pts',(51.7054714071276,44.1189759500224,-213.50459109405));
#210476=CARTESIAN_POINT('Ctrl Pts',(51.6884734636492,44.1278965425,-213.612607039845));
#210477=CARTESIAN_POINT('Ctrl Pts',(51.6441850919576,44.1484194974503,-213.787927031532));
#210478=CARTESIAN_POINT('Ctrl Pts',(51.6262866883493,44.1564463989509,-213.848578573237));
#210479=CARTESIAN_POINT('Ctrl Pts',(51.5944783226475,44.1699746414804,-213.942800966704));
#210480=CARTESIAN_POINT('Ctrl Pts',(51.5773336536473,44.1771103462579,-213.990722826982));
#210481=CARTESIAN_POINT('Ctrl Pts',(51.5551015148144,44.1860180080322,-214.048027515802));
#210482=CARTESIAN_POINT('Ctrl Pts',(51.5434203512994,44.190608779469,-214.077025395749));
#210483=CARTESIAN_POINT('Ctrl Pts',(51.5382922303731,44.1926046564484,-214.089526718781));
#210484=CARTESIAN_POINT('Ctrl Pts',(51.5348463012418,44.1939414477291,-214.097877258856));
#210485=CARTESIAN_POINT('Ctrl Pts',(51.5323282966788,44.1949141285707,-214.10393220042));
#210486=CARTESIAN_POINT('Ctrl Pts',(51.5003597777846,44.2072352608624,-214.180494287));
#210487=CARTESIAN_POINT('Ctrl Pts',(51.4589236498728,44.2227433939912,-214.271580524568));
#210488=CARTESIAN_POINT('Ctrl Pts',(51.3782047880098,44.2480465259769,-214.432816691758));
#210489=CARTESIAN_POINT('Ctrl Pts',(51.3481932423834,44.2568079154406,-214.490655269819));
#210490=CARTESIAN_POINT('Ctrl Pts',(51.2980611938582,44.2699144304708,-214.583366808615));
#210491=CARTESIAN_POINT('Ctrl Pts',(51.2717155778434,44.2764576509972,-214.631209651118));
#210492=CARTESIAN_POINT('Ctrl Pts',(51.2433573264094,44.2828773330698,-214.68123429109));
#210493=CARTESIAN_POINT('Ctrl Pts',(51.2239937443592,44.2871169811656,-214.7150623647));
#210494=CARTESIAN_POINT('Ctrl Pts',(51.214934183901,44.2890428011384,-214.730756571201));
#210495=CARTESIAN_POINT('Ctrl Pts',(51.1159651889466,44.3092682329707,-214.900388603229));
#210496=CARTESIAN_POINT('Ctrl Pts',(51.0372325599885,44.3187739897739,-215.025889321681));
#210497=CARTESIAN_POINT('Ctrl Pts',(50.9388506155471,44.3269983741609,-215.177851437473));
#210498=CARTESIAN_POINT('Ctrl Pts',(50.9093170633681,44.3287067824773,-215.222470642592));
#210499=CARTESIAN_POINT('Ctrl Pts',(50.870415210797,44.3303090954864,-215.280598871226));
#210500=CARTESIAN_POINT('Ctrl Pts',(50.8523116339892,44.3308676436715,-215.307462753606));
#210501=CARTESIAN_POINT('Ctrl Pts',(50.8336364266536,44.3311973019426,-215.335004734123));
#210502=CARTESIAN_POINT('Ctrl Pts',(50.8249195217816,44.3312925367348,-215.347831789202));
#210503=CARTESIAN_POINT('Ctrl Pts',(50.8213176701548,44.3313195626524,-215.353127434398));
#210504=CARTESIAN_POINT('Ctrl Pts',(50.8189463076488,44.3313346354746,-215.356613116074));
#210505=CARTESIAN_POINT('Ctrl Pts',(50.8189998321179,44.3313357734173,-215.356534797611));
#210506=CARTESIAN_POINT('Ctrl Pts',(50.6642979760868,44.3319582986941,-215.583833929845));
#210507=CARTESIAN_POINT('Ctrl Pts',(50.5215412302473,44.3141675772679,-215.779647760799));
#210508=CARTESIAN_POINT('Ctrl Pts',(50.3946839049651,44.2853208635448,-215.949517779663));
#210509=CARTESIAN_POINT('',(51.1992015578549,44.1752017469644,-215.438515904958));
#210510=CARTESIAN_POINT('Ctrl Pts',(51.1992016446529,44.1751487167426,-215.438515947409));
#210511=CARTESIAN_POINT('Ctrl Pts',(51.281838384943,44.1751487164063,-215.264092918614));
#210512=CARTESIAN_POINT('Ctrl Pts',(51.3570498862049,44.1683672671663,-215.096663697119));
#210513=CARTESIAN_POINT('Ctrl Pts',(51.4578268909383,44.153075442267,-214.856010573837));
#210514=CARTESIAN_POINT('Ctrl Pts',(51.4894281386649,44.1471157811946,-214.777541316661));
#210515=CARTESIAN_POINT('Ctrl Pts',(51.52643960228,44.1390383023429,-214.681640310082));
#210516=CARTESIAN_POINT('Ctrl Pts',(51.5330243552575,44.1375598470366,-214.664428060081));
#210517=CARTESIAN_POINT('Ctrl Pts',(51.5508612596177,44.1333734700322,-214.617109216616));
#210518=CARTESIAN_POINT('Ctrl Pts',(51.5769304234794,44.1269962078744,-214.546969728427));
#210519=CARTESIAN_POINT('Ctrl Pts',(51.600952481436,44.1204320662154,-214.479346571265));
#210520=CARTESIAN_POINT('Ctrl Pts',(51.6463079576364,44.1073102787278,-214.347455364974));
#210521=CARTESIAN_POINT('Ctrl Pts',(51.6729591850628,44.0985806227172,-214.264001371494));
#210522=CARTESIAN_POINT('Ctrl Pts',(51.7077592081449,44.0863610853566,-214.145530597343));
#210523=CARTESIAN_POINT('Ctrl Pts',(51.7184967630461,44.082431327535,-214.107158708638));
#210524=CARTESIAN_POINT('Ctrl Pts',(51.7382817589645,44.0749717043864,-214.032651669918));
#210525=CARTESIAN_POINT('Ctrl Pts',(51.7513941925948,44.06985843768,-213.980342118648));
#210526=CARTESIAN_POINT('Ctrl Pts',(51.8046067014177,44.0483179959303,-213.745999527886));
#210527=CARTESIAN_POINT('Ctrl Pts',(51.8284907824184,44.0367819547839,-213.572935771286));
#210528=CARTESIAN_POINT('Ctrl Pts',(51.8348891643276,44.0337882456516,-213.414282330697));
#210529=CARTESIAN_POINT('Ctrl Pts',(50.8056178277775,44.122591905242,-216.213154850207));
#210530=CARTESIAN_POINT('Ctrl Pts',(50.8518843754316,44.1351725469415,-216.127353743724));
#210531=CARTESIAN_POINT('Ctrl Pts',(50.898240202651,44.1454320264489,-216.039922027355));
#210532=CARTESIAN_POINT('Ctrl Pts',(50.9444825680174,44.1534284763442,-215.950864727423));
#210533=CARTESIAN_POINT('Ctrl Pts',(50.9642454094214,44.1568459609349,-215.912803843633));
#210534=CARTESIAN_POINT('Ctrl Pts',(50.9839873245558,44.1598506393414,-215.874445742745));
#210535=CARTESIAN_POINT('Ctrl Pts',(51.0036914984811,44.1624494574738,-215.835789521075));
#210536=CARTESIAN_POINT('Ctrl Pts',(51.03659613116,44.1667893073132,-215.771236255374));
#210537=CARTESIAN_POINT('Ctrl Pts',(51.0693950134981,44.1699966689994,-215.705853474845));
#210538=CARTESIAN_POINT('Ctrl Pts',(51.1020070264693,44.1721130516932,-215.639641199155));
#210539=CARTESIAN_POINT('Ctrl Pts',(51.1346190394405,44.174229434387,-215.573428923466));
#210540=CARTESIAN_POINT('Ctrl Pts',(51.1670439525282,44.175254960468,-215.506387152935));
#210541=CARTESIAN_POINT('Ctrl Pts',(51.1992014925245,44.1752416613785,-215.438515873006));
#210542=CARTESIAN_POINT('Ctrl Pts',(56.5618180211198,36.5289367340068,-217.254048694966));
#210543=CARTESIAN_POINT('Ctrl Pts',(56.2980271921268,36.6878565975336,-217.354444173088));
#210544=CARTESIAN_POINT('Ctrl Pts',(56.351930605989,36.892044198215,-217.60005));
#210545=CARTESIAN_POINT('Ctrl Pts',(56.6108961448827,36.7123872459292,-217.09039277187));
#210546=CARTESIAN_POINT('Ctrl Pts',(56.3465050213663,36.8714919357672,-217.190493004533));
#210547=CARTESIAN_POINT('Ctrl Pts',(56.4005154364319,37.0760848599628,-217.436382427969));
#210548=CARTESIAN_POINT('Ctrl Pts',(56.6599284966586,36.8956552674856,-216.926524548004));
#210549=CARTESIAN_POINT('Ctrl Pts',(56.394913005841,37.054862700115,-217.026399523816));
#210550=CARTESIAN_POINT('Ctrl Pts',(56.4490528535666,37.2599459188071,-217.272499319579));
#210551=CARTESIAN_POINT('Ctrl Pts',(56.7089132278424,37.0787382657863,-216.762440352386));
#210552=CARTESIAN_POINT('Ctrl Pts',(56.4432500919346,37.2379648996087,-216.862162585543));
#210553=CARTESIAN_POINT('Ctrl Pts',(56.4975419847625,37.4436240691992,-217.108396707512));
#210554=CARTESIAN_POINT('',(56.5618180211198,36.5289367340069,-217.254048694966));
#210555=CARTESIAN_POINT('',(56.351930605989,36.892044198215,-217.60005));
#210556=CARTESIAN_POINT('Origin',(56.8353687650353,36.7644215263347,-217.60005));
#210557=CARTESIAN_POINT('Origin',(1.5713232372253,-170.618389538147,32.0043824444259));
#210558=CARTESIAN_POINT('Origin',(3.60305208601888,-172.041642880457,32.426831165629));
#210559=CARTESIAN_POINT('Ctrl Pts',(50.3946838675078,44.2853208550272,-215.949517829821));
#210560=CARTESIAN_POINT('Ctrl Pts',(50.5733927277608,44.0594460487845,-216.033846066216));
#210561=CARTESIAN_POINT('Ctrl Pts',(50.8056178277775,44.122591905242,-216.213154850206));
#210562=CARTESIAN_POINT('Ctrl Pts',(50.1727811095107,44.2347300586007,-216.246332930804));
#210563=CARTESIAN_POINT('Ctrl Pts',(50.3446120279677,43.9972367818614,-216.339838795389));
#210564=CARTESIAN_POINT('Ctrl Pts',(50.5708296219181,44.0587490977934,-216.539715105359));
#210565=CARTESIAN_POINT('Ctrl Pts',(49.9199744021421,44.177167823471,-216.514858553214));
#210566=CARTESIAN_POINT('Ctrl Pts',(50.0849672365085,43.9266350565256,-216.613616901689));
#210567=CARTESIAN_POINT('Ctrl Pts',(50.3034496116678,43.9860440381524,-216.835170188754));
#210568=CARTESIAN_POINT('Ctrl Pts',(49.6396803417508,44.1134564636836,-216.757742122242));
#210569=CARTESIAN_POINT('Ctrl Pts',(49.8012110043667,43.8494770305304,-216.857236779929));
#210570=CARTESIAN_POINT('Ctrl Pts',(50.0071669705522,43.9054798737905,-217.102435280211));
#210571=CARTESIAN_POINT('',(50.0071669705522,43.9054798737905,-217.102435280211));
#210572=CARTESIAN_POINT('',(49.6397984855093,44.1135871370302,-216.757171052664));
#210573=CARTESIAN_POINT('Origin',(49.8759723669763,44.3879609366236,-217.102435280211));
#210574=CARTESIAN_POINT('Ctrl Pts',(50.3945871449586,44.285210229431,-215.949426636219));
#210575=CARTESIAN_POINT('Ctrl Pts',(50.3403778185267,44.2728463269777,-216.021921068329));
#210576=CARTESIAN_POINT('Ctrl Pts',(50.28355971832,44.2598869737324,-216.093705509569));
#210577=CARTESIAN_POINT('Ctrl Pts',(50.2241655077576,44.2463440207748,-216.164581859815));
#210578=CARTESIAN_POINT('Ctrl Pts',(50.1944684024764,44.239572544296,-216.200020034938));
#210579=CARTESIAN_POINT('Ctrl Pts',(50.1641272315725,44.2326551146929,-216.235231809947));
#210580=CARTESIAN_POINT('Ctrl Pts',(50.133147084301,44.2255941671355,-216.270193455524));
#210581=CARTESIAN_POINT('Ctrl Pts',(50.1156219255874,44.2215998598934,-216.289970907912));
#210582=CARTESIAN_POINT('Ctrl Pts',(50.0975181940928,44.2174787265865,-216.310078664585));
#210583=CARTESIAN_POINT('Ctrl Pts',(50.0794698516225,44.213366172549,-216.329813053606));
#210584=CARTESIAN_POINT('Ctrl Pts',(50.0656131873037,44.2102087479332,-216.344964184778));
#210585=CARTESIAN_POINT('Ctrl Pts',(50.051789719492,44.2070570535312,-216.35989596509));
#210586=CARTESIAN_POINT('Ctrl Pts',(50.0382957503063,44.203984129756,-216.374304437988));
#210587=CARTESIAN_POINT('Ctrl Pts',(50.0072258500349,44.1969087145151,-216.40747998551));
#210588=CARTESIAN_POINT('Ctrl Pts',(49.9754962336944,44.1896861667369,-216.440479352724));
#210589=CARTESIAN_POINT('Ctrl Pts',(49.943109870758,44.1823161715401,-216.473276174347));
#210590=CARTESIAN_POINT('Ctrl Pts',(49.9269166892898,44.1786311739417,-216.489674585158));
#210591=CARTESIAN_POINT('Ctrl Pts',(49.9105593293605,44.1749093239475,-216.506022369873));
#210592=CARTESIAN_POINT('Ctrl Pts',(49.8940382741992,44.1711506884566,-216.522316205284));
#210593=CARTESIAN_POINT('Ctrl Pts',(49.8857777466186,44.1692713707111,-216.53046312299));
#210594=CARTESIAN_POINT('Ctrl Pts',(49.8774762957926,44.1673828572408,-216.53859655406));
#210595=CARTESIAN_POINT('Ctrl Pts',(49.8691339870412,44.1654851614539,-216.54671608504));
#210596=CARTESIAN_POINT('Ctrl Pts',(49.8649628326655,44.1645363135605,-216.550775850529));
#210597=CARTESIAN_POINT('Ctrl Pts',(49.8607814638429,44.1635851701277,-216.554832141041));
#210598=CARTESIAN_POINT('Ctrl Pts',(49.8565898891525,44.162631733232,-216.558884904864));
#210599=CARTESIAN_POINT('Ctrl Pts',(49.8534462081347,44.1619166555603,-216.561924477731));
#210600=CARTESIAN_POINT('Ctrl Pts',(49.8502967863191,44.161200287819,-216.564962066839));
#210601=CARTESIAN_POINT('Ctrl Pts',(49.8471416274209,44.160482630978,-216.567997650376));
#210602=CARTESIAN_POINT('Ctrl Pts',(49.8460899077882,44.1602434120311,-216.569009511555));
#210603=CARTESIAN_POINT('Ctrl Pts',(49.846052776601,44.1602349647155,-216.569046012336));
#210604=CARTESIAN_POINT('Ctrl Pts',(49.8439845563056,44.1597645444787,-216.571032564579));
#210605=CARTESIAN_POINT('Ctrl Pts',(49.8163330530824,44.1534751628673,-216.597592189719));
#210606=CARTESIAN_POINT('Ctrl Pts',(49.7913737799107,44.1476814359235,-216.621099989597));
#210607=CARTESIAN_POINT('Ctrl Pts',(49.7691963068403,44.1424976436824,-216.641712338298));
#210608=CARTESIAN_POINT('Ctrl Pts',(49.7468039447084,44.1372636229844,-216.662524410758));
#210609=CARTESIAN_POINT('Ctrl Pts',(49.7272473454039,44.1326512141046,-216.680384949048));
#210610=CARTESIAN_POINT('Ctrl Pts',(49.7105929590235,44.1287463153261,-216.695420899773));
#210611=CARTESIAN_POINT('Ctrl Pts',(49.693882897516,44.1248283625851,-216.710507115242));
#210612=CARTESIAN_POINT('Ctrl Pts',(49.6800943060718,44.1216224781896,-216.722750012389));
#210613=CARTESIAN_POINT('Ctrl Pts',(49.6692714766647,44.1191865642665,-216.73224013285));
#210614=CARTESIAN_POINT('Ctrl Pts',(49.6584179235548,44.1167437353038,-216.741757193737));
#210615=CARTESIAN_POINT('Ctrl Pts',(49.6505468786249,44.1150751379176,-216.748505942923));
#210616=CARTESIAN_POINT('Ctrl Pts',(49.6456823274345,44.1142124382665,-216.752537603844));
#210617=CARTESIAN_POINT('Ctrl Pts',(49.6420995619744,44.1135770558044,-216.755506941596));
#210618=CARTESIAN_POINT('Ctrl Pts',(49.6401472140672,44.1133782759279,-216.757001588688));
#210619=CARTESIAN_POINT('Ctrl Pts',(49.6398281339281,44.1136199297753,-216.757027741579));
#210620=CARTESIAN_POINT('Ctrl Pts',(50.0071669705522,43.9054798737905,-217.102435280211));
#210621=CARTESIAN_POINT('Ctrl Pts',(50.1847337846587,43.9537632357284,-216.942259136119));
#210622=CARTESIAN_POINT('Ctrl Pts',(50.3518605126507,43.999207765089,-216.772016153339));
#210623=CARTESIAN_POINT('Ctrl Pts',(50.5078320264026,44.0416190066736,-216.591016782892));
#210624=CARTESIAN_POINT('Ctrl Pts',(50.612160077052,44.069987534065,-216.469947806684));
#210625=CARTESIAN_POINT('Ctrl Pts',(50.7114964522455,44.0969987421063,-216.344065601437));
#210626=CARTESIAN_POINT('Ctrl Pts',(50.8056178277775,44.1225919052419,-216.213154850207));
#210627=CARTESIAN_POINT('Ctrl Pts',(56.3926362809384,37.06446862304,-217.512497927056));
#210628=CARTESIAN_POINT('Ctrl Pts',(56.3025297216358,36.8538919311899,-217.234982111681));
#210629=CARTESIAN_POINT('Ctrl Pts',(56.6014172235551,36.7002760622361,-217.106014442417));
#210630=CARTESIAN_POINT('Ctrl Pts',(56.3494657971762,36.8595412342349,-217.614210849647));
#210631=CARTESIAN_POINT('Ctrl Pts',(56.3042743964622,36.6629877513575,-217.365043032676));
#210632=CARTESIAN_POINT('Ctrl Pts',(56.5644478950071,36.4938829304004,-217.276020812814));
#210633=CARTESIAN_POINT('Ctrl Pts',(56.2928585179201,36.6687695948746,-217.720014138817));
#210634=CARTESIAN_POINT('Ctrl Pts',(56.2815005063899,36.4738999535249,-217.512326327457));
#210635=CARTESIAN_POINT('Ctrl Pts',(56.5034547435963,36.3047735443712,-217.452585270555));
#210636=CARTESIAN_POINT('Ctrl Pts',(56.1826979052857,36.4485237337307,-217.873731285031));
#210637=CARTESIAN_POINT('Ctrl Pts',(56.1903893360325,36.2585417753414,-217.731401553872));
#210638=CARTESIAN_POINT('Ctrl Pts',(56.360210366167,36.0935380424276,-217.709357506335));
#210639=CARTESIAN_POINT('Ctrl Pts',(56.1505723352367,36.3946362936106,-217.914986052151));
#210640=CARTESIAN_POINT('Ctrl Pts',(56.1614999948485,36.2069207362181,-217.789469422921));
#210641=CARTESIAN_POINT('Ctrl Pts',(56.316755943097,36.0426866473361,-217.778283977819));
#210642=CARTESIAN_POINT('Ctrl Pts',(56.0799766262647,36.300874136992,-217.997168943781));
#210643=CARTESIAN_POINT('Ctrl Pts',(56.0918994632683,36.1185322173306,-217.904857915558));
#210644=CARTESIAN_POINT('Ctrl Pts',(56.2172639412631,35.9565745816487,-217.915612680145));
#210645=CARTESIAN_POINT('Ctrl Pts',(56.0407806740724,36.2602422377127,-218.038872206682));
#210646=CARTESIAN_POINT('Ctrl Pts',(56.0504566435121,36.0806895467743,-217.963493085148));
#210647=CARTESIAN_POINT('Ctrl Pts',(56.1601699153834,35.9206448721989,-217.98530951335));
#210648=CARTESIAN_POINT('Ctrl Pts',(55.9568722227823,36.2011920617794,-218.118554011763));
#210649=CARTESIAN_POINT('Ctrl Pts',(55.9559190189864,36.0280927685888,-218.074319363236));
#210650=CARTESIAN_POINT('Ctrl Pts',(56.0334146789495,35.8727684150699,-218.118501095087));
#210651=CARTESIAN_POINT('Ctrl Pts',(55.9109933553098,36.1822589517139,-218.15753647007));
#210652=CARTESIAN_POINT('Ctrl Pts',(55.9013096891468,36.012582278575,-218.128229973778));
#210653=CARTESIAN_POINT('Ctrl Pts',(55.9619426599398,35.8604753878485,-218.183672765375));
#210654=CARTESIAN_POINT('Ctrl Pts',(55.8172819109955,36.1744746994185,-218.226480768326));
#210655=CARTESIAN_POINT('Ctrl Pts',(55.7847759578152,36.0120234844064,-218.22108863219));
#210656=CARTESIAN_POINT('Ctrl Pts',(55.8109478702867,35.8674781880438,-218.298960241952));
#210657=CARTESIAN_POINT('Ctrl Pts',(55.7685414980389,36.1858554246731,-218.257001059377));
#210658=CARTESIAN_POINT('Ctrl Pts',(55.7213420795204,36.0271858039415,-218.261086960987));
#210659=CARTESIAN_POINT('Ctrl Pts',(55.7299143791894,35.8871614634557,-218.350008528068));
#210660=CARTESIAN_POINT('Ctrl Pts',(55.593234661827,36.2832559111648,-218.346964015346));
#210661=CARTESIAN_POINT('Ctrl Pts',(55.4860097606963,36.1376664348096,-218.372159308156));
#210662=CARTESIAN_POINT('Ctrl Pts',(55.4293178179656,36.0166622041161,-218.500532672009));
#210663=CARTESIAN_POINT('Ctrl Pts',(55.4818780387848,36.4672944339616,-218.361109888845));
#210664=CARTESIAN_POINT('Ctrl Pts',(55.3185434642075,36.3337248928643,-218.370180569382));
#210665=CARTESIAN_POINT('Ctrl Pts',(55.2179523418132,36.2266656323018,-218.52434896282));
#210666=CARTESIAN_POINT('Ctrl Pts',(55.4133688931145,36.6545388584683,-218.342531698738));
#210667=CARTESIAN_POINT('Ctrl Pts',(55.2229303298313,36.5126576021272,-218.321336607546));
#210668=CARTESIAN_POINT('Ctrl Pts',(55.0778128694631,36.4307605489773,-218.493419988678));
#210669=CARTESIAN_POINT('Ctrl Pts',(55.2146353748417,36.257836765148,-218.504776656654));
#210670=CARTESIAN_POINT('Ctrl Pts',(55.2853252387498,36.178323141292,-218.503619746298));
#210671=CARTESIAN_POINT('Ctrl Pts',(55.3572048505888,36.110335848808,-218.493333122548));
#210672=CARTESIAN_POINT('Ctrl Pts',(55.4666504076737,36.0261193376424,-218.464208616831));
#210673=CARTESIAN_POINT('Ctrl Pts',(55.5217803745163,35.9884509426223,-218.446222721449));
#210674=CARTESIAN_POINT('Ctrl Pts',(55.5774971758583,35.9575194484196,-218.423101362283));
#210675=CARTESIAN_POINT('Ctrl Pts',(55.6147698445988,35.9384032334131,-218.406545908665));
#210676=CARTESIAN_POINT('Ctrl Pts',(55.6324611397065,35.9300304583408,-218.398204123294));
#210677=CARTESIAN_POINT('Ctrl Pts',(55.7313233794382,35.8876181643618,-218.34857667575));
#210678=CARTESIAN_POINT('Ctrl Pts',(55.8079534193385,35.8685625899143,-218.300602301064));
#210679=CARTESIAN_POINT('Ctrl Pts',(55.9191591973471,35.8626148725108,-218.216232114058));
#210680=CARTESIAN_POINT('Ctrl Pts',(55.9738280789745,35.8652970767159,-218.17094486431));
#210681=CARTESIAN_POINT('Ctrl Pts',(56.0359726937985,35.8783633914484,-218.112680966177));
#210682=CARTESIAN_POINT('Ctrl Pts',(56.062256145949,35.8860946120971,-218.086547415529));
#210683=CARTESIAN_POINT('Ctrl Pts',(56.0797007647607,35.8917225550678,-218.068866535409));
#210684=CARTESIAN_POINT('Ctrl Pts',(56.089754223533,35.895294478457,-218.058454853419));
#210685=CARTESIAN_POINT('Ctrl Pts',(56.1552263829685,35.9201954539469,-217.989542144483));
#210686=CARTESIAN_POINT('Ctrl Pts',(56.2092799448895,35.952330746872,-217.924827472252));
#210687=CARTESIAN_POINT('Ctrl Pts',(56.284215107907,36.015451914569,-217.822567067476));
#210688=CARTESIAN_POINT('Ctrl Pts',(56.3201469433926,36.050740243414,-217.77013976598));
#210689=CARTESIAN_POINT('Ctrl Pts',(56.3594019560273,36.0983953590986,-217.706704657463));
#210690=CARTESIAN_POINT('Ctrl Pts',(56.375657213717,36.1202032964773,-217.679031770219));
#210691=CARTESIAN_POINT('Ctrl Pts',(56.3863680913675,36.1350489083464,-217.660475087131));
#210692=CARTESIAN_POINT('Ctrl Pts',(56.3924751485261,36.14382919598,-217.649680615388));
#210693=CARTESIAN_POINT('Ctrl Pts',(56.4675309888385,36.2547622702157,-217.514966686909));
#210694=CARTESIAN_POINT('Ctrl Pts',(56.5223283895667,36.3813273192802,-217.38573082968));
#210695=CARTESIAN_POINT('Ctrl Pts',(56.5618180211198,36.5289367340069,-217.254048694966));
#210696=CARTESIAN_POINT('Ctrl Pts',(56.351930605989,36.892044198215,-217.60005));
#210697=CARTESIAN_POINT('Ctrl Pts',(56.3106341552242,36.73561211731,-217.683519137624));
#210698=CARTESIAN_POINT('Ctrl Pts',(56.2620376674877,36.6063567109475,-217.763138346979));
#210699=CARTESIAN_POINT('Ctrl Pts',(56.1841151753959,36.4516751886226,-217.871613557135));
#210700=CARTESIAN_POINT('Ctrl Pts',(56.1573135581897,36.4066455053365,-217.905983993627));
#210701=CARTESIAN_POINT('Ctrl Pts',(56.1166432440885,36.3486930756933,-217.95452292113));
#210702=CARTESIAN_POINT('Ctrl Pts',(56.0961909694752,36.3221149231009,-217.978041235787));
#210703=CARTESIAN_POINT('Ctrl Pts',(56.0722901467882,36.2952600973141,-218.004121560642));
#210704=CARTESIAN_POINT('Ctrl Pts',(56.0603499093352,36.2828656242958,-218.01681895322));
#210705=CARTESIAN_POINT('Ctrl Pts',(56.0543848280906,36.2769259643628,-218.023081587245));
#210706=CARTESIAN_POINT('Ctrl Pts',(56.0518297096401,36.2744355207168,-218.025747097373));
#210707=CARTESIAN_POINT('Ctrl Pts',(56.0501266256028,36.2727874671719,-218.027519994919));
#210708=CARTESIAN_POINT('Ctrl Pts',(56.0499682211993,36.2726304501984,-218.027686065033));
#210709=CARTESIAN_POINT('Ctrl Pts',(55.9990105266362,36.2240321053245,-218.080507909176));
#210710=CARTESIAN_POINT('Ctrl Pts',(55.947907222693,36.1948194705703,-218.126920434258));
#210711=CARTESIAN_POINT('Ctrl Pts',(55.870874722202,36.1773006083812,-218.187476759461));
#210712=CARTESIAN_POINT('Ctrl Pts',(55.8451383675446,36.1758432616423,-218.206158299427));
#210713=CARTESIAN_POINT('Ctrl Pts',(55.8067444797832,36.1801517391582,-218.231754361591));
#210714=CARTESIAN_POINT('Ctrl Pts',(55.7939817881794,36.1826702714089,-218.239882441288));
#210715=CARTESIAN_POINT('Ctrl Pts',(55.7685784254658,36.189858492269,-218.25530756497));
#210716=CARTESIAN_POINT('Ctrl Pts',(55.7547799188749,36.1950574432706,-218.263238404901));
#210717=CARTESIAN_POINT('Ctrl Pts',(55.6522189990078,36.2419393110166,-218.319379639693));
#210718=CARTESIAN_POINT('Ctrl Pts',(55.5615769900803,36.3417129235347,-218.348549476024));
#210719=CARTESIAN_POINT('Ctrl Pts',(55.4814981831708,36.4969369346298,-218.349992971048));
#210720=CARTESIAN_POINT('Ctrl Pts',(49.6396803417518,44.1134564636829,-216.757742122242));
#210721=CARTESIAN_POINT('Ctrl Pts',(49.8012110043674,43.8494770305306,-216.85723677993));
#210722=CARTESIAN_POINT('Ctrl Pts',(50.0071669705522,43.9054798737905,-217.102435280211));
#210723=CARTESIAN_POINT('Ctrl Pts',(49.4561530329476,44.062897140813,-216.9238167844));
#210724=CARTESIAN_POINT('Ctrl Pts',(49.6176813002303,43.7995722598871,-217.023443915385));
#210725=CARTESIAN_POINT('Ctrl Pts',(49.8231124216493,43.8554323891537,-217.268463758512));
#210726=CARTESIAN_POINT('Ctrl Pts',(49.2724911599438,44.0123032282188,-217.089736149786));
#210727=CARTESIAN_POINT('Ctrl Pts',(49.4339330913007,43.7496080741896,-217.18956917487));
#210728=CARTESIAN_POINT('Ctrl Pts',(49.6389254121935,43.8053488862956,-217.43433427542));
#210729=CARTESIAN_POINT('Ctrl Pts',(49.0886970638134,43.9616759445554,-217.255503157469));
#210730=CARTESIAN_POINT('Ctrl Pts',(49.249970603928,43.6995856225942,-217.355612986355));
#210731=CARTESIAN_POINT('Ctrl Pts',(49.4546085996559,43.7552300878266,-217.60005));
#210732=CARTESIAN_POINT('',(49.4546085996559,43.7552300878266,-217.60005));
#210733=CARTESIAN_POINT('',(49.0886970638134,43.9616759445554,-217.255503157469));
#210734=CARTESIAN_POINT('Origin',(49.3234139960799,44.2377111506597,-217.60005));
#210735=CARTESIAN_POINT('Origin',(-245.875985088577,-31.0780147762713,132.706328537592));
#210736=CARTESIAN_POINT('Origin',(-243.323155334121,-35.8559000200963,132.120548472853));
#210737=CARTESIAN_POINT('Ctrl Pts',(49.2392068969802,42.8144262318624,-218.342424126527));
#210738=CARTESIAN_POINT('Ctrl Pts',(49.0981352490002,42.6214993839962,-218.320536202568));
#210739=CARTESIAN_POINT('Ctrl Pts',(49.0177848955319,42.4743719985975,-218.493933115956));
#210740=CARTESIAN_POINT('Ctrl Pts',(49.0491457939108,42.8840876677029,-218.360683589143));
#210741=CARTESIAN_POINT('Ctrl Pts',(48.9156261565165,42.7194999188607,-218.369201842649));
#210742=CARTESIAN_POINT('Ctrl Pts',(48.8090073140709,42.6180259879625,-218.524438151629));
#210743=CARTESIAN_POINT('Ctrl Pts',(48.8672534647879,42.9910417045365,-218.348178740586));
#210744=CARTESIAN_POINT('Ctrl Pts',(48.7219544884179,42.8806403242223,-218.373299555436));
#210745=CARTESIAN_POINT('Ctrl Pts',(48.6015262175029,42.8217286940762,-218.503553799908));
#210746=CARTESIAN_POINT('Ctrl Pts',(48.7646928214946,43.1655096926852,-218.259342211925));
#210747=CARTESIAN_POINT('Ctrl Pts',(48.6060096790964,43.1152569501545,-218.264332467645));
#210748=CARTESIAN_POINT('Ctrl Pts',(48.4659622753937,43.1213501679656,-218.355161400681));
#210749=CARTESIAN_POINT('Ctrl Pts',(48.7517775386604,43.2137285664805,-218.229368151499));
#210750=CARTESIAN_POINT('Ctrl Pts',(48.5892675478649,43.1781221617649,-218.225243782383));
#210751=CARTESIAN_POINT('Ctrl Pts',(48.4445750481121,43.2016010011096,-218.305092323547));
#210752=CARTESIAN_POINT('Ctrl Pts',(48.7563271074926,43.3078462492642,-218.160564679312));
#210753=CARTESIAN_POINT('Ctrl Pts',(48.5864539575163,43.2953660943901,-218.132916872251));
#210754=CARTESIAN_POINT('Ctrl Pts',(48.4338397167942,43.3533018519225,-218.190166022795));
#210755=CARTESIAN_POINT('Ctrl Pts',(48.7735288446776,43.353809900952,-218.121783538057));
#210756=CARTESIAN_POINT('Ctrl Pts',(48.600190391689,43.3502145581132,-218.079437137287));
#210757=CARTESIAN_POINT('Ctrl Pts',(48.4442068501562,43.4249009945937,-218.125389059377));
#210758=CARTESIAN_POINT('Ctrl Pts',(48.8590039851191,43.4820375499056,-218.000750329661));
#210759=CARTESIAN_POINT('Ctrl Pts',(48.6761884264651,43.4957516216008,-217.91062368486));
#210760=CARTESIAN_POINT('Ctrl Pts',(48.5121910139739,43.6184164248186,-217.923237587047));
#210761=CARTESIAN_POINT('Ctrl Pts',(48.9577162497748,43.553347797655,-217.915924150638));
#210762=CARTESIAN_POINT('Ctrl Pts',(48.7711504507846,43.5651821516904,-217.790160547008));
#210763=CARTESIAN_POINT('Ctrl Pts',(48.6033294989531,43.717527334291,-217.781577327593));
#210764=CARTESIAN_POINT('Ctrl Pts',(49.2312854327744,43.6941863378053,-217.721426214149));
#210765=CARTESIAN_POINT('Ctrl Pts',(49.036202633002,43.6813887518905,-217.516069552265));
#210766=CARTESIAN_POINT('Ctrl Pts',(48.8652456863714,43.9001875035932,-217.456834233708));
#210767=CARTESIAN_POINT('Ctrl Pts',(49.4219022397322,43.7527128881036,-217.614176933529));
#210768=CARTESIAN_POINT('Ctrl Pts',(49.2255719813905,43.7062052444277,-217.366811601907));
#210769=CARTESIAN_POINT('Ctrl Pts',(49.0541586904782,43.9632581572301,-217.27791260876));
#210770=CARTESIAN_POINT('Ctrl Pts',(49.6270070524957,43.7971127295262,-217.511593584289));
#210771=CARTESIAN_POINT('Ctrl Pts',(49.4168888445486,43.7053026630152,-217.236018678808));
#210772=CARTESIAN_POINT('Ctrl Pts',(49.2608016511118,44.0011146440645,-217.106570340894));
#210773=CARTESIAN_POINT('Ctrl Pts',(49.0801870931398,42.8824343798319,-218.350025764149));
#210774=CARTESIAN_POINT('Ctrl Pts',(49.0027571269435,42.9216296157716,-218.349558363419));
#210775=CARTESIAN_POINT('Ctrl Pts',(48.9387927753833,42.9635850473862,-218.342311230351));
#210776=CARTESIAN_POINT('Ctrl Pts',(48.8636071075648,43.0285900688282,-218.322357133335));
#210777=CARTESIAN_POINT('Ctrl Pts',(48.842004191093,43.0506080260999,-218.314196680044));
#210778=CARTESIAN_POINT('Ctrl Pts',(48.8148473949678,43.0839419698545,-218.299864963562));
#210779=CARTESIAN_POINT('Ctrl Pts',(48.8066696449585,43.0951047505369,-218.294739439232));
#210780=CARTESIAN_POINT('Ctrl Pts',(48.7920720413194,43.1175006398046,-218.283822966434));
#210781=CARTESIAN_POINT('Ctrl Pts',(48.7863005322459,43.1274160298958,-218.278747184425));
#210782=CARTESIAN_POINT('Ctrl Pts',(48.7553747751317,43.1902706205099,-218.244634347041));
#210783=CARTESIAN_POINT('Ctrl Pts',(48.7477937598005,43.2420701216404,-218.21038868015));
#210784=CARTESIAN_POINT('Ctrl Pts',(48.7628376713814,43.3195568794426,-218.149810572131));
#210785=CARTESIAN_POINT('Ctrl Pts',(48.7722543376512,43.3453523812971,-218.128090157083));
#210786=CARTESIAN_POINT('Ctrl Pts',(48.7930599541517,43.3837102238485,-218.093434197843));
#210787=CARTESIAN_POINT('Ctrl Pts',(48.8051328278828,43.4028056191118,-218.075588028891));
#210788=CARTESIAN_POINT('Ctrl Pts',(48.8221563815815,43.4248788632682,-218.053914616086));
#210789=CARTESIAN_POINT('Ctrl Pts',(48.8314046938857,43.4358573117923,-218.04287191288));
#210790=CARTESIAN_POINT('Ctrl Pts',(48.8355262866093,43.4405491551657,-218.038095968273));
#210791=CARTESIAN_POINT('Ctrl Pts',(48.8383091550492,43.4436740347655,-218.034902458652));
#210792=CARTESIAN_POINT('Ctrl Pts',(48.8403571964181,43.4459334904679,-218.032581409616));
#210793=CARTESIAN_POINT('Ctrl Pts',(48.9419508914772,43.5569843544506,-217.91819246589));
#210794=CARTESIAN_POINT('Ctrl Pts',(49.1434923162074,43.6706324100787,-217.767881223762));
#210795=CARTESIAN_POINT('Ctrl Pts',(49.4546085996559,43.7552300878266,-217.60005));
#210796=CARTESIAN_POINT('Ctrl Pts',(49.0886970638134,43.9616759445554,-217.255503157469));
#210797=CARTESIAN_POINT('Ctrl Pts',(49.0151399287483,43.9414141514911,-217.321845583205));
#210798=CARTESIAN_POINT('Ctrl Pts',(48.946963488087,43.9173173047126,-217.387552824715));
#210799=CARTESIAN_POINT('Ctrl Pts',(48.8529836892348,43.8753202935614,-217.485160910641));
#210800=CARTESIAN_POINT('Ctrl Pts',(48.8080643548638,43.8528590646516,-217.533726759519));
#210801=CARTESIAN_POINT('Ctrl Pts',(48.7593218903077,43.8240748429766,-217.589970076895));
#210802=CARTESIAN_POINT('Ctrl Pts',(48.7392211301387,43.8111840065362,-217.613985032988));
#210803=CARTESIAN_POINT('Ctrl Pts',(48.7259963435662,43.802466619305,-217.62997515421));
#210804=CARTESIAN_POINT('Ctrl Pts',(48.720651615937,43.7988677824946,-217.636498434306));
#210805=CARTESIAN_POINT('Ctrl Pts',(48.6521051529089,43.7511326433927,-217.721432036098));
#210806=CARTESIAN_POINT('Ctrl Pts',(48.6011058466663,43.7046963796237,-217.793420116029));
#210807=CARTESIAN_POINT('Ctrl Pts',(48.5396829829941,43.6289232846257,-217.896139553435));
#210808=CARTESIAN_POINT('Ctrl Pts',(48.5127389007901,43.5895075224444,-217.946183601514));
#210809=CARTESIAN_POINT('Ctrl Pts',(48.4879192797322,43.5408261485385,-218.002265900684));
#210810=CARTESIAN_POINT('Ctrl Pts',(48.4787011809696,43.51938296299,-218.025807795273));
#210811=CARTESIAN_POINT('Ctrl Pts',(48.4728712136029,43.5049584605067,-218.041392752447));
#210812=CARTESIAN_POINT('Ctrl Pts',(48.4704899065757,43.4987434520148,-218.048019264419));
#210813=CARTESIAN_POINT('Ctrl Pts',(48.4556126179059,43.4567276111961,-218.091989196291));
#210814=CARTESIAN_POINT('Ctrl Pts',(48.447318636186,43.4223097123662,-218.125369094889));
#210815=CARTESIAN_POINT('Ctrl Pts',(48.4379355955513,43.351853178451,-218.188536798286));
#210816=CARTESIAN_POINT('Ctrl Pts',(48.4367425363059,43.3173465388334,-218.217160970929));
#210817=CARTESIAN_POINT('Ctrl Pts',(48.4419528191108,43.2405774742888,-218.275471751038));
#210818=CARTESIAN_POINT('Ctrl Pts',(48.4484251786589,43.2018063387531,-218.302297507464));
#210819=CARTESIAN_POINT('Ctrl Pts',(48.4690551947459,43.1234942327623,-218.351289753058));
#210820=CARTESIAN_POINT('Ctrl Pts',(48.4840362288625,43.0821239108137,-218.374365224399));
#210821=CARTESIAN_POINT('Ctrl Pts',(48.5183278546908,43.0059380338195,-218.412220971132));
#210822=CARTESIAN_POINT('Ctrl Pts',(48.5490891293158,42.9488251961246,-218.437102070953));
#210823=CARTESIAN_POINT('Ctrl Pts',(48.5873397829352,42.8917692531179,-218.456717105432));
#210824=CARTESIAN_POINT('Ctrl Pts',(48.6144952712976,42.8537469019519,-218.468623558342));
#210825=CARTESIAN_POINT('Ctrl Pts',(48.6300405465755,42.8333212305513,-218.474349716168));
#210826=CARTESIAN_POINT('Ctrl Pts',(48.700481295165,42.745455745346,-218.496474416014));
#210827=CARTESIAN_POINT('Ctrl Pts',(48.7664496150731,42.6773021397737,-218.505675051354));
#210828=CARTESIAN_POINT('Ctrl Pts',(48.8417930108281,42.6113834075459,-218.506376562157));
#210829=CARTESIAN_POINT('Origin',(-2.81802535037841,-9.69927298715315,-227.60005));
#210830=CARTESIAN_POINT('',(48.1633319901564,41.4530789012665,-228.35005));
#210831=CARTESIAN_POINT('',(48.1633319901564,41.4530789012665,-228.35005));
#210832=CARTESIAN_POINT('',(47.632114758242,41.9825203546087,-227.60005));
#210833=CARTESIAN_POINT('',(41.9598150400404,36.2911954009805,-227.60005));
#210834=CARTESIAN_POINT('Origin',(48.1633319901564,41.4530789012665,-227.60005));
#210835=CARTESIAN_POINT('Ctrl Pts',(47.6321147582419,41.9825203546088,-227.60005));
#210836=CARTESIAN_POINT('Ctrl Pts',(48.6421799545279,42.9959733704936,-227.60005));
#210837=CARTESIAN_POINT('Ctrl Pts',(49.7021444432209,42.0348313420379,-227.60005));
#210838=CARTESIAN_POINT('Ctrl Pts',(47.6321147582419,41.9825203546088,-228.35005));
#210839=CARTESIAN_POINT('Ctrl Pts',(48.6421799545279,42.9959733704936,-228.35005));
#210840=CARTESIAN_POINT('Ctrl Pts',(49.7021444432209,42.0348313420379,-228.35005));
#210841=CARTESIAN_POINT('Ctrl Pts',(48.1633319901564,41.4530789012665,-228.35005));
#210842=CARTESIAN_POINT('Ctrl Pts',(48.6683645882994,41.9598054092088,-228.35005));
#210843=CARTESIAN_POINT('Ctrl Pts',(49.1983468326458,41.479234394981,-228.35005));
#210844=CARTESIAN_POINT('',(49.7021444432209,42.0348313420379,-227.60005));
#210845=CARTESIAN_POINT('Origin',(48.6945492220708,40.9236374479242,-227.60005));
#210846=CARTESIAN_POINT('',(49.1983468326459,41.4792343949811,-228.35005));
#210847=CARTESIAN_POINT('Origin',(49.1983468326459,41.4792343949811,-227.60005));
#210848=CARTESIAN_POINT('Origin',(48.6945492220708,40.9236374479242,-228.35005));
#210849=CARTESIAN_POINT('Origin',(0.128459562639233,-12.6359082483571,-227.60005));
#210850=CARTESIAN_POINT('',(54.0789914828443,36.6149049990089,-228.35005));
#210851=CARTESIAN_POINT('Origin',(0.128459562639233,-12.6359082483571,-228.35005));
#210852=CARTESIAN_POINT('Origin',(0.128459562639233,-12.6359082483571,-228.35005));
#210853=CARTESIAN_POINT('',(54.6328983814091,37.1205601658197,-227.60005));
#210854=CARTESIAN_POINT('Origin',(0.128459562639233,-12.6359082483571,-227.60005));
#210855=CARTESIAN_POINT('Origin',(54.0789914828443,36.6149049990089,-227.60005));
#210856=CARTESIAN_POINT('Ctrl Pts',(54.6328983814091,37.1205601658197,-227.60005));
#210857=CARTESIAN_POINT('Ctrl Pts',(55.5975842443944,36.0638199413983,-227.60005));
#210858=CARTESIAN_POINT('Ctrl Pts',(54.5875190481084,35.0503669255137,-227.60005));
#210859=CARTESIAN_POINT('Ctrl Pts',(54.6328983814091,37.1205601658197,-228.35005));
#210860=CARTESIAN_POINT('Ctrl Pts',(55.5975842443944,36.0638199413983,-228.35005));
#210861=CARTESIAN_POINT('Ctrl Pts',(54.5875190481084,35.0503669255137,-228.35005));
#210862=CARTESIAN_POINT('Ctrl Pts',(54.0789914828443,36.614904999009,-228.35005));
#210863=CARTESIAN_POINT('Ctrl Pts',(54.5613344143369,36.0865348867983,-228.35005));
#210864=CARTESIAN_POINT('Ctrl Pts',(54.056301816194,35.579808378856,-228.35005));
#210865=CARTESIAN_POINT('',(54.5875190481084,35.0503669255136,-227.60005));
#210866=CARTESIAN_POINT('',(54.056301816194,35.579808378856,-228.35005));
#210867=CARTESIAN_POINT('Origin',(54.056301816194,35.579808378856,-227.60005));
#210868=CARTESIAN_POINT('Origin',(53.5250845842796,36.1092498321983,-228.35005));
#210869=CARTESIAN_POINT('Origin',(53.5250845842796,36.1092498321983,-227.60005));
#210870=CARTESIAN_POINT('Origin',(3.07494447565784,-15.5725435095623,-227.60005));
#210871=CARTESIAN_POINT('',(54.5875190481084,35.0503669255136,-227.60005));
#210872=CARTESIAN_POINT('',(48.3142830765682,29.8185305620001,-228.35005));
#210873=CARTESIAN_POINT('Origin',(-10.7603008067452,26.6045648983079,-217.60005));
#210874=CARTESIAN_POINT('',(51.0024097331414,43.3988703109923,-218.35005));
#210875=CARTESIAN_POINT('',(-10.7603008067452,26.6045648983079,-218.35005));
#210876=CARTESIAN_POINT('',(50.8056178277775,44.122591905242,-217.60005));
#210877=CARTESIAN_POINT('',(51.6000409161409,44.3386087195339,-217.60005));
#210878=CARTESIAN_POINT('Origin',(51.0024097331414,43.3988703109923,-217.60005));
#210879=CARTESIAN_POINT('Ctrl Pts',(50.8056178277775,44.1225919052419,-217.60005));
#210880=CARTESIAN_POINT('Ctrl Pts',(51.6051500510689,44.3399979780626,-217.60005));
#210881=CARTESIAN_POINT('Ctrl Pts',(52.2148720050704,43.7789665035542,-217.60005));
#210882=CARTESIAN_POINT('Ctrl Pts',(50.8056178277775,44.1225919052419,-218.35005));
#210883=CARTESIAN_POINT('Ctrl Pts',(51.6051500510689,44.3399979780626,-218.35005));
#210884=CARTESIAN_POINT('Ctrl Pts',(52.2148720050704,43.7789665035542,-218.35005));
#210885=CARTESIAN_POINT('Ctrl Pts',(51.0024097331414,43.3988703109923,-218.35005));
#210886=CARTESIAN_POINT('Ctrl Pts',(51.4021758447871,43.5075733474026,-218.35005));
#210887=CARTESIAN_POINT('Ctrl Pts',(51.7070368217878,43.2270576101484,-218.35005));
#210888=CARTESIAN_POINT('',(52.2148720050704,43.7789665035542,-217.60005));
#210889=CARTESIAN_POINT('Origin',(51.1992016385053,42.6751487167426,-217.60005));
#210890=CARTESIAN_POINT('',(51.7070368217878,43.2270576101484,-218.35005));
#210891=CARTESIAN_POINT('Origin',(51.7070368217878,43.2270576101484,-217.60005));
#210892=CARTESIAN_POINT('Origin',(51.1992016385053,42.6751487167426,-218.35005));
#210893=CARTESIAN_POINT('Origin',(0.,-12.9675000200281,-217.60005));
#210894=CARTESIAN_POINT('',(56.3587426896623,39.6656306474361,-217.60005));
#210895=CARTESIAN_POINT('',(55.8106047487975,39.1537275337666,-218.35005));
#210896=CARTESIAN_POINT('Origin',(55.8106047487975,39.1537275337666,-217.60005));
#210897=CARTESIAN_POINT('Origin',(0.,-12.9675000200281,-218.35005));
#210898=CARTESIAN_POINT('Origin',(0.,-12.9675000200281,-217.60005));
#210899=CARTESIAN_POINT('Ctrl Pts',(56.3587426896623,39.6656306474361,-217.60005));
#210900=CARTESIAN_POINT('Ctrl Pts',(56.9242682147177,39.0600746573811,-217.60005));
#210901=CARTESIAN_POINT('Ctrl Pts',(56.7127812850717,38.2589564044561,-217.60005));
#210902=CARTESIAN_POINT('Ctrl Pts',(56.3587426896623,39.6656306474361,-218.35005));
#210903=CARTESIAN_POINT('Ctrl Pts',(56.9242682147177,39.0600746573811,-218.35005));
#210904=CARTESIAN_POINT('Ctrl Pts',(56.7127812850717,38.2589564044561,-218.35005));
#210905=CARTESIAN_POINT('Ctrl Pts',(55.8106047487975,39.1537275337666,-218.35005));
#210906=CARTESIAN_POINT('Ctrl Pts',(56.0933675113252,38.8509495387392,-218.35005));
#210907=CARTESIAN_POINT('Ctrl Pts',(55.9876240465022,38.4503904122767,-218.35005));
#210908=CARTESIAN_POINT('',(56.7127812850717,38.2589564044561,-217.60005));
#210909=CARTESIAN_POINT('',(55.9876240465022,38.4503904122767,-218.35005));
#210910=CARTESIAN_POINT('Origin',(55.9876240465022,38.4503904122767,-217.60005));
#210911=CARTESIAN_POINT('Origin',(55.2624668079327,38.6418244200972,-218.35005));
#210912=CARTESIAN_POINT('Origin',(55.2624668079327,38.6418244200972,-217.60005));
#210913=CARTESIAN_POINT('Origin',(39.6505639028577,-23.4348386281926,-217.60005));
#210914=CARTESIAN_POINT('',(39.6505639028577,-23.4348386281926,-218.35005));
#210915=CARTESIAN_POINT('',(51.3278340104563,17.8606293780317,-217.60005));
#210916=CARTESIAN_POINT('Origin',(39.6266165499379,-2.40986505017056,-217.60005));
#210917=CARTESIAN_POINT('',(56.1046081325044,-64.2577178902918,-218.35005));
#210918=CARTESIAN_POINT('',(56.1046081325044,-64.2577178902918,-218.35005));
#210919=CARTESIAN_POINT('',(56.8293274051384,-64.0646324794683,-217.60005));
#210920=CARTESIAN_POINT('',(56.0236521904458,-61.0406424582598,-217.60005));
#210921=CARTESIAN_POINT('Origin',(56.1046081325044,-64.2577178902918,-217.60005));
#210922=CARTESIAN_POINT('Ctrl Pts',(55.9291914878272,-64.9614564347782,
-218.35005));
#210923=CARTESIAN_POINT('Ctrl Pts',(56.2112637919648,-64.658035095081,-218.35005));
#210924=CARTESIAN_POINT('Ctrl Pts',(56.1046081325044,-64.2577178902918,
-218.35005));
#210925=CARTESIAN_POINT('Ctrl Pts',(56.478494115784,-65.4721095684411,-218.35005));
#210926=CARTESIAN_POINT('Ctrl Pts',(57.0426387240591,-64.8652668890467,
-218.35005));
#210927=CARTESIAN_POINT('Ctrl Pts',(56.8293274051384,-64.0646324794683,
-218.35005));
#210928=CARTESIAN_POINT('Ctrl Pts',(56.478494115784,-65.4721095684411,-217.60005));
#210929=CARTESIAN_POINT('Ctrl Pts',(57.0426387240591,-64.8652668890467,
-217.60005));
#210930=CARTESIAN_POINT('Ctrl Pts',(56.8293274051384,-64.0646324794683,
-217.60005));
#210931=CARTESIAN_POINT('',(56.478494115784,-65.4721095684411,-217.60005));
#210932=CARTESIAN_POINT('',(55.9291914878272,-64.9614564347782,-218.35005));
#210933=CARTESIAN_POINT('Origin',(55.9291914878272,-64.9614564347782,-217.60005));
#210934=CARTESIAN_POINT('Origin',(55.3798888598704,-64.4508033011153,-218.35005));
#210935=CARTESIAN_POINT('Origin',(55.3798888598704,-64.4508033011153,-217.60005));
#210936=CARTESIAN_POINT('Origin',(0.,-12.9675000200281,-217.60005));
#210937=CARTESIAN_POINT('',(52.3440043138885,-69.594874440935,-217.60005));
#210938=CARTESIAN_POINT('',(51.8349132062458,-69.0441238221254,-218.35005));
#210939=CARTESIAN_POINT('Origin',(51.8349132062458,-69.0441238221255,-217.60005));
#210940=CARTESIAN_POINT('Origin',(0.,-12.9675000200281,-218.35005));
#210941=CARTESIAN_POINT('Origin',(0.,-12.9675000200281,-217.60005));
#210942=CARTESIAN_POINT('Ctrl Pts',(51.1306793331593,-69.2175412094409,
-218.35005));
#210943=CARTESIAN_POINT('Ctrl Pts',(51.5306920318089,-69.3253333012854,
-218.35005));
#210944=CARTESIAN_POINT('Ctrl Pts',(51.8349132062458,-69.0441238221254,
-218.35005));
#210945=CARTESIAN_POINT('Ctrl Pts',(50.9355365677156,-69.9417092155658,
-218.35005));
#210946=CARTESIAN_POINT('Ctrl Pts',(51.7355619650149,-70.1572933992548,
-218.35005));
#210947=CARTESIAN_POINT('Ctrl Pts',(52.3440043138886,-69.5948744409349,
-218.35005));
#210948=CARTESIAN_POINT('Ctrl Pts',(50.9355365677156,-69.9417092155658,
-217.60005));
#210949=CARTESIAN_POINT('Ctrl Pts',(51.7355619650149,-70.1572933992548,
-217.60005));
#210950=CARTESIAN_POINT('Ctrl Pts',(52.3440043138886,-69.5948744409349,
-217.60005));
#210951=CARTESIAN_POINT('',(51.1306793331593,-69.2175412094409,-218.35005));
#210952=CARTESIAN_POINT('Origin',(51.325822098603,-68.4933732033159,-218.35005));
#210953=CARTESIAN_POINT('',(50.9355365677156,-69.9417092155658,-217.60005));
#210954=CARTESIAN_POINT('Origin',(51.325822098603,-68.4933732033159,-217.60005));
#210955=CARTESIAN_POINT('Origin',(51.1306793331593,-69.2175412094409,-217.60005));
#210956=CARTESIAN_POINT('Origin',(-10.6701281871898,-52.5639741032288,-217.60005));
#210957=CARTESIAN_POINT('',(48.0054978778587,-68.3753933286417,-218.35005));
#210958=CARTESIAN_POINT('',(50.9355365677156,-69.9417092155658,-217.60005));
#210959=CARTESIAN_POINT('Origin',(3.09688044790867,-9.95712216328114,-227.60005));
#210960=CARTESIAN_POINT('',(53.6770468827139,-61.5062120042031,-228.35005));
#210961=CARTESIAN_POINT('',(3.09688044790867,-9.95712216328114,-228.35005));
#210962=CARTESIAN_POINT('',(54.2123842387114,-60.9809369188682,-227.60005));
#210963=CARTESIAN_POINT('',(55.2047656166361,-61.9923285455256,-227.60005));
#210964=CARTESIAN_POINT('Origin',(53.6770468827139,-61.5062120042031,-227.60005));
#210965=CARTESIAN_POINT('Ctrl Pts',(53.6916490178651,-62.5414543003222,
-228.35005));
#210966=CARTESIAN_POINT('Ctrl Pts',(54.1781051950386,-62.0168686860244,
-228.35005));
#210967=CARTESIAN_POINT('Ctrl Pts',(53.6770468827138,-61.5062120042031,
-228.35005));
#210968=CARTESIAN_POINT('Ctrl Pts',(54.2415885090139,-63.0514215111064,
-228.35005));
#210969=CARTESIAN_POINT('Ctrl Pts',(55.2145008633609,-62.0022502825108,
-228.35005));
#210970=CARTESIAN_POINT('Ctrl Pts',(54.2123842387114,-60.9809369188682,
-228.35005));
#210971=CARTESIAN_POINT('Ctrl Pts',(54.2415885090139,-63.0514215111064,
-227.60005));
#210972=CARTESIAN_POINT('Ctrl Pts',(55.2145008633609,-62.0022502825108,
-227.60005));
#210973=CARTESIAN_POINT('Ctrl Pts',(54.2123842387114,-60.9809369188682,
-227.60005));
#210974=CARTESIAN_POINT('',(54.2415885090138,-63.0514215111064,-227.60005));
#210975=CARTESIAN_POINT('',(53.6916490178651,-62.5414543003222,-228.35005));
#210976=CARTESIAN_POINT('Origin',(53.6916490178651,-62.5414543003222,-227.60005));
#210977=CARTESIAN_POINT('Origin',(53.1417095267163,-62.031487089538,-228.35005));
#210978=CARTESIAN_POINT('Origin',(53.1417095267163,-62.031487089538,-227.60005));
#210979=CARTESIAN_POINT('Origin',(0.127542579976414,-12.8706479699377,-227.60005));
#210980=CARTESIAN_POINT('',(49.2725916132775,-67.9270204940557,-227.60005));
#210981=CARTESIAN_POINT('',(48.7731500580611,-67.3675045131195,-228.35005));
#210982=CARTESIAN_POINT('Origin',(48.7731500580611,-67.3675045131195,-227.60005));
#210983=CARTESIAN_POINT('Origin',(0.127542579976414,-12.8706479699377,-228.35005));
#210984=CARTESIAN_POINT('Origin',(0.127542579976414,-12.8706479699377,-227.60005));
#210985=CARTESIAN_POINT('Ctrl Pts',(47.738371146847,-67.3332636175182,-228.35005));
#210986=CARTESIAN_POINT('Ctrl Pts',(48.2394294591717,-67.8439202993396,
-228.35005));
#210987=CARTESIAN_POINT('Ctrl Pts',(48.7731500580611,-67.3675045131195,
-228.35005));
#210988=CARTESIAN_POINT('Ctrl Pts',(47.2030337908494,-67.858538702853,-228.35005));
#210989=CARTESIAN_POINT('Ctrl Pts',(48.2051504154989,-68.8798520664959,
-228.35005));
#210990=CARTESIAN_POINT('Ctrl Pts',(49.2725916132776,-67.9270204940556,
-228.35005));
#210991=CARTESIAN_POINT('Ctrl Pts',(47.2030337908494,-67.858538702853,-227.60005));
#210992=CARTESIAN_POINT('Ctrl Pts',(48.2051504154989,-68.8798520664959,
-227.60005));
#210993=CARTESIAN_POINT('Ctrl Pts',(49.2725916132776,-67.9270204940556,
-227.60005));
#210994=CARTESIAN_POINT('',(47.738371146847,-67.3332636175182,-228.35005));
#210995=CARTESIAN_POINT('Origin',(48.2737085028446,-66.8079885321834,-228.35005));
#210996=CARTESIAN_POINT('',(47.2030337908494,-67.858538702853,-227.60005));
#210997=CARTESIAN_POINT('Origin',(48.2737085028446,-66.8079885321834,-227.60005));
#210998=CARTESIAN_POINT('Origin',(47.738371146847,-67.3332636175182,-227.60005));
#210999=CARTESIAN_POINT('Origin',(-2.84179528795572,-15.7841737765938,-227.60005));
#211000=CARTESIAN_POINT('',(48.1954151687739,-68.8699303295103,-227.60005));
#211001=CARTESIAN_POINT('',(-2.84179528795573,-15.7841737765938,-228.35005));
#211002=CARTESIAN_POINT('Origin',(55.2624668079327,38.6418244200972,-167.906149834141));
#211003=CARTESIAN_POINT('',(56.3587426896623,39.6656306474361,-167.906149834141));
#211004=CARTESIAN_POINT('',(56.7127812850717,38.2589564044561,-167.906149834141));
#211005=CARTESIAN_POINT('Origin',(51.1992016385053,42.6751487167426,-167.906149834141));
#211006=CARTESIAN_POINT('',(52.2148720050704,43.7789665035542,-167.906149834141));
#211007=CARTESIAN_POINT('',(50.8056178277775,44.1225919052419,-167.906149834141));
#211008=CARTESIAN_POINT('Origin',(53.5250845842796,36.1092498321983,-228.35005));
#211009=CARTESIAN_POINT('',(54.6328983814091,37.1205601658197,-228.35005));
#211010=CARTESIAN_POINT('',(54.5875190481084,35.0503669255136,-228.35005));
#211011=CARTESIAN_POINT('Origin',(48.6945492220708,40.9236374479242,-228.35005));
#211012=CARTESIAN_POINT('',(47.632114758242,41.9825203546087,-228.35005));
#211013=CARTESIAN_POINT('',(49.7021444432209,42.0348313420379,-228.35005));
#211014=CARTESIAN_POINT('Origin',(53.1417095267163,-62.031487089538,-228.35005));
#211015=CARTESIAN_POINT('',(54.2123842387114,-60.9809369188682,-228.35005));
#211016=CARTESIAN_POINT('',(54.2415885090138,-63.0514215111064,-228.35005));
#211017=CARTESIAN_POINT('Origin',(48.2737085028446,-66.8079885321834,-228.35005));
#211018=CARTESIAN_POINT('',(49.2725916132775,-67.9270204940557,-228.35005));
#211019=CARTESIAN_POINT('',(47.2030337908494,-67.858538702853,-228.35005));
#211020=CARTESIAN_POINT('Origin',(51.325822098603,-68.4933732033159,-167.906149834141));
#211021=CARTESIAN_POINT('',(50.9355365677156,-69.9417092155658,-167.906149834141));
#211022=CARTESIAN_POINT('',(52.3440043138885,-69.594874440935,-167.906149834141));
#211023=CARTESIAN_POINT('Origin',(55.3798888598704,-64.4508033011153,-167.906149834141));
#211024=CARTESIAN_POINT('',(56.478494115784,-65.4721095684411,-167.906149834141));
#211025=CARTESIAN_POINT('',(56.8293274051384,-64.0646324794683,-167.906149834141));
#211026=CARTESIAN_POINT('Origin',(21.5,29.0311209585238,-234.90005));
#211027=CARTESIAN_POINT('',(21.6266284449832,30.2244211038859,-235.35005));
#211028=CARTESIAN_POINT('',(20.3,29.0311209585238,-235.35005));
#211029=CARTESIAN_POINT('Origin',(21.5,29.0311209585238,-235.35005));
#211030=CARTESIAN_POINT('',(21.5791427781145,29.7769335493751,-234.90005));
#211031=CARTESIAN_POINT('Origin',(21.6266284449832,30.2244211038859,-234.90005));
#211032=CARTESIAN_POINT('',(20.75,29.0311209585238,-234.90005));
#211033=CARTESIAN_POINT('Origin',(21.5,29.0311209585238,-234.90005));
#211034=CARTESIAN_POINT('Origin',(20.3,29.0311209585238,-234.90005));
#211035=CARTESIAN_POINT('Origin',(20.3,-25.4138432731711,-234.90005));
#211036=CARTESIAN_POINT('',(20.75,21.5631368321642,-234.90005));
#211037=CARTESIAN_POINT('',(20.3,21.5631368321642,-235.35005));
#211038=CARTESIAN_POINT('Origin',(20.3,21.5631368321642,-234.90005));
#211039=CARTESIAN_POINT('',(20.3,21.5631368321642,-235.35005));
#211040=CARTESIAN_POINT('',(20.75,29.0311209585238,-234.90005));
#211041=CARTESIAN_POINT('Origin',(-2.61456814389029E-14,-173.57701443073,
-234.90005));
#211042=CARTESIAN_POINT('',(25.0152849219089,29.8362882417925,-235.35005));
#211043=CARTESIAN_POINT('',(24.960358769668,29.3896529120211,-234.90005));
#211044=CARTESIAN_POINT('Origin',(25.0152849219089,29.8362882417925,-234.90005));
#211045=CARTESIAN_POINT('Origin',(-2.61456814389029E-14,-173.57701443073,
-234.90005));
#211046=CARTESIAN_POINT('Origin',(-2.61456814389029E-14,-173.57701443073,
-235.35005));
#211047=CARTESIAN_POINT('Origin',(21.5,21.5631368321642,-234.90005));
#211048=CARTESIAN_POINT('',(21.5,20.8131368321642,-234.90005));
#211049=CARTESIAN_POINT('',(21.5,20.3631368321642,-235.35005));
#211050=CARTESIAN_POINT('Origin',(21.5,20.3631368321642,-234.90005));
#211051=CARTESIAN_POINT('Origin',(21.5,21.5631368321642,-235.35005));
#211052=CARTESIAN_POINT('Origin',(21.5,21.5631368321642,-234.90005));
#211053=CARTESIAN_POINT('Origin',(24.838300653577,28.3971299569735,-234.90005));
#211054=CARTESIAN_POINT('',(25.604588652464,29.6281062779325,-235.35005));
#211055=CARTESIAN_POINT('',(25.366775135568,29.2460791438418,-234.90005));
#211056=CARTESIAN_POINT('Origin',(25.604588652464,29.6281062779325,-234.90005));
#211057=CARTESIAN_POINT('Origin',(24.838300653577,28.3971299569735,-234.90005));
#211058=CARTESIAN_POINT('Origin',(24.838300653577,28.3971299569735,-235.35005));
#211059=CARTESIAN_POINT('Origin',(-296.501483394397,20.3631368321642,-234.90005));
#211060=CARTESIAN_POINT('',(29.125,20.8131368321642,-234.90005));
#211061=CARTESIAN_POINT('',(29.125,20.3631368321642,-235.35005));
#211062=CARTESIAN_POINT('Origin',(29.125,20.3631368321642,-234.90005));
#211063=CARTESIAN_POINT('',(-296.501483394397,20.3631368321642,-235.35005));
#211064=CARTESIAN_POINT('',(-1.23757166668304E-15,20.8131368321642,-234.90005));
#211065=CARTESIAN_POINT('Origin',(-6.29739814579425E-15,-11.5034818258363,
-234.90005));
#211066=CARTESIAN_POINT('',(29.8646825396825,26.6475763089516,-235.35005));
#211067=CARTESIAN_POINT('',(29.5873015873016,26.2932321157492,-234.90005));
#211068=CARTESIAN_POINT('Origin',(29.8646825396825,26.6475763089516,-234.90005));
#211069=CARTESIAN_POINT('Origin',(-6.29739814579425E-15,-11.5034818258363,
-234.90005));
#211070=CARTESIAN_POINT('Origin',(-6.29739814579425E-15,-11.5034818258363,
-235.35005));
#211071=CARTESIAN_POINT('Origin',(29.125,21.5631368321642,-234.90005));
#211072=CARTESIAN_POINT('',(29.875,21.5631368321642,-234.90005));
#211073=CARTESIAN_POINT('',(30.325,21.5631368321642,-235.35005));
#211074=CARTESIAN_POINT('Origin',(30.325,21.5631368321642,-234.90005));
#211075=CARTESIAN_POINT('Origin',(29.125,21.5631368321642,-235.35005));
#211076=CARTESIAN_POINT('Origin',(29.125,21.5631368321642,-234.90005));
#211077=CARTESIAN_POINT('Origin',(29.125,25.702658460412,-234.90005));
#211078=CARTESIAN_POINT('',(30.325,25.702658460412,-235.35005));
#211079=CARTESIAN_POINT('',(29.875,25.702658460412,-234.90005));
#211080=CARTESIAN_POINT('Origin',(30.325,25.702658460412,-234.90005));
#211081=CARTESIAN_POINT('Origin',(29.125,25.702658460412,-234.90005));
#211082=CARTESIAN_POINT('Origin',(29.125,25.702658460412,-235.35005));
#211083=CARTESIAN_POINT('Origin',(30.325,-25.4138432731711,-234.90005));
#211084=CARTESIAN_POINT('',(29.875,21.5631368321642,-234.90005));
#211085=CARTESIAN_POINT('',(30.325,25.702658460412,-235.35005));
#211086=CARTESIAN_POINT('Origin',(11.3749999999999,29.8508988479304,-234.90005));
#211087=CARTESIAN_POINT('',(11.4419952819386,31.0490272351235,-235.35005));
#211088=CARTESIAN_POINT('',(10.1749999999999,29.8508988479304,-235.35005));
#211089=CARTESIAN_POINT('Origin',(11.3749999999999,29.8508988479304,-235.35005));
#211090=CARTESIAN_POINT('',(11.4168720512116,30.5997290899261,-234.90005));
#211091=CARTESIAN_POINT('Origin',(11.4419952819386,31.0490272351235,-234.90005));
#211092=CARTESIAN_POINT('',(10.6249999999999,29.8508988479304,-234.90005));
#211093=CARTESIAN_POINT('Origin',(11.3749999999999,29.8508988479304,-234.90005));
#211094=CARTESIAN_POINT('Origin',(10.1749999999999,29.8508988479304,-234.90005));
#211095=CARTESIAN_POINT('Origin',(10.1749999999999,-25.4138432731711,-234.90005));
#211096=CARTESIAN_POINT('',(10.6249999999999,21.5631368321642,-234.90005));
#211097=CARTESIAN_POINT('',(10.1749999999999,21.5631368321642,-235.35005));
#211098=CARTESIAN_POINT('Origin',(10.1749999999999,21.5631368321642,-234.90005));
#211099=CARTESIAN_POINT('',(10.1749999999999,21.5631368321642,-235.35005));
#211100=CARTESIAN_POINT('',(10.6249999999999,29.8508988479304,-234.90005));
#211101=CARTESIAN_POINT('Origin',(-2.61456814389029E-14,-173.57701443073,
-234.90005));
#211102=CARTESIAN_POINT('',(19.1119042071944,30.4756045219376,-235.35005));
#211103=CARTESIAN_POINT('',(19.0699401294965,30.0275654430807,-234.90005));
#211104=CARTESIAN_POINT('Origin',(19.1119042071944,30.4756045219376,-234.90005));
#211105=CARTESIAN_POINT('Origin',(-2.61456814389029E-14,-173.57701443073,
-234.90005));
#211106=CARTESIAN_POINT('Origin',(-2.61456814389029E-14,-173.57701443073,
-235.35005));
#211107=CARTESIAN_POINT('Origin',(11.3749999999999,21.5631368321642,-234.90005));
#211108=CARTESIAN_POINT('',(11.3749999999999,20.8131368321642,-234.90005));
#211109=CARTESIAN_POINT('',(11.3749999999999,20.3631368321642,-235.35005));
#211110=CARTESIAN_POINT('Origin',(11.3749999999999,20.3631368321642,-234.90005));
#211111=CARTESIAN_POINT('Origin',(11.3749999999999,21.5631368321642,-235.35005));
#211112=CARTESIAN_POINT('Origin',(11.3749999999999,21.5631368321642,-234.90005));
#211113=CARTESIAN_POINT('Origin',(19.,29.2808336449858,-234.90005));
#211114=CARTESIAN_POINT('',(20.2,29.2808336449858,-235.35005));
#211115=CARTESIAN_POINT('',(19.75,29.2808336449858,-234.90005));
#211116=CARTESIAN_POINT('Origin',(20.2,29.2808336449858,-234.90005));
#211117=CARTESIAN_POINT('Origin',(19.,29.2808336449858,-234.90005));
#211118=CARTESIAN_POINT('Origin',(19.,29.2808336449858,-235.35005));
#211119=CARTESIAN_POINT('Origin',(-296.501483394397,20.3631368321642,-234.90005));
#211120=CARTESIAN_POINT('',(19.,20.8131368321642,-234.90005));
#211121=CARTESIAN_POINT('',(19.,20.3631368321642,-235.35005));
#211122=CARTESIAN_POINT('Origin',(19.,20.3631368321642,-234.90005));
#211123=CARTESIAN_POINT('',(-296.501483394397,20.3631368321642,-235.35005));
#211124=CARTESIAN_POINT('',(-1.23757166668304E-15,20.8131368321642,-234.90005));
#211125=CARTESIAN_POINT('Origin',(20.2,-25.4138432731711,-234.90005));
#211126=CARTESIAN_POINT('',(20.2,21.5631368321642,-235.35005));
#211127=CARTESIAN_POINT('',(19.75,21.5631368321642,-234.90005));
#211128=CARTESIAN_POINT('Origin',(20.2,21.5631368321642,-234.90005));
#211129=CARTESIAN_POINT('',(19.75,21.5631368321642,-234.90005));
#211130=CARTESIAN_POINT('',(20.2,29.2808336449858,-235.35005));
#211131=CARTESIAN_POINT('Origin',(19.,21.5631368321642,-234.90005));
#211132=CARTESIAN_POINT('Origin',(19.,21.5631368321642,-234.90005));
#211133=CARTESIAN_POINT('Origin',(19.,21.5631368321642,-235.35005));
#211134=CARTESIAN_POINT('Origin',(1.25,30.1648419118246,-234.90005));
#211135=CARTESIAN_POINT('',(1.25736211889437,31.3648193279477,-235.35005));
#211136=CARTESIAN_POINT('',(0.0499999999999979,30.1648419118246,-235.35005));
#211137=CARTESIAN_POINT('Origin',(1.25,30.1648419118246,-235.35005));
#211138=CARTESIAN_POINT('',(1.25460132430898,30.9148277969016,-234.90005));
#211139=CARTESIAN_POINT('Origin',(1.25736211889437,31.3648193279477,-234.90005));
#211140=CARTESIAN_POINT('',(0.5,30.1648419118246,-234.90005));
#211141=CARTESIAN_POINT('Origin',(1.25,30.1648419118246,-234.90005));
#211142=CARTESIAN_POINT('Origin',(0.05,30.1648419118246,-234.90005));
#211143=CARTESIAN_POINT('Origin',(0.0499999999999945,-25.4138432731711,
-234.90005));
#211144=CARTESIAN_POINT('',(0.5,21.5631368321642,-234.90005));
#211145=CARTESIAN_POINT('',(0.0499999999999974,21.5631368321642,-235.35005));
#211146=CARTESIAN_POINT('Origin',(0.05,21.5631368321642,-234.90005));
#211147=CARTESIAN_POINT('',(0.0499999999999974,21.5631368321642,-235.35005));
#211148=CARTESIAN_POINT('',(0.5,30.1648419118246,-234.90005));
#211149=CARTESIAN_POINT('Origin',(-2.61456814389029E-14,-173.57701443073,
-234.90005));
#211150=CARTESIAN_POINT('',(8.9272710441499,31.1741516601419,-235.35005));
#211151=CARTESIAN_POINT('',(8.90766940259363,30.7245787787886,-234.90005));
#211152=CARTESIAN_POINT('Origin',(8.9272710441499,31.1741516601419,-234.90005));
#211153=CARTESIAN_POINT('Origin',(-2.61456814389029E-14,-173.57701443073,
-234.90005));
#211154=CARTESIAN_POINT('Origin',(-2.61456814389029E-14,-173.57701443073,
-235.35005));
#211155=CARTESIAN_POINT('Origin',(1.25,21.5631368321642,-234.90005));
#211156=CARTESIAN_POINT('',(1.25,20.8131368321642,-234.90005));
#211157=CARTESIAN_POINT('',(1.25,20.3631368321642,-235.35005));
#211158=CARTESIAN_POINT('Origin',(1.25,20.3631368321642,-234.90005));
#211159=CARTESIAN_POINT('Origin',(1.25,21.5631368321642,-235.35005));
#211160=CARTESIAN_POINT('Origin',(1.25,21.5631368321642,-234.90005));
#211161=CARTESIAN_POINT('Origin',(8.87499999999986,29.9752906431998,-234.90005));
#211162=CARTESIAN_POINT('',(10.075,29.9752906431998,-235.35005));
#211163=CARTESIAN_POINT('',(9.62499999999986,29.9752906431998,-234.90005));
#211164=CARTESIAN_POINT('Origin',(10.075,29.9752906431998,-234.90005));
#211165=CARTESIAN_POINT('Origin',(8.87499999999986,29.9752906431998,-234.90005));
#211166=CARTESIAN_POINT('Origin',(8.87499999999986,29.9752906431998,-235.35005));
#211167=CARTESIAN_POINT('Origin',(-296.501483394397,20.3631368321642,-234.90005));
#211168=CARTESIAN_POINT('',(8.87499999999986,20.8131368321642,-234.90005));
#211169=CARTESIAN_POINT('',(8.87499999999986,20.3631368321642,-235.35005));
#211170=CARTESIAN_POINT('Origin',(8.87499999999986,20.3631368321642,-234.90005));
#211171=CARTESIAN_POINT('',(-296.501483394397,20.3631368321642,-235.35005));
#211172=CARTESIAN_POINT('',(-1.23757166668304E-15,20.8131368321642,-234.90005));
#211173=CARTESIAN_POINT('Origin',(10.075,-25.4138432731712,-234.90005));
#211174=CARTESIAN_POINT('',(10.0749999999999,21.5631368321642,-235.35005));
#211175=CARTESIAN_POINT('',(9.62499999999986,21.5631368321642,-234.90005));
#211176=CARTESIAN_POINT('Origin',(10.0749999999999,21.5631368321642,-234.90005));
#211177=CARTESIAN_POINT('',(9.62499999999986,21.5631368321642,-234.90005));
#211178=CARTESIAN_POINT('',(10.075,29.9752906431998,-235.35005));
#211179=CARTESIAN_POINT('Origin',(8.87499999999986,21.5631368321642,-234.90005));
#211180=CARTESIAN_POINT('Origin',(8.87499999999986,21.5631368321642,-234.90005));
#211181=CARTESIAN_POINT('Origin',(8.87499999999986,21.5631368321642,-235.35005));
#211182=CARTESIAN_POINT('Origin',(1.25,19.0631368321642,-234.90005));
#211183=CARTESIAN_POINT('',(1.25,20.2631368321642,-235.35005));
#211184=CARTESIAN_POINT('',(1.25,19.8131368321642,-234.90005));
#211185=CARTESIAN_POINT('Origin',(1.25,20.2631368321642,-234.90005));
#211186=CARTESIAN_POINT('',(0.5,19.0631368321642,-234.90005));
#211187=CARTESIAN_POINT('Origin',(1.25,19.0631368321642,-234.90005));
#211188=CARTESIAN_POINT('',(0.0499999999999972,19.0631368321642,-235.35005));
#211189=CARTESIAN_POINT('Origin',(0.0499999999999994,19.0631368321642,-234.90005));
#211190=CARTESIAN_POINT('Origin',(1.25,19.0631368321642,-235.35005));
#211191=CARTESIAN_POINT('Origin',(0.0499999999999945,-25.4138432731711,
-234.90005));
#211192=CARTESIAN_POINT('',(0.5,10.9575972794973,-234.90005));
#211193=CARTESIAN_POINT('',(0.0499999999999967,10.9575972794973,-235.35005));
#211194=CARTESIAN_POINT('Origin',(0.0499999999999989,10.9575972794973,-234.90005));
#211195=CARTESIAN_POINT('',(0.0499999999999967,10.9575972794973,-235.35005));
#211196=CARTESIAN_POINT('',(0.5,19.0631368321642,-234.90005));
#211197=CARTESIAN_POINT('Origin',(-296.501483394397,20.2631368321643,-234.90005));
#211198=CARTESIAN_POINT('',(8.87499999999986,20.2631368321642,-235.35005));
#211199=CARTESIAN_POINT('',(8.87499999999986,19.8131368321642,-234.90005));
#211200=CARTESIAN_POINT('Origin',(8.87499999999986,20.2631368321642,-234.90005));
#211201=CARTESIAN_POINT('',(-1.54373336646988E-15,19.8131368321642,-234.90005));
#211202=CARTESIAN_POINT('',(-296.501483394397,20.2631368321643,-235.35005));
#211203=CARTESIAN_POINT('Origin',(1.25,10.9575972794973,-234.90005));
#211204=CARTESIAN_POINT('',(1.25,10.2075972794973,-234.90005));
#211205=CARTESIAN_POINT('',(1.25,9.75759727949733,-235.35005));
#211206=CARTESIAN_POINT('Origin',(1.25,9.75759727949733,-234.90005));
#211207=CARTESIAN_POINT('Origin',(1.25,10.9575972794973,-235.35005));
#211208=CARTESIAN_POINT('Origin',(1.25,10.9575972794973,-234.90005));
#211209=CARTESIAN_POINT('Origin',(8.87499999999986,19.0631368321642,-234.90005));
#211210=CARTESIAN_POINT('',(10.075,19.0631368321642,-235.35005));
#211211=CARTESIAN_POINT('',(9.62499999999986,19.0631368321642,-234.90005));
#211212=CARTESIAN_POINT('Origin',(10.075,19.0631368321642,-234.90005));
#211213=CARTESIAN_POINT('Origin',(8.87499999999986,19.0631368321642,-234.90005));
#211214=CARTESIAN_POINT('Origin',(8.87499999999986,19.0631368321642,-235.35005));
#211215=CARTESIAN_POINT('Origin',(-296.501483394397,9.75759727949737,-234.90005));
#211216=CARTESIAN_POINT('',(8.87499999999986,10.2075972794973,-234.90005));
#211217=CARTESIAN_POINT('',(8.87499999999986,9.75759727949733,-235.35005));
#211218=CARTESIAN_POINT('Origin',(8.87499999999986,9.75759727949733,-234.90005));
#211219=CARTESIAN_POINT('',(-296.501483394397,9.75759727949736,-235.35005));
#211220=CARTESIAN_POINT('',(-2.53637567332344E-15,10.2075972794973,-234.90005));
#211221=CARTESIAN_POINT('Origin',(10.075,-25.4138432731712,-234.90005));
#211222=CARTESIAN_POINT('',(10.0749999999998,10.9575972794973,-235.35005));
#211223=CARTESIAN_POINT('',(9.62499999999986,10.9575972794973,-234.90005));
#211224=CARTESIAN_POINT('Origin',(10.0749999999998,10.9575972794973,-234.90005));
#211225=CARTESIAN_POINT('',(9.62499999999986,10.9575972794973,-234.90005));
#211226=CARTESIAN_POINT('',(10.075,19.0631368321642,-235.35005));
#211227=CARTESIAN_POINT('Origin',(8.87499999999986,10.9575972794973,-234.90005));
#211228=CARTESIAN_POINT('Origin',(8.87499999999986,10.9575972794973,-234.90005));
#211229=CARTESIAN_POINT('Origin',(8.87499999999986,10.9575972794973,-235.35005));
#211230=CARTESIAN_POINT('Origin',(1.25,8.45759727949731,-234.90005));
#211231=CARTESIAN_POINT('',(1.25,9.65759727949731,-235.35005));
#211232=CARTESIAN_POINT('',(1.25,9.20759727949731,-234.90005));
#211233=CARTESIAN_POINT('Origin',(1.25,9.65759727949731,-234.90005));
#211234=CARTESIAN_POINT('',(0.5,8.45759727949731,-234.90005));
#211235=CARTESIAN_POINT('Origin',(1.25,8.45759727949731,-234.90005));
#211236=CARTESIAN_POINT('',(0.0499999999999966,8.45759727949731,-235.35005));
#211237=CARTESIAN_POINT('Origin',(0.0499999999999987,8.45759727949731,-234.90005));
#211238=CARTESIAN_POINT('Origin',(1.25,8.45759727949731,-235.35005));
#211239=CARTESIAN_POINT('Origin',(0.0499999999999945,-25.4138432731711,
-234.90005));
#211240=CARTESIAN_POINT('',(0.5,2.29555713691451,-234.90005));
#211241=CARTESIAN_POINT('',(0.0499999999999962,2.29555713691451,-235.35005));
#211242=CARTESIAN_POINT('Origin',(0.0499999999999985,2.29555713691451,-234.90005));
#211243=CARTESIAN_POINT('',(0.0499999999999962,2.29555713691451,-235.35005));
#211244=CARTESIAN_POINT('',(0.5,8.45759727949731,-234.90005));
#211245=CARTESIAN_POINT('Origin',(-296.501483394397,9.65759727949727,-234.90005));
#211246=CARTESIAN_POINT('',(8.87499999999986,9.65759727949731,-235.35005));
#211247=CARTESIAN_POINT('',(8.87499999999986,9.20759727949731,-234.90005));
#211248=CARTESIAN_POINT('Origin',(8.87499999999986,9.65759727949731,-234.90005));
#211249=CARTESIAN_POINT('',(-2.8425373731103E-15,9.20759727949731,-234.90005));
#211250=CARTESIAN_POINT('',(-296.501483394397,9.65759727949727,-235.35005));
#211251=CARTESIAN_POINT('Origin',(1.25,2.29555713691451,-234.90005));
#211252=CARTESIAN_POINT('',(1.18233753211584,1.54861551239502,-234.90005));
#211253=CARTESIAN_POINT('',(1.14174005138535,1.10045053768332,-235.35005));
#211254=CARTESIAN_POINT('Origin',(1.14174005138535,1.10045053768332,-234.90005));
#211255=CARTESIAN_POINT('Origin',(1.25,2.29555713691451,-235.35005));
#211256=CARTESIAN_POINT('Origin',(1.25,2.29555713691451,-234.90005));
#211257=CARTESIAN_POINT('Origin',(8.87499999999986,8.45759727949731,-234.90005));
#211258=CARTESIAN_POINT('',(10.075,8.45759727949731,-235.35005));
#211259=CARTESIAN_POINT('',(9.62499999999986,8.45759727949731,-234.90005));
#211260=CARTESIAN_POINT('Origin',(10.075,8.45759727949731,-234.90005));
#211261=CARTESIAN_POINT('Origin',(8.87499999999986,8.45759727949731,-234.90005));
#211262=CARTESIAN_POINT('Origin',(8.87499999999986,8.45759727949731,-235.35005));
#211263=CARTESIAN_POINT('Origin',(0.,-11.5034818258363,-234.90005));
#211264=CARTESIAN_POINT('',(5.33358654455957,0.46765101689032,-234.90005));
#211265=CARTESIAN_POINT('',(5.1504491822704,0.0566027149430096,-235.35005));
#211266=CARTESIAN_POINT('Origin',(5.1504491822704,0.0566027149430111,-234.90005));
#211267=CARTESIAN_POINT('Origin',(0.,-11.5034818258363,-235.35005));
#211268=CARTESIAN_POINT('Origin',(0.,-11.5034818258363,-234.90005));
#211269=CARTESIAN_POINT('Origin',(10.075,-25.4138432731712,-234.90005));
#211270=CARTESIAN_POINT('',(10.0749999999998,0.367156910880383,-235.35005));
#211271=CARTESIAN_POINT('',(9.62499999999985,0.367156910880383,-234.90005));
#211272=CARTESIAN_POINT('Origin',(10.0749999999998,0.367156910880383,-234.90005));
#211273=CARTESIAN_POINT('',(9.62499999999985,0.367156910880385,-234.90005));
#211274=CARTESIAN_POINT('',(10.075,8.45759727949732,-235.35005));
#211275=CARTESIAN_POINT('Origin',(9.40330570654115,9.60205772683049,-234.90005));
#211276=CARTESIAN_POINT('',(8.83216440217218,-0.38161883095341,-234.90005));
#211277=CARTESIAN_POINT('',(8.80646304347558,-0.830884276053686,-235.35005));
#211278=CARTESIAN_POINT('Origin',(8.80646304347558,-0.830884276053684,-234.90005));
#211279=CARTESIAN_POINT('Origin',(9.40330570654115,9.60205772683049,-235.35005));
#211280=CARTESIAN_POINT('Origin',(9.40330570654115,9.60205772683049,-234.90005));
#211281=CARTESIAN_POINT('Origin',(8.87499999999985,0.367156910880384,-234.90005));
#211282=CARTESIAN_POINT('Origin',(8.87499999999985,0.367156910880384,-235.35005));
#211283=CARTESIAN_POINT('Origin',(8.87499999999985,0.367156910880384,-234.90005));
#211284=CARTESIAN_POINT('Origin',(11.3749999999999,8.45759727949731,-234.90005));
#211285=CARTESIAN_POINT('',(11.3749999999999,9.65759727949731,-235.35005));
#211286=CARTESIAN_POINT('',(11.3749999999999,9.20759727949731,-234.90005));
#211287=CARTESIAN_POINT('Origin',(11.3749999999999,9.65759727949731,-234.90005));
#211288=CARTESIAN_POINT('',(10.6249999999999,8.45759727949731,-234.90005));
#211289=CARTESIAN_POINT('Origin',(11.3749999999999,8.45759727949731,-234.90005));
#211290=CARTESIAN_POINT('',(10.1749999999999,8.45759727949731,-235.35005));
#211291=CARTESIAN_POINT('Origin',(10.1749999999999,8.45759727949731,-234.90005));
#211292=CARTESIAN_POINT('Origin',(11.3749999999999,8.45759727949731,-235.35005));
#211293=CARTESIAN_POINT('Origin',(10.1749999999999,-25.4138432731711,-234.90005));
#211294=CARTESIAN_POINT('',(10.6249999999999,0.352057726830487,-234.90005));
#211295=CARTESIAN_POINT('',(10.1749999999999,0.352057726830488,-235.35005));
#211296=CARTESIAN_POINT('Origin',(10.1749999999999,0.352057726830487,-234.90005));
#211297=CARTESIAN_POINT('',(10.1749999999999,0.352057726830487,-235.35005));
#211298=CARTESIAN_POINT('',(10.6249999999999,8.45759727949731,-234.90005));
#211299=CARTESIAN_POINT('Origin',(-296.501483394397,9.65759727949727,-234.90005));
#211300=CARTESIAN_POINT('',(19.,9.65759727949731,-235.35005));
#211301=CARTESIAN_POINT('',(19.,9.20759727949731,-234.90005));
#211302=CARTESIAN_POINT('Origin',(19.,9.65759727949731,-234.90005));
#211303=CARTESIAN_POINT('',(-2.8425373731103E-15,9.20759727949731,-234.90005));
#211304=CARTESIAN_POINT('',(-296.501483394397,9.65759727949727,-235.35005));
#211305=CARTESIAN_POINT('Origin',(11.3749999999999,0.352057726830487,-234.90005));
#211306=CARTESIAN_POINT('',(11.3749999999999,-0.397942273169513,-234.90005));
#211307=CARTESIAN_POINT('',(11.3749999999999,-0.847942273169513,-235.35005));
#211308=CARTESIAN_POINT('Origin',(11.3749999999999,-0.847942273169513,-234.90005));
#211309=CARTESIAN_POINT('Origin',(11.3749999999999,0.352057726830487,-235.35005));
#211310=CARTESIAN_POINT('Origin',(11.3749999999999,0.352057726830487,-234.90005));
#211311=CARTESIAN_POINT('Origin',(19.,8.45759727949731,-234.90005));
#211312=CARTESIAN_POINT('',(20.2,8.45759727949731,-235.35005));
#211313=CARTESIAN_POINT('',(19.75,8.45759727949731,-234.90005));
#211314=CARTESIAN_POINT('Origin',(20.2,8.45759727949731,-234.90005));
#211315=CARTESIAN_POINT('Origin',(19.,8.45759727949731,-234.90005));
#211316=CARTESIAN_POINT('Origin',(19.,8.45759727949731,-235.35005));
#211317=CARTESIAN_POINT('Origin',(-296.501483394397,-0.84794227316963,-234.90005));
#211318=CARTESIAN_POINT('',(19.,-0.39794227316951,-234.90005));
#211319=CARTESIAN_POINT('',(19.,-0.847942273169513,-235.35005));
#211320=CARTESIAN_POINT('Origin',(19.,-0.84794227316951,-234.90005));
#211321=CARTESIAN_POINT('',(-296.501483394397,-0.84794227316963,-235.35005));
#211322=CARTESIAN_POINT('',(-1.11087130309497E-13,-0.397942273169517,-234.90005));
#211323=CARTESIAN_POINT('Origin',(20.2,-25.4138432731711,-234.90005));
#211324=CARTESIAN_POINT('',(20.2,0.352057726830487,-235.35005));
#211325=CARTESIAN_POINT('',(19.75,0.352057726830487,-234.90005));
#211326=CARTESIAN_POINT('Origin',(20.2,0.352057726830487,-234.90005));
#211327=CARTESIAN_POINT('',(19.75,0.352057726830487,-234.90005));
#211328=CARTESIAN_POINT('',(20.2,8.45759727949731,-235.35005));
#211329=CARTESIAN_POINT('Origin',(19.,0.35205772683049,-234.90005));
#211330=CARTESIAN_POINT('Origin',(19.,0.35205772683049,-234.90005));
#211331=CARTESIAN_POINT('Origin',(19.,0.35205772683049,-235.35005));
#211332=CARTESIAN_POINT('Origin',(11.3749999999999,19.0631368321642,-234.90005));
#211333=CARTESIAN_POINT('',(11.3749999999999,20.2631368321642,-235.35005));
#211334=CARTESIAN_POINT('',(11.3749999999999,19.8131368321642,-234.90005));
#211335=CARTESIAN_POINT('Origin',(11.3749999999999,20.2631368321642,-234.90005));
#211336=CARTESIAN_POINT('',(10.6249999999999,19.0631368321642,-234.90005));
#211337=CARTESIAN_POINT('Origin',(11.3749999999999,19.0631368321642,-234.90005));
#211338=CARTESIAN_POINT('',(10.1749999999999,19.0631368321642,-235.35005));
#211339=CARTESIAN_POINT('Origin',(10.1749999999999,19.0631368321642,-234.90005));
#211340=CARTESIAN_POINT('Origin',(11.3749999999999,19.0631368321642,-235.35005));
#211341=CARTESIAN_POINT('Origin',(10.1749999999999,-25.4138432731711,-234.90005));
#211342=CARTESIAN_POINT('',(10.6249999999999,10.9575972794973,-234.90005));
#211343=CARTESIAN_POINT('',(10.1749999999999,10.9575972794973,-235.35005));
#211344=CARTESIAN_POINT('Origin',(10.1749999999999,10.9575972794973,-234.90005));
#211345=CARTESIAN_POINT('',(10.1749999999999,10.9575972794973,-235.35005));
#211346=CARTESIAN_POINT('',(10.6249999999999,19.0631368321642,-234.90005));
#211347=CARTESIAN_POINT('Origin',(-296.501483394397,20.2631368321643,-234.90005));
#211348=CARTESIAN_POINT('',(19.,20.2631368321642,-235.35005));
#211349=CARTESIAN_POINT('',(19.,19.8131368321642,-234.90005));
#211350=CARTESIAN_POINT('Origin',(19.,20.2631368321642,-234.90005));
#211351=CARTESIAN_POINT('',(-1.54373336646988E-15,19.8131368321642,-234.90005));
#211352=CARTESIAN_POINT('',(-296.501483394397,20.2631368321643,-235.35005));
#211353=CARTESIAN_POINT('Origin',(11.3749999999999,10.9575972794973,-234.90005));
#211354=CARTESIAN_POINT('',(11.3749999999999,10.2075972794973,-234.90005));
#211355=CARTESIAN_POINT('',(11.3749999999999,9.75759727949733,-235.35005));
#211356=CARTESIAN_POINT('Origin',(11.3749999999999,9.75759727949733,-234.90005));
#211357=CARTESIAN_POINT('Origin',(11.3749999999999,10.9575972794973,-235.35005));
#211358=CARTESIAN_POINT('Origin',(11.3749999999999,10.9575972794973,-234.90005));
#211359=CARTESIAN_POINT('Origin',(19.,19.0631368321642,-234.90005));
#211360=CARTESIAN_POINT('',(20.2,19.0631368321642,-235.35005));
#211361=CARTESIAN_POINT('',(19.75,19.0631368321642,-234.90005));
#211362=CARTESIAN_POINT('Origin',(20.2,19.0631368321642,-234.90005));
#211363=CARTESIAN_POINT('Origin',(19.,19.0631368321642,-234.90005));
#211364=CARTESIAN_POINT('Origin',(19.,19.0631368321642,-235.35005));
#211365=CARTESIAN_POINT('Origin',(-296.501483394397,9.75759727949737,-234.90005));
#211366=CARTESIAN_POINT('',(19.,10.2075972794973,-234.90005));
#211367=CARTESIAN_POINT('',(19.,9.75759727949733,-235.35005));
#211368=CARTESIAN_POINT('Origin',(19.,9.75759727949733,-234.90005));
#211369=CARTESIAN_POINT('',(-296.501483394397,9.75759727949737,-235.35005));
#211370=CARTESIAN_POINT('',(-2.53637567332344E-15,10.2075972794973,-234.90005));
#211371=CARTESIAN_POINT('Origin',(20.2,-25.4138432731711,-234.90005));
#211372=CARTESIAN_POINT('',(20.2,10.9575972794973,-235.35005));
#211373=CARTESIAN_POINT('',(19.75,10.9575972794973,-234.90005));
#211374=CARTESIAN_POINT('Origin',(20.2,10.9575972794973,-234.90005));
#211375=CARTESIAN_POINT('',(19.75,10.9575972794973,-234.90005));
#211376=CARTESIAN_POINT('',(20.2,19.0631368321642,-235.35005));
#211377=CARTESIAN_POINT('Origin',(19.,10.9575972794973,-234.90005));
#211378=CARTESIAN_POINT('Origin',(19.,10.9575972794973,-234.90005));
#211379=CARTESIAN_POINT('Origin',(19.,10.9575972794973,-235.35005));
#211380=CARTESIAN_POINT('Origin',(21.5,19.0631368321642,-234.90005));
#211381=CARTESIAN_POINT('',(21.5,20.2631368321642,-235.35005));
#211382=CARTESIAN_POINT('',(21.5,19.8131368321642,-234.90005));
#211383=CARTESIAN_POINT('Origin',(21.5,20.2631368321642,-234.90005));
#211384=CARTESIAN_POINT('',(20.75,19.0631368321642,-234.90005));
#211385=CARTESIAN_POINT('Origin',(21.5,19.0631368321642,-234.90005));
#211386=CARTESIAN_POINT('',(20.3,19.0631368321642,-235.35005));
#211387=CARTESIAN_POINT('Origin',(20.3,19.0631368321642,-234.90005));
#211388=CARTESIAN_POINT('Origin',(21.5,19.0631368321642,-235.35005));
#211389=CARTESIAN_POINT('Origin',(20.3,-25.4138432731711,-234.90005));
#211390=CARTESIAN_POINT('',(20.75,10.9575972794973,-234.90005));
#211391=CARTESIAN_POINT('',(20.3,10.9575972794973,-235.35005));
#211392=CARTESIAN_POINT('Origin',(20.3,10.9575972794973,-234.90005));
#211393=CARTESIAN_POINT('',(20.3,10.9575972794973,-235.35005));
#211394=CARTESIAN_POINT('',(20.75,19.0631368321642,-234.90005));
#211395=CARTESIAN_POINT('Origin',(-296.501483394397,20.2631368321643,-234.90005));
#211396=CARTESIAN_POINT('',(29.125,20.2631368321642,-235.35005));
#211397=CARTESIAN_POINT('',(29.125,19.8131368321642,-234.90005));
#211398=CARTESIAN_POINT('Origin',(29.125,20.2631368321642,-234.90005));
#211399=CARTESIAN_POINT('',(-1.54373336646988E-15,19.8131368321642,-234.90005));
#211400=CARTESIAN_POINT('',(-296.501483394397,20.2631368321643,-235.35005));
#211401=CARTESIAN_POINT('Origin',(21.5,10.9575972794973,-234.90005));
#211402=CARTESIAN_POINT('',(21.5,10.2075972794973,-234.90005));
#211403=CARTESIAN_POINT('',(21.5,9.75759727949733,-235.35005));
#211404=CARTESIAN_POINT('Origin',(21.5,9.75759727949733,-234.90005));
#211405=CARTESIAN_POINT('Origin',(21.5,10.9575972794973,-235.35005));
#211406=CARTESIAN_POINT('Origin',(21.5,10.9575972794973,-234.90005));
#211407=CARTESIAN_POINT('Origin',(29.125,19.0631368321642,-234.90005));
#211408=CARTESIAN_POINT('',(30.325,19.0631368321642,-235.35005));
#211409=CARTESIAN_POINT('',(29.875,19.0631368321642,-234.90005));
#211410=CARTESIAN_POINT('Origin',(30.325,19.0631368321642,-234.90005));
#211411=CARTESIAN_POINT('Origin',(29.125,19.0631368321642,-234.90005));
#211412=CARTESIAN_POINT('Origin',(29.125,19.0631368321642,-235.35005));
#211413=CARTESIAN_POINT('Origin',(-296.501483394397,9.75759727949737,-234.90005));
#211414=CARTESIAN_POINT('',(29.125,10.2075972794973,-234.90005));
#211415=CARTESIAN_POINT('',(29.125,9.75759727949733,-235.35005));
#211416=CARTESIAN_POINT('Origin',(29.125,9.75759727949733,-234.90005));
#211417=CARTESIAN_POINT('',(-296.501483394397,9.75759727949737,-235.35005));
#211418=CARTESIAN_POINT('',(-2.53637567332344E-15,10.2075972794973,-234.90005));
#211419=CARTESIAN_POINT('Origin',(30.325,-25.4138432731711,-234.90005));
#211420=CARTESIAN_POINT('',(30.325,10.9575972794973,-235.35005));
#211421=CARTESIAN_POINT('',(29.875,10.9575972794973,-234.90005));
#211422=CARTESIAN_POINT('Origin',(30.325,10.9575972794973,-234.90005));
#211423=CARTESIAN_POINT('',(29.875,10.9575972794973,-234.90005));
#211424=CARTESIAN_POINT('',(30.325,19.0631368321642,-235.35005));
#211425=CARTESIAN_POINT('Origin',(29.125,10.9575972794973,-234.90005));
#211426=CARTESIAN_POINT('Origin',(29.125,10.9575972794973,-234.90005));
#211427=CARTESIAN_POINT('Origin',(29.125,10.9575972794973,-235.35005));
#211428=CARTESIAN_POINT('Origin',(21.5,8.45759727949731,-234.90005));
#211429=CARTESIAN_POINT('',(21.5,9.65759727949731,-235.35005));
#211430=CARTESIAN_POINT('',(21.5,9.20759727949731,-234.90005));
#211431=CARTESIAN_POINT('Origin',(21.5,9.65759727949731,-234.90005));
#211432=CARTESIAN_POINT('',(20.75,8.45759727949731,-234.90005));
#211433=CARTESIAN_POINT('Origin',(21.5,8.45759727949731,-234.90005));
#211434=CARTESIAN_POINT('',(20.3,8.45759727949731,-235.35005));
#211435=CARTESIAN_POINT('Origin',(20.3,8.45759727949731,-234.90005));
#211436=CARTESIAN_POINT('Origin',(21.5,8.45759727949731,-235.35005));
#211437=CARTESIAN_POINT('Origin',(20.3,-25.4138432731711,-234.90005));
#211438=CARTESIAN_POINT('',(20.75,0.352057726830487,-234.90005));
#211439=CARTESIAN_POINT('',(20.3,0.352057726830486,-235.35005));
#211440=CARTESIAN_POINT('Origin',(20.3,0.352057726830486,-234.90005));
#211441=CARTESIAN_POINT('',(20.3,0.352057726830487,-235.35005));
#211442=CARTESIAN_POINT('',(20.75,8.45759727949731,-234.90005));
#211443=CARTESIAN_POINT('Origin',(-296.501483394397,9.65759727949727,-234.90005));
#211444=CARTESIAN_POINT('',(29.125,9.65759727949731,-235.35005));
#211445=CARTESIAN_POINT('',(29.125,9.20759727949731,-234.90005));
#211446=CARTESIAN_POINT('Origin',(29.125,9.65759727949731,-234.90005));
#211447=CARTESIAN_POINT('',(-2.8425373731103E-15,9.20759727949731,-234.90005));
#211448=CARTESIAN_POINT('',(-296.501483394397,9.65759727949727,-235.35005));
#211449=CARTESIAN_POINT('Origin',(21.5,0.352057726830491,-234.90005));
#211450=CARTESIAN_POINT('',(21.5,-0.397942273169509,-234.90005));
#211451=CARTESIAN_POINT('',(21.5,-0.847942273169509,-235.35005));
#211452=CARTESIAN_POINT('Origin',(21.5,-0.847942273169509,-234.90005));
#211453=CARTESIAN_POINT('Origin',(21.5,0.352057726830491,-235.35005));
#211454=CARTESIAN_POINT('Origin',(21.5,0.352057726830491,-234.90005));
#211455=CARTESIAN_POINT('Origin',(29.125,8.45759727949731,-234.90005));
#211456=CARTESIAN_POINT('',(30.325,8.45759727949731,-235.35005));
#211457=CARTESIAN_POINT('',(29.875,8.45759727949731,-234.90005));
#211458=CARTESIAN_POINT('Origin',(30.325,8.45759727949731,-234.90005));
#211459=CARTESIAN_POINT('Origin',(29.125,8.45759727949731,-234.90005));
#211460=CARTESIAN_POINT('Origin',(29.125,8.45759727949731,-235.35005));
#211461=CARTESIAN_POINT('Origin',(-296.501483394397,-0.84794227316963,-234.90005));
#211462=CARTESIAN_POINT('',(29.125,-0.397942273169507,-234.90005));
#211463=CARTESIAN_POINT('',(29.125,-0.847942273169509,-235.35005));
#211464=CARTESIAN_POINT('Origin',(29.125,-0.847942273169506,-234.90005));
#211465=CARTESIAN_POINT('',(-296.501483394397,-0.84794227316963,-235.35005));
#211466=CARTESIAN_POINT('',(-1.11087130309497E-13,-0.397942273169517,-234.90005));
#211467=CARTESIAN_POINT('Origin',(30.325,-25.4138432731711,-234.90005));
#211468=CARTESIAN_POINT('',(30.325,0.352057726830494,-235.35005));
#211469=CARTESIAN_POINT('',(29.875,0.352057726830494,-234.90005));
#211470=CARTESIAN_POINT('Origin',(30.325,0.352057726830494,-234.90005));
#211471=CARTESIAN_POINT('',(29.875,0.352057726830494,-234.90005));
#211472=CARTESIAN_POINT('',(30.325,8.45759727949732,-235.35005));
#211473=CARTESIAN_POINT('Origin',(29.125,0.352057726830494,-234.90005));
#211474=CARTESIAN_POINT('Origin',(29.125,0.352057726830494,-234.90005));
#211475=CARTESIAN_POINT('Origin',(29.125,0.352057726830494,-235.35005));
#211476=CARTESIAN_POINT('Origin',(31.625,8.45759727949731,-234.90005));
#211477=CARTESIAN_POINT('',(31.625,9.65759727949731,-235.35005));
#211478=CARTESIAN_POINT('',(31.625,9.20759727949731,-234.90005));
#211479=CARTESIAN_POINT('Origin',(31.625,9.65759727949731,-234.90005));
#211480=CARTESIAN_POINT('',(30.875,8.45759727949731,-234.90005));
#211481=CARTESIAN_POINT('Origin',(31.625,8.45759727949731,-234.90005));
#211482=CARTESIAN_POINT('',(30.425,8.45759727949731,-235.35005));
#211483=CARTESIAN_POINT('Origin',(30.425,8.45759727949731,-234.90005));
#211484=CARTESIAN_POINT('Origin',(31.625,8.45759727949731,-235.35005));
#211485=CARTESIAN_POINT('Origin',(30.425,-25.4138432731711,-234.90005));
#211486=CARTESIAN_POINT('',(30.875,0.352057726830494,-234.90005));
#211487=CARTESIAN_POINT('',(30.425,0.352057726830494,-235.35005));
#211488=CARTESIAN_POINT('Origin',(30.425,0.352057726830494,-234.90005));
#211489=CARTESIAN_POINT('',(30.425,0.352057726830494,-235.35005));
#211490=CARTESIAN_POINT('',(30.875,8.45759727949732,-234.90005));
#211491=CARTESIAN_POINT('Origin',(-296.501483394397,9.65759727949727,-234.90005));
#211492=CARTESIAN_POINT('',(39.4555265729267,9.65759727949731,-235.35005));
#211493=CARTESIAN_POINT('',(39.4555265729267,9.20759727949731,-234.90005));
#211494=CARTESIAN_POINT('Origin',(39.4555265729267,9.65759727949731,-234.90005));
#211495=CARTESIAN_POINT('',(-2.8425373731103E-15,9.20759727949731,-234.90005));
#211496=CARTESIAN_POINT('',(-296.501483394397,9.65759727949727,-235.35005));
#211497=CARTESIAN_POINT('Origin',(31.625,0.352057726830494,-234.90005));
#211498=CARTESIAN_POINT('',(31.625,-0.397942273169506,-234.90005));
#211499=CARTESIAN_POINT('',(31.625,-0.847942273169506,-235.35005));
#211500=CARTESIAN_POINT('Origin',(31.625,-0.847942273169505,-234.90005));
#211501=CARTESIAN_POINT('Origin',(31.625,0.352057726830495,-235.35005));
#211502=CARTESIAN_POINT('Origin',(31.625,0.352057726830494,-234.90005));
#211503=CARTESIAN_POINT('Origin',(39.4555265729267,8.45759727949731,-234.90005));
#211504=CARTESIAN_POINT('',(40.6550043680477,8.49299528808125,-235.35005));
#211505=CARTESIAN_POINT('',(40.2052001948774,8.47972103486227,-234.90005));
#211506=CARTESIAN_POINT('Origin',(40.6550043680477,8.49299528808125,-234.90005));
#211507=CARTESIAN_POINT('Origin',(39.4555265729267,8.45759727949731,-234.90005));
#211508=CARTESIAN_POINT('Origin',(39.4555265729267,8.45759727949731,-235.35005));
#211509=CARTESIAN_POINT('Origin',(-296.501483394397,-0.84794227316963,-234.90005));
#211510=CARTESIAN_POINT('',(39.6461373136998,-0.397942273169503,-234.90005));
#211511=CARTESIAN_POINT('',(39.6461373136998,-0.847942273169505,-235.35005));
#211512=CARTESIAN_POINT('Origin',(39.6461373136998,-0.847942273169502,-234.90005));
#211513=CARTESIAN_POINT('',(-296.501483394397,-0.84794227316963,-235.35005));
#211514=CARTESIAN_POINT('',(-1.11087130309497E-13,-0.397942273169517,-234.90005));
#211515=CARTESIAN_POINT('Origin',(-636.934816028482,-11.5034818258361,-234.90005));
#211516=CARTESIAN_POINT('',(40.8459531286544,0.37308176509206,-235.35005));
#211517=CARTESIAN_POINT('',(40.3960221980464,0.365197750743974,-234.90005));
#211518=CARTESIAN_POINT('Origin',(40.8459531286544,0.37308176509206,-234.90005));
#211519=CARTESIAN_POINT('Origin',(-636.934816028482,-11.5034818258361,-234.90005));
#211520=CARTESIAN_POINT('Origin',(-636.934816028482,-11.5034818258361,-235.35005));
#211521=CARTESIAN_POINT('Origin',(39.6461373136998,0.352057726830498,-234.90005));
#211522=CARTESIAN_POINT('Origin',(39.6461373136998,0.352057726830498,-234.90005));
#211523=CARTESIAN_POINT('Origin',(39.6461373136998,0.352057726830498,-235.35005));
#211524=CARTESIAN_POINT('Origin',(31.625,19.0631368321642,-234.90005));
#211525=CARTESIAN_POINT('',(31.625,20.2631368321642,-235.35005));
#211526=CARTESIAN_POINT('',(31.625,19.8131368321642,-234.90005));
#211527=CARTESIAN_POINT('Origin',(31.625,20.2631368321642,-234.90005));
#211528=CARTESIAN_POINT('',(30.875,19.0631368321642,-234.90005));
#211529=CARTESIAN_POINT('Origin',(31.625,19.0631368321642,-234.90005));
#211530=CARTESIAN_POINT('',(30.425,19.0631368321642,-235.35005));
#211531=CARTESIAN_POINT('Origin',(30.425,19.0631368321642,-234.90005));
#211532=CARTESIAN_POINT('Origin',(31.625,19.0631368321642,-235.35005));
#211533=CARTESIAN_POINT('Origin',(30.425,-25.4138432731711,-234.90005));
#211534=CARTESIAN_POINT('',(30.875,10.9575972794973,-234.90005));
#211535=CARTESIAN_POINT('',(30.425,10.9575972794973,-235.35005));
#211536=CARTESIAN_POINT('Origin',(30.425,10.9575972794973,-234.90005));
#211537=CARTESIAN_POINT('',(30.425,10.9575972794973,-235.35005));
#211538=CARTESIAN_POINT('',(30.875,19.0631368321642,-234.90005));
#211539=CARTESIAN_POINT('Origin',(-296.501483394397,20.2631368321643,-234.90005));
#211540=CARTESIAN_POINT('',(36.0311576807679,20.2631368321642,-235.35005));
#211541=CARTESIAN_POINT('',(36.0311576807679,19.8131368321642,-234.90005));
#211542=CARTESIAN_POINT('Origin',(36.0311576807679,20.2631368321642,-234.90005));
#211543=CARTESIAN_POINT('',(-1.54373336646988E-15,19.8131368321642,-234.90005));
#211544=CARTESIAN_POINT('',(-296.501483394397,20.2631368321643,-235.35005));
#211545=CARTESIAN_POINT('Origin',(31.625,10.9575972794973,-234.90005));
#211546=CARTESIAN_POINT('',(31.625,10.2075972794973,-234.90005));
#211547=CARTESIAN_POINT('',(31.625,9.75759727949733,-235.35005));
#211548=CARTESIAN_POINT('Origin',(31.625,9.75759727949733,-234.90005));
#211549=CARTESIAN_POINT('Origin',(31.625,10.9575972794973,-235.35005));
#211550=CARTESIAN_POINT('Origin',(31.625,10.9575972794973,-234.90005));
#211551=CARTESIAN_POINT('Origin',(36.0311576807679,19.0631368321642,-234.90005));
#211552=CARTESIAN_POINT('',(36.9462347012319,19.8394319091927,-235.35005));
#211553=CARTESIAN_POINT('',(36.6030808185579,19.548321255307,-234.90005));
#211554=CARTESIAN_POINT('Origin',(36.9462347012319,19.8394319091927,-234.90005));
#211555=CARTESIAN_POINT('Origin',(36.0311576807679,19.0631368321642,-234.90005));
#211556=CARTESIAN_POINT('Origin',(36.0311576807679,19.0631368321642,-235.35005));
#211557=CARTESIAN_POINT('Origin',(-296.501483394397,9.75759727949737,-234.90005));
#211558=CARTESIAN_POINT('',(39.3771239584772,10.2075972794973,-234.90005));
#211559=CARTESIAN_POINT('',(39.3771239584772,9.75759727949732,-235.35005));
#211560=CARTESIAN_POINT('Origin',(39.3771239584772,9.75759727949733,-234.90005));
#211561=CARTESIAN_POINT('',(-296.501483394397,9.75759727949737,-235.35005));
#211562=CARTESIAN_POINT('',(-2.53637567332344E-15,10.2075972794973,-234.90005));
#211563=CARTESIAN_POINT('Origin',(-6.29739814579425E-15,-11.5034818258363,
-234.90005));
#211564=CARTESIAN_POINT('',(40.1936303108393,15.5496988085284,-235.35005));
#211565=CARTESIAN_POINT('',(39.8203148590359,15.2984308769399,-234.90005));
#211566=CARTESIAN_POINT('Origin',(40.1936303108393,15.5496988085284,-234.90005));
#211567=CARTESIAN_POINT('Origin',(-6.29739814579425E-15,-11.5034818258363,
-234.90005));
#211568=CARTESIAN_POINT('Origin',(-6.29739814579425E-15,-11.5034818258363,
-235.35005));
#211569=CARTESIAN_POINT('Origin',(39.3771239584772,10.9575972794973,-234.90005));
#211570=CARTESIAN_POINT('',(40.1267106833092,10.9824918965036,-234.90005));
#211571=CARTESIAN_POINT('',(40.5764627182082,10.9974286667074,-235.35005));
#211572=CARTESIAN_POINT('Origin',(40.5764627182083,10.9974286667074,-234.90005));
#211573=CARTESIAN_POINT('Origin',(39.3771239584772,10.9575972794973,-235.35005));
#211574=CARTESIAN_POINT('Origin',(39.3771239584772,10.9575972794973,-234.90005));
#211575=CARTESIAN_POINT('Origin',(38.9907249661392,14.740057695632,-234.90005));
#211576=CARTESIAN_POINT('',(40.4396332884467,14.7963131269086,-235.35005));
#211577=CARTESIAN_POINT('',(39.989972084972,14.7788545447883,-234.90005));
#211578=CARTESIAN_POINT('Origin',(40.4396332884467,14.7963131269086,-234.90005));
#211579=CARTESIAN_POINT('Origin',(38.9907249661392,14.740057695632,-234.90005));
#211580=CARTESIAN_POINT('Origin',(38.9907249661392,14.740057695632,-235.35005));
#211581=CARTESIAN_POINT('Origin',(-636.934816028482,-11.5034818258361,-234.90005));
#211582=CARTESIAN_POINT('Origin',(-636.934816028482,-11.5034818258361,-234.90005));
#211583=CARTESIAN_POINT('Origin',(-636.934816028482,-11.5034818258361,-235.35005));
#211584=CARTESIAN_POINT('Origin',(31.625,-2.14794227316952,-234.90005));
#211585=CARTESIAN_POINT('',(31.625,-0.947942273169512,-235.35005));
#211586=CARTESIAN_POINT('',(31.625,-1.39794227316951,-234.90005));
#211587=CARTESIAN_POINT('Origin',(31.625,-0.947942273169512,-234.90005));
#211588=CARTESIAN_POINT('',(30.875,-2.14794227316951,-234.90005));
#211589=CARTESIAN_POINT('Origin',(31.625,-2.14794227316952,-234.90005));
#211590=CARTESIAN_POINT('',(30.425,-2.14794227316951,-235.35005));
#211591=CARTESIAN_POINT('Origin',(30.425,-2.14794227316951,-234.90005));
#211592=CARTESIAN_POINT('Origin',(31.625,-2.14794227316952,-235.35005));
#211593=CARTESIAN_POINT('Origin',(30.425,-25.4138432731711,-234.90005));
#211594=CARTESIAN_POINT('',(30.875,-10.2534818258363,-234.90005));
#211595=CARTESIAN_POINT('',(30.425,-10.2534818258363,-235.35005));
#211596=CARTESIAN_POINT('Origin',(30.425,-10.2534818258363,-234.90005));
#211597=CARTESIAN_POINT('',(30.425,-10.2534818258363,-235.35005));
#211598=CARTESIAN_POINT('',(30.875,-2.14794227316951,-234.90005));
#211599=CARTESIAN_POINT('Origin',(-296.501483394397,-0.94794227316939,-234.90005));
#211600=CARTESIAN_POINT('',(39.6853241707135,-0.947942273169515,-235.35005));
#211601=CARTESIAN_POINT('',(39.6853241707135,-1.39794227316951,-234.90005));
#211602=CARTESIAN_POINT('Origin',(39.6853241707135,-0.947942273169515,-234.90005));
#211603=CARTESIAN_POINT('',(-1.11087130309497E-13,-1.3979422731695,-234.90005));
#211604=CARTESIAN_POINT('',(-296.501483394397,-0.94794227316939,-235.35005));
#211605=CARTESIAN_POINT('Origin',(31.625,-10.2534818258363,-234.90005));
#211606=CARTESIAN_POINT('',(31.625,-11.0034818258363,-234.90005));
#211607=CARTESIAN_POINT('',(31.625,-11.4534818258363,-235.35005));
#211608=CARTESIAN_POINT('Origin',(31.625,-11.4534818258363,-234.90005));
#211609=CARTESIAN_POINT('Origin',(31.625,-10.2534818258363,-235.35005));
#211610=CARTESIAN_POINT('Origin',(31.625,-10.2534818258363,-234.90005));
#211611=CARTESIAN_POINT('Origin',(39.6853241707135,-2.14794227316952,-234.90005));
#211612=CARTESIAN_POINT('',(40.8852094777378,-2.13135161353407,-235.35005));
#211613=CARTESIAN_POINT('',(40.4352524876037,-2.13757311089736,-234.90005));
#211614=CARTESIAN_POINT('Origin',(40.8852094777378,-2.13135161353407,-234.90005));
#211615=CARTESIAN_POINT('Origin',(39.6853241707135,-2.14794227316952,-234.90005));
#211616=CARTESIAN_POINT('Origin',(39.6853241707135,-2.14794227316952,-235.35005));
#211617=CARTESIAN_POINT('Origin',(-296.501483394397,-11.4534818258365,-234.90005));
#211618=CARTESIAN_POINT('',(39.7488454733312,-11.0034818258363,-234.90005));
#211619=CARTESIAN_POINT('',(39.7488454733312,-11.4534818258363,-235.35005));
#211620=CARTESIAN_POINT('Origin',(39.7488454733312,-11.4534818258363,-234.90005));
#211621=CARTESIAN_POINT('',(-296.501483394397,-11.4534818258365,-235.35005));
#211622=CARTESIAN_POINT('',(-2.22174260618994E-13,-11.0034818258363,-234.90005));
#211623=CARTESIAN_POINT('Origin',(-636.934816028482,-11.5034818258361,-234.90005));
#211624=CARTESIAN_POINT('',(40.9488434259496,-10.2512651365233,-235.35005));
#211625=CARTESIAN_POINT('',(40.4988441937178,-10.2520963950157,-234.90005));
#211626=CARTESIAN_POINT('Origin',(40.9488434259496,-10.2512651365233,-234.90005));
#211627=CARTESIAN_POINT('Origin',(-636.934816028482,-11.5034818258361,-234.90005));
#211628=CARTESIAN_POINT('Origin',(-636.934816028482,-11.5034818258361,-235.35005));
#211629=CARTESIAN_POINT('Origin',(39.7488454733312,-10.2534818258363,-234.90005));
#211630=CARTESIAN_POINT('Origin',(39.7488454733312,-10.2534818258363,-234.90005));
#211631=CARTESIAN_POINT('Origin',(39.7488454733312,-10.2534818258363,-235.35005));
#211632=CARTESIAN_POINT('Origin',(21.5,-2.14794227316951,-234.90005));
#211633=CARTESIAN_POINT('',(21.5,-0.947942273169508,-235.35005));
#211634=CARTESIAN_POINT('',(21.5,-1.39794227316951,-234.90005));
#211635=CARTESIAN_POINT('Origin',(21.5,-0.947942273169508,-234.90005));
#211636=CARTESIAN_POINT('',(20.75,-2.14794227316951,-234.90005));
#211637=CARTESIAN_POINT('Origin',(21.5,-2.14794227316951,-234.90005));
#211638=CARTESIAN_POINT('',(20.3,-2.14794227316951,-235.35005));
#211639=CARTESIAN_POINT('Origin',(20.3,-2.14794227316951,-234.90005));
#211640=CARTESIAN_POINT('Origin',(21.5,-2.14794227316951,-235.35005));
#211641=CARTESIAN_POINT('Origin',(20.3,-25.4138432731711,-234.90005));
#211642=CARTESIAN_POINT('',(20.75,-10.2534818258363,-234.90005));
#211643=CARTESIAN_POINT('',(20.3,-10.2534818258363,-235.35005));
#211644=CARTESIAN_POINT('Origin',(20.3,-10.2534818258363,-234.90005));
#211645=CARTESIAN_POINT('',(20.3,-10.2534818258363,-235.35005));
#211646=CARTESIAN_POINT('',(20.75,-2.14794227316951,-234.90005));
#211647=CARTESIAN_POINT('Origin',(-296.501483394397,-0.94794227316939,-234.90005));
#211648=CARTESIAN_POINT('',(29.125,-0.947942273169511,-235.35005));
#211649=CARTESIAN_POINT('',(29.125,-1.39794227316951,-234.90005));
#211650=CARTESIAN_POINT('Origin',(29.125,-0.947942273169511,-234.90005));
#211651=CARTESIAN_POINT('',(-1.11087130309497E-13,-1.3979422731695,-234.90005));
#211652=CARTESIAN_POINT('',(-296.501483394397,-0.94794227316939,-235.35005));
#211653=CARTESIAN_POINT('Origin',(21.5,-10.2534818258363,-234.90005));
#211654=CARTESIAN_POINT('',(21.5,-11.0034818258363,-234.90005));
#211655=CARTESIAN_POINT('',(21.5,-11.4534818258363,-235.35005));
#211656=CARTESIAN_POINT('Origin',(21.5,-11.4534818258363,-234.90005));
#211657=CARTESIAN_POINT('Origin',(21.5,-10.2534818258363,-235.35005));
#211658=CARTESIAN_POINT('Origin',(21.5,-10.2534818258363,-234.90005));
#211659=CARTESIAN_POINT('Origin',(29.125,-2.14794227316951,-234.90005));
#211660=CARTESIAN_POINT('',(30.325,-2.14794227316951,-235.35005));
#211661=CARTESIAN_POINT('',(29.875,-2.14794227316951,-234.90005));
#211662=CARTESIAN_POINT('Origin',(30.325,-2.14794227316951,-234.90005));
#211663=CARTESIAN_POINT('Origin',(29.125,-2.14794227316951,-234.90005));
#211664=CARTESIAN_POINT('Origin',(29.125,-2.14794227316951,-235.35005));
#211665=CARTESIAN_POINT('Origin',(-296.501483394397,-11.4534818258365,-234.90005));
#211666=CARTESIAN_POINT('',(29.125,-11.0034818258363,-234.90005));
#211667=CARTESIAN_POINT('',(29.125,-11.4534818258363,-235.35005));
#211668=CARTESIAN_POINT('Origin',(29.125,-11.4534818258363,-234.90005));
#211669=CARTESIAN_POINT('',(-296.501483394397,-11.4534818258365,-235.35005));
#211670=CARTESIAN_POINT('',(-2.22174260618994E-13,-11.0034818258363,-234.90005));
#211671=CARTESIAN_POINT('Origin',(30.325,-25.4138432731711,-234.90005));
#211672=CARTESIAN_POINT('',(30.325,-10.2534818258363,-235.35005));
#211673=CARTESIAN_POINT('',(29.875,-10.2534818258363,-234.90005));
#211674=CARTESIAN_POINT('Origin',(30.325,-10.2534818258363,-234.90005));
#211675=CARTESIAN_POINT('',(29.875,-10.2534818258363,-234.90005));
#211676=CARTESIAN_POINT('',(30.325,-2.14794227316951,-235.35005));
#211677=CARTESIAN_POINT('Origin',(29.125,-10.2534818258363,-234.90005));
#211678=CARTESIAN_POINT('Origin',(29.125,-10.2534818258363,-234.90005));
#211679=CARTESIAN_POINT('Origin',(29.125,-10.2534818258363,-235.35005));
#211680=CARTESIAN_POINT('Origin',(12.7946237611812,-10.2534818258363,-234.90005));
#211681=CARTESIAN_POINT('',(11.6003099441285,-10.370163042821,-235.35005));
#211682=CARTESIAN_POINT('',(12.0481776255232,-10.3264075864518,-234.90005));
#211683=CARTESIAN_POINT('Origin',(11.6003099441285,-10.370163042821,-234.90005));
#211684=CARTESIAN_POINT('',(12.7946237611812,-11.0034818258363,-234.90005));
#211685=CARTESIAN_POINT('Origin',(12.7946237611812,-10.2534818258363,-234.90005));
#211686=CARTESIAN_POINT('',(12.7946237611812,-11.4534818258363,-235.35005));
#211687=CARTESIAN_POINT('Origin',(12.7946237611812,-11.4534818258363,-234.90005));
#211688=CARTESIAN_POINT('Origin',(12.7946237611812,-10.2534818258363,-235.35005));
#211689=CARTESIAN_POINT('Origin',(-296.501483394397,-11.4534818258365,-234.90005));
#211690=CARTESIAN_POINT('',(19.,-11.0034818258363,-234.90005));
#211691=CARTESIAN_POINT('',(19.,-11.4534818258363,-235.35005));
#211692=CARTESIAN_POINT('Origin',(19.,-11.4534818258363,-234.90005));
#211693=CARTESIAN_POINT('',(-296.501483394397,-11.4534818258365,-235.35005));
#211694=CARTESIAN_POINT('',(-2.22174260618994E-13,-11.0034818258363,-234.90005));
#211695=CARTESIAN_POINT('Origin',(0.,-11.5034818258363,-234.90005));
#211696=CARTESIAN_POINT('',(10.8748986968178,-7.30965533947201,-235.35005));
#211697=CARTESIAN_POINT('',(11.294759518486,-7.14773903260897,-234.90005));
#211698=CARTESIAN_POINT('Origin',(10.8748986968178,-7.30965533947201,-234.90005));
#211699=CARTESIAN_POINT('Origin',(0.,-11.5034818258363,-234.90005));
#211700=CARTESIAN_POINT('Origin',(0.,-11.5034818258363,-235.35005));
#211701=CARTESIAN_POINT('Origin',(19.,-10.2534818258363,-234.90005));
#211702=CARTESIAN_POINT('',(19.75,-10.2534818258363,-234.90005));
#211703=CARTESIAN_POINT('',(20.2,-10.2534818258363,-235.35005));
#211704=CARTESIAN_POINT('Origin',(20.2,-10.2534818258363,-234.90005));
#211705=CARTESIAN_POINT('Origin',(19.,-10.2534818258363,-235.35005));
#211706=CARTESIAN_POINT('Origin',(19.,-10.2534818258363,-234.90005));
#211707=CARTESIAN_POINT('Origin',(20.625,-3.54959888009691,-234.90005));
#211708=CARTESIAN_POINT('',(10.1749999999999,-3.54959888009691,-235.35005));
#211709=CARTESIAN_POINT('',(10.6249999999999,-3.54959888009691,-234.90005));
#211710=CARTESIAN_POINT('Origin',(10.1749999999999,-3.54959888009691,-234.90005));
#211711=CARTESIAN_POINT('Origin',(20.625,-3.54959888009691,-234.90005));
#211712=CARTESIAN_POINT('Origin',(20.625,-3.54959888009691,-235.35005));
#211713=CARTESIAN_POINT('Origin',(20.2,-25.4138432731711,-234.90005));
#211714=CARTESIAN_POINT('',(19.75,-2.14794227316951,-234.90005));
#211715=CARTESIAN_POINT('',(20.2,-2.14794227316951,-235.35005));
#211716=CARTESIAN_POINT('Origin',(20.2,-2.14794227316951,-234.90005));
#211717=CARTESIAN_POINT('',(20.2,-2.14794227316951,-235.35005));
#211718=CARTESIAN_POINT('',(19.75,-10.2534818258363,-234.90005));
#211719=CARTESIAN_POINT('Origin',(10.1749999999999,-25.4138432731711,-234.90005));
#211720=CARTESIAN_POINT('',(10.1749999999999,-2.14794227316951,-235.35005));
#211721=CARTESIAN_POINT('',(10.6249999999999,-2.14794227316951,-234.90005));
#211722=CARTESIAN_POINT('Origin',(10.1749999999999,-2.14794227316951,-234.90005));
#211723=CARTESIAN_POINT('',(10.6249999999999,-2.14794227316951,-234.90005));
#211724=CARTESIAN_POINT('',(10.1749999999999,-3.54959888009691,-235.35005));
#211725=CARTESIAN_POINT('Origin',(19.,-2.14794227316951,-234.90005));
#211726=CARTESIAN_POINT('',(19.,-1.39794227316951,-234.90005));
#211727=CARTESIAN_POINT('',(19.,-0.947942273169507,-235.35005));
#211728=CARTESIAN_POINT('Origin',(19.,-0.947942273169508,-234.90005));
#211729=CARTESIAN_POINT('Origin',(19.,-2.14794227316951,-235.35005));
#211730=CARTESIAN_POINT('Origin',(19.,-2.14794227316951,-234.90005));
#211731=CARTESIAN_POINT('Origin',(11.3749999999999,-2.14794227316951,-234.90005));
#211732=CARTESIAN_POINT('',(11.3749999999999,-0.947942273169504,-235.35005));
#211733=CARTESIAN_POINT('',(11.3749999999999,-1.3979422731695,-234.90005));
#211734=CARTESIAN_POINT('Origin',(11.3749999999999,-0.947942273169504,-234.90005));
#211735=CARTESIAN_POINT('Origin',(11.3749999999999,-2.14794227316951,-234.90005));
#211736=CARTESIAN_POINT('Origin',(11.3749999999999,-2.14794227316951,-235.35005));
#211737=CARTESIAN_POINT('Origin',(-296.501483394397,-0.94794227316939,-234.90005));
#211738=CARTESIAN_POINT('',(-1.11087130309497E-13,-1.3979422731695,-234.90005));
#211739=CARTESIAN_POINT('',(-296.501483394397,-0.94794227316939,-235.35005));
#211740=CARTESIAN_POINT('Origin',(11.3749999999999,-20.8590213785032,-234.90005));
#211741=CARTESIAN_POINT('',(10.1749999999999,-20.8590213785032,-235.35005));
#211742=CARTESIAN_POINT('',(10.6249999999999,-20.8590213785032,-234.90005));
#211743=CARTESIAN_POINT('Origin',(10.1749999999999,-20.8590213785032,-234.90005));
#211744=CARTESIAN_POINT('',(11.3749999999999,-21.6090213785032,-234.90005));
#211745=CARTESIAN_POINT('Origin',(11.3749999999999,-20.8590213785032,-234.90005));
#211746=CARTESIAN_POINT('',(11.3749999999999,-22.0590213785032,-235.35005));
#211747=CARTESIAN_POINT('Origin',(11.3749999999999,-22.0590213785032,-234.90005));
#211748=CARTESIAN_POINT('Origin',(11.3749999999999,-20.8590213785032,-235.35005));
#211749=CARTESIAN_POINT('Origin',(-296.501483394397,-22.0590213785033,-234.90005));
#211750=CARTESIAN_POINT('',(19.,-21.6090213785031,-234.90005));
#211751=CARTESIAN_POINT('',(19.,-22.0590213785031,-235.35005));
#211752=CARTESIAN_POINT('Origin',(19.,-22.0590213785031,-234.90005));
#211753=CARTESIAN_POINT('',(-296.501483394397,-22.0590213785033,-235.35005));
#211754=CARTESIAN_POINT('',(-3.33261390928491E-13,-21.6090213785032,-234.90005));
#211755=CARTESIAN_POINT('Origin',(10.1749999999999,-25.4138432731711,-234.90005));
#211756=CARTESIAN_POINT('',(10.1749999999999,-19.4573647715757,-235.35005));
#211757=CARTESIAN_POINT('',(10.6249999999999,-19.4573647715757,-234.90005));
#211758=CARTESIAN_POINT('Origin',(10.1749999999999,-19.4573647715757,-234.90005));
#211759=CARTESIAN_POINT('',(10.6249999999999,-19.4573647715757,-234.90005));
#211760=CARTESIAN_POINT('',(10.1749999999999,-20.8590213785032,-235.35005));
#211761=CARTESIAN_POINT('Origin',(19.,-20.8590213785032,-234.90005));
#211762=CARTESIAN_POINT('',(19.75,-20.8590213785032,-234.90005));
#211763=CARTESIAN_POINT('',(20.2,-20.8590213785032,-235.35005));
#211764=CARTESIAN_POINT('Origin',(20.2,-20.8590213785032,-234.90005));
#211765=CARTESIAN_POINT('Origin',(19.,-20.8590213785032,-235.35005));
#211766=CARTESIAN_POINT('Origin',(19.,-20.8590213785032,-234.90005));
#211767=CARTESIAN_POINT('Origin',(20.625,-19.4573647715757,-234.90005));
#211768=CARTESIAN_POINT('',(10.8748986968178,-15.6973083122006,-235.35005));
#211769=CARTESIAN_POINT('',(11.294759518486,-15.8592246190636,-234.90005));
#211770=CARTESIAN_POINT('Origin',(10.8748986968178,-15.6973083122006,-234.90005));
#211771=CARTESIAN_POINT('Origin',(20.625,-19.4573647715757,-234.90005));
#211772=CARTESIAN_POINT('Origin',(20.625,-19.4573647715757,-235.35005));
#211773=CARTESIAN_POINT('Origin',(20.2,-25.4138432731711,-234.90005));
#211774=CARTESIAN_POINT('',(19.75,-12.7534818258363,-234.90005));
#211775=CARTESIAN_POINT('',(20.2,-12.7534818258363,-235.35005));
#211776=CARTESIAN_POINT('Origin',(20.2,-12.7534818258363,-234.90005));
#211777=CARTESIAN_POINT('',(20.2,-12.7534818258363,-235.35005));
#211778=CARTESIAN_POINT('',(19.75,-20.8590213785032,-234.90005));
#211779=CARTESIAN_POINT('Origin',(0.,-11.5034818258363,-234.90005));
#211780=CARTESIAN_POINT('',(11.6003099441285,-12.6368006088516,-235.35005));
#211781=CARTESIAN_POINT('',(12.0481776255232,-12.6805560652209,-234.90005));
#211782=CARTESIAN_POINT('Origin',(11.6003099441285,-12.6368006088516,-234.90005));
#211783=CARTESIAN_POINT('Origin',(0.,-11.5034818258363,-234.90005));
#211784=CARTESIAN_POINT('Origin',(0.,-11.5034818258363,-235.35005));
#211785=CARTESIAN_POINT('Origin',(19.,-12.7534818258363,-234.90005));
#211786=CARTESIAN_POINT('',(19.,-12.0034818258363,-234.90005));
#211787=CARTESIAN_POINT('',(19.,-11.5534818258363,-235.35005));
#211788=CARTESIAN_POINT('Origin',(19.,-11.5534818258363,-234.90005));
#211789=CARTESIAN_POINT('Origin',(19.,-12.7534818258363,-235.35005));
#211790=CARTESIAN_POINT('Origin',(19.,-12.7534818258363,-234.90005));
#211791=CARTESIAN_POINT('Origin',(12.7946237611812,-12.7534818258363,-234.90005));
#211792=CARTESIAN_POINT('',(12.7946237611812,-11.5534818258363,-235.35005));
#211793=CARTESIAN_POINT('',(12.7946237611812,-12.0034818258363,-234.90005));
#211794=CARTESIAN_POINT('Origin',(12.7946237611812,-11.5534818258363,-234.90005));
#211795=CARTESIAN_POINT('Origin',(12.7946237611812,-12.7534818258363,-234.90005));
#211796=CARTESIAN_POINT('Origin',(12.7946237611812,-12.7534818258363,-235.35005));
#211797=CARTESIAN_POINT('Origin',(-296.501483394397,-11.5534818258362,-234.90005));
#211798=CARTESIAN_POINT('',(-2.22174260618994E-13,-12.0034818258363,-234.90005));
#211799=CARTESIAN_POINT('',(-296.501483394397,-11.5534818258362,-235.35005));
#211800=CARTESIAN_POINT('Origin',(21.5,-20.8590213785032,-234.90005));
#211801=CARTESIAN_POINT('',(20.3,-20.8590213785032,-235.35005));
#211802=CARTESIAN_POINT('',(20.75,-20.8590213785032,-234.90005));
#211803=CARTESIAN_POINT('Origin',(20.3,-20.8590213785032,-234.90005));
#211804=CARTESIAN_POINT('',(21.5,-21.6090213785031,-234.90005));
#211805=CARTESIAN_POINT('Origin',(21.5,-20.8590213785032,-234.90005));
#211806=CARTESIAN_POINT('',(21.5,-22.0590213785031,-235.35005));
#211807=CARTESIAN_POINT('Origin',(21.5,-22.0590213785031,-234.90005));
#211808=CARTESIAN_POINT('Origin',(21.5,-20.8590213785032,-235.35005));
#211809=CARTESIAN_POINT('Origin',(-296.501483394397,-22.0590213785033,-234.90005));
#211810=CARTESIAN_POINT('',(29.125,-21.6090213785031,-234.90005));
#211811=CARTESIAN_POINT('',(29.125,-22.0590213785031,-235.35005));
#211812=CARTESIAN_POINT('Origin',(29.125,-22.0590213785031,-234.90005));
#211813=CARTESIAN_POINT('',(-296.501483394397,-22.0590213785033,-235.35005));
#211814=CARTESIAN_POINT('',(-3.33261390928491E-13,-21.6090213785032,-234.90005));
#211815=CARTESIAN_POINT('Origin',(20.3,-25.4138432731711,-234.90005));
#211816=CARTESIAN_POINT('',(20.3,-12.7534818258363,-235.35005));
#211817=CARTESIAN_POINT('',(20.75,-12.7534818258363,-234.90005));
#211818=CARTESIAN_POINT('Origin',(20.3,-12.7534818258363,-234.90005));
#211819=CARTESIAN_POINT('',(20.75,-12.7534818258363,-234.90005));
#211820=CARTESIAN_POINT('',(20.3,-20.8590213785032,-235.35005));
#211821=CARTESIAN_POINT('Origin',(29.125,-20.8590213785032,-234.90005));
#211822=CARTESIAN_POINT('',(29.875,-20.8590213785032,-234.90005));
#211823=CARTESIAN_POINT('',(30.325,-20.8590213785032,-235.35005));
#211824=CARTESIAN_POINT('Origin',(30.325,-20.8590213785032,-234.90005));
#211825=CARTESIAN_POINT('Origin',(29.125,-20.8590213785032,-235.35005));
#211826=CARTESIAN_POINT('Origin',(29.125,-20.8590213785032,-234.90005));
#211827=CARTESIAN_POINT('Origin',(21.5,-12.7534818258363,-234.90005));
#211828=CARTESIAN_POINT('',(21.5,-11.5534818258363,-235.35005));
#211829=CARTESIAN_POINT('',(21.5,-12.0034818258363,-234.90005));
#211830=CARTESIAN_POINT('Origin',(21.5,-11.5534818258363,-234.90005));
#211831=CARTESIAN_POINT('Origin',(21.5,-12.7534818258363,-234.90005));
#211832=CARTESIAN_POINT('Origin',(21.5,-12.7534818258363,-235.35005));
#211833=CARTESIAN_POINT('Origin',(30.325,-25.4138432731711,-234.90005));
#211834=CARTESIAN_POINT('',(29.875,-12.7534818258363,-234.90005));
#211835=CARTESIAN_POINT('',(30.325,-12.7534818258363,-235.35005));
#211836=CARTESIAN_POINT('Origin',(30.325,-12.7534818258363,-234.90005));
#211837=CARTESIAN_POINT('',(30.325,-12.7534818258363,-235.35005));
#211838=CARTESIAN_POINT('',(29.875,-20.8590213785032,-234.90005));
#211839=CARTESIAN_POINT('Origin',(-296.501483394397,-11.5534818258362,-234.90005));
#211840=CARTESIAN_POINT('',(29.125,-11.5534818258363,-235.35005));
#211841=CARTESIAN_POINT('',(29.125,-12.0034818258363,-234.90005));
#211842=CARTESIAN_POINT('Origin',(29.125,-11.5534818258363,-234.90005));
#211843=CARTESIAN_POINT('',(-2.22174260618994E-13,-12.0034818258363,-234.90005));
#211844=CARTESIAN_POINT('',(-296.501483394397,-11.5534818258362,-235.35005));
#211845=CARTESIAN_POINT('Origin',(29.125,-12.7534818258363,-234.90005));
#211846=CARTESIAN_POINT('Origin',(29.125,-12.7534818258363,-234.90005));
#211847=CARTESIAN_POINT('Origin',(29.125,-12.7534818258363,-235.35005));
#211848=CARTESIAN_POINT('Origin',(31.625,-20.8590213785032,-234.90005));
#211849=CARTESIAN_POINT('',(30.425,-20.8590213785032,-235.35005));
#211850=CARTESIAN_POINT('',(30.875,-20.8590213785032,-234.90005));
#211851=CARTESIAN_POINT('Origin',(30.425,-20.8590213785032,-234.90005));
#211852=CARTESIAN_POINT('',(31.625,-21.6090213785031,-234.90005));
#211853=CARTESIAN_POINT('Origin',(31.625,-20.8590213785032,-234.90005));
#211854=CARTESIAN_POINT('',(31.625,-22.0590213785031,-235.35005));
#211855=CARTESIAN_POINT('Origin',(31.625,-22.0590213785031,-234.90005));
#211856=CARTESIAN_POINT('Origin',(31.625,-20.8590213785032,-235.35005));
#211857=CARTESIAN_POINT('Origin',(-296.501483394397,-22.0590213785033,-234.90005));
#211858=CARTESIAN_POINT('',(39.6853241707135,-21.6090213785031,-234.90005));
#211859=CARTESIAN_POINT('',(39.6853241707135,-22.0590213785031,-235.35005));
#211860=CARTESIAN_POINT('Origin',(39.6853241707135,-22.0590213785031,-234.90005));
#211861=CARTESIAN_POINT('',(-296.501483394397,-22.0590213785033,-235.35005));
#211862=CARTESIAN_POINT('',(-3.33261390928491E-13,-21.6090213785032,-234.90005));
#211863=CARTESIAN_POINT('Origin',(30.425,-25.4138432731711,-234.90005));
#211864=CARTESIAN_POINT('',(30.425,-12.7534818258363,-235.35005));
#211865=CARTESIAN_POINT('',(30.875,-12.7534818258363,-234.90005));
#211866=CARTESIAN_POINT('Origin',(30.425,-12.7534818258363,-234.90005));
#211867=CARTESIAN_POINT('',(30.875,-12.7534818258363,-234.90005));
#211868=CARTESIAN_POINT('',(30.425,-20.8590213785032,-235.35005));
#211869=CARTESIAN_POINT('Origin',(39.6853241707135,-20.8590213785032,-234.90005));
#211870=CARTESIAN_POINT('',(40.4352524876037,-20.8693905407753,-234.90005));
#211871=CARTESIAN_POINT('',(40.8852094777378,-20.8756120381386,-235.35005));
#211872=CARTESIAN_POINT('Origin',(40.8852094777378,-20.8756120381386,-234.90005));
#211873=CARTESIAN_POINT('Origin',(39.6853241707135,-20.8590213785032,-235.35005));
#211874=CARTESIAN_POINT('Origin',(39.6853241707135,-20.8590213785032,-234.90005));
#211875=CARTESIAN_POINT('Origin',(31.625,-12.7534818258363,-234.90005));
#211876=CARTESIAN_POINT('',(31.625,-11.5534818258363,-235.35005));
#211877=CARTESIAN_POINT('',(31.625,-12.0034818258363,-234.90005));
#211878=CARTESIAN_POINT('Origin',(31.625,-11.5534818258363,-234.90005));
#211879=CARTESIAN_POINT('Origin',(31.625,-12.7534818258363,-234.90005));
#211880=CARTESIAN_POINT('Origin',(31.625,-12.7534818258363,-235.35005));
#211881=CARTESIAN_POINT('Origin',(-636.934816028482,-11.5034818258361,-234.90005));
#211882=CARTESIAN_POINT('',(40.4988441937178,-12.754867256657,-234.90005));
#211883=CARTESIAN_POINT('',(40.9488434259496,-12.7556985151494,-235.35005));
#211884=CARTESIAN_POINT('Origin',(40.9488434259496,-12.7556985151494,-234.90005));
#211885=CARTESIAN_POINT('Origin',(-636.934816028482,-11.5034818258361,-235.35005));
#211886=CARTESIAN_POINT('Origin',(-636.934816028482,-11.5034818258361,-234.90005));
#211887=CARTESIAN_POINT('Origin',(-296.501483394397,-11.5534818258362,-234.90005));
#211888=CARTESIAN_POINT('',(39.7488454733312,-11.5534818258363,-235.35005));
#211889=CARTESIAN_POINT('',(39.7488454733312,-12.0034818258363,-234.90005));
#211890=CARTESIAN_POINT('Origin',(39.7488454733312,-11.5534818258363,-234.90005));
#211891=CARTESIAN_POINT('',(-2.22174260618994E-13,-12.0034818258363,-234.90005));
#211892=CARTESIAN_POINT('',(-296.501483394397,-11.5534818258362,-235.35005));
#211893=CARTESIAN_POINT('Origin',(39.7488454733312,-12.7534818258363,-234.90005));
#211894=CARTESIAN_POINT('Origin',(39.7488454733312,-12.7534818258363,-234.90005));
#211895=CARTESIAN_POINT('Origin',(39.7488454733312,-12.7534818258363,-235.35005));
#211896=CARTESIAN_POINT('Origin',(29.125,-23.3590213785032,-234.90005));
#211897=CARTESIAN_POINT('',(30.325,-23.3590213785032,-235.35005));
#211898=CARTESIAN_POINT('',(29.875,-23.3590213785032,-234.90005));
#211899=CARTESIAN_POINT('Origin',(30.325,-23.3590213785032,-234.90005));
#211900=CARTESIAN_POINT('',(29.125,-22.6090213785032,-234.90005));
#211901=CARTESIAN_POINT('Origin',(29.125,-23.3590213785032,-234.90005));
#211902=CARTESIAN_POINT('',(29.125,-22.1590213785032,-235.35005));
#211903=CARTESIAN_POINT('Origin',(29.125,-22.1590213785032,-234.90005));
#211904=CARTESIAN_POINT('Origin',(29.125,-23.3590213785032,-235.35005));
#211905=CARTESIAN_POINT('Origin',(-296.501483394397,-22.1590213785031,-234.90005));
#211906=CARTESIAN_POINT('',(21.5,-22.6090213785032,-234.90005));
#211907=CARTESIAN_POINT('',(21.5,-22.1590213785032,-235.35005));
#211908=CARTESIAN_POINT('Origin',(21.5,-22.1590213785032,-234.90005));
#211909=CARTESIAN_POINT('',(-296.501483394397,-22.1590213785031,-235.35005));
#211910=CARTESIAN_POINT('',(-3.33261390928491E-13,-22.6090213785032,-234.90005));
#211911=CARTESIAN_POINT('Origin',(30.325,-25.4138432731711,-234.90005));
#211912=CARTESIAN_POINT('',(30.325,-31.46456093117,-235.35005));
#211913=CARTESIAN_POINT('',(29.875,-31.46456093117,-234.90005));
#211914=CARTESIAN_POINT('Origin',(30.325,-31.46456093117,-234.90005));
#211915=CARTESIAN_POINT('',(29.875,-31.46456093117,-234.90005));
#211916=CARTESIAN_POINT('',(30.325,-23.3590213785032,-235.35005));
#211917=CARTESIAN_POINT('Origin',(21.5,-23.3590213785032,-234.90005));
#211918=CARTESIAN_POINT('',(20.75,-23.3590213785032,-234.90005));
#211919=CARTESIAN_POINT('',(20.3,-23.3590213785032,-235.35005));
#211920=CARTESIAN_POINT('Origin',(20.3,-23.3590213785032,-234.90005));
#211921=CARTESIAN_POINT('Origin',(21.5,-23.3590213785032,-235.35005));
#211922=CARTESIAN_POINT('Origin',(21.5,-23.3590213785032,-234.90005));
#211923=CARTESIAN_POINT('Origin',(29.125,-31.46456093117,-234.90005));
#211924=CARTESIAN_POINT('',(29.125,-32.66456093117,-235.35005));
#211925=CARTESIAN_POINT('',(29.125,-32.21456093117,-234.90005));
#211926=CARTESIAN_POINT('Origin',(29.125,-32.66456093117,-234.90005));
#211927=CARTESIAN_POINT('Origin',(29.125,-31.46456093117,-234.90005));
#211928=CARTESIAN_POINT('Origin',(29.125,-31.46456093117,-235.35005));
#211929=CARTESIAN_POINT('Origin',(20.3,-25.4138432731711,-234.90005));
#211930=CARTESIAN_POINT('',(20.75,-31.46456093117,-234.90005));
#211931=CARTESIAN_POINT('',(20.3,-31.46456093117,-235.35005));
#211932=CARTESIAN_POINT('Origin',(20.3,-31.46456093117,-234.90005));
#211933=CARTESIAN_POINT('',(20.3,-31.46456093117,-235.35005));
#211934=CARTESIAN_POINT('',(20.75,-23.3590213785032,-234.90005));
#211935=CARTESIAN_POINT('Origin',(-296.501483394397,-32.6645609311701,-234.90005));
#211936=CARTESIAN_POINT('',(21.5,-32.66456093117,-235.35005));
#211937=CARTESIAN_POINT('',(21.5,-32.21456093117,-234.90005));
#211938=CARTESIAN_POINT('Origin',(21.5,-32.66456093117,-234.90005));
#211939=CARTESIAN_POINT('',(0.,-32.21456093117,-234.90005));
#211940=CARTESIAN_POINT('',(-296.501483394397,-32.6645609311701,-235.35005));
#211941=CARTESIAN_POINT('Origin',(21.5,-31.46456093117,-234.90005));
#211942=CARTESIAN_POINT('Origin',(21.5,-31.46456093117,-234.90005));
#211943=CARTESIAN_POINT('Origin',(21.5,-31.46456093117,-235.35005));
#211944=CARTESIAN_POINT('Origin',(19.,-23.3590213785032,-234.90005));
#211945=CARTESIAN_POINT('',(20.2,-23.3590213785032,-235.35005));
#211946=CARTESIAN_POINT('',(19.75,-23.3590213785032,-234.90005));
#211947=CARTESIAN_POINT('Origin',(20.2,-23.3590213785032,-234.90005));
#211948=CARTESIAN_POINT('',(19.,-22.6090213785032,-234.90005));
#211949=CARTESIAN_POINT('Origin',(19.,-23.3590213785032,-234.90005));
#211950=CARTESIAN_POINT('',(19.,-22.1590213785032,-235.35005));
#211951=CARTESIAN_POINT('Origin',(19.,-22.1590213785032,-234.90005));
#211952=CARTESIAN_POINT('Origin',(19.,-23.3590213785032,-235.35005));
#211953=CARTESIAN_POINT('Origin',(-296.501483394397,-22.1590213785031,-234.90005));
#211954=CARTESIAN_POINT('',(11.3749999999999,-22.6090213785032,-234.90005));
#211955=CARTESIAN_POINT('',(11.3749999999999,-22.1590213785032,-235.35005));
#211956=CARTESIAN_POINT('Origin',(11.3749999999999,-22.1590213785032,-234.90005));
#211957=CARTESIAN_POINT('',(-296.501483394397,-22.1590213785031,-235.35005));
#211958=CARTESIAN_POINT('',(-3.33261390928491E-13,-22.6090213785032,-234.90005));
#211959=CARTESIAN_POINT('Origin',(20.2,-25.4138432731711,-234.90005));
#211960=CARTESIAN_POINT('',(20.2,-31.46456093117,-235.35005));
#211961=CARTESIAN_POINT('',(19.75,-31.46456093117,-234.90005));
#211962=CARTESIAN_POINT('Origin',(20.2,-31.46456093117,-234.90005));
#211963=CARTESIAN_POINT('',(19.75,-31.46456093117,-234.90005));
#211964=CARTESIAN_POINT('',(20.2,-23.3590213785032,-235.35005));
#211965=CARTESIAN_POINT('Origin',(11.3749999999999,-23.3590213785032,-234.90005));
#211966=CARTESIAN_POINT('',(10.6249999999999,-23.3590213785032,-234.90005));
#211967=CARTESIAN_POINT('',(10.1749999999999,-23.3590213785032,-235.35005));
#211968=CARTESIAN_POINT('Origin',(10.1749999999999,-23.3590213785032,-234.90005));
#211969=CARTESIAN_POINT('Origin',(11.3749999999999,-23.3590213785032,-235.35005));
#211970=CARTESIAN_POINT('Origin',(11.3749999999999,-23.3590213785032,-234.90005));
#211971=CARTESIAN_POINT('Origin',(19.,-31.46456093117,-234.90005));
#211972=CARTESIAN_POINT('',(19.,-32.66456093117,-235.35005));
#211973=CARTESIAN_POINT('',(19.,-32.21456093117,-234.90005));
#211974=CARTESIAN_POINT('Origin',(19.,-32.66456093117,-234.90005));
#211975=CARTESIAN_POINT('Origin',(19.,-31.46456093117,-234.90005));
#211976=CARTESIAN_POINT('Origin',(19.,-31.46456093117,-235.35005));
#211977=CARTESIAN_POINT('Origin',(10.1749999999999,-25.4138432731711,-234.90005));
#211978=CARTESIAN_POINT('',(10.6249999999999,-31.46456093117,-234.90005));
#211979=CARTESIAN_POINT('',(10.1749999999999,-31.46456093117,-235.35005));
#211980=CARTESIAN_POINT('Origin',(10.1749999999999,-31.46456093117,-234.90005));
#211981=CARTESIAN_POINT('',(10.1749999999999,-31.46456093117,-235.35005));
#211982=CARTESIAN_POINT('',(10.6249999999999,-23.3590213785032,-234.90005));
#211983=CARTESIAN_POINT('Origin',(-296.501483394397,-32.6645609311701,-234.90005));
#211984=CARTESIAN_POINT('',(11.3749999999999,-32.66456093117,-235.35005));
#211985=CARTESIAN_POINT('',(11.3749999999999,-32.21456093117,-234.90005));
#211986=CARTESIAN_POINT('Origin',(11.3749999999999,-32.66456093117,-234.90005));
#211987=CARTESIAN_POINT('',(0.,-32.21456093117,-234.90005));
#211988=CARTESIAN_POINT('',(-296.501483394397,-32.6645609311701,-235.35005));
#211989=CARTESIAN_POINT('Origin',(11.3749999999999,-31.46456093117,-234.90005));
#211990=CARTESIAN_POINT('Origin',(11.3749999999999,-31.46456093117,-234.90005));
#211991=CARTESIAN_POINT('Origin',(11.3749999999999,-31.46456093117,-235.35005));
#211992=CARTESIAN_POINT('Origin',(1.25,-31.46456093117,-234.90005));
#211993=CARTESIAN_POINT('',(0.0499999999999941,-31.46456093117,-235.35005));
#211994=CARTESIAN_POINT('',(0.5,-31.46456093117,-234.90005));
#211995=CARTESIAN_POINT('Origin',(0.0499999999999941,-31.46456093117,-234.90005));
#211996=CARTESIAN_POINT('',(1.25,-32.21456093117,-234.90005));
#211997=CARTESIAN_POINT('Origin',(1.25,-31.46456093117,-234.90005));
#211998=CARTESIAN_POINT('',(1.25,-32.66456093117,-235.35005));
#211999=CARTESIAN_POINT('Origin',(1.25,-32.66456093117,-234.90005));
#212000=CARTESIAN_POINT('Origin',(1.25,-31.46456093117,-235.35005));
#212001=CARTESIAN_POINT('Origin',(-296.501483394397,-32.6645609311701,-234.90005));
#212002=CARTESIAN_POINT('',(8.87499999999984,-32.21456093117,-234.90005));
#212003=CARTESIAN_POINT('',(8.87499999999984,-32.66456093117,-235.35005));
#212004=CARTESIAN_POINT('Origin',(8.87499999999984,-32.66456093117,-234.90005));
#212005=CARTESIAN_POINT('',(-296.501483394397,-32.6645609311701,-235.35005));
#212006=CARTESIAN_POINT('',(0.,-32.21456093117,-234.90005));
#212007=CARTESIAN_POINT('Origin',(0.0499999999999945,-25.4138432731711,
-234.90005));
#212008=CARTESIAN_POINT('',(0.0499999999999967,-25.3025207885872,-235.35005));
#212009=CARTESIAN_POINT('',(0.5,-25.3025207885872,-234.90005));
#212010=CARTESIAN_POINT('Origin',(0.0499999999999967,-25.3025207885872,
-234.90005));
#212011=CARTESIAN_POINT('',(0.5,-25.3025207885872,-234.90005));
#212012=CARTESIAN_POINT('',(0.0499999999999941,-31.46456093117,-235.35005));
#212013=CARTESIAN_POINT('Origin',(8.87499999999984,-31.46456093117,-234.90005));
#212014=CARTESIAN_POINT('',(9.62499999999984,-31.46456093117,-234.90005));
#212015=CARTESIAN_POINT('',(10.0749999999998,-31.46456093117,-235.35005));
#212016=CARTESIAN_POINT('Origin',(10.0749999999998,-31.46456093117,-234.90005));
#212017=CARTESIAN_POINT('Origin',(8.87499999999984,-31.46456093117,-235.35005));
#212018=CARTESIAN_POINT('Origin',(8.87499999999984,-31.46456093117,-234.90005));
#212019=CARTESIAN_POINT('Origin',(1.25,-25.3025207885872,-234.90005));
#212020=CARTESIAN_POINT('',(1.14174005138534,-24.107414189356,-235.35005));
#212021=CARTESIAN_POINT('',(1.18233753211584,-24.5555791640676,-234.90005));
#212022=CARTESIAN_POINT('Origin',(1.14174005138534,-24.107414189356,-234.90005));
#212023=CARTESIAN_POINT('Origin',(1.25,-25.3025207885872,-234.90005));
#212024=CARTESIAN_POINT('Origin',(1.25,-25.3025207885872,-235.35005));
#212025=CARTESIAN_POINT('Origin',(10.075,-25.4138432731712,-234.90005));
#212026=CARTESIAN_POINT('',(9.62499999999985,-23.3741205625531,-234.90005));
#212027=CARTESIAN_POINT('',(10.075,-23.3741205625531,-235.35005));
#212028=CARTESIAN_POINT('Origin',(10.0749999999998,-23.3741205625531,-234.90005));
#212029=CARTESIAN_POINT('',(10.075,-23.3741205625531,-235.35005));
#212030=CARTESIAN_POINT('',(9.62499999999984,-31.46456093117,-234.90005));
#212031=CARTESIAN_POINT('Origin',(0.,-11.5034818258363,-234.90005));
#212032=CARTESIAN_POINT('',(5.15044918227034,-23.0635663666157,-235.35005));
#212033=CARTESIAN_POINT('',(5.33358654455951,-23.474614668563,-234.90005));
#212034=CARTESIAN_POINT('Origin',(5.15044918227034,-23.0635663666157,-234.90005));
#212035=CARTESIAN_POINT('Origin',(0.,-11.5034818258363,-234.90005));
#212036=CARTESIAN_POINT('Origin',(0.,-11.5034818258363,-235.35005));
#212037=CARTESIAN_POINT('Origin',(8.87499999999985,-23.3741205625531,-234.90005));
#212038=CARTESIAN_POINT('',(8.80646304347558,-22.176079375619,-235.35005));
#212039=CARTESIAN_POINT('Origin',(8.87499999999985,-23.3741205625531,-235.35005));
#212040=CARTESIAN_POINT('',(8.83216440217218,-22.6253448207192,-234.90005));
#212041=CARTESIAN_POINT('Origin',(8.87499999999985,-23.3741205625531,-234.90005));
#212042=CARTESIAN_POINT('Origin',(8.80646304347558,-22.176079375619,-234.90005));
#212043=CARTESIAN_POINT('Origin',(9.40330570654103,-32.6090213785032,-234.90005));
#212044=CARTESIAN_POINT('Origin',(9.40330570654103,-32.6090213785032,-235.35005));
#212045=CARTESIAN_POINT('Origin',(9.40330570654103,-32.6090213785032,-234.90005));
#212046=CARTESIAN_POINT('Origin',(31.625,-31.46456093117,-234.90005));
#212047=CARTESIAN_POINT('',(30.425,-31.46456093117,-235.35005));
#212048=CARTESIAN_POINT('',(30.875,-31.46456093117,-234.90005));
#212049=CARTESIAN_POINT('Origin',(30.425,-31.46456093117,-234.90005));
#212050=CARTESIAN_POINT('',(31.625,-32.21456093117,-234.90005));
#212051=CARTESIAN_POINT('Origin',(31.625,-31.46456093117,-234.90005));
#212052=CARTESIAN_POINT('',(31.625,-32.66456093117,-235.35005));
#212053=CARTESIAN_POINT('Origin',(31.625,-32.66456093117,-234.90005));
#212054=CARTESIAN_POINT('Origin',(31.625,-31.46456093117,-235.35005));
#212055=CARTESIAN_POINT('Origin',(-296.501483394397,-32.6645609311701,-234.90005));
#212056=CARTESIAN_POINT('',(39.4555265729267,-32.21456093117,-234.90005));
#212057=CARTESIAN_POINT('',(39.4555265729267,-32.66456093117,-235.35005));
#212058=CARTESIAN_POINT('Origin',(39.4555265729267,-32.66456093117,-234.90005));
#212059=CARTESIAN_POINT('',(-296.501483394397,-32.6645609311701,-235.35005));
#212060=CARTESIAN_POINT('',(0.,-32.21456093117,-234.90005));
#212061=CARTESIAN_POINT('Origin',(30.425,-25.4138432731711,-234.90005));
#212062=CARTESIAN_POINT('',(30.425,-23.3590213785032,-235.35005));
#212063=CARTESIAN_POINT('',(30.875,-23.3590213785032,-234.90005));
#212064=CARTESIAN_POINT('Origin',(30.425,-23.3590213785032,-234.90005));
#212065=CARTESIAN_POINT('',(30.875,-23.3590213785032,-234.90005));
#212066=CARTESIAN_POINT('',(30.425,-31.46456093117,-235.35005));
#212067=CARTESIAN_POINT('Origin',(39.4555265729267,-31.46456093117,-234.90005));
#212068=CARTESIAN_POINT('',(40.2052001948774,-31.486684686535,-234.90005));
#212069=CARTESIAN_POINT('',(40.6550043680477,-31.499958939754,-235.35005));
#212070=CARTESIAN_POINT('Origin',(40.6550043680476,-31.499958939754,-234.90005));
#212071=CARTESIAN_POINT('Origin',(39.4555265729267,-31.46456093117,-235.35005));
#212072=CARTESIAN_POINT('Origin',(39.4555265729267,-31.46456093117,-234.90005));
#212073=CARTESIAN_POINT('Origin',(31.625,-23.3590213785032,-234.90005));
#212074=CARTESIAN_POINT('',(31.625,-22.1590213785032,-235.35005));
#212075=CARTESIAN_POINT('',(31.625,-22.6090213785032,-234.90005));
#212076=CARTESIAN_POINT('Origin',(31.625,-22.1590213785032,-234.90005));
#212077=CARTESIAN_POINT('Origin',(31.625,-23.3590213785032,-234.90005));
#212078=CARTESIAN_POINT('Origin',(31.625,-23.3590213785032,-235.35005));
#212079=CARTESIAN_POINT('Origin',(-636.934816028482,-11.5034818258361,-234.90005));
#212080=CARTESIAN_POINT('',(40.3960221980465,-23.3721614024167,-234.90005));
#212081=CARTESIAN_POINT('',(40.8459531286544,-23.3800454167648,-235.35005));
#212082=CARTESIAN_POINT('Origin',(40.8459531286544,-23.3800454167648,-234.90005));
#212083=CARTESIAN_POINT('Origin',(-636.934816028482,-11.5034818258361,-235.35005));
#212084=CARTESIAN_POINT('Origin',(-636.934816028482,-11.5034818258361,-234.90005));
#212085=CARTESIAN_POINT('Origin',(-296.501483394397,-22.1590213785031,-234.90005));
#212086=CARTESIAN_POINT('',(39.6461373136998,-22.1590213785032,-235.35005));
#212087=CARTESIAN_POINT('',(39.6461373136998,-22.6090213785032,-234.90005));
#212088=CARTESIAN_POINT('Origin',(39.6461373136998,-22.1590213785032,-234.90005));
#212089=CARTESIAN_POINT('',(-3.33261390928491E-13,-22.6090213785032,-234.90005));
#212090=CARTESIAN_POINT('',(-296.501483394397,-22.1590213785031,-235.35005));
#212091=CARTESIAN_POINT('Origin',(39.6461373136998,-23.3590213785032,-234.90005));
#212092=CARTESIAN_POINT('Origin',(39.6461373136998,-23.3590213785032,-234.90005));
#212093=CARTESIAN_POINT('Origin',(39.6461373136998,-23.3590213785032,-235.35005));
#212094=CARTESIAN_POINT('Origin',(31.625,-42.0701004838368,-234.90005));
#212095=CARTESIAN_POINT('',(30.425,-42.0701004838368,-235.35005));
#212096=CARTESIAN_POINT('',(30.875,-42.0701004838368,-234.90005));
#212097=CARTESIAN_POINT('Origin',(30.425,-42.0701004838368,-234.90005));
#212098=CARTESIAN_POINT('',(31.625,-42.8201004838368,-234.90005));
#212099=CARTESIAN_POINT('Origin',(31.625,-42.0701004838368,-234.90005));
#212100=CARTESIAN_POINT('',(31.625,-43.2701004838368,-235.35005));
#212101=CARTESIAN_POINT('Origin',(31.625,-43.2701004838368,-234.90005));
#212102=CARTESIAN_POINT('Origin',(31.625,-42.0701004838368,-235.35005));
#212103=CARTESIAN_POINT('Origin',(-296.501483394397,-43.270100483837,-234.90005));
#212104=CARTESIAN_POINT('',(36.0311576807678,-42.8201004838368,-234.90005));
#212105=CARTESIAN_POINT('',(36.0311576807678,-43.2701004838368,-235.35005));
#212106=CARTESIAN_POINT('Origin',(36.0311576807678,-43.2701004838368,-234.90005));
#212107=CARTESIAN_POINT('',(-296.501483394397,-43.270100483837,-235.35005));
#212108=CARTESIAN_POINT('',(-1.54373336646987E-15,-42.8201004838369,-234.90005));
#212109=CARTESIAN_POINT('Origin',(30.425,-25.4138432731711,-234.90005));
#212110=CARTESIAN_POINT('',(30.425,-33.96456093117,-235.35005));
#212111=CARTESIAN_POINT('',(30.875,-33.96456093117,-234.90005));
#212112=CARTESIAN_POINT('Origin',(30.425,-33.96456093117,-234.90005));
#212113=CARTESIAN_POINT('',(30.875,-33.96456093117,-234.90005));
#212114=CARTESIAN_POINT('',(30.425,-42.0701004838368,-235.35005));
#212115=CARTESIAN_POINT('Origin',(36.0311576807678,-42.0701004838368,-234.90005));
#212116=CARTESIAN_POINT('',(36.6030808185578,-42.5552849069797,-234.90005));
#212117=CARTESIAN_POINT('',(36.9462347012318,-42.8463955608654,-235.35005));
#212118=CARTESIAN_POINT('Origin',(36.9462347012318,-42.8463955608654,-234.90005));
#212119=CARTESIAN_POINT('Origin',(36.0311576807678,-42.0701004838368,-235.35005));
#212120=CARTESIAN_POINT('Origin',(36.0311576807678,-42.0701004838368,-234.90005));
#212121=CARTESIAN_POINT('Origin',(31.625,-33.96456093117,-234.90005));
#212122=CARTESIAN_POINT('',(31.625,-32.76456093117,-235.35005));
#212123=CARTESIAN_POINT('',(31.625,-33.21456093117,-234.90005));
#212124=CARTESIAN_POINT('Origin',(31.625,-32.76456093117,-234.90005));
#212125=CARTESIAN_POINT('Origin',(31.625,-33.96456093117,-234.90005));
#212126=CARTESIAN_POINT('Origin',(31.625,-33.96456093117,-235.35005));
#212127=CARTESIAN_POINT('Origin',(-6.29739814579425E-15,-11.5034818258363,
-234.90005));
#212128=CARTESIAN_POINT('',(39.8203148590358,-38.3053945286125,-234.90005));
#212129=CARTESIAN_POINT('',(40.1936303108393,-38.5566624602009,-235.35005));
#212130=CARTESIAN_POINT('Origin',(40.1936303108393,-38.5566624602009,-234.90005));
#212131=CARTESIAN_POINT('Origin',(-6.29739814579425E-15,-11.5034818258363,
-235.35005));
#212132=CARTESIAN_POINT('Origin',(-6.29739814579425E-15,-11.5034818258363,
-234.90005));
#212133=CARTESIAN_POINT('Origin',(-296.501483394397,-32.7645609311699,-234.90005));
#212134=CARTESIAN_POINT('',(39.3771239584772,-32.76456093117,-235.35005));
#212135=CARTESIAN_POINT('',(39.3771239584772,-33.21456093117,-234.90005));
#212136=CARTESIAN_POINT('Origin',(39.3771239584772,-32.76456093117,-234.90005));
#212137=CARTESIAN_POINT('',(0.,-33.21456093117,-234.90005));
#212138=CARTESIAN_POINT('',(-296.501483394397,-32.7645609311699,-235.35005));
#212139=CARTESIAN_POINT('Origin',(38.9907249661392,-37.7470213473046,-234.90005));
#212140=CARTESIAN_POINT('',(39.989972084972,-37.7858181964606,-234.90005));
#212141=CARTESIAN_POINT('',(40.4396332884467,-37.8032767785809,-235.35005));
#212142=CARTESIAN_POINT('Origin',(40.4396332884467,-37.8032767785809,-234.90005));
#212143=CARTESIAN_POINT('Origin',(38.9907249661392,-37.7470213473046,-235.35005));
#212144=CARTESIAN_POINT('Origin',(38.9907249661392,-37.7470213473046,-234.90005));
#212145=CARTESIAN_POINT('Origin',(39.3771239584772,-33.96456093117,-234.90005));
#212146=CARTESIAN_POINT('',(40.5764627182082,-34.0043923183801,-235.35005));
#212147=CARTESIAN_POINT('',(40.1267106833092,-33.9894555481763,-234.90005));
#212148=CARTESIAN_POINT('Origin',(40.5764627182082,-34.0043923183801,-234.90005));
#212149=CARTESIAN_POINT('Origin',(39.3771239584772,-33.96456093117,-234.90005));
#212150=CARTESIAN_POINT('Origin',(39.3771239584772,-33.96456093117,-235.35005));
#212151=CARTESIAN_POINT('Origin',(-636.934816028482,-11.5034818258361,-234.90005));
#212152=CARTESIAN_POINT('Origin',(-636.934816028482,-11.5034818258361,-234.90005));
#212153=CARTESIAN_POINT('Origin',(-636.934816028482,-11.5034818258361,-235.35005));
#212154=CARTESIAN_POINT('Origin',(21.5,-42.0701004838368,-234.90005));
#212155=CARTESIAN_POINT('',(20.3,-42.0701004838368,-235.35005));
#212156=CARTESIAN_POINT('',(20.75,-42.0701004838368,-234.90005));
#212157=CARTESIAN_POINT('Origin',(20.3,-42.0701004838368,-234.90005));
#212158=CARTESIAN_POINT('',(21.5,-42.8201004838368,-234.90005));
#212159=CARTESIAN_POINT('Origin',(21.5,-42.0701004838368,-234.90005));
#212160=CARTESIAN_POINT('',(21.5,-43.2701004838368,-235.35005));
#212161=CARTESIAN_POINT('Origin',(21.5,-43.2701004838368,-234.90005));
#212162=CARTESIAN_POINT('Origin',(21.5,-42.0701004838368,-235.35005));
#212163=CARTESIAN_POINT('Origin',(-296.501483394397,-43.270100483837,-234.90005));
#212164=CARTESIAN_POINT('',(29.125,-42.8201004838368,-234.90005));
#212165=CARTESIAN_POINT('',(29.125,-43.2701004838368,-235.35005));
#212166=CARTESIAN_POINT('Origin',(29.125,-43.2701004838368,-234.90005));
#212167=CARTESIAN_POINT('',(-296.501483394397,-43.270100483837,-235.35005));
#212168=CARTESIAN_POINT('',(-1.54373336646987E-15,-42.8201004838369,-234.90005));
#212169=CARTESIAN_POINT('Origin',(20.3,-25.4138432731711,-234.90005));
#212170=CARTESIAN_POINT('',(20.3,-33.96456093117,-235.35005));
#212171=CARTESIAN_POINT('',(20.75,-33.96456093117,-234.90005));
#212172=CARTESIAN_POINT('Origin',(20.3,-33.96456093117,-234.90005));
#212173=CARTESIAN_POINT('',(20.75,-33.96456093117,-234.90005));
#212174=CARTESIAN_POINT('',(20.3,-42.0701004838368,-235.35005));
#212175=CARTESIAN_POINT('Origin',(29.125,-42.0701004838368,-234.90005));
#212176=CARTESIAN_POINT('',(29.875,-42.0701004838368,-234.90005));
#212177=CARTESIAN_POINT('',(30.325,-42.0701004838368,-235.35005));
#212178=CARTESIAN_POINT('Origin',(30.325,-42.0701004838368,-234.90005));
#212179=CARTESIAN_POINT('Origin',(29.125,-42.0701004838368,-235.35005));
#212180=CARTESIAN_POINT('Origin',(29.125,-42.0701004838368,-234.90005));
#212181=CARTESIAN_POINT('Origin',(21.5,-33.96456093117,-234.90005));
#212182=CARTESIAN_POINT('',(21.5,-32.76456093117,-235.35005));
#212183=CARTESIAN_POINT('',(21.5,-33.21456093117,-234.90005));
#212184=CARTESIAN_POINT('Origin',(21.5,-32.76456093117,-234.90005));
#212185=CARTESIAN_POINT('Origin',(21.5,-33.96456093117,-234.90005));
#212186=CARTESIAN_POINT('Origin',(21.5,-33.96456093117,-235.35005));
#212187=CARTESIAN_POINT('Origin',(30.325,-25.4138432731711,-234.90005));
#212188=CARTESIAN_POINT('',(29.875,-33.96456093117,-234.90005));
#212189=CARTESIAN_POINT('',(30.325,-33.96456093117,-235.35005));
#212190=CARTESIAN_POINT('Origin',(30.325,-33.96456093117,-234.90005));
#212191=CARTESIAN_POINT('',(30.325,-33.96456093117,-235.35005));
#212192=CARTESIAN_POINT('',(29.875,-42.0701004838368,-234.90005));
#212193=CARTESIAN_POINT('Origin',(-296.501483394397,-32.7645609311699,-234.90005));
#212194=CARTESIAN_POINT('',(29.125,-32.76456093117,-235.35005));
#212195=CARTESIAN_POINT('',(29.125,-33.21456093117,-234.90005));
#212196=CARTESIAN_POINT('Origin',(29.125,-32.76456093117,-234.90005));
#212197=CARTESIAN_POINT('',(0.,-33.21456093117,-234.90005));
#212198=CARTESIAN_POINT('',(-296.501483394397,-32.7645609311699,-235.35005));
#212199=CARTESIAN_POINT('Origin',(29.125,-33.96456093117,-234.90005));
#212200=CARTESIAN_POINT('Origin',(29.125,-33.96456093117,-234.90005));
#212201=CARTESIAN_POINT('Origin',(29.125,-33.96456093117,-235.35005));
#212202=CARTESIAN_POINT('Origin',(29.125,-44.5701004838368,-234.90005));
#212203=CARTESIAN_POINT('',(30.325,-44.5701004838368,-235.35005));
#212204=CARTESIAN_POINT('',(29.875,-44.5701004838368,-234.90005));
#212205=CARTESIAN_POINT('Origin',(30.325,-44.5701004838368,-234.90005));
#212206=CARTESIAN_POINT('',(29.125,-43.8201004838368,-234.90005));
#212207=CARTESIAN_POINT('Origin',(29.125,-44.5701004838368,-234.90005));
#212208=CARTESIAN_POINT('',(29.125,-43.3701004838369,-235.35005));
#212209=CARTESIAN_POINT('Origin',(29.125,-43.3701004838369,-234.90005));
#212210=CARTESIAN_POINT('Origin',(29.125,-44.5701004838368,-235.35005));
#212211=CARTESIAN_POINT('Origin',(-296.501483394397,-43.3701004838369,-234.90005));
#212212=CARTESIAN_POINT('',(21.5,-43.8201004838368,-234.90005));
#212213=CARTESIAN_POINT('',(21.5,-43.3701004838369,-235.35005));
#212214=CARTESIAN_POINT('Origin',(21.5,-43.3701004838369,-234.90005));
#212215=CARTESIAN_POINT('',(-296.501483394397,-43.3701004838369,-235.35005));
#212216=CARTESIAN_POINT('',(-1.23757166668304E-15,-43.8201004838368,-234.90005));
#212217=CARTESIAN_POINT('Origin',(30.325,-25.4138432731711,-234.90005));
#212218=CARTESIAN_POINT('',(30.325,-48.7096221120845,-235.35005));
#212219=CARTESIAN_POINT('',(29.875,-48.7096221120845,-234.90005));
#212220=CARTESIAN_POINT('Origin',(30.325,-48.7096221120845,-234.90005));
#212221=CARTESIAN_POINT('',(29.875,-48.7096221120845,-234.90005));
#212222=CARTESIAN_POINT('',(30.325,-44.5701004838368,-235.35005));
#212223=CARTESIAN_POINT('Origin',(21.5,-44.5701004838368,-234.90005));
#212224=CARTESIAN_POINT('',(20.75,-44.5701004838368,-234.90005));
#212225=CARTESIAN_POINT('',(20.3,-44.5701004838368,-235.35005));
#212226=CARTESIAN_POINT('Origin',(20.3,-44.5701004838368,-234.90005));
#212227=CARTESIAN_POINT('Origin',(21.5,-44.5701004838368,-235.35005));
#212228=CARTESIAN_POINT('Origin',(21.5,-44.5701004838368,-234.90005));
#212229=CARTESIAN_POINT('Origin',(29.125,-48.7096221120845,-234.90005));
#212230=CARTESIAN_POINT('',(29.8646825396825,-49.6545399606241,-235.35005));
#212231=CARTESIAN_POINT('',(29.5873015873016,-49.3001957674217,-234.90005));
#212232=CARTESIAN_POINT('Origin',(29.8646825396825,-49.6545399606241,-234.90005));
#212233=CARTESIAN_POINT('Origin',(29.125,-48.7096221120845,-234.90005));
#212234=CARTESIAN_POINT('Origin',(29.125,-48.7096221120845,-235.35005));
#212235=CARTESIAN_POINT('Origin',(20.3,-25.4138432731711,-234.90005));
#212236=CARTESIAN_POINT('',(20.75,-52.8339989151841,-234.90005));
#212237=CARTESIAN_POINT('',(20.3,-52.8339989151841,-235.35005));
#212238=CARTESIAN_POINT('Origin',(20.3,-52.8339989151841,-234.90005));
#212239=CARTESIAN_POINT('',(20.3,-52.8339989151841,-235.35005));
#212240=CARTESIAN_POINT('',(20.75,-44.5701004838368,-234.90005));
#212241=CARTESIAN_POINT('Origin',(-6.29739814579425E-15,-11.5034818258363,
-234.90005));
#212242=CARTESIAN_POINT('',(23.6248477671233,-53.8032344017111,-235.35005));
#212243=CARTESIAN_POINT('',(23.4054219364689,-53.410357442802,-234.90005));
#212244=CARTESIAN_POINT('Origin',(23.6248477671233,-53.8032344017111,-234.90005));
#212245=CARTESIAN_POINT('Origin',(-6.29739814579425E-15,-11.5034818258363,
-234.90005));
#212246=CARTESIAN_POINT('Origin',(-6.29739814579425E-15,-11.5034818258363,
-235.35005));
#212247=CARTESIAN_POINT('Origin',(21.5,-52.8339989151841,-234.90005));
#212248=CARTESIAN_POINT('',(21.5238294101154,-53.5836202590729,-234.90005));
#212249=CARTESIAN_POINT('',(21.5381270561845,-54.0333930654061,-235.35005));
#212250=CARTESIAN_POINT('Origin',(21.5381270561845,-54.0333930654061,-234.90005));
#212251=CARTESIAN_POINT('Origin',(21.5,-52.8339989151841,-235.35005));
#212252=CARTESIAN_POINT('Origin',(21.5,-52.8339989151841,-234.90005));
#212253=CARTESIAN_POINT('Origin',(22.9178089794592,-52.5372975341153,-234.90005));
#212254=CARTESIAN_POINT('',(22.9669354026308,-53.9864650863833,-235.35005));
#212255=CARTESIAN_POINT('',(22.9516892713016,-53.5367234322311,-234.90005));
#212256=CARTESIAN_POINT('Origin',(22.9669354026308,-53.9864650863833,-234.90005));
#212257=CARTESIAN_POINT('Origin',(22.9178089794592,-52.5372975341153,-234.90005));
#212258=CARTESIAN_POINT('Origin',(22.9178089794592,-52.5372975341153,-235.35005));
#212259=CARTESIAN_POINT('Origin',(7.14692237356698E-14,623.509175991979,
-234.90005));
#212260=CARTESIAN_POINT('Origin',(7.14692237356698E-14,623.509175991979,
-234.90005));
#212261=CARTESIAN_POINT('Origin',(7.14692237356698E-14,623.509175991979,
-235.35005));
#212262=CARTESIAN_POINT('Origin',(19.,-44.5701004838368,-234.90005));
#212263=CARTESIAN_POINT('',(20.2,-44.5701004838368,-235.35005));
#212264=CARTESIAN_POINT('',(19.75,-44.5701004838368,-234.90005));
#212265=CARTESIAN_POINT('Origin',(20.2,-44.5701004838368,-234.90005));
#212266=CARTESIAN_POINT('',(19.,-43.8201004838368,-234.90005));
#212267=CARTESIAN_POINT('Origin',(19.,-44.5701004838368,-234.90005));
#212268=CARTESIAN_POINT('',(19.,-43.3701004838369,-235.35005));
#212269=CARTESIAN_POINT('Origin',(19.,-43.3701004838369,-234.90005));
#212270=CARTESIAN_POINT('Origin',(19.,-44.5701004838368,-235.35005));
#212271=CARTESIAN_POINT('Origin',(-296.501483394397,-43.3701004838369,-234.90005));
#212272=CARTESIAN_POINT('',(11.3749999999999,-43.8201004838368,-234.90005));
#212273=CARTESIAN_POINT('',(11.3749999999999,-43.3701004838369,-235.35005));
#212274=CARTESIAN_POINT('Origin',(11.3749999999999,-43.3701004838369,-234.90005));
#212275=CARTESIAN_POINT('',(-296.501483394397,-43.3701004838369,-235.35005));
#212276=CARTESIAN_POINT('',(-1.23757166668304E-15,-43.8201004838368,-234.90005));
#212277=CARTESIAN_POINT('Origin',(20.2,-25.4138432731711,-234.90005));
#212278=CARTESIAN_POINT('',(20.2,-52.9088458284789,-235.35005));
#212279=CARTESIAN_POINT('',(19.75,-52.9088458284789,-234.90005));
#212280=CARTESIAN_POINT('Origin',(20.2,-52.9088458284789,-234.90005));
#212281=CARTESIAN_POINT('',(19.75,-52.9088458284789,-234.90005));
#212282=CARTESIAN_POINT('',(20.2,-44.5701004838368,-235.35005));
#212283=CARTESIAN_POINT('Origin',(11.3749999999999,-44.5701004838369,-234.90005));
#212284=CARTESIAN_POINT('',(10.6249999999999,-44.5701004838369,-234.90005));
#212285=CARTESIAN_POINT('',(10.1749999999999,-44.5701004838369,-235.35005));
#212286=CARTESIAN_POINT('Origin',(10.1749999999999,-44.5701004838369,-234.90005));
#212287=CARTESIAN_POINT('Origin',(11.3749999999999,-44.5701004838369,-235.35005));
#212288=CARTESIAN_POINT('Origin',(11.3749999999999,-44.5701004838369,-234.90005));
#212289=CARTESIAN_POINT('Origin',(19.,-52.9088458284789,-234.90005));
#212290=CARTESIAN_POINT('',(19.0336936775584,-54.1083727085831,-235.35005));
#212291=CARTESIAN_POINT('',(19.021058548474,-53.6585501285442,-234.90005));
#212292=CARTESIAN_POINT('Origin',(19.0336936775584,-54.1083727085831,-234.90005));
#212293=CARTESIAN_POINT('Origin',(19.,-52.9088458284789,-234.90005));
#212294=CARTESIAN_POINT('Origin',(19.,-52.9088458284789,-235.35005));
#212295=CARTESIAN_POINT('Origin',(10.1749999999999,-25.4138432731711,-234.90005));
#212296=CARTESIAN_POINT('',(10.6249999999999,-53.08002700974,-234.90005));
#212297=CARTESIAN_POINT('',(10.1749999999999,-53.08002700974,-235.35005));
#212298=CARTESIAN_POINT('Origin',(10.1749999999999,-53.08002700974,-234.90005));
#212299=CARTESIAN_POINT('',(10.1749999999999,-53.08002700974,-235.35005));
#212300=CARTESIAN_POINT('',(10.6249999999999,-44.5701004838369,-234.90005));
#212301=CARTESIAN_POINT('Origin',(7.14692237356698E-14,623.509175991979,
-234.90005));
#212302=CARTESIAN_POINT('',(11.3951718727487,-54.2798574542403,-235.35005));
#212303=CARTESIAN_POINT('',(11.3876074204679,-53.8299210375529,-234.90005));
#212304=CARTESIAN_POINT('Origin',(11.3951718727487,-54.2798574542403,-234.90005));
#212305=CARTESIAN_POINT('Origin',(7.14692237356698E-14,623.509175991979,
-234.90005));
#212306=CARTESIAN_POINT('Origin',(7.14692237356698E-14,623.509175991979,
-235.35005));
#212307=CARTESIAN_POINT('Origin',(11.3749999999999,-53.08002700974,-234.90005));
#212308=CARTESIAN_POINT('Origin',(11.3749999999999,-53.08002700974,-234.90005));
#212309=CARTESIAN_POINT('Origin',(11.3749999999999,-53.08002700974,-235.35005));
#212310=CARTESIAN_POINT('Origin',(11.3749999999999,-42.0701004838369,-234.90005));
#212311=CARTESIAN_POINT('',(10.1749999999999,-42.0701004838368,-235.35005));
#212312=CARTESIAN_POINT('',(10.6249999999999,-42.0701004838368,-234.90005));
#212313=CARTESIAN_POINT('Origin',(10.1749999999999,-42.0701004838368,-234.90005));
#212314=CARTESIAN_POINT('',(11.3749999999999,-42.8201004838369,-234.90005));
#212315=CARTESIAN_POINT('Origin',(11.3749999999999,-42.0701004838369,-234.90005));
#212316=CARTESIAN_POINT('',(11.3749999999999,-43.2701004838368,-235.35005));
#212317=CARTESIAN_POINT('Origin',(11.3749999999999,-43.2701004838368,-234.90005));
#212318=CARTESIAN_POINT('Origin',(11.3749999999999,-42.0701004838369,-235.35005));
#212319=CARTESIAN_POINT('Origin',(-296.501483394397,-43.270100483837,-234.90005));
#212320=CARTESIAN_POINT('',(19.,-42.8201004838368,-234.90005));
#212321=CARTESIAN_POINT('',(19.,-43.2701004838368,-235.35005));
#212322=CARTESIAN_POINT('Origin',(19.,-43.2701004838368,-234.90005));
#212323=CARTESIAN_POINT('',(-296.501483394397,-43.270100483837,-235.35005));
#212324=CARTESIAN_POINT('',(-1.54373336646987E-15,-42.8201004838369,-234.90005));
#212325=CARTESIAN_POINT('Origin',(10.1749999999999,-25.4138432731711,-234.90005));
#212326=CARTESIAN_POINT('',(10.1749999999999,-33.96456093117,-235.35005));
#212327=CARTESIAN_POINT('',(10.6249999999999,-33.96456093117,-234.90005));
#212328=CARTESIAN_POINT('Origin',(10.1749999999999,-33.96456093117,-234.90005));
#212329=CARTESIAN_POINT('',(10.6249999999999,-33.96456093117,-234.90005));
#212330=CARTESIAN_POINT('',(10.1749999999999,-42.0701004838368,-235.35005));
#212331=CARTESIAN_POINT('Origin',(19.,-42.0701004838368,-234.90005));
#212332=CARTESIAN_POINT('',(19.75,-42.0701004838368,-234.90005));
#212333=CARTESIAN_POINT('',(20.2,-42.0701004838368,-235.35005));
#212334=CARTESIAN_POINT('Origin',(20.2,-42.0701004838368,-234.90005));
#212335=CARTESIAN_POINT('Origin',(19.,-42.0701004838368,-235.35005));
#212336=CARTESIAN_POINT('Origin',(19.,-42.0701004838368,-234.90005));
#212337=CARTESIAN_POINT('Origin',(11.3749999999999,-33.96456093117,-234.90005));
#212338=CARTESIAN_POINT('',(11.3749999999999,-32.76456093117,-235.35005));
#212339=CARTESIAN_POINT('',(11.3749999999999,-33.21456093117,-234.90005));
#212340=CARTESIAN_POINT('Origin',(11.3749999999999,-32.76456093117,-234.90005));
#212341=CARTESIAN_POINT('Origin',(11.3749999999999,-33.96456093117,-234.90005));
#212342=CARTESIAN_POINT('Origin',(11.3749999999999,-33.96456093117,-235.35005));
#212343=CARTESIAN_POINT('Origin',(20.2,-25.4138432731711,-234.90005));
#212344=CARTESIAN_POINT('',(19.75,-33.96456093117,-234.90005));
#212345=CARTESIAN_POINT('',(20.2,-33.96456093117,-235.35005));
#212346=CARTESIAN_POINT('Origin',(20.2,-33.96456093117,-234.90005));
#212347=CARTESIAN_POINT('',(20.2,-33.96456093117,-235.35005));
#212348=CARTESIAN_POINT('',(19.75,-42.0701004838368,-234.90005));
#212349=CARTESIAN_POINT('Origin',(-296.501483394397,-32.7645609311699,-234.90005));
#212350=CARTESIAN_POINT('',(19.,-32.76456093117,-235.35005));
#212351=CARTESIAN_POINT('',(19.,-33.21456093117,-234.90005));
#212352=CARTESIAN_POINT('Origin',(19.,-32.76456093117,-234.90005));
#212353=CARTESIAN_POINT('',(0.,-33.21456093117,-234.90005));
#212354=CARTESIAN_POINT('',(-296.501483394397,-32.7645609311699,-235.35005));
#212355=CARTESIAN_POINT('Origin',(19.,-33.96456093117,-234.90005));
#212356=CARTESIAN_POINT('Origin',(19.,-33.96456093117,-234.90005));
#212357=CARTESIAN_POINT('Origin',(19.,-33.96456093117,-235.35005));
#212358=CARTESIAN_POINT('Origin',(8.87499999999984,-44.5701004838369,-234.90005));
#212359=CARTESIAN_POINT('',(10.075,-44.5701004838369,-235.35005));
#212360=CARTESIAN_POINT('',(9.62499999999984,-44.5701004838369,-234.90005));
#212361=CARTESIAN_POINT('Origin',(10.075,-44.5701004838369,-234.90005));
#212362=CARTESIAN_POINT('',(8.87499999999984,-43.8201004838368,-234.90005));
#212363=CARTESIAN_POINT('Origin',(8.87499999999984,-44.5701004838369,-234.90005));
#212364=CARTESIAN_POINT('',(8.87499999999984,-43.3701004838369,-235.35005));
#212365=CARTESIAN_POINT('Origin',(8.87499999999984,-43.3701004838369,-234.90005));
#212366=CARTESIAN_POINT('Origin',(8.87499999999984,-44.5701004838369,-235.35005));
#212367=CARTESIAN_POINT('Origin',(-296.501483394397,-43.3701004838369,-234.90005));
#212368=CARTESIAN_POINT('',(1.25,-43.8201004838368,-234.90005));
#212369=CARTESIAN_POINT('',(1.25,-43.3701004838369,-235.35005));
#212370=CARTESIAN_POINT('Origin',(1.25,-43.3701004838369,-234.90005));
#212371=CARTESIAN_POINT('',(-296.501483394397,-43.3701004838369,-235.35005));
#212372=CARTESIAN_POINT('',(-1.23757166668304E-15,-43.8201004838368,-234.90005));
#212373=CARTESIAN_POINT('Origin',(10.075,-25.4138432731712,-234.90005));
#212374=CARTESIAN_POINT('',(10.0749999999998,-53.1174378937751,-235.35005));
#212375=CARTESIAN_POINT('',(9.62499999999984,-53.1174378937751,-234.90005));
#212376=CARTESIAN_POINT('Origin',(10.0749999999998,-53.1174378937751,-234.90005));
#212377=CARTESIAN_POINT('',(9.62499999999984,-53.1174378937751,-234.90005));
#212378=CARTESIAN_POINT('',(10.075,-44.5701004838369,-235.35005));
#212379=CARTESIAN_POINT('Origin',(1.25,-44.5701004838369,-234.90005));
#212380=CARTESIAN_POINT('',(0.5,-44.5701004838369,-234.90005));
#212381=CARTESIAN_POINT('',(0.0499999999999953,-44.5701004838369,-235.35005));
#212382=CARTESIAN_POINT('Origin',(0.0499999999999955,-44.5701004838369,
-234.90005));
#212383=CARTESIAN_POINT('Origin',(1.25,-44.5701004838369,-235.35005));
#212384=CARTESIAN_POINT('Origin',(1.25,-44.5701004838369,-234.90005));
#212385=CARTESIAN_POINT('Origin',(8.87499999999984,-53.1174378937751,-234.90005));
#212386=CARTESIAN_POINT('',(8.89073849412256,-54.3173346809209,-235.35005));
#212387=CARTESIAN_POINT('',(8.88483655882654,-53.8673733857413,-234.90005));
#212388=CARTESIAN_POINT('Origin',(8.89073849412256,-54.3173346809209,-234.90005));
#212389=CARTESIAN_POINT('Origin',(8.87499999999984,-53.1174378937751,-234.90005));
#212390=CARTESIAN_POINT('Origin',(8.87499999999984,-53.1174378937751,-235.35005));
#212391=CARTESIAN_POINT('Origin',(0.0499999999999945,-25.4138432731711,
-234.90005));
#212392=CARTESIAN_POINT('',(0.5,-53.1744855098348,-234.90005));
#212393=CARTESIAN_POINT('',(0.0499999999999928,-53.1744855098348,-235.35005));
#212394=CARTESIAN_POINT('Origin',(0.049999999999995,-53.1744855098348,-234.90005));
#212395=CARTESIAN_POINT('',(0.0499999999999928,-53.1744855098348,-235.35005));
#212396=CARTESIAN_POINT('',(0.5,-44.5701004838369,-234.90005));
#212397=CARTESIAN_POINT('Origin',(7.14692237356698E-14,623.509175991979,
-234.90005));
#212398=CARTESIAN_POINT('',(1.25221668931305,-54.3744834624533,-235.35005));
#212399=CARTESIAN_POINT('',(1.25138543082066,-53.9244842302215,-234.90005));
#212400=CARTESIAN_POINT('Origin',(1.25221668931305,-54.3744834624533,-234.90005));
#212401=CARTESIAN_POINT('Origin',(7.14692237356698E-14,623.509175991979,
-234.90005));
#212402=CARTESIAN_POINT('Origin',(7.14692237356698E-14,623.509175991979,
-235.35005));
#212403=CARTESIAN_POINT('Origin',(1.25,-53.1744855098348,-234.90005));
#212404=CARTESIAN_POINT('Origin',(1.25,-53.1744855098348,-234.90005));
#212405=CARTESIAN_POINT('Origin',(1.25,-53.1744855098348,-235.35005));
#212406=CARTESIAN_POINT('Origin',(1.25,-42.0701004838369,-234.90005));
#212407=CARTESIAN_POINT('',(0.0499999999999935,-42.0701004838369,-235.35005));
#212408=CARTESIAN_POINT('',(0.5,-42.0701004838369,-234.90005));
#212409=CARTESIAN_POINT('Origin',(0.0499999999999935,-42.0701004838369,
-234.90005));
#212410=CARTESIAN_POINT('',(1.25,-42.8201004838369,-234.90005));
#212411=CARTESIAN_POINT('Origin',(1.25,-42.0701004838369,-234.90005));
#212412=CARTESIAN_POINT('',(1.25,-43.2701004838368,-235.35005));
#212413=CARTESIAN_POINT('Origin',(1.25,-43.2701004838368,-234.90005));
#212414=CARTESIAN_POINT('Origin',(1.25,-42.0701004838369,-235.35005));
#212415=CARTESIAN_POINT('Origin',(-296.501483394397,-43.270100483837,-234.90005));
#212416=CARTESIAN_POINT('',(8.87499999999984,-42.8201004838369,-234.90005));
#212417=CARTESIAN_POINT('',(8.87499999999984,-43.2701004838368,-235.35005));
#212418=CARTESIAN_POINT('Origin',(8.87499999999984,-43.2701004838368,-234.90005));
#212419=CARTESIAN_POINT('',(-296.501483394397,-43.270100483837,-235.35005));
#212420=CARTESIAN_POINT('',(-1.54373336646987E-15,-42.8201004838369,-234.90005));
#212421=CARTESIAN_POINT('Origin',(0.0499999999999945,-25.4138432731711,
-234.90005));
#212422=CARTESIAN_POINT('',(0.0499999999999959,-33.96456093117,-235.35005));
#212423=CARTESIAN_POINT('',(0.5,-33.96456093117,-234.90005));
#212424=CARTESIAN_POINT('Origin',(0.0499999999999959,-33.96456093117,-234.90005));
#212425=CARTESIAN_POINT('',(0.5,-33.96456093117,-234.90005));
#212426=CARTESIAN_POINT('',(0.0499999999999935,-42.0701004838369,-235.35005));
#212427=CARTESIAN_POINT('Origin',(8.87499999999984,-42.0701004838369,-234.90005));
#212428=CARTESIAN_POINT('',(9.62499999999984,-42.0701004838368,-234.90005));
#212429=CARTESIAN_POINT('',(10.0749999999998,-42.0701004838368,-235.35005));
#212430=CARTESIAN_POINT('Origin',(10.0749999999998,-42.0701004838368,-234.90005));
#212431=CARTESIAN_POINT('Origin',(8.87499999999984,-42.0701004838369,-235.35005));
#212432=CARTESIAN_POINT('Origin',(8.87499999999984,-42.0701004838369,-234.90005));
#212433=CARTESIAN_POINT('Origin',(1.25,-33.96456093117,-234.90005));
#212434=CARTESIAN_POINT('',(1.25,-32.76456093117,-235.35005));
#212435=CARTESIAN_POINT('',(1.25,-33.21456093117,-234.90005));
#212436=CARTESIAN_POINT('Origin',(1.25,-32.76456093117,-234.90005));
#212437=CARTESIAN_POINT('Origin',(1.25,-33.96456093117,-234.90005));
#212438=CARTESIAN_POINT('Origin',(1.25,-33.96456093117,-235.35005));
#212439=CARTESIAN_POINT('Origin',(10.075,-25.4138432731712,-234.90005));
#212440=CARTESIAN_POINT('',(9.62499999999984,-33.96456093117,-234.90005));
#212441=CARTESIAN_POINT('',(10.075,-33.96456093117,-235.35005));
#212442=CARTESIAN_POINT('Origin',(10.0749999999998,-33.96456093117,-234.90005));
#212443=CARTESIAN_POINT('',(10.075,-33.96456093117,-235.35005));
#212444=CARTESIAN_POINT('',(9.62499999999984,-42.0701004838368,-234.90005));
#212445=CARTESIAN_POINT('Origin',(-296.501483394397,-32.7645609311699,-234.90005));
#212446=CARTESIAN_POINT('',(8.87499999999984,-32.76456093117,-235.35005));
#212447=CARTESIAN_POINT('',(8.87499999999984,-33.21456093117,-234.90005));
#212448=CARTESIAN_POINT('Origin',(8.87499999999984,-32.76456093117,-234.90005));
#212449=CARTESIAN_POINT('',(0.,-33.21456093117,-234.90005));
#212450=CARTESIAN_POINT('',(-296.501483394397,-32.7645609311699,-235.35005));
#212451=CARTESIAN_POINT('Origin',(8.87499999999984,-33.96456093117,-234.90005));
#212452=CARTESIAN_POINT('Origin',(8.87499999999984,-33.96456093117,-234.90005));
#212453=CARTESIAN_POINT('Origin',(8.87499999999984,-33.96456093117,-235.35005));
#212454=CARTESIAN_POINT('Origin',(33.7514626427707,-44.5701004838368,-234.90005));
#212455=CARTESIAN_POINT('',(34.6086426463967,-45.4098876243575,-235.35005));
#212456=CARTESIAN_POINT('',(34.2872001450369,-45.0949674466622,-234.90005));
#212457=CARTESIAN_POINT('Origin',(34.6086426463967,-45.4098876243575,-234.90005));
#212458=CARTESIAN_POINT('',(33.7514626427707,-43.8201004838368,-234.90005));
#212459=CARTESIAN_POINT('Origin',(33.7514626427707,-44.5701004838368,-234.90005));
#212460=CARTESIAN_POINT('',(33.7514626427707,-43.3701004838369,-235.35005));
#212461=CARTESIAN_POINT('Origin',(33.7514626427707,-43.3701004838369,-234.90005));
#212462=CARTESIAN_POINT('Origin',(33.7514626427707,-44.5701004838368,-235.35005));
#212463=CARTESIAN_POINT('Origin',(-296.501483394397,-43.3701004838369,-234.90005));
#212464=CARTESIAN_POINT('',(31.625,-43.8201004838368,-234.90005));
#212465=CARTESIAN_POINT('',(31.625,-43.3701004838369,-235.35005));
#212466=CARTESIAN_POINT('Origin',(31.625,-43.3701004838369,-234.90005));
#212467=CARTESIAN_POINT('',(-296.501483394397,-43.3701004838369,-235.35005));
#212468=CARTESIAN_POINT('',(-1.23757166668304E-15,-43.8201004838368,-234.90005));
#212469=CARTESIAN_POINT('Origin',(-6.29739814579425E-15,-11.5034818258363,
-234.90005));
#212470=CARTESIAN_POINT('',(32.4281746031746,-47.5009260671432,-235.35005));
#212471=CARTESIAN_POINT('',(32.1269841269841,-47.1665844797626,-234.90005));
#212472=CARTESIAN_POINT('Origin',(32.4281746031746,-47.5009260671432,-234.90005));
#212473=CARTESIAN_POINT('Origin',(-6.29739814579425E-15,-11.5034818258363,
-234.90005));
#212474=CARTESIAN_POINT('Origin',(-6.29739814579425E-15,-11.5034818258363,
-235.35005));
#212475=CARTESIAN_POINT('Origin',(31.625,-44.5701004838368,-234.90005));
#212476=CARTESIAN_POINT('',(30.875,-44.5701004838368,-234.90005));
#212477=CARTESIAN_POINT('',(30.425,-44.5701004838368,-235.35005));
#212478=CARTESIAN_POINT('Origin',(30.425,-44.5701004838368,-234.90005));
#212479=CARTESIAN_POINT('Origin',(31.625,-44.5701004838368,-235.35005));
#212480=CARTESIAN_POINT('Origin',(31.625,-44.5701004838368,-234.90005));
#212481=CARTESIAN_POINT('Origin',(31.625,-46.609348500795,-234.90005));
#212482=CARTESIAN_POINT('',(30.425,-46.609348500795,-235.35005));
#212483=CARTESIAN_POINT('',(30.875,-46.609348500795,-234.90005));
#212484=CARTESIAN_POINT('Origin',(30.425,-46.609348500795,-234.90005));
#212485=CARTESIAN_POINT('Origin',(31.625,-46.609348500795,-234.90005));
#212486=CARTESIAN_POINT('Origin',(31.625,-46.609348500795,-235.35005));
#212487=CARTESIAN_POINT('Origin',(30.425,-25.4138432731711,-234.90005));
#212488=CARTESIAN_POINT('',(30.875,-44.5701004838368,-234.90005));
#212489=CARTESIAN_POINT('',(30.425,-46.609348500795,-235.35005));
#212490=CARTESIAN_POINT('Origin',(31.625,23.6023848491226,-234.90005));
#212491=CARTESIAN_POINT('',(32.4281746031746,24.4939624154707,-235.35005));
#212492=CARTESIAN_POINT('',(30.425,23.6023848491226,-235.35005));
#212493=CARTESIAN_POINT('Origin',(31.625,23.6023848491226,-235.35005));
#212494=CARTESIAN_POINT('',(32.1269841269841,24.1596208280901,-234.90005));
#212495=CARTESIAN_POINT('Origin',(32.4281746031746,24.4939624154707,-234.90005));
#212496=CARTESIAN_POINT('',(30.875,23.6023848491226,-234.90005));
#212497=CARTESIAN_POINT('Origin',(31.625,23.6023848491226,-234.90005));
#212498=CARTESIAN_POINT('Origin',(30.425,23.6023848491226,-234.90005));
#212499=CARTESIAN_POINT('Origin',(30.425,-25.4138432731711,-234.90005));
#212500=CARTESIAN_POINT('',(30.875,21.5631368321642,-234.90005));
#212501=CARTESIAN_POINT('',(30.425,21.5631368321642,-235.35005));
#212502=CARTESIAN_POINT('Origin',(30.425,21.5631368321642,-234.90005));
#212503=CARTESIAN_POINT('',(30.425,21.5631368321642,-235.35005));
#212504=CARTESIAN_POINT('',(30.875,23.6023848491225,-234.90005));
#212505=CARTESIAN_POINT('Origin',(-6.29739814579425E-15,-11.5034818258363,
-234.90005));
#212506=CARTESIAN_POINT('',(34.6086426463969,22.4029239726848,-235.35005));
#212507=CARTESIAN_POINT('',(34.2872001450371,22.0880037949896,-234.90005));
#212508=CARTESIAN_POINT('Origin',(34.6086426463969,22.4029239726848,-234.90005));
#212509=CARTESIAN_POINT('Origin',(-6.29739814579425E-15,-11.5034818258363,
-234.90005));
#212510=CARTESIAN_POINT('Origin',(-6.29739814579425E-15,-11.5034818258363,
-235.35005));
#212511=CARTESIAN_POINT('Origin',(31.625,21.5631368321642,-234.90005));
#212512=CARTESIAN_POINT('',(31.625,20.8131368321642,-234.90005));
#212513=CARTESIAN_POINT('',(31.625,20.3631368321642,-235.35005));
#212514=CARTESIAN_POINT('Origin',(31.625,20.3631368321642,-234.90005));
#212515=CARTESIAN_POINT('Origin',(31.625,21.5631368321642,-235.35005));
#212516=CARTESIAN_POINT('Origin',(31.625,21.5631368321642,-234.90005));
#212517=CARTESIAN_POINT('Origin',(33.751462642771,21.5631368321642,-234.90005));
#212518=CARTESIAN_POINT('',(33.751462642771,20.3631368321642,-235.35005));
#212519=CARTESIAN_POINT('',(33.751462642771,20.8131368321642,-234.90005));
#212520=CARTESIAN_POINT('Origin',(33.751462642771,20.3631368321642,-234.90005));
#212521=CARTESIAN_POINT('Origin',(33.751462642771,21.5631368321642,-234.90005));
#212522=CARTESIAN_POINT('Origin',(33.751462642771,21.5631368321642,-235.35005));
#212523=CARTESIAN_POINT('Origin',(-296.501483394397,20.3631368321642,-234.90005));
#212524=CARTESIAN_POINT('',(-1.23757166668304E-15,20.8131368321642,-234.90005));
#212525=CARTESIAN_POINT('',(-296.501483394397,20.3631368321642,-235.35005));
#212526=CARTESIAN_POINT('Origin',(0.,-11.5034818258363,-235.65005));
#212527=CARTESIAN_POINT('',(-9.37533200891943E-16,-19.1590213785032,-236.10005));
#212528=CARTESIAN_POINT('Origin',(0.,-11.5034818258363,-236.10005));
#212529=CARTESIAN_POINT('',(-9.92642306853574E-16,-19.6090213785032,-235.65005));
#212530=CARTESIAN_POINT('Origin',(-9.37533200891943E-16,-19.1590213785032,
-235.65005));
#212531=CARTESIAN_POINT('Origin',(0.,-11.5034818258363,-235.65005));
#212532=CARTESIAN_POINT('Origin',(0.,-11.5034818258363,-235.65005));
#212533=CARTESIAN_POINT('',(-5.66442007243621E-16,-16.1288318258363,-235.65005));
#212534=CARTESIAN_POINT('Origin',(0.,-11.5034818258363,-235.65005));
#212535=CARTESIAN_POINT('',(-6.21551113205252E-16,-16.5788318258363,-236.10005));
#212536=CARTESIAN_POINT('Origin',(-6.21551113205252E-16,-16.5788318258363,
-235.65005));
#212537=CARTESIAN_POINT('Origin',(0.,-11.5034818258363,-236.10005));
#212538=CARTESIAN_POINT('Origin',(7.14692237356698E-14,623.509175991979,
-234.90005));
#212539=CARTESIAN_POINT('',(23.121090730514,-58.5338529228103,-234.90005));
#212540=CARTESIAN_POINT('',(23.1363368618431,-58.9835945769624,-235.35005));
#212541=CARTESIAN_POINT('Origin',(23.1363368618431,-58.9835945769624,-234.90005));
#212542=CARTESIAN_POINT('Origin',(7.14692237356698E-14,623.509175991979,
-235.35005));
#212543=CARTESIAN_POINT('Origin',(7.14692237356698E-14,623.509175991979,
-234.90005));
#212544=CARTESIAN_POINT('Origin',(22.9178089794592,-52.5372975341153,-234.90005));
#212545=CARTESIAN_POINT('',(25.8434867215177,-57.775656986236,-234.90005));
#212546=CARTESIAN_POINT('',(26.0629125521721,-58.168533945145,-235.35005));
#212547=CARTESIAN_POINT('Origin',(26.0629125521721,-58.168533945145,-234.90005));
#212548=CARTESIAN_POINT('Origin',(22.9178089794592,-52.5372975341153,-235.35005));
#212549=CARTESIAN_POINT('Origin',(22.9178089794592,-52.5372975341153,-234.90005));
#212550=CARTESIAN_POINT('Origin',(-6.29739814579425E-15,-11.5034818258363,
-234.90005));
#212551=CARTESIAN_POINT('',(43.9682643235187,-41.0972604351516,-234.90005));
#212552=CARTESIAN_POINT('',(44.3415797753222,-41.3485283667401,-235.35005));
#212553=CARTESIAN_POINT('Origin',(44.3415797753222,-41.3485283667401,-234.90005));
#212554=CARTESIAN_POINT('Origin',(-6.29739814579425E-15,-11.5034818258363,
-235.35005));
#212555=CARTESIAN_POINT('Origin',(-6.29739814579425E-15,-11.5034818258363,
-234.90005));
#212556=CARTESIAN_POINT('Origin',(38.9907249661392,-37.7470213473046,-234.90005));
#212557=CARTESIAN_POINT('',(44.9862076791357,-37.9798024422418,-234.90005));
#212558=CARTESIAN_POINT('',(45.4358688826104,-37.9972610243621,-235.35005));
#212559=CARTESIAN_POINT('Origin',(45.4358688826105,-37.9972610243621,-234.90005));
#212560=CARTESIAN_POINT('Origin',(38.9907249661392,-37.7470213473046,-235.35005));
#212561=CARTESIAN_POINT('Origin',(38.9907249661392,-37.7470213473046,-234.90005));
#212562=CARTESIAN_POINT('Origin',(-636.934816028482,-11.5034818258361,-234.90005));
#212563=CARTESIAN_POINT('',(44.9862076791357,14.9728387905693,-234.90005));
#212564=CARTESIAN_POINT('',(45.4358688826104,14.9902973726896,-235.35005));
#212565=CARTESIAN_POINT('Origin',(45.4358688826104,14.9902973726896,-234.90005));
#212566=CARTESIAN_POINT('Origin',(-636.934816028482,-11.5034818258361,-235.35005));
#212567=CARTESIAN_POINT('Origin',(-636.934816028482,-11.5034818258361,-234.90005));
#212568=CARTESIAN_POINT('Origin',(38.9907249661392,14.740057695632,-234.90005));
#212569=CARTESIAN_POINT('',(43.9682643235187,18.0902967834791,-234.90005));
#212570=CARTESIAN_POINT('',(44.3415797753222,18.3415647150676,-235.35005));
#212571=CARTESIAN_POINT('Origin',(44.3415797753222,18.3415647150676,-234.90005));
#212572=CARTESIAN_POINT('Origin',(38.9907249661392,14.740057695632,-235.35005));
#212573=CARTESIAN_POINT('Origin',(38.9907249661392,14.740057695632,-234.90005));
#212574=CARTESIAN_POINT('Origin',(-6.29739814579425E-15,-11.5034818258363,
-234.90005));
#212575=CARTESIAN_POINT('',(28.0091475455229,33.4908250781833,-234.90005));
#212576=CARTESIAN_POINT('',(28.2469610624189,33.872852212274,-235.35005));
#212577=CARTESIAN_POINT('Origin',(28.2469610624189,33.872852212274,-234.90005));
#212578=CARTESIAN_POINT('Origin',(-6.29739814579425E-15,-11.5034818258363,
-235.35005));
#212579=CARTESIAN_POINT('Origin',(-6.29739814579425E-15,-11.5034818258363,
-234.90005));
#212580=CARTESIAN_POINT('Origin',(24.838300653577,28.3971299569735,-234.90005));
#212581=CARTESIAN_POINT('',(25.5706493501227,34.3522676872588,-234.90005));
#212582=CARTESIAN_POINT('',(25.6255755023637,34.7989030170302,-235.35005));
#212583=CARTESIAN_POINT('Origin',(25.6255755023637,34.7989030170302,-234.90005));
#212584=CARTESIAN_POINT('Origin',(24.838300653577,28.3971299569735,-235.35005));
#212585=CARTESIAN_POINT('Origin',(24.838300653577,28.3971299569735,-234.90005));
#212586=CARTESIAN_POINT('Origin',(-2.61456814389029E-14,-173.57701443073,
-234.90005));
#212587=CARTESIAN_POINT('Origin',(-2.61456814389029E-14,-173.57701443073,
-235.35005));
#212588=CARTESIAN_POINT('Origin',(-2.61456814389029E-14,-173.57701443073,
-234.90005));
#212589=CARTESIAN_POINT('Origin',(7.14692237356698E-14,623.509175991979,
-234.90005));
#212590=CARTESIAN_POINT('',(23.0651882489741,-56.8848001909192,-235.35005));
#212591=CARTESIAN_POINT('',(23.0804343803032,-57.3345418450714,-234.90005));
#212592=CARTESIAN_POINT('Origin',(23.0651882489741,-56.8848001909192,-234.90005));
#212593=CARTESIAN_POINT('Origin',(7.14692237356698E-14,623.509175991979,
-234.90005));
#212594=CARTESIAN_POINT('Origin',(7.14692237356698E-14,623.509175991979,
-235.35005));
#212595=CARTESIAN_POINT('Origin',(22.9178089794592,-52.5372975341153,-234.90005));
#212596=CARTESIAN_POINT('',(25.0389253424516,-56.3351081369028,-235.35005));
#212597=CARTESIAN_POINT('',(25.258351173106,-56.7279850958119,-234.90005));
#212598=CARTESIAN_POINT('Origin',(25.0389253424516,-56.3351081369028,-234.90005));
#212599=CARTESIAN_POINT('Origin',(22.9178089794592,-52.5372975341153,-234.90005));
#212600=CARTESIAN_POINT('Origin',(22.9178089794592,-52.5372975341153,-235.35005));
#212601=CARTESIAN_POINT('Origin',(-6.29739814579425E-15,-11.5034818258363,
-234.90005));
#212602=CARTESIAN_POINT('',(42.5994410002394,-40.1759446859937,-235.35005));
#212603=CARTESIAN_POINT('',(42.9727564520428,-40.4272126175822,-234.90005));
#212604=CARTESIAN_POINT('Origin',(42.5994410002394,-40.1759446859937,-234.90005));
#212605=CARTESIAN_POINT('Origin',(-6.29739814579425E-15,-11.5034818258363,
-234.90005));
#212606=CARTESIAN_POINT('Origin',(-6.29739814579425E-15,-11.5034818258363,
-235.35005));
#212607=CARTESIAN_POINT('Origin',(38.9907249661392,-37.7470213473046,-234.90005));
#212608=CARTESIAN_POINT('',(43.3374499330618,-37.915787641134,-235.35005));
#212609=CARTESIAN_POINT('',(43.7871111365364,-37.9332462232544,-234.90005));
#212610=CARTESIAN_POINT('Origin',(43.3374499330618,-37.915787641134,-234.90005));
#212611=CARTESIAN_POINT('Origin',(38.9907249661392,-37.7470213473046,-234.90005));
#212612=CARTESIAN_POINT('Origin',(38.9907249661392,-37.7470213473046,-235.35005));
#212613=CARTESIAN_POINT('Origin',(-636.934816028482,-11.5034818258361,-234.90005));
#212614=CARTESIAN_POINT('',(43.3374499330618,14.9088239894616,-235.35005));
#212615=CARTESIAN_POINT('',(43.7871111365364,14.9262825715819,-234.90005));
#212616=CARTESIAN_POINT('Origin',(43.3374499330618,14.9088239894616,-234.90005));
#212617=CARTESIAN_POINT('Origin',(-636.934816028482,-11.5034818258361,-234.90005));
#212618=CARTESIAN_POINT('Origin',(-636.934816028482,-11.5034818258361,-235.35005));
#212619=CARTESIAN_POINT('Origin',(38.9907249661392,14.740057695632,-234.90005));
#212620=CARTESIAN_POINT('',(42.5994410002394,17.1689810343211,-235.35005));
#212621=CARTESIAN_POINT('',(42.9727564520429,17.4202489659097,-234.90005));
#212622=CARTESIAN_POINT('Origin',(42.5994410002394,17.1689810343211,-234.90005));
#212623=CARTESIAN_POINT('Origin',(38.9907249661392,14.740057695632,-234.90005));
#212624=CARTESIAN_POINT('Origin',(38.9907249661392,14.740057695632,-235.35005));
#212625=CARTESIAN_POINT('Origin',(-6.29739814579425E-15,-11.5034818258363,
-234.90005));
#212626=CARTESIAN_POINT('',(27.1371646502378,32.0900589198506,-235.35005));
#212627=CARTESIAN_POINT('',(27.3749781671338,32.4720860539414,-234.90005));
#212628=CARTESIAN_POINT('Origin',(27.1371646502378,32.0900589198506,-234.90005));
#212629=CARTESIAN_POINT('Origin',(-6.29739814579425E-15,-11.5034818258363,
-234.90005));
#212630=CARTESIAN_POINT('Origin',(-6.29739814579425E-15,-11.5034818258363,
-235.35005));
#212631=CARTESIAN_POINT('Origin',(24.838300653577,28.3971299569735,-234.90005));
#212632=CARTESIAN_POINT('',(25.3692534585727,32.7146048114303,-235.35005));
#212633=CARTESIAN_POINT('',(25.4241796108136,33.1612401412018,-234.90005));
#212634=CARTESIAN_POINT('Origin',(25.3692534585727,32.7146048114303,-234.90005));
#212635=CARTESIAN_POINT('Origin',(24.838300653577,28.3971299569735,-234.90005));
#212636=CARTESIAN_POINT('Origin',(24.838300653577,28.3971299569735,-235.35005));
#212637=CARTESIAN_POINT('Origin',(-2.61456814389029E-14,-173.57701443073,
-234.90005));
#212638=CARTESIAN_POINT('Origin',(-2.61456814389029E-14,-173.57701443073,
-234.90005));
#212639=CARTESIAN_POINT('Origin',(-2.61456814389029E-14,-173.57701443073,
-235.35005));
#212640=CARTESIAN_POINT('Origin',(6.95148506756697,-6.01736880073005,-234.90005));
#212641=CARTESIAN_POINT('',(6.08254860609655,-5.18975208634635,-235.35005));
#212642=CARTESIAN_POINT('',(6.40839977914796,-5.50010835424024,-234.90005));
#212643=CARTESIAN_POINT('Origin',(6.08254860609655,-5.18975208634635,-234.90005));
#212644=CARTESIAN_POINT('',(6.36274467860838,-6.48200280121742,-234.90005));
#212645=CARTESIAN_POINT('Origin',(6.95148506756697,-6.01736880073005,-234.90005));
#212646=CARTESIAN_POINT('',(5.76949205973895,-5.81026368383122,-235.35005));
#212647=CARTESIAN_POINT('Ctrl Pts',(5.76949205973895,-5.81026368383121,
-235.35005));
#212648=CARTESIAN_POINT('Ctrl Pts',(5.82092507341363,-5.86238576252255,
-235.35005));
#212649=CARTESIAN_POINT('Ctrl Pts',(5.87146206806168,-5.91503600112616,
-235.33821291833));
#212650=CARTESIAN_POINT('Ctrl Pts',(6.00423457196882,-6.05699737629993,
-235.282379503985));
#212651=CARTESIAN_POINT('Ctrl Pts',(6.07889780142463,-6.14101690884923,
-235.222495970419));
#212652=CARTESIAN_POINT('Ctrl Pts',(6.22023885093968,-6.30512731290958,
-235.083822800187));
#212653=CARTESIAN_POINT('Ctrl Pts',(6.29326617328539,-6.39403176703485,
-234.990808270705));
#212654=CARTESIAN_POINT('Ctrl Pts',(6.36151501319033,-6.48044497931282,
-234.901656863128));
#212655=CARTESIAN_POINT('Ctrl Pts',(6.36212991841606,-6.48122383507554,
-234.900853430267));
#212656=CARTESIAN_POINT('Ctrl Pts',(6.36274467860838,-6.48200280121742,
-234.90005));
#212657=CARTESIAN_POINT('Origin',(6.95148506756697,-6.01736880073005,-235.35005));
#212658=CARTESIAN_POINT('Origin',(-147.944423723881,-166.906703884593,-234.90005));
#212659=CARTESIAN_POINT('',(7.1259980697973,-4.09420716929315,-235.35005));
#212660=CARTESIAN_POINT('',(7.45184924284871,-4.40456343718705,-234.90005));
#212661=CARTESIAN_POINT('Origin',(7.1259980697973,-4.09420716929315,-234.90005));
#212662=CARTESIAN_POINT('',(6.10697827817035,-5.81657868152891,-234.90005));
#212663=CARTESIAN_POINT('',(-147.944423723881,-166.906703884593,-235.35005));
#212664=CARTESIAN_POINT('Origin',(7.99493453126772,-4.92182388367686,-234.90005));
#212665=CARTESIAN_POINT('',(8.92138760391815,-4.15914131263135,-235.35005));
#212666=CARTESIAN_POINT('Origin',(7.99493453126772,-4.92182388367686,-235.35005));
#212667=CARTESIAN_POINT('',(8.57396770167424,-4.44514727677342,-234.90005));
#212668=CARTESIAN_POINT('Origin',(8.92138760391815,-4.15914131263135,-234.90005));
#212669=CARTESIAN_POINT('Origin',(7.99493453126772,-4.92182388367686,-234.90005));
#212670=CARTESIAN_POINT('Origin',(0.,-11.5034818258363,-234.90005));
#212671=CARTESIAN_POINT('',(11.4710456282303,-10.1086318165856,-235.35005));
#212672=CARTESIAN_POINT('',(11.0243360211906,-10.1629505700546,-234.90005));
#212673=CARTESIAN_POINT('Origin',(11.4710456282303,-10.1086318165856,-234.90005));
#212674=CARTESIAN_POINT('Origin',(0.,-11.5034818258363,-234.90005));
#212675=CARTESIAN_POINT('Origin',(0.,-11.5034818258363,-235.35005));
#212676=CARTESIAN_POINT('Origin',(10.2798200094577,-10.2534818258363,-234.90005));
#212677=CARTESIAN_POINT('',(10.2798200094577,-11.4534818258363,-235.35005));
#212678=CARTESIAN_POINT('',(10.2798200094577,-11.0034818258363,-234.90005));
#212679=CARTESIAN_POINT('Origin',(10.2798200094577,-11.4534818258363,-234.90005));
#212680=CARTESIAN_POINT('Origin',(10.2798200094577,-10.2534818258363,-234.90005));
#212681=CARTESIAN_POINT('Origin',(10.2798200094577,-10.2534818258363,-235.35005));
#212682=CARTESIAN_POINT('Origin',(-296.501483394397,-11.4534818258365,-234.90005));
#212683=CARTESIAN_POINT('',(8.76687405914145,-11.4534818258363,-235.35005));
#212684=CARTESIAN_POINT('',(8.76687405914145,-11.0034818258363,-234.90005));
#212685=CARTESIAN_POINT('Origin',(8.76687405914145,-11.4534818258363,-234.90005));
#212686=CARTESIAN_POINT('',(-2.22174260618994E-13,-11.0034818258363,-234.90005));
#212687=CARTESIAN_POINT('',(-296.501483394397,-11.4534818258365,-235.35005));
#212688=CARTESIAN_POINT('Origin',(8.76687405914145,-10.2534818258363,-234.90005));
#212689=CARTESIAN_POINT('',(8.02438338364376,-10.3593477636964,-234.90005));
#212690=CARTESIAN_POINT('',(8.1016440740309,-11.2522155575736,-235.35005));
#212691=CARTESIAN_POINT('Ctrl Pts',(8.02438338364377,-10.3593477636964,
-234.90005));
#212692=CARTESIAN_POINT('Ctrl Pts',(8.02452345554005,-10.3603301578355,
-234.900853430281));
#212693=CARTESIAN_POINT('Ctrl Pts',(8.02466334747473,-10.3613125808142,
-234.901656863113));
#212694=CARTESIAN_POINT('Ctrl Pts',(8.04016643948375,-10.4703300185997,
-234.990808271414));
#212695=CARTESIAN_POINT('Ctrl Pts',(8.05417784702261,-10.5845257804583,
-235.083822800183));
#212696=CARTESIAN_POINT('Ctrl Pts',(8.07553226267948,-10.8000565344901,
-235.222495970419));
#212697=CARTESIAN_POINT('Ctrl Pts',(8.08487817822972,-10.9120678443883,
-235.282379503985));
#212698=CARTESIAN_POINT('Ctrl Pts',(8.09610373786709,-11.1061182415686,
-235.33821291833));
#212699=CARTESIAN_POINT('Ctrl Pts',(8.09937411333572,-11.1790246205581,
-235.35005));
#212700=CARTESIAN_POINT('Ctrl Pts',(8.10164407403091,-11.2522155575736,
-235.35005));
#212701=CARTESIAN_POINT('Origin',(8.76687405914145,-10.2534818258363,-234.90005));
#212702=CARTESIAN_POINT('Origin',(8.76687405914145,-10.2534818258363,-235.35005));
#212703=CARTESIAN_POINT('Origin',(8.76687405914144,-12.7534818258363,-234.90005));
#212704=CARTESIAN_POINT('',(8.76687405914144,-11.5534818258363,-235.35005));
#212705=CARTESIAN_POINT('',(8.76687405914144,-12.0034818258363,-234.90005));
#212706=CARTESIAN_POINT('Origin',(8.76687405914144,-11.5534818258363,-234.90005));
#212707=CARTESIAN_POINT('',(8.02438338364376,-12.6476158879763,-234.90005));
#212708=CARTESIAN_POINT('Origin',(8.76687405914144,-12.7534818258363,-234.90005));
#212709=CARTESIAN_POINT('',(8.1016440740309,-11.7547480940991,-235.35005));
#212710=CARTESIAN_POINT('Ctrl Pts',(8.10164407403091,-11.7547480940991,
-235.35005));
#212711=CARTESIAN_POINT('Ctrl Pts',(8.09937411333572,-11.8279390311146,
-235.35005));
#212712=CARTESIAN_POINT('Ctrl Pts',(8.09610373786709,-11.9008454101041,
-235.33821291833));
#212713=CARTESIAN_POINT('Ctrl Pts',(8.08487817822972,-12.0948958072844,
-235.282379503985));
#212714=CARTESIAN_POINT('Ctrl Pts',(8.07553226267947,-12.2069071171825,
-235.222495970419));
#212715=CARTESIAN_POINT('Ctrl Pts',(8.05417784702484,-12.4224378711919,
-235.083822800197));
#212716=CARTESIAN_POINT('Ctrl Pts',(8.04016643880974,-12.5366336378126,
-234.990808267567));
#212717=CARTESIAN_POINT('Ctrl Pts',(8.02466334748842,-12.6456510707622,
-234.90165686319));
#212718=CARTESIAN_POINT('Ctrl Pts',(8.0245234555264,-12.6466334939328,-234.900853430203));
#212719=CARTESIAN_POINT('Ctrl Pts',(8.02438338364376,-12.6476158879763,
-234.90005));
#212720=CARTESIAN_POINT('Origin',(8.76687405914144,-12.7534818258363,-235.35005));
#212721=CARTESIAN_POINT('Origin',(-296.501483394397,-11.5534818258362,-234.90005));
#212722=CARTESIAN_POINT('',(10.2798200094577,-11.5534818258363,-235.35005));
#212723=CARTESIAN_POINT('',(10.2798200094577,-12.0034818258363,-234.90005));
#212724=CARTESIAN_POINT('Origin',(10.2798200094577,-11.5534818258363,-234.90005));
#212725=CARTESIAN_POINT('',(-2.22174260618994E-13,-12.0034818258363,-234.90005));
#212726=CARTESIAN_POINT('',(-296.501483394397,-11.5534818258362,-235.35005));
#212727=CARTESIAN_POINT('Origin',(10.2798200094577,-12.7534818258363,-234.90005));
#212728=CARTESIAN_POINT('',(11.4710456282303,-12.8983318350871,-235.35005));
#212729=CARTESIAN_POINT('',(11.0243360211906,-12.844013081618,-234.90005));
#212730=CARTESIAN_POINT('Origin',(11.4710456282303,-12.8983318350871,-234.90005));
#212731=CARTESIAN_POINT('Origin',(10.2798200094577,-12.7534818258363,-234.90005));
#212732=CARTESIAN_POINT('Origin',(10.2798200094577,-12.7534818258363,-235.35005));
#212733=CARTESIAN_POINT('Origin',(0.,-11.5034818258363,-234.90005));
#212734=CARTESIAN_POINT('',(8.92138760391814,-18.8478223390413,-235.35005));
#212735=CARTESIAN_POINT('',(8.57396770167423,-18.5618163748993,-234.90005));
#212736=CARTESIAN_POINT('Origin',(8.92138760391814,-18.8478223390413,-234.90005));
#212737=CARTESIAN_POINT('Origin',(0.,-11.5034818258363,-234.90005));
#212738=CARTESIAN_POINT('Origin',(0.,-11.5034818258363,-235.35005));
#212739=CARTESIAN_POINT('Origin',(7.99493453126771,-18.0851397679958,-234.90005));
#212740=CARTESIAN_POINT('',(7.1259980697973,-18.9127564823795,-235.35005));
#212741=CARTESIAN_POINT('',(7.4518492428487,-18.6024002144856,-234.90005));
#212742=CARTESIAN_POINT('Origin',(7.12599806979729,-18.9127564823795,-234.90005));
#212743=CARTESIAN_POINT('Origin',(7.99493453126771,-18.0851397679958,-234.90005));
#212744=CARTESIAN_POINT('Origin',(7.99493453126771,-18.0851397679958,-235.35005));
#212745=CARTESIAN_POINT('Origin',(-5.70871573332976,-5.43725435410305,-234.90005));
#212746=CARTESIAN_POINT('',(6.08254860609655,-17.8172115653263,-235.35005));
#212747=CARTESIAN_POINT('',(6.40839977914795,-17.5068552974324,-234.90005));
#212748=CARTESIAN_POINT('Origin',(6.08254860609655,-17.8172115653263,-234.90005));
#212749=CARTESIAN_POINT('',(6.40839977914795,-17.5068552974324,-234.90005));
#212750=CARTESIAN_POINT('',(7.1259980697973,-18.9127564823795,-235.35005));
#212751=CARTESIAN_POINT('Origin',(6.95148506756696,-16.9895948509426,-234.90005));
#212752=CARTESIAN_POINT('',(6.36274467860837,-16.5249608504553,-234.90005));
#212753=CARTESIAN_POINT('',(5.76949205973894,-17.1966999678414,-235.35005));
#212754=CARTESIAN_POINT('Ctrl Pts',(6.36274467860837,-16.5249608504552,
-234.90005));
#212755=CARTESIAN_POINT('Ctrl Pts',(6.36212991839126,-16.5257398166285,
-234.900853430299));
#212756=CARTESIAN_POINT('Ctrl Pts',(6.36151501321541,-16.5265186723281,
-234.901656863095));
#212757=CARTESIAN_POINT('Ctrl Pts',(6.2932661720145,-16.6129318862469,-234.990808272352));
#212758=CARTESIAN_POINT('Ctrl Pts',(6.22023885094755,-16.7018363387539,
-235.083822800179));
#212759=CARTESIAN_POINT('Ctrl Pts',(6.0788978014246,-16.8659467428234,-235.222495970419));
#212760=CARTESIAN_POINT('Ctrl Pts',(6.0042345719688,-16.9499662753727,-235.282379503985));
#212761=CARTESIAN_POINT('Ctrl Pts',(5.87146206806167,-17.0919276505465,
-235.33821291833));
#212762=CARTESIAN_POINT('Ctrl Pts',(5.82092507341363,-17.1445778891501,
-235.35005));
#212763=CARTESIAN_POINT('Ctrl Pts',(5.76949205973896,-17.1966999678414,
-235.35005));
#212764=CARTESIAN_POINT('Origin',(6.95148506756696,-16.9895948509426,-234.90005));
#212765=CARTESIAN_POINT('Origin',(6.95148506756696,-16.9895948509426,-235.35005));
#212766=CARTESIAN_POINT('Origin',(1.25,-2.73660776669487,-234.90005));
#212767=CARTESIAN_POINT('',(0.0499999999999959,-2.73660776669487,-235.35005));
#212768=CARTESIAN_POINT('',(0.5,-2.73660776669487,-234.90005));
#212769=CARTESIAN_POINT('Origin',(0.0499999999999959,-2.73660776669487,
-234.90005));
#212770=CARTESIAN_POINT('',(1.14413406213993,-3.47909844219256,-234.90005));
#212771=CARTESIAN_POINT('Origin',(1.25,-2.73660776669487,-234.90005));
#212772=CARTESIAN_POINT('',(0.251266268262739,-3.40183775180542,-235.35005));
#212773=CARTESIAN_POINT('Ctrl Pts',(0.251266268262739,-3.40183775180541,
-235.35005));
#212774=CARTESIAN_POINT('Ctrl Pts',(0.32445720527824,-3.4041077125006,-235.35005));
#212775=CARTESIAN_POINT('Ctrl Pts',(0.397363584267788,-3.40737808796923,
-235.33821291833));
#212776=CARTESIAN_POINT('Ctrl Pts',(0.591413981447983,-3.4186036476066,
-235.282379503985));
#212777=CARTESIAN_POINT('Ctrl Pts',(0.703425291346113,-3.42794956315684,
-235.222495970419));
#212778=CARTESIAN_POINT('Ctrl Pts',(0.918956045360102,-3.44930397881193,
-235.083822800194));
#212779=CARTESIAN_POINT('Ctrl Pts',(1.03315181082866,-3.46331538686338,
-234.990808268499));
#212780=CARTESIAN_POINT('Ctrl Pts',(1.14216924494769,-3.47881847835101,
-234.901656863173));
#212781=CARTESIAN_POINT('Ctrl Pts',(1.14315166807461,-3.4789583703068,-234.900853430221));
#212782=CARTESIAN_POINT('Ctrl Pts',(1.14413406213993,-3.47909844219256,
-234.90005));
#212783=CARTESIAN_POINT('Origin',(1.25,-2.73660776669487,-235.35005));
#212784=CARTESIAN_POINT('Origin',(0.0499999999999945,-25.4138432731711,
-234.90005));
#212785=CARTESIAN_POINT('',(0.0499999999999981,-1.22366181637858,-235.35005));
#212786=CARTESIAN_POINT('',(0.5,-1.22366181637858,-234.90005));
#212787=CARTESIAN_POINT('Origin',(0.0499999999999981,-1.22366181637858,
-234.90005));
#212788=CARTESIAN_POINT('',(0.5,-1.22366181637858,-234.90005));
#212789=CARTESIAN_POINT('',(0.0499999999999959,-2.73660776669487,-235.35005));
#212790=CARTESIAN_POINT('Origin',(1.25,-1.22366181637858,-234.90005));
#212791=CARTESIAN_POINT('',(1.39485000925072,-0.0324361976060192,-235.35005));
#212792=CARTESIAN_POINT('Origin',(1.25,-1.22366181637858,-235.35005));
#212793=CARTESIAN_POINT('',(1.3405312557817,-0.479145804645727,-234.90005));
#212794=CARTESIAN_POINT('Origin',(1.39485000925072,-0.0324361976060193,
-234.90005));
#212795=CARTESIAN_POINT('Origin',(1.25,-1.22366181637858,-234.90005));
#212796=CARTESIAN_POINT('Origin',(0.,-11.5034818258363,-234.90005));
#212797=CARTESIAN_POINT('',(6.90132755171766,-2.23513934310776,-235.35005));
#212798=CARTESIAN_POINT('',(6.63257355852517,-2.59607048770891,-234.90005));
#212799=CARTESIAN_POINT('Origin',(6.90132755171766,-2.23513934310776,-234.90005));
#212800=CARTESIAN_POINT('Origin',(0.,-11.5034818258363,-234.90005));
#212801=CARTESIAN_POINT('Origin',(0.,-11.5034818258363,-235.35005));
#212802=CARTESIAN_POINT('Origin',(6.18465023653769,-3.19762239537748,-234.90005));
#212803=CARTESIAN_POINT('',(7.05358669800811,-4.02523910976119,-235.35005));
#212804=CARTESIAN_POINT('',(6.7277355249567,-3.7148828418673,-234.90005));
#212805=CARTESIAN_POINT('Origin',(7.05358669800812,-4.0252391097612,-234.90005));
#212806=CARTESIAN_POINT('Origin',(6.18465023653769,-3.19762239537748,-234.90005));
#212807=CARTESIAN_POINT('Origin',(6.18465023653769,-3.19762239537748,-235.35005));
#212808=CARTESIAN_POINT('Origin',(-148.016835095671,-166.837735825062,-234.90005));
#212809=CARTESIAN_POINT('',(6.01013723430737,-5.12078402681439,-235.35005));
#212810=CARTESIAN_POINT('',(5.68428606125595,-4.81042775892049,-234.90005));
#212811=CARTESIAN_POINT('Origin',(6.01013723430736,-5.12078402681438,-234.90005));
#212812=CARTESIAN_POINT('',(5.38286456027834,-5.12689808620916,-234.90005));
#212813=CARTESIAN_POINT('',(-148.016835095671,-166.837735825062,-235.35005));
#212814=CARTESIAN_POINT('Origin',(5.14120077283694,-4.29316731243068,-234.90005));
#212815=CARTESIAN_POINT('',(4.70577833960231,-4.90382867901287,-234.90005));
#212816=CARTESIAN_POINT('',(5.40560135635379,-5.46367674487279,-235.35005));
#212817=CARTESIAN_POINT('Ctrl Pts',(4.70577833960231,-4.90382867901288,
-234.90005));
#212818=CARTESIAN_POINT('Ctrl Pts',(4.70658630944744,-4.9044047891374,-234.900853430186));
#212819=CARTESIAN_POINT('Ctrl Pts',(4.70739417634903,-4.90498104967104,
-234.901656863208));
#212820=CARTESIAN_POINT('Ctrl Pts',(4.79702737541902,-4.96894225601165,
-234.990808266726));
#212821=CARTESIAN_POINT('Ctrl Pts',(4.88938149377006,-5.03755500803373,
-235.083822800201));
#212822=CARTESIAN_POINT('Ctrl Pts',(5.0601779954728,-5.17073936145207,-235.222495970419));
#212823=CARTESIAN_POINT('Ctrl Pts',(5.14773261812957,-5.24122388268896,
-235.282379503985));
#212824=CARTESIAN_POINT('Ctrl Pts',(5.29598922334359,-5.36692809441377,
-235.33821291833));
#212825=CARTESIAN_POINT('Ctrl Pts',(5.35103724699188,-5.41484208553839,
-235.35005));
#212826=CARTESIAN_POINT('Ctrl Pts',(5.40560135635379,-5.46367674487279,
-235.35005));
#212827=CARTESIAN_POINT('Origin',(5.14120077283694,-4.29316731243068,-234.90005));
#212828=CARTESIAN_POINT('Origin',(5.14120077283694,-4.29316731243068,-235.35005));
#212829=CARTESIAN_POINT('Origin',(5.14120077283693,-18.713796339242,-234.90005));
#212830=CARTESIAN_POINT('',(5.40560135635378,-17.5432869067998,-235.35005));
#212831=CARTESIAN_POINT('',(4.7057783396023,-18.1031349726598,-234.90005));
#212832=CARTESIAN_POINT('Ctrl Pts',(5.40560135635379,-17.5432869067999,
-235.35005));
#212833=CARTESIAN_POINT('Ctrl Pts',(5.35103724699192,-17.5921215661342,
-235.35005));
#212834=CARTESIAN_POINT('Ctrl Pts',(5.29598922334368,-17.6400355572588,
-235.33821291833));
#212835=CARTESIAN_POINT('Ctrl Pts',(5.14773261813006,-17.7657397689833,
-235.282379503985));
#212836=CARTESIAN_POINT('Ctrl Pts',(5.06017799547341,-17.8362242902201,
-235.222495970419));
#212837=CARTESIAN_POINT('Ctrl Pts',(4.88938149380987,-17.9694086436079,
-235.083822800233));
#212838=CARTESIAN_POINT('Ctrl Pts',(4.79702736710125,-18.0380214015964,
-234.990808258517));
#212839=CARTESIAN_POINT('Ctrl Pts',(4.70739417651803,-18.101982601881,-234.901656863374));
#212840=CARTESIAN_POINT('Ctrl Pts',(4.70658630927984,-18.1025588626547,
-234.900853430019));
#212841=CARTESIAN_POINT('Ctrl Pts',(4.7057783396023,-18.1031349726598,-234.90005));
#212842=CARTESIAN_POINT('',(6.01013723430735,-17.8861796248583,-235.35005));
#212843=CARTESIAN_POINT('Origin',(5.14120077283693,-18.713796339242,-235.35005));
#212844=CARTESIAN_POINT('',(5.68428606125594,-18.1965358927522,-234.90005));
#212845=CARTESIAN_POINT('Origin',(6.01013723430735,-17.8861796248583,-234.90005));
#212846=CARTESIAN_POINT('Origin',(5.14120077283693,-18.713796339242,-234.90005));
#212847=CARTESIAN_POINT('Origin',(-5.78112710511895,-5.50622241363502,-234.90005));
#212848=CARTESIAN_POINT('',(7.0535866980081,-18.9817245419115,-235.35005));
#212849=CARTESIAN_POINT('',(6.72773552495669,-19.2920808098054,-234.90005));
#212850=CARTESIAN_POINT('Origin',(7.0535866980081,-18.9817245419115,-234.90005));
#212851=CARTESIAN_POINT('',(6.7277355249567,-19.2920808098054,-234.90005));
#212852=CARTESIAN_POINT('',(6.01013723430735,-17.8861796248583,-235.35005));
#212853=CARTESIAN_POINT('Origin',(6.18465023653768,-19.8093412562951,-234.90005));
#212854=CARTESIAN_POINT('',(6.90132755171765,-20.7718243085649,-235.35005));
#212855=CARTESIAN_POINT('',(6.63257355852516,-20.4108931639637,-234.90005));
#212856=CARTESIAN_POINT('Origin',(6.90132755171765,-20.7718243085649,-234.90005));
#212857=CARTESIAN_POINT('Origin',(6.18465023653768,-19.8093412562951,-234.90005));
#212858=CARTESIAN_POINT('Origin',(6.18465023653768,-19.8093412562951,-235.35005));
#212859=CARTESIAN_POINT('Origin',(0.,-11.5034818258363,-234.90005));
#212860=CARTESIAN_POINT('',(1.39485000925072,-22.9745274540666,-235.35005));
#212861=CARTESIAN_POINT('',(1.3405312557817,-22.5278178470269,-234.90005));
#212862=CARTESIAN_POINT('Origin',(1.39485000925072,-22.9745274540666,-234.90005));
#212863=CARTESIAN_POINT('Origin',(0.,-11.5034818258363,-234.90005));
#212864=CARTESIAN_POINT('Origin',(0.,-11.5034818258363,-235.35005));
#212865=CARTESIAN_POINT('Origin',(1.25,-21.7833018352941,-234.90005));
#212866=CARTESIAN_POINT('',(0.0499999999999969,-21.7833018352941,-235.35005));
#212867=CARTESIAN_POINT('',(0.5,-21.7833018352941,-234.90005));
#212868=CARTESIAN_POINT('Origin',(0.0499999999999947,-21.7833018352941,
-234.90005));
#212869=CARTESIAN_POINT('Origin',(1.25,-21.7833018352941,-234.90005));
#212870=CARTESIAN_POINT('Origin',(1.25,-21.7833018352941,-235.35005));
#212871=CARTESIAN_POINT('Origin',(0.0499999999999945,-25.4138432731711,
-234.90005));
#212872=CARTESIAN_POINT('',(0.0499999999999948,-20.2703558849778,-235.35005));
#212873=CARTESIAN_POINT('',(0.5,-20.2703558849778,-234.90005));
#212874=CARTESIAN_POINT('Origin',(0.049999999999997,-20.2703558849778,-234.90005));
#212875=CARTESIAN_POINT('',(0.5,-20.2703558849778,-234.90005));
#212876=CARTESIAN_POINT('',(0.0499999999999947,-21.7833018352941,-235.35005));
#212877=CARTESIAN_POINT('Origin',(1.25,-20.2703558849778,-234.90005));
#212878=CARTESIAN_POINT('',(1.14413406213993,-19.5278652094801,-234.90005));
#212879=CARTESIAN_POINT('',(0.251266268262739,-19.6051258998672,-235.35005));
#212880=CARTESIAN_POINT('Ctrl Pts',(1.14413406213993,-19.5278652094801,
-234.90005));
#212881=CARTESIAN_POINT('Ctrl Pts',(1.14315166831933,-19.5280052813309,
-234.900853430021));
#212882=CARTESIAN_POINT('Ctrl Pts',(1.14216924470093,-19.5281451733567,
-234.901656863372));
#212883=CARTESIAN_POINT('Ctrl Pts',(1.03315182300962,-19.543648263077,-234.990808258614));
#212884=CARTESIAN_POINT('Ctrl Pts',(0.918956045300628,-19.5576596728666,
-235.083822800233));
#212885=CARTESIAN_POINT('Ctrl Pts',(0.703425291345192,-19.5790140885159,
-235.222495970419));
#212886=CARTESIAN_POINT('Ctrl Pts',(0.591413981447227,-19.5883600040661,
-235.282379503985));
#212887=CARTESIAN_POINT('Ctrl Pts',(0.397363584267675,-19.5995855637034,
-235.33821291833));
#212888=CARTESIAN_POINT('Ctrl Pts',(0.324457205278181,-19.602855939172,
-235.35005));
#212889=CARTESIAN_POINT('Ctrl Pts',(0.25126626826274,-19.6051258998672,
-235.35005));
#212890=CARTESIAN_POINT('Origin',(1.25,-20.2703558849778,-234.90005));
#212891=CARTESIAN_POINT('Origin',(1.25,-20.2703558849778,-235.35005));
#212892=CARTESIAN_POINT('Origin',(0.,-178.58000002,-203.84995));
#212893=CARTESIAN_POINT('',(43.6624048158998,50.3711948984507,-205.34995));
#212894=CARTESIAN_POINT('Origin',(0.,-178.58000002,-205.34995));
#212895=CARTESIAN_POINT('',(43.9433571680673,51.844416014308,-203.876128609656));
#212896=CARTESIAN_POINT('Origin',(0.,-178.58000002,-203.876128609656));
#212897=CARTESIAN_POINT('Origin',(43.6624048158998,50.3711948984507,-203.84995));
#212898=CARTESIAN_POINT('Origin',(41.3132181298675,38.0528376956935,-203.84995));
#212899=CARTESIAN_POINT('',(50.148669624411,48.964302343774,-203.876128609656));
#212900=CARTESIAN_POINT('',(49.2048636720257,47.7987359558583,-205.34995));
#212901=CARTESIAN_POINT('Origin',(49.2048636720257,47.7987359558583,-203.84995));
#212902=CARTESIAN_POINT('Origin',(41.3132181298675,38.0528376956935,-205.34995));
#212903=CARTESIAN_POINT('Origin',(41.3132181298675,38.0528376956935,-203.876128609656));
#212904=CARTESIAN_POINT('Origin',(0.,-12.9675000200281,-203.84995));
#212905=CARTESIAN_POINT('',(61.5592179767879,37.6378345921813,-203.876128609656));
#212906=CARTESIAN_POINT('',(60.4006636863987,36.6854341319664,-205.34995));
#212907=CARTESIAN_POINT('Origin',(60.4006636863987,36.6854341319665,-203.84995));
#212908=CARTESIAN_POINT('Origin',(0.,-12.9675000200281,-205.34995));
#212909=CARTESIAN_POINT('Origin',(0.,-12.9675000200281,-203.876128609656));
#212910=CARTESIAN_POINT('Origin',(50.7133971693864,28.7219255026674,-203.84995));
#212911=CARTESIAN_POINT('',(64.7425725698088,29.2764536470619,-203.876128609656));
#212912=CARTESIAN_POINT('',(63.2439712523603,29.2172187609027,-205.34995));
#212913=CARTESIAN_POINT('Origin',(63.2439712523603,29.2172187609027,-203.84995));
#212914=CARTESIAN_POINT('Origin',(50.7133971693864,28.7219255026674,-205.34995));
#212915=CARTESIAN_POINT('Origin',(50.7133971693864,28.7219255026673,-203.876128609656));
#212916=CARTESIAN_POINT('Origin',(-1004.,-12.967500020028,-203.84995));
#212917=CARTESIAN_POINT('',(64.7425725698087,-55.2114536871185,-203.876128609656));
#212918=CARTESIAN_POINT('',(63.2439712523603,-55.1522188009592,-205.34995));
#212919=CARTESIAN_POINT('Origin',(63.2439712523603,-55.1522188009592,-203.84995));
#212920=CARTESIAN_POINT('Origin',(-1004.,-12.967500020028,-205.34995));
#212921=CARTESIAN_POINT('Origin',(-1004.,-12.967500020028,-203.87612860965));
#212922=CARTESIAN_POINT('Origin',(50.7133971693864,-54.6569255427236,-203.84995));
#212923=CARTESIAN_POINT('',(61.5592179767879,-63.5728346322375,-203.876128609656));
#212924=CARTESIAN_POINT('',(60.4006636863987,-62.6204341720228,-205.34995));
#212925=CARTESIAN_POINT('Origin',(60.4006636863987,-62.6204341720228,-203.84995));
#212926=CARTESIAN_POINT('Origin',(50.7133971693864,-54.6569255427236,-205.34995));
#212927=CARTESIAN_POINT('Origin',(50.7133971693864,-54.6569255427236,-203.876128609656));
#212928=CARTESIAN_POINT('Origin',(0.,-12.9675000200281,-203.84995));
#212929=CARTESIAN_POINT('',(50.4303082679829,-74.6701840550325,-203.876128609656));
#212930=CARTESIAN_POINT('',(49.481201831453,-73.5089297105696,-205.34995));
#212931=CARTESIAN_POINT('Origin',(49.481201831453,-73.5089297105696,-203.84995));
#212932=CARTESIAN_POINT('Origin',(0.,-12.9675000200281,-205.34995));
#212933=CARTESIAN_POINT('Origin',(0.,-12.9675000200281,-203.876128609656));
#212934=CARTESIAN_POINT('Origin',(41.5452362233251,-63.7990866568863,-203.84995));
#212935=CARTESIAN_POINT('',(42.0978464467214,-77.8283377352489,-203.876128609656));
#212936=CARTESIAN_POINT('',(42.0388164335396,-76.329728333857,-205.34995));
#212937=CARTESIAN_POINT('Origin',(42.0388164335396,-76.329728333857,-203.84995));
#212938=CARTESIAN_POINT('Origin',(41.5452362233251,-63.7990866568863,-205.34995));
#212939=CARTESIAN_POINT('Origin',(41.5452362233251,-63.7990866568863,-203.876128609656));
#212940=CARTESIAN_POINT('Origin',(0.,990.91999998,-203.84995));
#212941=CARTESIAN_POINT('Origin',(0.,990.91999998,-205.34995));
#212942=CARTESIAN_POINT('Origin',(0.,990.91999998,-203.876128609658));
#212943=CARTESIAN_POINT('Ctrl Pts',(23.5337713018193,37.7635770079652,-235.35005));
#212944=CARTESIAN_POINT('Ctrl Pts',(23.4412215482423,38.6445258986454,-235.35005));
#212945=CARTESIAN_POINT('Ctrl Pts',(23.3965311730095,39.0699180251918,-234.574369193282));
#212946=CARTESIAN_POINT('Ctrl Pts',(21.544967758244,37.5546394871334,-235.35005));
#212947=CARTESIAN_POINT('Ctrl Pts',(21.5595156328412,38.4042872399864,-235.350049999891));
#212948=CARTESIAN_POINT('Ctrl Pts',(21.528579903829,38.8428303292096,-234.630002261341));
#212949=CARTESIAN_POINT('Ctrl Pts',(19.5728087816907,37.6143598891719,-235.35005));
#212950=CARTESIAN_POINT('Ctrl Pts',(19.6460924738843,38.4272076002415,-235.350050000083));
#212951=CARTESIAN_POINT('Ctrl Pts',(19.6686531904506,38.8735235122781,-234.667980547948));
#212952=CARTESIAN_POINT('Ctrl Pts',(17.1293181155885,38.0221098575109,-235.35005));
#212953=CARTESIAN_POINT('Ctrl Pts',(17.2775595203712,38.7968938489773,-235.350049999979));
#212954=CARTESIAN_POINT('Ctrl Pts',(17.3605038451651,39.2363169917258,-234.700408624977));
#212955=CARTESIAN_POINT('Ctrl Pts',(16.6417036619234,38.1205664043706,-235.35005));
#212956=CARTESIAN_POINT('Ctrl Pts',(16.8064715779446,38.8874549017434,-235.350049999965));
#212957=CARTESIAN_POINT('Ctrl Pts',(16.8996732382546,39.3253279225055,-234.706109493926));
#212958=CARTESIAN_POINT('Ctrl Pts',(16.1400046127821,38.2400981929685,-235.35005));
#212959=CARTESIAN_POINT('Ctrl Pts',(16.321379078743,38.9989389430008,-235.350050000001));
#212960=CARTESIAN_POINT('Ctrl Pts',(16.42550941929,39.4346066602602,-234.71123368766));
#212961=CARTESIAN_POINT('Ctrl Pts',(16.1248016477258,38.2437210061727,-235.35005));
#212962=CARTESIAN_POINT('Ctrl Pts',(16.3049839983191,39.0030520275993,-235.350049999999));
#212963=CARTESIAN_POINT('Ctrl Pts',(16.4084002183571,39.4388699450819,-234.710975012385));
#212964=CARTESIAN_POINT('Ctrl Pts',(16.0943932017804,38.2509106189313,-235.35005));
#212965=CARTESIAN_POINT('Ctrl Pts',(16.2733843150407,39.0107061360713,-235.350050000001));
#212966=CARTESIAN_POINT('Ctrl Pts',(16.3760894567153,39.446674478502,-234.710745663099));
#212967=CARTESIAN_POINT('Ctrl Pts',(16.0791881134232,38.2544860973495,-235.35005));
#212968=CARTESIAN_POINT('Ctrl Pts',(16.2575832784277,39.014513360759,-235.350050000001));
#212969=CARTESIAN_POINT('Ctrl Pts',(16.3599327990296,39.4505564386636,-234.710630718465));
#212970=CARTESIAN_POINT('Ctrl Pts',(16.0335702546769,38.2651546047763,-235.35005));
#212971=CARTESIAN_POINT('Ctrl Pts',(16.2101754559538,39.0258758721752,-235.350049999999));
#212972=CARTESIAN_POINT('Ctrl Pts',(16.3114590264843,39.4621414418891,-234.710285080473));
#212973=CARTESIAN_POINT('Ctrl Pts',(16.0031548906349,38.2721897058173,-235.35005));
#212974=CARTESIAN_POINT('Ctrl Pts',(16.1785662488632,39.0333714350269,-235.350049999998));
#212975=CARTESIAN_POINT('Ctrl Pts',(16.2791381120791,39.4697836074978,-234.710053583084));
#212976=CARTESIAN_POINT('Ctrl Pts',(15.9118984440295,38.2930637479782,-235.35005));
#212977=CARTESIAN_POINT('Ctrl Pts',(16.0837198987913,39.0556218358223,-235.350050000004));
#212978=CARTESIAN_POINT('Ctrl Pts',(16.1821604215077,39.492466940349,-234.709355920323));
#212979=CARTESIAN_POINT('Ctrl Pts',(15.8510470069393,38.306671426842,-235.35005));
#212980=CARTESIAN_POINT('Ctrl Pts',(16.0204731962087,39.0701381365939,-235.35005));
#212981=CARTESIAN_POINT('Ctrl Pts',(16.1174886972092,39.5072649406307,-234.70888658509));
#212982=CARTESIAN_POINT('Ctrl Pts',(15.6684514409702,38.3465730643765,-235.35005));
#212983=CARTESIAN_POINT('Ctrl Pts',(15.8306591723873,39.1127448736401,-235.350049999999));
#212984=CARTESIAN_POINT('Ctrl Pts',(15.9234157668579,39.5506891483394,-234.707466239024));
#212985=CARTESIAN_POINT('Ctrl Pts',(15.5466660565693,38.3719456052131,-235.35005));
#212986=CARTESIAN_POINT('Ctrl Pts',(15.7040546546833,39.1398840785044,-235.350049999993));
#212987=CARTESIAN_POINT('Ctrl Pts',(15.7939567942534,39.5783455145344,-234.706502899802));
#212988=CARTESIAN_POINT('Ctrl Pts',(15.1811462193431,38.4444074431018,-235.35005));
#212989=CARTESIAN_POINT('Ctrl Pts',(15.3239537913802,39.2175582578027,-235.350050000014));
#212990=CARTESIAN_POINT('Ctrl Pts',(15.4053654748198,39.6574599908674,-234.703565858339));
#212991=CARTESIAN_POINT('Ctrl Pts',(14.9372480700734,38.4878406765044,-235.35005));
#212992=CARTESIAN_POINT('Ctrl Pts',(15.0703175067835,39.264312526642,-235.350050000014));
#212993=CARTESIAN_POINT('Ctrl Pts',(15.1460186735935,39.7050627091706,-234.701545340841));
#212994=CARTESIAN_POINT('Ctrl Pts',(13.7166846422703,38.6810491434111,-235.35005));
#212995=CARTESIAN_POINT('Ctrl Pts',(13.7992132146591,39.4736856374966,-235.350049999945));
#212996=CARTESIAN_POINT('Ctrl Pts',(13.8480833935374,39.9177504037689,-234.691149086225));
#212997=CARTESIAN_POINT('Ctrl Pts',(12.7368211879873,38.7593950182532,-235.35005));
#212998=CARTESIAN_POINT('Ctrl Pts',(12.7786543368479,39.5623177727158,-235.350049999973));
#212999=CARTESIAN_POINT('Ctrl Pts',(12.8051741258232,40.0075424243875,-234.681773511397));
#213000=CARTESIAN_POINT('Ctrl Pts',(11.2619727856902,38.7640531506662,-235.35005));
#213001=CARTESIAN_POINT('Ctrl Pts',(11.2431521551635,39.57939042452,-235.350050000013));
#213002=CARTESIAN_POINT('Ctrl Pts',(11.2337432072715,40.0228717807706,-234.665927297908));
#213003=CARTESIAN_POINT('Ctrl Pts',(10.7695125981793,38.7467544284527,-235.35005));
#213004=CARTESIAN_POINT('Ctrl Pts',(10.7295261233112,39.565608825609,-235.350049999918));
#213005=CARTESIAN_POINT('Ctrl Pts',(10.7088554256347,40.0080380899104,-234.660361333187));
#213006=CARTESIAN_POINT('Ctrl Pts',(10.0295286262227,38.6919125335409,-235.35005));
#213007=CARTESIAN_POINT('Ctrl Pts',(9.95766155311817,39.5152528143172,-235.350050000041));
#213008=CARTESIAN_POINT('Ctrl Pts',(9.91949508966786,39.9551826764288,-234.651499451358));
#213009=CARTESIAN_POINT('Ctrl Pts',(9.78265126231073,38.6688067779309,-235.35005));
#213010=CARTESIAN_POINT('Ctrl Pts',(9.69988287916204,39.4934693700283,-235.350049999959));
#213011=CARTESIAN_POINT('Ctrl Pts',(9.65607177918342,39.9324493818079,-234.648467075417));
#213012=CARTESIAN_POINT('Ctrl Pts',(9.52011153127327,38.6390634523758,-235.35005));
#213013=CARTESIAN_POINT('Ctrl Pts',(9.42586446285605,39.4649843060134,-235.350050000003));
#213014=CARTESIAN_POINT('Ctrl Pts',(9.37590715791402,39.9027865695414,-234.645166403075));
#213015=CARTESIAN_POINT('Ctrl Pts',(9.5046684949403,38.6373245042148,-235.35005));
#213016=CARTESIAN_POINT('Ctrl Pts',(9.41214667413609,39.4630372950313,-235.350049999998));
#213017=CARTESIAN_POINT('Ctrl Pts',(9.36306987593997,39.901015111022,-234.645686067046));
#213018=CARTESIAN_POINT('Ctrl Pts',(9.473784192795,38.6338861513583,-235.35005));
#213019=CARTESIAN_POINT('Ctrl Pts',(9.38247113793461,39.4594435790343,-235.350050000003));
#213020=CARTESIAN_POINT('Ctrl Pts',(9.33401274020438,39.8975447405836,-234.646059912476));
#213021=CARTESIAN_POINT('Ctrl Pts',(9.45834279379069,38.6321837719653,-235.35005));
#213022=CARTESIAN_POINT('Ctrl Pts',(9.36763359512751,39.4576634928911,-235.350049999998));
#213023=CARTESIAN_POINT('Ctrl Pts',(9.31948440605278,39.8958258095482,-234.646245966055));
#213024=CARTESIAN_POINT('Ctrl Pts',(9.41202084990189,38.6271269560786,-235.35005));
#213025=CARTESIAN_POINT('Ctrl Pts',(9.32312351171904,39.4523737016179,-235.350050000003));
#213026=CARTESIAN_POINT('Ctrl Pts',(9.27590015565431,39.8907177155567,-234.646801541337));
#213027=CARTESIAN_POINT('Ctrl Pts',(9.38114255812013,38.623822841143,-235.35005));
#213028=CARTESIAN_POINT('Ctrl Pts',(9.29344985904992,39.4489140122088,-235.35005));
#213029=CARTESIAN_POINT('Ctrl Pts',(9.24684499153364,39.8873772510059,-234.647168477753));
#213030=CARTESIAN_POINT('Ctrl Pts',(9.28851667185603,38.6141112621716,-235.35005));
#213031=CARTESIAN_POINT('Ctrl Pts',(9.20443932951169,39.4387362251899,-235.350049999998));
#213032=CARTESIAN_POINT('Ctrl Pts',(9.15968291091601,39.8775501712904,-234.648259112741));
#213033=CARTESIAN_POINT('Ctrl Pts',(9.22677806590085,38.6079045516347,-235.35005));
#213034=CARTESIAN_POINT('Ctrl Pts',(9.14509826755899,39.4322176005077,-235.350050000002));
#213035=CARTESIAN_POINT('Ctrl Pts',(9.10157940753183,39.8712578585209,-234.648972640385));
#213036=CARTESIAN_POINT('Ctrl Pts',(9.04159803643428,38.590083732581,-235.35005));
#213037=CARTESIAN_POINT('Ctrl Pts',(8.96711873611221,39.413462618403,-235.350049999995));
#213038=CARTESIAN_POINT('Ctrl Pts',(8.92728571898841,39.8531547209574,-234.65107374629));
#213039=CARTESIAN_POINT('Ctrl Pts',(8.9181923928208,38.5792687467551,-235.35005));
#213040=CARTESIAN_POINT('Ctrl Pts',(8.8484656438594,39.4020198774485,-235.350049999991));
#213041=CARTESIAN_POINT('Ctrl Pts',(8.8111123738377,39.8421175196046,-234.652421897231));
#213042=CARTESIAN_POINT('Ctrl Pts',(7.80796793746822,38.4914558622135,-235.35005));
#213043=CARTESIAN_POINT('Ctrl Pts',(7.78295663156236,39.308723576629,-235.350050000068));
#213044=CARTESIAN_POINT('Ctrl Pts',(7.76582808828186,39.7520042646446,-234.664105356254));
#213045=CARTESIAN_POINT('Ctrl Pts',(6.82559161716421,38.4810313542882,-235.35005));
#213046=CARTESIAN_POINT('Ctrl Pts',(6.83602241994642,39.2928501093446,-235.350049999919));
#213047=CARTESIAN_POINT('Ctrl Pts',(6.84026733134357,39.7374178092291,-234.671316797028));
#213048=CARTESIAN_POINT('Ctrl Pts',(5.35870346950635,38.5640529810103,-235.35005));
#213049=CARTESIAN_POINT('Ctrl Pts',(5.42261292444301,39.3678039902082,-235.350050000041));
#213050=CARTESIAN_POINT('Ctrl Pts',(5.45751451406658,39.8113778773929,-234.67782855951));
#213051=CARTESIAN_POINT('Ctrl Pts',(4.87084782996001,38.6081920655742,-235.35005));
#213052=CARTESIAN_POINT('Ctrl Pts',(4.95261115944054,39.4091800619321,-235.350049999987));
#213053=CARTESIAN_POINT('Ctrl Pts',(4.99768588356049,39.8520037968002,-234.679290572784));
#213054=CARTESIAN_POINT('Ctrl Pts',(4.14073989483365,38.6993202534944,-235.35005));
#213055=CARTESIAN_POINT('Ctrl Pts',(4.24935061898658,39.496080258275,-235.350050000007));
#213056=CARTESIAN_POINT('Ctrl Pts',(4.30944352059924,39.9371527903924,-234.680416520121));
#213057=CARTESIAN_POINT('Ctrl Pts',(3.8976491789597,38.7338397862931,-235.35005));
#213058=CARTESIAN_POINT('Ctrl Pts',(4.01519167481988,39.5291751697216,-235.350050000021));
#213059=CARTESIAN_POINT('Ctrl Pts',(4.08027426577388,39.9695612765499,-234.680616205795));
#213060=CARTESIAN_POINT('Ctrl Pts',(3.59413684714098,38.7822104560078,-235.35005));
#213061=CARTESIAN_POINT('Ctrl Pts',(3.72290333740421,39.5757342399723,-235.350049999995));
#213062=CARTESIAN_POINT('Ctrl Pts',(3.79420511631547,40.0151323858563,-234.680645380834));
#213063=CARTESIAN_POINT('Ctrl Pts',(3.53345194963507,38.7921458861338,-235.35005));
#213064=CARTESIAN_POINT('Ctrl Pts',(3.664465108349,39.5853059524361,-235.350049999998));
#213065=CARTESIAN_POINT('Ctrl Pts',(3.73701094502127,40.0244998494229,-234.68064014219));
#213066=CARTESIAN_POINT('Ctrl Pts',(3.41211742684046,38.8125413395452,-235.35005));
#213067=CARTESIAN_POINT('Ctrl Pts',(3.54762995410732,39.6049708499852,-235.350050000001));
#213068=CARTESIAN_POINT('Ctrl Pts',(3.62266424283369,40.0437428586239,-234.680607281213));
#213069=CARTESIAN_POINT('Ctrl Pts',(3.35147728959859,38.8231424752753,-235.35005));
#213070=CARTESIAN_POINT('Ctrl Pts',(3.49161331287685,39.6148541672734,-235.350050000006));
#213071=CARTESIAN_POINT('Ctrl Pts',(3.56919466402218,40.053171477784,-234.680497918826));
#213072=CARTESIAN_POINT('Ctrl Pts',(3.16954343825523,38.8547460002398,-235.35005));
#213073=CARTESIAN_POINT('Ctrl Pts',(3.30204310810083,39.6474891097825,-235.350049999988));
#213074=CARTESIAN_POINT('Ctrl Pts',(3.37542267175575,40.086577519758,-234.680874073307));
#213075=CARTESIAN_POINT('Ctrl Pts',(3.0481745839355,38.874630850895,-235.35005));
#213076=CARTESIAN_POINT('Ctrl Pts',(3.17556784923895,39.6680247489009,-235.350050000003));
#213077=CARTESIAN_POINT('Ctrl Pts',(3.24614026037888,40.107598873827,-234.681111548481));
#213078=CARTESIAN_POINT('Ctrl Pts',(1.95514022520376,39.0429654437216,-235.35005));
#213079=CARTESIAN_POINT('Ctrl Pts',(2.03697150224516,39.8418002800282,-235.350049999973));
#213080=CARTESIAN_POINT('Ctrl Pts',(2.08186324421676,40.2855474949375,-234.683127215883));
#213081=CARTESIAN_POINT('Ctrl Pts',(0.976538623334591,39.1173940813018,
-235.35005));
#213082=CARTESIAN_POINT('Ctrl Pts',(1.01727193036948,39.9186763854274,-235.350050000014));
#213083=CARTESIAN_POINT('Ctrl Pts',(1.03992075359521,40.3641796537732,-234.684031855599));
#213084=CARTESIAN_POINT('Ctrl Pts',(-1.46378262333123E-9,39.1173940795976,
-235.35005));
#213085=CARTESIAN_POINT('Ctrl Pts',(-2.52664204734146E-9,39.9186763848311,
-235.350050000001));
#213086=CARTESIAN_POINT('Ctrl Pts',(-3.11757902950382E-9,40.3641796532955,
-234.68403185425));
#213087=CARTESIAN_POINT('',(16.4332020134251,39.4328341554683,-234.711149933649));
#213088=CARTESIAN_POINT('',(9.39019403218236,39.9042967860601,-234.645338670229));
#213089=CARTESIAN_POINT('Ctrl Pts',(16.4332020134251,39.4328341554683,-234.711149933649));
#213090=CARTESIAN_POINT('Ctrl Pts',(16.4203687735928,39.4358646816662,-234.711186834089));
#213091=CARTESIAN_POINT('Ctrl Pts',(16.4059605185975,39.4394389786432,-234.71098583394));
#213092=CARTESIAN_POINT('Ctrl Pts',(16.3922402656679,39.4427528750883,-234.710888692203));
#213093=CARTESIAN_POINT('Ctrl Pts',(16.3760847365541,39.4466549715566,-234.710774308294));
#213094=CARTESIAN_POINT('Ctrl Pts',(16.3599280157032,39.4505367406652,-234.710659655018));
#213095=CARTESIAN_POINT('Ctrl Pts',(16.3437702132482,39.4543981737023,-234.710544734921));
#213096=CARTESIAN_POINT('Ctrl Pts',(16.3114533027793,39.4621213517823,-234.71031488544));
#213097=CARTESIAN_POINT('Ctrl Pts',(16.2791320654287,39.46976317781,-234.710083968637));
#213098=CARTESIAN_POINT('Ctrl Pts',(16.2468073837233,39.4773235962622,-234.709852004547));
#213099=CARTESIAN_POINT('Ctrl Pts',(16.1821472083185,39.4924469619834,-234.709387998781));
#213100=CARTESIAN_POINT('Ctrl Pts',(16.1174732492397,39.5072445696182,-234.708919803019));
#213101=CARTESIAN_POINT('Ctrl Pts',(16.0527925905293,39.5217162013998,-234.708447571674));
#213102=CARTESIAN_POINT('Ctrl Pts',(15.9233431638038,39.5506791785132,-234.707502465699));
#213103=CARTESIAN_POINT('Ctrl Pts',(15.7938668812152,39.578336176396,-234.706541204651));
#213104=CARTESIAN_POINT('Ctrl Pts',(15.664420813873,39.6046890583072,-234.70556492186));
#213105=CARTESIAN_POINT('Ctrl Pts',(15.4048133770445,39.65754044473,-234.703606961467));
#213106=CARTESIAN_POINT('Ctrl Pts',(15.1453273024862,39.705141822975,-234.701588751043));
#213107=CARTESIAN_POINT('Ctrl Pts',(14.8864260905022,39.7475653316504,-234.699517541149));
#213108=CARTESIAN_POINT('Ctrl Pts',(14.6384733849316,39.7881948199223,-234.697533919315));
#213109=CARTESIAN_POINT('Ctrl Pts',(14.391016124878,39.8241145499751,-234.695494894259));
#213110=CARTESIAN_POINT('Ctrl Pts',(14.1444226316741,39.8553859752978,-234.693402565929));
#213111=CARTESIAN_POINT('Ctrl Pts',(13.8954781303716,39.8869555405806,-234.691290289463));
#213112=CARTESIAN_POINT('Ctrl Pts',(13.6474139403796,39.9137877658293,-234.689123685087));
#213113=CARTESIAN_POINT('Ctrl Pts',(13.4006121728291,39.9359991936509,-234.686905722618));
#213114=CARTESIAN_POINT('Ctrl Pts',(13.2154735814038,39.9526611183254,-234.685241915865));
#213115=CARTESIAN_POINT('Ctrl Pts',(13.0310454540037,39.9667239118459,-234.683549225146));
#213116=CARTESIAN_POINT('Ctrl Pts',(12.8474902542086,39.9782559564172,-234.681829214244));
#213117=CARTESIAN_POINT('Ctrl Pts',(12.6339027438901,39.9916748118439,-234.679827784446));
#213118=CARTESIAN_POINT('Ctrl Pts',(12.421738466853,40.0015717217697,-234.677921264933));
#213119=CARTESIAN_POINT('Ctrl Pts',(12.2106113431622,40.0081508386869,-234.676039453921));
#213120=CARTESIAN_POINT('Ctrl Pts',(12.0591061036169,40.012872025937,-234.674689062634));
#213121=CARTESIAN_POINT('Ctrl Pts',(11.9081347609518,40.0158836098002,-234.673351340136));
#213122=CARTESIAN_POINT('Ctrl Pts',(11.7575518798804,40.0172447761073,-234.671999478744));
#213123=CARTESIAN_POINT('Ctrl Pts',(11.5451205475199,40.0191650101347,-234.670092371411));
#213124=CARTESIAN_POINT('Ctrl Pts',(11.3334790960771,40.0177944242705,-234.668159423378));
#213125=CARTESIAN_POINT('Ctrl Pts',(11.1221945383988,40.0132178609341,-234.666120035305));
#213126=CARTESIAN_POINT('Ctrl Pts',(10.9127324535587,40.0086807735653,-234.664098238339));
#213127=CARTESIAN_POINT('Ctrl Pts',(10.7036211597665,40.0009927930571,-234.661971856266));
#213128=CARTESIAN_POINT('Ctrl Pts',(10.4944307492036,39.9901862402078,-234.659659267466));
#213129=CARTESIAN_POINT('Ctrl Pts',(10.3905549522781,39.9848201276492,-234.658510926087));
#213130=CARTESIAN_POINT('Ctrl Pts',(10.2866595198607,39.9786842761451,-234.657316620765));
#213131=CARTESIAN_POINT('Ctrl Pts',(10.1826910350602,39.9717779243169,-234.656066034813));
#213132=CARTESIAN_POINT('Ctrl Pts',(9.97674280585096,39.9580973274317,-234.653588784491));
#213133=CARTESIAN_POINT('Ctrl Pts',(9.77052974306509,39.9413880055303,-234.650895256858));
#213134=CARTESIAN_POINT('Ctrl Pts',(9.56366756941837,39.9216004287237,-234.647908051821));
#213135=CARTESIAN_POINT('Ctrl Pts',(9.50662648274058,39.9161441151606,-234.647084346749));
#213136=CARTESIAN_POINT('Ctrl Pts',(9.44953599881491,39.9104534465954,-234.646238289762));
#213137=CARTESIAN_POINT('Ctrl Pts',(9.39238796798789,39.9045266899386,-234.645368206131));
#213138=CARTESIAN_POINT('Ctrl Pts',(9.39164951275459,39.9044501055943,-234.645356963087));
#213139=CARTESIAN_POINT('Ctrl Pts',(9.39091836077164,39.9043734691061,-234.645347149113));
#213140=CARTESIAN_POINT('Ctrl Pts',(9.39019403294204,39.9042967861422,-234.645338670235));
#213141=CARTESIAN_POINT('',(23.3965312474468,39.0699178884317,-234.574369311842));
#213142=CARTESIAN_POINT('Ctrl Pts',(23.3965311730095,39.0699180251917,-234.574369193282));
#213143=CARTESIAN_POINT('Ctrl Pts',(23.0945668978142,39.0332080891435,-234.583362575255));
#213144=CARTESIAN_POINT('Ctrl Pts',(22.7892825654022,39.0028096619222,-234.591999161059));
#213145=CARTESIAN_POINT('Ctrl Pts',(22.4810560648072,38.9792191234299,-234.600263558775));
#213146=CARTESIAN_POINT('Ctrl Pts',(22.1762733075222,38.955892156561,-234.608435620289));
#213147=CARTESIAN_POINT('Ctrl Pts',(21.8686137925994,38.9392219216893,-234.616243787899));
#213148=CARTESIAN_POINT('Ctrl Pts',(21.5584440197407,38.9296383570326,-234.623679503494));
#213149=CARTESIAN_POINT('Ctrl Pts',(21.2528094397991,38.9201949198749,-234.631006496681));
#213150=CARTESIAN_POINT('Ctrl Pts',(20.9447375071085,38.9176324870007,-234.637971880429));
#213151=CARTESIAN_POINT('Ctrl Pts',(20.6345794911481,38.9223123543167,-234.644573233207));
#213152=CARTESIAN_POINT('Ctrl Pts',(20.4201142239214,38.9255483467557,-234.649137877081));
#213153=CARTESIAN_POINT('Ctrl Pts',(20.2046515464032,38.9322460806201,-234.653528585768));
#213154=CARTESIAN_POINT('Ctrl Pts',(19.9883076390171,38.942510467933,-234.65774609101));
#213155=CARTESIAN_POINT('Ctrl Pts',(19.7072288045135,38.9558461890895,-234.66322556798));
#213156=CARTESIAN_POINT('Ctrl Pts',(19.4246735316766,38.9752044123415,-234.668412293426));
#213157=CARTESIAN_POINT('Ctrl Pts',(19.1409896021326,39.0007703112355,-234.67330953877));
#213158=CARTESIAN_POINT('Ctrl Pts',(18.8605201760056,39.0260465156463,-234.678151292031));
#213159=CARTESIAN_POINT('Ctrl Pts',(18.5789475541907,39.0573905103833,-234.682710118246));
#213160=CARTESIAN_POINT('Ctrl Pts',(18.2966065606005,39.0949307879218,-234.686992959889));
#213161=CARTESIAN_POINT('Ctrl Pts',(18.13867089569,39.1159300364496,-234.689388692205));
#213162=CARTESIAN_POINT('Ctrl Pts',(17.9804935567509,39.1388673942171,-234.691698151296));
#213163=CARTESIAN_POINT('Ctrl Pts',(17.8221337142222,39.1637582958363,-234.693923009571));
#213164=CARTESIAN_POINT('Ctrl Pts',(17.6071594454973,39.1975478177759,-234.696943265674));
#213165=CARTESIAN_POINT('Ctrl Pts',(17.3918441418382,39.234987417972,-234.699800486487));
#213166=CARTESIAN_POINT('Ctrl Pts',(17.1763463091445,39.276150383324,-234.702496183025));
#213167=CARTESIAN_POINT('Ctrl Pts',(16.9311343525973,39.3229891433482,-234.705563578247));
#213168=CARTESIAN_POINT('Ctrl Pts',(16.685681217613,39.3746501130852,-234.708421884368));
#213169=CARTESIAN_POINT('Ctrl Pts',(16.4401979186951,39.4312214602623,-234.711074951862));
#213170=CARTESIAN_POINT('Ctrl Pts',(16.4400911575267,39.4312460632522,-234.711076105687));
#213171=CARTESIAN_POINT('Ctrl Pts',(16.4399845215119,39.4312706239838,-234.711077278024));
#213172=CARTESIAN_POINT('Ctrl Pts',(16.4398780101602,39.4312951426272,-234.711078468791));
#213173=CARTESIAN_POINT('Ctrl Pts',(16.4376580748706,39.4318061661087,-234.711103287052));
#213174=CARTESIAN_POINT('Ctrl Pts',(16.4354272908939,39.4323210756196,-234.711126313563));
#213175=CARTESIAN_POINT('Ctrl Pts',(16.4332020134251,39.4328341554683,-234.711149933648));
#213176=CARTESIAN_POINT('',(23.5337713018193,37.7635770079652,-235.35005));
#213177=CARTESIAN_POINT('Origin',(23.5337713018193,37.7635770079652,-233.85005));
#213178=CARTESIAN_POINT('Ctrl Pts',(1.77635683940026E-15,39.1173940795976,
-235.35005));
#213179=CARTESIAN_POINT('Ctrl Pts',(0.356337369905621,39.1173940801923,
-235.35005));
#213180=CARTESIAN_POINT('Ctrl Pts',(0.71242141794696,39.1074881618969,-235.35005));
#213181=CARTESIAN_POINT('Ctrl Pts',(1.06804673827445,39.0877008656221,-235.35005));
#213182=CARTESIAN_POINT('Ctrl Pts',(1.42342108500666,39.0679275337324,-235.35005));
#213183=CARTESIAN_POINT('Ctrl Pts',(1.7783377368663,39.0382867784318,-235.35005));
#213184=CARTESIAN_POINT('Ctrl Pts',(2.13259518028593,38.9987512744367,-235.35005));
#213185=CARTESIAN_POINT('Ctrl Pts',(2.39770300797321,38.9691649615014,-235.35005));
#213186=CARTESIAN_POINT('Ctrl Pts',(2.66244176764352,38.9340362860626,-235.35005));
#213187=CARTESIAN_POINT('Ctrl Pts',(2.92672632283112,38.8933347008859,-235.35005));
#213188=CARTESIAN_POINT('Ctrl Pts',(2.92737060497439,38.8932354771363,-235.35005));
#213189=CARTESIAN_POINT('Ctrl Pts',(2.92801488526773,38.8931362200903,-235.35005));
#213190=CARTESIAN_POINT('Ctrl Pts',(2.92865916371251,38.8930369297473,-235.35005));
#213191=CARTESIAN_POINT('Ctrl Pts',(3.04946230489496,38.8744198466836,-235.35005));
#213192=CARTESIAN_POINT('Ctrl Pts',(3.17018687790291,38.8546342347918,-235.35005));
#213193=CARTESIAN_POINT('Ctrl Pts',(3.29083267335743,38.8336769886241,-235.35005));
#213194=CARTESIAN_POINT('Ctrl Pts',(3.35147729051483,38.8231424800179,-235.35005));
#213195=CARTESIAN_POINT('Ctrl Pts',(3.41211742776757,38.8125413442761,-235.35005));
#213196=CARTESIAN_POINT('Ctrl Pts',(3.47278468915089,38.8023436182718,-235.35005));
#213197=CARTESIAN_POINT('Ctrl Pts',(3.53345195083837,38.7921458922164,-235.35005));
#213198=CARTESIAN_POINT('Ctrl Pts',(3.5941368485939,38.7822104634589,-235.35005));
#213199=CARTESIAN_POINT('Ctrl Pts',(3.65483931509605,38.77253633205,-235.35005));
#213200=CARTESIAN_POINT('Ctrl Pts',(3.65546036588309,38.7724373553976,-235.35005));
#213201=CARTESIAN_POINT('Ctrl Pts',(3.65608141850748,38.772338406072,-235.35005));
#213202=CARTESIAN_POINT('Ctrl Pts',(3.6567024729692,38.7722394840726,-235.35005));
#213203=CARTESIAN_POINT('Ctrl Pts',(3.89889272031259,38.7336632480438,-235.35005));
#213204=CARTESIAN_POINT('Ctrl Pts',(4.14136237871588,38.6992425872422,-235.35005));
#213205=CARTESIAN_POINT('Ctrl Pts',(4.38410920892073,38.6689442099089,-235.35005));
#213206=CARTESIAN_POINT('Ctrl Pts',(4.38470863575882,38.6688693926167,-235.35005));
#213207=CARTESIAN_POINT('Ctrl Pts',(4.385308064291,38.6687946005203,-235.35005));
#213208=CARTESIAN_POINT('Ctrl Pts',(4.38590749451727,38.6687198336194,-235.35005));
#213209=CARTESIAN_POINT('Ctrl Pts',(4.87204943935151,38.6080833741744,-235.35005));
#213210=CARTESIAN_POINT('Ctrl Pts',(5.35930565181913,38.5640188991232,-235.35005));
#213211=CARTESIAN_POINT('Ctrl Pts',(5.84766618924905,38.5363791735804,-235.35005));
#213212=CARTESIAN_POINT('Ctrl Pts',(5.84822203464059,38.5363477144167,-235.35005));
#213213=CARTESIAN_POINT('Ctrl Pts',(5.84877788147003,38.5363162765022,-235.35005));
#213214=CARTESIAN_POINT('Ctrl Pts',(5.8493337297374,38.5362848598371,-235.35005));
#213215=CARTESIAN_POINT('Ctrl Pts',(6.82670834760912,38.4810434337187,-235.35005));
#213216=CARTESIAN_POINT('Ctrl Pts',(7.80852886296661,38.4915002286307,-235.35005));
#213217=CARTESIAN_POINT('Ctrl Pts',(8.79483411976782,38.569511762568,-235.35005));
#213218=CARTESIAN_POINT('Ctrl Pts',(8.79530155914491,38.5695487345527,-235.35005));
#213219=CARTESIAN_POINT('Ctrl Pts',(8.79576899920217,38.5695857217288,-235.35005));
#213220=CARTESIAN_POINT('Ctrl Pts',(8.79623643993962,38.5696227240969,-235.35005));
#213221=CARTESIAN_POINT('Ctrl Pts',(8.91912763117963,38.5793507275117,-235.35005));
#213222=CARTESIAN_POINT('Ctrl Pts',(9.04206583597103,38.5901287539636,-235.35005));
#213223=CARTESIAN_POINT('Ctrl Pts',(9.16505138923101,38.6019642804975,-235.35005));
#213224=CARTESIAN_POINT('Ctrl Pts',(9.22677806574757,38.6079045531424,-235.35005));
#213225=CARTESIAN_POINT('Ctrl Pts',(9.28851667172624,38.6141112633048,-235.35005));
#213226=CARTESIAN_POINT('Ctrl Pts',(9.35026726260429,38.6205856490536,-235.35005));
#213227=CARTESIAN_POINT('Ctrl Pts',(9.38114255802925,38.6238228419266,-235.35005));
#213228=CARTESIAN_POINT('Ctrl Pts',(9.41202084981748,38.6271269567803,-235.35005));
#213229=CARTESIAN_POINT('Ctrl Pts',(9.44290214575424,38.6304981673432,-235.35005));
#213230=CARTESIAN_POINT('Ctrl Pts',(9.4583427937156,38.6321837726239,-235.35005));
#213231=CARTESIAN_POINT('Ctrl Pts',(9.47378419271945,38.6338861520155,-235.35005));
#213232=CARTESIAN_POINT('Ctrl Pts',(9.4892263437929,38.635605328458,-235.35005));
#213233=CARTESIAN_POINT('Ctrl Pts',(9.50466849486033,38.6373245048999,-235.35005));
#213234=CARTESIAN_POINT('Ctrl Pts',(9.52011153118833,38.6390634530903,-235.35005));
#213235=CARTESIAN_POINT('Ctrl Pts',(9.53555504477742,38.6408130605231,-235.35005));
#213236=CARTESIAN_POINT('Ctrl Pts',(9.53599979556026,38.6408634466785,-235.35005));
#213237=CARTESIAN_POINT('Ctrl Pts',(9.53644454563409,38.6409138169984,-235.35005));
#213238=CARTESIAN_POINT('Ctrl Pts',(9.53688929499893,38.6409641714834,-235.35005));
#213239=CARTESIAN_POINT('Ctrl Pts',(9.78353997539554,38.6688899403824,-235.35005));
#213240=CARTESIAN_POINT('Ctrl Pts',(10.0299725953353,38.6919454677066,-235.35005));
#213241=CARTESIAN_POINT('Ctrl Pts',(10.2761899486978,38.7101931855589,-235.35005));
#213242=CARTESIAN_POINT('Ctrl Pts',(10.2766105499729,38.7102243572586,-235.35005));
#213243=CARTESIAN_POINT('Ctrl Pts',(10.2770311506211,38.710255514956,-235.35005));
#213244=CARTESIAN_POINT('Ctrl Pts',(10.2774517506423,38.7102866586516,-235.35005));
#213245=CARTESIAN_POINT('Ctrl Pts',(10.7703523227059,38.7467839115651,-235.35005));
#213246=CARTESIAN_POINT('Ctrl Pts',(11.2623919364771,38.7640519886161,-235.35005));
#213247=CARTESIAN_POINT('Ctrl Pts',(11.7535889201299,38.762500547725,-235.35005));
#213248=CARTESIAN_POINT('Ctrl Pts',(11.7539614946379,38.7624993709521,-235.35005));
#213249=CARTESIAN_POINT('Ctrl Pts',(11.7543340686623,38.7624981833755,-235.35005));
#213250=CARTESIAN_POINT('Ctrl Pts',(11.7547066422029,38.7624969849952,-235.35005));
#213251=CARTESIAN_POINT('Ctrl Pts',(12.7375637754513,38.759335631593,-235.35005));
#213252=CARTESIAN_POINT('Ctrl Pts',(13.7170546474298,38.6809905736403,-235.35005));
#213253=CARTESIAN_POINT('Ctrl Pts',(14.6931353846985,38.5264823710594,-235.35005));
#213254=CARTESIAN_POINT('Ctrl Pts',(14.6934128882961,38.5264384437689,-235.35005));
#213255=CARTESIAN_POINT('Ctrl Pts',(14.6936903916164,38.5263945102864,-235.35005));
#213256=CARTESIAN_POINT('Ctrl Pts',(14.6939678946594,38.5263505706118,-235.35005));
#213257=CARTESIAN_POINT('Ctrl Pts',(14.9378025763861,38.4877419252588,-235.35005));
#213258=CARTESIAN_POINT('Ctrl Pts',(15.1814232310733,38.4443525286098,-235.35005));
#213259=CARTESIAN_POINT('Ctrl Pts',(15.4248261113785,38.3960995539571,-235.35005));
#213260=CARTESIAN_POINT('Ctrl Pts',(15.5466660621667,38.3719456078342,-235.35005));
#213261=CARTESIAN_POINT('Ctrl Pts',(15.6684514484779,38.3465730678228,-235.35005));
#213262=CARTESIAN_POINT('Ctrl Pts',(15.7901818197943,38.3199719796031,-235.35005));
#213263=CARTESIAN_POINT('Ctrl Pts',(15.8510470109318,38.3066714342958,-235.35005));
#213264=CARTESIAN_POINT('Ctrl Pts',(15.9118984485245,38.2930637565816,-235.35005));
#213265=CARTESIAN_POINT('Ctrl Pts',(15.9727360775264,38.2791477304796,-235.35005));
#213266=CARTESIAN_POINT('Ctrl Pts',(16.0031548939305,38.2721897169932,-235.35005));
#213267=CARTESIAN_POINT('Ctrl Pts',(16.0335702581983,38.2651546167241,-235.35005));
#213268=CARTESIAN_POINT('Ctrl Pts',(16.0639821635381,38.258042279449,-235.35005));
#213269=CARTESIAN_POINT('Ctrl Pts',(16.0791881167504,38.2544861106846,-235.35005));
#213270=CARTESIAN_POINT('Ctrl Pts',(16.0943932052251,38.2509106327023,-235.35005));
#213271=CARTESIAN_POINT('Ctrl Pts',(16.1095974281268,38.2473158268211,-235.35005));
#213272=CARTESIAN_POINT('Ctrl Pts',(16.1248016514155,38.2437210208484,-235.35005));
#213273=CARTESIAN_POINT('Ctrl Pts',(16.140004616612,38.2400982081071,-235.35005));
#213274=CARTESIAN_POINT('Ctrl Pts',(16.1552076180073,38.2364760332375,-235.35005));
#213275=CARTESIAN_POINT('Ctrl Pts',(16.1554380518469,38.236421131469,-235.35005));
#213276=CARTESIAN_POINT('Ctrl Pts',(16.1556684859374,38.2363662336162,-235.35005));
#213277=CARTESIAN_POINT('Ctrl Pts',(16.1558989202787,38.2363113396791,-235.35005));
#213278=CARTESIAN_POINT('Ctrl Pts',(16.6421654924883,38.1204731945768,-235.35005));
#213279=CARTESIAN_POINT('Ctrl Pts',(17.1295496308336,38.0220712232916,-235.35005));
#213280=CARTESIAN_POINT('Ctrl Pts',(17.6180162768063,37.9405600316208,-235.35005));
#213281=CARTESIAN_POINT('Ctrl Pts',(17.6182014583502,37.9405291300875,-235.35005));
#213282=CARTESIAN_POINT('Ctrl Pts',(17.6183866400499,37.9404982309457,-235.35005));
#213283=CARTESIAN_POINT('Ctrl Pts',(17.6185718219055,37.9404673341953,-235.35005));
#213284=CARTESIAN_POINT('Ctrl Pts',(18.5958771217087,37.7774083899181,-235.35005));
#213285=CARTESIAN_POINT('Ctrl Pts',(19.5774518164961,37.6809633951712,-235.35005));
#213286=CARTESIAN_POINT('Ctrl Pts',(20.563312329756,37.6513870472214,-235.35005));
#213287=CARTESIAN_POINT('Ctrl Pts',(21.5491728430159,37.6218106992716,-235.35005));
#213288=CARTESIAN_POINT('Ctrl Pts',(22.5393191900798,37.6591029589904,-235.35005));
#213289=CARTESIAN_POINT('Ctrl Pts',(23.5337713018193,37.7635770079652,-235.35005));
#213290=CARTESIAN_POINT('Ctrl Pts',(9.39019403218236,39.9042967860601,-234.645338670229));
#213291=CARTESIAN_POINT('Ctrl Pts',(9.37475363168684,39.9026279307258,-234.645212295458));
#213292=CARTESIAN_POINT('Ctrl Pts',(9.36241909261664,39.9009373862515,-234.645694439942));
#213293=CARTESIAN_POINT('Ctrl Pts',(9.34854130807218,39.8992799258028,-234.645872989761));
#213294=CARTESIAN_POINT('Ctrl Pts',(9.33401289064803,39.8975447585514,-234.64605991054));
#213295=CARTESIAN_POINT('Ctrl Pts',(9.3194845954082,39.8958258317407,-234.646245963641));
#213296=CARTESIAN_POINT('Ctrl Pts',(9.30495632258662,39.894123111551,-234.646431157816));
#213297=CARTESIAN_POINT('Ctrl Pts',(9.27590137992507,39.8907178590417,-234.646801525732));
#213298=CARTESIAN_POINT('Ctrl Pts',(9.24684652697401,39.887377424119,-234.64716845854));
#213299=CARTESIAN_POINT('Ctrl Pts',(9.21779096466109,39.8841015577674,-234.647532022749));
#213300=CARTESIAN_POINT('Ctrl Pts',(9.15969278284146,39.8775512842996,-234.648258989216));
#213301=CARTESIAN_POINT('Ctrl Pts',(9.10159176571151,39.871259142112,-234.648972491407));
#213302=CARTESIAN_POINT('Ctrl Pts',(9.04348151135069,39.8652234793331,-234.64967300902));
#213303=CARTESIAN_POINT('Ctrl Pts',(8.92736484808448,39.8531629397571,-234.65107279239));
#213304=CARTESIAN_POINT('Ctrl Pts',(8.81121130823973,39.8421260486728,-234.652420791411));
#213305=CARTESIAN_POINT('Ctrl Pts',(8.69496967544261,39.8321049357202,-234.653720059344));
#213306=CARTESIAN_POINT('Ctrl Pts',(8.46608431126897,39.8123728824755,-234.656278380377));
#213307=CARTESIAN_POINT('Ctrl Pts',(8.23695543614247,39.7965715522408,-234.658649489037));
#213308=CARTESIAN_POINT('Ctrl Pts',(8.00713518629142,39.7847168766851,-234.660839220159));
#213309=CARTESIAN_POINT('Ctrl Pts',(7.83476999890313,39.7758258700182,-234.662481518501));
#213310=CARTESIAN_POINT('Ctrl Pts',(7.66201598405601,39.7691561378415,-234.664021730675));
#213311=CARTESIAN_POINT('Ctrl Pts',(7.48868554439324,39.7647375575943,-234.66546127314));
#213312=CARTESIAN_POINT('Ctrl Pts',(7.35868771464617,39.761423622409,-234.666540929989));
#213313=CARTESIAN_POINT('Ctrl Pts',(7.2283656693242,39.7593763654488,-234.667563941682));
#213314=CARTESIAN_POINT('Ctrl Pts',(7.09764070666038,39.758615755376,-234.668530586038));
#213315=CARTESIAN_POINT('Ctrl Pts',(7.06314672882331,39.7584150556285,-234.668785651393));
#213316=CARTESIAN_POINT('Ctrl Pts',(7.02862017588322,39.758304000414,-234.669036821695));
#213317=CARTESIAN_POINT('Ctrl Pts',(6.99409009464001,39.7582829607004,-234.669283884834));
#213318=CARTESIAN_POINT('Ctrl Pts',(6.75867700422119,39.7581395198566,-234.670968268276));
#213319=CARTESIAN_POINT('Ctrl Pts',(6.52286201588005,39.762181854609,-234.672463355194));
#213320=CARTESIAN_POINT('Ctrl Pts',(6.28701389358818,39.7704255684024,-234.673769643912));
#213321=CARTESIAN_POINT('Ctrl Pts',(6.16414506741507,39.7747202620691,-234.674450175773));
#213322=CARTESIAN_POINT('Ctrl Pts',(6.04126720097618,39.7801543731084,-234.67507950791));
#213323=CARTESIAN_POINT('Ctrl Pts',(5.91843211982557,39.7867245213383,-234.675657972016));
#213324=CARTESIAN_POINT('Ctrl Pts',(5.89988148264417,39.7877167495755,-234.675745332057));
#213325=CARTESIAN_POINT('Ctrl Pts',(5.88133207614076,39.7887348794358,-234.675831546829));
#213326=CARTESIAN_POINT('Ctrl Pts',(5.8627840714653,39.7897789158681,-234.675916615161));
#213327=CARTESIAN_POINT('Ctrl Pts',(5.66502610646588,39.8009103838531,-234.676823609769));
#213328=CARTESIAN_POINT('Ctrl Pts',(5.46740597226592,39.8149903643949,-234.677600277792));
#213329=CARTESIAN_POINT('Ctrl Pts',(5.27014966576015,39.8320105075238,-234.678245806341));
#213330=CARTESIAN_POINT('Ctrl Pts',(5.17152151250727,39.8405205790883,-234.678568570616));
#213331=CARTESIAN_POINT('Ctrl Pts',(5.07298423927242,39.8497646508467,-234.678859485214));
#213332=CARTESIAN_POINT('Ctrl Pts',(4.97456616129474,39.8597402211668,-234.679116775072));
#213333=CARTESIAN_POINT('Ctrl Pts',(4.9253571223059,39.8647280063269,-234.67924542));
#213334=CARTESIAN_POINT('Ctrl Pts',(4.87617787852371,39.8698986474593,-234.679365646105));
#213335=CARTESIAN_POINT('Ctrl Pts',(4.82703162371335,39.875251446779,-234.679477627772));
#213336=CARTESIAN_POINT('Ctrl Pts',(4.80245849630817,39.8779278464388,-234.679533618606));
#213337=CARTESIAN_POINT('Ctrl Pts',(4.77789361616645,39.8806497845711,-234.67958754763));
#213338=CARTESIAN_POINT('Ctrl Pts',(4.75333738875916,39.8834171708839,-234.679639426256));
#213339=CARTESIAN_POINT('Ctrl Pts',(4.73148831986303,39.8858794715136,-234.679685585614));
#213340=CARTESIAN_POINT('Ctrl Pts',(4.70816077797056,39.8885496195412,-234.679733064146));
#213341=CARTESIAN_POINT('Ctrl Pts',(4.68731978273058,39.8909689272488,-234.679774062183));
#213342=CARTESIAN_POINT('Ctrl Pts',(4.68473752726179,39.8912686859929,-234.679779141951));
#213343=CARTESIAN_POINT('Ctrl Pts',(4.68219344082424,39.8915645279947,-234.679784125136));
#213344=CARTESIAN_POINT('Ctrl Pts',(4.67969506209335,39.8918555273409,-234.679788999259));
#213345=CARTESIAN_POINT('Ctrl Pts',(4.63296703344735,39.8972981872607,-234.679880161636));
#213346=CARTESIAN_POINT('Ctrl Pts',(4.58600312877882,39.9029307496431,-234.679973381372));
#213347=CARTESIAN_POINT('Ctrl Pts',(4.53885549843968,39.9087526218986,-234.680067252505));
#213348=CARTESIAN_POINT('Ctrl Pts',(4.424673154427,39.9228520584111,-234.680294590038));
#213349=CARTESIAN_POINT('Ctrl Pts',(4.30941205520417,39.9380630127427,-234.680526134682));
#213350=CARTESIAN_POINT('Ctrl Pts',(4.19382133831405,39.9543414584605,-234.680743553396));
#213351=CARTESIAN_POINT('Ctrl Pts',(4.07974483468867,39.9704066600778,-234.680958123972));
#213352=CARTESIAN_POINT('Ctrl Pts',(3.96534735932018,39.9875115413643,-234.681158940829));
#213353=CARTESIAN_POINT('Ctrl Pts',(3.85134657577325,40.0055640599005,-234.681330634686));
#213354=CARTESIAN_POINT('Ctrl Pts',(3.79401158722453,40.0146433040193,-234.681416985542));
#213355=CARTESIAN_POINT('Ctrl Pts',(3.73677693279445,40.0239616791513,-234.681495952715));
#213356=CARTESIAN_POINT('Ctrl Pts',(3.67973367637223,40.0335031384469,-234.681565687655));
#213357=CARTESIAN_POINT('Ctrl Pts',(3.64924621527456,40.0386026872338,-234.68160295834));
#213358=CARTESIAN_POINT('Ctrl Pts',(3.61985573216485,40.0436394880348,-234.681614478861));
#213359=CARTESIAN_POINT('Ctrl Pts',(3.58934324812148,40.0488965317388,-234.681649314366));
#213360=CARTESIAN_POINT('Ctrl Pts',(3.58443348443461,40.0497424426204,-234.681654919747));
#213361=CARTESIAN_POINT('Ctrl Pts',(3.57949477874549,40.0505940414076,-234.681661126376));
#213362=CARTESIAN_POINT('Ctrl Pts',(3.57451801904532,40.0514524893135,-234.681668135715));
#213363=CARTESIAN_POINT('Ctrl Pts',(3.55480123180177,40.0548534641928,-234.681695905116));
#213364=CARTESIAN_POINT('Ctrl Pts',(3.53463540183366,40.0583388372962,-234.681732190185));
#213365=CARTESIAN_POINT('Ctrl Pts',(3.51349260734251,40.0619750592967,-234.681788699843));
#213366=CARTESIAN_POINT('Ctrl Pts',(3.51050442728484,40.0624889784038,-234.681796686538));
#213367=CARTESIAN_POINT('Ctrl Pts',(3.50749681626456,40.0630059003384,-234.681805075349));
#213368=CARTESIAN_POINT('Ctrl Pts',(3.50446836416328,40.0635260027774,-234.681813897546));
#213369=CARTESIAN_POINT('Ctrl Pts',(3.42074441322775,40.0779046456038,-234.682057794152));
#213370=CARTESIAN_POINT('Ctrl Pts',(3.33972206686012,40.0913287970994,-234.682233612489));
#213371=CARTESIAN_POINT('Ctrl Pts',(3.26040169897432,40.1040349279776,-234.682363606509));
#213372=CARTESIAN_POINT('Ctrl Pts',(3.211926012102,40.1118001267308,-234.682443050787));
#213373=CARTESIAN_POINT('Ctrl Pts',(3.16408589205622,40.1192960752724,-234.682505367319));
#213374=CARTESIAN_POINT('Ctrl Pts',(3.11665238015447,40.126567293819,-234.682555524582));
#213375=CARTESIAN_POINT('Ctrl Pts',(3.03672015498941,40.1388203329636,-234.682640046716));
#213376=CARTESIAN_POINT('Ctrl Pts',(2.95793206930389,40.1504404103641,-234.68268994071));
#213377=CARTESIAN_POINT('Ctrl Pts',(2.87918968065051,40.1615981162924,-234.682728533227));
#213378=CARTESIAN_POINT('Ctrl Pts',(2.8008095715495,40.1727044876248,-234.682766948186));
#213379=CARTESIAN_POINT('Ctrl Pts',(2.72247466309021,40.1833526657526,-234.682794164161));
#213380=CARTESIAN_POINT('Ctrl Pts',(2.64309811212022,40.193659954308,-234.682832586117));
#213381=CARTESIAN_POINT('Ctrl Pts',(2.57411475280095,40.2026176550564,-234.682865977282));
#213382=CARTESIAN_POINT('Ctrl Pts',(2.50434458908083,40.2113172116199,-234.682907824178));
#213383=CARTESIAN_POINT('Ctrl Pts',(2.43307271489723,40.21980369842,-234.682972457297));
#213384=CARTESIAN_POINT('Ctrl Pts',(2.21676521285307,40.2455598719722,-234.683168616421));
#213385=CARTESIAN_POINT('Ctrl Pts',(1.99806321819614,40.2681244085811,-234.683337166398));
#213386=CARTESIAN_POINT('Ctrl Pts',(1.77667857288155,40.2873136365197,-234.683478702563));
#213387=CARTESIAN_POINT('Ctrl Pts',(1.55768037275675,40.306296011627,-234.68361871302));
#213388=CARTESIAN_POINT('Ctrl Pts',(1.33605684155172,40.3219755131914,-234.683732289647));
#213389=CARTESIAN_POINT('Ctrl Pts',(1.11153890722954,40.3341248594886,-234.683819419986));
#213390=CARTESIAN_POINT('Ctrl Pts',(0.891158232169992,40.3460503261405,
-234.683904944748));
#213391=CARTESIAN_POINT('Ctrl Pts',(0.667988651385312,40.354574546182,-234.68396498895));
#213392=CARTESIAN_POINT('Ctrl Pts',(0.441788148323699,40.3594342654747,
-234.68399896599));
#213393=CARTESIAN_POINT('Ctrl Pts',(0.295808050543585,40.3625705197621,
-234.684020893315));
#213394=CARTESIAN_POINT('Ctrl Pts',(0.14856587322869,40.3641795877876,-234.684031952444));
#213395=CARTESIAN_POINT('Ctrl Pts',(2.66453525910038E-15,40.3641796532955,
-234.68403185425));
#213396=CARTESIAN_POINT('Ctrl Pts',(23.3814806446219,39.0698185248112,-234.571621167217));
#213397=CARTESIAN_POINT('Ctrl Pts',(23.4282937951356,38.6452631234932,-235.35005));
#213398=CARTESIAN_POINT('Ctrl Pts',(23.525610634336,37.7626986794242,-235.35005));
#213399=CARTESIAN_POINT('Ctrl Pts',(23.5896364911122,39.0717917430095,-234.609597560408));
#213400=CARTESIAN_POINT('Ctrl Pts',(23.6056657686035,38.6356324734982,-235.35005));
#213401=CARTESIAN_POINT('Ctrl Pts',(23.6385084238607,37.775139906398,-235.35005));
#213402=CARTESIAN_POINT('Ctrl Pts',(23.7999845563376,39.0524591845457,-234.643035391158));
#213403=CARTESIAN_POINT('Ctrl Pts',(23.7829033814932,38.6107706130362,-235.35005));
#213404=CARTESIAN_POINT('Ctrl Pts',(23.7514657535404,37.7755620251222,-235.35005));
#213405=CARTESIAN_POINT('Ctrl Pts',(24.0125934783339,39.0086422970752,-234.671185933941));
#213406=CARTESIAN_POINT('Ctrl Pts',(23.9601413389653,38.5676758646721,-235.35005));
#213407=CARTESIAN_POINT('Ctrl Pts',(23.8643244195193,37.7621460828182,-235.35005));
#213408=CARTESIAN_POINT('',(23.9972286459191,39.0117604146193,-234.669151583121));
#213409=CARTESIAN_POINT('',(23.8561664752437,37.7630917536256,-235.35005));
#213410=CARTESIAN_POINT('Origin',(23.8561664752439,37.7630917536255,-233.85005));
#213411=CARTESIAN_POINT('Ctrl Pts',(23.5337713018193,37.7635770079652,-235.35005));
#213412=CARTESIAN_POINT('Ctrl Pts',(23.6412535989187,37.7748687641791,-235.35005));
#213413=CARTESIAN_POINT('Ctrl Pts',(23.7487194439798,37.7752300509467,-235.35005));
#213414=CARTESIAN_POINT('Ctrl Pts',(23.8561664752437,37.7630917536256,-235.35005));
#213415=CARTESIAN_POINT('Origin',(23.3783761769639,36.3745931076819,-233.942512591795));
#213416=CARTESIAN_POINT('Ctrl Pts',(23.9972286658434,39.0117605909834,-234.669151698811));
#213417=CARTESIAN_POINT('Ctrl Pts',(23.9474058055448,38.5707334611872,-235.35005));
#213418=CARTESIAN_POINT('Ctrl Pts',(23.8561664752439,37.7630917536255,-235.35005));
#213419=CARTESIAN_POINT('Ctrl Pts',(25.2366484173464,38.8718330388058,-234.669014852156));
#213420=CARTESIAN_POINT('Ctrl Pts',(25.1842887597299,38.431109053993,-235.350049999742));
#213421=CARTESIAN_POINT('Ctrl Pts',(25.0882853750842,37.6238992104159,-235.35005));
#213422=CARTESIAN_POINT('Ctrl Pts',(26.4747606339603,38.7210799284767,-234.668852342857));
#213423=CARTESIAN_POINT('Ctrl Pts',(26.4198403391809,38.280686857661,-235.35005000043));
#213424=CARTESIAN_POINT('Ctrl Pts',(26.319091123968,37.47392953931,-235.35005));
#213425=CARTESIAN_POINT('Ctrl Pts',(27.711570814231,38.5594513301076,-234.668667513818));
#213426=CARTESIAN_POINT('Ctrl Pts',(27.654024085186,38.1194242486926,-235.35005));
#213427=CARTESIAN_POINT('Ctrl Pts',(27.5485779004777,37.3131372941855,-235.35005));
#213428=CARTESIAN_POINT('',(27.7115708142298,38.5594513301044,-234.66866751382));
#213429=CARTESIAN_POINT('',(27.5485779004777,37.3131372941855,-235.35005));
#213430=CARTESIAN_POINT('Origin',(27.5485779004728,37.3131372941843,-233.850050000003));
#213431=CARTESIAN_POINT('Origin',(0.0633608499796878,-172.860463397757,
-235.350049999539));
#213432=CARTESIAN_POINT('Origin',(0.0438186590672052,-173.169156331663,
-234.199437903576));
#213433=CARTESIAN_POINT('Ctrl Pts',(27.6870869834027,38.5647076063785,-234.665458925605));
#213434=CARTESIAN_POINT('Ctrl Pts',(27.6312386219367,38.1248642240496,-235.350050000001));
#213435=CARTESIAN_POINT('Ctrl Pts',(27.5285055536634,37.315722493921,-235.35005));
#213436=CARTESIAN_POINT('Ctrl Pts',(27.7719185087418,38.5485509850084,-234.673701202518));
#213437=CARTESIAN_POINT('Ctrl Pts',(27.710388063005,38.1083834979961,-235.350049999996));
#213438=CARTESIAN_POINT('Ctrl Pts',(27.5986154970304,37.3068273115645,-235.35005));
#213439=CARTESIAN_POINT('Ctrl Pts',(27.8660265843471,38.5268314825978,-234.686074077228));
#213440=CARTESIAN_POINT('Ctrl Pts',(27.7951602584987,38.0865442976545,-235.350049999997));
#213441=CARTESIAN_POINT('Ctrl Pts',(27.6684770389457,37.2966022256818,-235.35005));
#213442=CARTESIAN_POINT('Ctrl Pts',(28.0107486443927,38.4840136200808,-234.708383241074));
#213443=CARTESIAN_POINT('Ctrl Pts',(27.9227914578621,38.0449642852773,-235.350050000001));
#213444=CARTESIAN_POINT('Ctrl Pts',(27.7691733848276,37.2776980879525,-235.35005));
#213445=CARTESIAN_POINT('Ctrl Pts',(28.056519267283,38.4693001007684,-234.715635823842));
#213446=CARTESIAN_POINT('Ctrl Pts',(27.9627817556189,38.0309145591475,-235.350049999995));
#213447=CARTESIAN_POINT('Ctrl Pts',(27.8004215724929,37.2712202551586,-235.35005));
#213448=CARTESIAN_POINT('Ctrl Pts',(28.1424207276373,38.4415180788525,-234.727204794551));
#213449=CARTESIAN_POINT('Ctrl Pts',(28.0391835813355,38.0045168186177,-235.350050000004));
#213450=CARTESIAN_POINT('Ctrl Pts',(27.8627200032187,37.2572093770216,-235.35005));
#213451=CARTESIAN_POINT('Ctrl Pts',(28.1818076781825,38.4289988027469,-234.731157474203));
#213452=CARTESIAN_POINT('Ctrl Pts',(28.0752081342426,37.9926116568254,-235.350050000001));
#213453=CARTESIAN_POINT('Ctrl Pts',(27.8937776977631,37.249697476023,-235.35005));
#213454=CARTESIAN_POINT('Ctrl Pts',(28.2939062760355,38.3943578402229,-234.739890329309));
#213455=CARTESIAN_POINT('Ctrl Pts',(28.1794856739151,37.959489646501,-235.350049999998));
#213456=CARTESIAN_POINT('Ctrl Pts',(27.9867858054616,37.226404790223,-235.35005));
#213457=CARTESIAN_POINT('Ctrl Pts',(28.3725698489465,38.3676355099575,-234.747582193031));
#213458=CARTESIAN_POINT('Ctrl Pts',(28.2511672609651,37.9342399780936,-235.35004999998));
#213459=CARTESIAN_POINT('Ctrl Pts',(28.0485551598146,37.2098945175254,-235.35005));
#213460=CARTESIAN_POINT('Ctrl Pts',(28.499560264286,38.3162258363163,-234.763633757846));
#213461=CARTESIAN_POINT('Ctrl Pts',(28.3635285899708,37.8869011682613,-235.35005000001));
#213462=CARTESIAN_POINT('Ctrl Pts',(28.1402497418155,37.1819908028498,-235.35005));
#213463=CARTESIAN_POINT('Ctrl Pts',(28.5414369654236,38.2984968797705,-234.768759787037));
#213464=CARTESIAN_POINT('Ctrl Pts',(28.4005824927214,37.8706765859433,-235.350049999998));
#213465=CARTESIAN_POINT('Ctrl Pts',(28.1706617267493,37.1721527193585,-235.35005));
#213466=CARTESIAN_POINT('Ctrl Pts',(28.6210886692051,38.2646056135699,-234.777052100967));
#213467=CARTESIAN_POINT('Ctrl Pts',(28.4721423102288,37.8394910733453,-235.350050000002));
#213468=CARTESIAN_POINT('Ctrl Pts',(28.2311847426228,37.1515938768492,-235.35005));
#213469=CARTESIAN_POINT('Ctrl Pts',(28.6588366351122,38.2485358813461,-234.78021126702));
#213470=CARTESIAN_POINT('Ctrl Pts',(28.5066596950528,37.8245853061929,-235.350049999988));
#213471=CARTESIAN_POINT('Ctrl Pts',(28.2612972505945,37.1409013962204,-235.35005));
#213472=CARTESIAN_POINT('Ctrl Pts',(28.7710344960755,38.1996667667751,-234.789253190342));
#213473=CARTESIAN_POINT('Ctrl Pts',(28.6093471685584,37.7792838182322,-235.350050000025));
#213474=CARTESIAN_POINT('Ctrl Pts',(28.3512820909987,37.1078462406674,-235.35005));
#213475=CARTESIAN_POINT('Ctrl Pts',(28.8428008206516,38.1677622719788,-234.793805028219));
#213476=CARTESIAN_POINT('Ctrl Pts',(28.6759158482819,37.7494700953236,-235.350049999991));
#213477=CARTESIAN_POINT('Ctrl Pts',(28.4108519482495,37.0845842971443,-235.35005));
#213478=CARTESIAN_POINT('Ctrl Pts',(28.9948913431262,38.0914060325279,-234.807859220985));
#213479=CARTESIAN_POINT('Ctrl Pts',(28.8130624304243,37.6798186719204,-235.350050000009));
#213480=CARTESIAN_POINT('Ctrl Pts',(28.5284852992461,37.0351888006413,-235.35005));
#213481=CARTESIAN_POINT('Ctrl Pts',(29.0707345298403,38.0497116584053,-234.815474578403));
#213482=CARTESIAN_POINT('Ctrl Pts',(28.8810490621556,37.6420974921894,-235.350050000012));
#213483=CARTESIAN_POINT('Ctrl Pts',(28.5864462918562,37.0087322113245,-235.35005));
#213484=CARTESIAN_POINT('Ctrl Pts',(29.1729198726625,37.994577684537,-234.821977012417));
#213485=CARTESIAN_POINT('Ctrl Pts',(28.9761856145916,37.590712775769,-235.350049999993));
#213486=CARTESIAN_POINT('Ctrl Pts',(28.6725892746692,36.9674060120273,-235.35005));
#213487=CARTESIAN_POINT('Ctrl Pts',(29.2059516364469,37.9766885523724,-234.82374012897));
#213488=CARTESIAN_POINT('Ctrl Pts',(29.0072562987579,37.573898403251,-235.350049999995));
#213489=CARTESIAN_POINT('Ctrl Pts',(28.7011808463655,36.9533782896452,-235.35005));
#213490=CARTESIAN_POINT('Ctrl Pts',(29.2546260372023,37.9501878862571,-234.826062930886));
#213491=CARTESIAN_POINT('Ctrl Pts',(29.0533143455601,37.5488533460758,-235.350050000003));
#213492=CARTESIAN_POINT('Ctrl Pts',(28.7439306930081,36.9320540547938,-235.35005));
#213493=CARTESIAN_POINT('Ctrl Pts',(29.2703961112124,37.941727494487,-234.826631844201));
#213494=CARTESIAN_POINT('Ctrl Pts',(29.0684051119755,37.5407696411564,-235.350050000002));
#213495=CARTESIAN_POINT('Ctrl Pts',(28.7581616928441,36.9249070270844,-235.35005));
#213496=CARTESIAN_POINT('Ctrl Pts',(29.3050706121592,37.9214977173636,-234.829332507218));
#213497=CARTESIAN_POINT('Ctrl Pts',(29.1002611313985,37.5221587047774,-235.350049999998));
#213498=CARTESIAN_POINT('Ctrl Pts',(28.7865561585441,36.9104741568002,-235.35005));
#213499=CARTESIAN_POINT('Ctrl Pts',(29.3237188905298,37.9099446994752,-234.831343174629));
#213500=CARTESIAN_POINT('Ctrl Pts',(29.1168776732614,37.5117934675614,-235.350049999998));
#213501=CARTESIAN_POINT('Ctrl Pts',(28.8007140683774,36.9031768938705,-235.35005));
#213502=CARTESIAN_POINT('Ctrl Pts',(29.4267902669213,37.8438444640261,-234.843360679698));
#213503=CARTESIAN_POINT('Ctrl Pts',(29.2077156164998,37.4530850279629,-235.350050000008));
#213504=CARTESIAN_POINT('Ctrl Pts',(28.8771404183119,36.8629106275395,-235.35005));
#213505=CARTESIAN_POINT('Ctrl Pts',(29.5070851154047,37.7891356470415,-234.850802470886));
#213506=CARTESIAN_POINT('Ctrl Pts',(29.2794078069932,37.4043310205184,-235.350050000069));
#213507=CARTESIAN_POINT('Ctrl Pts',(28.938176463821,36.8274085232238,-235.35005));
#213508=CARTESIAN_POINT('Ctrl Pts',(29.57158663008,37.7472855488698,-234.853784838128));
#213509=CARTESIAN_POINT('Ctrl Pts',(29.3419504108669,37.3639149821511,-235.350049999978));
#213510=CARTESIAN_POINT('Ctrl Pts',(28.9987888521635,36.7910354495401,-235.35005));
#213511=CARTESIAN_POINT('',(29.5524353619882,37.7591803693089,-234.853368133768));
#213512=CARTESIAN_POINT('',(28.9814172171126,36.8014272692484,-235.35005));
#213513=CARTESIAN_POINT('Origin',(28.9814172171126,36.8014272692485,-233.85005));
#213514=CARTESIAN_POINT('Ctrl Pts',(27.5485779004777,37.3131372941856,-235.35005));
#213515=CARTESIAN_POINT('Ctrl Pts',(27.6119497053713,37.3048495466029,-235.35005));
#213516=CARTESIAN_POINT('Ctrl Pts',(27.6750965458531,37.2953595193401,-235.35005));
#213517=CARTESIAN_POINT('Ctrl Pts',(27.7378143932095,37.2835852418792,-235.35005));
#213518=CARTESIAN_POINT('Ctrl Pts',(27.7691734109443,37.2776980854911,-235.35005));
#213519=CARTESIAN_POINT('Ctrl Pts',(27.8004215957617,37.2712202529943,-235.35005));
#213520=CARTESIAN_POINT('Ctrl Pts',(27.8315707886446,37.2642148195972,-235.35005));
#213521=CARTESIAN_POINT('Ctrl Pts',(27.8627200211639,37.257209377286,-235.35005));
#213522=CARTESIAN_POINT('Ctrl Pts',(27.8937777129896,37.2496974771633,-235.35005));
#213523=CARTESIAN_POINT('Ctrl Pts',(27.9247804016332,37.2419332526298,-235.35005));
#213524=CARTESIAN_POINT('Ctrl Pts',(27.9867858296455,37.2264047908593,-235.35005));
#213525=CARTESIAN_POINT('Ctrl Pts',(28.0485551618066,37.2098945246507,-235.35005));
#213526=CARTESIAN_POINT('Ctrl Pts',(28.1096848833639,37.191292048355,-235.35005));
#213527=CARTESIAN_POINT('Ctrl Pts',(28.1402497358115,37.1819908127424,-235.35005));
#213528=CARTESIAN_POINT('Ctrl Pts',(28.1706617181455,37.1721527303683,-235.35005));
#213529=CARTESIAN_POINT('Ctrl Pts',(28.2009232370621,37.1618733050988,-235.35005));
#213530=CARTESIAN_POINT('Ctrl Pts',(28.2311847284776,37.151593889171,-235.35005));
#213531=CARTESIAN_POINT('Ctrl Pts',(28.2612972337604,37.1409014094734,-235.35005));
#213532=CARTESIAN_POINT('Ctrl Pts',(28.2912921994266,37.129883016559,-235.35005));
#213533=CARTESIAN_POINT('Ctrl Pts',(28.3512820882545,37.1078462463438,-235.35005));
#213534=CARTESIAN_POINT('Ctrl Pts',(28.4108519466395,37.0845843013711,-235.35005));
#213535=CARTESIAN_POINT('Ctrl Pts',(28.4696686246939,37.0598865511459,-235.35005));
#213536=CARTESIAN_POINT('Ctrl Pts',(28.5284852999082,37.0351888021132,-235.35005));
#213537=CARTESIAN_POINT('Ctrl Pts',(28.5864462936913,37.0087322116309,-235.35005));
#213538=CARTESIAN_POINT('Ctrl Pts',(28.6438749473726,36.9811814124344,-235.35005));
#213539=CARTESIAN_POINT('Ctrl Pts',(28.6725892757669,36.9674060120908,-235.35005));
#213540=CARTESIAN_POINT('Ctrl Pts',(28.7011808475711,36.9533782894892,-235.35005));
#213541=CARTESIAN_POINT('Ctrl Pts',(28.7296807442605,36.9391621333448,-235.35005));
#213542=CARTESIAN_POINT('Ctrl Pts',(28.7439306934412,36.9320540548556,-235.35005));
#213543=CARTESIAN_POINT('Ctrl Pts',(28.7581616932791,36.9249070270955,-235.35005));
#213544=CARTESIAN_POINT('Ctrl Pts',(28.7723589257722,36.9176905920959,-235.35005));
#213545=CARTESIAN_POINT('Ctrl Pts',(28.7865561589916,36.9104741567272,-235.35005));
#213546=CARTESIAN_POINT('Ctrl Pts',(28.8007140688312,36.9031768937556,-235.350049999999));
#213547=CARTESIAN_POINT('Ctrl Pts',(28.8148092348245,36.8957506630084,-235.350049999999));
#213548=CARTESIAN_POINT('Ctrl Pts',(28.8711899085552,36.8660457348789,-235.35005));
#213549=CARTESIAN_POINT('Ctrl Pts',(28.9265109173313,36.834162754371,-235.35005));
#213550=CARTESIAN_POINT('Ctrl Pts',(28.9814172171126,36.8014272692486,-235.35005));
#213551=CARTESIAN_POINT('Ctrl Pts',(29.5524353619882,37.7591803693089,-234.853368133768));
#213552=CARTESIAN_POINT('Ctrl Pts',(29.5491926324494,37.7613057727392,-234.853184787816));
#213553=CARTESIAN_POINT('Ctrl Pts',(29.5240197950341,37.7782295017975,-234.851479445173));
#213554=CARTESIAN_POINT('Ctrl Pts',(29.4656769295574,37.8169869705738,-234.846638436175));
#213555=CARTESIAN_POINT('Ctrl Pts',(29.4430292295003,37.8319697079636,-234.844644267336));
#213556=CARTESIAN_POINT('Ctrl Pts',(29.4064983288726,37.8559033707158,-234.841082265319));
#213557=CARTESIAN_POINT('Ctrl Pts',(29.393891920648,37.8641262032719,-234.839799806521));
#213558=CARTESIAN_POINT('Ctrl Pts',(29.3745220620691,37.8766873104466,-234.837733431133));
#213559=CARTESIAN_POINT('Ctrl Pts',(29.364720492403,37.8830256448728,-234.836664571642));
#213560=CARTESIAN_POINT('Ctrl Pts',(29.3547602107045,37.889436685229,-234.835542204454));
#213561=CARTESIAN_POINT('Ctrl Pts',(29.3480849681094,37.8937264029729,-234.834782069063));
#213562=CARTESIAN_POINT('Ctrl Pts',(29.3431599492174,37.896884697379,-234.834213609395));
#213563=CARTESIAN_POINT('Ctrl Pts',(29.3269344760838,37.9072780544614,-234.832328004808));
#213564=CARTESIAN_POINT('Ctrl Pts',(29.3106731982457,37.9172298129869,-234.830768462726));
#213565=CARTESIAN_POINT('Ctrl Pts',(29.2835927346762,37.9331272185667,-234.828603975926));
#213566=CARTESIAN_POINT('Ctrl Pts',(29.2741105557623,37.9385928841534,-234.827911618046));
#213567=CARTESIAN_POINT('Ctrl Pts',(29.2541227809703,37.949925161019,-234.826585177729));
#213568=CARTESIAN_POINT('Ctrl Pts',(29.2420295816336,37.9566673222368,-234.825864724755));
#213569=CARTESIAN_POINT('Ctrl Pts',(29.2136736977047,37.9722710985875,-234.824309002214));
#213570=CARTESIAN_POINT('Ctrl Pts',(29.1855684322557,37.9875854621943,-234.822771960206));
#213571=CARTESIAN_POINT('Ctrl Pts',(29.1532951346241,38.00489189903,-234.821011435464));
#213572=CARTESIAN_POINT('Ctrl Pts',(29.1372971866779,38.0133983224047,-234.820139345825));
#213573=CARTESIAN_POINT('Ctrl Pts',(29.1304716785934,38.0170117572164,-234.819767344423));
#213574=CARTESIAN_POINT('Ctrl Pts',(29.1259282891305,38.0194134838505,-234.819519732666));
#213575=CARTESIAN_POINT('Ctrl Pts',(29.1224601838887,38.021243126175,-234.8193307323));
#213576=CARTESIAN_POINT('Ctrl Pts',(29.112876957114,38.0262939218943,-234.818808483686));
#213577=CARTESIAN_POINT('Ctrl Pts',(29.099091972616,38.0337742454385,-234.817813387705));
#213578=CARTESIAN_POINT('Ctrl Pts',(29.0617166158013,38.0540345686262,-234.814761445759));
#213579=CARTESIAN_POINT('Ctrl Pts',(29.0401123377758,38.065758808627,-234.812888384745));
#213580=CARTESIAN_POINT('Ctrl Pts',(28.9806261264644,38.0973901660411,-234.807345372931));
#213581=CARTESIAN_POINT('Ctrl Pts',(28.9568964003388,38.1096526154491,-234.8050823928));
#213582=CARTESIAN_POINT('Ctrl Pts',(28.9290986853599,38.1238356761779,-234.802450711269));
#213583=CARTESIAN_POINT('Ctrl Pts',(28.9211478514516,38.1278509098975,-234.801700615536));
#213584=CARTESIAN_POINT('Ctrl Pts',(28.9111398006015,38.1328722652928,-234.800766169102));
#213585=CARTESIAN_POINT('Ctrl Pts',(28.9066160197033,38.1351319973066,-234.800346620177));
#213586=CARTESIAN_POINT('Ctrl Pts',(28.9028073007853,38.137023509385,-234.799998582689));
#213587=CARTESIAN_POINT('Ctrl Pts',(28.9004267038557,38.1382033549997,-234.799782449127));
#213588=CARTESIAN_POINT('Ctrl Pts',(28.9006519492602,38.138093475601,-234.799801689135));
#213589=CARTESIAN_POINT('Ctrl Pts',(28.8603923905194,38.1579548763275,-234.796205569945));
#213590=CARTESIAN_POINT('Ctrl Pts',(28.8225168056264,38.1758599748975,-234.793009488469));
#213591=CARTESIAN_POINT('Ctrl Pts',(28.764802173272,38.2020805237224,-234.788498118192));
#213592=CARTESIAN_POINT('Ctrl Pts',(28.7358063284038,38.2149869383765,-234.786313121037));
#213593=CARTESIAN_POINT('Ctrl Pts',(28.7018880369674,38.2296247093678,-234.783887661662));
#213594=CARTESIAN_POINT('Ctrl Pts',(28.6873487976685,38.2358013396985,-234.782874687066));
#213595=CARTESIAN_POINT('Ctrl Pts',(28.6776571681367,38.2398968528113,-234.782205261335));
#213596=CARTESIAN_POINT('Ctrl Pts',(28.6713086966326,38.2425619960944,-234.781771443078));
#213597=CARTESIAN_POINT('Ctrl Pts',(28.6412446469546,38.2551316958537,-234.77973049979));
#213598=CARTESIAN_POINT('Ctrl Pts',(28.6086604316154,38.2692123122386,-234.776707683702));
#213599=CARTESIAN_POINT('Ctrl Pts',(28.5510250123839,38.2938456778358,-234.770360493156));
#213600=CARTESIAN_POINT('Ctrl Pts',(28.5303190038827,38.3026476050971,-234.767942601905));
#213601=CARTESIAN_POINT('Ctrl Pts',(28.4966982222806,38.316676932562,-234.763862523424));
#213602=CARTESIAN_POINT('Ctrl Pts',(28.4792436754406,38.3238987297857,-234.761709173783));
#213603=CARTESIAN_POINT('Ctrl Pts',(28.4576361932315,38.3326807579169,-234.758998639333));
#213604=CARTESIAN_POINT('Ctrl Pts',(28.4480932800145,38.3365208563917,-234.757794490312));
#213605=CARTESIAN_POINT('Ctrl Pts',(28.4416666436022,38.3390979108861,-234.756982281764));
#213606=CARTESIAN_POINT('Ctrl Pts',(28.4365548603845,38.3411379275027,-234.756334962636));
#213607=CARTESIAN_POINT('Ctrl Pts',(28.4125359635179,38.3507010239759,-234.753291057889));
#213608=CARTESIAN_POINT('Ctrl Pts',(28.3816986646669,38.3623133318808,-234.74992258177));
#213609=CARTESIAN_POINT('Ctrl Pts',(28.322073080104,38.3831376740941,-234.7441144307));
#213610=CARTESIAN_POINT('Ctrl Pts',(28.2999760393941,38.3906429251353,-234.742052474195));
#213611=CARTESIAN_POINT('Ctrl Pts',(28.263501193126,38.4026421762831,-234.738770680216));
#213612=CARTESIAN_POINT('Ctrl Pts',(28.2444334747144,38.4088266683947,-234.73708256842));
#213613=CARTESIAN_POINT('Ctrl Pts',(28.2207628641438,38.4163370068423,-234.735030478749));
#213614=CARTESIAN_POINT('Ctrl Pts',(28.2103182751279,38.4196155083141,-234.734133306195));
#213615=CARTESIAN_POINT('Ctrl Pts',(28.203288896498,38.421814079242,-234.733531256592));
#213616=CARTESIAN_POINT('Ctrl Pts',(28.1980412534931,38.4234473771363,-234.733083597214));
#213617=CARTESIAN_POINT('Ctrl Pts',(28.1660285620671,38.433384328389,-234.730358631913));
#213618=CARTESIAN_POINT('Ctrl Pts',(28.1321616178479,38.4444861390464,-234.726389507244));
#213619=CARTESIAN_POINT('Ctrl Pts',(28.0734215990991,38.4634880588082,-234.718329143074));
#213620=CARTESIAN_POINT('Ctrl Pts',(28.0524938758821,38.4702132584191,-234.715291242156));
#213621=CARTESIAN_POINT('Ctrl Pts',(28.0071718419697,38.4843984690794,-234.708513214599));
#213622=CARTESIAN_POINT('Ctrl Pts',(27.9846241143607,38.4913191645377,-234.705055551881));
#213623=CARTESIAN_POINT('Ctrl Pts',(27.8419926047998,38.5330360338839,-234.683187034774));
#213624=CARTESIAN_POINT('Ctrl Pts',(27.7485282251975,38.5520905058658,-234.672515589894));
#213625=CARTESIAN_POINT('Ctrl Pts',(27.7115708142298,38.5594513301044,-234.66866751382));
#213626=CARTESIAN_POINT('Ctrl Pts',(29.5524353619883,37.7591803693089,-234.853368133768));
#213627=CARTESIAN_POINT('Ctrl Pts',(29.3235739752807,37.3753174315541,-235.35005));
#213628=CARTESIAN_POINT('Ctrl Pts',(28.9814172171125,36.8014272692485,-235.35005));
#213629=CARTESIAN_POINT('Ctrl Pts',(31.4648905505278,36.611137072351,-234.860838757985));
#213630=CARTESIAN_POINT('Ctrl Pts',(31.2186416313246,36.2384660822587,-235.350049999758));
#213631=CARTESIAN_POINT('Ctrl Pts',(30.8601181894623,35.6813344771098,-235.35005));
#213632=CARTESIAN_POINT('Ctrl Pts',(33.2921480182203,35.3641827858728,-234.867835939374));
#213633=CARTESIAN_POINT('Ctrl Pts',(33.0331144993804,35.001495733651,-235.35004999988));
#213634=CARTESIAN_POINT('Ctrl Pts',(32.655766056176,34.4636022590608,-235.35005));
#213635=CARTESIAN_POINT('Ctrl Pts',(36.7811408986291,32.6755312616936,-234.878440733198));
#213636=CARTESIAN_POINT('Ctrl Pts',(36.4951099976157,32.3351522367808,-235.35005000012));
#213637=CARTESIAN_POINT('Ctrl Pts',(36.0822840599884,31.8353365675869,-235.35005));
#213638=CARTESIAN_POINT('Ctrl Pts',(38.4421442470284,31.2387599869711,-234.881588663467));
#213639=CARTESIAN_POINT('Ctrl Pts',(38.1454280191491,30.9083681195947,-235.35004999988));
#213640=CARTESIAN_POINT('Ctrl Pts',(37.7150530376205,30.426874953249,-235.35005));
#213641=CARTESIAN_POINT('Ctrl Pts',(40.8137176069411,28.9351791157808,-234.88379235176));
#213642=CARTESIAN_POINT('Ctrl Pts',(40.4984745671759,28.6231683352463,-235.35005000006));
#213643=CARTESIAN_POINT('Ctrl Pts',(40.0413171754775,28.170164696784,-235.35005));
#213644=CARTESIAN_POINT('Ctrl Pts',(41.5826620989581,28.1429897152722,-234.884007663936));
#213645=CARTESIAN_POINT('Ctrl Pts',(41.2615827441429,27.8370429556774,-235.35005));
#213646=CARTESIAN_POINT('Ctrl Pts',(40.7957050001434,27.3932780662659,-235.35005));
#213647=CARTESIAN_POINT('Ctrl Pts',(43.0792410059956,26.5108878965485,-234.883573054699));
#213648=CARTESIAN_POINT('Ctrl Pts',(42.7465875350161,26.217481845266,-235.35005));
#213649=CARTESIAN_POINT('Ctrl Pts',(42.2637158381442,25.7917312522435,-235.35005));
#213650=CARTESIAN_POINT('Ctrl Pts',(43.8083339671196,25.6692406662039,-234.882926062436));
#213651=CARTESIAN_POINT('Ctrl Pts',(43.4701616566366,25.3820633016541,-235.35005));
#213652=CARTESIAN_POINT('Ctrl Pts',(42.9787004139624,24.9654368934267,-235.35005));
#213653=CARTESIAN_POINT('Ctrl Pts',(45.9226558299789,23.0793988618607,-234.879757408134));
#213654=CARTESIAN_POINT('Ctrl Pts',(45.5679898267064,22.8118032008958,-235.35005));
#213655=CARTESIAN_POINT('Ctrl Pts',(45.0499412762525,22.4237082823892,-235.35005));
#213656=CARTESIAN_POINT('Ctrl Pts',(47.2266045706789,21.2758301574159,-234.876040016386));
#213657=CARTESIAN_POINT('Ctrl Pts',(46.8615872941006,21.0215780313956,-235.350049999181));
#213658=CARTESIAN_POINT('Ctrl Pts',(46.326104449877,20.6527388844884,-235.350050000001));
#213659=CARTESIAN_POINT('Ctrl Pts',(48.4260896922586,19.3965417854656,-234.872874618363));
#213660=CARTESIAN_POINT('Ctrl Pts',(48.0508084453091,19.1577111488603,-235.35005));
#213661=CARTESIAN_POINT('Ctrl Pts',(47.500448334379,18.8074595529597,-235.350050000001));
#213662=CARTESIAN_POINT('',(48.4260896922586,19.3965417854656,-234.872874618363));
#213663=CARTESIAN_POINT('',(47.5004483343782,18.8074595529612,-235.35005));
#213664=CARTESIAN_POINT('Origin',(47.5004483343794,18.8074595529594,-233.85005));
#213665=CARTESIAN_POINT('Ctrl Pts',(28.9814172171126,36.8014272692485,-235.35005));
#213666=CARTESIAN_POINT('Ctrl Pts',(30.4445221387459,35.9291153361866,-235.35005));
#213667=CARTESIAN_POINT('Ctrl Pts',(31.8571523563316,34.997650520712,-235.35005));
#213668=CARTESIAN_POINT('Ctrl Pts',(33.219749332275,34.0075501952443,-235.35005));
#213669=CARTESIAN_POINT('Ctrl Pts',(33.6068768507225,33.7262527252077,-235.35005));
#213670=CARTESIAN_POINT('Ctrl Pts',(33.9899655501622,33.4402220370432,-235.35005));
#213671=CARTESIAN_POINT('Ctrl Pts',(34.3690250580976,33.1494694133448,-235.35005));
#213672=CARTESIAN_POINT('Ctrl Pts',(36.0822840600053,31.8353365675737,-235.35005));
#213673=CARTESIAN_POINT('Ctrl Pts',(37.7150530376344,30.4268749532356,-235.35005));
#213674=CARTESIAN_POINT('Ctrl Pts',(39.2658957962434,28.9224014489936,-235.35005));
#213675=CARTESIAN_POINT('Ctrl Pts',(40.0413171755479,28.1701646968727,-235.35005));
#213676=CARTESIAN_POINT('Ctrl Pts',(40.7957050001266,27.3932780662842,-235.35005));
#213677=CARTESIAN_POINT('Ctrl Pts',(41.52971041916,26.5925046592713,-235.35005));
#213678=CARTESIAN_POINT('Ctrl Pts',(42.2637158381934,25.7917312522584,-235.35005));
#213679=CARTESIAN_POINT('Ctrl Pts',(42.9787004139405,24.9654368934535,-235.35005));
#213680=CARTESIAN_POINT('Ctrl Pts',(43.669114034758,24.1181940231093,-235.35005));
#213681=CARTESIAN_POINT('Ctrl Pts',(45.0499412763931,22.423708282421,-235.35005));
#213682=CARTESIAN_POINT('Ctrl Pts',(46.3260905825898,20.6527606745438,-235.350050000001));
#213683=CARTESIAN_POINT('Ctrl Pts',(47.5004483343782,18.8074595529612,-235.350050000001));
#213684=CARTESIAN_POINT('Ctrl Pts',(48.4260896922586,19.3965417854656,-234.872874618363));
#213685=CARTESIAN_POINT('Ctrl Pts',(48.1436564566979,19.8390426530017,-234.873620088043));
#213686=CARTESIAN_POINT('Ctrl Pts',(47.8509659213957,20.2843345271102,-234.874408251377));
#213687=CARTESIAN_POINT('Ctrl Pts',(47.5478312881813,20.7314567814701,-234.875210279537));
#213688=CARTESIAN_POINT('Ctrl Pts',(47.2446966549669,21.17857903583,-234.876012307697));
#213689=CARTESIAN_POINT('Ctrl Pts',(46.9311176254783,21.6275314483713,-234.876828174927));
#213690=CARTESIAN_POINT('Ctrl Pts',(46.6069504587922,22.077383516232,-234.877623828772));
#213691=CARTESIAN_POINT('Ctrl Pts',(46.2853158480958,22.5237211148126,-234.878413266572));
#213692=CARTESIAN_POINT('Ctrl Pts',(45.9532587493137,22.9709428450799,-234.879182696605));
#213693=CARTESIAN_POINT('Ctrl Pts',(45.6106846858941,23.4181728809532,-234.879894109809));
#213694=CARTESIAN_POINT('Ctrl Pts',(45.438886706838,23.6424549400482,-234.880250877479));
#213695=CARTESIAN_POINT('Ctrl Pts',(45.2644444625615,23.8667396990142,-234.880592984785));
#213696=CARTESIAN_POINT('Ctrl Pts',(45.0873500700682,24.0909207476239,-234.880915242521));
#213697=CARTESIAN_POINT('Ctrl Pts',(44.9562263439977,24.256908241605,-234.881153847676));
#213698=CARTESIAN_POINT('Ctrl Pts',(44.8236483565289,24.4228393854534,-234.881381566083));
#213699=CARTESIAN_POINT('Ctrl Pts',(44.6896149039642,24.5886707122256,-234.881596204268));
#213700=CARTESIAN_POINT('Ctrl Pts',(44.6437008912031,24.6454772892997,-234.881669729945));
#213701=CARTESIAN_POINT('Ctrl Pts',(44.5976160952632,24.7022721553739,-234.881741720083));
#213702=CARTESIAN_POINT('Ctrl Pts',(44.5513620989383,24.7590516304435,-234.881812082364));
#213703=CARTESIAN_POINT('Ctrl Pts',(44.545635411938,24.7660814723512,-234.881820793888));
#213704=CARTESIAN_POINT('Ctrl Pts',(44.5389068663795,24.7743365414615,-234.881830990484));
#213705=CARTESIAN_POINT('Ctrl Pts',(44.5341724311188,24.7801389607782,-234.881840625232));
#213706=CARTESIAN_POINT('Ctrl Pts',(44.5271568104213,24.7887371505964,-234.881854902274));
#213707=CARTESIAN_POINT('Ctrl Pts',(44.5201320288114,24.7973415118698,-234.881869112118));
#213708=CARTESIAN_POINT('Ctrl Pts',(44.5130980691041,24.8059520361687,-234.881883254527));
#213709=CARTESIAN_POINT('Ctrl Pts',(44.3158466991869,25.0474145671404,-234.882279846158));
#213710=CARTESIAN_POINT('Ctrl Pts',(44.1115390894415,25.2935411331283,-234.882622828519));
#213711=CARTESIAN_POINT('Ctrl Pts',(43.8999455772027,25.5440099170768,-234.882911996411));
#213712=CARTESIAN_POINT('Ctrl Pts',(43.6836301225591,25.8000681879592,-234.883207617403));
#213713=CARTESIAN_POINT('Ctrl Pts',(43.4596994985199,26.0606651779403,-234.883446999152));
#213714=CARTESIAN_POINT('Ctrl Pts',(43.2279311288734,26.3254037209598,-234.883629298961));
#213715=CARTESIAN_POINT('Ctrl Pts',(43.0126714435026,26.5712851393899,-234.883798613693));
#213716=CARTESIAN_POINT('Ctrl Pts',(42.7906507648766,26.8207388317917,-234.883918683362));
#213717=CARTESIAN_POINT('Ctrl Pts',(42.5617130696684,27.0734008284491,-234.883988328101));
#213718=CARTESIAN_POINT('Ctrl Pts',(42.5441553921939,27.0927779687813,-234.883993669291));
#213719=CARTESIAN_POINT('Ctrl Pts',(42.5265570430006,27.1121739565691,-234.883998713658));
#213720=CARTESIAN_POINT('Ctrl Pts',(42.5089179577211,27.1315886162052,-234.88400346055));
#213721=CARTESIAN_POINT('Ctrl Pts',(42.4499887161555,27.1964497555151,-234.884019319121));
#213722=CARTESIAN_POINT('Ctrl Pts',(42.3906068528995,27.2615162095477,-234.884032443793));
#213723=CARTESIAN_POINT('Ctrl Pts',(42.3307745648553,27.3267765754063,-234.884042740597));
#213724=CARTESIAN_POINT('Ctrl Pts',(42.0118162244203,27.674671310354,-234.884097631552));
#213725=CARTESIAN_POINT('Ctrl Pts',(41.6797936742668,28.0283910413513,-234.884071798873));
#213726=CARTESIAN_POINT('Ctrl Pts',(41.3345347980372,28.3865291569703,-234.883944724371));
#213727=CARTESIAN_POINT('Ctrl Pts',(41.1295224027873,28.5991891578229,-234.883869268387));
#213728=CARTESIAN_POINT('Ctrl Pts',(40.9198276686865,28.813423315708,-234.883757772487));
#213729=CARTESIAN_POINT('Ctrl Pts',(40.7054078632846,29.0289348621045,-234.883611946477));
#213730=CARTESIAN_POINT('Ctrl Pts',(40.5981979605837,29.1366906353028,-234.883539033472));
#213731=CARTESIAN_POINT('Ctrl Pts',(40.4898070746579,29.2447653313473,-234.883457642229));
#213732=CARTESIAN_POINT('Ctrl Pts',(40.3802316765946,29.353119299156,-234.883368704201));
#213733=CARTESIAN_POINT('Ctrl Pts',(40.325443977563,29.4072962830604,-234.883324235188));
#213734=CARTESIAN_POINT('Ctrl Pts',(40.2703601511891,29.4615430861951,-234.883277880788));
#213735=CARTESIAN_POINT('Ctrl Pts',(40.2149798991556,29.5158545609305,-234.883229817462));
#213736=CARTESIAN_POINT('Ctrl Pts',(40.1872897731388,29.5430102982982,-234.883205785799));
#213737=CARTESIAN_POINT('Ctrl Pts',(40.1595255407743,29.5701822037018,-234.883181327038));
#213738=CARTESIAN_POINT('Ctrl Pts',(40.1316871684786,29.5973696282592,-234.883156466412));
#213739=CARTESIAN_POINT('Ctrl Pts',(40.1177679823308,29.6109633405379,-234.883144036099));
#213740=CARTESIAN_POINT('Ctrl Pts',(40.1038302612033,29.6245609326156,-234.883131505329));
#213741=CARTESIAN_POINT('Ctrl Pts',(40.0898740052607,29.63816232471,-234.883118873174));
#213742=CARTESIAN_POINT('Ctrl Pts',(40.0828958772893,29.6449630207572,-234.883112557097));
#213743=CARTESIAN_POINT('Ctrl Pts',(40.0759131156145,29.6517646668093,-234.883106215674));
#213744=CARTESIAN_POINT('Ctrl Pts',(40.0689257220724,29.6585672537589,-234.883099846813));
#213745=CARTESIAN_POINT('Ctrl Pts',(40.0654320253014,29.6619685472337,-234.883096662382));
#213746=CARTESIAN_POINT('Ctrl Pts',(40.0619371705636,29.6653700759328,-234.883093471092));
#213747=CARTESIAN_POINT('Ctrl Pts',(40.0584411579672,29.6687718386519,-234.88309027282));
#213748=CARTESIAN_POINT('Ctrl Pts',(40.0549451453709,29.672173601371,-234.883087074548));
#213749=CARTESIAN_POINT('Ctrl Pts',(40.0502325503488,29.6767576351331,-234.88308275321));
#213750=CARTESIAN_POINT('Ctrl Pts',(40.0479496434506,29.6789778242853,-234.883080661882));
#213751=CARTESIAN_POINT('Ctrl Pts',(40.0397122613223,29.6869889028178,-234.883073115772));
#213752=CARTESIAN_POINT('Ctrl Pts',(40.0314600881385,29.6950094293739,-234.88306551114));
#213753=CARTESIAN_POINT('Ctrl Pts',(40.0231931152336,29.7030393665907,-234.883057847064));
#213754=CARTESIAN_POINT('Ctrl Pts',(39.7340648184162,29.9838776005799,-234.882789804435));
#213755=CARTESIAN_POINT('Ctrl Pts',(39.4270515363959,30.2761740869847,-234.882462612569));
#213756=CARTESIAN_POINT('Ctrl Pts',(39.101843125911,30.5783620144702,-234.882040882582));
#213757=CARTESIAN_POINT('Ctrl Pts',(38.7766347154261,30.8805499419557,-234.881619152595));
#213758=CARTESIAN_POINT('Ctrl Pts',(38.4332306415388,31.1926281065363,-234.881102902623));
#213759=CARTESIAN_POINT('Ctrl Pts',(38.0712682413355,31.513016787025,-234.880453655042));
#213760=CARTESIAN_POINT('Ctrl Pts',(37.7729361607464,31.7770835011195,-234.879918540395));
#213761=CARTESIAN_POINT('Ctrl Pts',(37.4619590556278,32.0468022993597,-234.87930828589));
#213762=CARTESIAN_POINT('Ctrl Pts',(37.1385945228072,32.320888272906,-234.878607331997));
#213763=CARTESIAN_POINT('Ctrl Pts',(36.8341596152557,32.5789293675489,-234.877947411653));
#213764=CARTESIAN_POINT('Ctrl Pts',(36.5187448436518,32.8408411776355,-234.877207085432));
#213765=CARTESIAN_POINT('Ctrl Pts',(36.1925832819071,33.105593930084,-234.876373009221));
#213766=CARTESIAN_POINT('Ctrl Pts',(36.0125010781191,33.2517707476859,-234.87591249425));
#213767=CARTESIAN_POINT('Ctrl Pts',(35.8291431433675,33.3988143820157,-234.875423394975));
#213768=CARTESIAN_POINT('Ctrl Pts',(35.6425517526153,33.5465577186068,-234.874903437951));
#213769=CARTESIAN_POINT('Ctrl Pts',(35.4441641375414,33.7036413228997,-234.874350609477));
#213770=CARTESIAN_POINT('Ctrl Pts',(35.2421697499994,33.8614772542077,-234.873763030408));
#213771=CARTESIAN_POINT('Ctrl Pts',(35.0366444584247,34.0198570237832,-234.873138336286));
#213772=CARTESIAN_POINT('Ctrl Pts',(34.7129239504967,34.2693191656913,-234.872154387806));
#213773=CARTESIAN_POINT('Ctrl Pts',(34.380467076446,34.519959127306,-234.871093998833));
#213774=CARTESIAN_POINT('Ctrl Pts',(34.0396050005138,34.7709265774286,-234.869961744777));
#213775=CARTESIAN_POINT('Ctrl Pts',(33.7084194077682,35.0147694968892,-234.86886163345));
#213776=CARTESIAN_POINT('Ctrl Pts',(33.3692989638713,35.258921486016,-234.86769369779));
#213777=CARTESIAN_POINT('Ctrl Pts',(33.0225787895569,35.5026409891713,-234.866464203128));
#213778=CARTESIAN_POINT('Ctrl Pts',(32.9437420428357,35.5580575878139,-234.866184642357));
#213779=CARTESIAN_POINT('Ctrl Pts',(32.8645125168478,35.6134519903396,-234.865901906941));
#213780=CARTESIAN_POINT('Ctrl Pts',(32.7848943935183,35.668815773732,-234.865616084469));
#213781=CARTESIAN_POINT('Ctrl Pts',(32.4766529029193,35.8831566097681,-234.864509523031));
#213782=CARTESIAN_POINT('Ctrl Pts',(32.1625673629801,36.0970471664988,-234.863356567381));
#213783=CARTESIAN_POINT('Ctrl Pts',(31.8430678702853,36.3099026177018,-234.862163622325));
#213784=CARTESIAN_POINT('Ctrl Pts',(31.526926929929,36.5205205499423,-234.86098321741));
#213785=CARTESIAN_POINT('Ctrl Pts',(31.2054851825615,36.7301249484346,-234.85976367324));
#213786=CARTESIAN_POINT('Ctrl Pts',(30.8791919628904,36.9381880666467,-234.858512247707));
#213787=CARTESIAN_POINT('Ctrl Pts',(30.556834934552,37.1437412453529,-234.857275918566));
#213788=CARTESIAN_POINT('Ctrl Pts',(30.2297427352299,37.347790071322,-234.856008487168));
#213789=CARTESIAN_POINT('Ctrl Pts',(29.898381554584,37.549864558993,-234.854717774197));
#213790=CARTESIAN_POINT('Ctrl Pts',(29.7835715652017,37.6198793076691,-234.854270568094));
#213791=CARTESIAN_POINT('Ctrl Pts',(29.6682493871885,37.689657388203,-234.853820573372));
#213792=CARTESIAN_POINT('Ctrl Pts',(29.5524353619883,37.7591803693088,-234.853368133768));
#213793=CARTESIAN_POINT('Ctrl Pts',(48.4267513656518,19.3969628773257,-234.872032644088));
#213794=CARTESIAN_POINT('Ctrl Pts',(48.051385728879,19.1580785346661,-235.35005));
#213795=CARTESIAN_POINT('Ctrl Pts',(47.5004483343777,18.8074595529617,-235.35005));
#213796=CARTESIAN_POINT('Ctrl Pts',(48.4549570879676,19.355316987603,-234.870489902149));
#213797=CARTESIAN_POINT('Ctrl Pts',(48.077778833099,19.1189416686644,-235.350049999978));
#213798=CARTESIAN_POINT('Ctrl Pts',(47.5233281555475,18.7715078669293,-235.35005));
#213799=CARTESIAN_POINT('Ctrl Pts',(48.4839707017497,19.3121694435219,-234.86855017653));
#213800=CARTESIAN_POINT('Ctrl Pts',(48.1045857201146,19.0788852177624,-235.350050000005));
#213801=CARTESIAN_POINT('Ctrl Pts',(47.5458232280531,18.7353573183218,-235.35005));
#213802=CARTESIAN_POINT('Ctrl Pts',(48.5451033552256,19.2200302642562,-234.863016541227));
#213803=CARTESIAN_POINT('Ctrl Pts',(48.1599244780088,18.99523376352,-235.350049999995));
#213804=CARTESIAN_POINT('Ctrl Pts',(47.5895300323829,18.6623978031499,-235.35005));
#213805=CARTESIAN_POINT('Ctrl Pts',(48.5781288595687,19.1699035489294,-234.859044174147));
#213806=CARTESIAN_POINT('Ctrl Pts',(48.1890852791867,18.9509743482895,-235.350050000003));
#213807=CARTESIAN_POINT('Ctrl Pts',(47.6106972731343,18.625565406903,-235.35005));
#213808=CARTESIAN_POINT('Ctrl Pts',(48.6248763884555,19.0947802943512,-234.853271204071));
#213809=CARTESIAN_POINT('Ctrl Pts',(48.2306061221348,18.8843051626248,-235.350049999998));
#213810=CARTESIAN_POINT('Ctrl Pts',(47.6410934853577,18.569620618322,-235.35005));
#213811=CARTESIAN_POINT('Ctrl Pts',(48.6396028929279,19.0702227963992,-234.851536427768));
#213812=CARTESIAN_POINT('Ctrl Pts',(48.2438148297685,18.8622892880126,-235.350049999998));
#213813=CARTESIAN_POINT('Ctrl Pts',(47.6510095952452,18.550861366784,-235.35005));
#213814=CARTESIAN_POINT('Ctrl Pts',(48.6656509039339,19.0245062658543,-234.849261045971));
#213815=CARTESIAN_POINT('Ctrl Pts',(48.267810580405,18.8200790514748,-235.350050000002));
#213816=CARTESIAN_POINT('Ctrl Pts',(47.6705745922183,18.513205530003,-235.35005));
#213817=CARTESIAN_POINT('Ctrl Pts',(48.6767455877554,19.0036730196651,-234.848826976569));
#213818=CARTESIAN_POINT('Ctrl Pts',(48.2784387534682,18.8000789112269,-235.350050000001));
#213819=CARTESIAN_POINT('Ctrl Pts',(47.6802441619202,18.4943195741576,-235.35005));
#213820=CARTESIAN_POINT('Ctrl Pts',(48.7115701984993,18.9389677368683,-234.84683711776));
#213821=CARTESIAN_POINT('Ctrl Pts',(48.3113401572838,18.738781310839,-235.350049999999));
#213822=CARTESIAN_POINT('Ctrl Pts',(47.7090490788398,18.4375569718045,-235.35005));
#213823=CARTESIAN_POINT('Ctrl Pts',(48.7350953123161,18.8948187861069,-234.845248112377));
#213824=CARTESIAN_POINT('Ctrl Pts',(48.3333974993269,18.6972683757834,-235.350050000006));
#213825=CARTESIAN_POINT('Ctrl Pts',(47.7279282401082,18.3995486637502,-235.35005));
#213826=CARTESIAN_POINT('Ctrl Pts',(48.7834587614873,18.8028811954349,-234.841054202938));
#213827=CARTESIAN_POINT('Ctrl Pts',(48.3781881568565,18.6119741954475,-235.350049999994));
#213828=CARTESIAN_POINT('Ctrl Pts',(47.7647487546851,18.3230500802882,-235.35005));
#213829=CARTESIAN_POINT('Ctrl Pts',(48.8085457779383,18.754824580439,-234.838353991562));
#213830=CARTESIAN_POINT('Ctrl Pts',(48.4011086067165,18.5680238025553,-235.350050000015));
#213831=CARTESIAN_POINT('Ctrl Pts',(47.7827001660699,18.2845649741211,-235.35005));
#213832=CARTESIAN_POINT('Ctrl Pts',(48.8608504474587,18.6521989438873,-234.831101974325));
#213833=CARTESIAN_POINT('Ctrl Pts',(48.4481394235988,18.4760651492002,-235.350049999984));
#213834=CARTESIAN_POINT('Ctrl Pts',(47.81709615277,18.2068203539689,-235.35005));
#213835=CARTESIAN_POINT('Ctrl Pts',(48.8859768835832,18.6002207271149,-234.827451251642));
#213836=CARTESIAN_POINT('Ctrl Pts',(48.4707622377245,18.4294985425077,-235.350049999999));
#213837=CARTESIAN_POINT('Ctrl Pts',(47.8335233281929,18.1675458631259,-235.35005));
#213838=CARTESIAN_POINT('Ctrl Pts',(48.9317590979678,18.4991718431838,-234.821404066159));
#213839=CARTESIAN_POINT('Ctrl Pts',(48.5125008275188,18.3376757598027,-235.350050000001));
#213840=CARTESIAN_POINT('Ctrl Pts',(47.8650504941538,18.0883394728593,-235.35005));
#213841=CARTESIAN_POINT('Ctrl Pts',(48.9515891654281,18.4514986637869,-234.819445110721));
#213842=CARTESIAN_POINT('Ctrl Pts',(48.5309876753933,18.2932822237603,-235.350050000003));
#213843=CARTESIAN_POINT('Ctrl Pts',(47.8801543850424,18.0485058523287,-235.35005));
#213844=CARTESIAN_POINT('Ctrl Pts',(48.9911458371249,18.3546372294721,-234.814928550212));
#213845=CARTESIAN_POINT('Ctrl Pts',(48.5677267083794,18.2034775571371,-235.350049999996));
#213846=CARTESIAN_POINT('Ctrl Pts',(47.9094666156693,17.9685258021276,-235.35005));
#213847=CARTESIAN_POINT('Ctrl Pts',(49.0112209584123,18.3047581611111,-234.812156424171));
#213848=CARTESIAN_POINT('Ctrl Pts',(48.5862296950314,18.1576503455933,-235.350050000007));
#213849=CARTESIAN_POINT('Ctrl Pts',(47.9236194657386,17.9283599903447,-235.35005));
#213850=CARTESIAN_POINT('Ctrl Pts',(49.0522465206321,18.2003746116001,-234.805011039778));
#213851=CARTESIAN_POINT('Ctrl Pts',(48.6236963620426,18.0631017745501,-235.350049999994));
#213852=CARTESIAN_POINT('Ctrl Pts',(47.9505381729848,17.8475439007782,-235.35005));
#213853=CARTESIAN_POINT('Ctrl Pts',(49.0738330944827,18.1446322248529,-234.800204572025));
#213854=CARTESIAN_POINT('Ctrl Pts',(48.6431636354573,18.013619351879,-235.350050000009));
#213855=CARTESIAN_POINT('Ctrl Pts',(47.9632560597789,17.8068666429648,-235.35005));
#213856=CARTESIAN_POINT('Ctrl Pts',(49.1128299645569,18.0356471582971,-234.79145959571));
#213857=CARTESIAN_POINT('Ctrl Pts',(48.6787156361984,17.9158184822153,-235.350049999991));
#213858=CARTESIAN_POINT('Ctrl Pts',(47.9870034052699,17.7249653914156,-235.35005));
#213859=CARTESIAN_POINT('Ctrl Pts',(49.1305989485082,17.9820590712204,-234.787374959526));
#213860=CARTESIAN_POINT('Ctrl Pts',(48.695062620387,17.8673394303137,-235.35005000001));
#213861=CARTESIAN_POINT('Ctrl Pts',(47.9980630400304,17.6838206475214,-235.35005));
#213862=CARTESIAN_POINT('Ctrl Pts',(49.1628022975924,17.8778595100161,-234.780195549906));
#213863=CARTESIAN_POINT('Ctrl Pts',(48.7249821608991,17.7719530069924,-235.35004999999));
#213864=CARTESIAN_POINT('Ctrl Pts',(48.0189197776842,17.6012300921137,-235.35005));
#213865=CARTESIAN_POINT('Ctrl Pts',(49.1780152194113,17.8259868345273,-234.776643381592));
#213866=CARTESIAN_POINT('Ctrl Pts',(48.7391768429728,17.7243103604292,-235.350049999995));
#213867=CARTESIAN_POINT('Ctrl Pts',(48.0287613458656,17.5597948840364,-235.35005));
#213868=CARTESIAN_POINT('Ctrl Pts',(49.2088831316691,17.7175974214052,-234.76777083952));
#213869=CARTESIAN_POINT('Ctrl Pts',(48.7678666087892,17.6260826000281,-235.350050000005));
#213870=CARTESIAN_POINT('Ctrl Pts',(48.0470227250193,17.4765854309817,-235.35005));
#213871=CARTESIAN_POINT('Ctrl Pts',(49.2241633474364,17.6616758881998,-234.762670691852));
#213872=CARTESIAN_POINT('Ctrl Pts',(48.7820703212585,17.575815576902,-235.350050000005));
#213873=CARTESIAN_POINT('Ctrl Pts',(48.0554329780656,17.4347916601489,-235.35005));
#213874=CARTESIAN_POINT('Ctrl Pts',(49.252818588968,17.5488204678451,-234.751966143146));
#213875=CARTESIAN_POINT('Ctrl Pts',(48.8088973471943,17.474458441837,-235.350049999995));
#213876=CARTESIAN_POINT('Ctrl Pts',(48.0705953135359,17.3508835165529,-235.35005));
#213877=CARTESIAN_POINT('Ctrl Pts',(49.2656967371983,17.493038371525,-234.746774003745));
#213878=CARTESIAN_POINT('Ctrl Pts',(48.8210830469464,17.4240853616799,-235.35005));
#213879=CARTESIAN_POINT('Ctrl Pts',(48.0773499548877,17.3088369763077,-235.350050000001));
#213880=CARTESIAN_POINT('Ctrl Pts',(49.2886686943366,17.3835528691795,-234.737089395268));
#213881=CARTESIAN_POINT('Ctrl Pts',(48.8430358085064,17.3244453325067,-235.35005));
#213882=CARTESIAN_POINT('Ctrl Pts',(48.0894592880343,17.2245872750773,-235.350050000001));
#213883=CARTESIAN_POINT('Ctrl Pts',(49.2982406085014,17.331247813801,-234.733146358298));
#213884=CARTESIAN_POINT('Ctrl Pts',(48.8522983790287,17.2760488789422,-235.350050000014));
#213885=CARTESIAN_POINT('Ctrl Pts',(48.094834615712,17.1823864227582,-235.35005));
#213886=CARTESIAN_POINT('Ctrl Pts',(49.3275288703794,17.1670149718797,-234.71835081978));
#213887=CARTESIAN_POINT('Ctrl Pts',(48.8808279281815,17.1260157446175,-235.350049999972));
#213888=CARTESIAN_POINT('Ctrl Pts',(48.1091464500575,17.0555809060241,-235.35005));
#213889=CARTESIAN_POINT('Ctrl Pts',(49.3473085304738,17.0432902293076,-234.703208934491));
#213890=CARTESIAN_POINT('Ctrl Pts',(48.9006204915337,17.0169034054434,-235.35004999989));
#213891=CARTESIAN_POINT('Ctrl Pts',(48.1154436500424,16.9706923807857,-235.350050000001));
#213892=CARTESIAN_POINT('Ctrl Pts',(49.3584215990167,16.9360371933353,-234.693305891908));
#213893=CARTESIAN_POINT('Ctrl Pts',(48.9123686178224,16.9178382234301,-235.350050000001));
#213894=CARTESIAN_POINT('Ctrl Pts',(48.1189208895433,16.8854655414009,-235.350050000001));
#213895=CARTESIAN_POINT('',(49.3576635057812,16.9360062631145,-234.694420988467));
#213896=CARTESIAN_POINT('',(48.1189208895436,16.8854655414,-235.35005));
#213897=CARTESIAN_POINT('Origin',(48.1189208895436,16.8854655414,-233.85005));
#213898=CARTESIAN_POINT('Ctrl Pts',(47.5004483343782,18.8074595529612,-235.35005));
#213899=CARTESIAN_POINT('Ctrl Pts',(47.523328218883,18.7715077674088,-235.35005));
#213900=CARTESIAN_POINT('Ctrl Pts',(47.5458232845143,18.7353572240715,-235.35005));
#213901=CARTESIAN_POINT('Ctrl Pts',(47.5676766302509,18.6988775607556,-235.35005));
#213902=CARTESIAN_POINT('Ctrl Pts',(47.5895300808456,18.6623977224007,-235.35005));
#213903=CARTESIAN_POINT('Ctrl Pts',(47.6106973144047,18.6255653312655,-235.35005));
#213904=CARTESIAN_POINT('Ctrl Pts',(47.6309614148883,18.58826888133,-235.35005));
#213905=CARTESIAN_POINT('Ctrl Pts',(47.6410934945813,18.5696206021569,-235.35005));
#213906=CARTESIAN_POINT('Ctrl Pts',(47.6510096037987,18.5508613513732,-235.35005));
#213907=CARTESIAN_POINT('Ctrl Pts',(47.6607920942703,18.5320334486734,-235.35005));
#213908=CARTESIAN_POINT('Ctrl Pts',(47.6705746000884,18.513205516437,-235.35005));
#213909=CARTESIAN_POINT('Ctrl Pts',(47.6802441693448,18.4943195614609,-235.35005));
#213910=CARTESIAN_POINT('Ctrl Pts',(47.6898458018307,18.4753987071822,-235.35005));
#213911=CARTESIAN_POINT('Ctrl Pts',(47.70904910136,18.4375569305264,-235.35005));
#213912=CARTESIAN_POINT('Ctrl Pts',(47.7279282587774,18.3995486292809,-235.35005));
#213913=CARTESIAN_POINT('Ctrl Pts',(47.7463384996528,18.3612993731052,-235.35005));
#213914=CARTESIAN_POINT('Ctrl Pts',(47.7647487677154,18.323050060445,-235.35005));
#213915=CARTESIAN_POINT('Ctrl Pts',(47.7827001759863,18.2845649614141,-235.35005));
#213916=CARTESIAN_POINT('Ctrl Pts',(47.7998981639292,18.24569266604,-235.35005));
#213917=CARTESIAN_POINT('Ctrl Pts',(47.8170961582275,18.2068203563009,-235.35005));
#213918=CARTESIAN_POINT('Ctrl Pts',(47.8335233318918,18.1675458731571,-235.35005));
#213919=CARTESIAN_POINT('Ctrl Pts',(47.8492869191686,18.127942671175,-235.35005));
#213920=CARTESIAN_POINT('Ctrl Pts',(47.8650504948173,18.0883394984066,-235.35005));
#213921=CARTESIAN_POINT('Ctrl Pts',(47.8801543852333,18.0485058859946,-235.35005));
#213922=CARTESIAN_POINT('Ctrl Pts',(47.8948105132744,18.0085158319627,-235.35005));
#213923=CARTESIAN_POINT('Ctrl Pts',(47.909466614277,17.9685258517065,-235.35005));
#213924=CARTESIAN_POINT('Ctrl Pts',(47.9236194654021,17.9283600484622,-235.35005));
#213925=CARTESIAN_POINT('Ctrl Pts',(47.9370788390041,17.887951952103,-235.35005));
#213926=CARTESIAN_POINT('Ctrl Pts',(47.9505379989423,17.847544497211,-235.35005));
#213927=CARTESIAN_POINT('Ctrl Pts',(47.9632559353684,17.8068671621608,-235.35005));
#213928=CARTESIAN_POINT('Ctrl Pts',(47.9751297575526,17.7659160244471,-235.35005));
#213929=CARTESIAN_POINT('Ctrl Pts',(47.9870033323709,17.7249657398638,-235.35005));
#213930=CARTESIAN_POINT('Ctrl Pts',(47.9980630011651,17.6838209125432,-235.35005));
#213931=CARTESIAN_POINT('Ctrl Pts',(48.0084914348375,17.6425253763784,-235.35005));
#213932=CARTESIAN_POINT('Ctrl Pts',(48.0189197816014,17.6012301843623,-235.35005));
#213933=CARTESIAN_POINT('Ctrl Pts',(48.0287613705984,17.5597948897797,-235.35005));
#213934=CARTESIAN_POINT('Ctrl Pts',(48.0378920589035,17.5181901626578,-235.35005));
#213935=CARTESIAN_POINT('Ctrl Pts',(48.0470227852353,17.4765852622638,-235.35005));
#213936=CARTESIAN_POINT('Ctrl Pts',(48.0554330459596,17.4347914019545,-235.35005));
#213937=CARTESIAN_POINT('Ctrl Pts',(48.063014164453,17.3928375917214,-235.35005));
#213938=CARTESIAN_POINT('Ctrl Pts',(48.0705954092764,17.3508830823798,-235.35005));
#213939=CARTESIAN_POINT('Ctrl Pts',(48.0773500452528,17.3088364520712,-235.350050000001));
#213940=CARTESIAN_POINT('Ctrl Pts',(48.0834046340598,17.2667121275033,-235.350050000001));
#213941=CARTESIAN_POINT('Ctrl Pts',(48.0894593994455,17.2245865744039,-235.350050000001));
#213942=CARTESIAN_POINT('Ctrl Pts',(48.0948347135637,17.1823856312802,-235.35005));
#213943=CARTESIAN_POINT('Ctrl Pts',(48.0996052337066,17.140117917919,-235.35005));
#213944=CARTESIAN_POINT('Ctrl Pts',(48.1091469299998,17.0555766788456,-235.35005));
#213945=CARTESIAN_POINT('Ctrl Pts',(48.115443852909,16.9706874085479,-235.350050000001));
#213946=CARTESIAN_POINT('Ctrl Pts',(48.1189208895436,16.885465541401,-235.350050000001));
#213947=CARTESIAN_POINT('Ctrl Pts',(49.3576635057812,16.9360062631145,-234.694420988467));
#213948=CARTESIAN_POINT('Ctrl Pts',(49.3471263105466,17.0376600850593,-234.703795085131));
#213949=CARTESIAN_POINT('Ctrl Pts',(49.3364864909818,17.1066695044026,-234.711288975797));
#213950=CARTESIAN_POINT('Ctrl Pts',(49.3237382757546,17.184198787297,-234.719709502799));
#213951=CARTESIAN_POINT('Ctrl Pts',(49.3199917485045,17.2054352035257,-234.722046293634));
#213952=CARTESIAN_POINT('Ctrl Pts',(49.3153257977579,17.231486737478,-234.724846402637));
#213953=CARTESIAN_POINT('Ctrl Pts',(49.3139282901745,17.2391949265268,-234.72566225943));
#213954=CARTESIAN_POINT('Ctrl Pts',(49.3120847413681,17.2493712815277,-234.726709775306));
#213955=CARTESIAN_POINT('Ctrl Pts',(49.3112260642013,17.2541124666259,-234.727189465917));
#213956=CARTESIAN_POINT('Ctrl Pts',(49.3103374053008,17.2590488483845,-234.727671987138));
#213957=CARTESIAN_POINT('Ctrl Pts',(49.3099810386723,17.2610379965402,-234.727862256699));
#213958=CARTESIAN_POINT('Ctrl Pts',(49.3097489286637,17.2623361089118,-234.727985430796));
#213959=CARTESIAN_POINT('Ctrl Pts',(49.309846238275,17.2617880108445,-234.727934861414));
#213960=CARTESIAN_POINT('Ctrl Pts',(49.2992464648262,17.3213294243835,-234.733486618467));
#213961=CARTESIAN_POINT('Ctrl Pts',(49.2884703228539,17.3767076195097,-234.738564343094));
#213962=CARTESIAN_POINT('Ctrl Pts',(49.2716034836387,17.4576229182381,-234.745722233989));
#213963=CARTESIAN_POINT('Ctrl Pts',(49.2658594168752,17.4841982801646,-234.74803174828));
#213964=CARTESIAN_POINT('Ctrl Pts',(49.2541192293622,17.536662236027,-234.75249787818));
#213965=CARTESIAN_POINT('Ctrl Pts',(49.2486124761573,17.5605060465331,-234.754488334413));
#213966=CARTESIAN_POINT('Ctrl Pts',(49.2287650942653,17.6434371614011,-234.761227311344));
#213967=CARTESIAN_POINT('Ctrl Pts',(49.2145175041624,17.6969874216763,-234.765957475731));
#213968=CARTESIAN_POINT('Ctrl Pts',(49.1974893808914,17.7556761004413,-234.771546112902));
#213969=CARTESIAN_POINT('Ctrl Pts',(49.1955835644542,17.7621753990853,-234.77217078373));
#213970=CARTESIAN_POINT('Ctrl Pts',(49.1917448889839,17.7751320132382,-234.77342754767));
#213971=CARTESIAN_POINT('Ctrl Pts',(49.1922453722157,17.7734577366325,-234.773256809092));
#213972=CARTESIAN_POINT('Ctrl Pts',(49.1903887257174,17.7799422846575,-234.773791614339));
#213973=CARTESIAN_POINT('Ctrl Pts',(49.1884660325305,17.7867464598314,-234.774315162155));
#213974=CARTESIAN_POINT('Ctrl Pts',(49.1805664619759,17.8144826479086,-234.776386838561));
#213975=CARTESIAN_POINT('Ctrl Pts',(49.1724695390079,17.8427478887243,-234.778436000106));
#213976=CARTESIAN_POINT('Ctrl Pts',(49.1555043287524,17.8989903998451,-234.782511808337));
#213977=CARTESIAN_POINT('Ctrl Pts',(49.1490482401721,17.9200399629343,-234.784037422065));
#213978=CARTESIAN_POINT('Ctrl Pts',(49.139870853538,17.949153615481,-234.786153202958));
#213979=CARTESIAN_POINT('Ctrl Pts',(49.1382049819289,17.9543986428311,-234.786534456923));
#213980=CARTESIAN_POINT('Ctrl Pts',(49.1360928848702,17.9610269698035,-234.787017684095));
#213981=CARTESIAN_POINT('Ctrl Pts',(49.1329147871453,17.97096000841,-234.787743929867));
#213982=CARTESIAN_POINT('Ctrl Pts',(49.1211497879488,18.0072816681923,-234.790422286177));
#213983=CARTESIAN_POINT('Ctrl Pts',(49.1012598894988,18.0662235069236,-234.794889351849));
#213984=CARTESIAN_POINT('Ctrl Pts',(49.0825174881958,18.1181924771152,-234.798979971364));
#213985=CARTESIAN_POINT('Ctrl Pts',(49.0680042665894,18.1571143825403,-234.802092896427));
#213986=CARTESIAN_POINT('Ctrl Pts',(49.0630898685875,18.1700799530162,-234.803138031519));
#213987=CARTESIAN_POINT('Ctrl Pts',(49.0555990686584,18.1895248967006,-234.804716974264));
#213988=CARTESIAN_POINT('Ctrl Pts',(49.0518243968624,18.1992458491427,-234.805509255663));
#213989=CARTESIAN_POINT('Ctrl Pts',(49.0480071657046,18.2089635528941,-234.806305752102));
#213990=CARTESIAN_POINT('Ctrl Pts',(49.0454530370347,18.215441192851,-234.806837686404));
#213991=CARTESIAN_POINT('Ctrl Pts',(49.0436037898865,18.2201082125008,-234.807221882863));
#213992=CARTESIAN_POINT('Ctrl Pts',(49.0371348733642,18.236392118303,-234.808564168568));
#213993=CARTESIAN_POINT('Ctrl Pts',(49.02932205209,18.2565451559845,-234.809914794572));
#213994=CARTESIAN_POINT('Ctrl Pts',(49.0141489881303,18.2952634232637,-234.812176958313));
#213995=CARTESIAN_POINT('Ctrl Pts',(49.00569672982,18.3167439603432,-234.813367096367));
#213996=CARTESIAN_POINT('Ctrl Pts',(48.9958664941424,18.3413881453924,-234.814645818696));
#213997=CARTESIAN_POINT('Ctrl Pts',(48.9889979076846,18.3585171481307,-234.815517985643));
#213998=CARTESIAN_POINT('Ctrl Pts',(48.9858598222626,18.3663118599993,-234.815908817181));
#213999=CARTESIAN_POINT('Ctrl Pts',(48.9648229823787,18.4182202217313,-234.818463134686));
#214000=CARTESIAN_POINT('Ctrl Pts',(48.9507413163091,18.4516566711652,-234.820134628404));
#214001=CARTESIAN_POINT('Ctrl Pts',(48.9343809176692,18.4899400549726,-234.822083928554));
#214002=CARTESIAN_POINT('Ctrl Pts',(48.9297104857026,18.5007288856637,-234.822640705199));
#214003=CARTESIAN_POINT('Ctrl Pts',(48.923937278621,18.5139601119533,-234.82333638506));
#214004=CARTESIAN_POINT('Ctrl Pts',(48.9213588397062,18.5198371515105,-234.823649353714));
#214005=CARTESIAN_POINT('Ctrl Pts',(48.9192525948475,18.5246043300423,-234.823910015452));
#214006=CARTESIAN_POINT('Ctrl Pts',(48.9179543035251,18.52753551139,-234.824072166185));
#214007=CARTESIAN_POINT('Ctrl Pts',(48.9181500023951,18.5271000257874,-234.824046111913));
#214008=CARTESIAN_POINT('Ctrl Pts',(48.8954594683543,18.5780343181537,-234.826949191156));
#214009=CARTESIAN_POINT('Ctrl Pts',(48.8729488554902,18.6261902513722,-234.829886574551));
#214010=CARTESIAN_POINT('Ctrl Pts',(48.8363463911418,18.7002781537299,-234.834600259925));
#214011=CARTESIAN_POINT('Ctrl Pts',(48.8236560944642,18.7253040017816,-234.836222756763));
#214012=CARTESIAN_POINT('Ctrl Pts',(48.8038443429534,18.7634090756344,-234.83873340459));
#214013=CARTESIAN_POINT('Ctrl Pts',(48.7937510442086,18.7825948905538,-234.840007954146));
#214014=CARTESIAN_POINT('Ctrl Pts',(48.7807985548326,18.8068120782162,-234.841637189171));
#214015=CARTESIAN_POINT('Ctrl Pts',(48.7746647465271,18.8181753396998,-234.842407311938));
#214016=CARTESIAN_POINT('Ctrl Pts',(48.7711382294178,18.8246834174458,-234.842849785296));
#214017=CARTESIAN_POINT('Ctrl Pts',(48.7694150713952,18.8278574582801,-234.843065921241));
#214018=CARTESIAN_POINT('Ctrl Pts',(48.7686422398806,18.8292800854102,-234.843162847327));
#214019=CARTESIAN_POINT('Ctrl Pts',(48.7622006952152,18.8418648134774,-234.843660628641));
#214020=CARTESIAN_POINT('Ctrl Pts',(48.7432200186877,18.8782325404045,-234.845017135759));
#214021=CARTESIAN_POINT('Ctrl Pts',(48.7353260165666,18.8932819489295,-234.845570943989));
#214022=CARTESIAN_POINT('Ctrl Pts',(48.7209372066814,18.9204072865677,-234.846554115121));
#214023=CARTESIAN_POINT('Ctrl Pts',(48.7131049616897,18.9351084395387,-234.847083815383));
#214024=CARTESIAN_POINT('Ctrl Pts',(48.7028006926672,18.9542924498671,-234.847768499741));
#214025=CARTESIAN_POINT('Ctrl Pts',(48.6981288815276,18.9629542167293,-234.848076228906));
#214026=CARTESIAN_POINT('Ctrl Pts',(48.694956886559,18.9688270098263,-234.848284557907));
#214027=CARTESIAN_POINT('Ctrl Pts',(48.6926764803002,18.9730416096279,-234.848433780606));
#214028=CARTESIAN_POINT('Ctrl Pts',(48.6760489926829,19.0037412762689,-234.849519581485));
#214029=CARTESIAN_POINT('Ctrl Pts',(48.6614284555105,19.0299997531886,-234.850656844783));
#214030=CARTESIAN_POINT('Ctrl Pts',(48.6408431073285,19.065833411723,-234.852535739319));
#214031=CARTESIAN_POINT('Ctrl Pts',(48.6341892896175,19.077205959928,-234.853190870762));
#214032=CARTESIAN_POINT('Ctrl Pts',(48.6245121798185,19.0934316734949,-234.854216817824));
#214033=CARTESIAN_POINT('Ctrl Pts',(48.6197504107073,19.1013350867889,-234.85474060383));
#214034=CARTESIAN_POINT('Ctrl Pts',(48.6151090556708,19.1089199751746,-234.855280608546));
#214035=CARTESIAN_POINT('Ctrl Pts',(48.6120425369725,19.1139047949247,-234.855644215849));
#214036=CARTESIAN_POINT('Ctrl Pts',(48.6117051735357,19.1144605947675,-234.855682204168));
#214037=CARTESIAN_POINT('Ctrl Pts',(48.5230305908126,19.2570495990898,-234.866606036447));
#214038=CARTESIAN_POINT('Ctrl Pts',(48.4379564955549,19.37902047629,-234.872226499439));
#214039=CARTESIAN_POINT('Ctrl Pts',(48.4260896922586,19.3965417854656,-234.872874618363));
#214040=CARTESIAN_POINT('Ctrl Pts',(49.357663505782,16.9360062631151,-234.694420988466));
#214041=CARTESIAN_POINT('Ctrl Pts',(48.9115061644421,16.9178030353144,-235.35005));
#214042=CARTESIAN_POINT('Ctrl Pts',(48.1189208895436,16.8854655414,-235.35005));
#214043=CARTESIAN_POINT('Ctrl Pts',(49.4635649335608,14.3752531202943,-234.692333873014));
#214044=CARTESIAN_POINT('Ctrl Pts',(49.0175817386228,14.3575637238871,-235.350050000391));
#214045=CARTESIAN_POINT('Ctrl Pts',(48.2232158057592,14.3292187542857,-235.35005));
#214046=CARTESIAN_POINT('Ctrl Pts',(49.5551530156078,11.8140213189959,-234.690527234957));
#214047=CARTESIAN_POINT('Ctrl Pts',(49.1092649251398,11.7982892962054,-235.350049999822));
#214048=CARTESIAN_POINT('Ctrl Pts',(48.3134219778347,11.7724738102799,-235.35005));
#214049=CARTESIAN_POINT('Ctrl Pts',(49.6324230235364,9.25223577675678,-234.689044294154));
#214050=CARTESIAN_POINT('Ctrl Pts',(49.1866080561977,9.23896306516062,-235.35005));
#214051=CARTESIAN_POINT('Ctrl Pts',(48.3895556141632,9.21523338364434,-235.35005));
#214052=CARTESIAN_POINT('',(49.6324231701066,9.25223524236281,-234.689044137434));
#214053=CARTESIAN_POINT('',(48.3895556141631,9.21523338364434,-235.35005));
#214054=CARTESIAN_POINT('Origin',(48.3895556141631,9.21523338364435,-233.85005));
#214055=CARTESIAN_POINT('Origin',(-648.115804222842,-11.5202125232578,-235.35005));
#214056=CARTESIAN_POINT('Origin',(-637.557461367465,-11.4839373498759,-249.18849675272));
#214057=CARTESIAN_POINT('Ctrl Pts',(49.6182572724309,9.33632588644485,-234.704271307837));
#214058=CARTESIAN_POINT('Ctrl Pts',(49.1716671980127,9.3093937125164,-235.35005));
#214059=CARTESIAN_POINT('Ctrl Pts',(48.3874683444157,9.26207687868008,-235.35005));
#214060=CARTESIAN_POINT('Ctrl Pts',(49.6801828044406,8.99887464788128,-234.643882192716));
#214061=CARTESIAN_POINT('Ctrl Pts',(49.2361268524121,9.02379200969491,-235.35005));
#214062=CARTESIAN_POINT('Ctrl Pts',(48.3986160847539,9.0744362502198,-235.35005));
#214063=CARTESIAN_POINT('Ctrl Pts',(49.6817690797009,8.67461962826136,-234.572387045798));
#214064=CARTESIAN_POINT('Ctrl Pts',(49.2558123914512,8.74313449703487,-235.35005));
#214065=CARTESIAN_POINT('Ctrl Pts',(48.3759406125794,8.88996799364191,-235.35005));
#214066=CARTESIAN_POINT('Ctrl Pts',(49.6381916686217,8.36177935226001,-234.492922371952));
#214067=CARTESIAN_POINT('Ctrl Pts',(49.2451518560708,8.46585266699427,-235.35005));
#214068=CARTESIAN_POINT('Ctrl Pts',(48.3280835873607,8.70872798446653,-235.35005));
#214069=CARTESIAN_POINT('',(49.648078203028,8.44024209172928,-234.512742084672));
#214070=CARTESIAN_POINT('',(48.3395182384274,8.75410525715259,-235.35005));
#214071=CARTESIAN_POINT('Origin',(48.3395182384273,8.75410525715261,-233.85005));
#214072=CARTESIAN_POINT('Ctrl Pts',(48.3895556141631,9.21523338364434,-235.35005));
#214073=CARTESIAN_POINT('Ctrl Pts',(48.3942007072891,9.05921010043768,-235.35005));
#214074=CARTESIAN_POINT('Ctrl Pts',(48.3758739100739,8.90567951512196,-235.35005));
#214075=CARTESIAN_POINT('Ctrl Pts',(48.3395182384274,8.75410525715259,-235.35005));
#214076=CARTESIAN_POINT('Ctrl Pts',(49.6480782611736,8.44024207778281,-234.512742114119));
#214077=CARTESIAN_POINT('Ctrl Pts',(49.6564789856231,8.51381412335654,-234.530999061222));
#214078=CARTESIAN_POINT('Ctrl Pts',(49.6621158262273,8.58669833526729,-234.548485647682));
#214079=CARTESIAN_POINT('Ctrl Pts',(49.6651766405904,8.65862169244825,-234.565154268152));
#214080=CARTESIAN_POINT('Ctrl Pts',(49.6682696610215,8.73130183140451,-234.581998276824));
#214081=CARTESIAN_POINT('Ctrl Pts',(49.6687327302347,8.80300040771396,-234.598007149397));
#214082=CARTESIAN_POINT('Ctrl Pts',(49.6667833420853,8.8734684012847,-234.613167697683));
#214083=CARTESIAN_POINT('Ctrl Pts',(49.6647943790958,8.94536697684644,-234.62863602268));
#214084=CARTESIAN_POINT('Ctrl Pts',(49.6602945997359,9.01598417424433,-234.643221410519));
#214085=CARTESIAN_POINT('Ctrl Pts',(49.6535306620587,9.08509487754269,-234.656944741809));
#214086=CARTESIAN_POINT('Ctrl Pts',(49.6479751661887,9.14185829628876,-234.668216269421));
#214087=CARTESIAN_POINT('Ctrl Pts',(49.6408926996888,9.19760616622859,-234.678906993986));
#214088=CARTESIAN_POINT('Ctrl Pts',(49.6324234200406,9.25223473081225,-234.689043900262));
#214089=CARTESIAN_POINT('Ctrl Pts',(49.6728514995601,8.43430012080101,-234.458282759328));
#214090=CARTESIAN_POINT('Ctrl Pts',(49.288180041945,8.52656505676208,-235.35005));
#214091=CARTESIAN_POINT('Ctrl Pts',(48.3395182384273,8.75410525715258,-235.35005));
#214092=CARTESIAN_POINT('Ctrl Pts',(49.4713806247164,7.68476869375633,-234.505836736672));
#214093=CARTESIAN_POINT('Ctrl Pts',(49.068969900047,7.76950806478782,-235.350049999891));
#214094=CARTESIAN_POINT('Ctrl Pts',(48.1420785222883,7.9309385499425,-235.35005));
#214095=CARTESIAN_POINT('Ctrl Pts',(49.3314010681958,6.92971336337434,-234.544835134207));
#214096=CARTESIAN_POINT('Ctrl Pts',(48.9137610316686,6.99112774713473,-235.350049999976));
#214097=CARTESIAN_POINT('Ctrl Pts',(48.0110562568883,7.10334135417386,-235.35005));
#214098=CARTESIAN_POINT('Ctrl Pts',(49.1759346319862,5.40665728715258,-234.609024663255));
#214099=CARTESIAN_POINT('Ctrl Pts',(48.7409159667592,5.4240408590254,-235.350050000024));
#214100=CARTESIAN_POINT('Ctrl Pts',(47.8801847113252,5.43950276679566,-235.35005));
#214101=CARTESIAN_POINT('Ctrl Pts',(49.160538186931,4.63912183635817,-234.634271526073));
#214102=CARTESIAN_POINT('Ctrl Pts',(48.7206281129052,4.63059369203667,-235.350049999964));
#214103=CARTESIAN_POINT('Ctrl Pts',(47.8802911702592,4.60324650202951,-235.35005));
#214104=CARTESIAN_POINT('Ctrl Pts',(49.2373009570426,3.47966794651993,-234.663512775955));
#214105=CARTESIAN_POINT('Ctrl Pts',(48.7965371406365,3.43220404512792,-235.350050000019));
#214106=CARTESIAN_POINT('Ctrl Pts',(47.9840461137012,3.34200714134957,-235.35005));
#214107=CARTESIAN_POINT('Ctrl Pts',(49.2797408095797,3.09195832251735,-234.67177735372));
#214108=CARTESIAN_POINT('Ctrl Pts',(48.8394590156831,3.03198770182503,-235.350050000024));
#214109=CARTESIAN_POINT('Ctrl Pts',(48.0360840389224,2.92068200690756,-235.35005));
#214110=CARTESIAN_POINT('Ctrl Pts',(49.3686674721625,2.51417204308171,-234.682003885727));
#214111=CARTESIAN_POINT('Ctrl Pts',(48.9303472051771,2.43544747989523,-235.350049999988));
#214112=CARTESIAN_POINT('Ctrl Pts',(48.1401430583213,2.2930545562818,-235.35005));
#214113=CARTESIAN_POINT('Ctrl Pts',(49.402536303351,2.3219777357236,-234.685058224348));
#214114=CARTESIAN_POINT('Ctrl Pts',(48.9650330207291,2.23711886664551,-235.350050000003));
#214115=CARTESIAN_POINT('Ctrl Pts',(48.1791846215008,2.08432209117866,-235.35005));
#214116=CARTESIAN_POINT('Ctrl Pts',(49.4454504350533,2.10627534599544,-234.688106940244));
#214117=CARTESIAN_POINT('Ctrl Pts',(49.0090909802763,2.01443249512216,-235.35005));
#214118=CARTESIAN_POINT('Ctrl Pts',(48.228072252525,1.85004158947422,-235.35005));
#214119=CARTESIAN_POINT('Ctrl Pts',(49.4500656799736,2.08312047683055,-234.688585004576));
#214120=CARTESIAN_POINT('Ctrl Pts',(49.0138826721794,1.99021267182542,-235.35005));
#214121=CARTESIAN_POINT('Ctrl Pts',(48.2336222089945,1.8240233376047,-235.35005));
#214122=CARTESIAN_POINT('Ctrl Pts',(49.4627554357834,2.02616414735994,-234.687594881843));
#214123=CARTESIAN_POINT('Ctrl Pts',(49.0262880889212,1.93508456875412,-235.35005));
#214124=CARTESIAN_POINT('Ctrl Pts',(48.2445959867496,1.77197302819215,-235.35005));
#214125=CARTESIAN_POINT('Ctrl Pts',(49.4690104939933,1.99767348243289,-234.687098899761));
#214126=CARTESIAN_POINT('Ctrl Pts',(49.0324043256687,1.90750833138808,-235.350049999998));
#214127=CARTESIAN_POINT('Ctrl Pts',(48.2500003143967,1.7459388370457,-235.35005));
#214128=CARTESIAN_POINT('Ctrl Pts',(49.4875062569173,1.91216482959672,-234.68560826925));
#214129=CARTESIAN_POINT('Ctrl Pts',(49.0504957719995,1.82473476843569,-235.350050000004));
#214130=CARTESIAN_POINT('Ctrl Pts',(48.2659659469638,1.66780919078281,-235.35005));
#214131=CARTESIAN_POINT('Ctrl Pts',(49.4994778206697,1.85510901473098,-234.684610917049));
#214132=CARTESIAN_POINT('Ctrl Pts',(49.0622098134495,1.76950945951608,-235.350049999996));
#214133=CARTESIAN_POINT('Ctrl Pts',(48.2762799057323,1.61568666327167,-235.35005));
#214134=CARTESIAN_POINT('Ctrl Pts',(49.5343162437143,1.68379702048753,-234.681608641634));
#214135=CARTESIAN_POINT('Ctrl Pts',(49.0963241847283,1.60365506175308,-235.350050000008));
#214136=CARTESIAN_POINT('Ctrl Pts',(48.3062349042401,1.45921106566498,-235.35005));
#214137=CARTESIAN_POINT('Ctrl Pts',(49.5561079504651,1.56939161413912,-234.679593431468));
#214138=CARTESIAN_POINT('Ctrl Pts',(49.1176811340418,1.49291506667449,-235.35005));
#214139=CARTESIAN_POINT('Ctrl Pts',(48.3248891349689,1.35474998793845,-235.35005));
#214140=CARTESIAN_POINT('Ctrl Pts',(49.739315938348,0.538232976929953,-234.661348160278));
#214141=CARTESIAN_POINT('Ctrl Pts',(49.2980430840322,0.491601823769887,
-235.35005));
#214142=CARTESIAN_POINT('Ctrl Pts',(48.4809881192922,0.413309956198443,
-235.35005));
#214143=CARTESIAN_POINT('Ctrl Pts',(49.8115904444898,-0.39039417120445,
-234.644373027974));
#214144=CARTESIAN_POINT('Ctrl Pts',(49.3700829143943,-0.408162802666101,
-235.350050000012));
#214145=CARTESIAN_POINT('Ctrl Pts',(48.536801379512,-0.432603676106494,
-235.35005));
#214146=CARTESIAN_POINT('Ctrl Pts',(49.7792929465182,-1.80244463166521,
-234.617637729134));
#214147=CARTESIAN_POINT('Ctrl Pts',(49.3437540436927,-1.77379230904932,
-235.350049999994));
#214148=CARTESIAN_POINT('Ctrl Pts',(48.4927543039942,-1.71545839400357,
-235.35005));
#214149=CARTESIAN_POINT('Ctrl Pts',(49.7449472191672,-2.27243042723951,
-234.608607167038));
#214150=CARTESIAN_POINT('Ctrl Pts',(49.3121506898382,-2.22946376902224,
-235.350050000025));
#214151=CARTESIAN_POINT('Ctrl Pts',(48.4566916340738,-2.14207645769056,
-235.35005));
#214152=CARTESIAN_POINT('Ctrl Pts',(49.6724929766268,-2.85744653353658,
-234.597143764557));
#214153=CARTESIAN_POINT('Ctrl Pts',(49.2444209800414,-2.79595881961922,
-235.350049999994));
#214154=CARTESIAN_POINT('Ctrl Pts',(48.3849699272127,-2.67235166449409,
-235.35005));
#214155=CARTESIAN_POINT('Ctrl Pts',(49.6565229498012,-2.97433640738121,
-234.594843523884));
#214156=CARTESIAN_POINT('Ctrl Pts',(49.2294260564386,-2.90934026363395,
-235.350050000001));
#214157=CARTESIAN_POINT('Ctrl Pts',(48.3692885871419,-2.77828474965782,
-235.35005));
#214158=CARTESIAN_POINT('Ctrl Pts',(49.6303369251514,-3.14951121338623,
-234.59138274778));
#214159=CARTESIAN_POINT('Ctrl Pts',(49.2047903648279,-3.0792350757591,-235.350049999999));
#214160=CARTESIAN_POINT('Ctrl Pts',(48.3437536505604,-2.93700076554913,
-235.35005));
#214161=CARTESIAN_POINT('Ctrl Pts',(49.6212366617497,-3.2078747034095,-234.59022744472));
#214162=CARTESIAN_POINT('Ctrl Pts',(49.1962176139895,-3.13585840403236,
-235.350049999997));
#214163=CARTESIAN_POINT('Ctrl Pts',(48.3349064994216,-2.98987550056776,
-235.35005));
#214164=CARTESIAN_POINT('Ctrl Pts',(49.6093954409355,-3.28079495618834,
-234.588781243175));
#214165=CARTESIAN_POINT('Ctrl Pts',(49.1850545500923,-3.20659554539805,
-235.350050000001));
#214166=CARTESIAN_POINT('Ctrl Pts',(48.3234272698566,-3.05593058196302,
-235.35005));
#214167=CARTESIAN_POINT('Ctrl Pts',(49.6070039394402,-3.29537707660664,
-234.588491903602));
#214168=CARTESIAN_POINT('Ctrl Pts',(49.1827990425974,-3.22074419373563,
-235.350049999999));
#214169=CARTESIAN_POINT('Ctrl Pts',(48.3211104090697,-3.06913968133917,
-235.35005));
#214170=CARTESIAN_POINT('Ctrl Pts',(49.6021743356584,-3.32453778941096,
-234.587913021195));
#214171=CARTESIAN_POINT('Ctrl Pts',(49.1782430572807,-3.24903860274526,
-235.350050000001));
#214172=CARTESIAN_POINT('Ctrl Pts',(48.3164346335911,-3.09555404408755,
-235.35005));
#214173=CARTESIAN_POINT('Ctrl Pts',(49.5996474515442,-3.34085732030391,
-234.587220155499));
#214174=CARTESIAN_POINT('Ctrl Pts',(49.1760365449187,-3.26437756035475,
-235.350049999999));
#214175=CARTESIAN_POINT('Ctrl Pts',(48.3140690695237,-3.10875870092911,
-235.35005));
#214176=CARTESIAN_POINT('Ctrl Pts',(49.5926419005652,-3.37705346105833,
-234.588096930775));
#214177=CARTESIAN_POINT('Ctrl Pts',(49.1686572417052,-3.30163648990395,
-235.350050000002));
#214178=CARTESIAN_POINT('Ctrl Pts',(48.3069527703726,-3.14837088297125,
-235.35005));
#214179=CARTESIAN_POINT('Ctrl Pts',(49.5880379342478,-3.40119213175464,
-234.588675003203));
#214180=CARTESIAN_POINT('Ctrl Pts',(49.1638073722724,-3.32648654991977,
-235.350050000001));
#214181=CARTESIAN_POINT('Ctrl Pts',(48.3022780138372,-3.17478533866626,
-235.35005));
#214182=CARTESIAN_POINT('Ctrl Pts',(49.5471968352223,-3.61852378247012,
-234.593820523271));
#214183=CARTESIAN_POINT('Ctrl Pts',(49.120825236928,-3.55002422886253,-235.350049999991));
#214184=CARTESIAN_POINT('Ctrl Pts',(48.260829396598,-3.41257237641022,-235.35005));
#214185=CARTESIAN_POINT('Ctrl Pts',(49.5151390838467,-3.81220065571331,
-234.597986435595));
#214186=CARTESIAN_POINT('Ctrl Pts',(49.0870435716996,-3.7495062197225,-235.350049999982));
#214187=CARTESIAN_POINT('Ctrl Pts',(48.2284220495721,-3.6243432560285,-235.35005));
#214188=CARTESIAN_POINT('Ctrl Pts',(49.4316520932394,-4.39464147120427,
-234.609338953161));
#214189=CARTESIAN_POINT('Ctrl Pts',(48.999140659104,-4.34892292208159,-235.350050000037));
#214190=CARTESIAN_POINT('Ctrl Pts',(48.144430583747,-4.26086274000263,-235.35005));
#214191=CARTESIAN_POINT('Ctrl Pts',(49.3929212943256,-4.78464839371361,
-234.615391792126));
#214192=CARTESIAN_POINT('Ctrl Pts',(48.9581797211666,-4.75113501141927,
-235.350050000025));
#214193=CARTESIAN_POINT('Ctrl Pts',(48.1060703916391,-4.68681758304716,
-235.35005));
#214194=CARTESIAN_POINT('Ctrl Pts',(49.3496141347373,-5.56823512928163,
-234.624590481152));
#214195=CARTESIAN_POINT('Ctrl Pts',(48.9121267106381,-5.55882828684355,
-235.350049999975));
#214196=CARTESIAN_POINT('Ctrl Pts',(48.0648194622892,-5.541962664716,-235.35005));
#214197=CARTESIAN_POINT('Ctrl Pts',(49.3450624937163,-5.96264728287436,
-234.62775835361));
#214198=CARTESIAN_POINT('Ctrl Pts',(48.9069479295888,-5.96574880666937,
-235.350049999988));
#214199=CARTESIAN_POINT('Ctrl Pts',(48.0619566741598,-5.9722387873912,-235.35005));
#214200=CARTESIAN_POINT('Ctrl Pts',(49.3836522966543,-7.14335361784636,
-234.632954449768));
#214201=CARTESIAN_POINT('Ctrl Pts',(48.9459771364325,-7.18265905055676,
-235.350050000025));
#214202=CARTESIAN_POINT('Ctrl Pts',(48.10749380005,-7.25998633045287,-235.35005));
#214203=CARTESIAN_POINT('Ctrl Pts',(49.4781295444162,-7.92288565097549,
-234.630793193489));
#214204=CARTESIAN_POINT('Ctrl Pts',(49.0440042562222,-7.98854641142163,
-235.350050000012));
#214205=CARTESIAN_POINT('Ctrl Pts',(48.2090347928457,-8.11012177193449,
-235.35005));
#214206=CARTESIAN_POINT('Ctrl Pts',(49.6436637931067,-8.70555907873261,
-234.622711430443));
#214207=CARTESIAN_POINT('Ctrl Pts',(49.215549750052,-8.79378133618202,-235.35005));
#214208=CARTESIAN_POINT('Ctrl Pts',(48.3844338019353,-8.96504977313631,
-235.35005));
#214209=CARTESIAN_POINT('Ctrl Pts',(49.6467830757905,-8.72126520645183,
-234.622881194422));
#214210=CARTESIAN_POINT('Ctrl Pts',(49.2184641679714,-8.80863139937438,
-235.350050000001));
#214211=CARTESIAN_POINT('Ctrl Pts',(48.3871335037843,-8.97820236411209,
-235.35005));
#214212=CARTESIAN_POINT('Ctrl Pts',(49.652570743989,-8.75022091862852,-234.623023249691));
#214213=CARTESIAN_POINT('Ctrl Pts',(49.2240471314743,-8.83669877294023,
-235.35005));
#214214=CARTESIAN_POINT('Ctrl Pts',(48.392472005857,-9.00451470107218,-235.35005));
#214215=CARTESIAN_POINT('Ctrl Pts',(49.6554415168799,-8.76470121725064,
-234.623094268857));
#214216=CARTESIAN_POINT('Ctrl Pts',(49.2268162733382,-8.85073482443769,
-235.35005));
#214217=CARTESIAN_POINT('Ctrl Pts',(48.3951203393894,-9.01767332704875,
-235.35005));
#214218=CARTESIAN_POINT('Ctrl Pts',(49.6639847413244,-8.80814953817889,
-234.623307303822));
#214219=CARTESIAN_POINT('Ctrl Pts',(49.2350566242746,-8.89284947000431,
-235.35005));
#214220=CARTESIAN_POINT('Ctrl Pts',(48.4030026471238,-9.05715657045287,
-235.35005));
#214221=CARTESIAN_POINT('Ctrl Pts',(49.6695880826123,-8.83712489848571,
-234.62344929667));
#214222=CARTESIAN_POINT('Ctrl Pts',(49.2404610175429,-8.9209358282925,-235.350049999998));
#214223=CARTESIAN_POINT('Ctrl Pts',(48.4081739296747,-9.08348855318983,
-235.35005));
#214224=CARTESIAN_POINT('Ctrl Pts',(49.6861223185908,-8.92408111445968,
-234.623875207675));
#214225=CARTESIAN_POINT('Ctrl Pts',(49.256406444972,-9.00522113980889,-235.350050000003));
#214226=CARTESIAN_POINT('Ctrl Pts',(48.4234374397461,-9.16251391233196,
-235.35005));
#214227=CARTESIAN_POINT('Ctrl Pts',(49.6967773806612,-8.98209175593384,
-234.62415905619));
#214228=CARTESIAN_POINT('Ctrl Pts',(49.2666807798315,-9.06145141914929,
-235.350050000001));
#214229=CARTESIAN_POINT('Ctrl Pts',(48.4332793497998,-9.21523669725127,
-235.35005));
#214230=CARTESIAN_POINT('Ctrl Pts',(49.7276432253153,-9.15624775774307,
-234.625010528257));
#214231=CARTESIAN_POINT('Ctrl Pts',(49.2964363024444,-9.23024944441461,
-235.350049999999));
#214232=CARTESIAN_POINT('Ctrl Pts',(48.4618064955616,-9.37352237066705,
-235.35005));
#214233=CARTESIAN_POINT('Ctrl Pts',(49.7467547873477,-9.27251577845205,
-234.625578064603));
#214234=CARTESIAN_POINT('Ctrl Pts',(49.314854493951,-9.34294468497894,-235.350049999993));
#214235=CARTESIAN_POINT('Ctrl Pts',(48.4794934628256,-9.47920254067735,
-235.35005));
#214236=CARTESIAN_POINT('Ctrl Pts',(49.7997084497685,-9.62184541811456,
-234.627282202282));
#214237=CARTESIAN_POINT('Ctrl Pts',(49.3658541559959,-9.68147807603859,
-235.350050000013));
#214238=CARTESIAN_POINT('Ctrl Pts',(48.5285710814135,-9.79671102654565,
-235.35005));
#214239=CARTESIAN_POINT('Ctrl Pts',(49.8291648925442,-9.85534471123291,
-234.628414215299));
#214240=CARTESIAN_POINT('Ctrl Pts',(49.3941985373055,-9.90779071015971,
-235.350049999984));
#214241=CARTESIAN_POINT('Ctrl Pts',(48.5559827004535,-10.0090068188063,
-235.35005));
#214242=CARTESIAN_POINT('Ctrl Pts',(49.9000611961947,-10.5579169022257,
-234.631809953743));
#214243=CARTESIAN_POINT('Ctrl Pts',(49.46227163692,-10.5884986518548,-235.350050000031));
#214244=CARTESIAN_POINT('Ctrl Pts',(48.6223270802844,-10.6477610876399,
-235.35005));
#214245=CARTESIAN_POINT('Ctrl Pts',(49.9239345979392,-11.0302498028062,
-234.634065686046));
#214246=CARTESIAN_POINT('Ctrl Pts',(49.4850280286859,-11.0462297011433,
-235.350050000012));
#214247=CARTESIAN_POINT('Ctrl Pts',(48.6453046118701,-11.0773736644593,
-235.35005));
#214248=CARTESIAN_POINT('Ctrl Pts',(49.9251475272435,-12.4365683292309,
-234.640718339231));
#214249=CARTESIAN_POINT('Ctrl Pts',(49.4850454762624,-12.4082162297068,
-235.350049999975));
#214250=CARTESIAN_POINT('Ctrl Pts',(48.6501328458788,-12.3566962654659,
-235.35005));
#214251=CARTESIAN_POINT('Ctrl Pts',(49.8337365726491,-13.3641675740085,
-234.645001156777));
#214252=CARTESIAN_POINT('Ctrl Pts',(49.3959235241511,-13.306961117108,-235.350050000025));
#214253=CARTESIAN_POINT('Ctrl Pts',(48.5694097707421,-13.2010981453996,
-235.35005));
#214254=CARTESIAN_POINT('Ctrl Pts',(49.6449074151748,-14.31060701528,-234.649307954722));
#214255=CARTESIAN_POINT('Ctrl Pts',(49.2121335792871,-14.2245954491116,
-235.35005));
#214256=CARTESIAN_POINT('Ctrl Pts',(48.3999288819756,-14.0631760578291,
-235.35005));
#214257=CARTESIAN_POINT('Ctrl Pts',(49.6390944562837,-14.3392793335432,
-234.649438390436));
#214258=CARTESIAN_POINT('Ctrl Pts',(49.2064813038673,-14.2523696378793,
-235.350050000001));
#214259=CARTESIAN_POINT('Ctrl Pts',(48.3947106332052,-14.089291300339,-235.35005));
#214260=CARTESIAN_POINT('Ctrl Pts',(49.630238868934,-14.3822740481529,-234.649633936839));
#214261=CARTESIAN_POINT('Ctrl Pts',(49.1978709982769,-14.2940177686488,
-235.35005));
#214262=CARTESIAN_POINT('Ctrl Pts',(48.3867592982998,-14.1284516414382,
-235.35005));
#214263=CARTESIAN_POINT('Ctrl Pts',(49.6270184598194,-14.3976658139417,
-234.64972527904));
#214264=CARTESIAN_POINT('Ctrl Pts',(49.1948058416811,-14.3085889178777,
-235.35005));
#214265=CARTESIAN_POINT('Ctrl Pts',(48.3840780941576,-14.1415019811602,
-235.35005));
#214266=CARTESIAN_POINT('Ctrl Pts',(49.6220964416629,-14.4216069388598,
-234.649740099044));
#214267=CARTESIAN_POINT('Ctrl Pts',(49.189727776354,-14.3332801597934,-235.35005));
#214268=CARTESIAN_POINT('Ctrl Pts',(48.3787223515611,-14.1676033339819,
-235.35005));
#214269=CARTESIAN_POINT('Ctrl Pts',(49.6196521598081,-14.4335794112836,
-234.649746149776));
#214270=CARTESIAN_POINT('Ctrl Pts',(49.1872061637321,-14.3456277485269,
-235.350050000002));
#214271=CARTESIAN_POINT('Ctrl Pts',(48.3760618298762,-14.1806557630565,
-235.35005));
#214272=CARTESIAN_POINT('Ctrl Pts',(49.607514313622,-14.4934512680602,-234.649769617566));
#214273=CARTESIAN_POINT('Ctrl Pts',(49.1746851770632,-14.4073752083641,
-235.350049999995));
#214274=CARTESIAN_POINT('Ctrl Pts',(48.3628458825965,-14.2459266629983,
-235.35005));
#214275=CARTESIAN_POINT('Ctrl Pts',(49.5980714456629,-14.5413790514639,
-234.649766679825));
#214276=CARTESIAN_POINT('Ctrl Pts',(49.1649467606461,-14.4568049215079,
-235.35005));
#214277=CARTESIAN_POINT('Ctrl Pts',(48.3525504293568,-14.2981713963959,
-235.35005));
#214278=CARTESIAN_POINT('Ctrl Pts',(49.5705425974965,-14.685250739817,-234.64969306114));
#214279=CARTESIAN_POINT('Ctrl Pts',(49.1365644714732,-14.6051843071834,
-235.35005));
#214280=CARTESIAN_POINT('Ctrl Pts',(48.3224929218234,-14.4549893276864,
-235.35005));
#214281=CARTESIAN_POINT('Ctrl Pts',(49.5532562934944,-14.7812827163161,
-234.6495576116));
#214282=CARTESIAN_POINT('Ctrl Pts',(49.1187527743078,-14.7042280745193,
-235.350049999998));
#214283=CARTESIAN_POINT('Ctrl Pts',(48.3035595793916,-14.5596462424765,
-235.35005));
#214284=CARTESIAN_POINT('Ctrl Pts',(49.504581004737,-15.0697105777159,-234.648893466985));
#214285=CARTESIAN_POINT('Ctrl Pts',(49.0686321333853,-15.0017055627095,
-235.350050000003));
#214286=CARTESIAN_POINT('Ctrl Pts',(48.2500551817889,-14.8739499130376,
-235.35005));
#214287=CARTESIAN_POINT('Ctrl Pts',(49.4763738065104,-15.2624371474016,
-234.648107556722));
#214288=CARTESIAN_POINT('Ctrl Pts',(49.0396350389957,-15.2005009431667,
-235.350049999997));
#214289=CARTESIAN_POINT('Ctrl Pts',(48.2187775910813,-15.0839293763448,
-235.35005));
#214290=CARTESIAN_POINT('Ctrl Pts',(49.4044293239341,-15.8417822433236,
-234.644710178708));
#214291=CARTESIAN_POINT('Ctrl Pts',(48.9658409312175,-15.7981630905825,
-235.350050000006));
#214292=CARTESIAN_POINT('Ctrl Pts',(48.1380456036249,-15.7151912142403,
-235.35005));
#214293=CARTESIAN_POINT('Ctrl Pts',(49.3734327825549,-16.2296028510151,
-234.641058717396));
#214294=CARTESIAN_POINT('Ctrl Pts',(48.9343435468517,-16.1983923951185,
-235.350049999994));
#214295=CARTESIAN_POINT('Ctrl Pts',(48.1017687499515,-16.1377801895033,
-235.35005));
#214296=CARTESIAN_POINT('Ctrl Pts',(49.3308420035029,-17.3903901931505,
-234.625952625488));
#214297=CARTESIAN_POINT('Ctrl Pts',(48.8924366678536,-17.3966762449269,
-235.350050000012));
#214298=CARTESIAN_POINT('Ctrl Pts',(48.0452056587669,-17.4030250963116,
-235.35005));
#214299=CARTESIAN_POINT('Ctrl Pts',(49.3691048094434,-18.1627182776333,
-234.610348160686));
#214300=CARTESIAN_POINT('Ctrl Pts',(48.9347737531675,-18.1950555866989,
-235.350049999926));
#214301=CARTESIAN_POINT('Ctrl Pts',(48.0765553834797,-18.2457723122435,
-235.35005));
#214302=CARTESIAN_POINT('Ctrl Pts',(49.4996796913378,-19.1255806819443,
-234.582794859548));
#214303=CARTESIAN_POINT('Ctrl Pts',(49.073878318193,-19.1825305851387,-235.350050000018));
#214304=CARTESIAN_POINT('Ctrl Pts',(48.202136382695,-19.2982688285888,-235.35005));
#214305=CARTESIAN_POINT('Ctrl Pts',(49.52991658873,-19.3178023825667,-234.576884907736));
#214306=CARTESIAN_POINT('Ctrl Pts',(49.1061840742319,-19.3803813622115,
-235.350049999994));
#214307=CARTESIAN_POINT('Ctrl Pts',(48.2315724527526,-19.5085474359625,
-235.35005));
#214308=CARTESIAN_POINT('Ctrl Pts',(49.5728750024147,-19.557581971237,-234.568958963022));
#214309=CARTESIAN_POINT('Ctrl Pts',(49.1519829044983,-19.6267561009081,
-235.350050000002));
#214310=CARTESIAN_POINT('Ctrl Pts',(48.2737849902378,-19.7710257016811,
-235.35005));
#214311=CARTESIAN_POINT('Ctrl Pts',(49.581724296076,-19.6055101274536,-234.567346909248));
#214312=CARTESIAN_POINT('Ctrl Pts',(49.1614271182939,-19.6760521531559,
-235.350049999999));
#214313=CARTESIAN_POINT('Ctrl Pts',(48.2824987027496,-19.82350433647,-235.35005));
#214314=CARTESIAN_POINT('Ctrl Pts',(49.5953862717011,-19.6773655259788,
-234.564887454911));
#214315=CARTESIAN_POINT('Ctrl Pts',(49.1760035146459,-19.749934845904,-235.35005));
#214316=CARTESIAN_POINT('Ctrl Pts',(48.2959770869867,-19.9021966978926,
-235.35005));
#214317=CARTESIAN_POINT('Ctrl Pts',(49.6000048505966,-19.7013107519912,
-234.564060755941));
#214318=CARTESIAN_POINT('Ctrl Pts',(49.1809320849687,-19.7745590177076,
-235.350050000005));
#214319=CARTESIAN_POINT('Ctrl Pts',(48.3005378529525,-19.9284232197851,
-235.35005));
#214320=CARTESIAN_POINT('Ctrl Pts',(49.6070298089383,-19.737219250395,-234.562810247899));
#214321=CARTESIAN_POINT('Ctrl Pts',(49.1884276543306,-19.8114797947251,
-235.350049999998));
#214322=CARTESIAN_POINT('Ctrl Pts',(48.3074811028276,-19.9677565956903,
-235.35005));
#214323=CARTESIAN_POINT('Ctrl Pts',(49.609387621656,-19.7491870845315,-234.56239167244));
#214324=CARTESIAN_POINT('Ctrl Pts',(49.1909436535833,-19.823785851781,-235.350050000001));
#214325=CARTESIAN_POINT('Ctrl Pts',(48.3098125363869,-19.9808666531709,
-235.35005));
#214326=CARTESIAN_POINT('Ctrl Pts',(49.6141356106853,-19.773119545442,-234.561551017751));
#214327=CARTESIAN_POINT('Ctrl Pts',(49.1960101574545,-19.8483939155015,
-235.350049999999));
#214328=CARTESIAN_POINT('Ctrl Pts',(48.3145094629338,-20.0070846308637,
-235.35005));
#214329=CARTESIAN_POINT('Ctrl Pts',(49.616496536379,-19.7880921888268,-234.562161061286));
#214330=CARTESIAN_POINT('Ctrl Pts',(49.1981273776604,-19.8628075510617,
-235.35005));
#214331=CARTESIAN_POINT('Ctrl Pts',(48.3168699427918,-20.0201928656617,
-235.35005));
#214332=CARTESIAN_POINT('Ctrl Pts',(49.6374531557859,-19.9187122192786,
-234.566228111255));
#214333=CARTESIAN_POINT('Ctrl Pts',(49.2174467664976,-19.9895567213893,
-235.350050000002));
#214334=CARTESIAN_POINT('Ctrl Pts',(48.3378149961279,-20.1381857579918,
-235.35005));
#214335=CARTESIAN_POINT('Ctrl Pts',(49.6545821021411,-20.034869144394,-234.569823849718));
#214336=CARTESIAN_POINT('Ctrl Pts',(49.233200304514,-20.1023267809174,-235.350049999994));
#214337=CARTESIAN_POINT('Ctrl Pts',(48.3550896009133,-20.2431526171789,
-235.35005));
#214338=CARTESIAN_POINT('Ctrl Pts',(49.732804356096,-20.6159835232779,-234.587701863422));
#214339=CARTESIAN_POINT('Ctrl Pts',(49.3046815018901,-20.6649638076766,
-235.350050000025));
#214340=CARTESIAN_POINT('Ctrl Pts',(48.4347895563001,-20.7684056538746,
-235.35005));
#214341=CARTESIAN_POINT('Ctrl Pts',(49.771626989824,-21.0814436674373,-234.601632242406));
#214342=CARTESIAN_POINT('Ctrl Pts',(49.3394667389117,-21.1164600076538,
-235.35005));
#214343=CARTESIAN_POINT('Ctrl Pts',(48.4772403630273,-21.1899452510999,
-235.35005));
#214344=CARTESIAN_POINT('Ctrl Pts',(49.8182862151745,-22.480135809816,-234.642440475715));
#214345=CARTESIAN_POINT('Ctrl Pts',(49.3766026048063,-22.4678952988485,
-235.35005));
#214346=CARTESIAN_POINT('Ctrl Pts',(48.5415386498259,-22.458520743411,-235.35005));
#214347=CARTESIAN_POINT('Ctrl Pts',(49.7563614221941,-23.4171717990893,
-234.66832058589));
#214348=CARTESIAN_POINT('Ctrl Pts',(49.3136320941011,-23.3756815703655,
-235.35005));
#214349=CARTESIAN_POINT('Ctrl Pts',(48.5005032094983,-23.311667738302,-235.35005));
#214350=CARTESIAN_POINT('Ctrl Pts',(49.5587507160758,-24.5837933660124,
-234.698831294804));
#214351=CARTESIAN_POINT('Ctrl Pts',(49.1180235882351,-24.5091016284394,
-235.35005));
#214352=CARTESIAN_POINT('Ctrl Pts',(48.3390590324706,-24.3778343529881,
-235.35005));
#214353=CARTESIAN_POINT('Ctrl Pts',(49.5131812962588,-24.8168855068945,
-234.704842968893));
#214354=CARTESIAN_POINT('Ctrl Pts',(49.0732932499469,-24.7346294445711,
-235.350050000019));
#214355=CARTESIAN_POINT('Ctrl Pts',(48.3012455308433,-24.5909867391319,
-235.35005));
#214356=CARTESIAN_POINT('Ctrl Pts',(49.4550136911697,-25.0787190925436,
-234.711486940524));
#214357=CARTESIAN_POINT('Ctrl Pts',(49.0162880925532,-24.9882356999008,
-235.350049999998));
#214358=CARTESIAN_POINT('Ctrl Pts',(48.2523434883265,-24.8306899717521,
-235.35005));
#214359=CARTESIAN_POINT('Ctrl Pts',(49.4484542084783,-25.1078085522158,
-234.712223559563));
#214360=CARTESIAN_POINT('Ctrl Pts',(49.0098690957564,-25.016379242205,-235.350049999997));
#214361=CARTESIAN_POINT('Ctrl Pts',(48.2468215385715,-24.857322369352,-235.35005));
#214362=CARTESIAN_POINT('Ctrl Pts',(49.4351429030966,-25.1659768335314,
-234.713693433566));
#214363=CARTESIAN_POINT('Ctrl Pts',(48.9968469574703,-25.0726559928153,
-235.350050000003));
#214364=CARTESIAN_POINT('Ctrl Pts',(48.2356002982336,-24.910584566504,-235.35005));
#214365=CARTESIAN_POINT('Ctrl Pts',(49.4304748324618,-25.1900623132835,
-234.713025011659));
#214366=CARTESIAN_POINT('Ctrl Pts',(48.9920207550766,-25.0977237288005,
-235.350049999999));
#214367=CARTESIAN_POINT('Ctrl Pts',(48.2299135975692,-24.9372145504824,
-235.35005));
#214368=CARTESIAN_POINT('Ctrl Pts',(49.4162334358612,-25.2638138055417,
-234.711416035933));
#214369=CARTESIAN_POINT('Ctrl Pts',(48.9774072970604,-25.1738353442622,
-235.350050000003));
#214370=CARTESIAN_POINT('Ctrl Pts',(48.2132345171348,-25.0171100844526,
-235.35005));
#214371=CARTESIAN_POINT('Ctrl Pts',(49.4070241632922,-25.3129840569633,
-234.710320691744));
#214372=CARTESIAN_POINT('Ctrl Pts',(48.9679636427474,-25.224572425112,-235.350049999999));
#214373=CARTESIAN_POINT('Ctrl Pts',(48.2024091551349,-25.0703780812323,
-235.35005));
#214374=CARTESIAN_POINT('Ctrl Pts',(49.3802457522676,-25.4604973397937,
-234.70696606232));
#214375=CARTESIAN_POINT('Ctrl Pts',(48.940513122283,-25.3768184010969,-235.350050000001));
#214376=CARTESIAN_POINT('Ctrl Pts',(48.1708085736138,-25.2301948978772,
-235.35005));
#214377=CARTESIAN_POINT('Ctrl Pts',(49.3635250310457,-25.5588470628881,
-234.704638120292));
#214378=CARTESIAN_POINT('Ctrl Pts',(48.9233997772468,-25.4782980756233,
-235.350050000001));
#214379=CARTESIAN_POINT('Ctrl Pts',(48.1509087141736,-25.3367565417747,
-235.35005));
#214380=CARTESIAN_POINT('Ctrl Pts',(49.2855135355185,-26.0505522453803,
-234.692532681863));
#214381=CARTESIAN_POINT('Ctrl Pts',(48.8435554437265,-25.9864180900749,
-235.350049999994));
#214382=CARTESIAN_POINT('Ctrl Pts',(48.0571667807649,-25.8696491072789,
-235.35005));
#214383=CARTESIAN_POINT('Ctrl Pts',(49.24093071664,-26.443949521064,-234.681362278638));
#214384=CARTESIAN_POINT('Ctrl Pts',(48.7984910202732,-26.3925228008522,
-235.350049999982));
#214385=CARTESIAN_POINT('Ctrl Pts',(48.000556289185,-26.2962324730956,-235.35005));
#214386=CARTESIAN_POINT('Ctrl Pts',(49.1586792195434,-27.62308861654,-234.642841042967));
#214387=CARTESIAN_POINT('Ctrl Pts',(48.7173180681133,-27.612103610794,-235.350050000037));
#214388=CARTESIAN_POINT('Ctrl Pts',(47.8838810362842,-27.5767613139966,
-235.35005));
#214389=CARTESIAN_POINT('Ctrl Pts',(49.1719516846433,-28.4084423968299,
-234.610732565613));
#214390=CARTESIAN_POINT('Ctrl Pts',(48.7364227605218,-28.4243954137753,
-235.350049999951));
#214391=CARTESIAN_POINT('Ctrl Pts',(47.876633025442,-28.431480559278,-235.35005));
#214392=CARTESIAN_POINT('Ctrl Pts',(49.329058348282,-29.9760690458421,-234.530187142121));
#214393=CARTESIAN_POINT('Ctrl Pts',(48.9147174357445,-30.0364945671442,
-235.35005000005));
#214394=CARTESIAN_POINT('Ctrl Pts',(47.9998818090224,-30.1429370236128,
-235.35005));
#214395=CARTESIAN_POINT('Ctrl Pts',(49.4727250783003,-30.7578511157521,
-234.481690588048));
#214396=CARTESIAN_POINT('Ctrl Pts',(49.077384122066,-30.8424286009874,-235.350050000038));
#214397=CARTESIAN_POINT('Ctrl Pts',(48.1303803611475,-30.9997028426405,
-235.35005));
#214398=CARTESIAN_POINT('Ctrl Pts',(49.6820070592694,-31.5392028235171,
-234.422833933791));
#214399=CARTESIAN_POINT('Ctrl Pts',(49.3091456199776,-31.6271496259376,
-235.35005));
#214400=CARTESIAN_POINT('Ctrl Pts',(48.3327003568643,-31.8574637039839,
-235.35005));
#214401=CARTESIAN_POINT('',(49.658099715389,-31.5448418470982,-234.479004887568));
#214402=CARTESIAN_POINT('',(48.3327003568643,-31.8574637039841,-235.35005));
#214403=CARTESIAN_POINT('Origin',(48.3327003568642,-31.8574637039841,-233.85005));
#214404=CARTESIAN_POINT('Ctrl Pts',(48.3395182384274,8.75410525715256,-235.35005));
#214405=CARTESIAN_POINT('Ctrl Pts',(48.1420743191374,7.93092102614352,-235.35005));
#214406=CARTESIAN_POINT('Ctrl Pts',(48.0110562569534,7.1033413541692,-235.35005));
#214407=CARTESIAN_POINT('Ctrl Pts',(47.9456204841389,6.27142206048251,-235.35005));
#214408=CARTESIAN_POINT('Ctrl Pts',(47.8801847113245,5.43950276679582,-235.35005));
#214409=CARTESIAN_POINT('Ctrl Pts',(47.8802911706055,4.60324650205529,-235.35005));
#214410=CARTESIAN_POINT('Ctrl Pts',(47.9494611326687,3.76242026158568,-235.35005));
#214411=CARTESIAN_POINT('Ctrl Pts',(47.9840461137003,3.34200714135088,-235.35005));
#214412=CARTESIAN_POINT('Ctrl Pts',(48.0360840389923,2.92068200696516,-235.35005));
#214413=CARTESIAN_POINT('Ctrl Pts',(48.1054567185474,2.50226370649453,-235.35005));
#214414=CARTESIAN_POINT('Ctrl Pts',(48.140143058325,2.29305455625922,-235.35005));
#214415=CARTESIAN_POINT('Ctrl Pts',(48.1791846215669,2.08432209117834,-235.35005));
#214416=CARTESIAN_POINT('Ctrl Pts',(48.222640293554,1.87607275633673,-235.35005));
#214417=CARTESIAN_POINT('Ctrl Pts',(48.2280722525526,1.85004158948043,-235.35005));
#214418=CARTESIAN_POINT('Ctrl Pts',(48.2336222090191,1.82402333761035,-235.35005));
#214419=CARTESIAN_POINT('Ctrl Pts',(48.2391090978947,1.79799818290319,-235.35005));
#214420=CARTESIAN_POINT('Ctrl Pts',(48.2445959867701,1.77197302819679,-235.35005));
#214421=CARTESIAN_POINT('Ctrl Pts',(48.2500003144159,1.74593883705,-235.35005));
#214422=CARTESIAN_POINT('Ctrl Pts',(48.2553221919377,1.71989562162854,-235.35005));
#214423=CARTESIAN_POINT('Ctrl Pts',(48.265965946981,1.66780919078707,-235.35005));
#214424=CARTESIAN_POINT('Ctrl Pts',(48.2762799057506,1.61568666327577,-235.35005));
#214425=CARTESIAN_POINT('Ctrl Pts',(48.2862649052553,1.56352813074,-235.35005));
#214426=CARTESIAN_POINT('Ctrl Pts',(48.3062349042647,1.45921106566754,-235.35005));
#214427=CARTESIAN_POINT('Ctrl Pts',(48.3248891350009,1.35474998793937,-235.35005));
#214428=CARTESIAN_POINT('Ctrl Pts',(48.3422334665882,1.25014553997188,-235.35005));
#214429=CARTESIAN_POINT('Ctrl Pts',(48.4809881192878,0.41330995622679,-235.35005));
#214430=CARTESIAN_POINT('Ctrl Pts',(48.5368013795039,-0.432603676297867,
-235.35005));
#214431=CARTESIAN_POINT('Ctrl Pts',(48.5074366626247,-1.28784015470909,
-235.35005));
#214432=CARTESIAN_POINT('Ctrl Pts',(48.492754304185,-1.7154583939147,-235.35005));
#214433=CARTESIAN_POINT('Ctrl Pts',(48.4566916340691,-2.14207645772467,
-235.35005));
#214434=CARTESIAN_POINT('Ctrl Pts',(48.3993142685993,-2.56629662313498,
-235.35005));
#214435=CARTESIAN_POINT('Ctrl Pts',(48.3849699272317,-2.67235166448867,
-235.35005));
#214436=CARTESIAN_POINT('Ctrl Pts',(48.369288587157,-2.77828474965553,-235.35005));
#214437=CARTESIAN_POINT('Ctrl Pts',(48.3522652960998,-2.88409542692065,
-235.35005));
#214438=CARTESIAN_POINT('Ctrl Pts',(48.3437536505715,-2.93700076555112,
-235.35005));
#214439=CARTESIAN_POINT('Ctrl Pts',(48.3349064994319,-2.98987550057008,
-235.35005));
#214440=CARTESIAN_POINT('Ctrl Pts',(48.3257231157807,-3.04271956568589,
-235.35005));
#214441=CARTESIAN_POINT('Ctrl Pts',(48.3234272698678,-3.05593058196506,
-235.35005));
#214442=CARTESIAN_POINT('Ctrl Pts',(48.3211104090812,-3.06913968134127,
-235.35005));
#214443=CARTESIAN_POINT('Ctrl Pts',(48.3187725213423,-3.08234686271546,
-235.35005));
#214444=CARTESIAN_POINT('Ctrl Pts',(48.3164346336033,-3.09555404408982,
-235.35005));
#214445=CARTESIAN_POINT('Ctrl Pts',(48.3140690695364,-3.1087587009315,-235.35005));
#214446=CARTESIAN_POINT('Ctrl Pts',(48.31169696982,-3.12196276161221,-235.35005));
#214447=CARTESIAN_POINT('Ctrl Pts',(48.306952770387,-3.14837088297426,-235.35005));
#214448=CARTESIAN_POINT('Ctrl Pts',(48.3022780138533,-3.17478533866958,
-235.35005));
#214449=CARTESIAN_POINT('Ctrl Pts',(48.2976726119403,-3.20120612064097,
-235.35005));
#214450=CARTESIAN_POINT('Ctrl Pts',(48.2608293966366,-3.41257237640728,
-235.35005));
#214451=CARTESIAN_POINT('Ctrl Pts',(48.2284220495736,-3.62434325601736,
-235.35005));
#214452=CARTESIAN_POINT('Ctrl Pts',(48.2004248943047,-3.8365164173544,-235.35005));
#214453=CARTESIAN_POINT('Ctrl Pts',(48.144430583767,-4.2608627400285,-235.35005));
#214454=CARTESIAN_POINT('Ctrl Pts',(48.1060703916864,-4.6868175831452,-235.35005));
#214455=CARTESIAN_POINT('Ctrl Pts',(48.0854449269901,-5.11439012388267,
-235.35005));
#214456=CARTESIAN_POINT('Ctrl Pts',(48.0648194622937,-5.54196266462014,
-235.35005));
#214457=CARTESIAN_POINT('Ctrl Pts',(48.0619566741596,-5.97223878738515,
-235.35005));
#214458=CARTESIAN_POINT('Ctrl Pts',(48.0771357161752,-6.40148796840999,
-235.35005));
#214459=CARTESIAN_POINT('Ctrl Pts',(48.1074938002064,-7.25998633045966,
-235.35005));
#214460=CARTESIAN_POINT('Ctrl Pts',(48.2090347930406,-8.11012177188801,
-235.35005));
#214461=CARTESIAN_POINT('Ctrl Pts',(48.3817353557071,-8.95189703464271,
-235.35005));
#214462=CARTESIAN_POINT('Ctrl Pts',(48.3844338019987,-8.96504977312313,
-235.35005));
#214463=CARTESIAN_POINT('Ctrl Pts',(48.3871335038458,-8.97820236409949,
-235.35005));
#214464=CARTESIAN_POINT('Ctrl Pts',(48.3898027548802,-8.99135853258005,
-235.35005));
#214465=CARTESIAN_POINT('Ctrl Pts',(48.3924720059147,-9.00451470106053,
-235.35005));
#214466=CARTESIAN_POINT('Ctrl Pts',(48.3951203394452,-9.01767332703754,
-235.35005));
#214467=CARTESIAN_POINT('Ctrl Pts',(48.3977477753549,-9.03083440817268,
-235.35005));
#214468=CARTESIAN_POINT('Ctrl Pts',(48.4030026471742,-9.05715657044287,
-235.35005));
#214469=CARTESIAN_POINT('Ctrl Pts',(48.4081739297218,-9.08348855318059,
-235.35005));
#214470=CARTESIAN_POINT('Ctrl Pts',(48.4132617664092,-9.10983033956203,
-235.35005));
#214471=CARTESIAN_POINT('Ctrl Pts',(48.4234374397839,-9.16251391232474,
-235.35005));
#214472=CARTESIAN_POINT('Ctrl Pts',(48.4332793498323,-9.21523669724522,
-235.35005));
#214473=CARTESIAN_POINT('Ctrl Pts',(48.4427883984152,-9.2679985883848,-235.35005));
#214474=CARTESIAN_POINT('Ctrl Pts',(48.4618064955809,-9.37352237066414,
-235.35005));
#214475=CARTESIAN_POINT('Ctrl Pts',(48.4794934628395,-9.47920254067581,
-235.35005));
#214476=CARTESIAN_POINT('Ctrl Pts',(48.4958526690327,-9.58503870263171,
-235.35005));
#214477=CARTESIAN_POINT('Ctrl Pts',(48.5285710814205,-9.79671102655205,
-235.35005));
#214478=CARTESIAN_POINT('Ctrl Pts',(48.5559827004663,-10.0090068188147,
-235.35005));
#214479=CARTESIAN_POINT('Ctrl Pts',(48.5780974937539,-10.2219249084145,
-235.35005));
#214480=CARTESIAN_POINT('Ctrl Pts',(48.6223270803283,-10.6477610876057,
-235.35005));
#214481=CARTESIAN_POINT('Ctrl Pts',(48.6453046119738,-11.0773736644268,
-235.35005));
#214482=CARTESIAN_POINT('Ctrl Pts',(48.6469140232755,-11.5038145314612,
-235.35005));
#214483=CARTESIAN_POINT('Ctrl Pts',(48.6501328458788,-12.3566962655301,
-235.35005));
#214484=CARTESIAN_POINT('Ctrl Pts',(48.5694097707119,-13.201098145554,-235.35005));
#214485=CARTESIAN_POINT('Ctrl Pts',(48.4050646665376,-14.0370524847357,
-235.35005));
#214486=CARTESIAN_POINT('Ctrl Pts',(48.3999288820313,-14.0631760578391,
-235.35005));
#214487=CARTESIAN_POINT('Ctrl Pts',(48.3947106332613,-14.0892913003493,
-235.35005));
#214488=CARTESIAN_POINT('Ctrl Pts',(48.3894097433236,-14.1153981944164,
-235.35005));
#214489=CARTESIAN_POINT('Ctrl Pts',(48.3867592983549,-14.1284516414493,
-235.35005));
#214490=CARTESIAN_POINT('Ctrl Pts',(48.3840780942122,-14.1415019811713,
-235.35005));
#214491=CARTESIAN_POINT('Ctrl Pts',(48.3814002229133,-14.1545526575822,
-235.35005));
#214492=CARTESIAN_POINT('Ctrl Pts',(48.3787223516144,-14.1676033339926,
-235.35005));
#214493=CARTESIAN_POINT('Ctrl Pts',(48.3760618299286,-14.1806557630669,
-235.35005));
#214494=CARTESIAN_POINT('Ctrl Pts',(48.3734186404716,-14.1937099430552,
-235.35005));
#214495=CARTESIAN_POINT('Ctrl Pts',(48.3628458826442,-14.2459266630052,
-235.35005));
#214496=CARTESIAN_POINT('Ctrl Pts',(48.3525504293979,-14.2981713964018,
-235.35005));
#214497=CARTESIAN_POINT('Ctrl Pts',(48.3425312602132,-14.350444040166,-235.35005));
#214498=CARTESIAN_POINT('Ctrl Pts',(48.3224929218452,-14.4549893276876,
-235.35005));
#214499=CARTESIAN_POINT('Ctrl Pts',(48.3035595794002,-14.5596462424789,
-235.35005));
#214500=CARTESIAN_POINT('Ctrl Pts',(48.2857247802083,-14.6644141326663,
-235.35005));
#214501=CARTESIAN_POINT('Ctrl Pts',(48.2500551818223,-14.8739499130538,
-235.35005));
#214502=CARTESIAN_POINT('Ctrl Pts',(48.2187775910825,-15.0839293763357,
-235.35005));
#214503=CARTESIAN_POINT('Ctrl Pts',(48.1918669286016,-15.2943499889772,
-235.35005));
#214504=CARTESIAN_POINT('Ctrl Pts',(48.13804560364,-15.71519121426,-235.35005));
#214505=CARTESIAN_POINT('Ctrl Pts',(48.1017687499494,-16.1377801895464,
-235.35005));
#214506=CARTESIAN_POINT('Ctrl Pts',(48.0829143862637,-16.5595284917746,
-235.35005));
#214507=CARTESIAN_POINT('Ctrl Pts',(48.0452056588921,-17.4030250962311,
-235.35005));
#214508=CARTESIAN_POINT('Ctrl Pts',(48.076555383577,-18.2457723122303,-235.35005));
#214509=CARTESIAN_POINT('Ctrl Pts',(48.1770201828715,-19.0877695253175,
-235.35005));
#214510=CARTESIAN_POINT('Ctrl Pts',(48.2021363826951,-19.2982688285893,
-235.35005));
#214511=CARTESIAN_POINT('Ctrl Pts',(48.2315724527786,-19.5085474359751,
-235.35005));
#214512=CARTESIAN_POINT('Ctrl Pts',(48.2653424827524,-19.7185300485352,
-235.35005));
#214513=CARTESIAN_POINT('Ctrl Pts',(48.2737849902462,-19.7710257016774,
-235.35005));
#214514=CARTESIAN_POINT('Ctrl Pts',(48.282498702759,-19.8235043364666,-235.35005));
#214515=CARTESIAN_POINT('Ctrl Pts',(48.2914842922534,-19.8759659107496,
-235.35005));
#214516=CARTESIAN_POINT('Ctrl Pts',(48.2959770870004,-19.9021966978899,
-235.35005));
#214517=CARTESIAN_POINT('Ctrl Pts',(48.300537852968,-19.9284232197822,-235.35005));
#214518=CARTESIAN_POINT('Ctrl Pts',(48.3051666862202,-19.9546454703855,
-235.35005));
#214519=CARTESIAN_POINT('Ctrl Pts',(48.3074811028462,-19.967756595687,-235.35005));
#214520=CARTESIAN_POINT('Ctrl Pts',(48.3098125364066,-19.9808666531674,
-235.35005));
#214521=CARTESIAN_POINT('Ctrl Pts',(48.3121609996811,-19.9939756420136,
-235.35005));
#214522=CARTESIAN_POINT('Ctrl Pts',(48.3145094629556,-20.0070846308597,
-235.35005));
#214523=CARTESIAN_POINT('Ctrl Pts',(48.3168699428148,-20.0201928656576,
-235.35005));
#214524=CARTESIAN_POINT('Ctrl Pts',(48.3191971709643,-20.0333031870275,
-235.35005));
#214525=CARTESIAN_POINT('Ctrl Pts',(48.337814996161,-20.1381857579874,-235.35005));
#214526=CARTESIAN_POINT('Ctrl Pts',(48.3550896009548,-20.2431526171762,
-235.35005));
#214527=CARTESIAN_POINT('Ctrl Pts',(48.3710295920234,-20.3482032245128,
-235.35005));
#214528=CARTESIAN_POINT('Ctrl Pts',(48.4347895562984,-20.7684056538652,
-235.35005));
#214529=CARTESIAN_POINT('Ctrl Pts',(48.4772403630263,-21.1899452510779,
-235.35005));
#214530=CARTESIAN_POINT('Ctrl Pts',(48.4986731253089,-21.612803748536,-235.35005));
#214531=CARTESIAN_POINT('Ctrl Pts',(48.541538649874,-22.458520743452,-235.35005));
#214532=CARTESIAN_POINT('Ctrl Pts',(48.5005032095075,-23.3116677382499,
-235.35005));
#214533=CARTESIAN_POINT('Ctrl Pts',(48.3713478679476,-24.1646010300614,
-235.35005));
#214534=CARTESIAN_POINT('Ctrl Pts',(48.3390590325577,-24.3778343530143,
-235.35005));
#214535=CARTESIAN_POINT('Ctrl Pts',(48.3012455308435,-24.5909867391319,
-235.35005));
#214536=CARTESIAN_POINT('Ctrl Pts',(48.2577770486563,-24.8040562792487,
-235.35005));
#214537=CARTESIAN_POINT('Ctrl Pts',(48.2523434883829,-24.8306899717632,
-235.35005));
#214538=CARTESIAN_POINT('Ctrl Pts',(48.2468215386317,-24.8573223693642,
-235.35005));
#214539=CARTESIAN_POINT('Ctrl Pts',(48.2412109184648,-24.8839534679411,
-235.35005));
#214540=CARTESIAN_POINT('Ctrl Pts',(48.235600298298,-24.9105845665175,-235.35005));
#214541=CARTESIAN_POINT('Ctrl Pts',(48.2299135976341,-24.9372145504959,
-235.35005));
#214542=CARTESIAN_POINT('Ctrl Pts',(48.2243539041553,-24.9638463951525,
-235.35005));
#214543=CARTESIAN_POINT('Ctrl Pts',(48.2132345171977,-25.0171100844654,
-235.35005));
#214544=CARTESIAN_POINT('Ctrl Pts',(48.2024091551918,-25.0703780812439,
-235.35005));
#214545=CARTESIAN_POINT('Ctrl Pts',(48.1918756280125,-25.1236503534574,
-235.35005));
#214546=CARTESIAN_POINT('Ctrl Pts',(48.1708085736529,-25.2301948978888,
-235.35005));
#214547=CARTESIAN_POINT('Ctrl Pts',(48.1509087142019,-25.3367565417865,
-235.35005));
#214548=CARTESIAN_POINT('Ctrl Pts',(48.1321603275509,-25.4433350548857,
-235.35005));
#214549=CARTESIAN_POINT('Ctrl Pts',(48.0571667809486,-25.8696491072753,
-235.35005));
#214550=CARTESIAN_POINT('Ctrl Pts',(48.000556289184,-26.2962324731006,-235.35005));
#214551=CARTESIAN_POINT('Ctrl Pts',(47.9616645382748,-26.7230754200676,
-235.35005));
#214552=CARTESIAN_POINT('Ctrl Pts',(47.8838810364566,-27.5767613140017,
-235.35005));
#214553=CARTESIAN_POINT('Ctrl Pts',(47.87663302545,-28.4314805592623,-235.35005));
#214554=CARTESIAN_POINT('Ctrl Pts',(47.9382574172368,-29.287208791445,-235.35005));
#214555=CARTESIAN_POINT('Ctrl Pts',(47.9998818090236,-30.1429370236277,
-235.35005));
#214556=CARTESIAN_POINT('Ctrl Pts',(48.1303735979639,-30.9996741692801,
-235.35005));
#214557=CARTESIAN_POINT('Ctrl Pts',(48.3327003568643,-31.8574637039839,
-235.35005));
#214558=CARTESIAN_POINT('',(49.4221378995452,2.0719038723399,-234.730932718857));
#214559=CARTESIAN_POINT('Ctrl Pts',(49.4221408870095,2.07190450465514,-234.730934934417));
#214560=CARTESIAN_POINT('Ctrl Pts',(49.4182232852514,2.09035843187612,-234.730950730033));
#214561=CARTESIAN_POINT('Ctrl Pts',(49.4149015680381,2.10705572274098,-234.730654274928));
#214562=CARTESIAN_POINT('Ctrl Pts',(49.4115036991967,2.12415450023796,-234.73042449474));
#214563=CARTESIAN_POINT('Ctrl Pts',(49.3733014982797,2.31639586206113,-234.727841078683));
#214564=CARTESIAN_POINT('Ctrl Pts',(49.3393998324651,2.50907296397048,-234.72493425655));
#214565=CARTESIAN_POINT('Ctrl Pts',(49.3097659913891,2.70193509071576,-234.721698159298));
#214566=CARTESIAN_POINT('Ctrl Pts',(49.2774742385284,2.91209536379909,-234.718171810741));
#214567=CARTESIAN_POINT('Ctrl Pts',(49.2502357063853,3.12273707873325,-234.714246361282));
#214568=CARTESIAN_POINT('Ctrl Pts',(49.2280289779234,3.33299466926586,-234.709925176676));
#214569=CARTESIAN_POINT('Ctrl Pts',(49.2092927421519,3.51039296527072,-234.706279311698));
#214570=CARTESIAN_POINT('Ctrl Pts',(49.1941375830618,3.6875175390473,-234.702351808155));
#214571=CARTESIAN_POINT('Ctrl Pts',(49.1825231413468,3.86385721504412,-234.698147062218));
#214572=CARTESIAN_POINT('Ctrl Pts',(49.1681240737819,4.08247529169204,-234.692934205472));
#214573=CARTESIAN_POINT('Ctrl Pts',(49.1591074262883,4.29983617559454,-234.687308219309));
#214574=CARTESIAN_POINT('Ctrl Pts',(49.1552509845704,4.51563191357569,-234.681265027564));
#214575=CARTESIAN_POINT('Ctrl Pts',(49.1513139372653,4.73593811571876,-234.67509552378));
#214576=CARTESIAN_POINT('Ctrl Pts',(49.1527549634472,4.95461301468044,-234.668491134634));
#214577=CARTESIAN_POINT('Ctrl Pts',(49.1592840662806,5.17133527581149,-234.661454349866));
#214578=CARTESIAN_POINT('Ctrl Pts',(49.1613990646159,5.24153898269353,-234.659174896096));
#214579=CARTESIAN_POINT('Ctrl Pts',(49.1640475660896,5.31153784457789,-234.65685012576));
#214580=CARTESIAN_POINT('Ctrl Pts',(49.1672185750418,5.38132108902236,-234.654480287413));
#214581=CARTESIAN_POINT('Ctrl Pts',(49.1793032159329,5.64726340014486,-234.645448888945));
#214582=CARTESIAN_POINT('Ctrl Pts',(49.1990014495819,5.91050106767095,-234.635744155024));
#214583=CARTESIAN_POINT('Ctrl Pts',(49.2257531223812,6.1707314416152,-234.62537046774));
#214584=CARTESIAN_POINT('Ctrl Pts',(49.251986745657,6.42592242148932,-234.61519766822));
#214585=CARTESIAN_POINT('Ctrl Pts',(49.2850112790651,6.67820467251632,-234.604372700794));
#214586=CARTESIAN_POINT('Ctrl Pts',(49.3243732573171,6.92732901222819,-234.592891821915));
#214587=CARTESIAN_POINT('Ctrl Pts',(49.3653529024791,7.18669166359865,-234.580939111113));
#214588=CARTESIAN_POINT('Ctrl Pts',(49.4132016932428,7.44263148361976,-234.568275325636));
#214589=CARTESIAN_POINT('Ctrl Pts',(49.4673510903997,7.69487403972389,-234.554910952386));
#214590=CARTESIAN_POINT('Ctrl Pts',(49.5215004875566,7.94711659582802,-234.541546579136));
#214591=CARTESIAN_POINT('Ctrl Pts',(49.5819501731039,8.19566191358684,-234.52748158509));
#214592=CARTESIAN_POINT('Ctrl Pts',(49.6480781836462,8.44024209637807,-234.512742074857));
#214593=CARTESIAN_POINT('',(49.5702506762145,-3.34422295956514,-234.635326079404));
#214594=CARTESIAN_POINT('Ctrl Pts',(49.5702506762146,-3.34422295956515,
-234.635326079404));
#214595=CARTESIAN_POINT('Ctrl Pts',(49.731975358304,-2.38242690605151,-234.653464711487));
#214596=CARTESIAN_POINT('Ctrl Pts',(49.7872739145354,-1.4452195583889,-234.670501062853));
#214597=CARTESIAN_POINT('Ctrl Pts',(49.7263273644162,0.364338783416933,
-234.702369204151));
#214598=CARTESIAN_POINT('Ctrl Pts',(49.6098794126944,1.23676270601011,-234.717200994082));
#214599=CARTESIAN_POINT('Ctrl Pts',(49.4221349121291,2.07190323979717,-234.730930503297));
#214600=CARTESIAN_POINT('',(49.6141435772397,-8.70527256325991,-234.668819403276));
#214601=CARTESIAN_POINT('Ctrl Pts',(49.6141588085565,-8.70526917104303,
-234.668797544165));
#214602=CARTESIAN_POINT('Ctrl Pts',(49.5360287314272,-8.33694180550121,
-234.672403005448));
#214603=CARTESIAN_POINT('Ctrl Pts',(49.4735905740263,-7.96646653536758,
-234.674792519891));
#214604=CARTESIAN_POINT('Ctrl Pts',(49.4268342076459,-7.59523712284396,
-234.675966087494));
#214605=CARTESIAN_POINT('Ctrl Pts',(49.4174758208848,-7.52093476172361,
-234.67620097956));
#214606=CARTESIAN_POINT('Ctrl Pts',(49.4087456762641,-7.44660202278907,
-234.676387159727));
#214607=CARTESIAN_POINT('Ctrl Pts',(49.4006437153166,-7.37224983055676,
-234.676524627996));
#214608=CARTESIAN_POINT('Ctrl Pts',(49.3609559061817,-7.00803237342166,
-234.677198022304));
#214609=CARTESIAN_POINT('Ctrl Pts',(49.3363408447164,-6.64335215271695,
-234.676702539053));
#214610=CARTESIAN_POINT('Ctrl Pts',(49.3265733152131,-6.27948793853651,
-234.675038178241));
#214611=CARTESIAN_POINT('Ctrl Pts',(49.3242955632398,-6.19463614140473,
-234.674650055418));
#214612=CARTESIAN_POINT('Ctrl Pts',(49.3228252788021,-6.10982850191821,
-234.674198368419));
#214613=CARTESIAN_POINT('Ctrl Pts',(49.3221596987034,-6.02508083788686,
-234.673683117244));
#214614=CARTESIAN_POINT('Ctrl Pts',(49.3193496869264,-5.66728478229663,
-234.671507778961));
#214615=CARTESIAN_POINT('Ctrl Pts',(49.3308815436732,-5.31056154720834,
-234.668199445541));
#214616=CARTESIAN_POINT('Ctrl Pts',(49.3563581141433,-4.95604968380208,
-234.663758116984));
#214617=CARTESIAN_POINT('Ctrl Pts',(49.3630340858964,-4.86315212567135,
-234.662594295346));
#214618=CARTESIAN_POINT('Ctrl Pts',(49.3706676986219,-4.77040615738343,
-234.661352674513));
#214619=CARTESIAN_POINT('Ctrl Pts',(49.3792520240964,-4.67783171297721,
-234.660033254487));
#214620=CARTESIAN_POINT('Ctrl Pts',(49.411583041384,-4.32916996064808,-234.655063942478));
#214621=CARTESIAN_POINT('Ctrl Pts',(49.4573977378051,-3.98294469983329,
-234.648991056405));
#214622=CARTESIAN_POINT('Ctrl Pts',(49.5161582487585,-3.64013054346987,
-234.641814596268));
#214623=CARTESIAN_POINT('Ctrl Pts',(49.5331149974404,-3.54120333198457,
-234.639743657316));
#214624=CARTESIAN_POINT('Ctrl Pts',(49.5511499763925,-3.44255989539943,
-234.637580818362));
#214625=CARTESIAN_POINT('Ctrl Pts',(49.5702506762145,-3.34422295956514,
-234.635326079404));
#214626=CARTESIAN_POINT('',(49.5862818295591,-19.7758832613919,-234.611073195661));
#214627=CARTESIAN_POINT('Ctrl Pts',(49.5862817758785,-19.7758829597833,
-234.611073194947));
#214628=CARTESIAN_POINT('Ctrl Pts',(49.5856701841187,-19.7724466885745,
-234.611065064026));
#214629=CARTESIAN_POINT('Ctrl Pts',(49.5850559570526,-19.7691488444015,
-234.611102786428));
#214630=CARTESIAN_POINT('Ctrl Pts',(49.5844388227214,-19.7660482425881,
-234.611205858899));
#214631=CARTESIAN_POINT('Ctrl Pts',(49.5820527975357,-19.7540603922231,
-234.611604367782));
#214632=CARTESIAN_POINT('Ctrl Pts',(49.5796829994118,-19.7420708434331,
-234.612001236557));
#214633=CARTESIAN_POINT('Ctrl Pts',(49.5773293735759,-19.7300793556229,
-234.612396480909));
#214634=CARTESIAN_POINT('Ctrl Pts',(49.5726225928611,-19.7060987794809,
-234.613186890525));
#214635=CARTESIAN_POINT('Ctrl Pts',(49.5679804852513,-19.6821104490426,
-234.613970804101));
#214636=CARTESIAN_POINT('Ctrl Pts',(49.5634026502972,-19.6581124365314,
-234.614748341969));
#214637=CARTESIAN_POINT('Ctrl Pts',(49.5542514928455,-19.6101400667933,
-234.616302651271));
#214638=CARTESIAN_POINT('Ctrl Pts',(49.5453571228543,-19.5621290111651,
-234.617831489122));
#214639=CARTESIAN_POINT('Ctrl Pts',(49.5367169404556,-19.5140638167564,
-234.619335739067));
#214640=CARTESIAN_POINT('Ctrl Pts',(49.5113948055649,-19.3731971914697,
-234.623744305724));
#214641=CARTESIAN_POINT('Ctrl Pts',(49.4882494587589,-19.2318541056419,
-234.627942704));
#214642=CARTESIAN_POINT('Ctrl Pts',(49.4672600204691,-19.0896691715895,
-234.631947130515));
#214643=CARTESIAN_POINT('Ctrl Pts',(49.4597356917718,-19.0386984802903,
-234.633382643983));
#214644=CARTESIAN_POINT('Ctrl Pts',(49.4524888996529,-18.9876195779269,
-234.634793189811));
#214645=CARTESIAN_POINT('Ctrl Pts',(49.4455203099591,-18.9364155675292,
-234.636179383111));
#214646=CARTESIAN_POINT('Ctrl Pts',(49.4262703972779,-18.7949704871918,
-234.640008579715));
#214647=CARTESIAN_POINT('Ctrl Pts',(49.4091419635085,-18.6526552281547,
-234.64365180556));
#214648=CARTESIAN_POINT('Ctrl Pts',(49.3941865856165,-18.5090778608037,
-234.647113321184));
#214649=CARTESIAN_POINT('Ctrl Pts',(49.3912923261972,-18.4812918596174,
-234.647783215604));
#214650=CARTESIAN_POINT('Ctrl Pts',(49.3884796089816,-18.4534585861893,
-234.648446292274));
#214651=CARTESIAN_POINT('Ctrl Pts',(49.3857490339193,-18.4255751954284,
-234.649102564516));
#214652=CARTESIAN_POINT('Ctrl Pts',(49.3632387172659,-18.195710078709,-234.654512742091));
#214653=CARTESIAN_POINT('Ctrl Pts',(49.3464119095609,-17.9635945583682,
-234.659458943744));
#214654=CARTESIAN_POINT('Ctrl Pts',(49.335606787588,-17.7295172691397,-234.663920955939));
#214655=CARTESIAN_POINT('Ctrl Pts',(49.3275029461084,-17.5539593022183,
-234.667267465085));
#214656=CARTESIAN_POINT('Ctrl Pts',(49.3227855338785,-17.3772989895442,
-234.670341773446));
#214657=CARTESIAN_POINT('Ctrl Pts',(49.3215747712971,-17.1996717234086,
-234.673142723318));
#214658=CARTESIAN_POINT('Ctrl Pts',(49.3213242475783,-17.1629181567187,
-234.673722279037));
#214659=CARTESIAN_POINT('Ctrl Pts',(49.3212223306807,-17.1252656126309,
-234.674303302428));
#214660=CARTESIAN_POINT('Ctrl Pts',(49.3212757178132,-17.0883123223587,
-234.674861077993));
#214661=CARTESIAN_POINT('Ctrl Pts',(49.3213083360333,-17.065734774158,-234.675201865095));
#214662=CARTESIAN_POINT('Ctrl Pts',(49.3213978701176,-17.043418278368,-234.675534060606));
#214663=CARTESIAN_POINT('Ctrl Pts',(49.3215363071684,-17.0217275821295,
-234.675852798948));
#214664=CARTESIAN_POINT('Ctrl Pts',(49.3223986160657,-16.8866186625913,
-234.677838184415));
#214665=CARTESIAN_POINT('Ctrl Pts',(49.3252945480659,-16.751112237095,-234.679665550824));
#214666=CARTESIAN_POINT('Ctrl Pts',(49.3302536736133,-16.615291107567,-234.681335289665));
#214667=CARTESIAN_POINT('Ctrl Pts',(49.3336914636545,-16.52113649865,-234.682492794452));
#214668=CARTESIAN_POINT('Ctrl Pts',(49.3381279215342,-16.4267999770715,
-234.683574583287));
#214669=CARTESIAN_POINT('Ctrl Pts',(49.3435718218144,-16.3323432037176,
-234.684579451245));
#214670=CARTESIAN_POINT('Ctrl Pts',(49.3502202748289,-16.2169863111923,
-234.685806662815));
#214671=CARTESIAN_POINT('Ctrl Pts',(49.3583723481284,-16.1014265720288,
-234.686919192352));
#214672=CARTESIAN_POINT('Ctrl Pts',(49.3680488937542,-15.9857057851749,
-234.687916165977));
#214673=CARTESIAN_POINT('Ctrl Pts',(49.3728871665672,-15.9278453917479,
-234.68841465279));
#214674=CARTESIAN_POINT('Ctrl Pts',(49.3781065858137,-15.8699447363607,
-234.688884269287));
#214675=CARTESIAN_POINT('Ctrl Pts',(49.38370992444,-15.8120092127478,-234.689325001877));
#214676=CARTESIAN_POINT('Ctrl Pts',(49.3865115937531,-15.7830414509413,
-234.689545368171));
#214677=CARTESIAN_POINT('Ctrl Pts',(49.3894092446592,-15.7540649722185,
-234.689758514671));
#214678=CARTESIAN_POINT('Ctrl Pts',(49.3924032336974,-15.7250804564227,
-234.689964447131));
#214679=CARTESIAN_POINT('Ctrl Pts',(49.3939002282166,-15.7105881985248,
-234.690067413361));
#214680=CARTESIAN_POINT('Ctrl Pts',(49.3954213073818,-15.6960939313622,
-234.690168576157));
#214681=CARTESIAN_POINT('Ctrl Pts',(49.3969665114127,-15.6815977400521,
-234.690267944053));
#214682=CARTESIAN_POINT('Ctrl Pts',(49.3977391134282,-15.6743496443971,
-234.690317628001));
#214683=CARTESIAN_POINT('Ctrl Pts',(49.3985177466665,-15.6671010677085,
-234.690366863229));
#214684=CARTESIAN_POINT('Ctrl Pts',(49.3993024163132,-15.6598520206932,
-234.69041565065));
#214685=CARTESIAN_POINT('Ctrl Pts',(49.4000870859599,-15.6526029736779,
-234.690464438071));
#214686=CARTESIAN_POINT('Ctrl Pts',(49.4007213537353,-15.6467769609444,
-234.690503374121));
#214687=CARTESIAN_POINT('Ctrl Pts',(49.401674525209,-15.6381034777402,-234.690560691966));
#214688=CARTESIAN_POINT('Ctrl Pts',(49.4086356681561,-15.5747598317086,
-234.690979292108));
#214689=CARTESIAN_POINT('Ctrl Pts',(49.4159098086407,-15.5126755048401,
-234.691363775393));
#214690=CARTESIAN_POINT('Ctrl Pts',(49.4234484001886,-15.4518567697051,
-234.691714239976));
#214691=CARTESIAN_POINT('Ctrl Pts',(49.440661182049,-15.312990031236,-234.692514451843));
#214692=CARTESIAN_POINT('Ctrl Pts',(49.4592406606155,-15.1807154273791,
-234.693137686318));
#214693=CARTESIAN_POINT('Ctrl Pts',(49.478646954445,-15.0550006305544,-234.693583469978));
#214694=CARTESIAN_POINT('Ctrl Pts',(49.4879824635785,-14.9945248053252,
-234.693797916769));
#214695=CARTESIAN_POINT('Ctrl Pts',(49.4975100768272,-14.9355669998248,
-234.693971233389));
#214696=CARTESIAN_POINT('Ctrl Pts',(49.5071739782699,-14.8781235782245,
-234.694102988057));
#214697=CARTESIAN_POINT('Ctrl Pts',(49.5074893581282,-14.8762489214644,
-234.694107287849));
#214698=CARTESIAN_POINT('Ctrl Pts',(49.5078048831535,-14.8743758774791,
-234.694111543714));
#214699=CARTESIAN_POINT('Ctrl Pts',(49.508120551448,-14.8725044460541,-234.694115755664));
#214700=CARTESIAN_POINT('Ctrl Pts',(49.5251406418567,-14.7716012745984,
-234.694342854118));
#214701=CARTESIAN_POINT('Ctrl Pts',(49.5425755408943,-14.6753860554339,
-234.694442320262));
#214702=CARTESIAN_POINT('Ctrl Pts',(49.5601444764561,-14.5838256316434,
-234.694414310179));
#214703=CARTESIAN_POINT('Ctrl Pts',(49.5621650137457,-14.5732956112064,
-234.694411088844));
#214704=CARTESIAN_POINT('Ctrl Pts',(49.5641873542603,-14.5628271575438,
-234.694406178676));
#214705=CARTESIAN_POINT('Ctrl Pts',(49.566211095348,-14.552420220728,-234.694399577537));
#214706=CARTESIAN_POINT('Ctrl Pts',(49.5736604149337,-14.5141126532619,
-234.694375278974));
#214707=CARTESIAN_POINT('Ctrl Pts',(49.5811771868836,-14.4763331751919,
-234.694346304807));
#214708=CARTESIAN_POINT('Ctrl Pts',(49.5886002092495,-14.4397579604869,
-234.694321359156));
#214709=CARTESIAN_POINT('Ctrl Pts',(49.5910636104117,-14.4276201247147,
-234.694313080702));
#214710=CARTESIAN_POINT('Ctrl Pts',(49.593516501906,-14.4156148925837,-234.694305260061));
#214711=CARTESIAN_POINT('Ctrl Pts',(49.5959524605128,-14.4037669105823,
-234.694298256206));
#214712=CARTESIAN_POINT('Ctrl Pts',(49.5960037012185,-14.4035176867421,
-234.694298108879));
#214713=CARTESIAN_POINT('Ctrl Pts',(49.5960552484803,-14.4032670890162,
-234.694297928211));
#214714=CARTESIAN_POINT('Ctrl Pts',(49.5961070926888,-14.4030151592276,
-234.694297715194));
#214715=CARTESIAN_POINT('Ctrl Pts',(49.5968357955614,-14.399474128013,-234.694294721103));
#214716=CARTESIAN_POINT('Ctrl Pts',(49.5975953620603,-14.3958050469411,
-234.69428539975));
#214717=CARTESIAN_POINT('Ctrl Pts',(49.5983593106187,-14.3921217569436,
-234.694273113671));
#214718=CARTESIAN_POINT('Ctrl Pts',(49.5992007058072,-14.3880650669379,
-234.69425958207));
#214719=CARTESIAN_POINT('Ctrl Pts',(49.6000476775697,-14.3839900131974,
-234.694242427339));
#214720=CARTESIAN_POINT('Ctrl Pts',(49.6008803844364,-14.3799802633316,
-234.694224515693));
#214721=CARTESIAN_POINT('Ctrl Pts',(49.6019144604037,-14.3750008568475,
-234.694202272568));
#214722=CARTESIAN_POINT('Ctrl Pts',(49.6029268246743,-14.3701209564191,
-234.694178833582));
#214723=CARTESIAN_POINT('Ctrl Pts',(49.6038981183157,-14.3654180115775,
-234.694157721101));
#214724=CARTESIAN_POINT('Ctrl Pts',(49.6041263298015,-14.364313025419,-234.694152760592));
#214725=CARTESIAN_POINT('Ctrl Pts',(49.6043523256419,-14.3632175755733,
-234.694147922998));
#214726=CARTESIAN_POINT('Ctrl Pts',(49.6045759267312,-14.3621323392381,
-234.694143246236));
#214727=CARTESIAN_POINT('Ctrl Pts',(49.6059934793587,-14.3552523207936,
-234.694113597203));
#214728=CARTESIAN_POINT('Ctrl Pts',(49.6073707738684,-14.3485424439946,
-234.694084679769));
#214729=CARTESIAN_POINT('Ctrl Pts',(49.6087665891662,-14.3417169982584,
-234.694055262541));
#214730=CARTESIAN_POINT('Ctrl Pts',(49.6093905361203,-14.3386659383622,
-234.694042112671));
#214731=CARTESIAN_POINT('Ctrl Pts',(49.610018161141,-14.3355917831535,-234.694028862915));
#214732=CARTESIAN_POINT('Ctrl Pts',(49.6106546022253,-14.3324690009502,
-234.694015403194));
#214733=CARTESIAN_POINT('Ctrl Pts',(49.6109010631884,-14.3312597076973,
-234.694010190935));
#214734=CARTESIAN_POINT('Ctrl Pts',(49.6111485095382,-14.3300447656872,
-234.694004954272));
#214735=CARTESIAN_POINT('Ctrl Pts',(49.611395084026,-14.3288332896215,-234.693999732491));
#214736=CARTESIAN_POINT('Ctrl Pts',(49.6147850395021,-14.3121776738709,
-234.693927942397));
#214737=CARTESIAN_POINT('Ctrl Pts',(49.6181087457944,-14.2956937849329,
-234.693856881653));
#214738=CARTESIAN_POINT('Ctrl Pts',(49.621368056795,-14.2793823029497,-234.693786552336));
#214739=CARTESIAN_POINT('Ctrl Pts',(49.6215656402839,-14.2783934806131,
-234.693782288885));
#214740=CARTESIAN_POINT('Ctrl Pts',(49.6217729532503,-14.2773554051453,
-234.693777813415));
#214741=CARTESIAN_POINT('Ctrl Pts',(49.6219848206397,-14.2762938641407,
-234.693773237078));
#214742=CARTESIAN_POINT('Ctrl Pts',(49.6230024413037,-14.2711951745063,
-234.693751256464));
#214743=CARTESIAN_POINT('Ctrl Pts',(49.6241242489022,-14.2655550336701,
-234.69372694717));
#214744=CARTESIAN_POINT('Ctrl Pts',(49.6247840659456,-14.2622316392956,
-234.693712633033));
#214745=CARTESIAN_POINT('Ctrl Pts',(49.6426668794438,-14.1721587283643,
-234.693324681486));
#214746=CARTESIAN_POINT('Ctrl Pts',(49.6609091040036,-14.0757363427447,
-234.692911477574));
#214747=CARTESIAN_POINT('Ctrl Pts',(49.6791169932083,-13.9729211482607,
-234.692470892474));
#214748=CARTESIAN_POINT('Ctrl Pts',(49.6973032646488,-13.8702280236452,
-234.692030830469));
#214749=CARTESIAN_POINT('Ctrl Pts',(49.7154552845705,-13.7611572648343,
-234.691563453377));
#214750=CARTESIAN_POINT('Ctrl Pts',(49.7331290517043,-13.6456600080413,
-234.691066526182));
#214751=CARTESIAN_POINT('Ctrl Pts',(49.7482442014855,-13.5468831981776,
-234.690641538746));
#214752=CARTESIAN_POINT('Ctrl Pts',(49.7630087077081,-13.4434058299061,
-234.690194936374));
#214753=CARTESIAN_POINT('Ctrl Pts',(49.7771147668417,-13.3351940003421,
-234.689725245027));
#214754=CARTESIAN_POINT('Ctrl Pts',(49.7949428459257,-13.1984294343494,
-234.689131621082));
#214755=CARTESIAN_POINT('Ctrl Pts',(49.8117241545392,-13.0540845913291,
-234.68849815651));
#214756=CARTESIAN_POINT('Ctrl Pts',(49.8267588614032,-12.9022266763216,
-234.687827642294));
#214757=CARTESIAN_POINT('Ctrl Pts',(49.8421625163067,-12.7466422051183,
-234.687140673822));
#214758=CARTESIAN_POINT('Ctrl Pts',(49.8557327135801,-12.5831713881624,
-234.686414816221));
#214759=CARTESIAN_POINT('Ctrl Pts',(49.8666619592475,-12.4118807115379,
-234.685652912943));
#214760=CARTESIAN_POINT('Ctrl Pts',(49.8732556411801,-12.3085399802524,
-234.685193251954));
#214761=CARTESIAN_POINT('Ctrl Pts',(49.8788870231814,-12.2023528783246,
-234.684720467992));
#214762=CARTESIAN_POINT('Ctrl Pts',(49.8833697255501,-12.0933330559183,
-234.684235155878));
#214763=CARTESIAN_POINT('Ctrl Pts',(49.8880514882853,-11.9794720631608,
-234.683728292833));
#214764=CARTESIAN_POINT('Ctrl Pts',(49.8914804113678,-11.8626227426854,
-234.683207110347));
#214765=CARTESIAN_POINT('Ctrl Pts',(49.8934412608304,-11.7423757007386,
-234.682669394224));
#214766=CARTESIAN_POINT('Ctrl Pts',(49.894738686951,-11.6628124011977,-234.682313606105));
#214767=CARTESIAN_POINT('Ctrl Pts',(49.8953924076452,-11.5817614694099,
-234.681950577605));
#214768=CARTESIAN_POINT('Ctrl Pts',(49.8953275191994,-11.4991029504226,
-234.681579641099));
#214769=CARTESIAN_POINT('Ctrl Pts',(49.8952387203394,-11.3859860130922,
-234.681072020082));
#214770=CARTESIAN_POINT('Ctrl Pts',(49.8937813676868,-11.2697916883941,
-234.680549566865));
#214771=CARTESIAN_POINT('Ctrl Pts',(49.8907287252221,-11.1503225292933,
-234.680011055946));
#214772=CARTESIAN_POINT('Ctrl Pts',(49.8878360004288,-11.0371119576085,
-234.679500755802));
#214773=CARTESIAN_POINT('Ctrl Pts',(49.8835106413262,-10.9209603545162,
-234.678976034968));
#214774=CARTESIAN_POINT('Ctrl Pts',(49.8775253147662,-10.8017298269359,
-234.678435930759));
#214775=CARTESIAN_POINT('Ctrl Pts',(49.8728628910234,-10.7088521473173,
-234.678015202723));
#214776=CARTESIAN_POINT('Ctrl Pts',(49.8671925600611,-10.6141066390309,
-234.677585141172));
#214777=CARTESIAN_POINT('Ctrl Pts',(49.860391606809,-10.5174440725994,-234.677145336399));
#214778=CARTESIAN_POINT('Ctrl Pts',(49.8505015772869,-10.3768761845046,
-234.676505766912));
#214779=CARTESIAN_POINT('Ctrl Pts',(49.8384113869119,-10.235047932517,-234.675858297621));
#214780=CARTESIAN_POINT('Ctrl Pts',(49.8240396848632,-10.0925147954868,
-234.675205184815));
#214781=CARTESIAN_POINT('Ctrl Pts',(49.8087016745112,-9.94039817604559,
-234.674508158746));
#214782=CARTESIAN_POINT('Ctrl Pts',(49.7907738045307,-9.78735271922151,
-234.673805480482));
#214783=CARTESIAN_POINT('Ctrl Pts',(49.7701982149817,-9.6337741477004,-234.673097931498));
#214784=CARTESIAN_POINT('Ctrl Pts',(49.7594789629549,-9.55376441528764,
-234.672729320146));
#214785=CARTESIAN_POINT('Ctrl Pts',(49.7480419351235,-9.47360986582658,
-234.672359385541));
#214786=CARTESIAN_POINT('Ctrl Pts',(49.7358845215681,-9.39336568284322,
-234.671988232566));
#214787=CARTESIAN_POINT('Ctrl Pts',(49.7183214498908,-9.27744182033725,
-234.671452050568));
#214788=CARTESIAN_POINT('Ctrl Pts',(49.6992549877045,-9.16135102847471,
-234.670914760588));
#214789=CARTESIAN_POINT('Ctrl Pts',(49.678689170327,-9.04525751101117,-234.670376577874));
#214790=CARTESIAN_POINT('Ctrl Pts',(49.6684322730877,-8.98735758625207,
-234.670108167205));
#214791=CARTESIAN_POINT('Ctrl Pts',(49.657802596323,-8.92945695560662,-234.669839535815));
#214792=CARTESIAN_POINT('Ctrl Pts',(49.6468016237758,-8.87157583220034,
-234.669570719627));
#214793=CARTESIAN_POINT('Ctrl Pts',(49.6413045443101,-8.84265319526412,
-234.66943639478));
#214794=CARTESIAN_POINT('Ctrl Pts',(49.6357147660542,-8.81373542759733,
-234.669302023882));
#214795=CARTESIAN_POINT('Ctrl Pts',(49.6300325351597,-8.78482504213622,
-234.66916761209));
#214796=CARTESIAN_POINT('Ctrl Pts',(49.6271918438714,-8.77037200746602,
-234.669100416227));
#214797=CARTESIAN_POINT('Ctrl Pts',(49.6243280469705,-8.75592081772958,
-234.669033210143));
#214798=CARTESIAN_POINT('Ctrl Pts',(49.6214411790143,-8.74147178634651,
-234.668965994533));
#214799=CARTESIAN_POINT('Ctrl Pts',(49.6190101807009,-8.72930442315087,
-234.66890939304));
#214800=CARTESIAN_POINT('Ctrl Pts',(49.6164243458588,-8.71628499550421,
-234.668786528861));
#214801=CARTESIAN_POINT('Ctrl Pts',(49.6141435772397,-8.70527256325991,
-234.668819403276));
#214802=CARTESIAN_POINT('',(49.4065714250583,-25.1565443079239,-234.754646206088));
#214803=CARTESIAN_POINT('Ctrl Pts',(49.4065714250583,-25.1565443079239,
-234.754646206088));
#214804=CARTESIAN_POINT('Ctrl Pts',(49.4083237251269,-25.1482852903311,
-234.754641300908));
#214805=CARTESIAN_POINT('Ctrl Pts',(49.4102055948399,-25.1397156006737,
-234.754551679989));
#214806=CARTESIAN_POINT('Ctrl Pts',(49.4122790951397,-25.1306732453552,
-234.754333515752));
#214807=CARTESIAN_POINT('Ctrl Pts',(49.4189331800479,-25.1016553570693,
-234.753633403308));
#214808=CARTESIAN_POINT('Ctrl Pts',(49.425491479273,-25.0726317127091,-234.752931656091));
#214809=CARTESIAN_POINT('Ctrl Pts',(49.4319544654725,-25.0436011247394,
-234.752228286546));
#214810=CARTESIAN_POINT('Ctrl Pts',(49.4728120282646,-24.8600761976765,
-234.747781740559));
#214811=CARTESIAN_POINT('Ctrl Pts',(49.5098654845684,-24.6762738089479,
-234.743270532666));
#214812=CARTESIAN_POINT('Ctrl Pts',(49.5431992801992,-24.4918934418934,
-234.73869682228));
#214813=CARTESIAN_POINT('Ctrl Pts',(49.5519882195003,-24.4432788804942,
-234.737490897116));
#214814=CARTESIAN_POINT('Ctrl Pts',(49.5605182904898,-24.3946241281618,
-234.736280624611));
#214815=CARTESIAN_POINT('Ctrl Pts',(49.568790440235,-24.345923655823,-234.735066040129));
#214816=CARTESIAN_POINT('Ctrl Pts',(49.6017568726559,-24.1518409953682,
-234.73022563969));
#214817=CARTESIAN_POINT('Ctrl Pts',(49.6306454960324,-23.9570800797581,
-234.725316968833));
#214818=CARTESIAN_POINT('Ctrl Pts',(49.6554470702083,-23.7613422927836,
-234.720335856504));
#214819=CARTESIAN_POINT('Ctrl Pts',(49.6802486443842,-23.5656045058091,
-234.715354744174));
#214820=CARTESIAN_POINT('Ctrl Pts',(49.700963180708,-23.3688896486346,-234.710301186495));
#214821=CARTESIAN_POINT('Ctrl Pts',(49.7175182905949,-23.1709026248672,
-234.705170563269));
#214822=CARTESIAN_POINT('Ctrl Pts',(49.7356713244155,-22.9538055978434,
-234.699544724625));
#214823=CARTESIAN_POINT('Ctrl Pts',(49.7487978376448,-22.7356163428593,
-234.693812870551));
#214824=CARTESIAN_POINT('Ctrl Pts',(49.7567917730447,-22.5164167234237,
-234.687964276257));
#214825=CARTESIAN_POINT('Ctrl Pts',(49.7668009281025,-22.2419582909034,
-234.680641288987));
#214826=CARTESIAN_POINT('Ctrl Pts',(49.7687456636369,-21.965803803738,-234.673157766047));
#214827=CARTESIAN_POINT('Ctrl Pts',(49.7623994276333,-21.6883787893522,
-234.665517156773));
#214828=CARTESIAN_POINT('Ctrl Pts',(49.7613370439464,-21.6419368024084,
-234.664238090151));
#214829=CARTESIAN_POINT('Ctrl Pts',(49.7600424275965,-21.5954592431385,
-234.662954623012));
#214830=CARTESIAN_POINT('Ctrl Pts',(49.758514653018,-21.5489481463684,-234.661666773541));
#214831=CARTESIAN_POINT('Ctrl Pts',(49.7487383034572,-21.2513199839034,
-234.653425723591));
#214832=CARTESIAN_POINT('Ctrl Pts',(49.7293929801879,-20.9521046088994,
-234.645004832657));
#214833=CARTESIAN_POINT('Ctrl Pts',(49.7000390073759,-20.6515468050444,
-234.636394542428));
#214834=CARTESIAN_POINT('Ctrl Pts',(49.6839207729116,-20.4865108426676,
-234.631666641452));
#214835=CARTESIAN_POINT('Ctrl Pts',(49.6647857213185,-20.3210700797011,
-234.626881633434));
#214836=CARTESIAN_POINT('Ctrl Pts',(49.642567777647,-20.1552647178752,-234.622037937129));
#214837=CARTESIAN_POINT('Ctrl Pts',(49.6324559718875,-20.0798035664089,
-234.619833479465));
#214838=CARTESIAN_POINT('Ctrl Pts',(49.6217041325569,-20.0042701335921,
-234.617617831245));
#214839=CARTESIAN_POINT('Ctrl Pts',(49.610305223227,-19.9286703683168,-234.615391389004));
#214840=CARTESIAN_POINT('Ctrl Pts',(49.6042283741044,-19.8883675328454,
-234.614204454957));
#214841=CARTESIAN_POINT('Ctrl Pts',(49.5979490645606,-19.8479249986605,
-234.613010889523));
#214842=CARTESIAN_POINT('Ctrl Pts',(49.5914823407987,-19.8074583910592,
-234.611814120112));
#214843=CARTESIAN_POINT('Ctrl Pts',(49.5897664702623,-19.7967210436403,
-234.611496571158));
#214844=CARTESIAN_POINT('Ctrl Pts',(49.588035000243,-19.7857336252768,-234.611096518911));
#214845=CARTESIAN_POINT('Ctrl Pts',(49.5862818832396,-19.7758835630004,
-234.611073196375));
#214846=CARTESIAN_POINT('Ctrl Pts',(49.6580996754574,-31.5448418565169,
-234.479004868619));
#214847=CARTESIAN_POINT('Ctrl Pts',(49.5889692923824,-31.2886791266587,
-234.497358008625));
#214848=CARTESIAN_POINT('Ctrl Pts',(49.5259668643689,-31.0288090594549,
-234.514894203449));
#214849=CARTESIAN_POINT('Ctrl Pts',(49.4697189389541,-30.7654785287572,
-234.531587547898));
#214850=CARTESIAN_POINT('Ctrl Pts',(49.4152575562183,-30.5105118839856,
-234.547750679505));
#214851=CARTESIAN_POINT('Ctrl Pts',(49.3671284004809,-30.2523010935825,
-234.56312376229));
#214852=CARTESIAN_POINT('Ctrl Pts',(49.3258565664253,-29.9910701469485,
-234.577699648186));
#214853=CARTESIAN_POINT('Ctrl Pts',(49.2875821848102,-29.7488116389379,
-234.591216930176));
#214854=CARTESIAN_POINT('Ctrl Pts',(49.255208388255,-29.5039695196051,-234.604047867869));
#214855=CARTESIAN_POINT('Ctrl Pts',(49.2291203187707,-29.256794938899,-234.616195999337));
#214856=CARTESIAN_POINT('Ctrl Pts',(49.2269378044882,-29.2361164424324,
-234.617212305678));
#214857=CARTESIAN_POINT('Ctrl Pts',(49.2247992541417,-29.2154216216419,
-234.61822384072));
#214858=CARTESIAN_POINT('Ctrl Pts',(49.2227048770967,-29.1947106237874,
-234.619230610668));
#214859=CARTESIAN_POINT('Ctrl Pts',(49.2223959055597,-29.1916552480354,
-234.619379133714));
#214860=CARTESIAN_POINT('Ctrl Pts',(49.2220878948198,-29.1885995216247,
-234.619527554474));
#214861=CARTESIAN_POINT('Ctrl Pts',(49.2217808457243,-29.1855434451088,
-234.619675872946));
#214862=CARTESIAN_POINT('Ctrl Pts',(49.20814725871,-29.0498476045519,-234.626261506421));
#214863=CARTESIAN_POINT('Ctrl Pts',(49.1964096967195,-28.9134595989942,
-234.632645495629));
#214864=CARTESIAN_POINT('Ctrl Pts',(49.1866397428615,-28.7764255481263,
-234.638829547784));
#214865=CARTESIAN_POINT('Ctrl Pts',(49.1817547659324,-28.7079085226923,
-234.641921573861));
#214866=CARTESIAN_POINT('Ctrl Pts',(49.1773610716897,-28.639230013251,-234.644964533448));
#214867=CARTESIAN_POINT('Ctrl Pts',(49.1734686010682,-28.5703962137034,
-234.647956595317));
#214868=CARTESIAN_POINT('Ctrl Pts',(49.1715223657574,-28.5359793139296,
-234.649452626252));
#214869=CARTESIAN_POINT('Ctrl Pts',(49.1697014345782,-28.501523592874,-234.650935932901));
#214870=CARTESIAN_POINT('Ctrl Pts',(49.168006860434,-28.4670298366899,-234.652406563149));
#214871=CARTESIAN_POINT('Ctrl Pts',(49.1671595733619,-28.4497829585978,
-234.653141878273));
#214872=CARTESIAN_POINT('Ctrl Pts',(49.1663438753779,-28.4325265717615,
-234.653874024212));
#214873=CARTESIAN_POINT('Ctrl Pts',(49.16555989675,-28.4152607761411,-234.654603006956));
#214874=CARTESIAN_POINT('Ctrl Pts',(49.1647759181221,-28.3979949805206,
-234.655331989701));
#214875=CARTESIAN_POINT('Ctrl Pts',(49.1639715191952,-28.3794688098702,
-234.656110111894));
#214876=CARTESIAN_POINT('Ctrl Pts',(49.1633032261975,-28.3634352639083,
-234.656780506213));
#214877=CARTESIAN_POINT('Ctrl Pts',(49.1535492883436,-28.1294208250036,
-234.666565113486));
#214878=CARTESIAN_POINT('Ctrl Pts',(49.1495893664515,-27.8926629671012,
-234.67582098426));
#214879=CARTESIAN_POINT('Ctrl Pts',(49.1518827203227,-27.6535148424459,
-234.684541920212));
#214880=CARTESIAN_POINT('Ctrl Pts',(49.1541255209231,-27.4196383507616,
-234.69307061726));
#214881=CARTESIAN_POINT('Ctrl Pts',(49.1623490777284,-27.1834758646331,
-234.701087787783));
#214882=CARTESIAN_POINT('Ctrl Pts',(49.1769340405569,-26.9453619477479,
-234.708598340528));
#214883=CARTESIAN_POINT('Ctrl Pts',(49.1791954225708,-26.9084426538678,
-234.709762843249));
#214884=CARTESIAN_POINT('Ctrl Pts',(49.1816096339828,-26.8714764548459,
-234.710915186708));
#214885=CARTESIAN_POINT('Ctrl Pts',(49.1841779822909,-26.8344646058357,
-234.712055410861));
#214886=CARTESIAN_POINT('Ctrl Pts',(49.2006502999015,-26.5970860032813,
-234.719368334243));
#214887=CARTESIAN_POINT('Ctrl Pts',(49.2235079251189,-26.3577860189318,
-234.726160426343));
#214888=CARTESIAN_POINT('Ctrl Pts',(49.2531380562464,-26.1169359028825,
-234.732439631832));
#214889=CARTESIAN_POINT('Ctrl Pts',(49.27212838546,-25.962571989499,-234.736464054772));
#214890=CARTESIAN_POINT('Ctrl Pts',(49.2938996978226,-25.8075714743661,
-234.740277982051));
#214891=CARTESIAN_POINT('Ctrl Pts',(49.3185428121658,-25.6520333832136,
-234.743885335958));
#214892=CARTESIAN_POINT('Ctrl Pts',(49.3341255804144,-25.5536807969899,
-234.746166401539));
#214893=CARTESIAN_POINT('Ctrl Pts',(49.3508585425062,-25.4551134977549,
-234.748364421498));
#214894=CARTESIAN_POINT('Ctrl Pts',(49.3687672739086,-25.3563571553827,
-234.750479674118));
#214895=CARTESIAN_POINT('Ctrl Pts',(49.3708676149762,-25.3447749837087,
-234.750727751542));
#214896=CARTESIAN_POINT('Ctrl Pts',(49.3729841284433,-25.3331902121223,
-234.750974690391));
#214897=CARTESIAN_POINT('Ctrl Pts',(49.375116856777,-25.3216028823929,-234.751220490778));
#214898=CARTESIAN_POINT('Ctrl Pts',(49.3792883227327,-25.2989388840204,
-234.751701258972));
#214899=CARTESIAN_POINT('Ctrl Pts',(49.3835218907602,-25.2762647222862,
-234.752177679767));
#214900=CARTESIAN_POINT('Ctrl Pts',(49.3878178899344,-25.2535806672704,
-234.752649754833));
#214901=CARTESIAN_POINT('Ctrl Pts',(49.3906606768346,-25.2385699720099,
-234.752962140558));
#214902=CARTESIAN_POINT('Ctrl Pts',(49.3935301713084,-25.2235581768053,
-234.753272557438));
#214903=CARTESIAN_POINT('Ctrl Pts',(49.3964294158785,-25.2085301804932,
-234.753581316476));
#214904=CARTESIAN_POINT('Ctrl Pts',(49.3971175598791,-25.2049632425366,
-234.753654601318));
#214905=CARTESIAN_POINT('Ctrl Pts',(49.3978042781239,-25.2014054520326,
-234.753730521486));
#214906=CARTESIAN_POINT('Ctrl Pts',(49.3984958597482,-25.1978402612382,
-234.753804681903));
#214907=CARTESIAN_POINT('Ctrl Pts',(49.3999020438809,-25.1905912040789,
-234.753955471337));
#214908=CARTESIAN_POINT('Ctrl Pts',(49.4013130280618,-25.1833515220461,
-234.75410795772));
#214909=CARTESIAN_POINT('Ctrl Pts',(49.4027328290424,-25.176100384502,-234.754255739074));
#214910=CARTESIAN_POINT('Ctrl Pts',(49.4040083829467,-25.1695859385117,
-234.754388506332));
#214911=CARTESIAN_POINT('Ctrl Pts',(49.4052913934605,-25.1630613071466,
-234.754517219509));
#214912=CARTESIAN_POINT('Ctrl Pts',(49.4065714250583,-25.1565443079239,
-234.754646206088));
#214913=CARTESIAN_POINT('Ctrl Pts',(49.6484258549514,-31.4615165308374,
-234.455477481092));
#214914=CARTESIAN_POINT('Ctrl Pts',(49.2664731987108,-31.560789847093,-235.350058857215));
#214915=CARTESIAN_POINT('Ctrl Pts',(48.3201502075429,-31.80681617839,-235.350049999939));
#214916=CARTESIAN_POINT('Ctrl Pts',(49.6915640011734,-31.7936717862045,
-234.549499823154));
#214917=CARTESIAN_POINT('Ctrl Pts',(49.2699360139611,-31.8599982863635,
-235.350057753084));
#214918=CARTESIAN_POINT('Ctrl Pts',(48.3725632633062,-32.0091245803159,
-235.350049999945));
#214919=CARTESIAN_POINT('Ctrl Pts',(49.6857617267569,-32.1386243287738,
-234.636173317449));
#214920=CARTESIAN_POINT('Ctrl Pts',(49.2421194654545,-32.1629747549767,
-235.350056782343));
#214921=CARTESIAN_POINT('Ctrl Pts',(48.3981101575135,-32.2149613628368,
-235.350049999951));
#214922=CARTESIAN_POINT('Ctrl Pts',(49.6111587388972,-32.4987313250346,
-234.71178896734));
#214923=CARTESIAN_POINT('Ctrl Pts',(49.1639864030906,-32.4715648130799,
-235.350055966599));
#214924=CARTESIAN_POINT('Ctrl Pts',(48.3856187844907,-32.424238145886,-235.350049999956));
#214925=CARTESIAN_POINT('',(49.6282925238268,-32.4090163077321,-234.692796980487));
#214926=CARTESIAN_POINT('',(48.3879672519817,-32.371991693197,-235.35005));
#214927=CARTESIAN_POINT('Origin',(48.3879672519817,-32.371991693197,-233.85005));
#214928=CARTESIAN_POINT('Ctrl Pts',(48.3327003568643,-31.8574637039841,
-235.35005));
#214929=CARTESIAN_POINT('Ctrl Pts',(48.3726098627487,-32.0266650324685,
-235.35005));
#214930=CARTESIAN_POINT('Ctrl Pts',(48.3931627529261,-32.1979455093617,
-235.35005));
#214931=CARTESIAN_POINT('Ctrl Pts',(48.3879672519817,-32.371991693197,-235.35005));
#214932=CARTESIAN_POINT('Ctrl Pts',(49.628292885354,-32.4090157027691,-234.692796608792));
#214933=CARTESIAN_POINT('Ctrl Pts',(49.6398669805306,-32.3436091289938,
-234.67863584219));
#214934=CARTESIAN_POINT('Ctrl Pts',(49.6495418145593,-32.2762949055162,
-234.663608766721));
#214935=CARTESIAN_POINT('Ctrl Pts',(49.6570361968937,-32.2072402554883,
-234.647660035004));
#214936=CARTESIAN_POINT('Ctrl Pts',(49.6643123728975,-32.1401961996784,
-234.632175666335));
#214937=CARTESIAN_POINT('Ctrl Pts',(49.6695326571342,-32.0715117584191,
-234.615822291237));
#214938=CARTESIAN_POINT('Ctrl Pts',(49.6724397156995,-32.0013794966331,
-234.598579757521));
#214939=CARTESIAN_POINT('Ctrl Pts',(49.6753085015994,-31.9321705559741,
-234.581564229113));
#214940=CARTESIAN_POINT('Ctrl Pts',(49.6759239895025,-31.8615518482465,
-234.563682561565));
#214941=CARTESIAN_POINT('Ctrl Pts',(49.6740472933539,-31.7897450833274,
-234.544949166276));
#214942=CARTESIAN_POINT('Ctrl Pts',(49.6722003277704,-31.7190758790592,
-234.526512544884));
#214943=CARTESIAN_POINT('Ctrl Pts',(49.6679389519133,-31.6472562744759,
-234.507250841984));
#214944=CARTESIAN_POINT('Ctrl Pts',(49.6610521066377,-31.5745296567101,
-234.4872133978));
#214945=CARTESIAN_POINT('Ctrl Pts',(49.6601165710637,-31.5646501929824,
-234.484491434246));
#214946=CARTESIAN_POINT('Ctrl Pts',(49.6591326192859,-31.554754036246,-234.481755211493));
#214947=CARTESIAN_POINT('Ctrl Pts',(49.6580997553206,-31.5448418376796,
-234.479004906517));
#214948=CARTESIAN_POINT('Ctrl Pts',(49.6282923119739,-32.4090169808449,
-234.692797218109));
#214949=CARTESIAN_POINT('Ctrl Pts',(49.1821150693849,-32.3956980201291,
-235.35005));
#214950=CARTESIAN_POINT('Ctrl Pts',(48.3879672519816,-32.371991693197,-235.35005));
#214951=CARTESIAN_POINT('Ctrl Pts',(49.5510892026461,-34.9515478422503,
-234.694718333571));
#214952=CARTESIAN_POINT('Ctrl Pts',(49.1048103477618,-34.9355482471023,
-235.350050000493));
#214953=CARTESIAN_POINT('Ctrl Pts',(48.3122036088614,-34.9100285686315,
-235.35005));
#214954=CARTESIAN_POINT('Ctrl Pts',(49.4597789489883,-37.4935285423766,
-234.696950276065));
#214955=CARTESIAN_POINT('Ctrl Pts',(49.0133760622712,-37.4755964900674,
-235.350049998731));
#214956=CARTESIAN_POINT('Ctrl Pts',(48.2225732111533,-37.4475766604583,
-235.35005));
#214957=CARTESIAN_POINT('Ctrl Pts',(49.3543621196711,-40.035034230092,-234.699454871761));
#214958=CARTESIAN_POINT('Ctrl Pts',(48.9077504789076,-40.0168122617172,
-235.35005));
#214959=CARTESIAN_POINT('Ctrl Pts',(48.1190600870606,-39.984633316822,-235.35005));
#214960=CARTESIAN_POINT('',(49.354362119671,-40.035034230092,-234.699454871761));
#214961=CARTESIAN_POINT('',(48.1190600870606,-39.9846333168228,-235.35005));
#214962=CARTESIAN_POINT('Origin',(48.1190600870606,-39.9846333168229,-233.85005));
#214963=CARTESIAN_POINT('Origin',(-647.878174798583,-11.5883202246486,-235.350049998812));
#214964=CARTESIAN_POINT('Origin',(-637.300587775051,-11.5397323655281,-248.898224599212));
#214965=CARTESIAN_POINT('Ctrl Pts',(49.3609022886797,-39.9800961280749,
-234.692504927202));
#214966=CARTESIAN_POINT('Ctrl Pts',(48.9149071348731,-39.9654566603571,
-235.350050000012));
#214967=CARTESIAN_POINT('Ctrl Pts',(48.1206232659769,-39.9395442085637,
-235.35005));
#214968=CARTESIAN_POINT('Ctrl Pts',(49.3507612567607,-40.0954256905313,
-234.703448471667));
#214969=CARTESIAN_POINT('Ctrl Pts',(48.9035065741159,-40.0745135650163,
-235.350049999981));
#214970=CARTESIAN_POINT('Ctrl Pts',(48.1178051349119,-40.0381099761122,
-235.35005));
#214971=CARTESIAN_POINT('Ctrl Pts',(49.3228943382751,-40.244776142729,-234.728096777874));
#214972=CARTESIAN_POINT('Ctrl Pts',(48.8754605639482,-40.2044568428276,
-235.350049999988));
#214973=CARTESIAN_POINT('Ctrl Pts',(48.1111069487499,-40.1362115562182,
-235.35005));
#214974=CARTESIAN_POINT('Ctrl Pts',(49.2876708175288,-40.4241334874338,
-234.747884490557));
#214975=CARTESIAN_POINT('Ctrl Pts',(48.8411755148561,-40.3683318596352,
-235.350050000006));
#214976=CARTESIAN_POINT('Ctrl Pts',(48.0952241561347,-40.2752167333539,
-235.35005));
#214977=CARTESIAN_POINT('Ctrl Pts',(49.2773222483615,-40.475626983426,-234.752817419735));
#214978=CARTESIAN_POINT('Ctrl Pts',(48.8311900432947,-40.4158061621275,
-235.35005));
#214979=CARTESIAN_POINT('Ctrl Pts',(48.0899153448806,-40.3165225558374,
-235.35005));
#214980=CARTESIAN_POINT('Ctrl Pts',(49.2523679230428,-40.5833911338063,
-234.764877519172));
#214981=CARTESIAN_POINT('Ctrl Pts',(48.8074437529392,-40.5134891744514,
-235.350049999999));
#214982=CARTESIAN_POINT('Ctrl Pts',(48.0779218876032,-40.3989852515461,
-235.35005));
#214983=CARTESIAN_POINT('Ctrl Pts',(49.2383249044512,-40.6384352750634,
-234.77139445193));
#214984=CARTESIAN_POINT('Ctrl Pts',(48.7942305707784,-40.5629457939505,
-235.350050000007));
#214985=CARTESIAN_POINT('Ctrl Pts',(48.0712183175412,-40.4401628322643,
-235.350050000001));
#214986=CARTESIAN_POINT('Ctrl Pts',(49.2070746873817,-40.7497958270093,
-234.784872532159));
#214987=CARTESIAN_POINT('Ctrl Pts',(48.7651880041785,-40.6623792650696,
-235.350049999994));
#214988=CARTESIAN_POINT('Ctrl Pts',(48.0561422093234,-40.5222290742639,
-235.350050000001));
#214989=CARTESIAN_POINT('Ctrl Pts',(49.1909312076253,-40.8041772199255,
-234.790945411729));
#214990=CARTESIAN_POINT('Ctrl Pts',(48.7502801223134,-40.7112070153247,
-235.350050000008));
#214991=CARTESIAN_POINT('Ctrl Pts',(48.047773596518,-40.5630852304628,-235.35005));
#214992=CARTESIAN_POINT('Ctrl Pts',(49.158768490346,-40.9094426031434,-234.801416987774));
#214993=CARTESIAN_POINT('Ctrl Pts',(48.7205621630999,-40.8065834345606,
-235.35004999999));
#214994=CARTESIAN_POINT('Ctrl Pts',(48.0296425423562,-40.6445005636306,
-235.35005));
#214995=CARTESIAN_POINT('Ctrl Pts',(49.1434940929471,-40.9592475630511,
-234.805322215117));
#214996=CARTESIAN_POINT('Ctrl Pts',(48.7063433535266,-40.85254418824,-235.350049999989));
#214997=CARTESIAN_POINT('Ctrl Pts',(48.0199029877981,-40.6850741153181,
-235.35005));
#214998=CARTESIAN_POINT('Ctrl Pts',(49.1099224820002,-41.0612319847,-234.814142137496));
#214999=CARTESIAN_POINT('Ctrl Pts',(48.6753864506452,-40.9456620301775,
-235.35005000001));
#215000=CARTESIAN_POINT('Ctrl Pts',(47.9992940161415,-40.7659290146224,
-235.35005));
#215001=CARTESIAN_POINT('Ctrl Pts',(49.0911625161288,-41.1139396903979,
-234.819288114395));
#215002=CARTESIAN_POINT('Ctrl Pts',(48.658290096543,-40.9931106903451,-235.350049999994));
#215003=CARTESIAN_POINT('Ctrl Pts',(47.9883597239418,-40.8062069855079,
-235.35005));
#215004=CARTESIAN_POINT('Ctrl Pts',(49.0497612331153,-41.2211842972616,
-234.830393428202));
#215005=CARTESIAN_POINT('Ctrl Pts',(48.6209603093232,-41.0887634737107,
-235.350050000006));
#215006=CARTESIAN_POINT('Ctrl Pts',(47.9648484820867,-40.886240947879,-235.35005));
#215007=CARTESIAN_POINT('Ctrl Pts',(49.0271415726836,-41.2754545539969,
-234.836237946169));
#215008=CARTESIAN_POINT('Ctrl Pts',(48.6007577894006,-41.1368001922989,
-235.350050000005));
#215009=CARTESIAN_POINT('Ctrl Pts',(47.9522083925962,-40.9259746645696,
-235.35005));
#215010=CARTESIAN_POINT('Ctrl Pts',(48.9650627061772,-41.4259459193992,
-234.848433785789));
#215011=CARTESIAN_POINT('Ctrl Pts',(48.5443602555291,-41.2734119529302,
-235.350049999989));
#215012=CARTESIAN_POINT('Ctrl Pts',(47.9122208177014,-41.0445137282603,
-235.35005));
#215013=CARTESIAN_POINT('Ctrl Pts',(48.9305571766217,-41.5134474083714,
-234.850906132381));
#215014=CARTESIAN_POINT('Ctrl Pts',(48.5115159447976,-41.3570281892003,
-235.350049999988));
#215015=CARTESIAN_POINT('Ctrl Pts',(47.8834173029482,-41.1228515949417,
-235.35005));
#215016=CARTESIAN_POINT('Ctrl Pts',(48.8600618058509,-41.6614149400665,
-234.862519417299));
#215017=CARTESIAN_POINT('Ctrl Pts',(48.4478519693268,-41.491030261857,-235.350050000005));
#215018=CARTESIAN_POINT('Ctrl Pts',(47.8371337927352,-41.2386632571498,
-235.35005));
#215019=CARTESIAN_POINT('Ctrl Pts',(48.8336689082344,-41.7126402268251,
-234.867383172689));
#215020=CARTESIAN_POINT('Ctrl Pts',(48.4244367378701,-41.5365309708231,
-235.35005));
#215021=CARTESIAN_POINT('Ctrl Pts',(47.8210253111431,-41.2769359664061,
-235.35005));
#215022=CARTESIAN_POINT('Ctrl Pts',(48.7803894023132,-41.8118797264952,
-234.876221787666));
#215023=CARTESIAN_POINT('Ctrl Pts',(48.37695681055,-41.6253295090172,-235.35005));
#215024=CARTESIAN_POINT('Ctrl Pts',(47.787220073548,-41.3527085858238,-235.35005));
#215025=CARTESIAN_POINT('Ctrl Pts',(48.7561458319887,-41.8571965621144,
-234.87901210393));
#215026=CARTESIAN_POINT('Ctrl Pts',(48.3547551060156,-41.6671925154113,
-235.350050000011));
#215027=CARTESIAN_POINT('Ctrl Pts',(47.7696001307559,-41.3902458706063,
-235.35005));
#215028=CARTESIAN_POINT('Ctrl Pts',(48.709016314243,-41.9449099980397,-234.883574453964));
#215029=CARTESIAN_POINT('Ctrl Pts',(48.3110938377002,-41.7490915977428,
-235.350049999989));
#215030=CARTESIAN_POINT('Ctrl Pts',(47.7335555457799,-41.4649289014138,
-235.35005));
#215031=CARTESIAN_POINT('Ctrl Pts',(48.6862807786918,-41.9870730165852,
-234.885251664481));
#215032=CARTESIAN_POINT('Ctrl Pts',(48.2897285580126,-41.7890208404672,
-235.35005));
#215033=CARTESIAN_POINT('Ctrl Pts',(47.7151163766151,-41.5020675791261,
-235.35005));
#215034=CARTESIAN_POINT('Ctrl Pts',(48.6527827899951,-42.048957440397,-234.887309869629));
#215035=CARTESIAN_POINT('Ctrl Pts',(48.2579806505418,-41.8480729618835,
-235.35005));
#215036=CARTESIAN_POINT('Ctrl Pts',(47.6870475431915,-41.5575760651628,
-235.35005));
#215037=CARTESIAN_POINT('Ctrl Pts',(48.6419512689392,-42.0691542325064,
-234.887831081218));
#215038=CARTESIAN_POINT('Ctrl Pts',(48.2476153284943,-41.8675047923045,
-235.35005));
#215039=CARTESIAN_POINT('Ctrl Pts',(47.677640411345,-41.5760541500354,-235.35005));
#215040=CARTESIAN_POINT('Ctrl Pts',(48.6154192627871,-42.1141139023562,
-234.890846380581));
#215041=CARTESIAN_POINT('Ctrl Pts',(48.2234659120011,-41.9087902255785,
-235.35005));
#215042=CARTESIAN_POINT('Ctrl Pts',(47.6585760783126,-41.6128886447362,
-235.35005));
#215043=CARTESIAN_POINT('Ctrl Pts',(48.6001168001999,-42.1384070049637,
-234.893144732287));
#215044=CARTESIAN_POINT('Ctrl Pts',(48.209961041715,-41.9303746091141,-235.350050000003));
#215045=CARTESIAN_POINT('Ctrl Pts',(47.6488991764614,-41.6312354689061,
-235.35005));
#215046=CARTESIAN_POINT('Ctrl Pts',(48.5518764612557,-42.2121884412408,
-234.900509539638));
#215047=CARTESIAN_POINT('Ctrl Pts',(48.1677347868008,-41.9954128487312,
-235.350049999995));
#215048=CARTESIAN_POINT('Ctrl Pts',(47.6191741486339,-41.6859381083017,
-235.35005));
#215049=CARTESIAN_POINT('Ctrl Pts',(48.5187143379562,-42.2604201801686,
-234.905150950974));
#215050=CARTESIAN_POINT('Ctrl Pts',(48.1386929365721,-42.0380430577305,
-235.350050000006));
#215051=CARTESIAN_POINT('Ctrl Pts',(47.5984065010933,-41.7219438293822,
-235.35005));
#215052=CARTESIAN_POINT('Ctrl Pts',(48.4473494493779,-42.3648892943066,
-234.91261447131));
#215053=CARTESIAN_POINT('Ctrl Pts',(48.0743924192389,-42.1331831672681,
-235.350049999991));
#215054=CARTESIAN_POINT('Ctrl Pts',(47.5478537905194,-41.8061740914771,
-235.35005));
#215055=CARTESIAN_POINT('Ctrl Pts',(48.4096151874694,-42.4198711263575,
-234.915062488495));
#215056=CARTESIAN_POINT('Ctrl Pts',(48.0392460437368,-42.184970184094,-235.350049999918));
#215057=CARTESIAN_POINT('Ctrl Pts',(47.5175825331856,-41.8541635100818,
-235.350050000001));
#215058=CARTESIAN_POINT('Ctrl Pts',(48.3726352067242,-42.4735605612944,
-234.917093394062));
#215059=CARTESIAN_POINT('Ctrl Pts',(48.0044280594344,-42.2359419015206,
-235.350050000092));
#215060=CARTESIAN_POINT('Ctrl Pts',(47.486819007697,-41.9019089637004,-235.35005));
#215061=CARTESIAN_POINT('',(48.4015825627194,-42.4301635567086,-234.916111528175));
#215062=CARTESIAN_POINT('',(47.511140470057,-41.8639253579254,-235.35005));
#215063=CARTESIAN_POINT('Origin',(47.5111404700569,-41.8639253579254,-233.85005));
#215064=CARTESIAN_POINT('Ctrl Pts',(48.1190600870606,-39.9846333168228,
-235.35005));
#215065=CARTESIAN_POINT('Ctrl Pts',(48.1156573562241,-40.0680330690653,
-235.35005));
#215066=CARTESIAN_POINT('Ctrl Pts',(48.1094051493674,-40.1511056240727,
-235.35005));
#215067=CARTESIAN_POINT('Ctrl Pts',(48.0999509844461,-40.2338479048312,
-235.35005));
#215068=CARTESIAN_POINT('Ctrl Pts',(48.0952242649892,-40.2752158682241,
-235.35005));
#215069=CARTESIAN_POINT('Ctrl Pts',(48.089915468827,-40.3165217899444,-235.35005));
#215070=CARTESIAN_POINT('Ctrl Pts',(48.0839186309937,-40.3577539058372,
-235.35005));
#215071=CARTESIAN_POINT('Ctrl Pts',(48.0779219885029,-40.398984678624,-235.35005));
#215072=CARTESIAN_POINT('Ctrl Pts',(48.0712184248364,-40.4401623582127,
-235.350050000001));
#215073=CARTESIAN_POINT('Ctrl Pts',(48.0636802851834,-40.4811959572599,
-235.350050000001));
#215074=CARTESIAN_POINT('Ctrl Pts',(48.0561422858351,-40.5222287925639,
-235.350050000001));
#215075=CARTESIAN_POINT('Ctrl Pts',(48.0477736645017,-40.563085046475,-235.35005));
#215076=CARTESIAN_POINT('Ctrl Pts',(48.0387080967012,-40.6037929031184,
-235.35005));
#215077=CARTESIAN_POINT('Ctrl Pts',(48.0296425710794,-40.6445005703635,
-235.35005));
#215078=CARTESIAN_POINT('Ctrl Pts',(48.0199029935916,-40.6850742166469,
-235.350049999999));
#215079=CARTESIAN_POINT('Ctrl Pts',(48.0095985320967,-40.7255015726492,
-235.350049999999));
#215080=CARTESIAN_POINT('Ctrl Pts',(47.9992939746968,-40.7659293049141,
-235.35005));
#215081=CARTESIAN_POINT('Ctrl Pts',(47.9883596446658,-40.8062073663638,
-235.35005));
#215082=CARTESIAN_POINT('Ctrl Pts',(47.9766041319244,-40.8462239751862,
-235.35005));
#215083=CARTESIAN_POINT('Ctrl Pts',(47.9648483456559,-40.8862415151148,
-235.35005));
#215084=CARTESIAN_POINT('Ctrl Pts',(47.9522082011025,-40.9259753165071,
-235.35005));
#215085=CARTESIAN_POINT('Ctrl Pts',(47.9388792235724,-40.965487693427,-235.35005));
#215086=CARTESIAN_POINT('Ctrl Pts',(47.9122207498503,-41.0445139847866,
-235.35005));
#215087=CARTESIAN_POINT('Ctrl Pts',(47.8834172501653,-41.1228517627344,
-235.35005));
#215088=CARTESIAN_POINT('Ctrl Pts',(47.8525616386501,-41.2000593734148,
-235.35005));
#215089=CARTESIAN_POINT('Ctrl Pts',(47.8371337962268,-41.2386632705008,
-235.35005));
#215090=CARTESIAN_POINT('Ctrl Pts',(47.8210253173756,-41.2769359691183,
-235.35005));
#215091=CARTESIAN_POINT('Ctrl Pts',(47.8041226974982,-41.3148222784138,
-235.35005));
#215092=CARTESIAN_POINT('Ctrl Pts',(47.7872200865336,-41.3527085677318,
-235.35005));
#215093=CARTESIAN_POINT('Ctrl Pts',(47.7696001482572,-41.3902458425851,
-235.35005));
#215094=CARTESIAN_POINT('Ctrl Pts',(47.7515778408436,-41.4275873872532,
-235.35005));
#215095=CARTESIAN_POINT('Ctrl Pts',(47.7335555714763,-41.4649288530908,
-235.35005));
#215096=CARTESIAN_POINT('Ctrl Pts',(47.7151164076773,-41.5020675212465,
-235.35005));
#215097=CARTESIAN_POINT('Ctrl Pts',(47.69640382207,-41.5390732370252,-235.35005));
#215098=CARTESIAN_POINT('Ctrl Pts',(47.6870475533414,-41.5575760473041,
-235.35005));
#215099=CARTESIAN_POINT('Ctrl Pts',(47.6776404221482,-41.5760541309719,
-235.35005));
#215100=CARTESIAN_POINT('Ctrl Pts',(47.6681082454436,-41.594471397704,-235.35005));
#215101=CARTESIAN_POINT('Ctrl Pts',(47.6585760901228,-41.6128886231199,
-235.35005));
#215102=CARTESIAN_POINT('Ctrl Pts',(47.6488991892717,-41.6312354462549,
-235.35005));
#215103=CARTESIAN_POINT('Ctrl Pts',(47.6389908341615,-41.649469682206,-235.35005));
#215104=CARTESIAN_POINT('Ctrl Pts',(47.6191742063161,-41.6859380025145,
-235.35005));
#215105=CARTESIAN_POINT('Ctrl Pts',(47.5984065690065,-41.7219437163951,
-235.35005));
#215106=CARTESIAN_POINT('Ctrl Pts',(47.5769871577403,-41.7576324579108,
-235.35005));
#215107=CARTESIAN_POINT('Ctrl Pts',(47.5555678934573,-41.7933209545252,
-235.35005));
#215108=CARTESIAN_POINT('Ctrl Pts',(47.5335334800369,-41.8287110790685,
-235.35005));
#215109=CARTESIAN_POINT('Ctrl Pts',(47.511140470057,-41.8639253579254,-235.35005));
#215110=CARTESIAN_POINT('Ctrl Pts',(48.4015825627194,-42.4301635567086,
-234.916111528174));
#215111=CARTESIAN_POINT('Ctrl Pts',(48.4058765897107,-42.4239165186186,
-234.915842996972));
#215112=CARTESIAN_POINT('Ctrl Pts',(48.4111227611927,-42.416329788671,-234.91547953379));
#215113=CARTESIAN_POINT('Ctrl Pts',(48.4172018787063,-42.4075544680719,
-234.91502113863));
#215114=CARTESIAN_POINT('Ctrl Pts',(48.4238231471873,-42.3979965423427,
-234.914521862639));
#215115=CARTESIAN_POINT('Ctrl Pts',(48.4314320807197,-42.3870292212898,
-234.91390996708));
#215116=CARTESIAN_POINT('Ctrl Pts',(48.4398329206511,-42.3748999215492,
-234.913185451955));
#215117=CARTESIAN_POINT('Ctrl Pts',(48.4509908371859,-42.3587898997852,
-234.912223157785));
#215118=CARTESIAN_POINT('Ctrl Pts',(48.4635435696801,-42.3406331652534,
-234.911062192536));
#215119=CARTESIAN_POINT('Ctrl Pts',(48.4769757389003,-42.3210768087327,
-234.909702556209));
#215120=CARTESIAN_POINT('Ctrl Pts',(48.4863784017206,-42.3073871489806,
-234.908750796166));
#215121=CARTESIAN_POINT('Ctrl Pts',(48.4962100771077,-42.293014008753,-234.907701684306));
#215122=CARTESIAN_POINT('Ctrl Pts',(48.5063029203191,-42.2781654388557,
-234.906555220629));
#215123=CARTESIAN_POINT('Ctrl Pts',(48.5138301808973,-42.2670913487811,
-234.90570018596));
#215124=CARTESIAN_POINT('Ctrl Pts',(48.5215027350369,-42.2557527423761,
-234.904791002233));
#215125=CARTESIAN_POINT('Ctrl Pts',(48.5292625384515,-42.2442201250679,
-234.903827669447));
#215126=CARTESIAN_POINT('Ctrl Pts',(48.537856146493,-42.2314483075947,-234.902760824846));
#215127=CARTESIAN_POINT('Ctrl Pts',(48.5465557290762,-42.2184399076426,
-234.901627569163));
#215128=CARTESIAN_POINT('Ctrl Pts',(48.5553068112671,-42.2052580396029,
-234.900427902398));
#215129=CARTESIAN_POINT('Ctrl Pts',(48.555804381456,-42.2045085432061,-234.900359691586));
#215130=CARTESIAN_POINT('Ctrl Pts',(48.5563021267504,-42.2037584745262,
-234.900291266077));
#215131=CARTESIAN_POINT('Ctrl Pts',(48.5568000403903,-42.2030078408306,
-234.900222625872));
#215132=CARTESIAN_POINT('Ctrl Pts',(48.5614275585508,-42.1960315887655,
-234.899584696376));
#215133=CARTESIAN_POINT('Ctrl Pts',(48.5660693588968,-42.1890068770094,
-234.898928222472));
#215134=CARTESIAN_POINT('Ctrl Pts',(48.5707217342098,-42.1819372506444,
-234.898253201485));
#215135=CARTESIAN_POINT('Ctrl Pts',(48.5730479218663,-42.1784024374619,
-234.897915690992));
#215136=CARTESIAN_POINT('Ctrl Pts',(48.575376758472,-42.1748563984891,-234.897573549528));
#215137=CARTESIAN_POINT('Ctrl Pts',(48.5777081628181,-42.1712990551989,
-234.897226768105));
#215138=CARTESIAN_POINT('Ctrl Pts',(48.579199712736,-42.1690231929698,-234.897004909635));
#215139=CARTESIAN_POINT('Ctrl Pts',(48.5810284034547,-42.1662290700574,
-234.896730574233));
#215140=CARTESIAN_POINT('Ctrl Pts',(48.5825473157475,-42.1639047252987,
-234.89650083858));
#215141=CARTESIAN_POINT('Ctrl Pts',(48.5834025772443,-42.1625959449387,
-234.896371480184));
#215142=CARTESIAN_POINT('Ctrl Pts',(48.584160492484,-42.1614350500923,-234.896256262291));
#215143=CARTESIAN_POINT('Ctrl Pts',(48.5847100715227,-42.1605929713353,
-234.8961725155));
#215144=CARTESIAN_POINT('Ctrl Pts',(48.5908125145944,-42.1512426553382,
-234.895242603722));
#215145=CARTESIAN_POINT('Ctrl Pts',(48.5971231173876,-42.1413133697012,
-234.894353868029));
#215146=CARTESIAN_POINT('Ctrl Pts',(48.6036135949882,-42.1308340972216,
-234.893506308421));
#215147=CARTESIAN_POINT('Ctrl Pts',(48.6097093883376,-42.1209920665702,
-234.892710288691));
#215148=CARTESIAN_POINT('Ctrl Pts',(48.6159634161574,-42.1106654554493,
-234.891950589495));
#215149=CARTESIAN_POINT('Ctrl Pts',(48.6223788309257,-42.0998426538058,
-234.891227210831));
#215150=CARTESIAN_POINT('Ctrl Pts',(48.6227942097007,-42.0991419100111,
-234.891180374242));
#215151=CARTESIAN_POINT('Ctrl Pts',(48.623210276151,-42.0984390712821,-234.891133689915));
#215152=CARTESIAN_POINT('Ctrl Pts',(48.623627035934,-42.09773412807,-234.89108715785));
#215153=CARTESIAN_POINT('Ctrl Pts',(48.629575688281,-42.0876720677069,-234.890422978895));
#215154=CARTESIAN_POINT('Ctrl Pts',(48.635663107759,-42.077184554178,-234.88978982102));
#215155=CARTESIAN_POINT('Ctrl Pts',(48.6419213003412,-42.0662231638559,
-234.889187684224));
#215156=CARTESIAN_POINT('Ctrl Pts',(48.6428732361153,-42.0645558230952,
-234.889096092993));
#215157=CARTESIAN_POINT('Ctrl Pts',(48.643829182441,-42.0628774393602,-234.889005219515));
#215158=CARTESIAN_POINT('Ctrl Pts',(48.6447893182988,-42.0611877542926,
-234.888915063789));
#215159=CARTESIAN_POINT('Ctrl Pts',(48.6466073340208,-42.0579883383006,
-234.888744354064));
#215160=CARTESIAN_POINT('Ctrl Pts',(48.6484403551025,-42.0547484237675,
-234.888576217721));
#215161=CARTESIAN_POINT('Ctrl Pts',(48.6502897877342,-42.0514660037669,
-234.888410654761));
#215162=CARTESIAN_POINT('Ctrl Pts',(48.6521393090423,-42.0481834263811,
-234.888245083861));
#215163=CARTESIAN_POINT('Ctrl Pts',(48.6540052670553,-42.0448583089355,
-234.888082086591));
#215164=CARTESIAN_POINT('Ctrl Pts',(48.6558872405973,-42.0414910032139,
-234.887921662949));
#215165=CARTESIAN_POINT('Ctrl Pts',(48.6592992792251,-42.0353860410891,
-234.887630813131));
#215166=CARTESIAN_POINT('Ctrl Pts',(48.6632168889193,-42.0283198289059,
-234.887313508735));
#215167=CARTESIAN_POINT('Ctrl Pts',(48.6664055104559,-42.0225317772452,
-234.887064701553));
#215168=CARTESIAN_POINT('Ctrl Pts',(48.6667342919522,-42.0219349662835,
-234.887039046832));
#215169=CARTESIAN_POINT('Ctrl Pts',(48.6670553602036,-42.0213517167477,
-234.887014120362));
#215170=CARTESIAN_POINT('Ctrl Pts',(48.6673673861988,-42.0207844652683,
-234.886990026236));
#215171=CARTESIAN_POINT('Ctrl Pts',(48.6807199768326,-41.9965099596024,
-234.885958961507));
#215172=CARTESIAN_POINT('Ctrl Pts',(48.6938401681919,-41.9724057555076,
-234.884930841656));
#215173=CARTESIAN_POINT('Ctrl Pts',(48.7066812179049,-41.9485236867256,
-234.883905666796));
#215174=CARTESIAN_POINT('Ctrl Pts',(48.7131017427615,-41.9365826523345,
-234.883393079366));
#215175=CARTESIAN_POINT('Ctrl Pts',(48.7194524819989,-41.92469715167,-234.882881227964));
#215176=CARTESIAN_POINT('Ctrl Pts',(48.7257276051451,-41.9128736322774,
-234.882370112876));
#215177=CARTESIAN_POINT('Ctrl Pts',(48.7288651667182,-41.9069618725811,
-234.882114555332));
#215178=CARTESIAN_POINT('Ctrl Pts',(48.7319838242549,-41.901065608196,-234.881859181852));
#215179=CARTESIAN_POINT('Ctrl Pts',(48.7350828492338,-41.8951856441896,
-234.881603992432));
#215180=CARTESIAN_POINT('Ctrl Pts',(48.7366323617233,-41.8922456621864,
-234.881476397721));
#215181=CARTESIAN_POINT('Ctrl Pts',(48.7381769660725,-41.8893097552775,
-234.881348849025));
#215182=CARTESIAN_POINT('Ctrl Pts',(48.7397165712593,-41.8863780239848,
-234.881221346343));
#215183=CARTESIAN_POINT('Ctrl Pts',(48.7411462357431,-41.8836556428567,
-234.881102948421));
#215184=CARTESIAN_POINT('Ctrl Pts',(48.7432383291511,-41.8796630722582,
-234.880929090271));
#215185=CARTESIAN_POINT('Ctrl Pts',(48.7441353410803,-41.8779489284838,
-234.880854382132));
#215186=CARTESIAN_POINT('Ctrl Pts',(48.7442043209866,-41.8778171114219,
-234.880848637102));
#215187=CARTESIAN_POINT('Ctrl Pts',(48.7442662527949,-41.8776987516867,
-234.880843478401));
#215188=CARTESIAN_POINT('Ctrl Pts',(48.7443202983215,-41.8775954574424,
-234.880838976339));
#215189=CARTESIAN_POINT('Ctrl Pts',(48.7476473280508,-41.8712366883937,
-234.880561830447));
#215190=CARTESIAN_POINT('Ctrl Pts',(48.752120649118,-41.8628871264216,-234.880086152886));
#215191=CARTESIAN_POINT('Ctrl Pts',(48.7576520371428,-41.8526432824589,
-234.879415168295));
#215192=CARTESIAN_POINT('Ctrl Pts',(48.7629733267166,-41.8427885299392,
-234.878769669679));
#215193=CARTESIAN_POINT('Ctrl Pts',(48.7692740269242,-41.8311803879651,
-234.877943418939));
#215194=CARTESIAN_POINT('Ctrl Pts',(48.7764409233617,-41.8179366980267,
-234.876939287047));
#215195=CARTESIAN_POINT('Ctrl Pts',(48.7832004942317,-41.8054457039822,
-234.875992224293));
#215196=CARTESIAN_POINT('Ctrl Pts',(48.7907307080359,-41.7914996138868,
-234.874886925309));
#215197=CARTESIAN_POINT('Ctrl Pts',(48.7989031198614,-41.7762293180923,
-234.873625798856));
#215198=CARTESIAN_POINT('Ctrl Pts',(48.8024382459928,-41.7696238724967,
-234.873080275555));
#215199=CARTESIAN_POINT('Ctrl Pts',(48.8060930874268,-41.7627710843506,
-234.872505594547));
#215200=CARTESIAN_POINT('Ctrl Pts',(48.8098550401669,-41.7556837104237,
-234.871901950799));
#215201=CARTESIAN_POINT('Ctrl Pts',(48.8134774071706,-41.7488593106426,
-234.871320705007));
#215202=CARTESIAN_POINT('Ctrl Pts',(48.8171989254069,-41.7418176117972,
-234.870712605902));
#215203=CARTESIAN_POINT('Ctrl Pts',(48.8210118579088,-41.7345651533579,
-234.870077827541));
#215204=CARTESIAN_POINT('Ctrl Pts',(48.8301924033937,-41.7171031278577,
-234.868549447058));
#215205=CARTESIAN_POINT('Ctrl Pts',(48.8385003646315,-41.7010002940541,
-234.867138614139));
#215206=CARTESIAN_POINT('Ctrl Pts',(48.8460185003354,-41.6862191638892,
-234.865851393547));
#215207=CARTESIAN_POINT('Ctrl Pts',(48.8538337124274,-41.6708539627613,
-234.864513308903));
#215208=CARTESIAN_POINT('Ctrl Pts',(48.8607952956676,-41.6569173591826,
-234.863308798586));
#215209=CARTESIAN_POINT('Ctrl Pts',(48.8669592620571,-41.6444145134275,
-234.862244675083));
#215210=CARTESIAN_POINT('Ctrl Pts',(48.8737155325054,-41.6307102519249,
-234.861078298481));
#215211=CARTESIAN_POINT('Ctrl Pts',(48.8795135428262,-41.6187288760359,
-234.860080584889));
#215212=CARTESIAN_POINT('Ctrl Pts',(48.8843841498665,-41.6085277539861,
-234.859260505412));
#215213=CARTESIAN_POINT('Ctrl Pts',(48.8878940311451,-41.601176570241,-234.858669535625));
#215214=CARTESIAN_POINT('Ctrl Pts',(48.8909213502999,-41.5947510294145,
-234.858170811309));
#215215=CARTESIAN_POINT('Ctrl Pts',(48.8934661879285,-41.5892843316424,
-234.857767689636));
#215216=CARTESIAN_POINT('Ctrl Pts',(48.8976602145231,-41.5802749254691,
-234.857103323865));
#215217=CARTESIAN_POINT('Ctrl Pts',(48.9029891670216,-41.5686200787691,
-234.856310174717));
#215218=CARTESIAN_POINT('Ctrl Pts',(48.9093841848883,-41.5543296198375,
-234.855388242192));
#215219=CARTESIAN_POINT('Ctrl Pts',(48.9124409545253,-41.5474988897486,
-234.854947565495));
#215220=CARTESIAN_POINT('Ctrl Pts',(48.9157412142244,-41.5400655297535,
-234.854477464799));
#215221=CARTESIAN_POINT('Ctrl Pts',(48.9192785359752,-41.5320259773337,
-234.853977940102));
#215222=CARTESIAN_POINT('Ctrl Pts',(48.9245902297567,-41.5199536685074,
-234.853227846555));
#215223=CARTESIAN_POINT('Ctrl Pts',(48.9304354193403,-41.5065164174248,
-234.852411406412));
#215224=CARTESIAN_POINT('Ctrl Pts',(48.9368033953279,-41.4916782238494,
-234.851528619674));
#215225=CARTESIAN_POINT('Ctrl Pts',(48.9369918005099,-41.4912392158246,
-234.851502501235));
#215226=CARTESIAN_POINT('Ctrl Pts',(48.9371806647031,-41.4907989787993,
-234.851476324719));
#215227=CARTESIAN_POINT('Ctrl Pts',(48.9373699869613,-41.490357512501,-234.851450090126));
#215228=CARTESIAN_POINT('Ctrl Pts',(48.9406641343836,-41.482676138519,-234.850993616507));
#215229=CARTESIAN_POINT('Ctrl Pts',(48.9440970549571,-41.4746225678903,
-234.850519560243));
#215230=CARTESIAN_POINT('Ctrl Pts',(48.9476631731474,-41.4661955828763,
-234.850027921335));
#215231=CARTESIAN_POINT('Ctrl Pts',(48.9509358476483,-41.4584620256852,
-234.849576737714));
#215232=CARTESIAN_POINT('Ctrl Pts',(48.9547586284399,-41.4493659192662,
-234.849050547871));
#215233=CARTESIAN_POINT('Ctrl Pts',(48.9579205074998,-41.4417921180272,
-234.84861508577));
#215234=CARTESIAN_POINT('Ctrl Pts',(48.9582040167386,-41.4411130146892,
-234.84857604015));
#215235=CARTESIAN_POINT('Ctrl Pts',(48.9584822446429,-41.4404461645817,
-234.84853772396));
#215236=CARTESIAN_POINT('Ctrl Pts',(48.9587543366942,-41.4397936549064,
-234.848500256676));
#215237=CARTESIAN_POINT('Ctrl Pts',(48.9702361796019,-41.4122588057559,
-234.846919198117));
#215238=CARTESIAN_POINT('Ctrl Pts',(48.9805781788196,-41.3871430599868,
-234.845367224494));
#215239=CARTESIAN_POINT('Ctrl Pts',(48.9898477853363,-41.3645095999571,
-234.843844335809));
#215240=CARTESIAN_POINT('Ctrl Pts',(48.9912563407676,-41.3610703511607,
-234.843612926512));
#215241=CARTESIAN_POINT('Ctrl Pts',(48.992640183932,-41.3576883348653,-234.843382188788));
#215242=CARTESIAN_POINT('Ctrl Pts',(48.9939995973888,-41.3543636888088,
-234.843152122637));
#215243=CARTESIAN_POINT('Ctrl Pts',(48.9991524073963,-41.3417617321442,
-234.842280064797));
#215244=CARTESIAN_POINT('Ctrl Pts',(49.0039541458915,-41.3299843043351,
-234.841417655873));
#215245=CARTESIAN_POINT('Ctrl Pts',(49.008420983189,-41.3190366856309,-234.840564895866));
#215246=CARTESIAN_POINT('Ctrl Pts',(49.0120206385271,-41.3102144135211,
-234.839877688809));
#215247=CARTESIAN_POINT('Ctrl Pts',(49.0157608335646,-41.3010650320092,
-234.839119020287));
#215248=CARTESIAN_POINT('Ctrl Pts',(49.0187841251101,-41.2936834024839,
-234.838476803518));
#215249=CARTESIAN_POINT('Ctrl Pts',(49.0195124570307,-41.291905116689,-234.83832208904));
#215250=CARTESIAN_POINT('Ctrl Pts',(49.0201994351696,-41.2902294274288,
-234.838174132974));
#215251=CARTESIAN_POINT('Ctrl Pts',(49.0208334887382,-41.2886856196551,
-234.838035562593));
#215252=CARTESIAN_POINT('Ctrl Pts',(49.0254665777583,-41.2774048711525,
-234.837023015798));
#215253=CARTESIAN_POINT('Ctrl Pts',(49.0310689340646,-41.2637691132399,
-234.835742021356));
#215254=CARTESIAN_POINT('Ctrl Pts',(49.0375460910749,-41.2477860244353,
-234.834192579268));
#215255=CARTESIAN_POINT('Ctrl Pts',(49.0400028112789,-41.2417238003564,
-234.833604891541));
#215256=CARTESIAN_POINT('Ctrl Pts',(49.0425849033903,-41.235324028244,-234.832978584714));
#215257=CARTESIAN_POINT('Ctrl Pts',(49.0452852787953,-41.2285877985872,
-234.832313658788));
#215258=CARTESIAN_POINT('Ctrl Pts',(49.0455029061471,-41.2280449156167,
-234.832260071398));
#215259=CARTESIAN_POINT('Ctrl Pts',(49.0457213010957,-41.2274998476253,
-234.832206233178));
#215260=CARTESIAN_POINT('Ctrl Pts',(49.0459404605559,-41.2269525940909,
-234.832152144127));
#215261=CARTESIAN_POINT('Ctrl Pts',(49.0515466236979,-41.2129536884977,
-234.830768530369));
#215262=CARTESIAN_POINT('Ctrl Pts',(49.0578395655724,-41.1970562046521,
-234.829172346469));
#215263=CARTESIAN_POINT('Ctrl Pts',(49.0644525702741,-41.1800234821052,
-234.827444186758));
#215264=CARTESIAN_POINT('Ctrl Pts',(49.0697631798137,-41.1663452612475,
-234.826056378664));
#215265=CARTESIAN_POINT('Ctrl Pts',(49.0752808972514,-41.1519341090171,
-234.824583459623));
#215266=CARTESIAN_POINT('Ctrl Pts',(49.0808392958684,-41.1371776680563,
-234.823067168547));
#215267=CARTESIAN_POINT('Ctrl Pts',(49.0893164404596,-41.1146725380187,
-234.820754664608));
#215268=CARTESIAN_POINT('Ctrl Pts',(49.0968873906078,-41.0938932734194,
-234.818663052831));
#215269=CARTESIAN_POINT('Ctrl Pts',(49.1036612384437,-41.0748331083061,
-234.816792333217));
#215270=CARTESIAN_POINT('Ctrl Pts',(49.1068597766085,-41.0658331031365,
-234.815908999516));
#215271=CARTESIAN_POINT('Ctrl Pts',(49.109879986753,-41.0572169829317,-234.815074916526));
#215272=CARTESIAN_POINT('Ctrl Pts',(49.112730460048,-41.0489865939022,-234.814290084247));
#215273=CARTESIAN_POINT('Ctrl Pts',(49.117174055609,-41.036156261402,-234.813066611206));
#215274=CARTESIAN_POINT('Ctrl Pts',(49.1212055212028,-41.0242631572238,
-234.811962825292));
#215275=CARTESIAN_POINT('Ctrl Pts',(49.1248501216751,-41.0133192130477,
-234.810978749706));
#215276=CARTESIAN_POINT('Ctrl Pts',(49.1266724219112,-41.0078472409597,
-234.810486711913));
#215277=CARTESIAN_POINT('Ctrl Pts',(49.1283979454193,-41.0026125435169,
-234.810024549733));
#215278=CARTESIAN_POINT('Ctrl Pts',(49.1300290541854,-40.9976170734923,
-234.809592343969));
#215279=CARTESIAN_POINT('Ctrl Pts',(49.1314605616382,-40.9932329068943,
-234.809213027896));
#215280=CARTESIAN_POINT('Ctrl Pts',(49.1323831615919,-40.990393026695,-234.808969007844));
#215281=CARTESIAN_POINT('Ctrl Pts',(49.1339469038135,-40.9855179929412,
-234.808564744256));
#215282=CARTESIAN_POINT('Ctrl Pts',(49.1341649431961,-40.984838245771,-234.808508376025));
#215283=CARTESIAN_POINT('Ctrl Pts',(49.1343953996984,-40.9841188682892,
-234.808448892349));
#215284=CARTESIAN_POINT('Ctrl Pts',(49.1346413371297,-40.9833500834446,
-234.808385492057));
#215285=CARTESIAN_POINT('Ctrl Pts',(49.1362450929454,-40.9783368442662,
-234.807972059316));
#215286=CARTESIAN_POINT('Ctrl Pts',(49.1378471491999,-40.9733180924222,
-234.807552694279));
#215287=CARTESIAN_POINT('Ctrl Pts',(49.1394478251217,-40.9682932030464,
-234.807127396947));
#215288=CARTESIAN_POINT('Ctrl Pts',(49.153894351016,-40.9229422400596,-234.803288975409));
#215289=CARTESIAN_POINT('Ctrl Pts',(49.1682293317435,-40.8770918568449,
-234.798967336173));
#215290=CARTESIAN_POINT('Ctrl Pts',(49.1823259261447,-40.8304162239187,
-234.794162479238));
#215291=CARTESIAN_POINT('Ctrl Pts',(49.1901551750911,-40.8044925760139,
-234.791493861555));
#215292=CARTESIAN_POINT('Ctrl Pts',(49.1979107030446,-40.7783142410855,
-234.788676186103));
#215293=CARTESIAN_POINT('Ctrl Pts',(49.2055692912838,-40.7518248496597,
-234.785709456672));
#215294=CARTESIAN_POINT('Ctrl Pts',(49.2093985854034,-40.7385801539468,
-234.784226091957));
#215295=CARTESIAN_POINT('Ctrl Pts',(49.2132036340421,-40.7252576920657,
-234.782705455196));
#215296=CARTESIAN_POINT('Ctrl Pts',(49.2169814186128,-40.7118504077679,
-234.781147559695));
#215297=CARTESIAN_POINT('Ctrl Pts',(49.2185774997028,-40.7061859468821,
-234.780489362409));
#215298=CARTESIAN_POINT('Ctrl Pts',(49.2202313157489,-40.7002861074153,
-234.779797710544));
#215299=CARTESIAN_POINT('Ctrl Pts',(49.2218625039109,-40.6944280582757,
-234.779106576097));
#215300=CARTESIAN_POINT('Ctrl Pts',(49.2240921956936,-40.686420616625,-234.778161855658));
#215301=CARTESIAN_POINT('Ctrl Pts',(49.226279145818,-40.6784902613952,-234.777218101989));
#215302=CARTESIAN_POINT('Ctrl Pts',(49.2282305670252,-40.671366518235,-234.776362079861));
#215303=CARTESIAN_POINT('Ctrl Pts',(49.24174670062,-40.6220253181418,-234.770433011646));
#215304=CARTESIAN_POINT('Ctrl Pts',(49.2545091663963,-40.5712328733757,
-234.764537276227));
#215305=CARTESIAN_POINT('Ctrl Pts',(49.2665542178985,-40.5185843252109,
-234.758674858163));
#215306=CARTESIAN_POINT('Ctrl Pts',(49.2725767436496,-40.4922600511286,
-234.755743649131));
#215307=CARTESIAN_POINT('Ctrl Pts',(49.2784199545212,-40.4654717565139,
-234.752820799011));
#215308=CARTESIAN_POINT('Ctrl Pts',(49.2840885951191,-40.438170148677,-234.749906269699));
#215309=CARTESIAN_POINT('Ctrl Pts',(49.286922915418,-40.4245193447585,-234.748449005043));
#215310=CARTESIAN_POINT('Ctrl Pts',(49.289713595599,-40.4107402129128,-234.746993822495));
#215311=CARTESIAN_POINT('Ctrl Pts',(49.2924612425713,-40.3968266306292,
-234.745540722148));
#215312=CARTESIAN_POINT('Ctrl Pts',(49.2925978596127,-40.396134826891,-234.745468471865));
#215313=CARTESIAN_POINT('Ctrl Pts',(49.2927343702682,-40.3954426907519,
-234.745396226733));
#215314=CARTESIAN_POINT('Ctrl Pts',(49.2928707746132,-40.3947502214547,
-234.745323986752));
#215315=CARTESIAN_POINT('Ctrl Pts',(49.2941060548759,-40.3884792067363,
-234.744669780156));
#215316=CARTESIAN_POINT('Ctrl Pts',(49.2953326163964,-40.3821808691388,
-234.744015996031));
#215317=CARTESIAN_POINT('Ctrl Pts',(49.2965499595654,-40.3758501094821,
-234.743362635016));
#215318=CARTESIAN_POINT('Ctrl Pts',(49.2972258429813,-40.3723351963735,
-234.742999881204));
#215319=CARTESIAN_POINT('Ctrl Pts',(49.2978988843611,-40.3688103024198,
-234.742637256271));
#215320=CARTESIAN_POINT('Ctrl Pts',(49.2985689987828,-40.3652745392547,
-234.742274762142));
#215321=CARTESIAN_POINT('Ctrl Pts',(49.2989040559936,-40.3635066576721,
-234.742093515077));
#215322=CARTESIAN_POINT('Ctrl Pts',(49.299238381464,-40.361736058786,-234.741912300712));
#215323=CARTESIAN_POINT('Ctrl Pts',(49.2995719644862,-40.3599626349555,
-234.741731118898));
#215324=CARTESIAN_POINT('Ctrl Pts',(49.2999055475083,-40.3581892111249,
-234.741549937085));
#215325=CARTESIAN_POINT('Ctrl Pts',(49.300482383806,-40.3551057375624,-234.741235715341));
#215326=CARTESIAN_POINT('Ctrl Pts',(49.3005704755418,-40.3546337796992,
-234.741187671114));
#215327=CARTESIAN_POINT('Ctrl Pts',(49.301449545857,-40.3499240967321,-234.740708236199));
#215328=CARTESIAN_POINT('Ctrl Pts',(49.3026877797277,-40.3436857853011,
-234.739965356228));
#215329=CARTESIAN_POINT('Ctrl Pts',(49.3042704770971,-40.3358544197516,
-234.738959031199));
#215330=CARTESIAN_POINT('Ctrl Pts',(49.3057384845081,-40.3285905530845,
-234.738025629382));
#215331=CARTESIAN_POINT('Ctrl Pts',(49.3075028611123,-40.3199567707358,
-234.73686558014));
#215332=CARTESIAN_POINT('Ctrl Pts',(49.3095444690461,-40.3098592240976,
-234.735478883472));
#215333=CARTESIAN_POINT('Ctrl Pts',(49.3113961043595,-40.3007012591306,
-234.734221219611));
#215334=CARTESIAN_POINT('Ctrl Pts',(49.3134757704784,-40.2903395683248,
-234.732777125229));
#215335=CARTESIAN_POINT('Ctrl Pts',(49.3157628185814,-40.2786619114353,
-234.731146600328));
#215336=CARTESIAN_POINT('Ctrl Pts',(49.3169535045081,-40.272582274677,-234.730297714356));
#215337=CARTESIAN_POINT('Ctrl Pts',(49.3182002924174,-40.2661452034528,
-234.729398297039));
#215338=CARTESIAN_POINT('Ctrl Pts',(49.3194994819158,-40.2593291615188,
-234.728448348378));
#215339=CARTESIAN_POINT('Ctrl Pts',(49.32187762862,-40.2468524999698,-234.726709481738));
#215340=CARTESIAN_POINT('Ctrl Pts',(49.3244318189892,-40.2331097150377,
-234.724801300995));
#215341=CARTESIAN_POINT('Ctrl Pts',(49.3271338197985,-40.2179260150997,
-234.72272380615));
#215342=CARTESIAN_POINT('Ctrl Pts',(49.3295407090787,-40.2044006732534,
-234.720873214523));
#215343=CARTESIAN_POINT('Ctrl Pts',(49.3320648414618,-40.1897317952828,
-234.718888273905));
#215344=CARTESIAN_POINT('Ctrl Pts',(49.3346806252661,-40.1737501501656,
-234.716768984295));
#215345=CARTESIAN_POINT('Ctrl Pts',(49.3372028738137,-40.1583399770777,
-234.714725476292));
#215346=CARTESIAN_POINT('Ctrl Pts',(49.3398103617817,-40.1417095765092,
-234.712557055623));
#215347=CARTESIAN_POINT('Ctrl Pts',(49.3424746028141,-40.1236602909776,
-234.710263722287));
#215348=CARTESIAN_POINT('Ctrl Pts',(49.3450122884389,-40.1064683733255,
-234.708079325693));
#215349=CARTESIAN_POINT('Ctrl Pts',(49.3476014713131,-40.0879893317989,
-234.705781601654));
#215350=CARTESIAN_POINT('Ctrl Pts',(49.3502121977989,-40.0680047616935,
-234.703370550173));
#215351=CARTESIAN_POINT('Ctrl Pts',(49.3515912773287,-40.0574481937443,
-234.702096946154));
#215352=CARTESIAN_POINT('Ctrl Pts',(49.352976276403,-40.0464707209573,-234.700791720017));
#215353=CARTESIAN_POINT('Ctrl Pts',(49.3543621196709,-40.0350342300919,
-234.69945487176));
#215354=CARTESIAN_POINT('Ctrl Pts',(48.4015825627194,-42.4301635567087,
-234.916111528175));
#215355=CARTESIAN_POINT('Ctrl Pts',(48.0316514259825,-42.1949218242413,
-235.35005));
#215356=CARTESIAN_POINT('Ctrl Pts',(47.5111404700569,-41.8639253579254,
-235.35005));
#215357=CARTESIAN_POINT('Ctrl Pts',(47.0743964923321,-44.5052610020243,
-234.922474108526));
#215358=CARTESIAN_POINT('Ctrl Pts',(46.7171148693285,-44.2522653739478,
-235.350049999732));
#215359=CARTESIAN_POINT('Ctrl Pts',(46.213538446068,-43.9044790762502,-235.35005));
#215360=CARTESIAN_POINT('Ctrl Pts',(45.629301810778,-46.4737259710815,-234.928556938652));
#215361=CARTESIAN_POINT('Ctrl Pts',(45.2835112520428,-46.2075181206225,
-235.350050000331));
#215362=CARTESIAN_POINT('Ctrl Pts',(44.7999466948037,-45.8404400906418,
-235.35005));
#215363=CARTESIAN_POINT('Ctrl Pts',(42.5086646561594,-50.2018332312079,
-234.936094455435));
#215364=CARTESIAN_POINT('Ctrl Pts',(42.1882337316621,-49.9076193249785,
-235.350049999669));
#215365=CARTESIAN_POINT('Ctrl Pts',(41.7430470430268,-49.5044128120585,
-235.35005));
#215366=CARTESIAN_POINT('Ctrl Pts',(40.8389768825302,-51.962002922669,-234.93759503995));
#215367=CARTESIAN_POINT('Ctrl Pts',(40.5293161951324,-51.6569873869132,
-235.350049999933));
#215368=CARTESIAN_POINT('Ctrl Pts',(40.1030327246601,-51.2355371590317,
-235.35005));
#215369=CARTESIAN_POINT('Ctrl Pts',(38.1562303218321,-54.4502282641876,
-234.936060246629));
#215370=CARTESIAN_POINT('Ctrl Pts',(37.8678859707896,-54.1250209801684,
-235.350050000033));
#215371=CARTESIAN_POINT('Ctrl Pts',(37.4698285345256,-53.6756545350797,
-235.35005));
#215372=CARTESIAN_POINT('Ctrl Pts',(37.2328209647283,-55.2522203973821,
-234.934954372966));
#215373=CARTESIAN_POINT('Ctrl Pts',(36.9511651975887,-54.9208963823306,
-235.350050000067));
#215374=CARTESIAN_POINT('Ctrl Pts',(36.5624534933628,-54.4622301034484,
-235.35005));
#215375=CARTESIAN_POINT('Ctrl Pts',(35.3284631493583,-56.8039921969795,
-234.93163892731));
#215376=CARTESIAN_POINT('Ctrl Pts',(35.0607726001854,-56.4604474243018,
-235.350049999933));
#215377=CARTESIAN_POINT('Ctrl Pts',(34.6902365366833,-55.9834272130437,
-235.35005));
#215378=CARTESIAN_POINT('Ctrl Pts',(34.3488682961681,-57.5524285204314,
-234.929428785626));
#215379=CARTESIAN_POINT('Ctrl Pts',(34.0879972243562,-57.2030837074672,
-235.35005000005));
#215380=CARTESIAN_POINT('Ctrl Pts',(33.7267628103062,-56.7166866533048,
-235.35005));
#215381=CARTESIAN_POINT('Ctrl Pts',(31.3507316578327,-59.6945695123404,
-234.920814246822));
#215382=CARTESIAN_POINT('Ctrl Pts',(31.1105534689003,-59.3284635730008,
-235.3500499999));
#215383=CARTESIAN_POINT('Ctrl Pts',(30.7793083468736,-58.8119074053918,
-235.35005));
#215384=CARTESIAN_POINT('Ctrl Pts',(29.2648462613946,-60.9897453716254,
-234.912770791881));
#215385=CARTESIAN_POINT('Ctrl Pts',(29.0391623276262,-60.6125303361456,
-235.350050001106));
#215386=CARTESIAN_POINT('Ctrl Pts',(28.7279549137639,-60.0762241747571,
-235.35005));
#215387=CARTESIAN_POINT('Ctrl Pts',(27.0930165135311,-62.1526330725429,
-234.905475377596));
#215388=CARTESIAN_POINT('Ctrl Pts',(26.8863570828206,-61.7639375806376,
-235.35005));
#215389=CARTESIAN_POINT('Ctrl Pts',(26.5926469327274,-61.2115127003622,
-235.35005));
#215390=CARTESIAN_POINT('',(27.0930165135311,-62.1526330725429,-234.905475377596));
#215391=CARTESIAN_POINT('',(26.5926469327273,-61.2115127003622,-235.35005));
#215392=CARTESIAN_POINT('Origin',(26.5926469327274,-61.2115127003622,-233.85005));
#215393=CARTESIAN_POINT('Ctrl Pts',(47.511140470057,-41.8639253579254,-235.35005));
#215394=CARTESIAN_POINT('Ctrl Pts',(46.5263591620664,-43.4125505315973,
-235.35005));
#215395=CARTESIAN_POINT('Ctrl Pts',(45.4748377912596,-44.9008380775653,
-235.35005));
#215396=CARTESIAN_POINT('Ctrl Pts',(44.3570056200731,-46.3291760712338,
-235.35005));
#215397=CARTESIAN_POINT('Ctrl Pts',(44.0018587501823,-46.7829738600906,
-235.35005));
#215398=CARTESIAN_POINT('Ctrl Pts',(43.6400181829326,-47.2307200839806,
-235.35005));
#215399=CARTESIAN_POINT('Ctrl Pts',(43.2714968690733,-47.6724264514822,
-235.35005));
#215400=CARTESIAN_POINT('Ctrl Pts',(41.7430470430284,-49.5044128120552,
-235.35005));
#215401=CARTESIAN_POINT('Ctrl Pts',(40.1030327246406,-51.2355371590496,
-235.35005));
#215402=CARTESIAN_POINT('Ctrl Pts',(38.3475632646338,-52.8622820764655,
-235.35005));
#215403=CARTESIAN_POINT('Ctrl Pts',(37.4698285346305,-53.6756545351735,
-235.35005));
#215404=CARTESIAN_POINT('Ctrl Pts',(36.5624534933633,-54.462230103448,-235.35005));
#215405=CARTESIAN_POINT('Ctrl Pts',(35.626345015024,-55.2228286582473,-235.35005));
#215406=CARTESIAN_POINT('Ctrl Pts',(34.6902365366847,-55.9834272130465,
-235.35005));
#215407=CARTESIAN_POINT('Ctrl Pts',(33.7267628103146,-56.7166866532988,
-235.35005));
#215408=CARTESIAN_POINT('Ctrl Pts',(32.7442779891666,-57.4150935706736,
-235.35005));
#215409=CARTESIAN_POINT('Ctrl Pts',(30.9377005462611,-58.6993130881051,
-235.35005));
#215410=CARTESIAN_POINT('Ctrl Pts',(29.0581394327502,-59.8715157745109,
-235.35005));
#215411=CARTESIAN_POINT('Ctrl Pts',(27.107386123889,-60.934451225102,-235.35005));
#215412=CARTESIAN_POINT('Ctrl Pts',(26.9363532637854,-61.0276443979109,
-235.35005));
#215413=CARTESIAN_POINT('Ctrl Pts',(26.7647731343724,-61.1199976105731,
-235.35005));
#215414=CARTESIAN_POINT('Ctrl Pts',(26.5926469327274,-61.2115127003622,
-235.35005));
#215415=CARTESIAN_POINT('Ctrl Pts',(27.0930165135311,-62.1526330725429,
-234.905475377596));
#215416=CARTESIAN_POINT('Ctrl Pts',(27.5718634056311,-61.8962384288525,
-234.907084021714));
#215417=CARTESIAN_POINT('Ctrl Pts',(28.0545166383205,-61.6291332678087,
-234.908756275144));
#215418=CARTESIAN_POINT('Ctrl Pts',(28.5399619314692,-61.3510080909548,
-234.910457848288));
#215419=CARTESIAN_POINT('Ctrl Pts',(29.0121022833342,-61.0805056868413,
-234.912112785217));
#215420=CARTESIAN_POINT('Ctrl Pts',(29.4868836627188,-60.7995789487944,
-234.913795406111));
#215421=CARTESIAN_POINT('Ctrl Pts',(29.9633988567347,-60.5079852690017,
-234.915468296034));
#215422=CARTESIAN_POINT('Ctrl Pts',(30.0374913798313,-60.4626458722182,
-234.915728410794));
#215423=CARTESIAN_POINT('Ctrl Pts',(30.1116258743564,-60.4170486717776,
-234.915988279334));
#215424=CARTESIAN_POINT('Ctrl Pts',(30.1857989902024,-60.3711928529312,
-234.916247749045));
#215425=CARTESIAN_POINT('Ctrl Pts',(30.6507245319281,-60.0837633553934,
-234.917874134755));
#215426=CARTESIAN_POINT('Ctrl Pts',(31.1171631399868,-59.7861707844739,
-234.919485158613));
#215427=CARTESIAN_POINT('Ctrl Pts',(31.5843037844726,-59.4782406979995,
-234.921040433439));
#215428=CARTESIAN_POINT('Ctrl Pts',(31.87201222967,-59.2885888501998,-234.921998315625));
#215429=CARTESIAN_POINT('Ctrl Pts',(32.1599873997248,-59.0950166566419,
-234.922934957828));
#215430=CARTESIAN_POINT('Ctrl Pts',(32.4480464998279,-58.8974909316072,
-234.923840099263));
#215431=CARTESIAN_POINT('Ctrl Pts',(32.6348129815887,-58.7694228209008,
-234.924426958283));
#215432=CARTESIAN_POINT('Ctrl Pts',(32.821614887809,-58.6396928444983,-234.92500056282));
#215433=CARTESIAN_POINT('Ctrl Pts',(33.0084035159985,-58.5082933347905,
-234.925557985548));
#215434=CARTESIAN_POINT('Ctrl Pts',(33.1097081454347,-58.4370289394787,
-234.925860303218));
#215435=CARTESIAN_POINT('Ctrl Pts',(33.2110100103575,-58.365272666291,-234.92615786251));
#215436=CARTESIAN_POINT('Ctrl Pts',(33.3122940517528,-58.2930287462961,
-234.926450163542));
#215437=CARTESIAN_POINT('Ctrl Pts',(33.316387149019,-58.2901092203041,-234.92646197603));
#215438=CARTESIAN_POINT('Ctrl Pts',(33.321463602919,-58.2864870754898,-234.926476613876));
#215439=CARTESIAN_POINT('Ctrl Pts',(33.3245722526722,-58.2842663723945,
-234.92648725201));
#215440=CARTESIAN_POINT('Ctrl Pts',(33.3328657245494,-58.278341826328,-234.926515633166));
#215441=CARTESIAN_POINT('Ctrl Pts',(33.341168468048,-58.2724073561477,-234.926543964589));
#215442=CARTESIAN_POINT('Ctrl Pts',(33.3494804760251,-58.2664629403962,
-234.926572246023));
#215443=CARTESIAN_POINT('Ctrl Pts',(33.5646083444542,-58.1126120907339,
-234.927304214122));
#215444=CARTESIAN_POINT('Ctrl Pts',(33.7860387420253,-57.9520450780028,
-234.927998708321));
#215445=CARTESIAN_POINT('Ctrl Pts',(34.0135675131175,-57.7844501465415,
-234.928655297153));
#215446=CARTESIAN_POINT('Ctrl Pts',(34.235288686026,-57.6211330214203,-234.929295126768));
#215447=CARTESIAN_POINT('Ctrl Pts',(34.4628010919038,-57.451141894775,-234.929898956642));
#215448=CARTESIAN_POINT('Ctrl Pts',(34.6958680422294,-57.2741939857683,
-234.930466305562));
#215449=CARTESIAN_POINT('Ctrl Pts',(34.9199081829414,-57.104099365415,-234.93101168075));
#215450=CARTESIAN_POINT('Ctrl Pts',(35.1490810038441,-56.9275761879985,
-234.931523341738));
#215451=CARTESIAN_POINT('Ctrl Pts',(35.3831297990818,-56.7443821331988,
-234.932000850011));
#215452=CARTESIAN_POINT('Ctrl Pts',(35.5724418873646,-56.5962042755007,
-234.932387086088));
#215453=CARTESIAN_POINT('Ctrl Pts',(35.7649433100188,-56.4436620936211,
-234.932750976463));
#215454=CARTESIAN_POINT('Ctrl Pts',(35.960473894234,-56.2866333907678,-234.933092313615));
#215455=CARTESIAN_POINT('Ctrl Pts',(36.0662372035414,-56.2016959098275,
-234.933276944305));
#215456=CARTESIAN_POINT('Ctrl Pts',(36.1728989271569,-56.1154340648653,
-234.93345627913));
#215457=CARTESIAN_POINT('Ctrl Pts',(36.2804224686007,-56.0278360381834,
-234.933630086089));
#215458=CARTESIAN_POINT('Ctrl Pts',(36.5772019915719,-55.7860536319977,
-234.934109816813));
#215459=CARTESIAN_POINT('Ctrl Pts',(36.8804171401314,-55.534226139737,-234.934547586812));
#215460=CARTESIAN_POINT('Ctrl Pts',(37.1894567165655,-55.2718686224767,
-234.934933522473));
#215461=CARTESIAN_POINT('Ctrl Pts',(37.2748942546821,-55.1993368754436,
-234.935040218817));
#215462=CARTESIAN_POINT('Ctrl Pts',(37.3607767694189,-55.1260000686736,
-234.935142946982));
#215463=CARTESIAN_POINT('Ctrl Pts',(37.4470909107402,-55.0518474005779,
-234.935241483442));
#215464=CARTESIAN_POINT('Ctrl Pts',(37.7029102456755,-54.832072448924,-234.935533527494));
#215465=CARTESIAN_POINT('Ctrl Pts',(37.9624741146055,-54.6051743831383,
-234.935786928809));
#215466=CARTESIAN_POINT('Ctrl Pts',(38.2252850299414,-54.3709827841254,
-234.936003250157));
#215467=CARTESIAN_POINT('Ctrl Pts',(38.3566904876093,-54.253886984619,-234.936111410831));
#215468=CARTESIAN_POINT('Ctrl Pts',(38.4889066221193,-54.1349682821895,
-234.936210475769));
#215469=CARTESIAN_POINT('Ctrl Pts',(38.6218645904408,-54.0142085592077,
-234.936301926129));
#215470=CARTESIAN_POINT('Ctrl Pts',(38.6883435746016,-53.9538286977168,
-234.936347651309));
#215471=CARTESIAN_POINT('Ctrl Pts',(38.755008016081,-53.8929885788722,-234.936391470356));
#215472=CARTESIAN_POINT('Ctrl Pts',(38.8218488051652,-53.8316862034097,
-234.936433688495));
#215473=CARTESIAN_POINT('Ctrl Pts',(38.8552691997073,-53.8010350156784,
-234.936454797565));
#215474=CARTESIAN_POINT('Ctrl Pts',(38.8887336811994,-53.7702682637168,
-234.936475506388));
#215475=CARTESIAN_POINT('Ctrl Pts',(38.9222410962122,-53.7393857057027,
-234.936495856913));
#215476=CARTESIAN_POINT('Ctrl Pts',(38.9389948037186,-53.7239444266957,
-234.936506032176));
#215477=CARTESIAN_POINT('Ctrl Pts',(38.9557592446103,-53.708474196172,-234.936516117866));
#215478=CARTESIAN_POINT('Ctrl Pts',(38.9725342729942,-53.69297498485,-234.936526119693));
#215479=CARTESIAN_POINT('Ctrl Pts',(38.9809217871861,-53.685225379189,-234.936531120606));
#215480=CARTESIAN_POINT('Ctrl Pts',(38.9893119482516,-53.6774685283282,
-234.936536100554));
#215481=CARTESIAN_POINT('Ctrl Pts',(38.9977047378706,-53.6697044286973,
-234.936541060243));
#215482=CARTESIAN_POINT('Ctrl Pts',(39.0039993300848,-53.6638813539741,
-234.93654478001));
#215483=CARTESIAN_POINT('Ctrl Pts',(39.0102954008607,-53.6580542018176,
-234.936548488382));
#215484=CARTESIAN_POINT('Ctrl Pts',(39.0165929428998,-53.6522229713257,
-234.936552184957));
#215485=CARTESIAN_POINT('Ctrl Pts',(39.0186921235795,-53.6502792278285,
-234.936553417148));
#215486=CARTESIAN_POINT('Ctrl Pts',(39.0216364393619,-53.6475523824562,
-234.936555143819));
#215487=CARTESIAN_POINT('Ctrl Pts',(39.0228909745786,-53.6463903808042,
-234.9365558783));
#215488=CARTESIAN_POINT('Ctrl Pts',(39.0320742480229,-53.6378844586339,
-234.936561254746));
#215489=CARTESIAN_POINT('Ctrl Pts',(39.0412703185288,-53.6293609283746,
-234.936566595268));
#215490=CARTESIAN_POINT('Ctrl Pts',(39.0504791367371,-53.6208197752944,
-234.93657189854));
#215491=CARTESIAN_POINT('Ctrl Pts',(39.3274433571275,-53.363936237084,-234.936731399627));
#215492=CARTESIAN_POINT('Ctrl Pts',(39.6158887006704,-53.0913151175466,
-234.936853712323));
#215493=CARTESIAN_POINT('Ctrl Pts',(39.9144891613816,-52.8026211254396,
-234.936903652261));
#215494=CARTESIAN_POINT('Ctrl Pts',(40.2324498159691,-52.4952092397139,
-234.936956830128));
#215495=CARTESIAN_POINT('Ctrl Pts',(40.561924137625,-52.1695726799131,-234.936927935723));
#215496=CARTESIAN_POINT('Ctrl Pts',(40.9012922354414,-51.8252513187329,
-234.936774253452));
#215497=CARTESIAN_POINT('Ctrl Pts',(40.9738029689377,-51.7516822513449,
-234.936741417089));
#215498=CARTESIAN_POINT('Ctrl Pts',(41.0467653441068,-51.6772599921148,
-234.936702883362));
#215499=CARTESIAN_POINT('Ctrl Pts',(41.1201635288383,-51.6019797568265,
-234.936658234884));
#215500=CARTESIAN_POINT('Ctrl Pts',(41.3966959063802,-51.3183566328712,
-234.936490018876));
#215501=CARTESIAN_POINT('Ctrl Pts',(41.6794226629877,-51.0225062183936,
-234.936257951047));
#215502=CARTESIAN_POINT('Ctrl Pts',(41.967065292056,-50.7146281499219,-234.935948979951));
#215503=CARTESIAN_POINT('Ctrl Pts',(42.2375329352271,-50.425133314496,-234.935658457352));
#215504=CARTESIAN_POINT('Ctrl Pts',(42.5123468242956,-50.1250040109044,
-234.935299940635));
#215505=CARTESIAN_POINT('Ctrl Pts',(42.7904844944196,-49.8144264272255,
-234.934863512671));
#215506=CARTESIAN_POINT('Ctrl Pts',(43.0190718299255,-49.5591783614407,
-234.934504834519));
#215507=CARTESIAN_POINT('Ctrl Pts',(43.2499047920019,-49.2968734040297,
-234.934093547199));
#215508=CARTESIAN_POINT('Ctrl Pts',(43.4824389229629,-49.0276279049742,
-234.933624664599));
#215509=CARTESIAN_POINT('Ctrl Pts',(43.6769491609346,-48.8024093279093,
-234.933232453504));
#215510=CARTESIAN_POINT('Ctrl Pts',(43.8725744141091,-48.5724217941096,
-234.932800098487));
#215511=CARTESIAN_POINT('Ctrl Pts',(44.0689832334687,-48.3377796011447,
-234.932325697043));
#215512=CARTESIAN_POINT('Ctrl Pts',(44.3317420558166,-48.0238715673934,
-234.931691035294));
#215513=CARTESIAN_POINT('Ctrl Pts',(44.5957361857819,-47.7016164793283,
-234.930979638848));
#215514=CARTESIAN_POINT('Ctrl Pts',(44.8601324618043,-47.3713165826379,
-234.930197051073));
#215515=CARTESIAN_POINT('Ctrl Pts',(45.1173862882891,-47.0499394679923,
-234.929435604267));
#215516=CARTESIAN_POINT('Ctrl Pts',(45.3750207433328,-46.7209462483979,
-234.928606783073));
#215517=CARTESIAN_POINT('Ctrl Pts',(45.6323048563377,-46.3846485512081,
-234.927718070288));
#215518=CARTESIAN_POINT('Ctrl Pts',(45.7425217833411,-46.2405833063328,
-234.927337358121));
#215519=CARTESIAN_POINT('Ctrl Pts',(45.8526748883602,-46.0951780116808,
-234.926945683224));
#215520=CARTESIAN_POINT('Ctrl Pts',(45.962708890812,-45.9484591535881,-234.926543756567));
#215521=CARTESIAN_POINT('Ctrl Pts',(46.1928389583745,-45.6416047270182,
-234.925703149056));
#215522=CARTESIAN_POINT('Ctrl Pts',(46.4224725107643,-45.3289660350924,
-234.92481754019));
#215523=CARTESIAN_POINT('Ctrl Pts',(46.6510236316563,-45.0109435350599,
-234.923894778246));
#215524=CARTESIAN_POINT('Ctrl Pts',(46.8773755380714,-44.6959811805359,
-234.922980895504));
#215525=CARTESIAN_POINT('Ctrl Pts',(47.1026656676339,-44.375738062674,-234.922030588858));
#215526=CARTESIAN_POINT('Ctrl Pts',(47.3263623726596,-44.0506372276144,
-234.921052672002));
#215527=CARTESIAN_POINT('Ctrl Pts',(47.5474575032212,-43.7293172887939,
-234.92008612824));
#215528=CARTESIAN_POINT('Ctrl Pts',(47.7669960212512,-43.4032519354286,
-234.919092631132));
#215529=CARTESIAN_POINT('Ctrl Pts',(47.9845022423295,-43.0728837348188,
-234.918081590818));
#215530=CARTESIAN_POINT('Ctrl Pts',(48.1244084772295,-42.8603814401771,
-234.917431260712));
#215531=CARTESIAN_POINT('Ctrl Pts',(48.2634746257799,-42.6460995632716,
-234.916773689743));
#215532=CARTESIAN_POINT('Ctrl Pts',(48.4015825627194,-42.4301635567087,
-234.916111528175));
#215533=CARTESIAN_POINT('Ctrl Pts',(27.2453371921567,-62.0684961123336,
-234.910710085558));
#215534=CARTESIAN_POINT('Ctrl Pts',(27.0364433475168,-61.680487024444,-235.350050000041));
#215535=CARTESIAN_POINT('Ctrl Pts',(26.7410849731316,-61.1326062593409,
-235.35005));
#215536=CARTESIAN_POINT('Ctrl Pts',(27.1368513731105,-62.1258987971579,
-234.905003039976));
#215537=CARTESIAN_POINT('Ctrl Pts',(26.9274704864059,-61.7399494328241,
-235.350049999987));
#215538=CARTESIAN_POINT('Ctrl Pts',(26.6293474091419,-61.1908379190527,
-235.35005));
#215539=CARTESIAN_POINT('Ctrl Pts',(27.0227991977541,-62.194936761442,-234.90610242041));
#215540=CARTESIAN_POINT('Ctrl Pts',(26.8144283136556,-61.8059798077595,
-235.350049999995));
#215541=CARTESIAN_POINT('Ctrl Pts',(26.5194896368383,-61.2532914016042,
-235.35005));
#215542=CARTESIAN_POINT('Ctrl Pts',(26.8369281750275,-62.3093205660776,
-234.878288708869));
#215543=CARTESIAN_POINT('Ctrl Pts',(26.6548033201846,-61.9041872098222,
-235.350050000001));
#215544=CARTESIAN_POINT('Ctrl Pts',(26.3891388204284,-61.3131722991992,
-235.35005));
#215545=CARTESIAN_POINT('Ctrl Pts',(26.8144498855472,-62.3225830053421,
-234.875056610216));
#215546=CARTESIAN_POINT('Ctrl Pts',(26.6353007694942,-61.9157019040657,
-235.350050000004));
#215547=CARTESIAN_POINT('Ctrl Pts',(26.3731447836042,-61.3202661527697,
-235.35005));
#215548=CARTESIAN_POINT('Ctrl Pts',(26.7749796776064,-62.3432491826028,
-234.871626009621));
#215549=CARTESIAN_POINT('Ctrl Pts',(26.5991763051683,-61.9344632905112,
-235.350049999996));
#215550=CARTESIAN_POINT('Ctrl Pts',(26.341052548261,-61.3342311248494,-235.35005));
#215551=CARTESIAN_POINT('Ctrl Pts',(26.7581168332245,-62.3505983495205,
-234.871489925227));
#215552=CARTESIAN_POINT('Ctrl Pts',(26.5826449857937,-61.9416583310242,
-235.350050000003));
#215553=CARTESIAN_POINT('Ctrl Pts',(26.324963993434,-61.3411228649431,-235.35005));
#215554=CARTESIAN_POINT('Ctrl Pts',(26.7067367940551,-62.3734047916896,
-234.870670602159));
#215555=CARTESIAN_POINT('Ctrl Pts',(26.5326026130778,-61.9637882105777,
-235.350049999995));
#215556=CARTESIAN_POINT('Ctrl Pts',(26.2766869482483,-61.3617737493097,
-235.35005));
#215557=CARTESIAN_POINT('Ctrl Pts',(26.6716855174712,-62.3892096482857,
-234.8697429112));
#215558=CARTESIAN_POINT('Ctrl Pts',(26.4987789702316,-61.9789513787255,
-235.350049999998));
#215559=CARTESIAN_POINT('Ctrl Pts',(26.2444517981386,-61.3754399401447,
-235.35005));
#215560=CARTESIAN_POINT('Ctrl Pts',(26.5986640911394,-62.42280983363,-234.866517684792));
#215561=CARTESIAN_POINT('Ctrl Pts',(26.4294605199159,-62.0106164563224,
-235.350050000002));
#215562=CARTESIAN_POINT('Ctrl Pts',(26.1797908377429,-61.4023344685258,
-235.35005));
#215563=CARTESIAN_POINT('Ctrl Pts',(26.5610650568712,-62.4403313244474,
-234.864401737979));
#215564=CARTESIAN_POINT('Ctrl Pts',(26.3941508721394,-62.0269255784061,
-235.350050000003));
#215565=CARTESIAN_POINT('Ctrl Pts',(26.1473795281051,-61.4155758832315,
-235.35005));
#215566=CARTESIAN_POINT('Ctrl Pts',(26.4769925160474,-62.4815712743123,
-234.855888967911));
#215567=CARTESIAN_POINT('Ctrl Pts',(26.3184924821692,-62.0639340677589,
-235.350049999997));
#215568=CARTESIAN_POINT('Ctrl Pts',(26.0821804763413,-61.4411000467081,
-235.35005));
#215569=CARTESIAN_POINT('Ctrl Pts',(26.4301202849281,-62.5051629518579,
-234.849380577206));
#215570=CARTESIAN_POINT('Ctrl Pts',(26.2778418840239,-62.0845719406398,
-235.350050000008));
#215571=CARTESIAN_POINT('Ctrl Pts',(26.0493312864126,-61.4532499966124,
-235.350050000001));
#215572=CARTESIAN_POINT('Ctrl Pts',(26.3002982623345,-62.5629144928957,
-234.836228995997));
#215573=CARTESIAN_POINT('Ctrl Pts',(26.16131341017,-62.1365284085563,-235.350049999985));
#215574=CARTESIAN_POINT('Ctrl Pts',(25.9501566901715,-61.4879342004266,
-235.350050000001));
#215575=CARTESIAN_POINT('Ctrl Pts',(26.2295575379109,-62.5856716502435,
-234.836161050761));
#215576=CARTESIAN_POINT('Ctrl Pts',(26.0922007161114,-62.1587949666646,
-235.350049999986));
#215577=CARTESIAN_POINT('Ctrl Pts',(25.8834819572284,-61.509419252042,-235.35005));
#215578=CARTESIAN_POINT('Ctrl Pts',(26.1240410793217,-62.6259950512244,
-234.826760990814));
#215579=CARTESIAN_POINT('Ctrl Pts',(25.9961215559071,-62.1956472548967,
-235.350050000004));
#215580=CARTESIAN_POINT('Ctrl Pts',(25.7996807895498,-61.534730893345,-235.35005));
#215581=CARTESIAN_POINT('Ctrl Pts',(26.1022708897306,-62.6344209388075,
-234.824528171248));
#215582=CARTESIAN_POINT('Ctrl Pts',(25.9764874702381,-62.203301257273,-235.35005000001));
#215583=CARTESIAN_POINT('Ctrl Pts',(25.7828903569215,-61.5396828918313,
-235.35005));
#215584=CARTESIAN_POINT('Ctrl Pts',(26.0564405135317,-62.6525017477888,
-234.818855409686));
#215585=CARTESIAN_POINT('Ctrl Pts',(25.9358759255667,-62.2195777671254,
-235.35004999999));
#215586=CARTESIAN_POINT('Ctrl Pts',(25.7492255098059,-61.5492800686396,
-235.35005));
#215587=CARTESIAN_POINT('Ctrl Pts',(26.031750683035,-62.662585347949,-234.815081952429));
#215588=CARTESIAN_POINT('Ctrl Pts',(25.9145289583069,-62.2285531296847,
-235.350050000002));
#215589=CARTESIAN_POINT('Ctrl Pts',(25.7323477164287,-61.5539129022783,
-235.35005));
#215590=CARTESIAN_POINT('Ctrl Pts',(25.9599138929427,-62.6902172126436,
-234.80493035963));
#215591=CARTESIAN_POINT('Ctrl Pts',(25.8516066550585,-62.253415598874,-235.350049999996));
#215592=CARTESIAN_POINT('Ctrl Pts',(25.6815605387409,-61.5672495175189,
-235.35005));
#215593=CARTESIAN_POINT('Ctrl Pts',(25.9137933010533,-62.7061668420416,
-234.799088724657));
#215594=CARTESIAN_POINT('Ctrl Pts',(25.8105734511642,-62.2679937524898,
-235.350050000001));
#215595=CARTESIAN_POINT('Ctrl Pts',(25.6474983161402,-61.5754339876196,
-235.35005));
#215596=CARTESIAN_POINT('Ctrl Pts',(25.8266199989672,-62.7334072231405,
-234.790014747185));
#215597=CARTESIAN_POINT('Ctrl Pts',(25.731270624734,-62.2932633630891,-235.350049999999));
#215598=CARTESIAN_POINT('Ctrl Pts',(25.5791807904238,-61.5908730316921,
-235.35005));
#215599=CARTESIAN_POINT('Ctrl Pts',(25.7854381790837,-62.7449250317595,
-234.786716919552));
#215600=CARTESIAN_POINT('Ctrl Pts',(25.6929582970791,-62.3041171818887,
-235.350050000007));
#215601=CARTESIAN_POINT('Ctrl Pts',(25.5449390466137,-61.5981933980485,
-235.35005));
#215602=CARTESIAN_POINT('Ctrl Pts',(25.6958511722237,-62.7713816730825,
-234.776088976192));
#215603=CARTESIAN_POINT('Ctrl Pts',(25.6120006673653,-62.3287974984487,
-235.350049999993));
#215604=CARTESIAN_POINT('Ctrl Pts',(25.4762602753847,-61.6118947761917,
-235.35005));
#215605=CARTESIAN_POINT('Ctrl Pts',(25.6487938388611,-62.7853359206876,
-234.769502178759));
#215606=CARTESIAN_POINT('Ctrl Pts',(25.5700865112867,-62.3418086817178,
-235.350049999994));
#215607=CARTESIAN_POINT('Ctrl Pts',(25.441793602875,-61.6182439225594,-235.35005));
#215608=CARTESIAN_POINT('Ctrl Pts',(25.5505975885659,-62.8135734388872,
-234.753817940405));
#215609=CARTESIAN_POINT('Ctrl Pts',(25.4836760281485,-62.3684020864125,
-235.350050000006));
#215610=CARTESIAN_POINT('Ctrl Pts',(25.3727171465013,-61.6295518156141,
-235.35005));
#215611=CARTESIAN_POINT('Ctrl Pts',(25.502761747094,-62.8258892566092,-234.746546441306));
#215612=CARTESIAN_POINT('Ctrl Pts',(25.4411294647291,-62.3802077997125,
-235.350050000011));
#215613=CARTESIAN_POINT('Ctrl Pts',(25.3381059806223,-61.6345074287981,
-235.35005));
#215614=CARTESIAN_POINT('Ctrl Pts',(25.410643515485,-62.8470998764316,-234.733871650706));
#215615=CARTESIAN_POINT('Ctrl Pts',(25.3580077967086,-62.4008089763377,
-235.350049999988));
#215616=CARTESIAN_POINT('Ctrl Pts',(25.2687752030225,-61.6433803535082,
-235.35005));
#215617=CARTESIAN_POINT('Ctrl Pts',(25.3675251946155,-62.8554316040649,
-234.729139544076));
#215618=CARTESIAN_POINT('Ctrl Pts',(25.3181720881824,-62.409019950067,-235.350049999987));
#215619=CARTESIAN_POINT('Ctrl Pts',(25.2340567625657,-61.647308878831,-235.35005));
#215620=CARTESIAN_POINT('Ctrl Pts',(25.2771548984166,-62.8731739889417,
-234.717216506631));
#215621=CARTESIAN_POINT('Ctrl Pts',(25.2358632414137,-62.4266817100688,
-235.350050000013));
#215622=CARTESIAN_POINT('Ctrl Pts',(25.1645355171699,-61.6543581913618,
-235.35005));
#215623=CARTESIAN_POINT('Ctrl Pts',(25.2265358924182,-62.8840570732042,
-234.708065708185));
#215624=CARTESIAN_POINT('Ctrl Pts',(25.1912608438073,-62.4376905785948,
-235.350049999998));
#215625=CARTESIAN_POINT('Ctrl Pts',(25.1297211288812,-61.6573680755603,
-235.350050000001));
#215626=CARTESIAN_POINT('Ctrl Pts',(25.0487310537601,-62.917065316072,-234.677362912941));
#215627=CARTESIAN_POINT('Ctrl Pts',(25.0325598226048,-62.4721861510005,
-235.350050000007));
#215628=CARTESIAN_POINT('Ctrl Pts',(25.0041328693965,-61.6657481959627,
-235.350050000001));
#215629=CARTESIAN_POINT('Ctrl Pts',(24.9305963304298,-62.9289465193204,
-234.661234678933));
#215630=CARTESIAN_POINT('Ctrl Pts',(24.9242386165759,-62.4861572040979,
-235.350050000174));
#215631=CARTESIAN_POINT('Ctrl Pts',(24.9129804805611,-61.6674900659302,
-235.350049999997));
#215632=CARTESIAN_POINT('Ctrl Pts',(24.8442395506814,-62.9300850046651,
-234.661061515112));
#215633=CARTESIAN_POINT('Ctrl Pts',(24.8365458571667,-62.4875347473503,
-235.350049999113));
#215634=CARTESIAN_POINT('Ctrl Pts',(24.8217422065604,-61.6684388365039,
-235.350050000008));
#215635=CARTESIAN_POINT('',(25.0347190704488,-62.9143710634153,-234.678897682319));
#215636=CARTESIAN_POINT('',(24.9899997248189,-61.6649665253882,-235.35005));
#215637=CARTESIAN_POINT('Origin',(24.9899997248189,-61.6649665253882,-233.85005));
#215638=CARTESIAN_POINT('Ctrl Pts',(26.5926469327273,-61.2115127003622,
-235.35005));
#215639=CARTESIAN_POINT('Ctrl Pts',(26.5307857619515,-61.2444027172302,
-235.35005));
#215640=CARTESIAN_POINT('Ctrl Pts',(26.4686189787879,-61.276660497005,-235.35005));
#215641=CARTESIAN_POINT('Ctrl Pts',(26.4050352616636,-61.3058697511684,
-235.35005));
#215642=CARTESIAN_POINT('Ctrl Pts',(26.3891387194065,-61.3131723462998,
-235.35005));
#215643=CARTESIAN_POINT('Ctrl Pts',(26.3731446870696,-61.3202661956383,
-235.35005));
#215644=CARTESIAN_POINT('Ctrl Pts',(26.3570986663275,-61.327248639717,-235.35005));
#215645=CARTESIAN_POINT('Ctrl Pts',(26.3410524626378,-61.3342311634055,
-235.35005));
#215646=CARTESIAN_POINT('Ctrl Pts',(26.3249639130519,-61.3411229008801,
-235.35005));
#215647=CARTESIAN_POINT('Ctrl Pts',(26.3088716457128,-61.3480064946411,
-235.35005));
#215648=CARTESIAN_POINT('Ctrl Pts',(26.2766866901153,-61.3617738622147,
-235.35005));
#215649=CARTESIAN_POINT('Ctrl Pts',(26.2444515824955,-61.3754400331407,
-235.35005));
#215650=CARTESIAN_POINT('Ctrl Pts',(26.212121319506,-61.3888872080985,-235.35005));
#215651=CARTESIAN_POINT('Ctrl Pts',(26.1797907095899,-61.4023345273539,
-235.35005));
#215652=CARTESIAN_POINT('Ctrl Pts',(26.1473794430666,-61.4155759233805,
-235.350049999999));
#215653=CARTESIAN_POINT('Ctrl Pts',(26.1147800051491,-61.4283379724439,
-235.350049999999));
#215654=CARTESIAN_POINT('Ctrl Pts',(26.0821804798061,-61.4411000557326,
-235.35005));
#215655=CARTESIAN_POINT('Ctrl Pts',(26.0493313347784,-61.4532499920652,
-235.350050000001));
#215656=CARTESIAN_POINT('Ctrl Pts',(26.0162730923146,-61.464811411177,-235.350050000001));
#215657=CARTESIAN_POINT('Ctrl Pts',(25.9501574057461,-61.4879339701914,
-235.350050000001));
#215658=CARTESIAN_POINT('Ctrl Pts',(25.8834830443658,-61.5094189499966,
-235.35005));
#215659=CARTESIAN_POINT('Ctrl Pts',(25.816441032895,-61.5296685975531,-235.35005));
#215660=CARTESIAN_POINT('Ctrl Pts',(25.799680801709,-61.5347309273823,-235.35005));
#215661=CARTESIAN_POINT('Ctrl Pts',(25.7828903692931,-61.5396829277202,
-235.35005));
#215662=CARTESIAN_POINT('Ctrl Pts',(25.7660579441618,-61.5444815181131,
-235.35005));
#215663=CARTESIAN_POINT('Ctrl Pts',(25.7492255222735,-61.5492801075815,
-235.35005));
#215664=CARTESIAN_POINT('Ctrl Pts',(25.7323477287723,-61.5539129424998,
-235.35005));
#215665=CARTESIAN_POINT('Ctrl Pts',(25.7154186680902,-61.558358482165,-235.35005));
#215666=CARTESIAN_POINT('Ctrl Pts',(25.6815605534858,-61.5672495597203,
-235.35005));
#215667=CARTESIAN_POINT('Ctrl Pts',(25.6474983294595,-61.5754340306918,
-235.35005));
#215668=CARTESIAN_POINT('Ctrl Pts',(25.6133395630491,-61.5831535528751,
-235.35005));
#215669=CARTESIAN_POINT('Ctrl Pts',(25.5791808006497,-61.590873074152,-235.35005));
#215670=CARTESIAN_POINT('Ctrl Pts',(25.5449390551878,-61.5981934391817,
-235.35005));
#215671=CARTESIAN_POINT('Ctrl Pts',(25.510599668782,-61.6050441261316,-235.35005));
#215672=CARTESIAN_POINT('Ctrl Pts',(25.4762602802774,-61.6118948135003,
-235.35005));
#215673=CARTESIAN_POINT('Ctrl Pts',(25.4417936057803,-61.6182439572411,
-235.35005));
#215674=CARTESIAN_POINT('Ctrl Pts',(25.4072553797815,-61.6238979002003,
-235.35005));
#215675=CARTESIAN_POINT('Ctrl Pts',(25.3727171455055,-61.6295518445145,
-235.35005));
#215676=CARTESIAN_POINT('Ctrl Pts',(25.3381059777677,-61.6345074541881,
-235.35005));
#215677=CARTESIAN_POINT('Ctrl Pts',(25.3034405945236,-61.6389439122599,
-235.35005));
#215678=CARTESIAN_POINT('Ctrl Pts',(25.2687751967828,-61.6433803721869,
-235.35005));
#215679=CARTESIAN_POINT('Ctrl Pts',(25.234056754758,-61.6473088938803,-235.35005));
#215680=CARTESIAN_POINT('Ctrl Pts',(25.1992961409817,-61.6508335460814,
-235.35005));
#215681=CARTESIAN_POINT('Ctrl Pts',(25.1645355064627,-61.6543582003856,
-235.35005));
#215682=CARTESIAN_POINT('Ctrl Pts',(25.1297211167782,-61.6573680815383,
-235.350050000001));
#215683=CARTESIAN_POINT('Ctrl Pts',(25.0948355014582,-61.6596958899581,
-235.350050000001));
#215684=CARTESIAN_POINT('Ctrl Pts',(25.0599498590945,-61.6620237001823,
-235.350050000001));
#215685=CARTESIAN_POINT('Ctrl Pts',(25.0249976982331,-61.6637138708522,
-235.35005));
#215686=CARTESIAN_POINT('Ctrl Pts',(24.9899997248189,-61.6649665253882,
-235.35005));
#215687=CARTESIAN_POINT('Ctrl Pts',(25.0347190704488,-62.9143710634153,
-234.678897682319));
#215688=CARTESIAN_POINT('Ctrl Pts',(25.085638797075,-62.9079339622688,-234.685853660663));
#215689=CARTESIAN_POINT('Ctrl Pts',(25.1307592161118,-62.9007252008369,
-234.693073023235));
#215690=CARTESIAN_POINT('Ctrl Pts',(25.2129670148129,-62.8850210310273,
-234.708038516839));
#215691=CARTESIAN_POINT('Ctrl Pts',(25.2539844298917,-62.8766122328458,
-234.715332558096));
#215692=CARTESIAN_POINT('Ctrl Pts',(25.3485821128302,-62.8579473644628,
-234.728553576946));
#215693=CARTESIAN_POINT('Ctrl Pts',(25.3980516305474,-62.8481335841612,
-234.734457037752));
#215694=CARTESIAN_POINT('Ctrl Pts',(25.4895958658201,-62.8274748181031,
-234.746824327757));
#215695=CARTESIAN_POINT('Ctrl Pts',(25.533635925427,-62.8165570077274,-234.753066555306));
#215696=CARTESIAN_POINT('Ctrl Pts',(25.5975770701915,-62.7992049833544,
-234.762517770449));
#215697=CARTESIAN_POINT('Ctrl Pts',(25.6185393383981,-62.7932542900658,
-234.765682821134));
#215698=CARTESIAN_POINT('Ctrl Pts',(25.6443444802103,-62.7856261939461,
-234.769657441535));
#215699=CARTESIAN_POINT('Ctrl Pts',(25.6484523849535,-62.7843918496431,
-234.770299887365));
#215700=CARTESIAN_POINT('Ctrl Pts',(25.652628706954,-62.7831642653728,-234.770916217284));
#215701=CARTESIAN_POINT('Ctrl Pts',(25.6597400602254,-62.7811052939532,
-234.771918572547));
#215702=CARTESIAN_POINT('Ctrl Pts',(25.6693705433464,-62.7783833175895,
-234.773154508962));
#215703=CARTESIAN_POINT('Ctrl Pts',(25.7069387835634,-62.7677747710471,
-234.77779336624));
#215704=CARTESIAN_POINT('Ctrl Pts',(25.7545226931024,-62.7543762597918,
-234.78316547359));
#215705=CARTESIAN_POINT('Ctrl Pts',(25.833006557455,-62.730226116854,-234.791956884686));
#215706=CARTESIAN_POINT('Ctrl Pts',(25.8496500291877,-62.7250326332926,
-234.793818980751));
#215707=CARTESIAN_POINT('Ctrl Pts',(25.8760257651527,-62.7166320351824,
-234.796767845616));
#215708=CARTESIAN_POINT('Ctrl Pts',(25.8811350256815,-62.7149847988613,
-234.797339569667));
#215709=CARTESIAN_POINT('Ctrl Pts',(25.8921320345629,-62.7114127360742,
-234.79858954494));
#215710=CARTESIAN_POINT('Ctrl Pts',(25.9195496279942,-62.7024190863312,
-234.801742188854));
#215711=CARTESIAN_POINT('Ctrl Pts',(25.9682935210718,-62.6856232102758,
-234.807666299498));
#215712=CARTESIAN_POINT('Ctrl Pts',(26.0111347436968,-62.6696270999718,
-234.813286809008));
#215713=CARTESIAN_POINT('Ctrl Pts',(26.0432243998012,-62.6571545277768,
-234.81763517866));
#215714=CARTESIAN_POINT('Ctrl Pts',(26.053917370438,-62.6529155819281,-234.819106799797));
#215715=CARTESIAN_POINT('Ctrl Pts',(26.069946869197,-62.6464402766788,-234.821347478383));
#215716=CARTESIAN_POINT('Ctrl Pts',(26.0752878196045,-62.6442627279254,
-234.822099912391));
#215717=CARTESIAN_POINT('Ctrl Pts',(26.0859624874598,-62.6398716269047,
-234.823615862701));
#215718=CARTESIAN_POINT('Ctrl Pts',(26.0933426421007,-62.6368014947894,
-234.824674728087));
#215719=CARTESIAN_POINT('Ctrl Pts',(26.1097539748075,-62.629932182154,-234.827043269906));
#215720=CARTESIAN_POINT('Ctrl Pts',(26.127149009414,-62.623171180736,-234.828880694613));
#215721=CARTESIAN_POINT('Ctrl Pts',(26.1595790621099,-62.610935853299,-234.831550718551));
#215722=CARTESIAN_POINT('Ctrl Pts',(26.1773763976045,-62.6042947500805,
-234.83286420224));
#215723=CARTESIAN_POINT('Ctrl Pts',(26.2008584346582,-62.5956002463696,
-234.834358925386));
#215724=CARTESIAN_POINT('Ctrl Pts',(26.2114956462486,-62.5916697030229,
-234.834991447915));
#215725=CARTESIAN_POINT('Ctrl Pts',(26.2187133945384,-62.589003865943,-234.835411335577));
#215726=CARTESIAN_POINT('Ctrl Pts',(26.221061526754,-62.5881368485382,-234.835546593076));
#215727=CARTESIAN_POINT('Ctrl Pts',(26.2665871887173,-62.5713334384756,
-234.838084045232));
#215728=CARTESIAN_POINT('Ctrl Pts',(26.2972309978204,-62.5596102150849,
-234.83984397804));
#215729=CARTESIAN_POINT('Ctrl Pts',(26.3294801453437,-62.5471044172847,
-234.841740506921));
#215730=CARTESIAN_POINT('Ctrl Pts',(26.3379381999395,-62.5437783530276,
-234.842248788159));
#215731=CARTESIAN_POINT('Ctrl Pts',(26.347189205665,-62.5401070985879,-234.842825367435));
#215732=CARTESIAN_POINT('Ctrl Pts',(26.3509546787848,-62.5386010471326,
-234.843067196427));
#215733=CARTESIAN_POINT('Ctrl Pts',(26.3534261833428,-62.5375977021866,
-234.84323933445));
#215734=CARTESIAN_POINT('Ctrl Pts',(26.3547859197358,-62.5370411263274,
-234.84333860625));
#215735=CARTESIAN_POINT('Ctrl Pts',(26.3541676061889,-62.5373072030569,
-234.84327989792));
#215736=CARTESIAN_POINT('Ctrl Pts',(26.3680817365266,-62.5314220268562,
-234.844492646197));
#215737=CARTESIAN_POINT('Ctrl Pts',(26.3844680819482,-62.5242262989439,
-234.846153717548));
#215738=CARTESIAN_POINT('Ctrl Pts',(26.4155766034196,-62.5099916470183,
-234.849519933896));
#215739=CARTESIAN_POINT('Ctrl Pts',(26.427040628927,-62.5046685272578,-234.850787774233));
#215740=CARTESIAN_POINT('Ctrl Pts',(26.446033018801,-62.4956922588524,-234.852908187069));
#215741=CARTESIAN_POINT('Ctrl Pts',(26.4526640361999,-62.4925343615046,
-234.853651433403));
#215742=CARTESIAN_POINT('Ctrl Pts',(26.4665640540616,-62.4858586717679,
-234.85521081018));
#215743=CARTESIAN_POINT('Ctrl Pts',(26.4749973336765,-62.4817726451067,
-234.856157358164));
#215744=CARTESIAN_POINT('Ctrl Pts',(26.5072332853527,-62.466039545056,-234.85976813296));
#215745=CARTESIAN_POINT('Ctrl Pts',(26.5309786196337,-62.4543565533579,
-234.862139767001));
#215746=CARTESIAN_POINT('Ctrl Pts',(26.5624741628734,-62.4390041084162,
-234.864921739368));
#215747=CARTESIAN_POINT('Ctrl Pts',(26.5722895346858,-62.4342454913545,
-234.865719817041));
#215748=CARTESIAN_POINT('Ctrl Pts',(26.5859073445181,-62.4277104752076,
-234.866723063878));
#215749=CARTESIAN_POINT('Ctrl Pts',(26.5902627632415,-62.4256323661044,
-234.867025167878));
#215750=CARTESIAN_POINT('Ctrl Pts',(26.5985962243179,-62.4216846633567,
-234.867564752653));
#215751=CARTESIAN_POINT('Ctrl Pts',(26.6015303784991,-62.4203009685482,
-234.867745656129));
#215752=CARTESIAN_POINT('Ctrl Pts',(26.6449954022435,-62.400069202433,-234.870101374292));
#215753=CARTESIAN_POINT('Ctrl Pts',(26.688860555794,-62.3801117723142,-234.871572851604));
#215754=CARTESIAN_POINT('Ctrl Pts',(26.7775907302196,-62.3406277132562,
-234.873133640282));
#215755=CARTESIAN_POINT('Ctrl Pts',(26.8144719921791,-62.3216949396143,
-234.876263859502));
#215756=CARTESIAN_POINT('Ctrl Pts',(26.8975997530553,-62.2706957884666,
-234.888648102498));
#215757=CARTESIAN_POINT('Ctrl Pts',(26.9407411513415,-62.2442733553417,
-234.893662446297));
#215758=CARTESIAN_POINT('Ctrl Pts',(27.023757211477,-62.1938596418189,-234.901335578495));
#215759=CARTESIAN_POINT('Ctrl Pts',(27.06303730244,-62.1702331394993,-234.903994366895));
#215760=CARTESIAN_POINT('Ctrl Pts',(27.0930165135311,-62.1526330725429,
-234.905475377596));
#215761=CARTESIAN_POINT('Ctrl Pts',(25.0347190704499,-62.9143710634155,
-234.678897682318));
#215762=CARTESIAN_POINT('Ctrl Pts',(25.0188032481045,-62.4697021984296,
-235.35005));
#215763=CARTESIAN_POINT('Ctrl Pts',(24.9899997248189,-61.6649665253882,
-235.35005));
#215764=CARTESIAN_POINT('Ctrl Pts',(23.6367128243542,-62.9652114948589,
-234.677688363322));
#215765=CARTESIAN_POINT('Ctrl Pts',(23.6213321581711,-62.5206566084218,
-235.350050000019));
#215766=CARTESIAN_POINT('Ctrl Pts',(23.5944744924679,-61.7149158997446,
-235.35005));
#215767=CARTESIAN_POINT('Ctrl Pts',(22.2385723540716,-63.0117706699204,
-234.676581567471));
#215768=CARTESIAN_POINT('Ctrl Pts',(22.2241440176956,-62.567306445692,-235.350049999981));
#215769=CARTESIAN_POINT('Ctrl Pts',(22.1988114399884,-61.7606622187164,
-235.35005));
#215770=CARTESIAN_POINT('Ctrl Pts',(20.8402921969906,-63.0540783161444,
-234.675571538939));
#215771=CARTESIAN_POINT('Ctrl Pts',(20.8270581434285,-62.6096929286678,
-235.35005));
#215772=CARTESIAN_POINT('Ctrl Pts',(20.8030114294341,-61.8022299494809,
-235.35005));
#215773=CARTESIAN_POINT('',(20.8402919657626,-63.0540783750575,-234.675571454956));
#215774=CARTESIAN_POINT('',(20.803011429434,-61.8022299494809,-235.35005));
#215775=CARTESIAN_POINT('Origin',(20.803011429434,-61.802229949481,-233.85005));
#215776=CARTESIAN_POINT('Origin',(0.0402464096705391,635.45788043407,-235.35005));
#215777=CARTESIAN_POINT('Origin',(0.0417395060045145,624.033047422002,-250.70813398415));
#215778=CARTESIAN_POINT('Ctrl Pts',(20.9272939729598,-63.0388412169436,
-234.6925317176));
#215779=CARTESIAN_POINT('Ctrl Pts',(20.9003239325236,-62.593292071215,-235.350055395714));
#215780=CARTESIAN_POINT('Ctrl Pts',(20.8522739306831,-61.8000205942923,
-235.350049999965));
#215781=CARTESIAN_POINT('Ctrl Pts',(20.5781346200028,-63.1054079859869,
-234.625170203823));
#215782=CARTESIAN_POINT('Ctrl Pts',(20.6028008281919,-62.6639924158116,
-235.350056035508));
#215783=CARTESIAN_POINT('Ctrl Pts',(20.6549442779816,-61.8117755329686,
-235.350049999962));
#215784=CARTESIAN_POINT('Ctrl Pts',(20.242946602916,-63.1075402490427,-234.546724224386));
#215785=CARTESIAN_POINT('Ctrl Pts',(20.3103268001138,-62.6871623715535,
-235.35005680618));
#215786=CARTESIAN_POINT('Ctrl Pts',(20.4609420978131,-61.7877616583069,
-235.350049999958));
#215787=CARTESIAN_POINT('Ctrl Pts',(19.919830853961,-63.0620777407187,-234.460509579399));
#215788=CARTESIAN_POINT('Ctrl Pts',(20.0212058153521,-62.6789324639497,
-235.350057690633));
#215789=CARTESIAN_POINT('Ctrl Pts',(20.2703537543378,-61.7374827788075,
-235.350049999953));
#215790=CARTESIAN_POINT('',(20.00087676599,-63.0723813030746,-234.482033943277));
#215791=CARTESIAN_POINT('',(20.3180691938068,-61.7495111937247,-235.35005));
#215792=CARTESIAN_POINT('Origin',(20.3180691938068,-61.7495111937247,-233.85005));
#215793=CARTESIAN_POINT('Ctrl Pts',(20.803011429434,-61.8022299494809,-235.35005));
#215794=CARTESIAN_POINT('Ctrl Pts',(20.6389224043824,-61.8071166154417,
-235.35005));
#215795=CARTESIAN_POINT('Ctrl Pts',(20.4774719299468,-61.7877321350851,
-235.35005));
#215796=CARTESIAN_POINT('Ctrl Pts',(20.3180691938068,-61.7495111937247,
-235.35005));
#215797=CARTESIAN_POINT('Ctrl Pts',(20.0008767612649,-63.072381322781,-234.482033952692));
#215798=CARTESIAN_POINT('Ctrl Pts',(20.0757818263204,-63.0809990670768,
-234.501590108694));
#215799=CARTESIAN_POINT('Ctrl Pts',(20.1499241690099,-63.0867716849007,
-234.520358077193));
#215800=CARTESIAN_POINT('Ctrl Pts',(20.2230384024983,-63.0899033965466,
-234.53828908067));
#215801=CARTESIAN_POINT('Ctrl Pts',(20.2970171665463,-63.0930721387444,
-234.556432107166));
#215802=CARTESIAN_POINT('Ctrl Pts',(20.3699430474527,-63.0935377434988,
-234.573718420067));
#215803=CARTESIAN_POINT('Ctrl Pts',(20.4415762107852,-63.0915317581419,
-234.590133855307));
#215804=CARTESIAN_POINT('Ctrl Pts',(20.5148301934923,-63.0894803840323,
-234.606920717051));
#215805=CARTESIAN_POINT('Ctrl Pts',(20.586732029596,-63.0848449037923,-234.622797043541));
#215806=CARTESIAN_POINT('Ctrl Pts',(20.6570663042979,-63.0778846196563,
-234.637782820744));
#215807=CARTESIAN_POINT('Ctrl Pts',(20.7194133551344,-63.0717147516836,
-234.651066799531));
#215808=CARTESIAN_POINT('Ctrl Pts',(20.7805292610771,-63.0637185342414,
-234.663651683389));
#215809=CARTESIAN_POINT('Ctrl Pts',(20.8402917354589,-63.0540784607098,
-234.675571320208));
#215810=CARTESIAN_POINT('Ctrl Pts',(20.0002454535025,-63.0750142297972,
-234.47617280861));
#215811=CARTESIAN_POINT('Ctrl Pts',(20.0938415017253,-62.6846662779265,
-235.35005));
#215812=CARTESIAN_POINT('Ctrl Pts',(20.3180691938068,-61.7495111937247,
-235.35005));
#215813=CARTESIAN_POINT('Ctrl Pts',(19.2551174895925,-62.8664467612893,
-234.539479091859));
#215814=CARTESIAN_POINT('Ctrl Pts',(19.3413406300525,-62.4544294433442,
-235.350049999953));
#215815=CARTESIAN_POINT('Ctrl Pts',(19.4874388572759,-61.5503460219505,
-235.35005));
#215816=CARTESIAN_POINT('Ctrl Pts',(18.5025522393628,-62.7270802386455,
-234.590416060416));
#215817=CARTESIAN_POINT('Ctrl Pts',(18.5599245998347,-62.2978562023724,
-235.350049999989));
#215818=CARTESIAN_POINT('Ctrl Pts',(18.6516615360795,-61.4277914392832,
-235.35005));
#215819=CARTESIAN_POINT('Ctrl Pts',(16.981042115573,-62.595164303197,-234.672122377017));
#215820=CARTESIAN_POINT('Ctrl Pts',(16.9850135818407,-62.1499515126842,
-235.350050000011));
#215821=CARTESIAN_POINT('Ctrl Pts',(16.9698436721481,-61.3371563394037,
-235.35005));
#215822=CARTESIAN_POINT('Ctrl Pts',(16.2106145315025,-62.6026718111486,
-234.703184254722));
#215823=CARTESIAN_POINT('Ctrl Pts',(16.1826608962456,-62.1548361758855,
-235.350049999952));
#215824=CARTESIAN_POINT('Ctrl Pts',(16.121735346724,-61.369283189915,-235.35005));
#215825=CARTESIAN_POINT('Ctrl Pts',(15.0509341311275,-62.736562693307,-234.736945141873));
#215826=CARTESIAN_POINT('Ctrl Pts',(14.9766556245768,-62.2929910538471,
-235.350050000024));
#215827=CARTESIAN_POINT('Ctrl Pts',(14.8481785970025,-61.5432262204531,
-235.35005));
#215828=CARTESIAN_POINT('Ctrl Pts',(14.6645397729193,-62.8015403926739,
-234.745992774078));
#215829=CARTESIAN_POINT('Ctrl Pts',(14.5754142156998,-62.3603004171988,
-235.350050000024));
#215830=CARTESIAN_POINT('Ctrl Pts',(14.4244572553949,-61.622006959983,-235.35005));
#215831=CARTESIAN_POINT('Ctrl Pts',(14.254950802522,-62.8933063624506,-234.753437327716));
#215832=CARTESIAN_POINT('Ctrl Pts',(14.1497802084409,-62.455665562112,-235.350049999998));
#215833=CARTESIAN_POINT('Ctrl Pts',(13.9751463716102,-61.7290008746058,
-235.35005));
#215834=CARTESIAN_POINT('Ctrl Pts',(14.2240132142558,-62.9018295132189,
-234.751997072706));
#215835=CARTESIAN_POINT('Ctrl Pts',(14.120632865605,-62.4638031966455,-235.350050000002));
#215836=CARTESIAN_POINT('Ctrl Pts',(13.9487177749326,-61.7353325867798,
-235.35005));
#215837=CARTESIAN_POINT('Ctrl Pts',(14.1654272334655,-62.9170176450018,
-234.750024084914));
#215838=CARTESIAN_POINT('Ctrl Pts',(14.0643317181977,-62.4785194469356,
-235.350049999999));
#215839=CARTESIAN_POINT('Ctrl Pts',(13.8958479018872,-61.7476653413416,
-235.35005));
#215840=CARTESIAN_POINT('Ctrl Pts',(14.1361228513778,-62.9244932940189,
-234.749035483871));
#215841=CARTESIAN_POINT('Ctrl Pts',(14.0361704849244,-62.4857653670867,
-235.35005));
#215842=CARTESIAN_POINT('Ctrl Pts',(13.8694088478247,-61.7537243383813,
-235.35005));
#215843=CARTESIAN_POINT('Ctrl Pts',(14.0481763635734,-62.9465655811834,
-234.746063719071));
#215844=CARTESIAN_POINT('Ctrl Pts',(13.9516379184633,-62.50717186034,-235.350049999999));
#215845=CARTESIAN_POINT('Ctrl Pts',(13.7900793792485,-61.771580394972,-235.35005));
#215846=CARTESIAN_POINT('Ctrl Pts',(13.9895006559527,-62.9608076271989,
-234.744074583615));
#215847=CARTESIAN_POINT('Ctrl Pts',(13.8952521434001,-62.5209918829364,
-235.350050000002));
#215848=CARTESIAN_POINT('Ctrl Pts',(13.7371766585364,-61.7830565245145,
-235.35005));
#215849=CARTESIAN_POINT('Ctrl Pts',(13.8133459471977,-63.0021201512081,
-234.738086226961));
#215850=CARTESIAN_POINT('Ctrl Pts',(13.7259015486268,-62.5611319850931,
-235.350049999995));
#215851=CARTESIAN_POINT('Ctrl Pts',(13.5784196345718,-61.8162106597038,
-235.35005));
#215852=CARTESIAN_POINT('Ctrl Pts',(13.6957382843772,-63.0277772664849,
-234.734066004735));
#215853=CARTESIAN_POINT('Ctrl Pts',(13.6128816245493,-62.5860948115319,
-235.350050000005));
#215854=CARTESIAN_POINT('Ctrl Pts',(13.4725164724631,-61.8366144889431,
-235.35005));
#215855=CARTESIAN_POINT('Ctrl Pts',(13.3424531489291,-63.0991349765239,
-234.721945421981));
#215856=CARTESIAN_POINT('Ctrl Pts',(13.2730684458465,-62.6557423796767,
-235.350049999991));
#215857=CARTESIAN_POINT('Ctrl Pts',(13.154614345307,-61.8928021529216,-235.35005));
#215858=CARTESIAN_POINT('Ctrl Pts',(13.1063157328584,-63.1392203334766,
-234.713787004588));
#215859=CARTESIAN_POINT('Ctrl Pts',(13.0460848802442,-62.6950332686297,
-235.350050000015));
#215860=CARTESIAN_POINT('Ctrl Pts',(12.9424227890118,-61.9235634536356,
-235.35005));
#215861=CARTESIAN_POINT('Ctrl Pts',(11.9231858767189,-63.3028113134546,
-234.672904284763));
#215862=CARTESIAN_POINT('Ctrl Pts',(11.9024438740355,-62.8576130316748,
-235.35004999994));
#215863=CARTESIAN_POINT('Ctrl Pts',(11.880215388165,-62.0447815017487,-235.35005));
#215864=CARTESIAN_POINT('Ctrl Pts',(10.9664919615506,-63.3177886529725,
-234.639295809699));
#215865=CARTESIAN_POINT('Ctrl Pts',(10.9815452295666,-62.8759003715857,
-235.350049999988));
#215866=CARTESIAN_POINT('Ctrl Pts',(11.0264981771774,-62.0387113664218,
-235.35005));
#215867=CARTESIAN_POINT('Ctrl Pts',(9.76047598411976,-63.1848698641477,
-234.598624589264));
#215868=CARTESIAN_POINT('Ctrl Pts',(9.82464543906513,-62.7568110742575,
-235.350050000003));
#215869=CARTESIAN_POINT('Ctrl Pts',(9.9542943769832,-61.8992361752613,-235.35005));
#215870=CARTESIAN_POINT('Ctrl Pts',(9.51868087246522,-63.1506217143349,
-234.590521575213));
#215871=CARTESIAN_POINT('Ctrl Pts',(9.59134079921566,-62.7255327835753,
-235.350049999985));
#215872=CARTESIAN_POINT('Ctrl Pts',(9.73959722556094,-61.864654779516,-235.35005));
#215873=CARTESIAN_POINT('Ctrl Pts',(9.1552088910392,-63.0872746466928,-234.578477639126));
#215874=CARTESIAN_POINT('Ctrl Pts',(9.24074450396521,-62.6672453065271,
-235.350050000007));
#215875=CARTESIAN_POINT('Ctrl Pts',(9.41715218707317,-61.8023691603538,
-235.35005));
#215876=CARTESIAN_POINT('Ctrl Pts',(9.03392287836112,-63.0641627844476,
-234.574481372606));
#215877=CARTESIAN_POINT('Ctrl Pts',(9.12361630525094,-62.6458843797158,
-235.350049999991));
#215878=CARTESIAN_POINT('Ctrl Pts',(9.30960392193887,-61.7798708192789,
-235.35005));
#215879=CARTESIAN_POINT('Ctrl Pts',(8.88216619994883,-63.0327225023551,
-234.569514805913));
#215880=CARTESIAN_POINT('Ctrl Pts',(8.97711320863088,-62.6167596520512,
-235.350050000002));
#215881=CARTESIAN_POINT('Ctrl Pts',(9.17508354831589,-61.7495301015501,
-235.35005));
#215882=CARTESIAN_POINT('Ctrl Pts',(8.85180758078057,-63.0263069459882,
-234.568522933821));
#215883=CARTESIAN_POINT('Ctrl Pts',(8.9477835000243,-62.6108083839332,-235.350050000001));
#215884=CARTESIAN_POINT('Ctrl Pts',(9.14817522070154,-61.7433510482094,
-235.35005));
#215885=CARTESIAN_POINT('Ctrl Pts',(8.8062587329115,-63.0164912333735,-234.567037380941));
#215886=CARTESIAN_POINT('Ctrl Pts',(8.90377970937159,-62.6016978624724,
-235.35005));
#215887=CARTESIAN_POINT('Ctrl Pts',(9.10780631361874,-61.7339151558469,
-235.35005));
#215888=CARTESIAN_POINT('Ctrl Pts',(8.78987315391243,-63.013132382654,-234.566105822447));
#215889=CARTESIAN_POINT('Ctrl Pts',(8.88825779030318,-62.5987600395459,
-235.350050000003));
#215890=CARTESIAN_POINT('Ctrl Pts',(9.09434840397257,-61.7307279424447,
-235.35005));
#215891=CARTESIAN_POINT('Ctrl Pts',(8.7656898169978,-63.0067092336391,-234.567370926259));
#215892=CARTESIAN_POINT('Ctrl Pts',(8.86330821605581,-62.5918614567545,
-235.350049999997));
#215893=CARTESIAN_POINT('Ctrl Pts',(9.06743306640637,-61.7243660786321,
-235.35005));
#215894=CARTESIAN_POINT('Ctrl Pts',(8.75359794781792,-63.0035181040683,
-234.56800033754));
#215895=CARTESIAN_POINT('Ctrl Pts',(8.85083241058327,-62.5884344265496,
-235.350049999999));
#215896=CARTESIAN_POINT('Ctrl Pts',(9.05397622529392,-61.7212067312174,
-235.35005));
#215897=CARTESIAN_POINT('Ctrl Pts',(8.69313745814224,-62.9876644929304,
-234.571131795369));
#215898=CARTESIAN_POINT('Ctrl Pts',(8.78847489870271,-62.5714176461548,
-235.350050000005));
#215899=CARTESIAN_POINT('Ctrl Pts',(8.98669614980007,-61.7055177010037,
-235.35005));
#215900=CARTESIAN_POINT('Ctrl Pts',(8.64476611487728,-62.9753083012394,
-234.573587012594));
#215901=CARTESIAN_POINT('Ctrl Pts',(8.7385510630932,-62.5581533934216,-235.350050000003));
#215902=CARTESIAN_POINT('Ctrl Pts',(8.93288530505372,-61.6933111243076,
-235.35005));
#215903=CARTESIAN_POINT('Ctrl Pts',(8.20938920381546,-62.8670241015852,
-234.595245743017));
#215904=CARTESIAN_POINT('Ctrl Pts',(8.29080672382282,-62.4423929773204,
-235.350049999976));
#215905=CARTESIAN_POINT('Ctrl Pts',(8.4487057336385,-61.5865300359515,-235.35005));
#215906=CARTESIAN_POINT('Ctrl Pts',(7.82222359068918,-62.7915296928953,
-234.611394249339));
#215907=CARTESIAN_POINT('Ctrl Pts',(7.88989268115682,-62.3613610544617,
-235.350049999994));
#215908=CARTESIAN_POINT('Ctrl Pts',(8.01916095024903,-61.5134429064026,
-235.35005));
#215909=CARTESIAN_POINT('Ctrl Pts',(6.66116371746047,-62.6255181896041,
-234.651995705069));
#215910=CARTESIAN_POINT('Ctrl Pts',(6.69156996858306,-62.1840858314768,
-235.350050000012));
#215911=CARTESIAN_POINT('Ctrl Pts',(6.73293045659356,-61.3568710016287,
-235.35005));
#215912=CARTESIAN_POINT('Ctrl Pts',(5.88732128025216,-62.5951782831116,
-234.668619732153));
#215913=CARTESIAN_POINT('Ctrl Pts',(5.88578405769122,-62.150383637914,-235.350049999964));
#215914=CARTESIAN_POINT('Ctrl Pts',(5.87863226335204,-61.3356495997417,
-235.35005));
#215915=CARTESIAN_POINT('Ctrl Pts',(4.73022316785671,-62.6693442476172,
-234.680424870605));
#215916=CARTESIAN_POINT('Ctrl Pts',(4.68487052924521,-62.226315867779,-235.350050000018));
#215917=CARTESIAN_POINT('Ctrl Pts',(4.60187420700122,-61.426106672458,-235.35005));
#215918=CARTESIAN_POINT('Ctrl Pts',(4.34523442762013,-62.714083360949,-234.682140423453));
#215919=CARTESIAN_POINT('Ctrl Pts',(4.28518237892104,-62.2726127748062,
-235.350049999988));
#215920=CARTESIAN_POINT('Ctrl Pts',(4.1770740790426,-61.4767540523636,-235.35005));
#215921=CARTESIAN_POINT('Ctrl Pts',(3.76915274784454,-62.8120240257835,
-234.681325996944));
#215922=CARTESIAN_POINT('Ctrl Pts',(3.68781576212144,-62.3742400764792,
-235.350050000006));
#215923=CARTESIAN_POINT('Ctrl Pts',(3.54108358671642,-61.5842725312083,
-235.35005));
#215924=CARTESIAN_POINT('Ctrl Pts',(3.57736454720535,-62.8498101374656,
-234.680488798365));
#215925=CARTESIAN_POINT('Ctrl Pts',(3.48889544140117,-62.413503321465,-235.350049999997));
#215926=CARTESIAN_POINT('Ctrl Pts',(3.32928846564854,-61.6253723533426,
-235.35005));
#215927=CARTESIAN_POINT('Ctrl Pts',(3.29014195104425,-62.9143448304384,
-234.678356484935));
#215928=CARTESIAN_POINT('Ctrl Pts',(3.19114060354514,-62.4805904586232,
-235.350050000002));
#215929=CARTESIAN_POINT('Ctrl Pts',(3.01190491992465,-61.6950839540996,
-235.35005));
#215930=CARTESIAN_POINT('Ctrl Pts',(3.1944780537155,-62.9371661600342,-234.677499402921));
#215931=CARTESIAN_POINT('Ctrl Pts',(3.09195226458871,-62.5043289573996,
-235.350049999992));
#215932=CARTESIAN_POINT('Ctrl Pts',(2.90616195484145,-61.7196655152859,
-235.35005));
#215933=CARTESIAN_POINT('Ctrl Pts',(3.07500525353187,-62.9673499718945,
-234.676240441763));
#215934=CARTESIAN_POINT('Ctrl Pts',(2.96811329314043,-62.5357301121157,
-235.350050000002));
#215935=CARTESIAN_POINT('Ctrl Pts',(2.77404858885074,-61.7520964605576,
-235.35005));
#215936=CARTESIAN_POINT('Ctrl Pts',(3.05111608590414,-62.9734695946934,
-234.675979264585));
#215937=CARTESIAN_POINT('Ctrl Pts',(2.94334732448096,-62.5420981916043,
-235.350050000001));
#215938=CARTESIAN_POINT('Ctrl Pts',(2.74762918327784,-61.7586678648919,
-235.35005));
#215939=CARTESIAN_POINT('Ctrl Pts',(3.0152905878955,-62.9827737431109,-234.675573317217));
#215940=CARTESIAN_POINT('Ctrl Pts',(2.906208743664,-62.5517806373196,-235.350049999999));
#215941=CARTESIAN_POINT('Ctrl Pts',(2.70800499509792,-61.7686532835183,
-235.35005));
#215942=CARTESIAN_POINT('Ctrl Pts',(3.00335013472062,-62.98589591073,-234.675435637832));
#215943=CARTESIAN_POINT('Ctrl Pts',(2.89383036974431,-62.5550299942805,
-235.35005));
#215944=CARTESIAN_POINT('Ctrl Pts',(2.6947977524096,-61.7720031419126,-235.35005));
#215945=CARTESIAN_POINT('Ctrl Pts',(2.97947201822115,-62.9921818874314,
-234.675155533715));
#215946=CARTESIAN_POINT('Ctrl Pts',(2.8690767376369,-62.5615723327899,-235.35005));
#215947=CARTESIAN_POINT('Ctrl Pts',(2.66838491033016,-61.7787457138043,
-235.35005));
#215948=CARTESIAN_POINT('Ctrl Pts',(2.96304225688233,-62.9964242380372,
-234.675077639757));
#215949=CARTESIAN_POINT('Ctrl Pts',(2.85379759446374,-62.5655303634271,
-235.35005));
#215950=CARTESIAN_POINT('Ctrl Pts',(2.65517833661466,-61.7821130182165,
-235.35005));
#215951=CARTESIAN_POINT('Ctrl Pts',(2.88938127733355,-63.0153416312828,
-234.674574704412));
#215952=CARTESIAN_POINT('Ctrl Pts',(2.78287887281784,-62.5838153796612,
-235.350050000001));
#215953=CARTESIAN_POINT('Ctrl Pts',(2.58913846773959,-61.7987669810389,
-235.35005));
#215954=CARTESIAN_POINT('Ctrl Pts',(2.83042206824581,-63.0299995242519,
-234.674181109462));
#215955=CARTESIAN_POINT('Ctrl Pts',(2.72611963520325,-62.5979826576736,
-235.35005));
#215956=CARTESIAN_POINT('Ctrl Pts',(2.53629033417451,-61.8116666733557,
-235.35005));
#215957=CARTESIAN_POINT('Ctrl Pts',(2.29957200197046,-63.1576513891524,
-234.670723008053));
#215958=CARTESIAN_POINT('Ctrl Pts',(2.21477240222884,-62.721441734,-235.35005));
#215959=CARTESIAN_POINT('Ctrl Pts',(2.06051214976267,-61.9239829504865,
-235.35005));
#215960=CARTESIAN_POINT('Ctrl Pts',(1.82561741918027,-63.2408549075195,
-234.668259126929));
#215961=CARTESIAN_POINT('Ctrl Pts',(1.75845914439681,-62.8018876347933,
-235.350050000006));
#215962=CARTESIAN_POINT('Ctrl Pts',(1.63573306964857,-61.997098140329,-235.35005));
#215963=CARTESIAN_POINT('Ctrl Pts',(0.88215860141345,-63.34926053199,-234.664972573172));
#215964=CARTESIAN_POINT('Ctrl Pts',(0.849715125954841,-62.9067900502082,
-235.350049999994));
#215965=CARTESIAN_POINT('Ctrl Pts',(0.790392115670831,-62.0923066687554,
-235.35005));
#215966=CARTESIAN_POINT('Ctrl Pts',(0.412136733768758,-63.3746270691585,
-234.664093426845));
#215967=CARTESIAN_POINT('Ctrl Pts',(0.397111998278993,-62.9313429315101,
-235.350050000035));
#215968=CARTESIAN_POINT('Ctrl Pts',(0.36940841555812,-62.1145237664284,
-235.35005));
#215969=CARTESIAN_POINT('Ctrl Pts',(-0.991515792586106,-63.3680438675972,
-234.664322262232));
#215970=CARTESIAN_POINT('Ctrl Pts',(-0.95532554440835,-62.9249658076674,
-235.35004999993));
#215971=CARTESIAN_POINT('Ctrl Pts',(-0.88873098344401,-62.1087555751507,
-235.35005));
#215972=CARTESIAN_POINT('Ctrl Pts',(-1.92100220733562,-63.2544619761069,
-234.668143932231));
#215973=CARTESIAN_POINT('Ctrl Pts',(-1.84945562689762,-62.8152272225558,
-235.35005));
#215974=CARTESIAN_POINT('Ctrl Pts',(-1.7211315285284,-62.0092019215959,
-235.35005));
#215975=CARTESIAN_POINT('Ctrl Pts',(-2.87097991613647,-63.0198283709189,
-234.674453520452));
#215976=CARTESIAN_POINT('Ctrl Pts',(-2.76516804634539,-62.5881510724421,
-235.35005));
#215977=CARTESIAN_POINT('Ctrl Pts',(-2.57264640705579,-61.8027147274169,
-235.35005));
#215978=CARTESIAN_POINT('Ctrl Pts',(-2.89975790044207,-63.0126057280022,
-234.674646875394));
#215979=CARTESIAN_POINT('Ctrl Pts',(-2.79287250767241,-62.581170184688,
-235.35005));
#215980=CARTESIAN_POINT('Ctrl Pts',(-2.5984432576946,-61.7963577456803,
-235.35005));
#215981=CARTESIAN_POINT('Ctrl Pts',(-2.94290959864959,-63.0016028905584,
-234.674940028084));
#215982=CARTESIAN_POINT('Ctrl Pts',(-2.83441572839343,-62.5705355559834,
-235.35005));
#215983=CARTESIAN_POINT('Ctrl Pts',(-2.63712855614808,-61.7866721046702,
-235.35005));
#215984=CARTESIAN_POINT('Ctrl Pts',(-2.95729095518362,-62.9979071324124,
-234.67503826564));
#215985=CARTESIAN_POINT('Ctrl Pts',(-2.84826077962461,-62.5669635813212,
-235.35005));
#215986=CARTESIAN_POINT('Ctrl Pts',(-2.65002199274596,-61.7834185300358,
-235.35005));
#215987=CARTESIAN_POINT('Ctrl Pts',(-2.98604840419677,-62.9904593061707,
-234.675235761569));
#215988=CARTESIAN_POINT('Ctrl Pts',(-2.87594598022536,-62.5597652489865,
-235.35005));
#215989=CARTESIAN_POINT('Ctrl Pts',(-2.67580553519198,-61.7768612507126,
-235.35005));
#215990=CARTESIAN_POINT('Ctrl Pts',(-2.9978333877905,-62.9873435276064,
-234.675371450446));
#215991=CARTESIAN_POINT('Ctrl Pts',(-2.88811134765541,-62.5565366104963,
-235.35005));
#215992=CARTESIAN_POINT('Ctrl Pts',(-2.68869554564646,-61.7735561102329,
-235.35005));
#215993=CARTESIAN_POINT('Ctrl Pts',(-3.05611228962128,-62.9721057909015,
-234.676043337161));
#215994=CARTESIAN_POINT('Ctrl Pts',(-2.94852233650361,-62.5406795307465,
-235.35005));
#215995=CARTESIAN_POINT('Ctrl Pts',(-2.75315733717204,-61.7572070918297,
-235.35005));
#215996=CARTESIAN_POINT('Ctrl Pts',(-3.10276465859771,-62.9602306309284,
-234.676544840607));
#215997=CARTESIAN_POINT('Ctrl Pts',(-2.99688788645165,-62.5283225924192,
-235.35005));
#215998=CARTESIAN_POINT('Ctrl Pts',(-2.80474830172023,-61.7444519385904,
-235.35005));
#215999=CARTESIAN_POINT('Ctrl Pts',(-3.24280643592837,-62.9255451527486,
-234.677942742714));
#216000=CARTESIAN_POINT('Ctrl Pts',(-3.14205961162902,-62.4922406313808,
-235.350050000002));
#216001=CARTESIAN_POINT('Ctrl Pts',(-2.95958538043147,-61.7071525092866,
-235.35005));
#216002=CARTESIAN_POINT('Ctrl Pts',(-3.33628023959272,-62.9036747672035,
-234.678732585306));
#216003=CARTESIAN_POINT('Ctrl Pts',(-3.23897853980704,-62.4694942379193,
-235.350050000002));
#216004=CARTESIAN_POINT('Ctrl Pts',(-3.06289566840461,-61.6835740933876,
-235.35005));
#216005=CARTESIAN_POINT('Ctrl Pts',(-3.61701461689342,-62.8417880653747,
-234.68068504518));
#216006=CARTESIAN_POINT('Ctrl Pts',(-3.53001543785944,-62.4051669357519,
-235.350049999997));
#216007=CARTESIAN_POINT('Ctrl Pts',(-3.37308038697823,-61.6166595365466,
-235.35005));
#216008=CARTESIAN_POINT('Ctrl Pts',(-3.80452881266942,-62.8055092013148,
-234.681430782666));
#216009=CARTESIAN_POINT('Ctrl Pts',(-3.72450262338561,-62.3674750906498,
-235.350050000018));
#216010=CARTESIAN_POINT('Ctrl Pts',(-3.58014437735177,-61.5771574345827,
-235.35005));
#216011=CARTESIAN_POINT('Ctrl Pts',(-4.36760854874154,-62.7114158369336,
-234.682047690539));
#216012=CARTESIAN_POINT('Ctrl Pts',(-4.3083998660853,-62.2698516038986,
-235.350049999965));
#216013=CARTESIAN_POINT('Ctrl Pts',(-4.20176187344348,-61.4737420228677,
-235.35005));
#216014=CARTESIAN_POINT('Ctrl Pts',(-4.74383676949718,-62.668310555781,
-234.680303868519));
#216015=CARTESIAN_POINT('Ctrl Pts',(-4.6989741743333,-62.2252554074114,
-235.350050000029));
#216016=CARTESIAN_POINT('Ctrl Pts',(-4.61689483741499,-61.4248774566823,
-235.35005));
#216017=CARTESIAN_POINT('Ctrl Pts',(-5.87442448212421,-62.5963302145134,
-234.668715190654));
#216018=CARTESIAN_POINT('Ctrl Pts',(-5.87235395168802,-62.1515742909292,
-235.350049999942));
#216019=CARTESIAN_POINT('Ctrl Pts',(-5.86440266843056,-61.3369909474474,
-235.35005));
#216020=CARTESIAN_POINT('Ctrl Pts',(-6.630328727236,-62.6245394292558,-234.652628616953));
#216021=CARTESIAN_POINT('Ctrl Pts',(-6.65928611702461,-62.1829590506774,
-235.350049999988));
#216022=CARTESIAN_POINT('Ctrl Pts',(-6.69887188182861,-61.3562699588587,
-235.35005));
#216023=CARTESIAN_POINT('Ctrl Pts',(-7.764209767566,-62.7816811580039,-234.613624648391));
#216024=CARTESIAN_POINT('Ctrl Pts',(-7.82979546040407,-62.3508034677975,
-235.350050000006));
#216025=CARTESIAN_POINT('Ctrl Pts',(-7.95484405860484,-61.5040080281448,
-235.35005));
#216026=CARTESIAN_POINT('Ctrl Pts',(-8.14142530534439,-62.8532056007147,
-234.598165828659));
#216027=CARTESIAN_POINT('Ctrl Pts',(-8.22039383870565,-62.4275509346929,
-235.35005));
#216028=CARTESIAN_POINT('Ctrl Pts',(-8.37327068677123,-61.573105256355,
-235.35005));
#216029=CARTESIAN_POINT('Ctrl Pts',(-8.5629236763468,-62.9549034336122,
-234.577665757063));
#216030=CARTESIAN_POINT('Ctrl Pts',(-8.65406374113881,-62.5362556404638,
-235.35005));
#216031=CARTESIAN_POINT('Ctrl Pts',(-8.84186416774843,-61.6731857859409,
-235.35005));
#216032=CARTESIAN_POINT('Ctrl Pts',(-8.60972279857098,-62.966499174667,
-234.575344423268));
#216033=CARTESIAN_POINT('Ctrl Pts',(-8.70237757817563,-62.5486988611875,
-235.350050000009));
#216034=CARTESIAN_POINT('Ctrl Pts',(-8.89390821376875,-61.6846177854791,
-235.35005));
#216035=CARTESIAN_POINT('Ctrl Pts',(-8.67987147174762,-62.9843376272339,
-234.571795714236));
#216036=CARTESIAN_POINT('Ctrl Pts',(-8.7747593225483,-62.5678413783773,
-235.350049999996));
#216037=CARTESIAN_POINT('Ctrl Pts',(-8.9719413326839,-61.7022352005211,
-235.35005));
#216038=CARTESIAN_POINT('Ctrl Pts',(-8.70324596171864,-62.9903579019877,
-234.570601696122));
#216039=CARTESIAN_POINT('Ctrl Pts',(-8.79888168729908,-62.5743045962304,
-235.350050000003));
#216040=CARTESIAN_POINT('Ctrl Pts',(-8.99794688049398,-61.7081859103136,
-235.35005));
#216041=CARTESIAN_POINT('Ctrl Pts',(-8.74997809315458,-63.0025468085543,
-234.568191202621));
#216042=CARTESIAN_POINT('Ctrl Pts',(-8.84710303258602,-62.5873924023601,
-235.350049999997));
#216043=CARTESIAN_POINT('Ctrl Pts',(-9.04994697297616,-61.7202440833036,
-235.35005));
#216044=CARTESIAN_POINT('Ctrl Pts',(-8.77030020255578,-63.0086617980509,
-234.565865719937));
#216045=CARTESIAN_POINT('Ctrl Pts',(-8.86903102195205,-62.594426558538,
-235.350049999999));
#216046=CARTESIAN_POINT('Ctrl Pts',(-9.07593838869885,-61.7263961224781,
-235.35005));
#216047=CARTESIAN_POINT('Ctrl Pts',(-8.91694881903725,-63.0405575039938,
-234.570644549592));
#216048=CARTESIAN_POINT('Ctrl Pts',(-9.01063474350099,-62.624024386533,
-235.350050000003));
#216049=CARTESIAN_POINT('Ctrl Pts',(-9.20590431013486,-61.7570303410545,
-235.35005));
#216050=CARTESIAN_POINT('Ctrl Pts',(-9.03436031698127,-63.0642013014708,
-234.574496870482));
#216051=CARTESIAN_POINT('Ctrl Pts',(-9.12404358218876,-62.6459210827606,
-235.35005));
#216052=CARTESIAN_POINT('Ctrl Pts',(-9.30999109039434,-61.7799130279695,
-235.35005));
#216053=CARTESIAN_POINT('Ctrl Pts',(-9.38683707975019,-63.1295777507455,
-234.58612993111));
#216054=CARTESIAN_POINT('Ctrl Pts',(-9.464112377,-62.7062240376773,-235.35005));
#216055=CARTESIAN_POINT('Ctrl Pts',(-9.62258974276106,-61.8437414130309,
-235.35005));
#216056=CARTESIAN_POINT('Ctrl Pts',(-9.62214011478876,-63.1657558644233,
-234.593987078423));
#216057=CARTESIAN_POINT('Ctrl Pts',(-9.6911920092531,-62.7393844961485,
-235.350049999994));
#216058=CARTESIAN_POINT('Ctrl Pts',(-9.83143975137235,-61.8798699303951,
-235.35005));
#216059=CARTESIAN_POINT('Ctrl Pts',(-10.7997915248163,-63.3103622575713,
-234.633595136481));
#216060=CARTESIAN_POINT('Ctrl Pts',(-10.8212304548731,-62.8697460481048,
-235.350050000023));
#216061=CARTESIAN_POINT('Ctrl Pts',(-10.8779045135963,-62.0289610481999,
-235.35005));
#216062=CARTESIAN_POINT('Ctrl Pts',(-11.7461619842447,-63.3113988762096,
-234.666687842414));
#216063=CARTESIAN_POINT('Ctrl Pts',(-11.7320939393461,-62.8666836322213,
-235.350049999928));
#216064=CARTESIAN_POINT('Ctrl Pts',(-11.7220571315963,-62.0487835216839,
-235.35005));
#216065=CARTESIAN_POINT('Ctrl Pts',(-13.1699413526949,-63.1363620280083,
-234.716022189278));
#216066=CARTESIAN_POINT('Ctrl Pts',(-13.10608590161,-62.6921044640064,-235.350050000036));
#216067=CARTESIAN_POINT('Ctrl Pts',(-12.9992495965492,-61.9223278044926,
-235.35005));
#216068=CARTESIAN_POINT('Ctrl Pts',(-13.6468010556902,-63.0478428317766,
-234.732508264035));
#216069=CARTESIAN_POINT('Ctrl Pts',(-13.5644252452197,-62.6057426040311,
-235.350049999994));
#216070=CARTESIAN_POINT('Ctrl Pts',(-13.4279947259813,-61.8535648232588,
-235.35005));
#216071=CARTESIAN_POINT('Ctrl Pts',(-14.1487244112426,-62.9212890657887,
-234.749460742189));
#216072=CARTESIAN_POINT('Ctrl Pts',(-14.0482803552132,-62.4826593861811,
-235.35005));
#216073=CARTESIAN_POINT('Ctrl Pts',(-13.880777738108,-61.7511282800593,
-235.35005));
#216074=CARTESIAN_POINT('Ctrl Pts',(-14.1782348713718,-62.9137255409854,
-234.750455807673));
#216075=CARTESIAN_POINT('Ctrl Pts',(-14.0766397091771,-62.4753290557739,
-235.350050000002));
#216076=CARTESIAN_POINT('Ctrl Pts',(-13.9074044897115,-61.7449947684686,
-235.35005));
#216077=CARTESIAN_POINT('Ctrl Pts',(-14.2224775170047,-62.9022015555295,
-234.751944983515));
#216078=CARTESIAN_POINT('Ctrl Pts',(-14.1191614632759,-62.4641631011826,
-235.350049999999));
#216079=CARTESIAN_POINT('Ctrl Pts',(-13.9473332680511,-61.7356322629881,
-235.35005));
#216080=CARTESIAN_POINT('Ctrl Pts',(-14.2372212410967,-62.8983304396559,
-234.75244080564));
#216081=CARTESIAN_POINT('Ctrl Pts',(-14.1333303258632,-62.4604132959301,
-235.35005));
#216082=CARTESIAN_POINT('Ctrl Pts',(-13.9606409693201,-61.7324843881166,
-235.35005));
#216083=CARTESIAN_POINT('Ctrl Pts',(-14.2667009590697,-62.89052860958,-234.753431279982));
#216084=CARTESIAN_POINT('Ctrl Pts',(-14.1616608142962,-62.4528572201639,
-235.350049999999));
#216085=CARTESIAN_POINT('Ctrl Pts',(-13.9872525830674,-61.7261344765805,
-235.35005));
#216086=CARTESIAN_POINT('Ctrl Pts',(-14.2781153460893,-62.8881093785209,
-234.753016968105));
#216087=CARTESIAN_POINT('Ctrl Pts',(-14.1738174996514,-62.4502724992987,
-235.35005));
#216088=CARTESIAN_POINT('Ctrl Pts',(-14.000557201923,-61.7229425377452,
-235.35005));
#216089=CARTESIAN_POINT('Ctrl Pts',(-14.3387700345776,-62.8745860683453,
-234.75190829161));
#216090=CARTESIAN_POINT('Ctrl Pts',(-14.2367701819519,-62.4362364690685,
-235.350049999998));
#216091=CARTESIAN_POINT('Ctrl Pts',(-14.067093113681,-61.7071660730871,
-235.35005));
#216092=CARTESIAN_POINT('Ctrl Pts',(-14.3873180956111,-62.8641049651357,
-234.750988490225));
#216093=CARTESIAN_POINT('Ctrl Pts',(-14.2871495014114,-62.4253613242066,
-235.350050000003));
#216094=CARTESIAN_POINT('Ctrl Pts',(-14.1203460326614,-61.6948906982809,
-235.35005));
#216095=CARTESIAN_POINT('Ctrl Pts',(-14.5330297353877,-62.8336671798573,
-234.748130090176));
#216096=CARTESIAN_POINT('Ctrl Pts',(-14.4383810376854,-62.3937793044535,
-235.350049999996));
#216097=CARTESIAN_POINT('Ctrl Pts',(-14.2801767898011,-61.6590938369543,
-235.35005));
#216098=CARTESIAN_POINT('Ctrl Pts',(-14.6302610598049,-62.814715723775,
-234.746092558));
#216099=CARTESIAN_POINT('Ctrl Pts',(-14.5392754781889,-62.3741280970256,
-235.35005));
#216100=CARTESIAN_POINT('Ctrl Pts',(-14.3868266096958,-61.6366013501929,
-235.35005));
#216101=CARTESIAN_POINT('Ctrl Pts',(-14.9221858666243,-62.7618333918368,
-234.739578254538));
#216102=CARTESIAN_POINT('Ctrl Pts',(-14.8423074294462,-62.3193023231595,
-235.35005));
#216103=CARTESIAN_POINT('Ctrl Pts',(-14.707060162972,-61.5731850879451,
-235.35005));
#216104=CARTESIAN_POINT('Ctrl Pts',(-15.1171107050774,-62.7318713397189,
-234.73470073075));
#216105=CARTESIAN_POINT('Ctrl Pts',(-15.0445895988711,-62.2883058945919,
-235.350050000006));
#216106=CARTESIAN_POINT('Ctrl Pts',(-14.9209277353048,-61.5363188718154,
-235.35005));
#216107=CARTESIAN_POINT('Ctrl Pts',(-16.092794467113,-62.6080592508531,
-234.70749886562));
#216108=CARTESIAN_POINT('Ctrl Pts',(-16.0603371959058,-62.1601711109026,
-235.350049999976));
#216109=CARTESIAN_POINT('Ctrl Pts',(-15.9921235684109,-61.3785480216598,
-235.35005));
#216110=CARTESIAN_POINT('Ctrl Pts',(-16.8769323685421,-62.5917011576633,
-234.676953449944));
#216111=CARTESIAN_POINT('Ctrl Pts',(-16.877440790753,-62.1458673443692,
-235.350050000024));
#216112=CARTESIAN_POINT('Ctrl Pts',(-16.8549897301619,-61.3368092608675,
-235.35005));
#216113=CARTESIAN_POINT('Ctrl Pts',(-18.4490580403513,-62.7174106638047,
-234.59397567041));
#216114=CARTESIAN_POINT('Ctrl Pts',(-18.5050342407488,-62.2871579302411,
-235.350049999975));
#216115=CARTESIAN_POINT('Ctrl Pts',(-18.5923327067712,-61.4193093323336,
-235.35005));
#216116=CARTESIAN_POINT('Ctrl Pts',(-19.243264596634,-62.8631291742346,
-234.540485831164));
#216117=CARTESIAN_POINT('Ctrl Pts',(-19.3295880835876,-62.4508333719574,
-235.350049999916));
#216118=CARTESIAN_POINT('Ctrl Pts',(-19.4741956661812,-61.5471706223108,
-235.35005));
#216119=CARTESIAN_POINT('Ctrl Pts',(-20.0002454535025,-63.0750142297971,
-234.47617280861));
#216120=CARTESIAN_POINT('Ctrl Pts',(-20.0938415017253,-62.6846662779264,
-235.35005));
#216121=CARTESIAN_POINT('Ctrl Pts',(-20.3180691938068,-61.7495111937247,
-235.35005));
#216122=CARTESIAN_POINT('',(-5.58372807339351E-13,-63.3694498996295,-234.668963364338));
#216123=CARTESIAN_POINT('',(8.78586952537018,-63.0089774131351,-234.571825729504));
#216124=CARTESIAN_POINT('Ctrl Pts',(-1.5702990355655E-14,-63.3694498182033,
-234.66896331128));
#216125=CARTESIAN_POINT('Ctrl Pts',(0.217773905612689,-63.3694496543811,
-234.668963562687));
#216126=CARTESIAN_POINT('Ctrl Pts',(0.438520411739192,-63.3634719988444,
-234.669163036834));
#216127=CARTESIAN_POINT('Ctrl Pts',(0.662407453077813,-63.3509495177584,
-234.669561733719));
#216128=CARTESIAN_POINT('Ctrl Pts',(0.692105148220668,-63.3492884621498,
-234.669614619221));
#216129=CARTESIAN_POINT('Ctrl Pts',(0.721858175028539,-63.347512237878,
-234.669671010034));
#216130=CARTESIAN_POINT('Ctrl Pts',(0.751666994640722,-63.3456195093547,
-234.669730906157));
#216131=CARTESIAN_POINT('Ctrl Pts',(0.967065625823832,-63.3319426466531,
-234.670163715742));
#216132=CARTESIAN_POINT('Ctrl Pts',(1.18537391652108,-63.3121847391183,
-234.670779555548));
#216133=CARTESIAN_POINT('Ctrl Pts',(1.40676856118831,-63.2857272692194,
-234.671578425574));
#216134=CARTESIAN_POINT('Ctrl Pts',(1.43728891440615,-63.2820799753665,
-234.671688553781));
#216135=CARTESIAN_POINT('Ctrl Pts',(1.46786798998409,-63.2783053208916,
-234.671802160294));
#216136=CARTESIAN_POINT('Ctrl Pts',(1.49850631840134,-63.2744016447649,
-234.671919245112));
#216137=CARTESIAN_POINT('Ctrl Pts',(1.54099258502891,-63.2689884047705,
-234.672081606998));
#216138=CARTESIAN_POINT('Ctrl Pts',(1.58359278893985,-63.2633270675726,
-234.672250657476));
#216139=CARTESIAN_POINT('Ctrl Pts',(1.62630844138418,-63.2574121891646,
-234.672426396546));
#216140=CARTESIAN_POINT('Ctrl Pts',(1.71981144698678,-63.2444647360117,
-234.672811082962));
#216141=CARTESIAN_POINT('Ctrl Pts',(1.81386752908635,-63.2303025361026,
-234.673227818233));
#216142=CARTESIAN_POINT('Ctrl Pts',(1.90849366367972,-63.2148672638034,
-234.673676608004));
#216143=CARTESIAN_POINT('Ctrl Pts',(1.95580673097641,-63.2071496276537,
-234.673901002889));
#216144=CARTESIAN_POINT('Ctrl Pts',(2.00326230890218,-63.199113708202,-234.674133401273));
#216145=CARTESIAN_POINT('Ctrl Pts',(2.05086269848244,-63.1907520420292,
-234.674373816126));
#216146=CARTESIAN_POINT('Ctrl Pts',(2.07466289327257,-63.1865712089429,
-234.674494023553));
#216147=CARTESIAN_POINT('Ctrl Pts',(2.09849929082736,-63.1823089381926,
-234.674616234444));
#216148=CARTESIAN_POINT('Ctrl Pts',(2.12237218364187,-63.1779642886395,
-234.674740448649));
#216149=CARTESIAN_POINT('Ctrl Pts',(2.13430863004912,-63.1757919638629,
-234.674802555751));
#216150=CARTESIAN_POINT('Ctrl Pts',(2.1462542002606,-63.1735990443261,-234.674865163642));
#216151=CARTESIAN_POINT('Ctrl Pts',(2.15820893145162,-63.1713854117438,
-234.674928272312));
#216152=CARTESIAN_POINT('Ctrl Pts',(2.16418629704713,-63.1702785954526,
-234.674959826647));
#216153=CARTESIAN_POINT('Ctrl Pts',(2.17016595288684,-63.1691666008963,
-234.674991506174));
#216154=CARTESIAN_POINT('Ctrl Pts',(2.17614790365865,-63.1680494132478,
-234.675023310893));
#216155=CARTESIAN_POINT('Ctrl Pts',(2.18212985443046,-63.1669322255993,
-234.675055115613));
#216156=CARTESIAN_POINT('Ctrl Pts',(2.18934094285044,-63.1655787643479,
-234.675093614681));
#216157=CARTESIAN_POINT('Ctrl Pts',(2.19410064546927,-63.1646822561782,
-234.675119100623));
#216158=CARTESIAN_POINT('Ctrl Pts',(2.21009843956643,-63.1616690105507,
-234.675204761195));
#216159=CARTESIAN_POINT('Ctrl Pts',(2.22625301394984,-63.158591438058,-234.675293116861));
#216160=CARTESIAN_POINT('Ctrl Pts',(2.24256443067466,-63.15544746846,-234.675384167619));
#216161=CARTESIAN_POINT('Ctrl Pts',(2.33086547491839,-63.1384277452036,
-234.675877066377));
#216162=CARTESIAN_POINT('Ctrl Pts',(2.42376183912149,-63.1194662392236,
-234.676448946035));
#216163=CARTESIAN_POINT('Ctrl Pts',(2.52127275503764,-63.0981948799086,
-234.677099806595));
#216164=CARTESIAN_POINT('Ctrl Pts',(2.61627973210451,-63.0774697382397,
-234.677733954));
#216165=CARTESIAN_POINT('Ctrl Pts',(2.71566715620675,-63.0545518959675,
-234.678443078155));
#216166=CARTESIAN_POINT('Ctrl Pts',(2.81946610010958,-63.0290534318913,
-234.67922717906));
#216167=CARTESIAN_POINT('Ctrl Pts',(2.870498985797,-63.0165170788854,-234.679612683289));
#216168=CARTESIAN_POINT('Ctrl Pts',(2.92259844844719,-63.0033561960728,
-234.680016310973));
#216169=CARTESIAN_POINT('Ctrl Pts',(2.97576958847413,-62.989520236264,-234.680438062112));
#216170=CARTESIAN_POINT('Ctrl Pts',(2.97914177857081,-62.9886427398135,
-234.680464810175));
#216171=CARTESIAN_POINT('Ctrl Pts',(2.98251827959221,-62.9877625270014,
-234.680491631136));
#216172=CARTESIAN_POINT('Ctrl Pts',(2.98589909297911,-62.9868795845193,
-234.680518524994));
#216173=CARTESIAN_POINT('Ctrl Pts',(3.03144670211263,-62.9749842461911,
-234.680880849326));
#216174=CARTESIAN_POINT('Ctrl Pts',(3.07784469384026,-62.9631470419589,
-234.681256404939));
#216175=CARTESIAN_POINT('Ctrl Pts',(3.12509757339216,-62.9513965645584,
-234.681645191834));
#216176=CARTESIAN_POINT('Ctrl Pts',(3.15047770749805,-62.9450852308352,
-234.681854014315));
#216177=CARTESIAN_POINT('Ctrl Pts',(3.17610446179225,-62.9387989363886,
-234.682066653893));
#216178=CARTESIAN_POINT('Ctrl Pts',(3.20197848411835,-62.9325422483476,
-234.682283110295));
#216179=CARTESIAN_POINT('Ctrl Pts',(3.2149154952814,-62.929413904327,-234.682391338496));
#216180=CARTESIAN_POINT('Ctrl Pts',(3.22791432366225,-62.9262929628025,
-234.682500521516));
#216181=CARTESIAN_POINT('Ctrl Pts',(3.24097504554104,-62.9231800045925,
-234.682610658402));
#216182=CARTESIAN_POINT('Ctrl Pts',(3.25276701314493,-62.9203694476642,
-234.682710096289));
#216183=CARTESIAN_POINT('Ctrl Pts',(3.26621068276329,-62.9171883489843,
-234.682823921931));
#216184=CARTESIAN_POINT('Ctrl Pts',(3.2769690464069,-62.9146585345259,-234.682915271999));
#216185=CARTESIAN_POINT('Ctrl Pts',(3.27812659028102,-62.9143863396711,
-234.68292510079));
#216186=CARTESIAN_POINT('Ctrl Pts',(3.27925303445033,-62.9141216361366,
-234.68293466939));
#216187=CARTESIAN_POINT('Ctrl Pts',(3.28034296828758,-62.9138656646226,
-234.682943931882));
#216188=CARTESIAN_POINT('Ctrl Pts',(3.42311597107787,-62.8803353525691,
-234.684157247518));
#216189=CARTESIAN_POINT('Ctrl Pts',(3.56630723773157,-62.8496695059215,
-234.685050927405));
#216190=CARTESIAN_POINT('Ctrl Pts',(3.71018636154233,-62.8218113840577,
-234.685624000546));
#216191=CARTESIAN_POINT('Ctrl Pts',(3.85344884246849,-62.7940726576432,
-234.686194617587));
#216192=CARTESIAN_POINT('Ctrl Pts',(3.99739358369234,-62.7691175748496,
-234.686447370131));
#216193=CARTESIAN_POINT('Ctrl Pts',(4.14229793497986,-62.7469404019187,
-234.686381299612));
#216194=CARTESIAN_POINT('Ctrl Pts',(4.21783125916824,-62.7353802549826,
-234.686346859474));
#216195=CARTESIAN_POINT('Ctrl Pts',(4.2936254830793,-62.7245757451169,-234.686225790181));
#216196=CARTESIAN_POINT('Ctrl Pts',(4.3697207132042,-62.7145316285495,-234.686017955969));
#216197=CARTESIAN_POINT('Ctrl Pts',(4.38025306702375,-62.7131414206571,
-234.6859891896));
#216198=CARTESIAN_POINT('Ctrl Pts',(4.39078527443694,-62.7117665649021,
-234.685958779806));
#216199=CARTESIAN_POINT('Ctrl Pts',(4.40131730214741,-62.710407049675,-234.685926726586));
#216200=CARTESIAN_POINT('Ctrl Pts',(4.67608260672618,-62.6749392721778,
-234.685090504658));
#216201=CARTESIAN_POINT('Ctrl Pts',(4.95072126703645,-62.6499130118094,
-234.683135747384));
#216202=CARTESIAN_POINT('Ctrl Pts',(5.22463708211698,-62.6350433636936,
-234.680062454763));
#216203=CARTESIAN_POINT('Ctrl Pts',(5.43392972328729,-62.623681814794,-234.677714224051));
#216204=CARTESIAN_POINT('Ctrl Pts',(5.64280142810662,-62.6182496913347,
-234.674712977953));
#216205=CARTESIAN_POINT('Ctrl Pts',(5.85100656062646,-62.61861720167,-234.671058716468));
#216206=CARTESIAN_POINT('Ctrl Pts',(5.99971161321492,-62.6188796862835,
-234.668448756091));
#216207=CARTESIAN_POINT('Ctrl Pts',(6.14807698913752,-62.622100557494,-234.665505682392));
#216208=CARTESIAN_POINT('Ctrl Pts',(6.29601532503752,-62.6282206073021,
-234.662229495371));
#216209=CARTESIAN_POINT('Ctrl Pts',(6.34701415223957,-62.6303303739203,
-234.66110009443));
#216210=CARTESIAN_POINT('Ctrl Pts',(6.39734769704919,-62.6327538032416,
-234.659946480854));
#216211=CARTESIAN_POINT('Ctrl Pts',(6.44804640347912,-62.6355359592762,
-234.658742787956));
#216212=CARTESIAN_POINT('Ctrl Pts',(6.48774806684274,-62.6377146385776,
-234.657800187767));
#216213=CARTESIAN_POINT('Ctrl Pts',(6.52767372357854,-62.640114284633,-234.656826877418));
#216214=CARTESIAN_POINT('Ctrl Pts',(6.56831866038382,-62.6427788180075,
-234.655810435343));
#216215=CARTESIAN_POINT('Ctrl Pts',(6.81815541742719,-62.6591572018768,
-234.649562557711));
#216216=CARTESIAN_POINT('Ctrl Pts',(7.06823871599811,-62.6839230792243,
-234.642231150492));
#216217=CARTESIAN_POINT('Ctrl Pts',(7.31818157745278,-62.7170814615928,
-234.633816213689));
#216218=CARTESIAN_POINT('Ctrl Pts',(7.76071788223362,-62.7757900317054,
-234.618917148293));
#216219=CARTESIAN_POINT('Ctrl Pts',(8.20281103349084,-62.8608087797858,
-234.600621383538));
#216220=CARTESIAN_POINT('Ctrl Pts',(8.64229067170807,-62.9718223083916,
-234.578928919424));
#216221=CARTESIAN_POINT('Ctrl Pts',(8.69017528132899,-62.9839180666877,
-234.576565362423));
#216222=CARTESIAN_POINT('Ctrl Pts',(8.73802891188869,-62.9963224091943,
-234.574161480689));
#216223=CARTESIAN_POINT('Ctrl Pts',(8.78584879256821,-63.0090349136113,
-234.571717274223));
#216224=CARTESIAN_POINT('',(-8.78585690854571,-63.009043156862,-234.571720019294));
#216225=CARTESIAN_POINT('Ctrl Pts',(-1.10089718099767E-12,-63.3694499810558,
-234.668963417397));
#216226=CARTESIAN_POINT('Ctrl Pts',(-0.0185810354048697,-63.3694498388901,
-234.668963445136));
#216227=CARTESIAN_POINT('Ctrl Pts',(-0.0371587302925499,-63.3694061680557,
-234.668964958478));
#216228=CARTESIAN_POINT('Ctrl Pts',(-0.0557330586443233,-63.3693190483712,
-234.668967969332));
#216229=CARTESIAN_POINT('Ctrl Pts',(-0.991261546562719,-63.3649311133023,
-234.669119616233));
#216230=CARTESIAN_POINT('Ctrl Pts',(-1.92049921579277,-63.2513737473296,
-234.67291846854));
#216231=CARTESIAN_POINT('Ctrl Pts',(-2.84145511359989,-63.0238979202665,
-234.679000216158));
#216232=CARTESIAN_POINT('Ctrl Pts',(-2.87023498540635,-63.0167893006708,
-234.679190270771));
#216233=CARTESIAN_POINT('Ctrl Pts',(-2.89900538169324,-63.0095682375878,
-234.679382465876));
#216234=CARTESIAN_POINT('Ctrl Pts',(-2.92776559984891,-63.0022346175025,
-234.679576728533));
#216235=CARTESIAN_POINT('Ctrl Pts',(-2.94214570892675,-62.9985678074598,
-234.679673859862));
#216236=CARTESIAN_POINT('Ctrl Pts',(-2.95652327372903,-62.9948728588666,
-234.679771508003));
#216237=CARTESIAN_POINT('Ctrl Pts',(-2.97089820746555,-62.9911497618158,
-234.679869663442));
#216238=CARTESIAN_POINT('Ctrl Pts',(-2.98527314120207,-62.9874266647649,
-234.679967818882));
#216239=CARTESIAN_POINT('Ctrl Pts',(-2.99706078139591,-62.9843100059298,
-234.680102693504));
#216240=CARTESIAN_POINT('Ctrl Pts',(-3.00871954326037,-62.9812615014743,
-234.680236264292));
#216241=CARTESIAN_POINT('Ctrl Pts',(-3.05535459071823,-62.9690674836524,
-234.680770547444));
#216242=CARTESIAN_POINT('Ctrl Pts',(-3.10201894695471,-62.9571886136925,
-234.681269039807));
#216243=CARTESIAN_POINT('Ctrl Pts',(-3.14871151468708,-62.9456232134564,
-234.681732208063));
#216244=CARTESIAN_POINT('Ctrl Pts',(-3.24209665015184,-62.9224924129843,
-234.682658544576));
#216245=CARTESIAN_POINT('Ctrl Pts',(-3.33559461282545,-62.9006153539932,
-234.68344363964));
#216246=CARTESIAN_POINT('Ctrl Pts',(-3.42919685501764,-62.8799803049587,
-234.684090544914));
#216247=CARTESIAN_POINT('Ctrl Pts',(-3.616401339402,-62.8387102068898,-234.685384355463));
#216248=CARTESIAN_POINT('Ctrl Pts',(-3.80396460003819,-62.8024209051424,
-234.686125603876));
#216249=CARTESIAN_POINT('Ctrl Pts',(-3.99170675162661,-62.7710480212593,
-234.686330001583));
#216250=CARTESIAN_POINT('Ctrl Pts',(-4.36719105480346,-62.7083022534931,
-234.686738796995));
#216251=CARTESIAN_POINT('Ctrl Pts',(-4.74352052971821,-62.6651875901659,
-234.685005473986));
#216252=CARTESIAN_POINT('Ctrl Pts',(-5.12048363858745,-62.6411926630512,
-234.681165753978));
#216253=CARTESIAN_POINT('Ctrl Pts',(-5.87440985632592,-62.5932028088217,
-234.673486313963));
#216254=CARTESIAN_POINT('Ctrl Pts',(-6.6305314355631,-62.6214447067006,
-234.657495585896));
#216255=CARTESIAN_POINT('Ctrl Pts',(-7.38662085898429,-62.7262724152159,
-234.631645385162));
#216256=CARTESIAN_POINT('Ctrl Pts',(-7.76466557069487,-62.7786862694735,
-234.618720284795));
#216257=CARTESIAN_POINT('Ctrl Pts',(-8.14197229631615,-62.8502567352985,
-234.603350759003));
#216258=CARTESIAN_POINT('Ctrl Pts',(-8.51671007390683,-62.9407093175552,
-234.585232582824));
#216259=CARTESIAN_POINT('Ctrl Pts',(-8.56355229610568,-62.9520158903373,
-234.582967810801));
#216260=CARTESIAN_POINT('Ctrl Pts',(-8.61036154587541,-62.9636189189669,
-234.580659656259));
#216261=CARTESIAN_POINT('Ctrl Pts',(-8.65713725766767,-62.9755186803616,
-234.578307258395));
#216262=CARTESIAN_POINT('Ctrl Pts',(-8.68052511356379,-62.9814685610589,
-234.577131059463));
#216263=CARTESIAN_POINT('Ctrl Pts',(-8.70390458536919,-62.9874926264074,
-234.575943799166));
#216264=CARTESIAN_POINT('Ctrl Pts',(-8.72727560477769,-62.993590919855,
-234.574745366521));
#216265=CARTESIAN_POINT('Ctrl Pts',(-8.73694813662187,-62.9961148122251,
-234.574249372841));
#216266=CARTESIAN_POINT('Ctrl Pts',(-8.746100261435,-62.9986429068519,-234.573562586431));
#216267=CARTESIAN_POINT('Ctrl Pts',(-8.75558085258196,-63.0012075165445,
-234.572965026759));
#216268=CARTESIAN_POINT('Ctrl Pts',(-8.76506144329811,-63.0037721261205,
-234.572367467114));
#216269=CARTESIAN_POINT('Ctrl Pts',(-8.77487050775363,-63.0063732152886,
-234.571859113242));
#216270=CARTESIAN_POINT('Ctrl Pts',(-8.7858569085457,-63.009043156862,-234.571720019294));
#216271=CARTESIAN_POINT('',(-14.2619204088508,-62.8884591070428,-234.75755030089));
#216272=CARTESIAN_POINT('Ctrl Pts',(-8.78585826084274,-63.0090374306747,
-234.571716790273));
#216273=CARTESIAN_POINT('Ctrl Pts',(-8.81155642576436,-63.0149922863215,
-234.571920323696));
#216274=CARTESIAN_POINT('Ctrl Pts',(-8.84178103342904,-63.0211625331105,
-234.573531555121));
#216275=CARTESIAN_POINT('Ctrl Pts',(-8.89842888688522,-63.0331158852246,
-234.575374277387));
#216276=CARTESIAN_POINT('Ctrl Pts',(-8.98341642645075,-63.0507193140023,
-234.578143293289));
#216277=CARTESIAN_POINT('Ctrl Pts',(-9.18182719302696,-63.0895137607373,
-234.584637642812));
#216278=CARTESIAN_POINT('Ctrl Pts',(-9.352062705706,-63.1188793895947,-234.590257702624));
#216279=CARTESIAN_POINT('Ctrl Pts',(-9.69272498154921,-63.1724789879354,
-234.601556701877));
#216280=CARTESIAN_POINT('Ctrl Pts',(-9.92006685579639,-63.2013610418528,
-234.609159841967));
#216281=CARTESIAN_POINT('Ctrl Pts',(-10.6028030210204,-63.2680315051849,
-234.632189424261));
#216282=CARTESIAN_POINT('Ctrl Pts',(-11.0589190335537,-63.2856900244449,
-234.647828473024));
#216283=CARTESIAN_POINT('Ctrl Pts',(-11.9727448912346,-63.2667333947121,
-234.679318210709));
#216284=CARTESIAN_POINT('Ctrl Pts',(-12.4302348513601,-63.2302711749144,
-234.695155702502));
#216285=CARTESIAN_POINT('Ctrl Pts',(-13.1181865020587,-63.1338298835409,
-234.718846244067));
#216286=CARTESIAN_POINT('Ctrl Pts',(-13.4626300973589,-63.0750435786505,
-234.730677939129));
#216287=CARTESIAN_POINT('Ctrl Pts',(-13.863319330679,-62.9878449235659,
-234.744290120853));
#216288=CARTESIAN_POINT('Ctrl Pts',(-14.0631260174647,-62.9395763466499,
-234.751027385112));
#216289=CARTESIAN_POINT('Ctrl Pts',(-14.1486155628969,-62.9178876098048,
-234.753897783854));
#216290=CARTESIAN_POINT('Ctrl Pts',(-14.2055812445659,-62.9032067723758,
-234.755807151484));
#216291=CARTESIAN_POINT('Ctrl Pts',(-14.2362308220828,-62.894753041772,
-234.757354927317));
#216292=CARTESIAN_POINT('Ctrl Pts',(-14.2619201924805,-62.8884582017248,
-234.757549593623));
#216293=CARTESIAN_POINT('Ctrl Pts',(-14.2619206252211,-62.8884600123608,
-234.757551008158));
#216294=CARTESIAN_POINT('Ctrl Pts',(-14.2718178205262,-62.8860359678618,
-234.757626045819));
#216295=CARTESIAN_POINT('Ctrl Pts',(-14.2804506465911,-62.884181158001,
-234.75735599456));
#216296=CARTESIAN_POINT('Ctrl Pts',(-14.2894789617138,-62.8821685292642,
-234.757191860054));
#216297=CARTESIAN_POINT('Ctrl Pts',(-14.2953100040955,-62.8808686495743,
-234.757085851873));
#216298=CARTESIAN_POINT('Ctrl Pts',(-14.3011413964139,-62.8795736434999,
-234.756979372388));
#216299=CARTESIAN_POINT('Ctrl Pts',(-14.3069731357651,-62.8782835068473,
-234.756872421387));
#216300=CARTESIAN_POINT('Ctrl Pts',(-14.3218342693705,-62.8749958267903,
-234.756599876094));
#216301=CARTESIAN_POINT('Ctrl Pts',(-14.3366976561142,-62.8717397684931,
-234.756324268863));
#216302=CARTESIAN_POINT('Ctrl Pts',(-14.3515632470811,-62.8685152641695,
-234.75604559438));
#216303=CARTESIAN_POINT('Ctrl Pts',(-14.379422206322,-62.8624723604785,
-234.755523342619));
#216304=CARTESIAN_POINT('Ctrl Pts',(-14.407288906641,-62.8565402762579,
-234.754990319625));
#216305=CARTESIAN_POINT('Ctrl Pts',(-14.4351630270212,-62.8507185672364,
-234.754446487672));
#216306=CARTESIAN_POINT('Ctrl Pts',(-14.4965309925101,-62.8379014295673,
-234.753249181352));
#216307=CARTESIAN_POINT('Ctrl Pts',(-14.5579349104097,-62.8256192347497,
-234.751999468502));
#216308=CARTESIAN_POINT('Ctrl Pts',(-14.6193714363495,-62.8138676057989,
-234.750697175335));
#216309=CARTESIAN_POINT('Ctrl Pts',(-14.6552123969003,-62.8070119175387,
-234.749937441003));
#216310=CARTESIAN_POINT('Ctrl Pts',(-14.6910644795143,-62.8003368602371,
-234.749159725648));
#216311=CARTESIAN_POINT('Ctrl Pts',(-14.7269270374636,-62.7938416077259,
-234.748363934128));
#216312=CARTESIAN_POINT('Ctrl Pts',(-14.8102586445982,-62.7787489913186,
-234.746514802607));
#216313=CARTESIAN_POINT('Ctrl Pts',(-14.8936466504724,-62.7646266721235,
-234.744568250047));
#216314=CARTESIAN_POINT('Ctrl Pts',(-14.977083853841,-62.7514672570885,
-234.742522108686));
#216315=CARTESIAN_POINT('Ctrl Pts',(-15.088565550686,-62.7338847656054,
-234.739788228574));
#216316=CARTESIAN_POINT('Ctrl Pts',(-15.2001350737935,-62.718021254317,
-234.736876561928));
#216317=CARTESIAN_POINT('Ctrl Pts',(-15.3117752750282,-62.7038591699904,
-234.733781825198));
#216318=CARTESIAN_POINT('Ctrl Pts',(-16.0925594070578,-62.60481303252,-234.712137997038));
#216319=CARTESIAN_POINT('Ctrl Pts',(-16.876935604951,-62.5885044241157,
-234.681761165031));
#216320=CARTESIAN_POINT('Ctrl Pts',(-17.6631922964109,-62.6514552500384,
-234.640496870595));
#216321=CARTESIAN_POINT('Ctrl Pts',(-18.4494489878708,-62.714406075961,
-234.59923257616));
#216322=CARTESIAN_POINT('Ctrl Pts',(-19.2438574482263,-62.8602959530961,
-234.546023767266));
#216323=CARTESIAN_POINT('Ctrl Pts',(-20.0008767707152,-63.072381283368,
-234.482033933863));
#216324=CARTESIAN_POINT('Ctrl Pts',(20.3180691938068,-61.7495111937247,
-235.35005));
#216325=CARTESIAN_POINT('Ctrl Pts',(19.4916837568995,-61.5513638467584,
-235.35005));
#216326=CARTESIAN_POINT('Ctrl Pts',(18.6602407015577,-61.4290562345849,
-235.350049999995));
#216327=CARTESIAN_POINT('Ctrl Pts',(17.8237010076361,-61.383180131545,-235.350049999998));
#216328=CARTESIAN_POINT('Ctrl Pts',(17.8193849653698,-61.3829434384136,
-235.350049999998));
#216329=CARTESIAN_POINT('Ctrl Pts',(17.8150687901225,-61.3827087804827,
-235.350049999998));
#216330=CARTESIAN_POINT('Ctrl Pts',(17.8107524818627,-61.3824761578263,
-235.350049999998));
#216331=CARTESIAN_POINT('Ctrl Pts',(17.2147892952599,-61.3503573814946,
-235.350050000001));
#216332=CARTESIAN_POINT('Ctrl Pts',(16.6152523367041,-61.3571390739688,
-235.350049999997));
#216333=CARTESIAN_POINT('Ctrl Pts',(16.0142818448677,-61.4050925383354,
-235.350049999997));
#216334=CARTESIAN_POINT('Ctrl Pts',(15.7759845903776,-61.4241070807416,
-235.350049999997));
#216335=CARTESIAN_POINT('Ctrl Pts',(15.5374618755672,-61.4495955645057,
-235.350049999998));
#216336=CARTESIAN_POINT('Ctrl Pts',(15.2988469678936,-61.4817018895299,
-235.350049999999));
#216337=CARTESIAN_POINT('Ctrl Pts',(15.2901306232776,-61.4828746988736,
-235.350049999999));
#216338=CARTESIAN_POINT('Ctrl Pts',(15.281414209221,-61.4840563352562,-235.350049999999));
#216339=CARTESIAN_POINT('Ctrl Pts',(15.2726977314404,-61.4852468054071,
-235.350049999999));
#216340=CARTESIAN_POINT('Ctrl Pts',(14.8590353180584,-61.5417435656889,
-235.350050000001));
#216341=CARTESIAN_POINT('Ctrl Pts',(14.4462075587129,-61.6179810575818,
-235.350049999997));
#216342=CARTESIAN_POINT('Ctrl Pts',(14.0341375328623,-61.7149985037554,
-235.350049999999));
#216343=CARTESIAN_POINT('Ctrl Pts',(14.0232833701672,-61.7175539993726,
-235.350049999999));
#216344=CARTESIAN_POINT('Ctrl Pts',(14.0124297591075,-61.7201239178539,
-235.350049999999));
#216345=CARTESIAN_POINT('Ctrl Pts',(14.0015767005386,-61.7227082779102,
-235.35005));
#216346=CARTESIAN_POINT('Ctrl Pts',(13.9751466240921,-61.7290018801626,
-235.35005));
#216347=CARTESIAN_POINT('Ctrl Pts',(13.9487179907097,-61.7353334612271,
-235.35005));
#216348=CARTESIAN_POINT('Ctrl Pts',(13.9222830160342,-61.7414997255267,
-235.35005));
#216349=CARTESIAN_POINT('Ctrl Pts',(13.8958480583747,-61.7476659858572,
-235.35005));
#216350=CARTESIAN_POINT('Ctrl Pts',(13.8694089796451,-61.7537248852831,
-235.35005));
#216351=CARTESIAN_POINT('Ctrl Pts',(13.8429657964072,-61.7596768227289,
-235.35005));
#216352=CARTESIAN_POINT('Ctrl Pts',(13.790079463996,-61.7715806899532,-235.35005));
#216353=CARTESIAN_POINT('Ctrl Pts',(13.7371767136853,-61.7830567143073,
-235.35005));
#216354=CARTESIAN_POINT('Ctrl Pts',(13.6842576766592,-61.7941080279422,
-235.35005));
#216355=CARTESIAN_POINT('Ctrl Pts',(13.590371291234,-61.8137147318752,-235.35005));
#216356=CARTESIAN_POINT('Ctrl Pts',(13.4964336431291,-61.8319846711038,
-235.35005));
#216357=CARTESIAN_POINT('Ctrl Pts',(13.4024454496957,-61.8489346854786,
-235.35005));
#216358=CARTESIAN_POINT('Ctrl Pts',(13.3904808193454,-61.8510924102844,
-235.35005));
#216359=CARTESIAN_POINT('Ctrl Pts',(13.3785153688655,-61.8532287455714,
-235.35005));
#216360=CARTESIAN_POINT('Ctrl Pts',(13.3665490995956,-61.8553437264012,
-235.35005));
#216361=CARTESIAN_POINT('Ctrl Pts',(13.1676684598094,-61.8904949277558,
-235.35005));
#216362=CARTESIAN_POINT('Ctrl Pts',(12.9685616944886,-61.9197485683524,
-235.35005));
#216363=CARTESIAN_POINT('Ctrl Pts',(12.769234453532,-61.9432531346425,-235.35005));
#216364=CARTESIAN_POINT('Ctrl Pts',(12.7561510301933,-61.94479592523,-235.35005));
#216365=CARTESIAN_POINT('Ctrl Pts',(12.7430666547525,-61.9463139461232,
-235.35005));
#216366=CARTESIAN_POINT('Ctrl Pts',(12.7299813289277,-61.9478072392615,
-235.35005));
#216367=CARTESIAN_POINT('Ctrl Pts',(11.8976622152407,-62.0427912265134,
-235.35005));
#216368=CARTESIAN_POINT('Ctrl Pts',(11.0615444015933,-62.0389160797901,
-235.350050000034));
#216369=CARTESIAN_POINT('Ctrl Pts',(10.2215623565589,-61.9338804974863,
-235.350049999966));
#216370=CARTESIAN_POINT('Ctrl Pts',(10.2039545597188,-61.9316787299544,
-235.350049999965));
#216371=CARTESIAN_POINT('Ctrl Pts',(10.1863450394511,-61.9294324012865,
-235.350049999964));
#216372=CARTESIAN_POINT('Ctrl Pts',(10.1687337982121,-61.9271415054827,
-235.350049999964));
#216373=CARTESIAN_POINT('Ctrl Pts',(9.97300635380698,-61.9016809956297,
-235.350049999962));
#216374=CARTESIAN_POINT('Ctrl Pts',(9.77706380796946,-61.8706389534041,
-235.35005));
#216375=CARTESIAN_POINT('Ctrl Pts',(9.58090054516818,-61.8338427891411,
-235.35005));
#216376=CARTESIAN_POINT('Ctrl Pts',(9.56214700042038,-61.8303250126563,
-235.35005));
#216377=CARTESIAN_POINT('Ctrl Pts',(9.54339143257748,-61.8267545360138,
-235.35005));
#216378=CARTESIAN_POINT('Ctrl Pts',(9.52463383590975,-61.8231311921276,
-235.35005));
#216379=CARTESIAN_POINT('Ctrl Pts',(9.43646147497583,-61.8060992241956,
-235.35005));
#216380=CARTESIAN_POINT('Ctrl Pts',(9.34824426520709,-61.7878985163246,
-235.35005));
#216381=CARTESIAN_POINT('Ctrl Pts',(9.25998147071924,-61.7685085402422,
-235.35005));
#216382=CARTESIAN_POINT('Ctrl Pts',(9.24065237676121,-61.7642622361034,
-235.35005));
#216383=CARTESIAN_POINT('Ctrl Pts',(9.2213210949948,-61.7599588859415,-235.35005));
#216384=CARTESIAN_POINT('Ctrl Pts',(9.20198761712391,-61.7555982713279,
-235.35005));
#216385=CARTESIAN_POINT('Ctrl Pts',(9.17508354314347,-61.7495301288578,
-235.35005));
#216386=CARTESIAN_POINT('Ctrl Pts',(9.14817521564248,-61.7433510739016,
-235.35005));
#216387=CARTESIAN_POINT('Ctrl Pts',(9.12126261063577,-61.7370604761635,
-235.35005));
#216388=CARTESIAN_POINT('Ctrl Pts',(9.10780630869731,-61.7339151774265,
-235.35005));
#216389=CARTESIAN_POINT('Ctrl Pts',(9.09434839935842,-61.7307279624413,
-235.35005));
#216390=CARTESIAN_POINT('Ctrl Pts',(9.0808907308651,-61.7275470288336,-235.35005));
#216391=CARTESIAN_POINT('Ctrl Pts',(9.06743306257898,-61.724366095275,-235.35005));
#216392=CARTESIAN_POINT('Ctrl Pts',(9.0539762218753,-61.7212067460947,-235.35005));
#216393=CARTESIAN_POINT('Ctrl Pts',(9.04052020712007,-61.7180689383617,
-235.35005));
#216394=CARTESIAN_POINT('Ctrl Pts',(9.00658789206205,-61.7101562626903,
-235.35005));
#216395=CARTESIAN_POINT('Ctrl Pts',(8.97266082904071,-61.7023805649868,
-235.35005));
#216396=CARTESIAN_POINT('Ctrl Pts',(8.93873899316592,-61.6947411877276,
-235.35005));
#216397=CARTESIAN_POINT('Ctrl Pts',(8.91885339025561,-61.6902628445383,
-235.35005));
#216398=CARTESIAN_POINT('Ctrl Pts',(8.8989695829772,-61.6858313592565,-235.35005));
#216399=CARTESIAN_POINT('Ctrl Pts',(8.87908756640826,-61.681446597423,-235.35005));
#216400=CARTESIAN_POINT('Ctrl Pts',(8.47079682602659,-61.5914025292461,
-235.35005));
#216401=CARTESIAN_POINT('Ctrl Pts',(8.06325955820407,-61.5210088750398,
-235.350049999991));
#216402=CARTESIAN_POINT('Ctrl Pts',(7.65644449495009,-61.4694578795698,
-235.350049999996));
#216403=CARTESIAN_POINT('Ctrl Pts',(7.63443323033068,-61.4666686450867,
-235.350049999996));
#216404=CARTESIAN_POINT('Ctrl Pts',(7.6124240795152,-61.4639346190844,-235.350049999996));
#216405=CARTESIAN_POINT('Ctrl Pts',(7.59041703822612,-61.4612556735992,
-235.350049999996));
#216406=CARTESIAN_POINT('Ctrl Pts',(6.81378158900793,-61.3667148399189,
-235.35005));
#216407=CARTESIAN_POINT('Ctrl Pts',(6.03976429892115,-61.3404212594767,
-235.350049999767));
#216408=CARTESIAN_POINT('Ctrl Pts',(5.26831576742253,-61.3810871329348,
-235.350049999921));
#216409=CARTESIAN_POINT('Ctrl Pts',(5.21423514782724,-61.3839379201788,
-235.350049999931));
#216410=CARTESIAN_POINT('Ctrl Pts',(5.16016713150992,-61.3871177761328,
-235.350049999943));
#216411=CARTESIAN_POINT('Ctrl Pts',(5.10611169220526,-61.3906262588808,
-235.350049999955));
#216412=CARTESIAN_POINT('Ctrl Pts',(5.07989180169939,-61.392328067888,-235.35004999996));
#216413=CARTESIAN_POINT('Ctrl Pts',(5.05367487339116,-61.3941073070012,
-235.350049999965));
#216414=CARTESIAN_POINT('Ctrl Pts',(5.02746090657059,-61.3959639238493,
-235.350049999969));
#216415=CARTESIAN_POINT('Ctrl Pts',(4.63027321936536,-61.4240949334362,
-235.350050000029));
#216416=CARTESIAN_POINT('Ctrl Pts',(4.2337696766697,-61.4700888214833,-235.350049999999));
#216417=CARTESIAN_POINT('Ctrl Pts',(3.83796788150582,-61.5343657809992,
-235.35005));
#216418=CARTESIAN_POINT('Ctrl Pts',(3.8096685116519,-61.5389615091455,-235.35005));
#216419=CARTESIAN_POINT('Ctrl Pts',(3.78137272363524,-61.5436507557365,
-235.35005));
#216420=CARTESIAN_POINT('Ctrl Pts',(3.75308052471073,-61.5484336724786,
-235.35005));
#216421=CARTESIAN_POINT('Ctrl Pts',(3.57046403317894,-61.5793057682484,
-235.35005));
#216422=CARTESIAN_POINT('Ctrl Pts',(3.38799716939791,-61.6140822120622,
-235.35005));
#216423=CARTESIAN_POINT('Ctrl Pts',(3.20568284456817,-61.6528339368697,
-235.35005));
#216424=CARTESIAN_POINT('Ctrl Pts',(3.17635110102161,-61.6590685300927,
-235.35005));
#216425=CARTESIAN_POINT('Ctrl Pts',(3.14702330190727,-61.6654060761275,
-235.35005));
#216426=CARTESIAN_POINT('Ctrl Pts',(3.11769946035167,-61.671846868513,-235.35005));
#216427=CARTESIAN_POINT('Ctrl Pts',(3.04177180936077,-61.6885238866119,
-235.35005));
#216428=CARTESIAN_POINT('Ctrl Pts',(2.96587070637591,-61.705893475931,-235.35005));
#216429=CARTESIAN_POINT('Ctrl Pts',(2.88999643518129,-61.7239624137673,
-235.35005));
#216430=CARTESIAN_POINT('Ctrl Pts',(2.86015055692824,-61.7310700051857,
-235.35005));
#216431=CARTESIAN_POINT('Ctrl Pts',(2.830308828251,-61.7382858215616,-235.35005));
#216432=CARTESIAN_POINT('Ctrl Pts',(2.80047126555685,-61.7456102857936,
-235.35005));
#216433=CARTESIAN_POINT('Ctrl Pts',(2.7740485916509,-61.7520964700681,-235.35005));
#216434=CARTESIAN_POINT('Ctrl Pts',(2.74762918531567,-61.7586678715823,
-235.35005));
#216435=CARTESIAN_POINT('Ctrl Pts',(2.72121305914134,-61.7653248158681,
-235.35005));
#216436=CARTESIAN_POINT('Ctrl Pts',(2.70800499628476,-61.7686532879529,
-235.35005));
#216437=CARTESIAN_POINT('Ctrl Pts',(2.69479775347656,-61.7720031458945,
-235.35005));
#216438=CARTESIAN_POINT('Ctrl Pts',(2.68159133233768,-61.7753744316497,
-235.35005));
#216439=CARTESIAN_POINT('Ctrl Pts',(2.66838491128433,-61.778745717383,-235.35005));
#216440=CARTESIAN_POINT('Ctrl Pts',(2.65517833756298,-61.7821130218478,
-235.35005));
#216441=CARTESIAN_POINT('Ctrl Pts',(2.64197036381524,-61.7854438146496,
-235.35005));
#216442=CARTESIAN_POINT('Ctrl Pts',(2.61951079935543,-61.7911076777874,
-235.35005));
#216443=CARTESIAN_POINT('Ctrl Pts',(2.59704830033213,-61.796695009813,-235.35005));
#216444=CARTESIAN_POINT('Ctrl Pts',(2.57458287671426,-61.8022060694146,
-235.35005));
#216445=CARTESIAN_POINT('Ctrl Pts',(2.5442030896625,-61.8096586249493,-235.35005));
#216446=CARTESIAN_POINT('Ctrl Pts',(2.51381779758875,-61.8169717426775,
-235.35005));
#216447=CARTESIAN_POINT('Ctrl Pts',(2.4834260939684,-61.8241462703205,-235.35005));
#216448=CARTESIAN_POINT('Ctrl Pts',(2.29145411020807,-61.8694648322997,
-235.35005));
#216449=CARTESIAN_POINT('Ctrl Pts',(2.09905435586468,-61.9092920576156,
-235.35005));
#216450=CARTESIAN_POINT('Ctrl Pts',(1.90636342421814,-61.9437627651672,
-235.35005));
#216451=CARTESIAN_POINT('Ctrl Pts',(1.71259196379615,-61.9784267697832,
-235.35005));
#216452=CARTESIAN_POINT('Ctrl Pts',(1.51852542212224,-62.0076738986067,
-235.35005));
#216453=CARTESIAN_POINT('Ctrl Pts',(1.32430920160843,-62.0315892709352,
-235.35005));
#216454=CARTESIAN_POINT('Ctrl Pts',(1.28723208664458,-62.0361548680149,
-235.35005));
#216455=CARTESIAN_POINT('Ctrl Pts',(1.25014955173931,-62.0405259994938,
-235.35005));
#216456=CARTESIAN_POINT('Ctrl Pts',(1.21306266525719,-62.0447030491234,
-235.35005));
#216457=CARTESIAN_POINT('Ctrl Pts',(1.01359698141616,-62.0671686195675,
-235.35005));
#216458=CARTESIAN_POINT('Ctrl Pts',(0.813911238500945,-62.0840519390958,
-235.35005));
#216459=CARTESIAN_POINT('Ctrl Pts',(0.61374718436545,-62.0953851249273,
-235.350049999999));
#216460=CARTESIAN_POINT('Ctrl Pts',(0.420827571211818,-62.1063081342351,
-235.350049999998));
#216461=CARTESIAN_POINT('Ctrl Pts',(0.227463671021064,-62.112075061559,
-235.350049999997));
#216462=CARTESIAN_POINT('Ctrl Pts',(0.0334272952674007,-62.1126689560032,
-235.350049999994));
#216463=CARTESIAN_POINT('Ctrl Pts',(0.00561364330087405,-62.1127540862954,
-235.350049999994));
#216464=CARTESIAN_POINT('Ctrl Pts',(-0.0221859314783799,-62.112732748585,
-235.350049999994));
#216465=CARTESIAN_POINT('Ctrl Pts',(-0.0499714044288816,-62.1126054680541,
-235.350049999993));
#216466=CARTESIAN_POINT('Ctrl Pts',(-0.390902815368587,-62.1110437191836,
-235.35004999999));
#216467=CARTESIAN_POINT('Ctrl Pts',(-0.72972011692128,-62.093667945123,
-235.350049999991));
#216468=CARTESIAN_POINT('Ctrl Pts',(-1.06631300987704,-62.0604683301881,
-235.350049999993));
#216469=CARTESIAN_POINT('Ctrl Pts',(-1.40121239647694,-62.0274357531202,
-235.350049999995));
#216470=CARTESIAN_POINT('Ctrl Pts',(-1.73390970131595,-61.9787381431651,
-235.350049999997));
#216471=CARTESIAN_POINT('Ctrl Pts',(-2.06430030241362,-61.914417278251,
-235.350049999996));
#216472=CARTESIAN_POINT('Ctrl Pts',(-2.20642338591151,-61.8867485745274,
-235.350049999995));
#216473=CARTESIAN_POINT('Ctrl Pts',(-2.34811967953794,-61.856189539284,
-235.350049999994));
#216474=CARTESIAN_POINT('Ctrl Pts',(-2.48938108575845,-61.8227464619276,
-235.350049999991));
#216475=CARTESIAN_POINT('Ctrl Pts',(-2.50854491166961,-61.8182095021908,
-235.35004999999));
#216476=CARTESIAN_POINT('Ctrl Pts',(-2.52769858741776,-61.8136197387286,
-235.350049999991));
#216477=CARTESIAN_POINT('Ctrl Pts',(-2.54684411204869,-61.8089768066246,
-235.350049999992));
#216478=CARTESIAN_POINT('Ctrl Pts',(-2.57265412059171,-61.8027176876096,
-235.350049999993));
#216479=CARTESIAN_POINT('Ctrl Pts',(-2.59844921754894,-61.7963604695819,
-235.350049999995));
#216480=CARTESIAN_POINT('Ctrl Pts',(-2.62423428592014,-61.7899039637969,
-235.350049999996));
#216481=CARTESIAN_POINT('Ctrl Pts',(-2.63712994504912,-61.7866749284277,
-235.350049999997));
#216482=CARTESIAN_POINT('Ctrl Pts',(-2.65002309577879,-61.7834210571593,
-235.350049999998));
#216483=CARTESIAN_POINT('Ctrl Pts',(-2.66291434866892,-61.780142189443,
-235.350049999998));
#216484=CARTESIAN_POINT('Ctrl Pts',(-2.6758060675559,-61.7768632032012,
-235.350049999999));
#216485=CARTESIAN_POINT('Ctrl Pts',(-2.68869578886317,-61.7735577831395,
-235.350049999999));
#216486=CARTESIAN_POINT('Ctrl Pts',(-2.7015882408541,-61.7702876349097,
-235.350049999999));
#216487=CARTESIAN_POINT('Ctrl Pts',(-2.73400113694554,-61.7620661596735,
-235.35005));
#216488=CARTESIAN_POINT('Ctrl Pts',(-2.76642495453173,-61.7539722710786,
-235.35005));
#216489=CARTESIAN_POINT('Ctrl Pts',(-2.79886940013938,-61.7460035995909,
-235.35005));
#216490=CARTESIAN_POINT('Ctrl Pts',(-2.81802683545117,-61.7412983470989,
-235.35005));
#216491=CARTESIAN_POINT('Ctrl Pts',(-2.83719059223805,-61.7366367673477,
-235.35005));
#216492=CARTESIAN_POINT('Ctrl Pts',(-2.85636066288065,-61.7320188020896,
-235.35005));
#216493=CARTESIAN_POINT('Ctrl Pts',(-2.94045564063812,-61.7117607815058,
-235.35005));
#216494=CARTESIAN_POINT('Ctrl Pts',(-3.02467211402759,-61.6923419671876,
-235.35005));
#216495=CARTESIAN_POINT('Ctrl Pts',(-3.10900951525852,-61.6737585224186,
-235.35005));
#216496=CARTESIAN_POINT('Ctrl Pts',(-3.12809762617752,-61.669552525437,
-235.35005));
#216497=CARTESIAN_POINT('Ctrl Pts',(-3.14719143793448,-61.6653894344847,
-235.35005));
#216498=CARTESIAN_POINT('Ctrl Pts',(-3.16629058179914,-61.6612692744985,
-235.35005));
#216499=CARTESIAN_POINT('Ctrl Pts',(-3.3544366248314,-61.6206814971847,
-235.35005));
#216500=CARTESIAN_POINT('Ctrl Pts',(-3.5430471591718,-61.5842760792721,
-235.35005));
#216501=CARTESIAN_POINT('Ctrl Pts',(-3.73167328165468,-61.5520701874165,
-235.35005));
#216502=CARTESIAN_POINT('Ctrl Pts',(-3.75023101873764,-61.5489016524028,
-235.35005));
#216503=CARTESIAN_POINT('Ctrl Pts',(-3.76879003495516,-61.5457735306668,
-235.35005));
#216504=CARTESIAN_POINT('Ctrl Pts',(-3.78735023209142,-61.5426857671793,
-235.35005));
#216505=CARTESIAN_POINT('Ctrl Pts',(-4.18439312155204,-61.4766318062188,
-235.35005));
#216506=CARTESIAN_POINT('Ctrl Pts',(-4.58211759857741,-61.4290090167846,
-235.350049999998));
#216507=CARTESIAN_POINT('Ctrl Pts',(-4.98047798851508,-61.3993682153446,
-235.350049999999));
#216508=CARTESIAN_POINT('Ctrl Pts',(-4.99789438884674,-61.3980723132492,
-235.350049999999));
#216509=CARTESIAN_POINT('Ctrl Pts',(-5.01531202614922,-61.3968107958183,
-235.350049999999));
#216510=CARTESIAN_POINT('Ctrl Pts',(-5.03273089884151,-61.3955836250763,
-235.350049999999));
#216511=CARTESIAN_POINT('Ctrl Pts',(-5.84939476240443,-61.3380491326227,
-235.35005));
#216512=CARTESIAN_POINT('Ctrl Pts',(-6.66875666758943,-61.3556213316307,
-235.350049999913));
#216513=CARTESIAN_POINT('Ctrl Pts',(-7.4908586829273,-61.4495145762377,
-235.350049999982));
#216514=CARTESIAN_POINT('Ctrl Pts',(-7.50596678336512,-61.4512400902779,
-235.350049999983));
#216515=CARTESIAN_POINT('Ctrl Pts',(-7.52107585673405,-61.4529914065635,
-235.350049999985));
#216516=CARTESIAN_POINT('Ctrl Pts',(-7.53618589852398,-61.4547685325697,
-235.350049999986));
#216517=CARTESIAN_POINT('Ctrl Pts',(-7.94094824234007,-61.5023735423717,
-235.350050000014));
#216518=CARTESIAN_POINT('Ctrl Pts',(-8.34552450700488,-61.5685466677726,
-235.35005));
#216519=CARTESIAN_POINT('Ctrl Pts',(-8.74831622488394,-61.6532732073253,
-235.35005));
#216520=CARTESIAN_POINT('Ctrl Pts',(-8.7621454779902,-61.656182166741,-235.35005));
#216521=CARTESIAN_POINT('Ctrl Pts',(-8.77597283009793,-61.6591130351084,
-235.35005));
#216522=CARTESIAN_POINT('Ctrl Pts',(-8.78979820740338,-61.6620658114437,
-235.35005));
#216523=CARTESIAN_POINT('Ctrl Pts',(-8.84186271017304,-61.6731855681264,
-235.35005));
#216524=CARTESIAN_POINT('Ctrl Pts',(-8.89390698318748,-61.6846175978045,
-235.35005));
#216525=CARTESIAN_POINT('Ctrl Pts',(-8.94593027529996,-61.6963628074412,
-235.35005));
#216526=CARTESIAN_POINT('Ctrl Pts',(-8.97194109726227,-61.7022352262052,
-235.35005));
#216527=CARTESIAN_POINT('Ctrl Pts',(-8.99794667422061,-61.708185936652,
-235.35005));
#216528=CARTESIAN_POINT('Ctrl Pts',(-9.02394691154399,-61.7142150623191,
-235.35005));
#216529=CARTESIAN_POINT('Ctrl Pts',(-9.04994682503898,-61.7202441128945,
-235.35005));
#216530=CARTESIAN_POINT('Ctrl Pts',(-9.07593826995543,-61.7263961529626,
-235.35005));
#216531=CARTESIAN_POINT('Ctrl Pts',(-9.10193156111664,-61.7325230165495,
-235.35005));
#216532=CARTESIAN_POINT('Ctrl Pts',(-9.19270265836824,-61.7539186192474,
-235.35005));
#216533=CARTESIAN_POINT('Ctrl Pts',(-9.28356162147515,-61.7740761143559,
-235.35005));
#216534=CARTESIAN_POINT('Ctrl Pts',(-9.37450399412181,-61.7930068611338,
-235.35005));
#216535=CARTESIAN_POINT('Ctrl Pts',(-9.38773105410519,-61.7957602324817,
-235.35005));
#216536=CARTESIAN_POINT('Ctrl Pts',(-9.40095993474415,-61.798487664451,
-235.35005));
#216537=CARTESIAN_POINT('Ctrl Pts',(-9.41419063343487,-61.8011891942708,
-235.35005));
#216538=CARTESIAN_POINT('Ctrl Pts',(-9.60996310615498,-61.8411632867438,
-235.35005));
#216539=CARTESIAN_POINT('Ctrl Pts',(-9.80613347328001,-61.8754684024255,
-235.35005));
#216540=CARTESIAN_POINT('Ctrl Pts',(-10.0026951820956,-61.9041989502093,
-235.35005));
#216541=CARTESIAN_POINT('Ctrl Pts',(-10.0153727130177,-61.9060519683283,
-235.35005));
#216542=CARTESIAN_POINT('Ctrl Pts',(-10.0280518731001,-61.907881795828,
-235.35005));
#216543=CARTESIAN_POINT('Ctrl Pts',(-10.0407326605036,-61.9096884579721,
-235.35005));
#216544=CARTESIAN_POINT('Ctrl Pts',(-10.8676504683673,-62.0275014180156,
-235.35005));
#216545=CARTESIAN_POINT('Ctrl Pts',(-11.701383578359,-62.0482829945994,
-235.350050000035));
#216546=CARTESIAN_POINT('Ctrl Pts',(-12.542235654937,-61.9675412878384,
-235.350049999962));
#216547=CARTESIAN_POINT('Ctrl Pts',(-12.5526626108316,-61.9665400532114,
-235.350049999961));
#216548=CARTESIAN_POINT('Ctrl Pts',(-12.563090680639,-61.9655231957799,
-235.35004999996));
#216549=CARTESIAN_POINT('Ctrl Pts',(-12.5735198637114,-61.9644907071475,
-235.350049999959));
#216550=CARTESIAN_POINT('Ctrl Pts',(-12.9900551329717,-61.9232537351325,
-235.350049999926));
#216551=CARTESIAN_POINT('Ctrl Pts',(-13.4095020772858,-61.8565248169554,
-235.350049999993));
#216552=CARTESIAN_POINT('Ctrl Pts',(-13.8265285083935,-61.7633636199134,
-235.350049999999));
#216553=CARTESIAN_POINT('Ctrl Pts',(-13.8357346646875,-61.7613070199559,
-235.350049999999));
#216554=CARTESIAN_POINT('Ctrl Pts',(-13.8449397537504,-61.7592375264678,
-235.350049999999));
#216555=CARTESIAN_POINT('Ctrl Pts',(-13.8541437081179,-61.7571551297028,
-235.350049999999));
#216556=CARTESIAN_POINT('Ctrl Pts',(-13.8807773975261,-61.7511292514281,
-235.35005));
#216557=CARTESIAN_POINT('Ctrl Pts',(-13.9074041843247,-61.7449954922066,
-235.35005));
#216558=CARTESIAN_POINT('Ctrl Pts',(-13.9340237809303,-61.7387535487581,
-235.35005));
#216559=CARTESIAN_POINT('Ctrl Pts',(-13.947333274867,-61.7356326484036,
-235.35005));
#216560=CARTESIAN_POINT('Ctrl Pts',(-13.9606409713357,-61.7324847033371,
-235.35005));
#216561=CARTESIAN_POINT('Ctrl Pts',(-13.9739468343463,-61.729309676058,
-235.35005));
#216562=CARTESIAN_POINT('Ctrl Pts',(-13.9872525811354,-61.7261346765115,
-235.35005));
#216563=CARTESIAN_POINT('Ctrl Pts',(-14.0005572003786,-61.7229426931068,
-235.35005));
#216564=CARTESIAN_POINT('Ctrl Pts',(-14.0138644113966,-61.7197873591981,
-235.35005));
#216565=CARTESIAN_POINT('Ctrl Pts',(-14.0582045235932,-61.7092736715937,
-235.35005));
#216566=CARTESIAN_POINT('Ctrl Pts',(-14.1025617323967,-61.6989999801743,
-235.35005));
#216567=CARTESIAN_POINT('Ctrl Pts',(-14.1469346979652,-61.6889648766594,
-235.35005));
#216568=CARTESIAN_POINT('Ctrl Pts',(-14.1558301130274,-61.6869531469989,
-235.35005));
#216569=CARTESIAN_POINT('Ctrl Pts',(-14.1647261982595,-61.6849509976523,
-235.35005));
#216570=CARTESIAN_POINT('Ctrl Pts',(-14.1736229527744,-61.6829584159335,
-235.35005));
#216571=CARTESIAN_POINT('Ctrl Pts',(-14.2715888956296,-61.6610172522806,
-235.35005));
#216572=CARTESIAN_POINT('Ctrl Pts',(-14.36963597373,-61.6402359551837,-235.35005));
#216573=CARTESIAN_POINT('Ctrl Pts',(-14.4677631872782,-61.6206001654354,
-235.35005));
#216574=CARTESIAN_POINT('Ctrl Pts',(-14.476365220368,-61.6188788517748,
-235.35005));
#216575=CARTESIAN_POINT('Ctrl Pts',(-14.4849678693149,-61.6171663419628,
-235.35005));
#216576=CARTESIAN_POINT('Ctrl Pts',(-14.4935711334409,-61.6154626263395,
-235.35005));
#216577=CARTESIAN_POINT('Ctrl Pts',(-14.6990757335377,-61.5747662821716,
-235.35005));
#216578=CARTESIAN_POINT('Ctrl Pts',(-14.9049310961046,-61.5390843579523,
-235.35005));
#216579=CARTESIAN_POINT('Ctrl Pts',(-15.1111310124904,-61.5083276273384,
-235.35005));
#216580=CARTESIAN_POINT('Ctrl Pts',(-15.119142468619,-61.5071326404427,
-235.35005));
#216581=CARTESIAN_POINT('Ctrl Pts',(-15.1271544450248,-61.505945089522,
-235.35005));
#216582=CARTESIAN_POINT('Ctrl Pts',(-15.1351669413377,-61.5047649693728,
-235.35005));
#216583=CARTESIAN_POINT('Ctrl Pts',(-15.9865951750349,-61.3793624013096,
-235.35005));
#216584=CARTESIAN_POINT('Ctrl Pts',(-16.843857444274,-61.3373584768896,
-235.350049999987));
#216585=CARTESIAN_POINT('Ctrl Pts',(-17.7068495304908,-61.3772749311671,
-235.350049999996));
#216586=CARTESIAN_POINT('Ctrl Pts',(-17.7124533012131,-61.3775341254997,
-235.350049999996));
#216587=CARTESIAN_POINT('Ctrl Pts',(-17.7180571389861,-61.3777967664626,
-235.350049999996));
#216588=CARTESIAN_POINT('Ctrl Pts',(-17.7236610495722,-61.3780628532939,
-235.350049999996));
#216589=CARTESIAN_POINT('Ctrl Pts',(-17.9268662020405,-61.387711511008,
-235.350049999998));
#216590=CARTESIAN_POINT('Ctrl Pts',(-18.1305704995353,-61.4020849580281,
-235.350049999999));
#216591=CARTESIAN_POINT('Ctrl Pts',(-18.3343978331705,-61.421036350068,
-235.350049999999));
#216592=CARTESIAN_POINT('Ctrl Pts',(-18.5413055198001,-61.4402741461744,
-235.35005));
#216593=CARTESIAN_POINT('Ctrl Pts',(-18.7483412532968,-61.4642294656438,
-235.35005));
#216594=CARTESIAN_POINT('Ctrl Pts',(-18.95511001473,-61.4928010494512,-235.35005));
#216595=CARTESIAN_POINT('Ctrl Pts',(-19.1581684655807,-61.5208599375833,
-235.35005));
#216596=CARTESIAN_POINT('Ctrl Pts',(-19.3609706050519,-61.5533713065191,
-235.35005));
#216597=CARTESIAN_POINT('Ctrl Pts',(-19.5631227327773,-61.5902847141104,
-235.35005));
#216598=CARTESIAN_POINT('Ctrl Pts',(-19.7559941247032,-61.6255034396464,
-235.35005));
#216599=CARTESIAN_POINT('Ctrl Pts',(-19.9482746078014,-61.6647297766438,
-235.35005));
#216600=CARTESIAN_POINT('Ctrl Pts',(-20.1395905386961,-61.7079550103905,
-235.35005));
#216601=CARTESIAN_POINT('Ctrl Pts',(-20.1991813366268,-61.7214187410775,
-235.35005));
#216602=CARTESIAN_POINT('Ctrl Pts',(-20.2586782689426,-61.7352706787151,
-235.35005));
#216603=CARTESIAN_POINT('Ctrl Pts',(-20.3180691938068,-61.7495111937247,
-235.35005));
#216604=CARTESIAN_POINT('',(14.2619189241969,-62.8884528813233,-234.757545437753));
#216605=CARTESIAN_POINT('Ctrl Pts',(14.2619189241969,-62.8884528813233,
-234.757545437753));
#216606=CARTESIAN_POINT('Ctrl Pts',(14.2676221315376,-62.8870512825747,
-234.757599285427));
#216607=CARTESIAN_POINT('Ctrl Pts',(14.27309559464,-62.8857530533057,-234.757590335366));
#216608=CARTESIAN_POINT('Ctrl Pts',(14.2782562309469,-62.8845979535437,
-234.75749584595));
#216609=CARTESIAN_POINT('Ctrl Pts',(14.4728210423908,-62.8410487177465,
-234.753933433427));
#216610=CARTESIAN_POINT('Ctrl Pts',(14.6676054707436,-62.8029521711093,
-234.749855174901));
#216611=CARTESIAN_POINT('Ctrl Pts',(14.862267472532,-62.7701957889222,-234.74525442655));
#216612=CARTESIAN_POINT('Ctrl Pts',(15.0540973159843,-62.7379159828518,
-234.74072061498));
#216613=CARTESIAN_POINT('Ctrl Pts',(15.2458081247477,-62.7108217116278,
-234.735679369408));
#216614=CARTESIAN_POINT('Ctrl Pts',(15.4370736548847,-62.6887561762043,
-234.730130586681));
#216615=CARTESIAN_POINT('Ctrl Pts',(15.5314733326893,-62.6778656648139,
-234.727391968273));
#216616=CARTESIAN_POINT('Ctrl Pts',(15.6257144198455,-62.6682049982271,
-234.72453379674));
#216617=CARTESIAN_POINT('Ctrl Pts',(15.7197562183719,-62.6597512994103,
-234.721556787451));
#216618=CARTESIAN_POINT('Ctrl Pts',(15.9194398772557,-62.6418011374898,
-234.715235554589));
#216619=CARTESIAN_POINT('Ctrl Pts',(16.1183147406937,-62.6293052674362,
-234.708351013767));
#216620=CARTESIAN_POINT('Ctrl Pts',(16.3159941005111,-62.6220209771202,
-234.700911847004));
#216621=CARTESIAN_POINT('Ctrl Pts',(16.3574225292628,-62.6204943801976,
-234.699352792025));
#216622=CARTESIAN_POINT('Ctrl Pts',(16.3987984837776,-62.6191965047478,
-234.69776940586));
#216623=CARTESIAN_POINT('Ctrl Pts',(16.4401184612598,-62.6181248397371,
-234.696161814787));
#216624=CARTESIAN_POINT('Ctrl Pts',(16.5593593875656,-62.615032235715,-234.691522638766));
#216625=CARTESIAN_POINT('Ctrl Pts',(16.6781351876571,-62.6138244557668,
-234.68668086609));
#216626=CARTESIAN_POINT('Ctrl Pts',(16.7963700013562,-62.6144400515916,
-234.681635659345));
#216627=CARTESIAN_POINT('Ctrl Pts',(16.8554874082058,-62.6147478495039,
-234.679113055972));
#216628=CARTESIAN_POINT('Ctrl Pts',(16.9144695680729,-62.6155114373711,
-234.676539558438));
#216629=CARTESIAN_POINT('Ctrl Pts',(16.9733077389818,-62.6167227855682,
-234.673914918543));
#216630=CARTESIAN_POINT('Ctrl Pts',(17.0027268244363,-62.6173284596667,
-234.672602598595));
#216631=CARTESIAN_POINT('Ctrl Pts',(17.0321099129192,-62.6180460709255,
-234.671277491313));
#216632=CARTESIAN_POINT('Ctrl Pts',(17.0614559345793,-62.6188745972855,
-234.669939556944));
#216633=CARTESIAN_POINT('Ctrl Pts',(17.0847044612134,-62.6195309730414,
-234.668879617605));
#216634=CARTESIAN_POINT('Ctrl Pts',(17.1070374630585,-62.6202275257495,
-234.667852866661));
#216635=CARTESIAN_POINT('Ctrl Pts',(17.1305750905829,-62.621033000521,-234.666761357511));
#216636=CARTESIAN_POINT('Ctrl Pts',(17.136748409392,-62.6212442559907,-234.666475082526));
#216637=CARTESIAN_POINT('Ctrl Pts',(17.1430045641319,-62.6214632738738,
-234.666184319474));
#216638=CARTESIAN_POINT('Ctrl Pts',(17.1493817430919,-62.6216918876598,
-234.665887227365));
#216639=CARTESIAN_POINT('Ctrl Pts',(17.3478766374233,-62.6288076781356,
-234.656639993278));
#216640=CARTESIAN_POINT('Ctrl Pts',(17.5455520004757,-62.6410046705095,
-234.646771670025));
#216641=CARTESIAN_POINT('Ctrl Pts',(17.742009985154,-62.6580565731071,-234.636283597108));
#216642=CARTESIAN_POINT('Ctrl Pts',(17.9389575403572,-62.6751509688054,
-234.625769388061));
#216643=CARTESIAN_POINT('Ctrl Pts',(18.1347846733241,-62.6971222883386,
-234.614612391247));
#216644=CARTESIAN_POINT('Ctrl Pts',(18.3292291451991,-62.7237598595182,
-234.602804984691));
#216645=CARTESIAN_POINT('Ctrl Pts',(18.5259098814926,-62.7507037837252,
-234.590861783669));
#216646=CARTESIAN_POINT('Ctrl Pts',(18.7211759890429,-62.7824217829876,
-234.57825304333));
#216647=CARTESIAN_POINT('Ctrl Pts',(18.9147618610651,-62.8186429668106,
-234.56498137667));
#216648=CARTESIAN_POINT('Ctrl Pts',(19.1126402616024,-62.8556673108167,
-234.551415427131));
#216649=CARTESIAN_POINT('Ctrl Pts',(19.3087631000518,-62.8973966834212,
-234.537156722191));
#216650=CARTESIAN_POINT('Ctrl Pts',(19.5028524817591,-62.943488244167,-234.522220426416));
#216651=CARTESIAN_POINT('Ctrl Pts',(19.6704349995014,-62.9832850621511,
-234.509323986488));
#216652=CARTESIAN_POINT('Ctrl Pts',(19.8365016601851,-63.0263329686421,
-234.49592257589));
#216653=CARTESIAN_POINT('Ctrl Pts',(20.0008767707152,-63.0723812833681,
-234.482033933862));
#216654=CARTESIAN_POINT('Ctrl Pts',(8.7858832621216,-63.0089393155471,-234.571897587772));
#216655=CARTESIAN_POINT('Ctrl Pts',(8.79681567493446,-63.0115709797409,
-234.57181396807));
#216656=CARTESIAN_POINT('Ctrl Pts',(8.80985252396294,-63.0142665213595,
-234.572494303784));
#216657=CARTESIAN_POINT('Ctrl Pts',(8.82210928715347,-63.0169068663223,
-234.572891922504));
#216658=CARTESIAN_POINT('Ctrl Pts',(8.85244345145974,-63.0234414347627,
-234.573875985863));
#216659=CARTESIAN_POINT('Ctrl Pts',(8.88278396117814,-63.0298509579082,
-234.574862091849));
#216660=CARTESIAN_POINT('Ctrl Pts',(8.91316422636502,-63.0361424884105,
-234.575851272007));
#216661=CARTESIAN_POINT('Ctrl Pts',(8.99242293231775,-63.0525563861501,
-234.578431932142));
#216662=CARTESIAN_POINT('Ctrl Pts',(9.0719524711103,-63.0681709773559,-234.581033503827));
#216663=CARTESIAN_POINT('Ctrl Pts',(9.15234381497248,-63.0830750262618,
-234.583674547358));
#216664=CARTESIAN_POINT('Ctrl Pts',(9.19361826977972,-63.0907270502666,
-234.585030509663));
#216665=CARTESIAN_POINT('Ctrl Pts',(9.23511984058779,-63.0981909396172,
-234.586396884075));
#216666=CARTESIAN_POINT('Ctrl Pts',(9.27692812757237,-63.1054733788026,
-234.587776220271));
#216667=CARTESIAN_POINT('Ctrl Pts',(9.35723190012809,-63.1194612118898,
-234.590425596942));
#216668=CARTESIAN_POINT('Ctrl Pts',(9.4386674796978,-63.1327830283328,-234.593122828895));
#216669=CARTESIAN_POINT('Ctrl Pts',(9.52179594456459,-63.1454466317045,
-234.595885927164));
#216670=CARTESIAN_POINT('Ctrl Pts',(9.60320028398561,-63.1578475856835,
-234.598591717408));
#216671=CARTESIAN_POINT('Ctrl Pts',(9.68622805619257,-63.1696173756771,
-234.60136068521));
#216672=CARTESIAN_POINT('Ctrl Pts',(9.77140172737696,-63.1807142389001,
-234.604209720771));
#216673=CARTESIAN_POINT('Ctrl Pts',(9.84650123949516,-63.1904985889522,
-234.606721778519));
#216674=CARTESIAN_POINT('Ctrl Pts',(9.92326901592422,-63.1997592047957,
-234.60929609172));
#216675=CARTESIAN_POINT('Ctrl Pts',(10.0020597851061,-63.2084339698903,
-234.611944069746));
#216676=CARTESIAN_POINT('Ctrl Pts',(10.0079176914778,-63.2090789180518,
-234.612140940617));
#216677=CARTESIAN_POINT('Ctrl Pts',(10.0137868348703,-63.2097206627102,
-234.61233823974));
#216678=CARTESIAN_POINT('Ctrl Pts',(10.0196673616597,-63.2103591682456,
-234.61253597217));
#216679=CARTESIAN_POINT('Ctrl Pts',(10.1775217355446,-63.2274989407736,
-234.617843817891));
#216680=CARTESIAN_POINT('Ctrl Pts',(10.3408423339544,-63.2420090474358,
-234.623376571456));
#216681=CARTESIAN_POINT('Ctrl Pts',(10.5096382176533,-63.2531987375938,
-234.629123175597));
#216682=CARTESIAN_POINT('Ctrl Pts',(10.5851067962263,-63.2582016440177,
-234.631692480231));
#216683=CARTESIAN_POINT('Ctrl Pts',(10.6616697717933,-63.2625401196258,
-234.634304495196));
#216684=CARTESIAN_POINT('Ctrl Pts',(10.7393274396082,-63.2661491027286,
-234.636958032241));
#216685=CARTESIAN_POINT('Ctrl Pts',(10.8650023153563,-63.2719895884886,
-234.641252301536));
#216686=CARTESIAN_POINT('Ctrl Pts',(10.9935433905513,-63.2759200262142,
-234.645655597734));
#216687=CARTESIAN_POINT('Ctrl Pts',(11.124943865751,-63.2776525377261,-234.650163351666));
#216688=CARTESIAN_POINT('Ctrl Pts',(11.1906441033508,-63.278518793482,-234.652417228633));
#216689=CARTESIAN_POINT('Ctrl Pts',(11.2570590826227,-63.2788353452046,
-234.654697219748));
#216690=CARTESIAN_POINT('Ctrl Pts',(11.3241872747982,-63.2785648884929,
-234.657002776486));
#216691=CARTESIAN_POINT('Ctrl Pts',(11.3577513708859,-63.278429660137,-234.658155554855));
#216692=CARTESIAN_POINT('Ctrl Pts',(11.3914937693878,-63.2781476704804,
-234.659314718289));
#216693=CARTESIAN_POINT('Ctrl Pts',(11.4254142273421,-63.2777141703294,
-234.660480209155));
#216694=CARTESIAN_POINT('Ctrl Pts',(11.4423744563193,-63.2774974202539,
-234.661062954589));
#216695=CARTESIAN_POINT('Ctrl Pts',(11.4593792001185,-63.2772427919946,
-234.661647281495));
#216696=CARTESIAN_POINT('Ctrl Pts',(11.4764284266816,-63.2769496876593,
-234.662233181745));
#216697=CARTESIAN_POINT('Ctrl Pts',(11.4849530399631,-63.2768031354916,
-234.662526131871));
#216698=CARTESIAN_POINT('Ctrl Pts',(11.4934887739323,-63.2766469642703,
-234.662819475307));
#216699=CARTESIAN_POINT('Ctrl Pts',(11.5020356243932,-63.2764810989383,
-234.663113211071));
#216700=CARTESIAN_POINT('Ctrl Pts',(11.510582474854,-63.2763152336063,-234.663406946834));
#216701=CARTESIAN_POINT('Ctrl Pts',(11.5206164958058,-63.2761077505405,
-234.663751807062));
#216702=CARTESIAN_POINT('Ctrl Pts',(11.5277095211746,-63.2759543445152,
-234.663995595652));
#216703=CARTESIAN_POINT('Ctrl Pts',(11.7959382858705,-63.2701531656785,
-234.673214667765));
#216704=CARTESIAN_POINT('Ctrl Pts',(12.0647257367003,-63.2549839288532,
-234.682485491612));
#216705=CARTESIAN_POINT('Ctrl Pts',(12.3338331099587,-63.2303282374309,
-234.691756583846));
#216706=CARTESIAN_POINT('Ctrl Pts',(12.5122102573677,-63.2139852742112,
-234.697901904081));
#216707=CARTESIAN_POINT('Ctrl Pts',(12.6907279881409,-63.1934753535059,
-234.704047292337));
#216708=CARTESIAN_POINT('Ctrl Pts',(12.8693171326838,-63.1687765962808,
-234.710177274085));
#216709=CARTESIAN_POINT('Ctrl Pts',(13.1051691938716,-63.1361584166303,
-234.718272776385));
#216710=CARTESIAN_POINT('Ctrl Pts',(13.3412824605714,-63.0961134334835,
-234.726378967533));
#216711=CARTESIAN_POINT('Ctrl Pts',(13.5774175745815,-63.0484087566338,
-234.734431297969));
#216712=CARTESIAN_POINT('Ctrl Pts',(13.6949932812573,-63.0246557831895,
-234.738440690835));
#216713=CARTESIAN_POINT('Ctrl Pts',(13.8125727957745,-62.9990048475027,
-234.742436205742));
#216714=CARTESIAN_POINT('Ctrl Pts',(13.9301247417777,-62.9714309612777,
-234.746409185644));
#216715=CARTESIAN_POINT('Ctrl Pts',(13.9887912132901,-62.9576697036745,
-234.748391974702));
#216716=CARTESIAN_POINT('Ctrl Pts',(14.0474508288688,-62.9434295279964,
-234.750369153456));
#216717=CARTESIAN_POINT('Ctrl Pts',(14.1060997648205,-62.9287075009776,
-234.75233966774));
#216718=CARTESIAN_POINT('Ctrl Pts',(14.1112871883718,-62.9274053564725,
-234.752513957214));
#216719=CARTESIAN_POINT('Ctrl Pts',(14.1164745284042,-62.9260994424293,
-234.752688194559));
#216720=CARTESIAN_POINT('Ctrl Pts',(14.1216617823046,-62.9247897568609,
-234.752862379056));
#216721=CARTESIAN_POINT('Ctrl Pts',(14.1456979383595,-62.9187210724837,
-234.753669497011));
#216722=CARTESIAN_POINT('Ctrl Pts',(14.1698178995471,-62.9125255294095,
-234.754509575307));
#216723=CARTESIAN_POINT('Ctrl Pts',(14.1939742871885,-62.9062259828314,
-234.755364712355));
#216724=CARTESIAN_POINT('Ctrl Pts',(14.216952479753,-62.9002336881023,-234.756178141251));
#216725=CARTESIAN_POINT('Ctrl Pts',(14.2409845451924,-62.8936465131962,
-234.757285208748));
#216726=CARTESIAN_POINT('Ctrl Pts',(14.2619189241969,-62.8884528813233,
-234.757545437753));
#216727=CARTESIAN_POINT('Ctrl Pts',(55.6596124147223,-63.9410622767582,
-216.790642532039));
#216728=CARTESIAN_POINT('Ctrl Pts',(56.7746082597229,-64.9675904302956,
-215.348143273993));
#216729=CARTESIAN_POINT('Ctrl Pts',(56.7978769236249,-64.9962486583172,
-213.25615446688));
#216730=CARTESIAN_POINT('Ctrl Pts',(56.5646546671649,-62.9482476744138,
-216.79031846553));
#216731=CARTESIAN_POINT('Ctrl Pts',(57.7003423851772,-63.9568776617924,
-215.347378844935));
#216732=CARTESIAN_POINT('Ctrl Pts',(57.7238224635575,-63.9855135774693,
-213.252837709798));
#216733=CARTESIAN_POINT('Ctrl Pts',(57.4569850684519,-61.9095456344264,
-216.789947870949));
#216734=CARTESIAN_POINT('Ctrl Pts',(58.611700878634,-62.9065844937097,-215.346095403267));
#216735=CARTESIAN_POINT('Ctrl Pts',(58.6299194066537,-62.9418272935278,
-213.246154460278));
#216736=CARTESIAN_POINT('Ctrl Pts',(58.3016167962822,-60.8701016111416,
-216.790073419041));
#216737=CARTESIAN_POINT('Ctrl Pts',(59.4805126951739,-61.8494200250926,
-215.345222444811));
#216738=CARTESIAN_POINT('Ctrl Pts',(59.5017489787801,-61.8814728748856,
-213.239284157696));
#216739=CARTESIAN_POINT('',(59.5017489787801,-61.8814728748856,-213.239284157696));
#216740=CARTESIAN_POINT('Ctrl Pts',(56.8144552684302,-64.9781463796361,
-213.256094898505));
#216741=CARTESIAN_POINT('Ctrl Pts',(56.9294188925119,-64.8525744128834,
-213.255680555424));
#216742=CARTESIAN_POINT('Ctrl Pts',(57.0524106752843,-64.7173956850926,
-213.255183250552));
#216743=CARTESIAN_POINT('Ctrl Pts',(57.1833118747465,-64.5723463396209,
-213.254587821642));
#216744=CARTESIAN_POINT('Ctrl Pts',(57.3081863588042,-64.4339750928097,
-213.254019806389));
#216745=CARTESIAN_POINT('Ctrl Pts',(57.4402589750224,-64.2866205890543,
-213.253362393774));
#216746=CARTESIAN_POINT('Ctrl Pts',(57.5793799148568,-64.1300563307852,
-213.252605702994));
#216747=CARTESIAN_POINT('Ctrl Pts',(57.7142502997413,-63.9782755722807,
-213.251872131349));
#216748=CARTESIAN_POINT('Ctrl Pts',(57.8557452334703,-63.8178386808859,
-213.251045156913));
#216749=CARTESIAN_POINT('Ctrl Pts',(58.0036788274559,-63.6485500668985,
-213.250120374855));
#216750=CARTESIAN_POINT('Ctrl Pts',(58.1403782530185,-63.4921173347321,
-213.249265821317));
#216751=CARTESIAN_POINT('Ctrl Pts',(58.2825754484112,-63.3281259468563,
-213.248327716734));
#216752=CARTESIAN_POINT('Ctrl Pts',(58.4300800100018,-63.1564365856218,
-213.247307421374));
#216753=CARTESIAN_POINT('Ctrl Pts',(58.5727477993223,-62.9903770322558,
-213.246320582175));
#216754=CARTESIAN_POINT('Ctrl Pts',(58.7203807787913,-62.817115737271,-213.245256795861));
#216755=CARTESIAN_POINT('Ctrl Pts',(58.8727631035814,-62.6365458514646,
-213.244122705959));
#216756=CARTESIAN_POINT('Ctrl Pts',(59.0185109355358,-62.4638377016922,
-213.243037992593));
#216757=CARTESIAN_POINT('Ctrl Pts',(59.1686036195926,-62.2844432836784,
-213.241888927712));
#216758=CARTESIAN_POINT('Ctrl Pts',(59.3228101732188,-62.0982909448199,
-213.240687014781));
#216759=CARTESIAN_POINT('Ctrl Pts',(59.381858614956,-62.0270098917333,-213.240226780867));
#216760=CARTESIAN_POINT('Ctrl Pts',(59.4415097985946,-61.9547382044033,
-213.239758862166));
#216761=CARTESIAN_POINT('Ctrl Pts',(59.5017489787801,-61.8814728748856,
-213.239284157696));
#216762=CARTESIAN_POINT('',(58.3016167962821,-60.8701016111416,-216.790073419041));
#216763=CARTESIAN_POINT('Origin',(1.94104476119577,-15.0690951428036,-217.435380395218));
#216764=CARTESIAN_POINT('Origin',(55.6399013441494,-58.7068046741696,-213.15202212551));
#216765=CARTESIAN_POINT('Ctrl Pts',(60.0946517248888,-61.0923008758321,
-213.257460793579));
#216766=CARTESIAN_POINT('Ctrl Pts',(59.9794428890559,-61.1951119486122,
-215.368374394716));
#216767=CARTESIAN_POINT('Ctrl Pts',(58.6463245735781,-60.4071924582901,
-216.811211134516));
#216768=CARTESIAN_POINT('Ctrl Pts',(59.9074639858676,-61.3655831923349,
-213.24427462457));
#216769=CARTESIAN_POINT('Ctrl Pts',(59.8200433378112,-61.4202510270675,
-215.35259069506));
#216770=CARTESIAN_POINT('Ctrl Pts',(58.537453097357,-60.5671124334832,-216.797054630904));
#216771=CARTESIAN_POINT('Ctrl Pts',(59.7097127443643,-61.6285208837114,
-213.238301674021));
#216772=CARTESIAN_POINT('Ctrl Pts',(59.653667582921,-61.6382804704428,-215.344967772288));
#216773=CARTESIAN_POINT('Ctrl Pts',(58.4224878547945,-60.7213519315114,
-216.790091385297));
#216774=CARTESIAN_POINT('Ctrl Pts',(59.5017489787801,-61.8814728748855,
-213.239284157696));
#216775=CARTESIAN_POINT('Ctrl Pts',(59.4805126951738,-61.8494200250926,
-215.345222444811));
#216776=CARTESIAN_POINT('Ctrl Pts',(58.3016167962821,-60.8701016111416,
-216.790073419041));
#216777=CARTESIAN_POINT('',(58.6463245735781,-60.4071924582901,-216.811211134516));
#216778=CARTESIAN_POINT('',(60.094651724889,-61.0923008758319,-213.257460793579));
#216779=CARTESIAN_POINT('Origin',(55.9721510687884,-58.2643380616866,-213.170198761392));
#216780=CARTESIAN_POINT('Origin',(52.480669683245,-56.0916407951787,-217.694018753789));
#216781=CARTESIAN_POINT('Origin',(54.9927878736021,-61.8053486253609,-218.50906240554));
#216782=CARTESIAN_POINT('Ctrl Pts',(58.6074055114448,-60.4543100647495,
-216.811910699149));
#216783=CARTESIAN_POINT('Ctrl Pts',(59.9363259578221,-61.2556965846773,
-215.36842105937));
#216784=CARTESIAN_POINT('Ctrl Pts',(60.0500816328534,-61.1568904110335,
-213.254375849603));
#216785=CARTESIAN_POINT('Ctrl Pts',(58.6843926594325,-60.3569715803453,
-216.813280762464));
#216786=CARTESIAN_POINT('Ctrl Pts',(60.0245567355929,-61.1325327891189,
-215.370731335637));
#216787=CARTESIAN_POINT('Ctrl Pts',(60.1415615520333,-61.0252958819011,
-213.260597914992));
#216788=CARTESIAN_POINT('Ctrl Pts',(58.7617161401563,-60.257380322437,-216.813794119462));
#216789=CARTESIAN_POINT('Ctrl Pts',(60.1108245046652,-61.0067372913192,
-215.372344710318));
#216790=CARTESIAN_POINT('Ctrl Pts',(60.2301284165771,-60.8919475940444,
-213.267282154519));
#216791=CARTESIAN_POINT('Ctrl Pts',(58.8637629875194,-60.118929962275,-216.816300847937));
#216792=CARTESIAN_POINT('Ctrl Pts',(60.2274193821809,-60.8294290656787,
-215.376497710853));
#216793=CARTESIAN_POINT('Ctrl Pts',(60.351618647282,-60.7003634878413,-213.277642216535));
#216794=CARTESIAN_POINT('Ctrl Pts',(58.8929787543517,-60.0784113786681,
-216.817245287021));
#216795=CARTESIAN_POINT('Ctrl Pts',(60.2611173232929,-60.7772510392266,
-215.377939075409));
#216796=CARTESIAN_POINT('Ctrl Pts',(60.3869441313173,-60.6435508076928,
-213.280811345684));
#216797=CARTESIAN_POINT('Ctrl Pts',(58.9495124986678,-59.9981405703258,
-216.819674866848));
#216798=CARTESIAN_POINT('Ctrl Pts',(60.3271235407812,-60.6732372865155,
-215.381384415719));
#216799=CARTESIAN_POINT('Ctrl Pts',(60.4565718022466,-60.5293282073925,
-213.287428511102));
#216800=CARTESIAN_POINT('Ctrl Pts',(58.9761430287399,-59.9590023263254,
-216.821371021085));
#216801=CARTESIAN_POINT('Ctrl Pts',(60.359173711659,-60.6218554219661,-215.383594060466));
#216802=CARTESIAN_POINT('Ctrl Pts',(60.4908728037641,-60.4719198229408,
-213.290891213227));
#216803=CARTESIAN_POINT('Ctrl Pts',(59.0642485460056,-59.8329939373022,
-216.824171668603));
#216804=CARTESIAN_POINT('Ctrl Pts',(60.4575238287991,-60.4610669137915,
-215.388063886973));
#216805=CARTESIAN_POINT('Ctrl Pts',(60.5922460955355,-60.2987937845113,
-213.30164664474));
#216806=CARTESIAN_POINT('Ctrl Pts',(59.1308552045038,-59.7401265656055,
-216.823603457484));
#216807=CARTESIAN_POINT('Ctrl Pts',(60.5247139239745,-60.3469167156672,
-215.388758628301));
#216808=CARTESIAN_POINT('Ctrl Pts',(60.6577989462605,-60.182163619438,-213.309190814847));
#216809=CARTESIAN_POINT('Ctrl Pts',(59.2607825507709,-59.5528560555646,
-216.821806470031));
#216810=CARTESIAN_POINT('Ctrl Pts',(60.6547502248839,-60.1166039110421,
-215.389715911556));
#216811=CARTESIAN_POINT('Ctrl Pts',(60.7848819389693,-59.9464002293942,
-213.324386876106));
#216812=CARTESIAN_POINT('Ctrl Pts',(59.3235037477498,-59.4590534661329,
-216.82085617928));
#216813=CARTESIAN_POINT('Ctrl Pts',(60.7174143058776,-60.0009016819405,
-215.390241225136));
#216814=CARTESIAN_POINT('Ctrl Pts',(60.846408364718,-59.8272707789861,-213.332077521816));
#216815=CARTESIAN_POINT('Ctrl Pts',(59.497535989523,-59.1844462404644,-216.821411068371));
#216816=CARTESIAN_POINT('Ctrl Pts',(60.8959799414287,-59.6576852666735,
-215.395296546354));
#216817=CARTESIAN_POINT('Ctrl Pts',(61.0248485990128,-59.4661777527895,
-213.356063148757));
#216818=CARTESIAN_POINT('Ctrl Pts',(59.6013476331263,-59.0045621852585,
-216.824786693514));
#216819=CARTESIAN_POINT('Ctrl Pts',(61.0052029790378,-59.4294490925104,
-215.401835242901));
#216820=CARTESIAN_POINT('Ctrl Pts',(61.1355702178776,-59.2205125002805,
-213.373562975867));
#216821=CARTESIAN_POINT('Ctrl Pts',(59.7620679015636,-58.7165983993849,
-216.825507837644));
#216822=CARTESIAN_POINT('Ctrl Pts',(61.160929555377,-59.0728872758639,-215.408140407826));
#216823=CARTESIAN_POINT('Ctrl Pts',(61.2879458897801,-58.8475849978508,
-213.401799673797));
#216824=CARTESIAN_POINT('Ctrl Pts',(59.8184700980811,-58.6152752114856,
-216.824157923918));
#216825=CARTESIAN_POINT('Ctrl Pts',(61.2120467193731,-58.9500553531654,
-215.408866560461));
#216826=CARTESIAN_POINT('Ctrl Pts',(61.3365745411598,-58.7222537891958,
-213.411505588844));
#216827=CARTESIAN_POINT('Ctrl Pts',(59.9269424397347,-58.4123215093298,
-216.821223970727));
#216828=CARTESIAN_POINT('Ctrl Pts',(61.3093200563378,-58.7041349241579,
-215.410324805557));
#216829=CARTESIAN_POINT('Ctrl Pts',(61.429120358173,-58.4706258869242,-213.431043252633));
#216830=CARTESIAN_POINT('Ctrl Pts',(59.9776849531454,-58.3122310671642,
-216.820297737876));
#216831=CARTESIAN_POINT('Ctrl Pts',(61.3551328190027,-58.5821325532565,
-215.411652153446));
#216832=CARTESIAN_POINT('Ctrl Pts',(61.4730253186173,-58.3443774821519,
-213.440939227853));
#216833=CARTESIAN_POINT('Ctrl Pts',(60.1230288656398,-58.0127552603068,
-216.818391671956));
#216834=CARTESIAN_POINT('Ctrl Pts',(61.4853151645514,-58.2168872743818,
-215.416733820586));
#216835=CARTESIAN_POINT('Ctrl Pts',(61.5977142939005,-57.9644548465746,
-213.471381381577));
#216836=CARTESIAN_POINT('Ctrl Pts',(60.2105402005316,-57.8145726066615,
-216.818537217051));
#216837=CARTESIAN_POINT('Ctrl Pts',(61.5626251138468,-57.9742502615569,
-215.421806822622));
#216838=CARTESIAN_POINT('Ctrl Pts',(61.6714754954738,-57.7096224301994,
-213.49274435759));
#216839=CARTESIAN_POINT('Ctrl Pts',(60.3806025831265,-57.4045491967827,
-216.81529811369));
#216840=CARTESIAN_POINT('Ctrl Pts',(61.7018225456774,-57.4799411928046,
-215.429818040078));
#216841=CARTESIAN_POINT('Ctrl Pts',(61.8007144046227,-57.1969944641333,
-213.537796166961));
#216842=CARTESIAN_POINT('Ctrl Pts',(60.4634339941568,-57.1919229894312,
-216.811338644603));
#216843=CARTESIAN_POINT('Ctrl Pts',(61.7636221410114,-57.2279080669269,
-215.432277259244));
#216844=CARTESIAN_POINT('Ctrl Pts',(61.8562081200067,-56.9391516851297,
-213.561315895501));
#216845=CARTESIAN_POINT('Ctrl Pts',(60.6152405963767,-56.762184327613,-216.802302824218));
#216846=CARTESIAN_POINT('Ctrl Pts',(61.8694772718262,-56.7213693952703,
-215.43746654745));
#216847=CARTESIAN_POINT('Ctrl Pts',(61.9491342563802,-56.4203496749288,
-213.610036002497));
#216848=CARTESIAN_POINT('Ctrl Pts',(60.6824463640865,-56.5477747378356,
-216.798434344268));
#216849=CARTESIAN_POINT('Ctrl Pts',(61.9133532267272,-56.4685867807556,
-215.441201542271));
#216850=CARTESIAN_POINT('Ctrl Pts',(61.9865582056432,-56.1594017179448,
-213.635279158434));
#216851=CARTESIAN_POINT('Ctrl Pts',(60.8073533359841,-56.0969490021232,
-216.792401635896));
#216852=CARTESIAN_POINT('Ctrl Pts',(61.9872021354889,-55.9382448925313,
-215.452237086731));
#216853=CARTESIAN_POINT('Ctrl Pts',(62.0459484757164,-55.6091885457502,
-213.691499099128));
#216854=CARTESIAN_POINT('Ctrl Pts',(60.8666693908396,-55.8585138307279,
-216.788165726564));
#216855=CARTESIAN_POINT('Ctrl Pts',(62.0158520694785,-55.6592576800417,
-215.457808501477));
#216856=CARTESIAN_POINT('Ctrl Pts',(62.0660566009803,-55.3196727763676,
-213.722940188816));
#216857=CARTESIAN_POINT('Ctrl Pts',(60.9269250208923,-55.5935705192412,
-216.775920823856));
#216858=CARTESIAN_POINT('Ctrl Pts',(62.0343090115749,-55.3647134586715,
-215.458374400723));
#216859=CARTESIAN_POINT('Ctrl Pts',(62.0750191951853,-55.0282471371092,
-213.755373099554));
#216860=CARTESIAN_POINT('',(60.9119170756758,-55.6633990141858,-216.777770284882));
#216861=CARTESIAN_POINT('',(62.0723653519316,-55.1059089910534,-213.746749287634));
#216862=CARTESIAN_POINT('Origin',(57.0770276271036,-54.9084593705222,-213.659487255448));
#216863=CARTESIAN_POINT('Ctrl Pts',(60.0946517248888,-61.0923008758318,
-213.257460793579));
#216864=CARTESIAN_POINT('Ctrl Pts',(60.1688733048961,-60.9839420408379,
-213.262689226369));
#216865=CARTESIAN_POINT('Ctrl Pts',(60.2426760592975,-60.8721561614362,
-213.268476733384));
#216866=CARTESIAN_POINT('Ctrl Pts',(60.3157714398376,-60.7568862808627,
-213.274784382698));
#216867=CARTESIAN_POINT('Ctrl Pts',(60.3512737868304,-60.7008998249785,
-213.277848001124));
#216868=CARTESIAN_POINT('Ctrl Pts',(60.3866089369293,-60.6440917231958,
-213.281039224211));
#216869=CARTESIAN_POINT('Ctrl Pts',(60.4217426652322,-60.5864561384688,
-213.284371063984));
#216870=CARTESIAN_POINT('Ctrl Pts',(60.4435624323821,-60.5506616156829,
-213.286440299775));
#216871=CARTESIAN_POINT('Ctrl Pts',(60.4653040350053,-60.514548553946,-213.288569677611));
#216872=CARTESIAN_POINT('Ctrl Pts',(60.4869604790493,-60.4781138482913,
-213.290748336221));
#216873=CARTESIAN_POINT('Ctrl Pts',(60.4995551781952,-60.4569245821652,
-213.292015374783));
#216874=CARTESIAN_POINT('Ctrl Pts',(60.5121204198581,-60.4356273698192,
-213.293306640679));
#216875=CARTESIAN_POINT('Ctrl Pts',(60.5246547397792,-60.4142217745433,
-213.294620659626));
#216876=CARTESIAN_POINT('Ctrl Pts',(60.591150130146,-60.3006636858019,-213.301591616443));
#216877=CARTESIAN_POINT('Ctrl Pts',(60.6567843084902,-60.1840449613726,
-213.309095887413));
#216878=CARTESIAN_POINT('Ctrl Pts',(60.7213395261845,-60.0642830904757,
-213.316803279816));
#216879=CARTESIAN_POINT('Ctrl Pts',(60.7685965359593,-59.9766125952661,
-213.322445400331));
#216880=CARTESIAN_POINT('Ctrl Pts',(60.8152737419114,-59.8872593538088,
-213.328214013836));
#216881=CARTESIAN_POINT('Ctrl Pts',(60.8612668418636,-59.7962116928738,
-213.334193694335));
#216882=CARTESIAN_POINT('Ctrl Pts',(60.8762151842007,-59.7666200452991,
-213.336137166535));
#216883=CARTESIAN_POINT('Ctrl Pts',(60.8910888831917,-59.7368539552651,
-213.338107798564));
#216884=CARTESIAN_POINT('Ctrl Pts',(60.9058862461468,-59.7069094955419,
-213.340107694982));
#216885=CARTESIAN_POINT('Ctrl Pts',(60.9637435733099,-59.5898273905627,
-213.347927241053));
#216886=CARTESIAN_POINT('Ctrl Pts',(61.0204246813107,-59.4700172291252,
-213.356262962161));
#216887=CARTESIAN_POINT('Ctrl Pts',(61.0757281447404,-59.3474693357667,
-213.365036420254));
#216888=CARTESIAN_POINT('Ctrl Pts',(61.1204542243354,-59.2483600487051,
-213.372131859865));
#216889=CARTESIAN_POINT('Ctrl Pts',(61.1642786072501,-59.1474602983931,
-213.37951365019));
#216890=CARTESIAN_POINT('Ctrl Pts',(61.2070729743782,-59.0447771657053,
-213.387142007677));
#216891=CARTESIAN_POINT('Ctrl Pts',(61.2171558757692,-59.0205837035538,
-213.388939346473));
#216892=CARTESIAN_POINT('Ctrl Pts',(61.2271793702854,-58.996296378915,-213.390750959789));
#216893=CARTESIAN_POINT('Ctrl Pts',(61.2371418312946,-58.9719150325815,
-213.392578681107));
#216894=CARTESIAN_POINT('Ctrl Pts',(61.2783750144538,-58.8710041714885,
-213.400143354916));
#216895=CARTESIAN_POINT('Ctrl Pts',(61.3186449470215,-58.7682927383909,
-213.407960918625));
#216896=CARTESIAN_POINT('Ctrl Pts',(61.3577808239653,-58.6639330018756,
-213.416038726705));
#216897=CARTESIAN_POINT('Ctrl Pts',(61.3604129670204,-58.6569141287302,
-213.416582012));
#216898=CARTESIAN_POINT('Ctrl Pts',(61.3630399688414,-58.649887813559,-213.417126466415));
#216899=CARTESIAN_POINT('Ctrl Pts',(61.3656617724452,-58.642854108928,-213.417672088598));
#216900=CARTESIAN_POINT('Ctrl Pts',(61.3714146872104,-58.6274203429637,
-213.418869324694));
#216901=CARTESIAN_POINT('Ctrl Pts',(61.3771434762636,-58.6119486844701,
-213.420070235415));
#216902=CARTESIAN_POINT('Ctrl Pts',(61.3828474496664,-58.59643983806,-213.421274420738));
#216903=CARTESIAN_POINT('Ctrl Pts',(61.4066350315578,-58.5317624758125,
-213.426296298467));
#216904=CARTESIAN_POINT('Ctrl Pts',(61.4299886141107,-58.4664490159562,
-213.431392104351));
#216905=CARTESIAN_POINT('Ctrl Pts',(61.4528841092791,-58.4004915334073,
-213.436581849268));
#216906=CARTESIAN_POINT('Ctrl Pts',(61.4671034320988,-58.3595284212386,
-213.439804957473));
#216907=CARTESIAN_POINT('Ctrl Pts',(61.48114539916,-58.318318751907,-213.443064189012));
#216908=CARTESIAN_POINT('Ctrl Pts',(61.4950031156842,-58.2768639431237,
-213.446364418246));
#216909=CARTESIAN_POINT('Ctrl Pts',(61.4998241791749,-58.2624419231042,
-213.447512559402));
#216910=CARTESIAN_POINT('Ctrl Pts',(61.5050437465624,-58.2467173872201,
-213.448767386496));
#216911=CARTESIAN_POINT('Ctrl Pts',(61.5096349176404,-58.2327939136108,
-213.449881149215));
#216912=CARTESIAN_POINT('Ctrl Pts',(61.5106925269236,-58.2295865413098,
-213.450137712469));
#216913=CARTESIAN_POINT('Ctrl Pts',(61.5117170122721,-58.2264747787118,
-213.450386767174));
#216914=CARTESIAN_POINT('Ctrl Pts',(61.5126961916284,-58.2234966253952,
-213.450625245251));
#216915=CARTESIAN_POINT('Ctrl Pts',(61.5133274243917,-58.221576744287,-213.450778981311));
#216916=CARTESIAN_POINT('Ctrl Pts',(61.5139581302282,-58.2196567378002,
-213.450932777525));
#216917=CARTESIAN_POINT('Ctrl Pts',(61.5145883090845,-58.2177366063309,
-213.451086634312));
#216918=CARTESIAN_POINT('Ctrl Pts',(61.5754675922918,-58.0322397011969,
-213.465950177932));
#216919=CARTESIAN_POINT('Ctrl Pts',(61.6314260330506,-57.8455859554956,
-213.481413045566));
#216920=CARTESIAN_POINT('Ctrl Pts',(61.6824475740234,-57.6580324650191,
-213.49749706447));
#216921=CARTESIAN_POINT('Ctrl Pts',(61.7009806262513,-57.5899055804081,
-213.503339419615));
#216922=CARTESIAN_POINT('Ctrl Pts',(61.7188627796439,-57.5216600629364,
-213.509263678944));
#216923=CARTESIAN_POINT('Ctrl Pts',(61.736094926277,-57.4533085098064,-213.51527069985));
#216924=CARTESIAN_POINT('Ctrl Pts',(61.7840826055166,-57.2629647019827,
-213.531998911289));
#216925=CARTESIAN_POINT('Ctrl Pts',(61.8270345946187,-57.0717719007629,
-213.549276027728));
#216926=CARTESIAN_POINT('Ctrl Pts',(61.8649529491542,-56.8799677222285,
-213.567015134291));
#216927=CARTESIAN_POINT('Ctrl Pts',(61.8781328721527,-56.8132991039609,
-213.573181015206));
#216928=CARTESIAN_POINT('Ctrl Pts',(61.8907051028513,-56.7465566994706,
-213.579402669573));
#216929=CARTESIAN_POINT('Ctrl Pts',(61.9026711707414,-56.6797507397666,
-213.585676324044));
#216930=CARTESIAN_POINT('Ctrl Pts',(61.9367372826433,-56.4895613375432,
-213.60353674546));
#216931=CARTESIAN_POINT('Ctrl Pts',(61.9658823716952,-56.2988624688379,
-213.621842648317));
#216932=CARTESIAN_POINT('Ctrl Pts',(61.9901097322645,-56.1079785002405,
-213.640827105813));
#216933=CARTESIAN_POINT('Ctrl Pts',(61.9990293863389,-56.0377017995089,
-213.647816509102));
#216934=CARTESIAN_POINT('Ctrl Pts',(62.0072829516351,-55.9674000675249,
-213.654897754168));
#216935=CARTESIAN_POINT('Ctrl Pts',(62.0148722891561,-55.8970896752966,
-213.662081941508));
#216936=CARTESIAN_POINT('Ctrl Pts',(62.0354032478553,-55.7068833819308,
-213.68151687284));
#216937=CARTESIAN_POINT('Ctrl Pts',(62.0510721347403,-55.5166252894532,
-213.701767805664));
#216938=CARTESIAN_POINT('Ctrl Pts',(62.0619255431476,-55.3264908015158,
-213.722497227011));
#216939=CARTESIAN_POINT('Ctrl Pts',(62.0661239505739,-55.2529413674403,
-213.730515957465));
#216940=CARTESIAN_POINT('Ctrl Pts',(62.0696023181198,-55.1794105511713,
-213.738606363368));
#216941=CARTESIAN_POINT('Ctrl Pts',(62.0723653519315,-55.1059089910535,
-213.746749287634));
#216942=CARTESIAN_POINT('Ctrl Pts',(60.9119170756758,-55.6633990141858,
-216.777770284882));
#216943=CARTESIAN_POINT('Ctrl Pts',(60.9073907830727,-55.6830113627593,
-216.778588585298));
#216944=CARTESIAN_POINT('Ctrl Pts',(60.9027344732998,-55.7030660698564,
-216.779382142226));
#216945=CARTESIAN_POINT('Ctrl Pts',(60.8979388924468,-55.7235631928626,
-216.780150955665));
#216946=CARTESIAN_POINT('Ctrl Pts',(60.8855667250161,-55.7764439273244,
-216.782134425215));
#216947=CARTESIAN_POINT('Ctrl Pts',(60.8722672911103,-55.8322729157864,
-216.783953203688));
#216948=CARTESIAN_POINT('Ctrl Pts',(60.8579173895963,-55.8910134972092,
-216.785607291083));
#216949=CARTESIAN_POINT('Ctrl Pts',(60.8525552968731,-55.9129629470987,
-216.786225369888));
#216950=CARTESIAN_POINT('Ctrl Pts',(60.8470465325387,-55.9353184362973,
-216.786820453299));
#216951=CARTESIAN_POINT('Ctrl Pts',(60.8413847105074,-55.9580761274448,
-216.787392541314));
#216952=CARTESIAN_POINT('Ctrl Pts',(60.8280412423979,-56.0117101916013,
-216.788740806617));
#216953=CARTESIAN_POINT('Ctrl Pts',(60.8138474727369,-56.0675809540217,
-216.789961349869));
#216954=CARTESIAN_POINT('Ctrl Pts',(60.7987212695568,-56.1256111309988,
-216.791054171069));
#216955=CARTESIAN_POINT('Ctrl Pts',(60.7911581679667,-56.1546262194874,
-216.791600581669));
#216956=CARTESIAN_POINT('Ctrl Pts',(60.7833619960081,-56.1841805428932,
-216.792115061728));
#216957=CARTESIAN_POINT('Ctrl Pts',(60.7753227949662,-56.2142603888131,
-216.792597612924));
#216958=CARTESIAN_POINT('Ctrl Pts',(60.7713031944453,-56.2293003117731,
-216.792838888522));
#216959=CARTESIAN_POINT('Ctrl Pts',(60.7672228324461,-56.2444716142868,
-216.793072178277));
#216960=CARTESIAN_POINT('Ctrl Pts',(60.7630805012708,-56.2597722389012,
-216.793297487807));
#216961=CARTESIAN_POINT('Ctrl Pts',(60.7595341573754,-56.2728714514941,
-216.793490380419));
#216962=CARTESIAN_POINT('Ctrl Pts',(60.7555793881087,-56.2873946780629,
-216.793695306117));
#216963=CARTESIAN_POINT('Ctrl Pts',(60.7521474474415,-56.2999266198356,
-216.793866332403));
#216964=CARTESIAN_POINT('Ctrl Pts',(60.7515706864043,-56.3020326981266,
-216.793895074536));
#216965=CARTESIAN_POINT('Ctrl Pts',(60.7510088127115,-56.3040825498413,
-216.793922859246));
#216966=CARTESIAN_POINT('Ctrl Pts',(60.7504663829785,-56.3060599824529,
-216.793949468515));
#216967=CARTESIAN_POINT('Ctrl Pts',(60.726744928692,-56.3925367635904,-216.795113141008));
#216968=CARTESIAN_POINT('Ctrl Pts',(60.7021402838857,-56.4777392222418,
-216.796372991844));
#216969=CARTESIAN_POINT('Ctrl Pts',(60.6768135902453,-56.5613350649519,
-216.797729021024));
#216970=CARTESIAN_POINT('Ctrl Pts',(60.6619983636042,-56.610235698157,-216.798522250488));
#216971=CARTESIAN_POINT('Ctrl Pts',(60.6469357952424,-56.6585875450376,
-216.799348390635));
#216972=CARTESIAN_POINT('Ctrl Pts',(60.6316559403284,-56.7063320203518,
-216.800207441465));
#216973=CARTESIAN_POINT('Ctrl Pts',(60.6232394165903,-56.7326308636398,
-216.800680628007));
#216974=CARTESIAN_POINT('Ctrl Pts',(60.6147569210123,-56.7587455902481,
-216.801163799913));
#216975=CARTESIAN_POINT('Ctrl Pts',(60.6062090667045,-56.7846826419487,
-216.801656957185));
#216976=CARTESIAN_POINT('Ctrl Pts',(60.5977766165011,-56.8102695189606,
-216.802143456368));
#216977=CARTESIAN_POINT('Ctrl Pts',(60.5892805607033,-56.8356834853934,
-216.802639673109));
#216978=CARTESIAN_POINT('Ctrl Pts',(60.5807215482445,-56.8609304861147,
-216.803145607486));
#216979=CARTESIAN_POINT('Ctrl Pts',(60.5764420420152,-56.8735539864754,
-216.803398574674));
#216980=CARTESIAN_POINT('Ctrl Pts',(60.5721467964869,-56.8861357453652,
-216.803653971149));
#216981=CARTESIAN_POINT('Ctrl Pts',(60.5678358994622,-56.8986764798207,
-216.803911797061));
#216982=CARTESIAN_POINT('Ctrl Pts',(60.5656804509498,-56.9049468470485,
-216.804040710018));
#216983=CARTESIAN_POINT('Ctrl Pts',(60.5635210895554,-56.9112069581651,
-216.804170230326));
#216984=CARTESIAN_POINT('Ctrl Pts',(60.5613578264237,-56.9174569020256,
-216.804300357988));
#216985=CARTESIAN_POINT('Ctrl Pts',(60.5591945632921,-56.923706845886,-216.80443048565));
#216986=CARTESIAN_POINT('Ctrl Pts',(60.5576872782576,-56.9280531415995,
-216.8045212999));
#216987=CARTESIAN_POINT('Ctrl Pts',(60.5548563430524,-56.9361763202472,
-216.804692563016));
#216988=CARTESIAN_POINT('Ctrl Pts',(60.531775183356,-57.002406159512,-216.806088904177));
#216989=CARTESIAN_POINT('Ctrl Pts',(60.5092923413343,-57.0649063224503,
-216.80735534074));
#216990=CARTESIAN_POINT('Ctrl Pts',(60.4875747703621,-57.1238418980249,
-216.808491872706));
#216991=CARTESIAN_POINT('Ctrl Pts',(60.4666733138366,-57.1805627611569,
-216.809585695468));
#216992=CARTESIAN_POINT('Ctrl Pts',(60.4464808877171,-57.2339808981995,
-216.810559193437));
#216993=CARTESIAN_POINT('Ctrl Pts',(60.4271400166051,-57.2841984344429,
-216.811412366612));
#216994=CARTESIAN_POINT('Ctrl Pts',(60.4074215554359,-57.3353963630518,
-216.812282196209));
#216995=CARTESIAN_POINT('Ctrl Pts',(60.3885884660559,-57.3832669787684,
-216.813026956971));
#216996=CARTESIAN_POINT('Ctrl Pts',(60.3707817467398,-57.4278816294471,
-216.813646648899));
#216997=CARTESIAN_POINT('Ctrl Pts',(60.3618783870818,-57.4501889547864,
-216.813956494863));
#216998=CARTESIAN_POINT('Ctrl Pts',(60.353231441283,-57.4716817687946,-216.814235073607));
#216999=CARTESIAN_POINT('Ctrl Pts',(60.344857338237,-57.4923662297235,-216.814482391391));
#217000=CARTESIAN_POINT('Ctrl Pts',(60.340670286714,-57.502708460188,-216.814606050283));
#217001=CARTESIAN_POINT('Ctrl Pts',(60.3365514347898,-57.5128485980101,
-216.814721883031));
#217002=CARTESIAN_POINT('Ctrl Pts',(60.3325027491553,-57.5227872445278,
-216.814829903421));
#217003=CARTESIAN_POINT('Ctrl Pts',(60.330478406338,-57.5277565677866,-216.814883913616));
#217004=CARTESIAN_POINT('Ctrl Pts',(60.3284716044061,-57.5326755179509,
-216.814935970048));
#217005=CARTESIAN_POINT('Ctrl Pts',(60.3264825839235,-57.5375441656945,
-216.814986072732));
#217006=CARTESIAN_POINT('Ctrl Pts',(60.3244935634409,-57.5424128134381,
-216.815036175415));
#217007=CARTESIAN_POINT('Ctrl Pts',(60.3231512484711,-57.5456958600444,
-216.815069449648));
#217008=CARTESIAN_POINT('Ctrl Pts',(60.3205691041673,-57.5519992691854,
-216.815130518181));
#217009=CARTESIAN_POINT('Ctrl Pts',(60.3057977046936,-57.5880585143369,
-216.815479866468));
#217010=CARTESIAN_POINT('Ctrl Pts',(60.2908264545178,-57.6241214719244,
-216.815797788964));
#217011=CARTESIAN_POINT('Ctrl Pts',(60.2756504796204,-57.6602025647167,
-216.816084285669));
#217012=CARTESIAN_POINT('Ctrl Pts',(60.2483805836785,-57.7250371241154,
-216.816599095121));
#217013=CARTESIAN_POINT('Ctrl Pts',(60.2204496607956,-57.7899302381468,
-216.81701243403));
#217014=CARTESIAN_POINT('Ctrl Pts',(60.1919174451317,-57.854738387928,-216.817324302395));
#217015=CARTESIAN_POINT('Ctrl Pts',(60.1697121029587,-57.9051756606042,
-216.817567015538));
#217016=CARTESIAN_POINT('Ctrl Pts',(60.1471425664518,-57.9555614731162,
-216.817748269903));
#217017=CARTESIAN_POINT('Ctrl Pts',(60.124236944089,-58.0058281702384,-216.817868065669));
#217018=CARTESIAN_POINT('Ctrl Pts',(60.1127841329077,-58.0309615187996,
-216.817927963552));
#217019=CARTESIAN_POINT('Ctrl Pts',(60.1012472999562,-58.0560650883737,
-216.817972496468));
#217020=CARTESIAN_POINT('Ctrl Pts',(60.0896299548045,-58.0811304205851,
-216.818001664822));
#217021=CARTESIAN_POINT('Ctrl Pts',(60.0794647777968,-58.1030625862702,
-216.818027187132));
#217022=CARTESIAN_POINT('Ctrl Pts',(60.0692379586165,-58.1249654764669,
-216.81804094593));
#217023=CARTESIAN_POINT('Ctrl Pts',(60.0589518474159,-58.146833423864,-216.818042941059));
#217024=CARTESIAN_POINT('Ctrl Pts',(60.0574824029587,-58.1499574163493,
-216.818043226077));
#217025=CARTESIAN_POINT('Ctrl Pts',(60.0554334228072,-58.1543076149849,
-216.818043194359));
#217026=CARTESIAN_POINT('Ctrl Pts',(60.0545398907524,-58.156203245427,-216.818043075904));
#217027=CARTESIAN_POINT('Ctrl Pts',(60.0450523572134,-58.1763310710596,
-216.818041818146));
#217028=CARTESIAN_POINT('Ctrl Pts',(60.0333692392358,-58.2007570838859,
-216.818133804124));
#217029=CARTESIAN_POINT('Ctrl Pts',(60.019406065471,-58.2294040937821,-216.818319033837));
#217030=CARTESIAN_POINT('Ctrl Pts',(60.0123285027026,-58.2439245039755,
-216.81841292187));
#217031=CARTESIAN_POINT('Ctrl Pts',(60.0046647473224,-58.2595287307156,
-216.818530766153));
#217032=CARTESIAN_POINT('Ctrl Pts',(59.9964016741368,-58.2762019403733,
-216.818672566686));
#217033=CARTESIAN_POINT('Ctrl Pts',(59.9841191164583,-58.3009856563962,
-216.818883344587));
#217034=CARTESIAN_POINT('Ctrl Pts',(59.9705125067986,-58.32813243013,-216.819147053873));
#217035=CARTESIAN_POINT('Ctrl Pts',(59.955534532171,-58.35757651355,-216.819463694545));
#217036=CARTESIAN_POINT('Ctrl Pts',(59.9480455448571,-58.37229855526,-216.819622014881));
#217037=CARTESIAN_POINT('Ctrl Pts',(59.9402136478829,-58.3875945819531,
-216.819793568053));
#217038=CARTESIAN_POINT('Ctrl Pts',(59.9320326268601,-58.4034540498328,
-216.819978358033));
#217039=CARTESIAN_POINT('Ctrl Pts',(59.9279421163487,-58.4113837837727,
-216.820070753024));
#217040=CARTESIAN_POINT('Ctrl Pts',(59.9237643184495,-58.4194543747942,
-216.82016645031));
#217041=CARTESIAN_POINT('Ctrl Pts',(59.9194984513664,-58.4276643114252,
-216.820265458625));
#217042=CARTESIAN_POINT('Ctrl Pts',(59.9173655178249,-58.4317692797407,
-216.820314962783));
#217043=CARTESIAN_POINT('Ctrl Pts',(59.9152105665835,-58.4359090842562,
-216.820365294261));
#217044=CARTESIAN_POINT('Ctrl Pts',(59.9130334990711,-58.4400835282948,
-216.820416453085));
#217045=CARTESIAN_POINT('Ctrl Pts',(59.9108564315587,-58.4442579723333,
-216.82046761191));
#217046=CARTESIAN_POINT('Ctrl Pts',(59.9093877396424,-58.447071603812,-216.820502230613));
#217047=CARTESIAN_POINT('Ctrl Pts',(59.9064358482483,-58.4527105781537,
-216.820572410718));
#217048=CARTESIAN_POINT('Ctrl Pts',(59.8836567049482,-58.4962253920307,
-216.821113976256));
#217049=CARTESIAN_POINT('Ctrl Pts',(59.863123350219,-58.5347073198221,-216.821591266887));
#217050=CARTESIAN_POINT('Ctrl Pts',(59.8449810090749,-58.5683168623629,
-216.82200428261));
#217051=CARTESIAN_POINT('Ctrl Pts',(59.8406893207328,-58.5762674174075,
-216.822101984155));
#217052=CARTESIAN_POINT('Ctrl Pts',(59.8365311992246,-58.5839453291258,
-216.822196088943));
#217053=CARTESIAN_POINT('Ctrl Pts',(59.8325081565776,-58.5913526920526,
-216.822286596973));
#217054=CARTESIAN_POINT('Ctrl Pts',(59.8182762284612,-58.6175570020629,
-216.822606778461));
#217055=CARTESIAN_POINT('Ctrl Pts',(59.8057378540362,-58.6403753963495,
-216.822881947839));
#217056=CARTESIAN_POINT('Ctrl Pts',(59.7949528527874,-58.6598895003186,
-216.823112105107));
#217057=CARTESIAN_POINT('Ctrl Pts',(59.7823725663588,-58.6826519471338,
-216.82338057465));
#217058=CARTESIAN_POINT('Ctrl Pts',(59.7721774792337,-58.7009207038603,
-216.82358779928));
#217059=CARTESIAN_POINT('Ctrl Pts',(59.764413184972,-58.7148074027386,-216.823733778996));
#217060=CARTESIAN_POINT('Ctrl Pts',(59.7639315295643,-58.715668859477,-216.823742834799));
#217061=CARTESIAN_POINT('Ctrl Pts',(59.7634592167051,-58.7165134410566,
-216.823751654913));
#217062=CARTESIAN_POINT('Ctrl Pts',(59.7629962529251,-58.7173411691037,
-216.823760239338));
#217063=CARTESIAN_POINT('Ctrl Pts',(59.7590332786009,-58.7244265289962,
-216.823833722101));
#217064=CARTESIAN_POINT('Ctrl Pts',(59.7557554978705,-58.7302773052047,
-216.823889935053));
#217065=CARTESIAN_POINT('Ctrl Pts',(59.7531659200656,-58.7349047974698,
-216.82392889424));
#217066=CARTESIAN_POINT('Ctrl Pts',(59.7518711311631,-58.7372185436024,
-216.823948373834));
#217067=CARTESIAN_POINT('Ctrl Pts',(59.7507483680804,-58.739226455036,-216.823963511933));
#217068=CARTESIAN_POINT('Ctrl Pts',(59.7497978555437,-58.7409294698187,
-216.823974344221));
#217069=CARTESIAN_POINT('Ctrl Pts',(59.7493225992753,-58.7417809772101,
-216.823979760365));
#217070=CARTESIAN_POINT('Ctrl Pts',(59.7488904041548,-58.7425562596209,
-216.823984098381));
#217071=CARTESIAN_POINT('Ctrl Pts',(59.7485012918142,-58.7432554149837,
-216.823987357719));
#217072=CARTESIAN_POINT('Ctrl Pts',(59.7483067356439,-58.743604992665,-216.823988987388));
#217073=CARTESIAN_POINT('Ctrl Pts',(59.7481229499662,-58.7439355379926,
-216.823990347285));
#217074=CARTESIAN_POINT('Ctrl Pts',(59.7479553264888,-58.74423756571,-216.823991302489));
#217075=CARTESIAN_POINT('Ctrl Pts',(59.7477877030115,-58.7445395934275,
-216.823992257693));
#217076=CARTESIAN_POINT('Ctrl Pts',(59.7476255091587,-58.7448323222523,
-216.823993077977));
#217077=CARTESIAN_POINT('Ctrl Pts',(59.7467469666766,-58.7464181291695,
-216.823996273977));
#217078=CARTESIAN_POINT('Ctrl Pts',(59.7093801477012,-58.8138668424792,
-216.824132208612));
#217079=CARTESIAN_POINT('Ctrl Pts',(59.671557263908,-58.8808174952574,-216.824072812657));
#217080=CARTESIAN_POINT('Ctrl Pts',(59.6338697911996,-58.9464350884605,
-216.823817390672));
#217081=CARTESIAN_POINT('Ctrl Pts',(59.6148480499456,-58.9795538090835,
-216.823688473274));
#217082=CARTESIAN_POINT('Ctrl Pts',(59.5958613342072,-59.012333442612,-216.823509619128));
#217083=CARTESIAN_POINT('Ctrl Pts',(59.576987047306,-59.0446718084732,-216.823280738817));
#217084=CARTESIAN_POINT('Ctrl Pts',(59.5488522419803,-59.0928767357806,
-216.822939560206));
#217085=CARTESIAN_POINT('Ctrl Pts',(59.520967162405,-59.1401021366816,-216.822487212211));
#217086=CARTESIAN_POINT('Ctrl Pts',(59.4934981529907,-59.1861679523762,
-216.821923708002));
#217087=CARTESIAN_POINT('Ctrl Pts',(59.4797636482836,-59.2092008602235,
-216.821641955898));
#217088=CARTESIAN_POINT('Ctrl Pts',(59.4661331607649,-59.2319438715733,
-216.821332414342));
#217089=CARTESIAN_POINT('Ctrl Pts',(59.4526274993308,-59.2543744490891,
-216.82099508287));
#217090=CARTESIAN_POINT('Ctrl Pts',(59.4458746686138,-59.2655897378471,
-216.820826417134));
#217091=CARTESIAN_POINT('Ctrl Pts',(59.4391530444012,-59.2767269181358,
-216.820650803898));
#217092=CARTESIAN_POINT('Ctrl Pts',(59.4324652288841,-59.2877831705383,
-216.820468243147));
#217093=CARTESIAN_POINT('Ctrl Pts',(59.4266133903066,-59.2974573913905,
-216.820308502491));
#217094=CARTESIAN_POINT('Ctrl Pts',(59.4207874365105,-59.307069651829,-216.820143442642));
#217095=CARTESIAN_POINT('Ctrl Pts',(59.4149891112262,-59.3166180621561,
-216.81997306359));
#217096=CARTESIAN_POINT('Ctrl Pts',(59.4141607790427,-59.3179821207743,
-216.819948723726));
#217097=CARTESIAN_POINT('Ctrl Pts',(59.4127237069262,-59.3203476995733,
-216.819906186974));
#217098=CARTESIAN_POINT('Ctrl Pts',(59.412505811316,-59.3207063232844,-216.819899718332));
#217099=CARTESIAN_POINT('Ctrl Pts',(59.4101950050686,-59.3245095660916,
-216.81983111769));
#217100=CARTESIAN_POINT('Ctrl Pts',(59.4065064701905,-59.3304507048173,
-216.819787891195));
#217101=CARTESIAN_POINT('Ctrl Pts',(59.4014629664427,-59.3384677889279,
-216.819770038848));
#217102=CARTESIAN_POINT('Ctrl Pts',(59.3965571326525,-59.3462660347695,
-216.819752673807));
#217103=CARTESIAN_POINT('Ctrl Pts',(59.390369086223,-59.3560285473249,-216.819759316569));
#217104=CARTESIAN_POINT('Ctrl Pts',(59.3829384292983,-59.3676532194846,
-216.819789967134));
#217105=CARTESIAN_POINT('Ctrl Pts',(59.3755077723737,-59.3792778916444,
-216.819820617699));
#217106=CARTESIAN_POINT('Ctrl Pts',(59.3668340747563,-59.3927651891293,
-216.819875276067));
#217107=CARTESIAN_POINT('Ctrl Pts',(59.3569807137444,-59.4079627143511,
-216.819953942239));
#217108=CARTESIAN_POINT('Ctrl Pts',(59.345244910556,-59.4260636613008,-216.820047637243));
#217109=CARTESIAN_POINT('Ctrl Pts',(59.3318368966217,-59.446588707006,-216.820175389473));
#217110=CARTESIAN_POINT('Ctrl Pts',(59.3168812995138,-59.4692357632739,
-216.820337198929));
#217111=CARTESIAN_POINT('Ctrl Pts',(59.3114313506556,-59.4774885463329,
-216.820396163693));
#217112=CARTESIAN_POINT('Ctrl Pts',(59.3057761218172,-59.486022628311,-216.820459651041));
#217113=CARTESIAN_POINT('Ctrl Pts',(59.299922358357,-59.4948219380608,-216.820527660973));
#217114=CARTESIAN_POINT('Ctrl Pts',(59.2894628196999,-59.5105445959898,
-216.820649181515));
#217115=CARTESIAN_POINT('Ctrl Pts',(59.2783692893878,-59.5271142151468,
-216.820785141153));
#217116=CARTESIAN_POINT('Ctrl Pts',(59.2666825624745,-59.5444352646829,
-216.820935540058));
#217117=CARTESIAN_POINT('Ctrl Pts',(59.2608391990179,-59.553095789451,-216.821010739511));
#217118=CARTESIAN_POINT('Ctrl Pts',(59.2548475363252,-59.561944171757,-216.821089548675));
#217119=CARTESIAN_POINT('Ctrl Pts',(59.248712924834,-59.5709681710487,-216.821171967444));
#217120=CARTESIAN_POINT('Ctrl Pts',(59.2456456190885,-59.5754801706945,
-216.821213176829));
#217121=CARTESIAN_POINT('Ctrl Pts',(59.2425425764809,-59.5800360748127,
-216.821255289034));
#217122=CARTESIAN_POINT('Ctrl Pts',(59.2394044660912,-59.5846343656262,
-216.821298303416));
#217123=CARTESIAN_POINT('Ctrl Pts',(59.2368833700425,-59.5883285418536,
-216.821332860324));
#217124=CARTESIAN_POINT('Ctrl Pts',(59.2338763518166,-59.5927271064996,
-216.821374460242));
#217125=CARTESIAN_POINT('Ctrl Pts',(59.231500599681,-59.5961969430932,-216.821407532326));
#217126=CARTESIAN_POINT('Ctrl Pts',(59.2309191568838,-59.5970461526822,
-216.821415626405));
#217127=CARTESIAN_POINT('Ctrl Pts',(59.2303754231141,-59.5978399769206,
-216.821423209684));
#217128=CARTESIAN_POINT('Ctrl Pts',(59.2298856041354,-59.5985548823212,
-216.821430053904));
#217129=CARTESIAN_POINT('Ctrl Pts',(59.209665444883,-59.6280668074965,-216.821712589333));
#217130=CARTESIAN_POINT('Ctrl Pts',(59.190618034438,-59.6556168075343,-216.821931387029));
#217131=CARTESIAN_POINT('Ctrl Pts',(59.1726374240291,-59.6814738124503,
-216.822086446994));
#217132=CARTESIAN_POINT('Ctrl Pts',(59.1551735707798,-59.7065876950744,
-216.822237050583));
#217133=CARTESIAN_POINT('Ctrl Pts',(59.1387162929886,-59.7301038456633,
-216.822327527399));
#217134=CARTESIAN_POINT('Ctrl Pts',(59.1231840355727,-59.752224284079,-216.822357877443));
#217135=CARTESIAN_POINT('Ctrl Pts',(59.1074219776338,-59.7746719954842,
-216.822388676518));
#217136=CARTESIAN_POINT('Ctrl Pts',(59.0926126061971,-59.7956820867913,
-216.822357556502));
#217137=CARTESIAN_POINT('Ctrl Pts',(59.0786847843651,-59.8154259777699,
-216.822264517394));
#217138=CARTESIAN_POINT('Ctrl Pts',(59.0717208734491,-59.8252979232592,
-216.82221799784));
#217139=CARTESIAN_POINT('Ctrl Pts',(59.0649775596332,-59.8348527320287,
-216.822155998507));
#217140=CARTESIAN_POINT('Ctrl Pts',(59.0584471400814,-59.8441085381158,
-216.82207852147));
#217141=CARTESIAN_POINT('Ctrl Pts',(59.0551819303055,-59.8487364411594,
-216.822039782951));
#217142=CARTESIAN_POINT('Ctrl Pts',(59.0519699404847,-59.8532895909422,
-216.821997170372));
#217143=CARTESIAN_POINT('Ctrl Pts',(59.0488102987358,-59.8577700233926,
-216.821950690937));
#217144=CARTESIAN_POINT('Ctrl Pts',(59.0465865056734,-59.8609234045008,
-216.821917978162));
#217145=CARTESIAN_POINT('Ctrl Pts',(59.0449907155021,-59.8631849981604,
-216.821893998581));
#217146=CARTESIAN_POINT('Ctrl Pts',(59.0427507400838,-59.8663637683885,
-216.82185626504));
#217147=CARTESIAN_POINT('Ctrl Pts',(59.0418080813048,-59.8677015043465,
-216.821840385467));
#217148=CARTESIAN_POINT('Ctrl Pts',(59.0407515417077,-59.8692012370604,
-216.821822070046));
#217149=CARTESIAN_POINT('Ctrl Pts',(59.0394875349051,-59.8709951915532,
-216.821799642799));
#217150=CARTESIAN_POINT('Ctrl Pts',(59.0135515911386,-59.9078050431719,
-216.821339461873));
#217151=CARTESIAN_POINT('Ctrl Pts',(58.9883333235131,-59.9434790847653,
-216.820707237385));
#217152=CARTESIAN_POINT('Ctrl Pts',(58.9637410153438,-59.9783059369304,
-216.819902969334));
#217153=CARTESIAN_POINT('Ctrl Pts',(58.9559613748387,-59.989323218753,-216.81964854359));
#217154=CARTESIAN_POINT('Ctrl Pts',(58.9482443777768,-60.0002557171563,
-216.819376900789));
#217155=CARTESIAN_POINT('Ctrl Pts',(58.9405878012406,-60.0111070272961,
-216.819088040933));
#217156=CARTESIAN_POINT('Ctrl Pts',(58.9246578683285,-60.033683780982,-216.81848705195));
#217157=CARTESIAN_POINT('Ctrl Pts',(58.9089894699818,-60.055909105829,-216.817811535297));
#217158=CARTESIAN_POINT('Ctrl Pts',(58.8935626743483,-60.0778152568291,
-216.817061490999));
#217159=CARTESIAN_POINT('Ctrl Pts',(58.8858492765315,-60.0887683323292,
-216.81668646885));
#217160=CARTESIAN_POINT('Ctrl Pts',(58.8781962793657,-60.099641614347,-216.816292814753));
#217161=CARTESIAN_POINT('Ctrl Pts',(58.8706012070292,-60.110439113199,-216.815880528753));
#217162=CARTESIAN_POINT('Ctrl Pts',(58.866803670861,-60.115837862625,-216.815674385752));
#217163=CARTESIAN_POINT('Ctrl Pts',(58.863020615899,-60.1212176662587,-216.815463584775));
#217164=CARTESIAN_POINT('Ctrl Pts',(58.8592517332946,-60.1265790245349,
-216.815248125819));
#217165=CARTESIAN_POINT('Ctrl Pts',(58.8564250713412,-60.1306000432421,
-216.815086531601));
#217166=CARTESIAN_POINT('Ctrl Pts',(58.8536063813388,-60.1346106864355,
-216.814922317271));
#217167=CARTESIAN_POINT('Ctrl Pts',(58.8507955332033,-60.1386111649472,
-216.814755482828));
#217168=CARTESIAN_POINT('Ctrl Pts',(58.8498585838248,-60.1399446577845,
-216.814699871346));
#217169=CARTESIAN_POINT('Ctrl Pts',(58.8480958402674,-60.1424537514167,
-216.814594297181));
#217170=CARTESIAN_POINT('Ctrl Pts',(58.847987294226,-60.1426082630128,-216.814587775013));
#217171=CARTESIAN_POINT('Ctrl Pts',(58.8468665099384,-60.1442036613052,
-216.81452043084));
#217172=CARTESIAN_POINT('Ctrl Pts',(58.8440935586267,-60.1480106610434,
-216.814434654858));
#217173=CARTESIAN_POINT('Ctrl Pts',(58.8396892604093,-60.1539873399552,
-216.814330447067));
#217174=CARTESIAN_POINT('Ctrl Pts',(58.8351105470343,-60.1602007020666,
-216.814222112531));
#217175=CARTESIAN_POINT('Ctrl Pts',(58.8287688656326,-60.1687588230416,
-216.81409385744));
#217176=CARTESIAN_POINT('Ctrl Pts',(58.8207128959423,-60.1795626343486,
-216.813945681793));
#217177=CARTESIAN_POINT('Ctrl Pts',(58.811869777269,-60.191422086306,-216.813783027901));
#217178=CARTESIAN_POINT('Ctrl Pts',(58.8009614040296,-60.2059870821187,
-216.813596370391));
#217179=CARTESIAN_POINT('Ctrl Pts',(58.7880784139399,-60.2230686165378,
-216.813385709263));
#217180=CARTESIAN_POINT('Ctrl Pts',(58.7710458173898,-60.2456521070313,
-216.813107194263));
#217181=CARTESIAN_POINT('Ctrl Pts',(58.7505644746547,-60.2726315580116,
-216.8127867222));
#217182=CARTESIAN_POINT('Ctrl Pts',(58.7268679369996,-60.3034884132764,
-216.812424293076));
#217183=CARTESIAN_POINT('Ctrl Pts',(58.7099212444828,-60.3255558412619,
-216.812165100149));
#217184=CARTESIAN_POINT('Ctrl Pts',(58.6913314136815,-60.3496032862428,
-216.811884448436));
#217185=CARTESIAN_POINT('Ctrl Pts',(58.6711668129565,-60.3754537841668,
-216.811582337935));
#217186=CARTESIAN_POINT('Ctrl Pts',(58.6631352792496,-60.3857500031817,
-216.811462007723));
#217187=CARTESIAN_POINT('Ctrl Pts',(58.6548536162727,-60.3963326193122,
-216.81133827325));
#217188=CARTESIAN_POINT('Ctrl Pts',(58.6463245735781,-60.4071924582901,
-216.811211134516));
#217189=CARTESIAN_POINT('Ctrl Pts',(62.1098409646983,-54.1012044962367,
-213.84767448904));
#217190=CARTESIAN_POINT('Ctrl Pts',(62.0847752059267,-54.0775469760354,
-215.334866061346));
#217191=CARTESIAN_POINT('Ctrl Pts',(61.2512793605065,-54.0263658558187,
-216.565923216592));
#217192=CARTESIAN_POINT('Ctrl Pts',(62.1058460411768,-54.2039809660857,
-213.849362952052));
#217193=CARTESIAN_POINT('Ctrl Pts',(62.0790252058314,-54.2159363746381,
-215.358533969393));
#217194=CARTESIAN_POINT('Ctrl Pts',(61.2229035024388,-54.1935258578861,
-216.601366064467));
#217195=CARTESIAN_POINT('Ctrl Pts',(62.1019433372586,-54.3058734208768,
-213.846873799599));
#217196=CARTESIAN_POINT('Ctrl Pts',(62.0728759814261,-54.3629917147794,
-215.384322257423));
#217197=CARTESIAN_POINT('Ctrl Pts',(61.1851466716199,-54.3765718104657,
-216.640959213404));
#217198=CARTESIAN_POINT('Ctrl Pts',(62.0951493333585,-54.4857552569347,
-213.835536336055));
#217199=CARTESIAN_POINT('Ctrl Pts',(62.062450771888,-54.6155445114012,-215.41819658183));
#217200=CARTESIAN_POINT('Ctrl Pts',(61.1204223943136,-54.6858014957792,
-216.694930502363));
#217201=CARTESIAN_POINT('Ctrl Pts',(62.0922232746455,-54.5640610712165,
-213.828298048138));
#217202=CARTESIAN_POINT('Ctrl Pts',(62.058075754172,-54.7227158315903,-215.428854453095));
#217203=CARTESIAN_POINT('Ctrl Pts',(61.0933565049856,-54.8149488052244,
-216.712883469383));
#217204=CARTESIAN_POINT('Ctrl Pts',(62.0827290302579,-54.8200529665633,
-213.798945603707));
#217205=CARTESIAN_POINT('Ctrl Pts',(62.0441877755472,-55.0659530526541,
-215.453222968095));
#217206=CARTESIAN_POINT('Ctrl Pts',(61.0091373101189,-55.2224505676427,
-216.757651828807));
#217207=CARTESIAN_POINT('Ctrl Pts',(62.076302448301,-54.9963150897595,-213.769847381886));
#217208=CARTESIAN_POINT('Ctrl Pts',(62.0350662400492,-55.2949984649606,
-215.456884065042));
#217209=CARTESIAN_POINT('Ctrl Pts',(60.9535367563429,-55.4889120684891,
-216.77161448955));
#217210=CARTESIAN_POINT('Ctrl Pts',(62.0700163106713,-55.1711147821028,
-213.733564105162));
#217211=CARTESIAN_POINT('Ctrl Pts',(62.0256791069586,-55.5302233529213,
-215.457837347772));
#217212=CARTESIAN_POINT('Ctrl Pts',(60.8876885241678,-55.7663600659722,
-216.781995879541));
#217213=CARTESIAN_POINT('',(61.2313176176752,-54.1392424392486,-216.589725631893));
#217214=CARTESIAN_POINT('',(62.1072060041622,-54.1692103455281,-213.848185004792));
#217215=CARTESIAN_POINT('Origin',(57.1116967348753,-53.976149530741,-213.760922972606));
#217216=CARTESIAN_POINT('Ctrl Pts',(62.072365351932,-55.1059089910533,-213.746749287634));
#217217=CARTESIAN_POINT('Ctrl Pts',(62.0768793934982,-54.9808272265131,
-213.771366922161));
#217218=CARTESIAN_POINT('Ctrl Pts',(62.0814562559799,-54.8552883750893,
-213.792161075658));
#217219=CARTESIAN_POINT('Ctrl Pts',(62.0861030190974,-54.7293175780445,
-213.808641588953));
#217220=CARTESIAN_POINT('Ctrl Pts',(62.0871755724076,-54.7002413389646,
-213.812445576512));
#217221=CARTESIAN_POINT('Ctrl Pts',(62.088251845208,-54.6711421307964,-213.816019960792));
#217222=CARTESIAN_POINT('Ctrl Pts',(62.0893319159673,-54.6420203440083,
-213.819359111929));
#217223=CARTESIAN_POINT('Ctrl Pts',(62.0922302587967,-54.5638727585909,
-213.828319640368));
#217224=CARTESIAN_POINT('Ctrl Pts',(62.0951568916034,-54.4855551406274,
-213.835548948843));
#217225=CARTESIAN_POINT('Ctrl Pts',(62.0981243813907,-54.4069862261454,
-213.840500934119));
#217226=CARTESIAN_POINT('Ctrl Pts',(62.1011078230656,-54.3279949605924,
-213.845479539036));
#217227=CARTESIAN_POINT('Ctrl Pts',(62.1041343851103,-54.2487398377214,
-213.848073534587));
#217228=CARTESIAN_POINT('Ctrl Pts',(62.1072060041623,-54.1692103455281,
-213.848185004792));
#217229=CARTESIAN_POINT('Ctrl Pts',(61.2313176176752,-54.1392424392486,
-216.589725631893));
#217230=CARTESIAN_POINT('Ctrl Pts',(61.2129639729121,-54.2384590041938,
-216.610734004428));
#217231=CARTESIAN_POINT('Ctrl Pts',(61.1963872015487,-54.3223059115667,
-216.627485554306));
#217232=CARTESIAN_POINT('Ctrl Pts',(61.1768147446742,-54.4186192835125,
-216.64622764514));
#217233=CARTESIAN_POINT('Ctrl Pts',(61.1711748801229,-54.4458286746357,
-216.651410803087));
#217234=CARTESIAN_POINT('Ctrl Pts',(61.1643153908603,-54.4787172038371,
-216.657589231512));
#217235=CARTESIAN_POINT('Ctrl Pts',(61.1612845711754,-54.4931830366251,
-216.660279368601));
#217236=CARTESIAN_POINT('Ctrl Pts',(61.158491861122,-54.5065045129988,-216.662719476904));
#217237=CARTESIAN_POINT('Ctrl Pts',(61.157285649663,-54.51226760884,-216.663764934813));
#217238=CARTESIAN_POINT('Ctrl Pts',(61.1568098734461,-54.5145442864167,
-216.664175574723));
#217239=CARTESIAN_POINT('Ctrl Pts',(61.1565018821742,-54.5160190449251,
-216.664441020556));
#217240=CARTESIAN_POINT('Ctrl Pts',(61.1566637740706,-54.5152420950941,
-216.664302098725));
#217241=CARTESIAN_POINT('Ctrl Pts',(61.1416133774214,-54.5874172342758,
-216.677234683339));
#217242=CARTESIAN_POINT('Ctrl Pts',(61.1274208796436,-54.6546260509771,
-216.68825404635));
#217243=CARTESIAN_POINT('Ctrl Pts',(61.1005609955658,-54.7818940695041,
-216.707250122171));
#217244=CARTESIAN_POINT('Ctrl Pts',(61.0876513362582,-54.8431501608505,
-216.71536360823));
#217245=CARTESIAN_POINT('Ctrl Pts',(61.031332251096,-55.115600279193,-216.746956680543));
#217246=CARTESIAN_POINT('Ctrl Pts',(60.9789434732668,-55.3729747777418,
-216.765652701273));
#217247=CARTESIAN_POINT('Ctrl Pts',(60.9119170756758,-55.6633990141858,
-216.777770284882));
#217248=CARTESIAN_POINT('Ctrl Pts',(61.2313176176758,-54.1392424392492,
-216.589725631893));
#217249=CARTESIAN_POINT('Ctrl Pts',(62.080918261728,-54.1703109655354,-215.35065029375));
#217250=CARTESIAN_POINT('Ctrl Pts',(62.1072060041624,-54.1692103455281,
-213.848185004792));
#217251=CARTESIAN_POINT('Ctrl Pts',(61.3352033242247,-51.5493321211752,
-216.587755286045));
#217252=CARTESIAN_POINT('Ctrl Pts',(62.1810780798069,-51.5788094394057,
-215.35057926127));
#217253=CARTESIAN_POINT('Ctrl Pts',(62.2073146990362,-51.5772242306454,
-213.851818178003));
#217254=CARTESIAN_POINT('Ctrl Pts',(61.4293178843645,-48.9588621990231,
-216.585940879273));
#217255=CARTESIAN_POINT('Ctrl Pts',(62.2718155001796,-48.9862078816508,
-215.350513478332));
#217256=CARTESIAN_POINT('Ctrl Pts',(62.2979780119688,-48.9848138223875,
-213.855140923936));
#217257=CARTESIAN_POINT('Ctrl Pts',(61.5136373793521,-46.3682170785133,
-216.584262774589));
#217258=CARTESIAN_POINT('Ctrl Pts',(62.3531001006731,-46.3930946875274,
-215.350420378609));
#217259=CARTESIAN_POINT('Ctrl Pts',(62.3791894693652,-46.3921971636372,
-213.85810601718));
#217260=CARTESIAN_POINT('',(61.7446212189112,-46.4961938534599,-216.203488006702));
#217261=CARTESIAN_POINT('',(62.3685680449238,-46.7295402395978,-213.85775323375));
#217262=CARTESIAN_POINT('Ctrl Pts',(61.744621222757,-46.4961938535833,-216.203488008845));
#217263=CARTESIAN_POINT('Ctrl Pts',(61.823821619514,-46.5121026275102,-216.060434887725));
#217264=CARTESIAN_POINT('Ctrl Pts',(61.9058788067412,-46.5300994083013,
-215.895819447354));
#217265=CARTESIAN_POINT('Ctrl Pts',(62.0235044292652,-46.5599185298986,
-215.613803489315));
#217266=CARTESIAN_POINT('Ctrl Pts',(62.0617695753442,-46.5703278495255,
-215.513967395468));
#217267=CARTESIAN_POINT('Ctrl Pts',(62.1162526519497,-46.586598946888,-215.355377457539));
#217268=CARTESIAN_POINT('Ctrl Pts',(62.1427627631244,-46.5948986888364,
-215.273876942239));
#217269=CARTESIAN_POINT('Ctrl Pts',(62.1720569338811,-46.6048578961246,
-215.174955056835));
#217270=CARTESIAN_POINT('Ctrl Pts',(62.1862495019753,-46.6099050968833,
-215.124540908492));
#217271=CARTESIAN_POINT('Ctrl Pts',(62.1922296880582,-46.6120825122955,
-215.10273136339));
#217272=CARTESIAN_POINT('Ctrl Pts',(62.1961931824135,-46.6135372894546,
-215.088146545192));
#217273=CARTESIAN_POINT('Ctrl Pts',(62.1984567548069,-46.614375749181,-215.07973190005));
#217274=CARTESIAN_POINT('Ctrl Pts',(62.3066601348565,-46.6547437913238,
-214.674282540586));
#217275=CARTESIAN_POINT('Ctrl Pts',(62.3626521870614,-46.692922721645,-214.26279861847));
#217276=CARTESIAN_POINT('Ctrl Pts',(62.3685682383788,-46.7295544375158,
-213.857742675887));
#217277=CARTESIAN_POINT('Origin',(-1003.27568749664,-12.9672887026865,-175.207747633911));
#217278=CARTESIAN_POINT('',(61.5121276274299,-46.4145707938174,-216.584292818064));
#217279=CARTESIAN_POINT('Origin',(-967.127514096642,-12.8777453687604,-231.930774818293));
#217280=CARTESIAN_POINT('Origin',(59.4886098259839,-41.5000831614117,-215.164704043177));
#217281=CARTESIAN_POINT('Ctrl Pts',(61.6670578759491,-45.7769853366197,
-216.220244871724));
#217282=CARTESIAN_POINT('Ctrl Pts',(61.620109783049,-46.0863015287385,-216.444037055829));
#217283=CARTESIAN_POINT('Ctrl Pts',(61.4891978237332,-46.4033111269098,
-216.618195686949));
#217284=CARTESIAN_POINT('Ctrl Pts',(61.7028325176855,-45.8210961670719,
-216.166526245294));
#217285=CARTESIAN_POINT('Ctrl Pts',(61.6781627682026,-46.1318587895498,
-216.346038562299));
#217286=CARTESIAN_POINT('Ctrl Pts',(61.5806679860909,-46.4492865503325,
-216.484073286616));
#217287=CARTESIAN_POINT('Ctrl Pts',(61.7397430092403,-45.8565257688032,
-216.106843396371));
#217288=CARTESIAN_POINT('Ctrl Pts',(61.7393332826304,-46.1679717108974,
-216.237169913932));
#217289=CARTESIAN_POINT('Ctrl Pts',(61.674934118594,-46.4851009680931,-216.332569263343));
#217290=CARTESIAN_POINT('Ctrl Pts',(61.7761254129207,-45.8740236618143,
-216.040906882924));
#217291=CARTESIAN_POINT('Ctrl Pts',(61.8021587798992,-46.1846331282861,
-216.116674563313));
#217292=CARTESIAN_POINT('Ctrl Pts',(61.7678808137169,-46.5004734283573,
-216.161019659926));
#217293=CARTESIAN_POINT('',(61.7670326019138,-45.86927832895,-216.057267272101));
#217294=CARTESIAN_POINT('',(61.6760242364037,-45.7878268313144,-216.206690793879));
#217295=CARTESIAN_POINT('Ctrl Pts',(61.7670197730419,-45.8692809645528,
-216.057260894207));
#217296=CARTESIAN_POINT('Ctrl Pts',(61.7550845763212,-45.8625955283723,
-216.078505375557));
#217297=CARTESIAN_POINT('Ctrl Pts',(61.7431797213835,-45.854115763207,-216.09895572692));
#217298=CARTESIAN_POINT('Ctrl Pts',(61.7313327680375,-45.8441875378893,
-216.118692871638));
#217299=CARTESIAN_POINT('Ctrl Pts',(61.7181196261084,-45.8331143913684,
-216.140706100425));
#217300=CARTESIAN_POINT('Ctrl Pts',(61.7049782714986,-45.8202388908385,
-216.161832418214));
#217301=CARTESIAN_POINT('Ctrl Pts',(61.691944051632,-45.8059771378073,-216.182163997265));
#217302=CARTESIAN_POINT('Ctrl Pts',(61.6866187535004,-45.8001503152166,
-216.190470725327));
#217303=CARTESIAN_POINT('Ctrl Pts',(61.6813113300833,-45.7940914684588,
-216.198644553705));
#217304=CARTESIAN_POINT('Ctrl Pts',(61.6760242364037,-45.7878268313144,
-216.206690793879));
#217305=CARTESIAN_POINT('Origin',(59.1250215884199,-46.412156871143,-214.743818340268));
#217306=CARTESIAN_POINT('Origin',(59.0334256450291,-46.3348777618666,-214.896191665971));
#217307=CARTESIAN_POINT('Ctrl Pts',(61.7670197730426,-45.8692809645531,
-216.057260894206));
#217308=CARTESIAN_POINT('Ctrl Pts',(61.7864942538559,-46.1800624966811,
-216.146540979352));
#217309=CARTESIAN_POINT('Ctrl Pts',(61.744621222757,-46.4961938535834,-216.203488008845));
#217310=CARTESIAN_POINT('Ctrl Pts',(61.9631621369174,-46.0106807568515,
-215.721163036308));
#217311=CARTESIAN_POINT('Ctrl Pts',(61.9754348687076,-46.2721634433876,
-215.791058678043));
#217312=CARTESIAN_POINT('Ctrl Pts',(61.9444015484922,-46.5363231985591,
-215.842641422359));
#217313=CARTESIAN_POINT('Ctrl Pts',(62.1106980495454,-46.1537572969976,
-215.368567684276));
#217314=CARTESIAN_POINT('Ctrl Pts',(62.1171497321372,-46.3642951884269,
-215.421651993854));
#217315=CARTESIAN_POINT('Ctrl Pts',(62.0956418404433,-46.5759866556878,
-215.465343832486));
#217316=CARTESIAN_POINT('Ctrl Pts',(62.3127271221,-46.4421422876624,-214.631724106531));
#217317=CARTESIAN_POINT('Ctrl Pts',(62.3119048875977,-46.5481874588022,
-214.656051542736));
#217318=CARTESIAN_POINT('Ctrl Pts',(62.3051790602976,-46.6542226656792,
-214.679477777819));
#217319=CARTESIAN_POINT('Ctrl Pts',(62.3662837353377,-46.5885519083916,
-214.24418481767));
#217320=CARTESIAN_POINT('Ctrl Pts',(62.3644265280729,-46.6408054190759,
-214.25579858017));
#217321=CARTESIAN_POINT('Ctrl Pts',(62.3625689806341,-46.6930535773299,
-214.267441525086));
#217322=CARTESIAN_POINT('Ctrl Pts',(62.3685685933127,-46.7295566356152,
-213.857718370431));
#217323=CARTESIAN_POINT('Ctrl Pts',(62.3685685933127,-46.7295566356152,
-213.857718370431));
#217324=CARTESIAN_POINT('Ctrl Pts',(62.3685685933127,-46.7295566356152,
-213.857718370431));
#217325=CARTESIAN_POINT('Ctrl Pts',(61.7670326019138,-45.86927832895,-216.057267272101));
#217326=CARTESIAN_POINT('Ctrl Pts',(61.8196450544845,-45.9072070747506,
-215.96711325074));
#217327=CARTESIAN_POINT('Ctrl Pts',(61.8687216511235,-45.9452722675006,
-215.875738558968));
#217328=CARTESIAN_POINT('Ctrl Pts',(61.9143495212748,-45.9834416652426,
-215.783201258363));
#217329=CARTESIAN_POINT('Ctrl Pts',(61.9604188031332,-46.0219803201725,
-215.689768736313));
#217330=CARTESIAN_POINT('Ctrl Pts',(62.0029730973334,-46.0606255964866,
-215.595150355294));
#217331=CARTESIAN_POINT('Ctrl Pts',(62.0420704302675,-46.099363287737,-215.499366831777));
#217332=CARTESIAN_POINT('Ctrl Pts',(62.081415222604,-46.1383461621038,-215.402977064004));
#217333=CARTESIAN_POINT('Ctrl Pts',(62.1172597709746,-46.177423080767,-215.305406534752));
#217334=CARTESIAN_POINT('Ctrl Pts',(62.1496206711299,-46.2165922631161,
-215.206648172333));
#217335=CARTESIAN_POINT('Ctrl Pts',(62.1719889253612,-46.2436664861635,
-215.138385171383));
#217336=CARTESIAN_POINT('Ctrl Pts',(62.1926918700032,-46.2707850609034,
-215.069554047601));
#217337=CARTESIAN_POINT('Ctrl Pts',(62.2117212103626,-46.2979491248436,
-215.000147998789));
#217338=CARTESIAN_POINT('Ctrl Pts',(62.2374034026224,-46.3346100231978,
-214.906476885869));
#217339=CARTESIAN_POINT('Ctrl Pts',(62.2600776278325,-46.3714179102784,
-214.811587750487));
#217340=CARTESIAN_POINT('Ctrl Pts',(62.2796089098324,-46.4082437749361,
-214.71578939826));
#217341=CARTESIAN_POINT('Ctrl Pts',(62.2991036321638,-46.4450007070266,
-214.620170366368));
#217342=CARTESIAN_POINT('Ctrl Pts',(62.3154669417998,-46.4817752829743,
-214.523646019044));
#217343=CARTESIAN_POINT('Ctrl Pts',(62.3286125540718,-46.5184396641695,
-214.426543203837));
#217344=CARTESIAN_POINT('Ctrl Pts',(62.3417577176969,-46.555102794045,-214.329443702654));
#217345=CARTESIAN_POINT('Ctrl Pts',(62.3516852860051,-46.5916554724708,
-214.231766313919));
#217346=CARTESIAN_POINT('Ctrl Pts',(62.3583595568947,-46.6279743143229,
-214.133849819246));
#217347=CARTESIAN_POINT('Ctrl Pts',(62.3646248451903,-46.6620676285631,
-214.041933401983));
#217348=CARTESIAN_POINT('Ctrl Pts',(62.3680237825966,-46.6959547578441,
-213.949806767614));
#217349=CARTESIAN_POINT('Ctrl Pts',(62.3685680449238,-46.7295402395978,
-213.85775323375));
#217350=CARTESIAN_POINT('Ctrl Pts',(62.3422326083537,21.4655488148376,-214.137178092368));
#217351=CARTESIAN_POINT('Ctrl Pts',(62.3412085237329,20.8691191735829,-215.298600946727));
#217352=CARTESIAN_POINT('Ctrl Pts',(61.7024165239503,20.3282348619418,-216.300609606759));
#217353=CARTESIAN_POINT('Ctrl Pts',(62.3680533687935,20.8390832881022,-213.816997587882));
#217354=CARTESIAN_POINT('Ctrl Pts',(62.3638965167735,20.3074474023936,-215.017927985833));
#217355=CARTESIAN_POINT('Ctrl Pts',(61.7172757020854,19.824196871917,-216.053279622787));
#217356=CARTESIAN_POINT('Ctrl Pts',(62.3936763768326,20.1737977939208,-213.547199312721));
#217357=CARTESIAN_POINT('Ctrl Pts',(62.3866033956745,19.7050928579686,-214.784132304911));
#217358=CARTESIAN_POINT('Ctrl Pts',(61.7283519101567,19.2781211138106,-215.848545883872));
#217359=CARTESIAN_POINT('Ctrl Pts',(62.4421294023084,18.8292102512288,-213.116884807332));
#217360=CARTESIAN_POINT('Ctrl Pts',(62.4297715597234,18.480223357531,-214.418244849069));
#217361=CARTESIAN_POINT('Ctrl Pts',(61.7440121152497,18.1590865773314,-215.532301635935));
#217362=CARTESIAN_POINT('Ctrl Pts',(62.465140608479,18.1462075363528,-212.953486548188));
#217363=CARTESIAN_POINT('Ctrl Pts',(62.4504011796583,17.8540628328224,-214.283557758829));
#217364=CARTESIAN_POINT('Ctrl Pts',(61.7487288909466,17.58324508504,-215.418454515118));
#217365=CARTESIAN_POINT('Ctrl Pts',(62.5088056235126,16.7621631730818,-212.713827714098));
#217366=CARTESIAN_POINT('Ctrl Pts',(62.4897025499552,16.5802648276791,-214.096157268913));
#217367=CARTESIAN_POINT('Ctrl Pts',(61.7533580267159,16.4056510722738,-215.266990172273));
#217368=CARTESIAN_POINT('Ctrl Pts',(62.5294585302,16.0610980086273,-212.637681074457));
#217369=CARTESIAN_POINT('Ctrl Pts',(62.5083765259719,15.9323648740618,-214.043664436094));
#217370=CARTESIAN_POINT('Ctrl Pts',(61.7532369224541,15.8039519787059,-215.229498767323));
#217371=CARTESIAN_POINT('Ctrl Pts',(62.568416048291,14.6428357290655,-212.563275779244));
#217372=CARTESIAN_POINT('Ctrl Pts',(62.5437053983983,14.6184979888445,-214.012589278034));
#217373=CARTESIAN_POINT('Ctrl Pts',(61.7487163900049,14.5792839170071,-215.224013067664));
#217374=CARTESIAN_POINT('Ctrl Pts',(62.5864410346862,13.9358240577698,-212.565541839207));
#217375=CARTESIAN_POINT('Ctrl Pts',(62.5601079803605,13.9617491203001,-214.034345816612));
#217376=CARTESIAN_POINT('Ctrl Pts',(61.7443571097689,13.9650597457188,-215.256029021813));
#217377=CARTESIAN_POINT('Ctrl Pts',(62.6364325628104,11.8237195743705,-212.673714044577));
#217378=CARTESIAN_POINT('Ctrl Pts',(62.6057492551312,11.9950165428146,-214.195845570981));
#217379=CARTESIAN_POINT('Ctrl Pts',(61.7256266748608,12.1232209481819,-215.442654533669));
#217380=CARTESIAN_POINT('Ctrl Pts',(62.6643973443486,10.4250272317226,-212.879944055009));
#217381=CARTESIAN_POINT('Ctrl Pts',(62.6313772356455,10.6897808013045,-214.431496688937));
#217382=CARTESIAN_POINT('Ctrl Pts',(61.7057160584319,10.8942002544619,-215.687059023784));
#217383=CARTESIAN_POINT('Ctrl Pts',(62.6882099634729,8.99324453840434,-213.207737243319));
#217384=CARTESIAN_POINT('Ctrl Pts',(62.6531941668671,9.35784434440792,-214.783414534773));
#217385=CARTESIAN_POINT('Ctrl Pts',(61.6775843047233,9.63385243594079,-216.04393851968));
#217386=CARTESIAN_POINT('Ctrl Pts',(62.6889267575668,8.94986797085776,-213.217780919801));
#217387=CARTESIAN_POINT('Ctrl Pts',(62.6538525956858,9.31739109066463,-214.794211638116));
#217388=CARTESIAN_POINT('Ctrl Pts',(61.676724484433,9.59566774192812,-216.054853410616));
#217389=CARTESIAN_POINT('Ctrl Pts',(62.6899947648924,8.88481924519104,-213.233011700935));
#217390=CARTESIAN_POINT('Ctrl Pts',(62.6548336726685,9.25672938439221,-214.810565067534));
#217391=CARTESIAN_POINT('Ctrl Pts',(61.6754236852739,9.53840185263947,-216.071375999175));
#217392=CARTESIAN_POINT('Ctrl Pts',(62.6903499578519,8.86313707307649,-213.238096257503));
#217393=CARTESIAN_POINT('Ctrl Pts',(62.6552786040791,9.23183909531466,-214.814707920553));
#217394=CARTESIAN_POINT('Ctrl Pts',(61.6776818994437,9.51109461514074,-216.07534089488));
#217395=CARTESIAN_POINT('Ctrl Pts',(62.6910610727136,8.81976237959028,-213.248159965146));
#217396=CARTESIAN_POINT('Ctrl Pts',(62.6561013689098,9.18470089827482,-214.823639829792));
#217397=CARTESIAN_POINT('Ctrl Pts',(61.6806556143609,9.46114018087874,-216.084046497709));
#217398=CARTESIAN_POINT('Ctrl Pts',(62.6914166532021,8.79807157636304,-213.253156652719));
#217399=CARTESIAN_POINT('Ctrl Pts',(62.6565126981162,9.16112631942749,-214.82807085154));
#217400=CARTESIAN_POINT('Ctrl Pts',(61.6821392223453,9.43615432575777,-216.088363130015));
#217401=CARTESIAN_POINT('Ctrl Pts',(62.693194685499,8.68960018849763,-213.277963347887));
#217402=CARTESIAN_POINT('Ctrl Pts',(62.658568741826,9.04324596366052,-214.850046563724));
#217403=CARTESIAN_POINT('Ctrl Pts',(61.6895409461648,9.31118142695972,-216.109764509573));
#217404=CARTESIAN_POINT('Ctrl Pts',(62.6946175261465,8.60276749258736,-213.297243169367));
#217405=CARTESIAN_POINT('Ctrl Pts',(62.6602130641221,8.94883672773494,-214.867068548325));
#217406=CARTESIAN_POINT('Ctrl Pts',(61.6954101007806,9.21106386992964,-216.126303896624));
#217407=CARTESIAN_POINT('Ctrl Pts',(62.6988878681185,8.34209912341666,-213.353350073391));
#217408=CARTESIAN_POINT('Ctrl Pts',(62.665143127837,8.66539857132349,-214.916400103904));
#217409=CARTESIAN_POINT('Ctrl Pts',(61.7128578780018,8.91027943593482,-216.174139388407));
#217410=CARTESIAN_POINT('Ctrl Pts',(62.7017371797686,8.16809322423106,-213.388445162621));
#217411=CARTESIAN_POINT('Ctrl Pts',(62.6684282615003,8.47602746148447,-214.947001892893));
#217412=CARTESIAN_POINT('Ctrl Pts',(61.724276890348,8.70918150967842,-216.203653357584));
#217413=CARTESIAN_POINT('Ctrl Pts',(62.7102973061953,7.64536444866494,-213.486494648388));
#217414=CARTESIAN_POINT('Ctrl Pts',(62.6782774788102,7.90698464843204,-215.031562829203));
#217415=CARTESIAN_POINT('Ctrl Pts',(61.7578672711065,8.10404764104899,-216.284743705441));
#217416=CARTESIAN_POINT('Ctrl Pts',(62.7160201318226,7.29593153216955,-213.542223849032));
#217417=CARTESIAN_POINT('Ctrl Pts',(62.684844443005,7.52585577339385,-215.078390952383));
#217418=CARTESIAN_POINT('Ctrl Pts',(61.7793738539193,7.69817704538221,-216.328880163446));
#217419=CARTESIAN_POINT('Ctrl Pts',(62.7332823333847,6.24451635056923,-213.677692349319));
#217420=CARTESIAN_POINT('Ctrl Pts',(62.7045693598837,6.37797772727193,-215.187097629475));
#217421=CARTESIAN_POINT('Ctrl Pts',(61.8409395976697,6.47220794885748,-216.42854185076));
#217422=CARTESIAN_POINT('Ctrl Pts',(62.7449139403618,5.53942734608012,-213.725811404425));
#217423=CARTESIAN_POINT('Ctrl Pts',(62.7177658905222,5.6055034086315,-215.217916782497));
#217424=CARTESIAN_POINT('Ctrl Pts',(61.8776376267353,5.64552562952192,-216.451762661138));
#217425=CARTESIAN_POINT('Ctrl Pts',(62.7627331655823,4.47441539748971,-213.722866226851));
#217426=CARTESIAN_POINT('Ctrl Pts',(62.7377858408184,4.43512030427846,-215.189372776564));
#217427=CARTESIAN_POINT('Ctrl Pts',(61.9246048946113,4.38883323215275,-216.409638751896));
#217428=CARTESIAN_POINT('Ctrl Pts',(62.7687354860423,4.11817803008359,-213.709326696013));
#217429=CARTESIAN_POINT('Ctrl Pts',(62.7444894112431,4.04343699957454,-215.167470850043));
#217430=CARTESIAN_POINT('Ctrl Pts',(61.9388297011265,3.96768865050412,-216.38283829128));
#217431=CARTESIAN_POINT('Ctrl Pts',(62.7808960763514,3.40303826436503,-213.655109821484));
#217432=CARTESIAN_POINT('Ctrl Pts',(62.7579914493339,3.25632764876865,-215.096816607535));
#217433=CARTESIAN_POINT('Ctrl Pts',(61.9642060846595,3.12029037299094,-216.301632685202));
#217434=CARTESIAN_POINT('Ctrl Pts',(62.7870578417518,3.04396622992889,-213.614329768932));
#217435=CARTESIAN_POINT('Ctrl Pts',(62.764798254127,2.86044742865292,-215.047932027892));
#217436=CARTESIAN_POINT('Ctrl Pts',(61.9753669262453,2.69358808816948,-216.247065417161));
#217437=CARTESIAN_POINT('Ctrl Pts',(62.7994785535875,2.32831168170424,-213.504372226852));
#217438=CARTESIAN_POINT('Ctrl Pts',(62.7784280077131,2.07098012791206,-214.922299288837));
#217439=CARTESIAN_POINT('Ctrl Pts',(61.9941529245256,1.84204963832674,-216.109426235826));
#217440=CARTESIAN_POINT('Ctrl Pts',(62.8057475169848,1.97109323824117,-213.43520790963));
#217441=CARTESIAN_POINT('Ctrl Pts',(62.7852637475919,1.67660733927831,-214.845546681094));
#217442=CARTESIAN_POINT('Ctrl Pts',(62.0018065488482,1.41657236335453,-216.026373118398));
#217443=CARTESIAN_POINT('Ctrl Pts',(62.8136699413683,1.52535840970665,-213.330389729488));
#217444=CARTESIAN_POINT('Ctrl Pts',(62.7938456712648,1.18416909955933,-214.731582640628));
#217445=CARTESIAN_POINT('Ctrl Pts',(62.0091417138508,0.88496462984438,-215.904115945249));
#217446=CARTESIAN_POINT('Ctrl Pts',(62.8152587437295,1.43625087081009,-213.308507593617));
#217447=CARTESIAN_POINT('Ctrl Pts',(62.7955641544421,1.08569455170218,-214.70788534455));
#217448=CARTESIAN_POINT('Ctrl Pts',(62.0104970411636,0.778654812026788,
-215.878741948443));
#217449=CARTESIAN_POINT('Ctrl Pts',(62.81764868783,1.3026492637952,-213.274293620792));
#217450=CARTESIAN_POINT('Ctrl Pts',(62.7981450769487,0.938013811545139,
-214.670972759063));
#217451=CARTESIAN_POINT('Ctrl Pts',(62.0123610115366,0.619204373827452,
-215.839283178847));
#217452=CARTESIAN_POINT('Ctrl Pts',(62.8184464593903,1.25812534522924,-213.262657162745));
#217453=CARTESIAN_POINT('Ctrl Pts',(62.7990059459185,0.888790452628964,
-214.658440360413));
#217454=CARTESIAN_POINT('Ctrl Pts',(62.0129541628601,0.566056612067846,
-215.825897286883));
#217455=CARTESIAN_POINT('Ctrl Pts',(62.8194451065877,1.20248294550228,-213.247820438255));
#217456=CARTESIAN_POINT('Ctrl Pts',(62.8000827277237,0.827267573996727,
-214.642488734758));
#217457=CARTESIAN_POINT('Ctrl Pts',(62.0136602192421,0.499624509372178,
-215.808872193624));
#217458=CARTESIAN_POINT('Ctrl Pts',(62.8196449076661,1.19135509048132,-213.24483853566));
#217459=CARTESIAN_POINT('Ctrl Pts',(62.8002981228947,0.814963083819151,
-214.639284042805));
#217460=CARTESIAN_POINT('Ctrl Pts',(62.0137996613151,0.486338219736283,
-215.805452538661));
#217461=CARTESIAN_POINT('Ctrl Pts',(62.8200446538203,1.16910063183232,-213.238845579474));
#217462=CARTESIAN_POINT('Ctrl Pts',(62.8007289854141,0.790354624727844,
-214.632845981801));
#217463=CARTESIAN_POINT('Ctrl Pts',(62.0140750027388,0.45976589102507,-215.798583917059));
#217464=CARTESIAN_POINT('Ctrl Pts',(62.8202446769491,1.15797422719196,-213.235829903834));
#217465=CARTESIAN_POINT('Ctrl Pts',(62.8009680223541,0.776644373992607,
-214.629327854389));
#217466=CARTESIAN_POINT('Ctrl Pts',(62.0141560873609,0.443889927808329,
-215.794583971007));
#217467=CARTESIAN_POINT('Ctrl Pts',(62.8208444503325,1.12459558460624,-213.226769479739));
#217468=CARTESIAN_POINT('Ctrl Pts',(62.8015104527899,0.745946623824953,
-214.620839027899));
#217469=CARTESIAN_POINT('Ctrl Pts',(62.0148004761842,0.41547430450863,-215.786623443142));
#217470=CARTESIAN_POINT('Ctrl Pts',(62.8212428505405,1.102341230911,-213.22077375003));
#217471=CARTESIAN_POINT('Ctrl Pts',(62.8018707964773,0.725477633258065,
-214.615222311207));
#217472=CARTESIAN_POINT('Ctrl Pts',(62.0152269887982,0.396525463221588,
-215.781356665904));
#217473=CARTESIAN_POINT('Ctrl Pts',(62.8248154365303,0.902034785229426,
-213.167211635172));
#217474=CARTESIAN_POINT('Ctrl Pts',(62.805102284956,0.541229956352993,-214.565055000306));
#217475=CARTESIAN_POINT('Ctrl Pts',(62.0190380353134,0.225940477598872,
-215.734316604759));
#217476=CARTESIAN_POINT('Ctrl Pts',(62.8278985261067,0.72386189685476,-213.122440498364));
#217477=CARTESIAN_POINT('Ctrl Pts',(62.8078932046147,0.377207549051993,
-214.523169982245));
#217478=CARTESIAN_POINT('Ctrl Pts',(62.0222296924439,0.0739868204750567,
-215.695069192559));
#217479=CARTESIAN_POINT('Ctrl Pts',(62.8548240427874,-0.880767445010574,
-212.744334484548));
#217480=CARTESIAN_POINT('Ctrl Pts',(62.8322777445444,-1.10067369440056,
-214.170022992711));
#217481=CARTESIAN_POINT('Ctrl Pts',(62.0492626355665,-1.29628340734911,
-215.364351700278));
#217482=CARTESIAN_POINT('Ctrl Pts',(62.8729565843244,-2.31461725004268,
-212.582049783317));
#217483=CARTESIAN_POINT('Ctrl Pts',(62.8488210432101,-2.42949334313602,
-214.022238296534));
#217484=CARTESIAN_POINT('Ctrl Pts',(62.0615715076119,-2.53314160129442,
-215.228142992244));
#217485=CARTESIAN_POINT('Ctrl Pts',(62.8981414605001,-5.19559191584348,
-212.564399664962));
#217486=CARTESIAN_POINT('Ctrl Pts',(62.8718519000548,-5.1001878562054,-214.022587242802));
#217487=CARTESIAN_POINT('Ctrl Pts',(62.0663646755723,-5.02417617024219,
-215.238634491797));
#217488=CARTESIAN_POINT('Ctrl Pts',(62.9051900334741,-6.64273030664321,
-212.709348944425));
#217489=CARTESIAN_POINT('Ctrl Pts',(62.8783440818401,-6.44396797060244,
-214.171257323535));
#217490=CARTESIAN_POINT('Ctrl Pts',(62.0588087843662,-6.27849882636757,
-215.385574614432));
#217491=CARTESIAN_POINT('Ctrl Pts',(62.9066422728629,-8.27861416050181,
-213.053996708501));
#217492=CARTESIAN_POINT('Ctrl Pts',(62.8797610895578,-7.95625364053062,
-214.512708735063));
#217493=CARTESIAN_POINT('Ctrl Pts',(62.0376955265922,-7.69029576577868,
-215.717956609814));
#217494=CARTESIAN_POINT('Ctrl Pts',(62.9067130375752,-8.46050513615589,
-213.09485254092));
#217495=CARTESIAN_POINT('Ctrl Pts',(62.8798363892243,-8.12450410435317,
-214.553151196536));
#217496=CARTESIAN_POINT('Ctrl Pts',(62.0351702942178,-7.84718504561344,
-215.757241843704));
#217497=CARTESIAN_POINT('Ctrl Pts',(62.9066818269245,-8.7334636680148,-213.160032454394));
#217498=CARTESIAN_POINT('Ctrl Pts',(62.8798247003438,-8.37686367832318,
-214.617556180156));
#217499=CARTESIAN_POINT('Ctrl Pts',(62.0311058209299,-8.08247086921434,
-215.819744443959));
#217500=CARTESIAN_POINT('Ctrl Pts',(62.9066485485958,-8.82432470155739,
-213.182373733743));
#217501=CARTESIAN_POINT('Ctrl Pts',(62.8798000295548,-8.46085638262443,
-214.639616572718));
#217502=CARTESIAN_POINT('Ctrl Pts',(62.0297070531108,-8.16076599954354,
-215.841141115965));
#217503=CARTESIAN_POINT('Ctrl Pts',(62.9065784769814,-8.9377445621295,-213.211068643959));
#217504=CARTESIAN_POINT('Ctrl Pts',(62.879743353183,-8.56567236571989,-214.66792785609));
#217505=CARTESIAN_POINT('Ctrl Pts',(62.0279032485469,-8.25846566363754,
-215.868589453836));
#217506=CARTESIAN_POINT('Ctrl Pts',(62.9065630389366,-8.96042071227823,
-213.21684604351));
#217507=CARTESIAN_POINT('Ctrl Pts',(62.8797307248969,-8.58662834582749,
-214.673627324421));
#217508=CARTESIAN_POINT('Ctrl Pts',(62.0275397202892,-8.27799712775361,
-215.8741142462));
#217509=CARTESIAN_POINT('Ctrl Pts',(62.9065377484219,-8.99442320332278,
-213.225569775073));
#217510=CARTESIAN_POINT('Ctrl Pts',(62.8797098464659,-8.61804933049181,
-214.682231763241));
#217511=CARTESIAN_POINT('Ctrl Pts',(62.0269902683634,-8.3072815813721,-215.882454117388));
#217512=CARTESIAN_POINT('Ctrl Pts',(62.9065289038154,-9.00575475318705,
-213.228490523492));
#217513=CARTESIAN_POINT('Ctrl Pts',(62.8796976742588,-8.62706334820223,
-214.685080386211));
#217514=CARTESIAN_POINT('Ctrl Pts',(62.0264604156775,-8.31439581090885,
-215.885082867452));
#217515=CARTESIAN_POINT('Ctrl Pts',(62.9065107565238,-9.02841676696405,
-213.234337353352));
#217516=CARTESIAN_POINT('Ctrl Pts',(62.879695591268,-8.65191985769815,-214.690932006268));
#217517=CARTESIAN_POINT('Ctrl Pts',(62.0270215450733,-8.3410207670247,-215.89110921259));
#217518=CARTESIAN_POINT('Ctrl Pts',(62.9065017229464,-9.03975023999172,
-213.237248654769));
#217519=CARTESIAN_POINT('Ctrl Pts',(62.8796945523615,-8.66435102539255,
-214.693845992121));
#217520=CARTESIAN_POINT('Ctrl Pts',(62.0273007300244,-8.35433682400823,
-215.894110381235));
#217521=CARTESIAN_POINT('Ctrl Pts',(62.9064567562113,-9.0964299581106,-213.251744484892));
#217522=CARTESIAN_POINT('Ctrl Pts',(62.8796893713575,-8.72651863071803,
-214.708356037324));
#217523=CARTESIAN_POINT('Ctrl Pts',(62.0286897292193,-8.42093498218168,
-215.909056095157));
#217524=CARTESIAN_POINT('Ctrl Pts',(62.906421426558,-9.14181326257087,-213.263146980914));
#217525=CARTESIAN_POINT('Ctrl Pts',(62.8796852689654,-8.77630162451325,
-214.719775098578));
#217526=CARTESIAN_POINT('Ctrl Pts',(62.0297787648922,-8.47427065578853,
-215.920820239223));
#217527=CARTESIAN_POINT('Ctrl Pts',(62.9061093426684,-9.55062130297945,
-213.364009501424));
#217528=CARTESIAN_POINT('Ctrl Pts',(62.8796487835579,-9.22458700993411,
-214.82078775372));
#217529=CARTESIAN_POINT('Ctrl Pts',(62.0393775573417,-8.95480295651162,
-216.024953117001));
#217530=CARTESIAN_POINT('Ctrl Pts',(62.9058739446102,-9.91655549914845,
-213.44114324688));
#217531=CARTESIAN_POINT('Ctrl Pts',(62.8796194018479,-9.62623601331707,
-214.898410179928));
#217532=CARTESIAN_POINT('Ctrl Pts',(62.0464615113934,-9.38552114236539,
-216.105099157688));
#217533=CARTESIAN_POINT('Ctrl Pts',(62.9054945382152,-10.6537874440521,
-213.569065352509));
#217534=CARTESIAN_POINT('Ctrl Pts',(62.8795693127297,-10.435460010221,-215.027900806566));
#217535=CARTESIAN_POINT('Ctrl Pts',(62.0574632007413,-10.2539989076757,
-216.239254263903));
#217536=CARTESIAN_POINT('Ctrl Pts',(62.905350423994,-11.0264379343114,-213.619939162974));
#217537=CARTESIAN_POINT('Ctrl Pts',(62.87954862193,-10.8446388729512,-215.079895997074));
#217538=CARTESIAN_POINT('Ctrl Pts',(62.0613821604612,-10.6933250732436,
-216.293358240871));
#217539=CARTESIAN_POINT('Ctrl Pts',(62.9051593336146,-11.7684901551169,
-213.693446645343));
#217540=CARTESIAN_POINT('Ctrl Pts',(62.8795160056152,-11.6592885823963,
-215.156242176727));
#217541=CARTESIAN_POINT('Ctrl Pts',(62.0658080661948,-11.5683522558103,
-216.37343912484));
#217542=CARTESIAN_POINT('Ctrl Pts',(62.9051117861205,-12.1381923296176,
-213.716251957739));
#217543=CARTESIAN_POINT('Ctrl Pts',(62.8795039952751,-12.0652013454517,
-215.180780877871));
#217544=CARTESIAN_POINT('Ctrl Pts',(62.0663326131717,-12.0043471050542,
-216.399586213771));
#217545=CARTESIAN_POINT('Ctrl Pts',(62.9051036527997,-13.243445563085,-213.744071341037));
#217546=CARTESIAN_POINT('Ctrl Pts',(62.8794748263331,-13.2783114028496,
-215.214676585691));
#217547=CARTESIAN_POINT('Ctrl Pts',(62.0629721988681,-13.3072813139657,
-216.437555879606));
#217548=CARTESIAN_POINT('Ctrl Pts',(62.9052789204624,-13.9751373806058,
-213.708426173576));
#217549=CARTESIAN_POINT('Ctrl Pts',(62.8794655689834,-14.081457450616,-215.184200160213));
#217550=CARTESIAN_POINT('Ctrl Pts',(62.0541257046421,-14.1689833911665,
-216.408834050813));
#217551=CARTESIAN_POINT('Ctrl Pts',(62.9057445940404,-15.0655774299771,
-213.580180828239));
#217552=CARTESIAN_POINT('Ctrl Pts',(62.8794187494639,-15.2755977889231,
-215.065402979219));
#217553=CARTESIAN_POINT('Ctrl Pts',(62.0320573263821,-15.4490848449937,
-216.291038336921));
#217554=CARTESIAN_POINT('Ctrl Pts',(62.9059331942183,-15.4278764578799,
-213.524990067775));
#217555=CARTESIAN_POINT('Ctrl Pts',(62.8793972253274,-15.6723243016018,
-215.013586287052));
#217556=CARTESIAN_POINT('Ctrl Pts',(62.0232381588368,-15.8737432145396,
-216.239343311923));
#217557=CARTESIAN_POINT('Ctrl Pts',(62.9062547760745,-15.9696430762788,
-213.424484058149));
#217558=CARTESIAN_POINT('Ctrl Pts',(62.8793480927401,-16.2648134030746,
-214.918541783998));
#217559=CARTESIAN_POINT('Ctrl Pts',(62.0080259576815,-16.5073872973098,
-216.144071868544));
#217560=CARTESIAN_POINT('Ctrl Pts',(62.9063683773708,-16.1499518187337,
-213.38803074649));
#217561=CARTESIAN_POINT('Ctrl Pts',(62.8793288120533,-16.4619892047426,
-214.883956414301));
#217562=CARTESIAN_POINT('Ctrl Pts',(62.0026218050749,-16.7180652996643,
-216.109363202134));
#217563=CARTESIAN_POINT('Ctrl Pts',(62.9065468872613,-16.4200061599841,
-213.329044171076));
#217564=CARTESIAN_POINT('Ctrl Pts',(62.8792944775105,-16.7571264425052,
-214.827867382111));
#217565=CARTESIAN_POINT('Ctrl Pts',(61.994042677577,-17.0332563013891,-216.052989402922));
#217566=CARTESIAN_POINT('Ctrl Pts',(62.9066077402092,-16.5099561526457,
-213.308664291015));
#217567=CARTESIAN_POINT('Ctrl Pts',(62.8792821285777,-16.8554254196337,
-214.808463837074));
#217568=CARTESIAN_POINT('Ctrl Pts',(61.9911043964934,-17.1381808858366,
-216.033479730101));
#217569=CARTESIAN_POINT('Ctrl Pts',(62.9067008407091,-16.644780457911,-213.277033722408));
#217570=CARTESIAN_POINT('Ctrl Pts',(62.8792621149752,-17.0027153104515,
-214.778320560607));
#217571=CARTESIAN_POINT('Ctrl Pts',(61.9865832503263,-17.2953539198766,
-216.003152916317));
#217572=CARTESIAN_POINT('Ctrl Pts',(62.9067321776173,-16.6897051128861,
-213.266313413053));
#217573=CARTESIAN_POINT('Ctrl Pts',(62.8792551943321,-17.0517917499927,
-214.768098452986));
#217574=CARTESIAN_POINT('Ctrl Pts',(61.985057249836,-17.3477092677032,-215.992866939259));
#217575=CARTESIAN_POINT('Ctrl Pts',(62.9067796117351,-16.7570671165656,
-213.249969786042));
#217576=CARTESIAN_POINT('Ctrl Pts',(62.879244422478,-17.1253666622028,-214.75250769517));
#217577=CARTESIAN_POINT('Ctrl Pts',(61.9827403503223,-17.4261881952898,
-215.977174377362));
#217578=CARTESIAN_POINT('Ctrl Pts',(62.9067954945617,-16.7795169546794,
-213.244478050128));
#217579=CARTESIAN_POINT('Ctrl Pts',(62.8792407664544,-17.1498865664599,
-214.747267502411));
#217580=CARTESIAN_POINT('Ctrl Pts',(61.9819634009862,-17.4523388156653,
-215.971899592409));
#217581=CARTESIAN_POINT('Ctrl Pts',(62.9068194226298,-16.8131854913724,
-213.236174910655));
#217582=CARTESIAN_POINT('Ctrl Pts',(62.8792351823635,-17.1866564730818,
-214.739343052782));
#217583=CARTESIAN_POINT('Ctrl Pts',(61.9807910694282,-17.4915511452329,
-215.963921765975));
#217584=CARTESIAN_POINT('Ctrl Pts',(62.9068274159574,-16.8244073001866,
-213.233396274889));
#217585=CARTESIAN_POINT('Ctrl Pts',(62.8792333042642,-17.1989118397669,
-214.736690790842));
#217586=CARTESIAN_POINT('Ctrl Pts',(61.9803991410476,-17.5046196532664,
-215.961251549351));
#217587=CARTESIAN_POINT('Ctrl Pts',(62.9068434366578,-16.8468488483916,
-213.227817200875));
#217588=CARTESIAN_POINT('Ctrl Pts',(62.8792295142709,-17.223419512581,-214.731364863971));
#217589=CARTESIAN_POINT('Ctrl Pts',(61.9796129930294,-17.5307521218042,
-215.955889275238));
#217590=CARTESIAN_POINT('Ctrl Pts',(62.9068512246001,-16.8580698646293,
-213.225030214802));
#217591=CARTESIAN_POINT('Ctrl Pts',(62.8792447756866,-17.2324410430089,
-214.728381164571));
#217592=CARTESIAN_POINT('Ctrl Pts',(61.980377068186,-17.5380100722587,-215.952980774701));
#217593=CARTESIAN_POINT('Ctrl Pts',(62.9078064251384,-18.3057228153494,
-212.867003491606));
#217594=CARTESIAN_POINT('Ctrl Pts',(62.8802082957154,-18.5725016104741,
-214.363427060571));
#217595=CARTESIAN_POINT('Ctrl Pts',(62.0149243105808,-18.7952395296689,
-215.59183941935));
#217596=CARTESIAN_POINT('Ctrl Pts',(62.9033129898347,-19.7553919607571,
-212.653495577744));
#217597=CARTESIAN_POINT('Ctrl Pts',(62.8762357607657,-19.9205453051955,
-214.136541643927));
#217598=CARTESIAN_POINT('Ctrl Pts',(62.0392411361479,-20.0571576067025,
-215.363703521968));
#217599=CARTESIAN_POINT('Ctrl Pts',(62.8830851680151,-22.6547081034196,
-212.52986856343));
#217600=CARTESIAN_POINT('Ctrl Pts',(62.8581004822445,-22.6112951161231,
-213.975521928866));
#217601=CARTESIAN_POINT('Ctrl Pts',(62.0686653400334,-22.5711272294273,
-215.185493388832));
#217602=CARTESIAN_POINT('Ctrl Pts',(62.8673563795338,-24.1094370634719,
-212.617838162876));
#217603=CARTESIAN_POINT('Ctrl Pts',(62.8439525084138,-23.9605649484755,
-214.038745368151));
#217604=CARTESIAN_POINT('Ctrl Pts',(62.0739679487614,-23.8279590992824,
-215.233708940831));
#217605=CARTESIAN_POINT('Ctrl Pts',(62.8399085993617,-25.9282456355318,
-212.959941102886));
#217606=CARTESIAN_POINT('Ctrl Pts',(62.8193618641866,-25.6370453624972,
-214.33907548895));
#217607=CARTESIAN_POINT('Ctrl Pts',(62.0659506819248,-25.3798830245726,
-215.502362302155));
#217608=CARTESIAN_POINT('Ctrl Pts',(62.8340297350381,-26.2918276350351,
-213.040124650367));
#217609=CARTESIAN_POINT('Ctrl Pts',(62.8141018085935,-25.9715146998356,
-214.410299819559));
#217610=CARTESIAN_POINT('Ctrl Pts',(62.0635946113577,-25.6891136834931,
-215.566638111475));
#217611=CARTESIAN_POINT('Ctrl Pts',(62.8261731592033,-26.7460613321157,
-213.156334850829));
#217612=CARTESIAN_POINT('Ctrl Pts',(62.8070813385858,-26.3885631025506,
-214.514477388603));
#217613=CARTESIAN_POINT('Ctrl Pts',(62.0595992131559,-26.0739174525129,
-215.661200292517));
#217614=CARTESIAN_POINT('Ctrl Pts',(62.8245764208424,-26.8368958608164,
-213.180377302499));
#217615=CARTESIAN_POINT('Ctrl Pts',(62.8056550731544,-26.4719143407304,
-214.536069637883));
#217616=CARTESIAN_POINT('Ctrl Pts',(62.0587474792527,-26.1507912740874,
-215.680824692928));
#217617=CARTESIAN_POINT('Ctrl Pts',(62.8225483225521,-26.950423403808,-213.211454506225));
#217618=CARTESIAN_POINT('Ctrl Pts',(62.8038440965971,-26.5760357433315,
-214.564029548489));
#217619=CARTESIAN_POINT('Ctrl Pts',(62.0576149086873,-26.2467696827909,
-215.706264227521));
#217620=CARTESIAN_POINT('Ctrl Pts',(62.8221410940189,-26.9731281314207,
-213.217721160271));
#217621=CARTESIAN_POINT('Ctrl Pts',(62.8034805008598,-26.5968562497989,
-214.56966990827));
#217622=CARTESIAN_POINT('Ctrl Pts',(62.0573849987646,-26.2659596714963,
-215.71139759155));
#217623=CARTESIAN_POINT('Ctrl Pts',(62.8215278301372,-27.0071840444279,
-213.227198424036));
#217624=CARTESIAN_POINT('Ctrl Pts',(62.8029329912778,-26.6280818473612,
-214.57820358626));
#217625=CARTESIAN_POINT('Ctrl Pts',(62.0570349989822,-26.2947360125198,
-215.719166196104));
#217626=CARTESIAN_POINT('Ctrl Pts',(62.8213230053295,-27.0185358190149,
-213.230370392442));
#217627=CARTESIAN_POINT('Ctrl Pts',(62.8027501360862,-26.6384894816988,
-214.581060324812));
#217628=CARTESIAN_POINT('Ctrl Pts',(62.0569174765794,-26.3043266859831,
-215.721767157448));
#217629=CARTESIAN_POINT('Ctrl Pts',(62.8210151618606,-27.0355631854271,
-213.235147724465));
#217630=CARTESIAN_POINT('Ctrl Pts',(62.8024753235955,-26.6540996350435,
-214.585363770433));
#217631=CARTESIAN_POINT('Ctrl Pts',(62.0567399040033,-26.3187105229747,
-215.725685786475));
#217632=CARTESIAN_POINT('Ctrl Pts',(62.8209124463284,-27.0412389249793,
-213.236743398352));
#217633=CARTESIAN_POINT('Ctrl Pts',(62.8023836313177,-26.659302793678,-214.586801305957));
#217634=CARTESIAN_POINT('Ctrl Pts',(62.0566804983261,-26.3235047731397,
-215.726994860647));
#217635=CARTESIAN_POINT('Ctrl Pts',(62.8207068130133,-27.0525903054424,
-213.239941215787));
#217636=CARTESIAN_POINT('Ctrl Pts',(62.8022000701859,-26.669708670566,-214.589682496766));
#217637=CARTESIAN_POINT('Ctrl Pts',(62.0565612564283,-26.3330925469615,
-215.729618745949));
#217638=CARTESIAN_POINT('Ctrl Pts',(62.8206039569716,-27.0582660000666,
-213.241539781896));
#217639=CARTESIAN_POINT('Ctrl Pts',(62.8020756172633,-26.6766427063805,
-214.591683103012));
#217640=CARTESIAN_POINT('Ctrl Pts',(62.0563759404316,-26.3410999882819,
-215.731950428965));
#217641=CARTESIAN_POINT('Ctrl Pts',(62.8196787974583,-27.1093480735134,
-213.255871682944));
#217642=CARTESIAN_POINT('Ctrl Pts',(62.8010604891949,-26.7335035083587,
-214.607839142305));
#217643=CARTESIAN_POINT('Ctrl Pts',(62.0551041668616,-26.4028713900106,
-215.749611986012));
#217644=CARTESIAN_POINT('Ctrl Pts',(62.8188583609006,-27.1547585116387,
-213.268331481197));
#217645=CARTESIAN_POINT('Ctrl Pts',(62.8001595869042,-26.7840369239728,
-214.621921517333));
#217646=CARTESIAN_POINT('Ctrl Pts',(62.0539403091928,-26.4577601301325,
-215.765023583509));
#217647=CARTESIAN_POINT('Ctrl Pts',(62.8147655328413,-27.3818312159601,
-213.329248041548));
#217648=CARTESIAN_POINT('Ctrl Pts',(62.7956617726082,-27.0366682767733,
-214.690959778013));
#217649=CARTESIAN_POINT('Ctrl Pts',(62.0479560084918,-26.7321109243143,
-215.840660860072));
#217650=CARTESIAN_POINT('Ctrl Pts',(62.811521179222,-27.5635550010564,-213.373559009004));
#217651=CARTESIAN_POINT('Ctrl Pts',(62.792085332894,-27.238636566617,-214.741789248302));
#217652=CARTESIAN_POINT('Ctrl Pts',(62.0426408175475,-26.9512950299888,
-215.89662634158));
#217653=CARTESIAN_POINT('Ctrl Pts',(62.7954319749737,-28.4724876729194,
-213.573958234288));
#217654=CARTESIAN_POINT('Ctrl Pts',(62.7742896842574,-28.2481778367032,
-214.974978243553));
#217655=CARTESIAN_POINT('Ctrl Pts',(62.0135384026934,-28.0458953208882,
-216.15474774953));
#217656=CARTESIAN_POINT('Ctrl Pts',(62.7829855880237,-29.2006385623099,
-213.666528824371));
#217657=CARTESIAN_POINT('Ctrl Pts',(62.7603316101004,-29.0547579215752,
-215.09426369493));
#217658=CARTESIAN_POINT('Ctrl Pts',(61.9820535417445,-28.9180045033719,
-216.291912296996));
#217659=CARTESIAN_POINT('Ctrl Pts',(62.7463293349581,-31.3876040979605,
-213.774365476532));
#217660=CARTESIAN_POINT('Ctrl Pts',(62.7188256094512,-31.4679377673016,
-215.282340428597));
#217661=CARTESIAN_POINT('Ctrl Pts',(61.8687456407067,-31.514819604097,-216.526229178884));
#217662=CARTESIAN_POINT('Ctrl Pts',(62.7227759583408,-32.8489094531929,
-213.621230861582));
#217663=CARTESIAN_POINT('Ctrl Pts',(62.6915950430413,-33.0690705517719,
-215.181307910843));
#217664=CARTESIAN_POINT('Ctrl Pts',(61.7680050000962,-33.2220331134748,
-216.448292898274));
#217665=CARTESIAN_POINT('Ctrl Pts',(62.6973153894392,-34.4039131251247,
-213.297292874274));
#217666=CARTESIAN_POINT('Ctrl Pts',(62.6621683869121,-34.7487344411069,
-214.913581096992));
#217667=CARTESIAN_POINT('Ctrl Pts',(61.6490045697264,-35.0057699870247,
-216.194181682595));
#217668=CARTESIAN_POINT('Ctrl Pts',(62.6958162562235,-34.4953927542909,
-213.277636702595));
#217669=CARTESIAN_POINT('Ctrl Pts',(62.6604275289915,-34.8479236941524,
-214.897160427577));
#217670=CARTESIAN_POINT('Ctrl Pts',(61.6419554736938,-35.1105969222302,
-216.178600343238));
#217671=CARTESIAN_POINT('Ctrl Pts',(62.6939402205335,-34.609753063567,-213.252332432689));
#217672=CARTESIAN_POINT('Ctrl Pts',(62.6582484377325,-34.9718435394741,
-214.875901505568));
#217673=CARTESIAN_POINT('Ctrl Pts',(61.6330839192102,-35.241514474014,-216.158350002109));
#217674=CARTESIAN_POINT('Ctrl Pts',(62.6935649074929,-34.632625664123,-213.247234872736));
#217675=CARTESIAN_POINT('Ctrl Pts',(62.657812349987,-34.9966309075331,-214.871611881384));
#217676=CARTESIAN_POINT('Ctrl Pts',(61.6313066004446,-35.267692149343,-216.15426125142));
#217677=CARTESIAN_POINT('Ctrl Pts',(62.6930017735534,-34.6669353682869,
-213.23953378686));
#217678=CARTESIAN_POINT('Ctrl Pts',(62.6571579734683,-35.0338077059872,
-214.865122644271));
#217679=CARTESIAN_POINT('Ctrl Pts',(61.6286361305327,-35.306950041299,-216.148070435334));
#217680=CARTESIAN_POINT('Ctrl Pts',(62.6928140348451,-34.6783720702322,
-213.23695763384));
#217681=CARTESIAN_POINT('Ctrl Pts',(62.6569397952362,-35.0461999389248,
-214.86295031173));
#217682=CARTESIAN_POINT('Ctrl Pts',(61.6277452254698,-35.3200345655743,
-216.145997215361));
#217683=CARTESIAN_POINT('Ctrl Pts',(62.6924385017241,-34.7012457411244,
-213.231787130787));
#217684=CARTESIAN_POINT('Ctrl Pts',(62.6565033481798,-35.0709834459169,
-214.858587353424));
#217685=CARTESIAN_POINT('Ctrl Pts',(61.6259619219035,-35.3462007537114,
-216.141831601746));
#217686=CARTESIAN_POINT('Ctrl Pts',(62.6922505031027,-34.7126825313609,
-213.229204685838));
#217687=CARTESIAN_POINT('Ctrl Pts',(62.6563676105427,-35.0803506782823,
-214.855199499274));
#217688=CARTESIAN_POINT('Ctrl Pts',(61.6272019533633,-35.3540299418295,
-216.138259961343));
#217689=CARTESIAN_POINT('Ctrl Pts',(62.6913088110138,-34.7698657850159,
-213.216337901175));
#217690=CARTESIAN_POINT('Ctrl Pts',(62.6555047555815,-35.1338645553915,
-214.840975106258));
#217691=CARTESIAN_POINT('Ctrl Pts',(61.6286902735705,-35.4047784879965,
-216.12373712742));
#217692=CARTESIAN_POINT('Ctrl Pts',(62.6905505732427,-34.8156106395255,
-213.206157663252));
#217693=CARTESIAN_POINT('Ctrl Pts',(62.6548100127451,-35.176676489797,-214.829703015251));
#217694=CARTESIAN_POINT('Ctrl Pts',(61.6298739292442,-35.4453709799185,
-216.112221039658));
#217695=CARTESIAN_POINT('Ctrl Pts',(62.6867349314903,-35.0443261388968,
-213.15582449853));
#217696=CARTESIAN_POINT('Ctrl Pts',(62.6513153166306,-35.3906577352144,
-214.773903124995));
#217697=CARTESIAN_POINT('Ctrl Pts',(61.635757391351,-35.6483009438719,-216.05515295758));
#217698=CARTESIAN_POINT('Ctrl Pts',(62.6836041752042,-35.227270469835,-213.117375270577));
#217699=CARTESIAN_POINT('Ctrl Pts',(62.6484482028618,-35.561854520356,-214.730986421537));
#217700=CARTESIAN_POINT('Ctrl Pts',(61.6403527485721,-35.810539975685,-216.011138030016));
#217701=CARTESIAN_POINT('Ctrl Pts',(62.6739757829552,-35.7760179301671,
-213.007568080911));
#217702=CARTESIAN_POINT('Ctrl Pts',(62.6396380425831,-36.0750857329258,
-214.607582586062));
#217703=CARTESIAN_POINT('Ctrl Pts',(61.6538107373805,-36.2969010033139,
-215.884077811248));
#217704=CARTESIAN_POINT('Ctrl Pts',(62.6672458339371,-36.1415480006374,
-212.941772621246));
#217705=CARTESIAN_POINT('Ctrl Pts',(62.6334830510151,-36.4170090776854,
-214.532350962691));
#217706=CARTESIAN_POINT('Ctrl Pts',(61.6623415978292,-36.6205004660809,
-215.806047787868));
#217707=CARTESIAN_POINT('Ctrl Pts',(62.6460655421939,-37.2394079985843,
-212.767180740501));
#217708=CARTESIAN_POINT('Ctrl Pts',(62.6141474585686,-37.4426606009465,
-214.328492936668));
#217709=CARTESIAN_POINT('Ctrl Pts',(61.6866935200193,-37.5909455865243,
-215.592253113864));
#217710=CARTESIAN_POINT('Ctrl Pts',(62.6306238454731,-37.9731020337408,
-212.681065126087));
#217711=CARTESIAN_POINT('Ctrl Pts',(62.6000692240083,-38.1280246284507,
-214.221120830614));
#217712=CARTESIAN_POINT('Ctrl Pts',(61.7012950170652,-38.2375005898279,
-215.476682421731));
#217713=CARTESIAN_POINT('Ctrl Pts',(62.5969132094228,-39.4445711917938,
-212.577895377786));
#217714=CARTESIAN_POINT('Ctrl Pts',(62.5694213181663,-39.4999857528758,
-214.071635186044));
#217715=CARTESIAN_POINT('Ctrl Pts',(61.7271079946506,-39.52809238237,-215.306122006413));
#217716=CARTESIAN_POINT('Ctrl Pts',(62.5786465561153,-40.1823394734562,
-212.56072643116));
#217717=CARTESIAN_POINT('Ctrl Pts',(62.5528572913972,-40.186716811975,-214.029227841839));
#217718=CARTESIAN_POINT('Ctrl Pts',(61.7383115771298,-40.1721899106378,
-215.251065883709));
#217719=CARTESIAN_POINT('Ctrl Pts',(62.5489095967688,-41.2926666211419,
-212.597076537344));
#217720=CARTESIAN_POINT('Ctrl Pts',(62.5259796592712,-41.2177253956526,
-214.023715172298));
#217721=CARTESIAN_POINT('Ctrl Pts',(61.7522529494064,-41.1345693196256,
-215.221901979336));
#217722=CARTESIAN_POINT('Ctrl Pts',(62.5385733023658,-41.6645079426499,
-212.619734584269));
#217723=CARTESIAN_POINT('Ctrl Pts',(62.5166614548086,-41.5622368317271,
-214.031654331973));
#217724=CARTESIAN_POINT('Ctrl Pts',(61.7564322562654,-41.4556717679246,
-215.221175362458));
#217725=CARTESIAN_POINT('Ctrl Pts',(62.5172963966415,-42.4017436060864,
-212.687617475152));
#217726=CARTESIAN_POINT('Ctrl Pts',(62.4975235652628,-42.243965739272,-214.068785079329));
#217727=CARTESIAN_POINT('Ctrl Pts',(61.763623688336,-42.0895206278039,-215.239343116333));
#217728=CARTESIAN_POINT('Ctrl Pts',(62.5063477838447,-42.7675314704579,
-212.732780967694));
#217729=CARTESIAN_POINT('Ctrl Pts',(62.4876965212927,-42.5815841800676,
-214.097879730704));
#217730=CARTESIAN_POINT('Ctrl Pts',(61.7666445972041,-42.4026166823129,
-215.258164485443));
#217731=CARTESIAN_POINT('Ctrl Pts',(62.4725701813139,-43.8557232524475,
-212.904651540613));
#217732=CARTESIAN_POINT('Ctrl Pts',(62.4574785572312,-43.5829084833784,
-214.219091484158));
#217733=CARTESIAN_POINT('Ctrl Pts',(61.773814934178,-43.3290662887116,-215.345785453686));
#217734=CARTESIAN_POINT('Ctrl Pts',(62.4488123543698,-44.5690597591882,
-213.067323574869));
#217735=CARTESIAN_POINT('Ctrl Pts',(62.4363119561656,-44.236699042062,-214.344774294021));
#217736=CARTESIAN_POINT('Ctrl Pts',(61.7761368886402,-43.9296800867984,
-215.445400831427));
#217737=CARTESIAN_POINT('Ctrl Pts',(62.411269138031,-45.6166733720249,-213.400195879719));
#217738=CARTESIAN_POINT('Ctrl Pts',(62.4031003559944,-45.1899483809382,
-214.615484592056));
#217739=CARTESIAN_POINT('Ctrl Pts',(61.7744895314065,-44.7976174234393,
-215.668902106843));
#217740=CARTESIAN_POINT('Ctrl Pts',(62.3984364151383,-45.962125223904,-213.526046844514));
#217741=CARTESIAN_POINT('Ctrl Pts',(62.39179260267,-45.5029471693551,-214.719404394484));
#217742=CARTESIAN_POINT('Ctrl Pts',(61.7730731774584,-45.0814095354759,
-215.755816696107));
#217743=CARTESIAN_POINT('Ctrl Pts',(62.3721154800596,-46.6444314431214,
-213.811880088235));
#217744=CARTESIAN_POINT('Ctrl Pts',(62.3687040669745,-46.1180536806806,
-214.958482420413));
#217745=CARTESIAN_POINT('Ctrl Pts',(61.7680734151979,-45.6360416008198,
-215.957640236994));
#217746=CARTESIAN_POINT('Ctrl Pts',(62.3585615338657,-46.9827912699497,
-213.972791370421));
#217747=CARTESIAN_POINT('Ctrl Pts',(62.3568641610027,-46.4215724898018,
-215.094442901992));
#217748=CARTESIAN_POINT('Ctrl Pts',(61.7644619516127,-45.9080672741359,
-216.073240699382));
#217749=CARTESIAN_POINT('Ctrl Pts',(62.3449264240553,-47.3099624311764,
-214.150201433913));
#217750=CARTESIAN_POINT('Ctrl Pts',(62.3450159671272,-46.7131851982871,
-215.245597852421));
#217751=CARTESIAN_POINT('Ctrl Pts',(61.7595433353131,-46.167485490306,-216.202399824357));
#217752=CARTESIAN_POINT('',(61.7131038227433,20.038950662233,-216.160137831863));
#217753=CARTESIAN_POINT('',(62.3650463286435,20.9007637244406,-213.866522994717));
#217754=CARTESIAN_POINT('Ctrl Pts',(61.7131038227445,20.0389506617929,-216.160137831687));
#217755=CARTESIAN_POINT('Ctrl Pts',(61.7368124258176,20.0546467655865,-216.121235415936));
#217756=CARTESIAN_POINT('Ctrl Pts',(61.761719571167,20.0715966718075,-216.079068639254));
#217757=CARTESIAN_POINT('Ctrl Pts',(61.7875162077924,20.0898264294659,-216.033490938998));
#217758=CARTESIAN_POINT('Ctrl Pts',(61.8136580552382,20.1083001379032,-215.987303317552));
#217759=CARTESIAN_POINT('Ctrl Pts',(61.8407134872745,20.1280882012577,-215.937612918845));
#217760=CARTESIAN_POINT('Ctrl Pts',(61.8683094332131,20.1492190576661,-215.884248757928));
#217761=CARTESIAN_POINT('Ctrl Pts',(61.8959053791516,20.1703499140744,-215.83088459701));
#217762=CARTESIAN_POINT('Ctrl Pts',(61.924041838205,20.1928235921681,-215.773846675231));
#217763=CARTESIAN_POINT('Ctrl Pts',(61.9522938471338,20.2166694774165,-215.712945365588));
#217764=CARTESIAN_POINT('Ctrl Pts',(61.9839298364388,20.2433715846044,-215.644749394626));
#217765=CARTESIAN_POINT('Ctrl Pts',(62.0157021939934,20.2717882751306,-215.571724442015));
#217766=CARTESIAN_POINT('Ctrl Pts',(62.0468955895493,20.3019109118738,-215.493710167469));
#217767=CARTESIAN_POINT('Ctrl Pts',(62.0660815959063,20.3204383305708,-215.445726216356));
#217768=CARTESIAN_POINT('Ctrl Pts',(62.085048844248,20.3396125459156,-215.395850629491));
#217769=CARTESIAN_POINT('Ctrl Pts',(62.1036166227799,20.3594252104984,-215.344058873871));
#217770=CARTESIAN_POINT('Ctrl Pts',(62.1253168115682,20.3825802993589,-215.283529776506));
#217771=CARTESIAN_POINT('Ctrl Pts',(62.1464708764804,20.4066073064949,-215.220383743453));
#217772=CARTESIAN_POINT('Ctrl Pts',(62.1667783859581,20.4314829485095,-215.154604313644));
#217773=CARTESIAN_POINT('Ctrl Pts',(62.1721575938579,20.4380721981753,-215.137180156887));
#217774=CARTESIAN_POINT('Ctrl Pts',(62.1773035625962,20.4445030896074,-215.120148444136));
#217775=CARTESIAN_POINT('Ctrl Pts',(62.1825121872622,20.4511480694473,-215.10252207976));
#217776=CARTESIAN_POINT('Ctrl Pts',(62.1864240742462,20.4561387170388,-215.089283969933));
#217777=CARTESIAN_POINT('Ctrl Pts',(62.1903704548995,20.4612501557837,-215.075710136272));
#217778=CARTESIAN_POINT('Ctrl Pts',(62.1944585031203,20.4666408209093,-215.061375901005));
#217779=CARTESIAN_POINT('Ctrl Pts',(62.1945458745928,20.4667560324539,-215.061069543747));
#217780=CARTESIAN_POINT('Ctrl Pts',(62.1946331997095,20.466871226232,-215.060763226167));
#217781=CARTESIAN_POINT('Ctrl Pts',(62.1947204784964,20.4669864022318,-215.0604569483));
#217782=CARTESIAN_POINT('Ctrl Pts',(62.2137408953005,20.4920863789936,-214.993710687232));
#217783=CARTESIAN_POINT('Ctrl Pts',(62.2305183466783,20.5163680122445,-214.928763782419));
#217784=CARTESIAN_POINT('Ctrl Pts',(62.2453129380165,20.5396752117267,-214.866095687917));
#217785=CARTESIAN_POINT('Ctrl Pts',(62.2602442721621,20.5631978339817,-214.802848367469));
#217786=CARTESIAN_POINT('Ctrl Pts',(62.2731565800729,20.5857280016135,-214.74192226384));
#217787=CARTESIAN_POINT('Ctrl Pts',(62.2843394053267,20.6071284880971,-214.683764654696));
#217788=CARTESIAN_POINT('Ctrl Pts',(62.2959819233376,20.6294086850662,-214.623216358844));
#217789=CARTESIAN_POINT('Ctrl Pts',(62.305750679233,20.6504644959011,-214.565668984582));
#217790=CARTESIAN_POINT('Ctrl Pts',(62.3139850117542,20.6701651459376,-214.511575895126));
#217791=CARTESIAN_POINT('Ctrl Pts',(62.3213517958911,20.6877901854663,-214.463181916342));
#217792=CARTESIAN_POINT('Ctrl Pts',(62.3274911569473,20.7043310817668,-214.417551780352));
#217793=CARTESIAN_POINT('Ctrl Pts',(62.332644851844,20.7197079144591,-214.374977598554));
#217794=CARTESIAN_POINT('Ctrl Pts',(62.3385799996162,20.7374163306779,-214.325947909116));
#217795=CARTESIAN_POINT('Ctrl Pts',(62.343548092569,20.7545910669149,-214.278189339776));
#217796=CARTESIAN_POINT('Ctrl Pts',(62.3476965833135,20.7713604195755,-214.231380372206));
#217797=CARTESIAN_POINT('Ctrl Pts',(62.3519241262657,20.7884493232321,-214.183679429109));
#217798=CARTESIAN_POINT('Ctrl Pts',(62.3553004212001,20.8051173944794,-214.136964144099));
#217799=CARTESIAN_POINT('Ctrl Pts',(62.3579284930835,20.8215000454921,-214.090879110919));
#217800=CARTESIAN_POINT('Ctrl Pts',(62.3605956251293,20.8381261864238,-214.044109131146));
#217801=CARTESIAN_POINT('Ctrl Pts',(62.3624920885415,20.8544585042312,-213.997987834824));
#217802=CARTESIAN_POINT('Ctrl Pts',(62.3636727291745,20.8706359516702,-213.95213530026));
#217803=CARTESIAN_POINT('Ctrl Pts',(62.364409404324,20.8807300676777,-213.923525051031));
#217804=CARTESIAN_POINT('Ctrl Pts',(62.364866354255,20.8907638289918,-213.895019299259));
#217805=CARTESIAN_POINT('Ctrl Pts',(62.3650466932196,20.9007701135701,-213.866525240701));
#217806=CARTESIAN_POINT('Ctrl Pts',(62.3685680730117,-46.7295395343351,
-213.857752904022));
#217807=CARTESIAN_POINT('Ctrl Pts',(62.3741929789703,-46.5883029740106,
-213.791721229881));
#217808=CARTESIAN_POINT('Ctrl Pts',(62.379769730669,-46.4460136161633,-213.728758447291));
#217809=CARTESIAN_POINT('Ctrl Pts',(62.3852759446209,-46.3032780419763,
-213.66896415876));
#217810=CARTESIAN_POINT('Ctrl Pts',(62.3975426120195,-45.9852937010517,
-213.535755268559));
#217811=CARTESIAN_POINT('Ctrl Pts',(62.4095164075117,-45.6637866135429,
-213.417460796858));
#217812=CARTESIAN_POINT('Ctrl Pts',(62.4212099409829,-45.3390922762075,
-213.312250040624));
#217813=CARTESIAN_POINT('Ctrl Pts',(62.4220692467669,-45.3152319329839,
-213.304518569927));
#217814=CARTESIAN_POINT('Ctrl Pts',(62.4229270386808,-45.2913543736635,
-213.296857775458));
#217815=CARTESIAN_POINT('Ctrl Pts',(62.423783321531,-45.2674597292971,-213.289266941104));
#217816=CARTESIAN_POINT('Ctrl Pts',(62.4306555056666,-45.0756908577114,
-213.228345936535));
#217817=CARTESIAN_POINT('Ctrl Pts',(62.4374306715992,-44.882827891531,-213.171905711604));
#217818=CARTESIAN_POINT('Ctrl Pts',(62.4441103360269,-44.688905615938,-213.119707758193));
#217819=CARTESIAN_POINT('Ctrl Pts',(62.4591991199772,-44.2508519754838,
-213.001797098131));
#217820=CARTESIAN_POINT('Ctrl Pts',(62.4737962270731,-43.807586665038,-212.90545317022));
#217821=CARTESIAN_POINT('Ctrl Pts',(62.487910617321,-43.3597345734855,-212.828052812568));
#217822=CARTESIAN_POINT('Ctrl Pts',(62.4903171662194,-43.2833743525594,
-212.814855802838));
#217823=CARTESIAN_POINT('Ctrl Pts',(62.4927096777594,-43.2068808554448,
-212.802209610105));
#217824=CARTESIAN_POINT('Ctrl Pts',(62.4950881915083,-43.1302572609202,
-212.790101352926));
#217825=CARTESIAN_POINT('Ctrl Pts',(62.5008761037459,-42.9438002178856,
-212.760636932155));
#217826=CARTESIAN_POINT('Ctrl Pts',(62.5065809373473,-42.7565658493193,
-212.734385263862));
#217827=CARTESIAN_POINT('Ctrl Pts',(62.5122027551557,-42.5685838171507,
-212.711227872825));
#217828=CARTESIAN_POINT('Ctrl Pts',(62.5175209296256,-42.3907549941012,
-212.68932124938));
#217829=CARTESIAN_POINT('Ctrl Pts',(62.5227648065833,-42.21226341704,-212.670174115219));
#217830=CARTESIAN_POINT('Ctrl Pts',(62.527934793664,-42.0331254267331,-212.653679770052));
#217831=CARTESIAN_POINT('Ctrl Pts',(62.5385750526626,-41.6644446962851,
-212.619733049905));
#217832=CARTESIAN_POINT('Ctrl Pts',(62.5489103696869,-41.2926330468725,
-212.597082683292));
#217833=CARTESIAN_POINT('Ctrl Pts',(62.5588215912844,-40.9225569182794,
-212.584979442347));
#217834=CARTESIAN_POINT('Ctrl Pts',(62.563546913138,-40.7461176367326,-212.579209042767));
#217835=CARTESIAN_POINT('Ctrl Pts',(62.5681836632464,-40.569818240452,-212.575793047685));
#217836=CARTESIAN_POINT('Ctrl Pts',(62.5727340550042,-40.3936434675018,
-212.574637782399));
#217837=CARTESIAN_POINT('Ctrl Pts',(62.5872728250113,-39.830754678735,-212.570946641683));
#217838=CARTESIAN_POINT('Ctrl Pts',(62.6009299850148,-39.2692127837649,
-212.590224636208));
#217839=CARTESIAN_POINT('Ctrl Pts',(62.6137680988129,-38.7088381795347,
-212.62950263278));
#217840=CARTESIAN_POINT('Ctrl Pts',(62.6174709897939,-38.5472096022638,
-212.640831566418));
#217841=CARTESIAN_POINT('Ctrl Pts',(62.621105625632,-38.3856786969335,-212.653829961871));
#217842=CARTESIAN_POINT('Ctrl Pts',(62.624672913913,-38.2242434316524,-212.668455765851));
#217843=CARTESIAN_POINT('Ctrl Pts',(62.6373436782581,-37.6508363946395,
-212.720405622716));
#217844=CARTESIAN_POINT('Ctrl Pts',(62.6491674651189,-37.0786070163394,
-212.792770228162));
#217845=CARTESIAN_POINT('Ctrl Pts',(62.6601855978898,-36.5075023878112,
-212.883581944354));
#217846=CARTESIAN_POINT('Ctrl Pts',(62.6630243100176,-36.3603629705465,
-212.906978678217));
#217847=CARTESIAN_POINT('Ctrl Pts',(62.6658095819956,-36.2132944881765,
-212.93160444825));
#217848=CARTESIAN_POINT('Ctrl Pts',(62.6685426178707,-36.0662511671652,
-212.957447775204));
#217849=CARTESIAN_POINT('Ctrl Pts',(62.6726066835548,-35.8475955247613,
-212.995877193271));
#217850=CARTESIAN_POINT('Ctrl Pts',(62.67655631062,-35.6289441133066,-213.037001059776));
#217851=CARTESIAN_POINT('Ctrl Pts',(62.6803946782102,-35.4101865945502,
-213.080774391982));
#217852=CARTESIAN_POINT('Ctrl Pts',(62.6828563633534,-35.2698894184096,
-213.108847826594));
#217853=CARTESIAN_POINT('Ctrl Pts',(62.6852717293958,-35.1295761809506,
-213.138007694812));
#217854=CARTESIAN_POINT('Ctrl Pts',(62.6876407845124,-34.9892589138444,
-213.16823854491));
#217855=CARTESIAN_POINT('Ctrl Pts',(62.6883605905984,-34.9466253667735,
-213.177423789158));
#217856=CARTESIAN_POINT('Ctrl Pts',(62.6890761418335,-34.9039903123139,
-213.186708083956));
#217857=CARTESIAN_POINT('Ctrl Pts',(62.6897874443054,-34.8613537452904,
-213.196091056993));
#217858=CARTESIAN_POINT('Ctrl Pts',(62.6905505729892,-34.8156106352106,
-213.206157682861));
#217859=CARTESIAN_POINT('Ctrl Pts',(62.6913088108168,-34.7698657837733,
-213.216337913904));
#217860=CARTESIAN_POINT('Ctrl Pts',(62.6920621645108,-34.7241191838738,
-213.2266313368));
#217861=CARTESIAN_POINT('Ctrl Pts',(62.6922505029487,-34.7126825330211,
-213.229204692721));
#217862=CARTESIAN_POINT('Ctrl Pts',(62.6924385015879,-34.701245742664,-213.231787136791));
#217863=CARTESIAN_POINT('Ctrl Pts',(62.692626268168,-34.6898089068763,-213.234372387596));
#217864=CARTESIAN_POINT('Ctrl Pts',(62.6928140347403,-34.678372071559,-213.236957638295));
#217865=CARTESIAN_POINT('Ctrl Pts',(62.6930017734619,-34.6669353695333,
-213.239533790651));
#217866=CARTESIAN_POINT('Ctrl Pts',(62.6931894847934,-34.6554988009795,
-213.242100818803));
#217867=CARTESIAN_POINT('Ctrl Pts',(62.6935649074065,-34.6326256669264,
-213.247234874423));
#217868=CARTESIAN_POINT('Ctrl Pts',(62.6939402204544,-34.6097530667514,
-213.252332433524));
#217869=CARTESIAN_POINT('Ctrl Pts',(62.6943154276501,-34.5868810019283,
-213.257393287646));
#217870=CARTESIAN_POINT('Ctrl Pts',(62.6950609186324,-34.5414369958777,
-213.267448588167));
#217871=CARTESIAN_POINT('Ctrl Pts',(62.6958059915227,-34.4959951029891,
-213.277359001683));
#217872=CARTESIAN_POINT('Ctrl Pts',(62.6965506762906,-34.450555335488,-213.287122844289));
#217873=CARTESIAN_POINT('Ctrl Pts',(62.6973051981913,-34.4045153179871,
-213.297015665251));
#217874=CARTESIAN_POINT('Ctrl Pts',(62.6980593192824,-34.3584776267158,
-213.306757986268));
#217875=CARTESIAN_POINT('Ctrl Pts',(62.6988130699628,-34.3124423208934,
-213.316348049998));
#217876=CARTESIAN_POINT('Ctrl Pts',(62.7009988974642,-34.1789429555056,
-213.344158605375));
#217877=CARTESIAN_POINT('Ctrl Pts',(62.7031812969115,-34.0454633873906,
-213.370706259287));
#217878=CARTESIAN_POINT('Ctrl Pts',(62.7053612372102,-33.9120052530642,
-213.395935334584));
#217879=CARTESIAN_POINT('Ctrl Pts',(62.7241253003464,-32.7632504637629,
-213.613097227511));
#217880=CARTESIAN_POINT('Ctrl Pts',(62.7427109763742,-31.6158487719858,
-213.732605809556));
#217881=CARTESIAN_POINT('Ctrl Pts',(62.7617431549812,-30.470412971391,-213.718959456451));
#217882=CARTESIAN_POINT('Ctrl Pts',(62.7647391511292,-30.2901014412562,
-213.716811282971));
#217883=CARTESIAN_POINT('Ctrl Pts',(62.767746212059,-30.1098386199596,-213.711363604099));
#217884=CARTESIAN_POINT('Ctrl Pts',(62.770766775426,-29.9296268901167,-213.702478069901));
#217885=CARTESIAN_POINT('Ctrl Pts',(62.7725414402335,-29.8237474974408,
-213.697257571961));
#217886=CARTESIAN_POINT('Ctrl Pts',(62.7743209052535,-29.7178858577718,
-213.690842589647));
#217887=CARTESIAN_POINT('Ctrl Pts',(62.7761057740119,-29.6120425444016,
-213.683199054815));
#217888=CARTESIAN_POINT('Ctrl Pts',(62.7866097971823,-28.989150462946,-213.638216550309));
#217889=CARTESIAN_POINT('Ctrl Pts',(62.7973012895257,-28.3668822616731,
-213.550676253015));
#217890=CARTESIAN_POINT('Ctrl Pts',(62.8083033340944,-27.7453414694754,
-213.413639151457));
#217891=CARTESIAN_POINT('Ctrl Pts',(62.8099338015368,-27.6532311331184,
-213.39333069596));
#217892=CARTESIAN_POINT('Ctrl Pts',(62.811571077252,-27.5611367494674,-213.371935988233));
#217893=CARTESIAN_POINT('Ctrl Pts',(62.8132156027367,-27.4690586781095,
-213.349430181196));
#217894=CARTESIAN_POINT('Ctrl Pts',(62.8148166574626,-27.3794145633349,
-213.32751928407));
#217895=CARTESIAN_POINT('Ctrl Pts',(62.8164245864001,-27.2897858690399,
-213.3045551313));
#217896=CARTESIAN_POINT('Ctrl Pts',(62.8180397952865,-27.2001730524583,
-213.280514793433));
#217897=CARTESIAN_POINT('Ctrl Pts',(62.818858360563,-27.1547585301625,-213.268331486382));
#217898=CARTESIAN_POINT('Ctrl Pts',(62.8196787972069,-27.1093480871571,
-213.25587168702));
#217899=CARTESIAN_POINT('Ctrl Pts',(62.8205011614668,-27.063941785938,-213.243132215583));
#217900=CARTESIAN_POINT('Ctrl Pts',(62.820603956966,-27.0582660001277,-213.24153978217));
#217901=CARTESIAN_POINT('Ctrl Pts',(62.8207068130079,-27.0525903054936,
-213.239941216059));
#217902=CARTESIAN_POINT('Ctrl Pts',(62.8208096296676,-27.046914615143,-213.238342307309));
#217903=CARTESIAN_POINT('Ctrl Pts',(62.8209124463233,-27.0412389250115,
-213.23674339862));
#217904=CARTESIAN_POINT('Ctrl Pts',(62.8210151618557,-27.03556318545,-213.23514772473));
#217905=CARTESIAN_POINT('Ctrl Pts',(62.821117776347,-27.0298873965556,-213.233555280696));
#217906=CARTESIAN_POINT('Ctrl Pts',(62.8213230053217,-27.0185358191961,
-213.230370392749));
#217907=CARTESIAN_POINT('Ctrl Pts',(62.8215278301309,-27.0071840445339,
-213.22719842432));
#217908=CARTESIAN_POINT('Ctrl Pts',(62.8217322514279,-26.9958320733607,
-213.224039336346));
#217909=CARTESIAN_POINT('Ctrl Pts',(62.8221023145259,-26.9752816430423,
-213.218320451379));
#217910=CARTESIAN_POINT('Ctrl Pts',(62.8224710552458,-26.9547305687673,
-213.212643777775));
#217911=CARTESIAN_POINT('Ctrl Pts',(62.8228384774045,-26.9341788553177,
-213.207009087125));
#217912=CARTESIAN_POINT('Ctrl Pts',(62.8228769801512,-26.9320252088913,
-213.206418619015));
#217913=CARTESIAN_POINT('Ctrl Pts',(62.8229154684173,-26.9298715555002,
-213.205828611962));
#217914=CARTESIAN_POINT('Ctrl Pts',(62.8229539422071,-26.9277178951481,
-213.205239065704));
#217915=CARTESIAN_POINT('Ctrl Pts',(62.8245764233091,-26.8368957212833,
-213.180377265789));
#217916=CARTESIAN_POINT('Ctrl Pts',(62.8261731614529,-26.7460611681055,
-213.156334842928));
#217917=CARTESIAN_POINT('Ctrl Pts',(62.8277444695764,-26.6552145055668,
-213.133093149396));
#217918=CARTESIAN_POINT('Ctrl Pts',(62.8292202126583,-26.5698930261205,
-213.111264987287));
#217919=CARTESIAN_POINT('Ctrl Pts',(62.8306735455578,-26.4845608838062,
-213.090141906316));
#217920=CARTESIAN_POINT('Ctrl Pts',(62.8321046858337,-26.3992182785356,
-213.069710892685));
#217921=CARTESIAN_POINT('Ctrl Pts',(62.8367688988909,-26.1210791607011,
-213.003124407662));
#217922=CARTESIAN_POINT('Ctrl Pts',(62.8411971255009,-25.8428597458081,
-212.943883039828));
#217923=CARTESIAN_POINT('Ctrl Pts',(62.8453976824702,-25.5644780440299,
-212.891551576529));
#217924=CARTESIAN_POINT('Ctrl Pts',(62.8465846366303,-25.4858155424996,
-212.876764240344));
#217925=CARTESIAN_POINT('Ctrl Pts',(62.8477534065636,-25.407149458358,-212.862521456414));
#217926=CARTESIAN_POINT('Ctrl Pts',(62.8489040944972,-25.3284786414785,
-212.848818315902));
#217927=CARTESIAN_POINT('Ctrl Pts',(62.8589719385763,-24.640155165815,-212.728923878815));
#217928=CARTESIAN_POINT('Ctrl Pts',(62.867653735289,-23.9520875862966,-212.650037662992));
#217929=CARTESIAN_POINT('Ctrl Pts',(62.8750146865603,-23.2647003090921,
-212.608425061389));
#217930=CARTESIAN_POINT('Ctrl Pts',(62.8823756378316,-22.5773130318876,
-212.566812459786));
#217931=CARTESIAN_POINT('Ctrl Pts',(62.8884156923502,-21.8906064258735,
-212.562474309897));
#217932=CARTESIAN_POINT('Ctrl Pts',(62.8931986251439,-21.2050511218171,
-212.591707581156));
#217933=CARTESIAN_POINT('Ctrl Pts',(62.8935577382081,-21.1535781288824,
-212.593902479154));
#217934=CARTESIAN_POINT('Ctrl Pts',(62.8939097569274,-21.1021052395343,
-212.596289051621));
#217935=CARTESIAN_POINT('Ctrl Pts',(62.8942546885952,-21.0506330432678,
-212.598866899388));
#217936=CARTESIAN_POINT('Ctrl Pts',(62.8968212608728,-20.6676380203924,
-212.618048184355));
#217937=CARTESIAN_POINT('Ctrl Pts',(62.898993894224,-20.2848774438081,-212.647828821471));
#217938=CARTESIAN_POINT('Ctrl Pts',(62.900778786722,-19.9023518511915,-212.687972680865));
#217939=CARTESIAN_POINT('Ctrl Pts',(62.9023087147126,-19.5744684565815,
-212.722382156061));
#217940=CARTESIAN_POINT('Ctrl Pts',(62.9035537360166,-19.2467573919566,
-212.764406500889));
#217941=CARTESIAN_POINT('Ctrl Pts',(62.9045166573415,-18.9192122497013,
-212.81392668013));
#217942=CARTESIAN_POINT('Ctrl Pts',(62.9053466520591,-18.6368831218555,
-212.856610839387));
#217943=CARTESIAN_POINT('Ctrl Pts',(62.9059670124065,-18.3545500700666,
-212.904900139622));
#217944=CARTESIAN_POINT('Ctrl Pts',(62.9063776080623,-18.0726457860283,
-212.958691242021));
#217945=CARTESIAN_POINT('Ctrl Pts',(62.9064830589281,-18.0002459678496,
-212.972506094273));
#217946=CARTESIAN_POINT('Ctrl Pts',(62.9065746841136,-17.9278744301198,
-212.986683569855));
#217947=CARTESIAN_POINT('Ctrl Pts',(62.9066525023395,-17.8555384962728,
-213.00122136616));
#217948=CARTESIAN_POINT('Ctrl Pts',(62.9070069220114,-17.5260876814359,
-213.06743311714));
#217949=CARTESIAN_POINT('Ctrl Pts',(62.9070749640207,-17.197340288906,-213.141130341411));
#217950=CARTESIAN_POINT('Ctrl Pts',(62.9068586171446,-16.8692921444043,
-213.222255473336));
#217951=CARTESIAN_POINT('Ctrl Pts',(62.9068512161578,-16.8580699810933,
-213.225030674155));
#217952=CARTESIAN_POINT('Ctrl Pts',(62.9068434310689,-16.8468489287218,
-213.227817504345));
#217953=CARTESIAN_POINT('Ctrl Pts',(62.9068354227292,-16.8356281229708,
-213.230606932774));
#217954=CARTESIAN_POINT('Ctrl Pts',(62.9068274143987,-16.8244073300739,
-213.233396358007));
#217955=CARTESIAN_POINT('Ctrl Pts',(62.9068194222443,-16.81318550769,-213.236174929377));
#217956=CARTESIAN_POINT('Ctrl Pts',(62.9068114465212,-16.8019626469682,
-213.238942628495));
#217957=CARTESIAN_POINT('Ctrl Pts',(62.9068100308831,-16.7999706633578,
-213.239433876798));
#217958=CARTESIAN_POINT('Ctrl Pts',(62.9068086157626,-16.7979786470357,
-213.239924782582));
#217959=CARTESIAN_POINT('Ctrl Pts',(62.9068072011611,-16.7959865979526,
-213.240415345746));
#217960=CARTESIAN_POINT('Ctrl Pts',(62.9067926759976,-16.7755321875305,
-213.245452460734));
#217961=CARTESIAN_POINT('Ctrl Pts',(62.9067782084953,-16.755074364096,-213.250453275771));
#217962=CARTESIAN_POINT('Ctrl Pts',(62.9067638003454,-16.7346131155667,
-213.255417662646));
#217963=CARTESIAN_POINT('Ctrl Pts',(62.9067321774736,-16.6897049597551,
-213.266313452264));
#217964=CARTESIAN_POINT('Ctrl Pts',(62.9067008405294,-16.6447803048274,
-213.277033762557));
#217965=CARTESIAN_POINT('Ctrl Pts',(62.9066698070808,-16.5998390244792,
-213.287577252305));
#217966=CARTESIAN_POINT('Ctrl Pts',(62.9066077395427,-16.5099555355157,
-213.308664449577));
#217967=CARTESIAN_POINT('Ctrl Pts',(62.9065468864317,-16.4200055414544,
-213.329044330242));
#217968=CARTESIAN_POINT('Ctrl Pts',(62.9064873833149,-16.3299880540902,
-213.348706398678));
#217969=CARTESIAN_POINT('Ctrl Pts',(62.9063683745862,-16.14994930492,-213.388031359981));
#217970=CARTESIAN_POINT('Ctrl Pts',(62.9062547727652,-15.9696405404371,
-213.424484631683));
#217971=CARTESIAN_POINT('Ctrl Pts',(62.9061475795573,-15.7890542301196,
-213.457986204279));
#217972=CARTESIAN_POINT('Ctrl Pts',(62.9059331838863,-15.4278660176251,
-213.524992242004));
#217973=CARTESIAN_POINT('Ctrl Pts',(62.9057445834295,-15.0655667619647,
-213.58018242881));
#217974=CARTESIAN_POINT('Ctrl Pts',(62.905589362047,-14.7020974635233,-213.622929699831));
#217975=CARTESIAN_POINT('Ctrl Pts',(62.9052798509934,-13.9773405794218,
-213.708167652755));
#217976=CARTESIAN_POINT('Ctrl Pts',(62.9051047269462,-13.2479237446018,
-213.743849925036));
#217977=CARTESIAN_POINT('Ctrl Pts',(62.9051090261727,-12.5134449350678,
-213.725695782834));
#217978=CARTESIAN_POINT('Ctrl Pts',(62.9051090395082,-12.5111666950214,
-213.725639471484));
#217979=CARTESIAN_POINT('Ctrl Pts',(62.9051090545696,-12.5088884062743,
-213.725582642177));
#217980=CARTESIAN_POINT('Ctrl Pts',(62.9051090713583,-12.5066100688143,
-213.725525294786));
#217981=CARTESIAN_POINT('Ctrl Pts',(62.9051117186635,-12.1473516978959,
-213.716482503419));
#217982=CARTESIAN_POINT('Ctrl Pts',(62.9051569926989,-11.7868835043618,
-213.694572753784));
#217983=CARTESIAN_POINT('Ctrl Pts',(62.9052478305722,-11.4251692471516,
-213.659411822611));
#217984=CARTESIAN_POINT('Ctrl Pts',(62.9052501495695,-11.4159350548302,
-213.658514200263));
#217985=CARTESIAN_POINT('Ctrl Pts',(62.905252498141,-11.4066999814362,-213.657607942971));
#217986=CARTESIAN_POINT('Ctrl Pts',(62.9052548763439,-11.3974640308012,
-213.656693043944));
#217987=CARTESIAN_POINT('Ctrl Pts',(62.9053396597116,-11.0682006948942,
-213.624076725649));
#217988=CARTESIAN_POINT('Ctrl Pts',(62.9054625664031,-10.7375855896784,
-213.580337710379));
#217989=CARTESIAN_POINT('Ctrl Pts',(62.9056218033686,-10.409778663214,-213.526208718247));
#217990=CARTESIAN_POINT('Ctrl Pts',(62.9056341733888,-10.3843136067658,
-213.522003810635));
#217991=CARTESIAN_POINT('Ctrl Pts',(62.905646762572,-10.358865493353,-213.517736228733));
#217992=CARTESIAN_POINT('Ctrl Pts',(62.9056595700396,-10.3334362698611,
-213.513406328741));
#217993=CARTESIAN_POINT('Ctrl Pts',(62.9056676765601,-10.317340775653,-213.510665707099));
#217994=CARTESIAN_POINT('Ctrl Pts',(62.9056758700813,-10.3012520481916,
-213.507900031565));
#217995=CARTESIAN_POINT('Ctrl Pts',(62.9056841503679,-10.2851705845394,
-213.505109387712));
#217996=CARTESIAN_POINT('Ctrl Pts',(62.9058495001971,-9.96403831223543,
-213.449382756036));
#217997=CARTESIAN_POINT('Ctrl Pts',(62.9060495440864,-9.64477667567345,
-213.383630454476));
#217998=CARTESIAN_POINT('Ctrl Pts',(62.9062818494613,-9.32750692224311,
-213.308308849075));
#217999=CARTESIAN_POINT('Ctrl Pts',(62.9062995203884,-9.30337295346862,
-213.302579310558));
#218000=CARTESIAN_POINT('Ctrl Pts',(62.9063173779087,-9.27925050600009,
-213.296794425732));
#218001=CARTESIAN_POINT('Ctrl Pts',(62.9063354209129,-9.25513963110861,
-213.290954407383));
#218002=CARTESIAN_POINT('Ctrl Pts',(62.9063523663721,-9.23249540595939,
-213.28546963377));
#218003=CARTESIAN_POINT('Ctrl Pts',(62.9063694755794,-9.20986097578642,
-213.279936139709));
#218004=CARTESIAN_POINT('Ctrl Pts',(62.9063867476374,-9.18723633851541,
-213.274354087607));
#218005=CARTESIAN_POINT('Ctrl Pts',(62.9064214242477,-9.14181351020547,
-213.263147163439));
#218006=CARTESIAN_POINT('Ctrl Pts',(62.9064567545313,-9.09643013343645,
-213.251744618045));
#218007=CARTESIAN_POINT('Ctrl Pts',(62.9064927284741,-9.05108616789961,
-213.240147881952));
#218008=CARTESIAN_POINT('Ctrl Pts',(62.9065017219161,-9.03975023169194,
-213.23724871204));
#218009=CARTESIAN_POINT('Ctrl Pts',(62.9065107555831,-9.02841675862816,
-213.234337405481));
#218010=CARTESIAN_POINT('Ctrl Pts',(62.9065198293118,-9.01708574800015,
-213.231413985003));
#218011=CARTESIAN_POINT('Ctrl Pts',(62.9065289030347,-9.00575474452809,
-213.228490566372));
#218012=CARTESIAN_POINT('Ctrl Pts',(62.9065377477119,-8.99442319446877,
-213.225569813864));
#218013=CARTESIAN_POINT('Ctrl Pts',(62.9065461779452,-8.98308903056771,
-213.222661899751));
#218014=CARTESIAN_POINT('Ctrl Pts',(62.9065630384181,-8.96042069442155,
-213.216846069384));
#218015=CARTESIAN_POINT('Ctrl Pts',(62.9065784765558,-8.93774453557201,
-213.211068662567));
#218016=CARTESIAN_POINT('Ctrl Pts',(62.9065924909309,-8.91506058486269,
-213.205329682185));
#218017=CARTESIAN_POINT('Ctrl Pts',(62.906632507978,-8.85028818379569,-213.188942433607));
#218018=CARTESIAN_POINT('Ctrl Pts',(62.9066609166417,-8.7854522548987,-213.172868479925));
#218019=CARTESIAN_POINT('Ctrl Pts',(62.9066776826504,-8.72055350098855,
-213.157107960246));
#218020=CARTESIAN_POINT('Ctrl Pts',(62.9066844034019,-8.69453846021989,
-213.1507902648));
#218021=CARTESIAN_POINT('Ctrl Pts',(62.9066892533842,-8.66851311367876,
-213.144522883906));
#218022=CARTESIAN_POINT('Ctrl Pts',(62.9066922303343,-8.64247748890024,
-213.13830582419));
#218023=CARTESIAN_POINT('Ctrl Pts',(62.9067096741274,-8.48991865034706,
-213.101876223688));
#218024=CARTESIAN_POINT('Ctrl Pts',(62.9066627545095,-8.33741593724109,
-213.067272060264));
#218025=CARTESIAN_POINT('Ctrl Pts',(62.906552054195,-8.18500124845787,-213.034473300197));
#218026=CARTESIAN_POINT('Ctrl Pts',(62.9065307100423,-8.15561413774858,
-213.02814936383));
#218027=CARTESIAN_POINT('Ctrl Pts',(62.906506993431,-8.12623007030402,-213.021892565579));
#218028=CARTESIAN_POINT('Ctrl Pts',(62.9064809085264,-8.09684923724608,
-213.015702751583));
#218029=CARTESIAN_POINT('Ctrl Pts',(62.9056899601275,-7.20596145140312,
-212.828014755284));
#218030=CARTESIAN_POINT('Ctrl Pts',(62.9027366747181,-6.31764267914539,
-212.700961335132));
#218031=CARTESIAN_POINT('Ctrl Pts',(62.8976715771841,-5.43185195165195,
-212.632707606633));
#218032=CARTESIAN_POINT('Ctrl Pts',(62.8947900085006,-4.92791953904146,
-212.593877592946));
#218033=CARTESIAN_POINT('Ctrl Pts',(62.8912249487153,-4.42480439538323,
-212.574078170132));
#218034=CARTESIAN_POINT('Ctrl Pts',(62.8869856905768,-3.92249156539548,
-212.572970530223));
#218035=CARTESIAN_POINT('Ctrl Pts',(62.8865147226824,-3.8666862314995,-212.572847475005));
#218036=CARTESIAN_POINT('Ctrl Pts',(62.8860354164368,-3.81089071961118,
-212.572956060008));
#218037=CARTESIAN_POINT('Ctrl Pts',(62.885547785291,-3.75510503118202,-212.573295788909));
#218038=CARTESIAN_POINT('Ctrl Pts',(62.8793243758262,-3.04313824163497,
-212.577631590838));
#218039=CARTESIAN_POINT('Ctrl Pts',(62.8717459291031,-2.332772344863,-212.619539913621));
#218040=CARTESIAN_POINT('Ctrl Pts',(62.862782948286,-1.62412895620658,-212.701365863942));
#218041=CARTESIAN_POINT('Ctrl Pts',(62.8546488502804,-0.981019828565715,
-212.775624675034));
#218042=CARTESIAN_POINT('Ctrl Pts',(62.8453744839341,-0.339328956701179,
-212.882759122652));
#218043=CARTESIAN_POINT('Ctrl Pts',(62.8349373318117,0.300889820690812,
-213.0245235881));
#218044=CARTESIAN_POINT('Ctrl Pts',(62.833607314137,0.382473597531864,-213.0425887885));
#218045=CARTESIAN_POINT('Ctrl Pts',(62.8322582595392,0.464033344884034,
-213.0612252722));
#218046=CARTESIAN_POINT('Ctrl Pts',(62.8308901810048,0.545568613619925,
-213.080433504715));
#218047=CARTESIAN_POINT('Ctrl Pts',(62.8293216865052,0.639048349845703,
-213.102455637427));
#218048=CARTESIAN_POINT('Ctrl Pts',(62.8277279878957,0.732495388150152,
-213.125241286057));
#218049=CARTESIAN_POINT('Ctrl Pts',(62.8261090055383,0.825909081274457,
-213.148796974995));
#218050=CARTESIAN_POINT('Ctrl Pts',(62.8246401331402,0.910661577070946,
-213.170168610789));
#218051=CARTESIAN_POINT('Ctrl Pts',(62.8231504392874,0.995387120789026,
-213.19217425345));
#218052=CARTESIAN_POINT('Ctrl Pts',(62.8216398034464,1.08008493804852,-213.214822482474));
#218053=CARTESIAN_POINT('Ctrl Pts',(62.8212428495944,1.10234121180029,-213.220773818665));
#218054=CARTESIAN_POINT('Ctrl Pts',(62.8208444494793,1.12459557041626,-213.226769539353));
#218055=CARTESIAN_POINT('Ctrl Pts',(62.8204446007168,1.1468479993255,-213.232809812552));
#218056=CARTESIAN_POINT('Ctrl Pts',(62.8202446762942,1.15797421608229,-213.235829949777));
#218057=CARTESIAN_POINT('Ctrl Pts',(62.8200446532189,1.16910062229262,-213.238845621166));
#218058=CARTESIAN_POINT('Ctrl Pts',(62.8198447802284,1.18022785110113,-213.241842094699));
#218059=CARTESIAN_POINT('Ctrl Pts',(62.8196449071674,1.19135508383185,-213.244838569288));
#218060=CARTESIAN_POINT('Ctrl Pts',(62.8194451061373,1.20248294022609,-213.247820468069));
#218061=CARTESIAN_POINT('Ctrl Pts',(62.8192453767934,1.21361141859933,-213.250787808692));
#218062=CARTESIAN_POINT('Ctrl Pts',(62.8184464580711,1.25812540713238,-213.262657191193));
#218063=CARTESIAN_POINT('Ctrl Pts',(62.8176486863074,1.30264934735082,-213.27429364379));
#218064=CARTESIAN_POINT('Ctrl Pts',(62.8168520397832,1.34718313255599,-213.285698279349));
#218065=CARTESIAN_POINT('Ctrl Pts',(62.8168331493297,1.34823913841709,-213.28596871138));
#218066=CARTESIAN_POINT('Ctrl Pts',(62.8168142595089,1.3492951498137,-213.286239013068));
#218067=CARTESIAN_POINT('Ctrl Pts',(62.8167953703204,1.35035116674446,-213.286509184428));
#218068=CARTESIAN_POINT('Ctrl Pts',(62.8152210633643,1.43836420129823,-213.309026438185));
#218069=CARTESIAN_POINT('Ctrl Pts',(62.8136511488776,1.52641572030258,-213.330638365248));
#218070=CARTESIAN_POINT('Ctrl Pts',(62.8120854563785,1.61450537353353,-213.351353373465));
#218071=CARTESIAN_POINT('Ctrl Pts',(62.8074297466584,1.87644688185748,-213.412951078738));
#218072=CARTESIAN_POINT('Ctrl Pts',(62.8028113125304,2.13872544174159,-213.466621196677));
#218073=CARTESIAN_POINT('Ctrl Pts',(62.7982260322374,2.40133274732117,-213.512564584869));
#218074=CARTESIAN_POINT('Ctrl Pts',(62.7965691479007,2.4962255136348,-213.529166161088));
#218075=CARTESIAN_POINT('Ctrl Pts',(62.7949165988104,2.59116092814633,-213.544758707681));
#218076=CARTESIAN_POINT('Ctrl Pts',(62.7932681861794,2.6861388388309,-213.559351754428));
#218077=CARTESIAN_POINT('Ctrl Pts',(62.7870578081227,3.04396716487127,-213.614330911704));
#218078=CARTESIAN_POINT('Ctrl Pts',(62.7808961247407,3.40303459047103,-213.655110348135));
#218079=CARTESIAN_POINT('Ctrl Pts',(62.7748157638915,3.76060806585576,-213.682219323134));
#218080=CARTESIAN_POINT('Ctrl Pts',(62.7705733532611,4.0100954812797,-213.701133891952));
#218081=CARTESIAN_POINT('Ctrl Pts',(62.7663688307482,4.25893819616771,-213.71344333557));
#218082=CARTESIAN_POINT('Ctrl Pts',(62.7621968858992,4.50717455612251,-213.719490676919));
#218083=CARTESIAN_POINT('Ctrl Pts',(62.760389727327,4.61470293486154,-213.722110199743));
#218084=CARTESIAN_POINT('Ctrl Pts',(62.758588694089,4.72211697151828,-213.723554528345));
#218085=CARTESIAN_POINT('Ctrl Pts',(62.756793361705,4.8294193693953,-213.723851522448));
#218086=CARTESIAN_POINT('Ctrl Pts',(62.744914568547,5.53938427675417,-213.725816580036));
#218087=CARTESIAN_POINT('Ctrl Pts',(62.7332829196987,6.24447623948652,-213.677701667471));
#218088=CARTESIAN_POINT('Ctrl Pts',(62.7217741472389,6.94546014142257,-213.587382621443));
#218089=CARTESIAN_POINT('Ctrl Pts',(62.7160202469305,7.29592249555947,-213.542226911865));
#218090=CARTESIAN_POINT('Ctrl Pts',(62.7102974318193,7.64535562408464,-213.486497387274));
#218091=CARTESIAN_POINT('Ctrl Pts',(62.7045905440092,7.99385039894293,-213.421128855621));
#218092=CARTESIAN_POINT('Ctrl Pts',(62.7017372091522,8.16809112729064,-213.388445838864));
#218093=CARTESIAN_POINT('Ctrl Pts',(62.6988879008502,8.34209702777281,-213.353350616144));
#218094=CARTESIAN_POINT('Ctrl Pts',(62.6960409729441,8.51587804140931,-213.31594549485));
#218095=CARTESIAN_POINT('Ctrl Pts',(62.6953306860554,8.55923508435001,-213.306613201199));
#218096=CARTESIAN_POINT('Ctrl Pts',(62.6946205479401,8.6025781254609,-213.297137089371));
#218097=CARTESIAN_POINT('Ctrl Pts',(62.693910534767,8.64590730924635,-213.287518647044));
#218098=CARTESIAN_POINT('Ctrl Pts',(62.6931976571302,8.68941129946275,-213.277861400257));
#218099=CARTESIAN_POINT('Ctrl Pts',(62.6924849069969,8.73290123523708,-213.268060682277));
#218100=CARTESIAN_POINT('Ctrl Pts',(62.6917722569378,8.77637732701844,-213.258118114802));
#218101=CARTESIAN_POINT('Ctrl Pts',(62.6914166494633,8.79807159758174,-213.253156842064));
#218102=CARTESIAN_POINT('Ctrl Pts',(62.6910610669504,8.81976242088063,-213.248160247012));
#218103=CARTESIAN_POINT('Ctrl Pts',(62.6907055060663,8.84144982288392,-213.243128526156));
#218104=CARTESIAN_POINT('Ctrl Pts',(62.69034994597,8.86313717683587,-213.238096816449));
#218105=CARTESIAN_POINT('Ctrl Pts',(62.6899947488889,8.88481939248927,-213.233012444835));
#218106=CARTESIAN_POINT('Ctrl Pts',(62.6896387405559,8.90650238461306,-213.227935756798));
#218107=CARTESIAN_POINT('Ctrl Pts',(62.6889267268058,8.94986819125055,-213.217782422308));
#218108=CARTESIAN_POINT('Ctrl Pts',(62.6882099166076,8.99324491620445,-213.20773948302));
#218109=CARTESIAN_POINT('Ctrl Pts',(62.6874882954834,9.03663265289044,-213.197807426414));
#218110=CARTESIAN_POINT('Ctrl Pts',(62.6868204901171,9.0767846972564,-213.1886160648));
#218111=CARTESIAN_POINT('Ctrl Pts',(62.6861485996542,9.11694554599575,-213.179518348821));
#218112=CARTESIAN_POINT('Ctrl Pts',(62.6854726096978,9.15711522005327,-213.170514913905));
#218113=CARTESIAN_POINT('Ctrl Pts',(62.6826037415343,9.3275933432039,-213.132304778465));
#218114=CARTESIAN_POINT('Ctrl Pts',(62.6796606062759,9.49823764842399,-213.0958088569));
#218115=CARTESIAN_POINT('Ctrl Pts',(62.6766425417446,9.66904980342632,-213.061049681902));
#218116=CARTESIAN_POINT('Ctrl Pts',(62.6706064126818,10.010674113431,-212.991531331906));
#218117=CARTESIAN_POINT('Ctrl Pts',(62.664270812359,10.3529550669585,-212.928960848345));
#218118=CARTESIAN_POINT('Ctrl Pts',(62.6576327768096,10.6957266313347,-212.873621170708));
#218119=CARTESIAN_POINT('Ctrl Pts',(62.6473143570134,11.2285440393083,-212.787599030422));
#218120=CARTESIAN_POINT('Ctrl Pts',(62.6362643202696,11.7626593744765,-212.718966127623));
#218121=CARTESIAN_POINT('Ctrl Pts',(62.6244492722701,12.298183791666,-212.669131165341));
#218122=CARTESIAN_POINT('Ctrl Pts',(62.6210626304398,12.4516854441756,-212.654846570993));
#218123=CARTESIAN_POINT('Ctrl Pts',(62.6176131332116,12.6053025653798,-212.642106558566));
#218124=CARTESIAN_POINT('Ctrl Pts',(62.6140999935327,12.7590370278545,-212.630944584506));
#218125=CARTESIAN_POINT('Ctrl Pts',(62.6105014211192,12.9165100139116,-212.619511172914));
#218126=CARTESIAN_POINT('Ctrl Pts',(62.6068362958068,13.0740938080762,-212.609737755954));
#218127=CARTESIAN_POINT('Ctrl Pts',(62.6031038882692,13.2317919256033,-212.60165208257));
#218128=CARTESIAN_POINT('Ctrl Pts',(62.5920978381641,13.696809040022,-212.577809207562));
#218129=CARTESIAN_POINT('Ctrl Pts',(62.5804979949266,14.1630945001764,-212.568752968163));
#218130=CARTESIAN_POINT('Ctrl Pts',(62.5682752553844,14.6305393352631,-212.5760493123));
#218131=CARTESIAN_POINT('Ctrl Pts',(62.5664789095161,14.699238549155,-212.577121637993));
#218132=CARTESIAN_POINT('Ctrl Pts',(62.564669105666,14.7679628448817,-212.578547253472));
#218133=CARTESIAN_POINT('Ctrl Pts',(62.5628457474452,14.8367119180636,-212.580331218975));
#218134=CARTESIAN_POINT('Ctrl Pts',(62.5582940634694,15.0083315434169,-212.584784566155));
#218135=CARTESIAN_POINT('Ctrl Pts',(62.5536582189233,15.1800866651588,-212.591481763735));
#218136=CARTESIAN_POINT('Ctrl Pts',(62.5489369347187,15.3519656949738,-212.600500512767));
#218137=CARTESIAN_POINT('Ctrl Pts',(62.5345339878629,15.8763070446592,-212.628013485379));
#218138=CARTESIAN_POINT('Ctrl Pts',(62.5194888785073,16.3962308632545,-212.676843393471));
#218139=CARTESIAN_POINT('Ctrl Pts',(62.5037997387388,16.9113773860641,-212.748829194443));
#218140=CARTESIAN_POINT('Ctrl Pts',(62.4982710429057,17.0929098649717,-212.774196270252));
#218141=CARTESIAN_POINT('Ctrl Pts',(62.4926620464245,17.2738497478371,-212.802456316523));
#218142=CARTESIAN_POINT('Ctrl Pts',(62.4869727360513,17.4541800510743,-212.833687547545));
#218143=CARTESIAN_POINT('Ctrl Pts',(62.471224815544,17.953331458564,-212.920135097635));
#218144=CARTESIAN_POINT('Ctrl Pts',(62.4548621630433,18.4478214139081,-213.029285839066));
#218145=CARTESIAN_POINT('Ctrl Pts',(62.4378715929549,18.937051788145,-213.164110067595));
#218146=CARTESIAN_POINT('Ctrl Pts',(62.4313084944047,19.126031153945,-213.216189820905));
#218147=CARTESIAN_POINT('Ctrl Pts',(62.4246524255105,19.3141920754888,-213.27211651907));
#218148=CARTESIAN_POINT('Ctrl Pts',(62.4179027766836,19.5014992838758,-213.332056784808));
#218149=CARTESIAN_POINT('Ctrl Pts',(62.4127593088452,19.6442339100702,-213.377733358058));
#218150=CARTESIAN_POINT('Ctrl Pts',(62.407553332654,19.7866395914419,-213.425870497296));
#218151=CARTESIAN_POINT('Ctrl Pts',(62.4022963811677,19.9284129896787,-213.476422874377));
#218152=CARTESIAN_POINT('Ctrl Pts',(62.3923400029788,20.1969240409302,-213.572166307785));
#218153=CARTESIAN_POINT('Ctrl Pts',(62.3821761384627,20.4638252083206,-213.676819485766));
#218154=CARTESIAN_POINT('Ctrl Pts',(62.3718829557378,20.7269505827977,-213.790195793082));
#218155=CARTESIAN_POINT('Ctrl Pts',(62.3696094190776,20.7850691648823,-213.815238114585));
#218156=CARTESIAN_POINT('Ctrl Pts',(62.3673295818174,20.8430033464101,-213.840705944543));
#218157=CARTESIAN_POINT('Ctrl Pts',(62.3650443003753,20.9007294710424,-213.866597158579));
#218158=CARTESIAN_POINT('',(61.6307906445947,-35.3347454921122,-216.138336328427));
#218159=CARTESIAN_POINT('Ctrl Pts',(61.6307906445947,-35.3347454921122,
-216.138336328427));
#218160=CARTESIAN_POINT('Ctrl Pts',(61.6308040666128,-35.3417600414872,
-216.136573459783));
#218161=CARTESIAN_POINT('Ctrl Pts',(61.6308188619637,-35.3487748507191,
-216.134811634988));
#218162=CARTESIAN_POINT('Ctrl Pts',(61.6310464376898,-35.3557090446008,
-216.132792415564));
#218163=CARTESIAN_POINT('Ctrl Pts',(61.6312601624137,-35.3622212007881,
-216.130896092432));
#218164=CARTESIAN_POINT('Ctrl Pts',(61.6316614890751,-35.3686622440919,
-216.128772703321));
#218165=CARTESIAN_POINT('Ctrl Pts',(61.6319689130928,-35.375140928003,-216.1267658518));
#218166=CARTESIAN_POINT('Ctrl Pts',(61.6326034322233,-35.3885128464071,
-216.122623736647));
#218167=CARTESIAN_POINT('Ctrl Pts',(61.632838216593,-35.4020451702368,-216.118978299824));
#218168=CARTESIAN_POINT('Ctrl Pts',(61.6331431613905,-35.4155525532659,
-216.115257033341));
#218169=CARTESIAN_POINT('Ctrl Pts',(61.633753020954,-35.4425659890872,-216.107814866852));
#218170=CARTESIAN_POINT('Ctrl Pts',(61.6346427632318,-35.4694795358603,
-216.100068857125));
#218171=CARTESIAN_POINT('Ctrl Pts',(61.6354796087042,-35.4964244671033,
-216.092424963586));
#218172=CARTESIAN_POINT('Ctrl Pts',(61.6371531603808,-35.5503098454024,
-216.077138448608));
#218173=CARTESIAN_POINT('Ctrl Pts',(61.6386161988779,-35.6043209298415,
-216.062261116095));
#218174=CARTESIAN_POINT('Ctrl Pts',(61.6401043809673,-35.658364025579,-216.047507238149));
#218175=CARTESIAN_POINT('Ctrl Pts',(61.6430804365425,-35.766439010163,-216.018002541761));
#218176=CARTESIAN_POINT('Ctrl Pts',(61.646155530417,-35.8746417481196,-215.98899042091));
#218177=CARTESIAN_POINT('Ctrl Pts',(61.649162113972,-35.9830350128333,-215.960691861929));
#218178=CARTESIAN_POINT('Ctrl Pts',(61.6551756296919,-36.1998341103363,
-215.904091462781));
#218179=CARTESIAN_POINT('Ctrl Pts',(61.6609168613943,-36.4173956880617,
-215.850346973261));
#218180=CARTESIAN_POINT('Ctrl Pts',(61.6665143671927,-36.6356225549127,
-215.799441647033));
#218181=CARTESIAN_POINT('Ctrl Pts',(61.6721571209959,-36.855613480733,-215.748124822448));
#218182=CARTESIAN_POINT('Ctrl Pts',(61.6776529206739,-37.0762803739165,
-215.699692593711));
#218183=CARTESIAN_POINT('Ctrl Pts',(61.682966870277,-37.2975828727595,-215.654351989951));
#218184=CARTESIAN_POINT('Ctrl Pts',(61.6881722529671,-37.5143640398369,
-215.609937719663));
#218185=CARTESIAN_POINT('Ctrl Pts',(61.6932031661431,-37.7317551162009,
-215.568490060376));
#218186=CARTESIAN_POINT('Ctrl Pts',(61.6980595479273,-37.9497193529901,
-215.530178847675));
#218187=CARTESIAN_POINT('Ctrl Pts',(61.7021486633458,-38.1332471234445,
-215.497920475596));
#218188=CARTESIAN_POINT('Ctrl Pts',(61.7061154994121,-38.3171775092552,
-215.467884589685));
#218189=CARTESIAN_POINT('Ctrl Pts',(61.7099526889049,-38.5014704241579,
-215.440197130652));
#218190=CARTESIAN_POINT('Ctrl Pts',(61.7155196281875,-38.7688399323387,
-215.400028563628));
#218191=CARTESIAN_POINT('Ctrl Pts',(61.7208119697472,-39.0369744580731,
-215.364802915884));
#218192=CARTESIAN_POINT('Ctrl Pts',(61.7258355244156,-39.305719263793,-215.334904757817));
#218193=CARTESIAN_POINT('Ctrl Pts',(61.7303410289492,-39.5467499722198,
-215.30808982385));
#218194=CARTESIAN_POINT('Ctrl Pts',(61.7346309998384,-39.7882688950653,
-215.285559347836));
#218195=CARTESIAN_POINT('Ctrl Pts',(61.7386614013115,-40.0301288296822,
-215.267705907674));
#218196=CARTESIAN_POINT('Ctrl Pts',(61.7418669752936,-40.2224917788592,
-215.253506199865));
#218197=CARTESIAN_POINT('Ctrl Pts',(61.7449089826414,-40.4150698378095,
-215.242265088223));
#218198=CARTESIAN_POINT('Ctrl Pts',(61.7477803186499,-40.6077707354279,
-215.234180086954));
#218199=CARTESIAN_POINT('Ctrl Pts',(61.7510847334047,-40.8295363830086,
-215.224875638639));
#218200=CARTESIAN_POINT('Ctrl Pts',(61.7541605291425,-41.0514720876124,
-215.21975341874));
#218201=CARTESIAN_POINT('Ctrl Pts',(61.7569816337569,-41.2734309002291,
-215.219176498584));
#218202=CARTESIAN_POINT('Ctrl Pts',(61.7577170450897,-41.3312915784105,
-215.219026105855));
#218203=CARTESIAN_POINT('Ctrl Pts',(61.7584352929738,-41.3891536203518,
-215.219184613554));
#218204=CARTESIAN_POINT('Ctrl Pts',(61.7591360681483,-41.4470135072824,
-215.21965872786));
#218205=CARTESIAN_POINT('Ctrl Pts',(61.7610546287376,-41.6054205154189,
-215.220956743338));
#218206=CARTESIAN_POINT('Ctrl Pts',(61.7628416990792,-41.7638121989732,
-215.224620350087));
#218207=CARTESIAN_POINT('Ctrl Pts',(61.7644946995693,-41.9221090036954,
-215.230787163063));
#218208=CARTESIAN_POINT('Ctrl Pts',(61.7666911381223,-42.1324472382017,
-215.238981368601));
#218209=CARTESIAN_POINT('Ctrl Pts',(61.7686498260413,-42.3426193701357,
-215.251595075326));
#218210=CARTESIAN_POINT('Ctrl Pts',(61.7703482765748,-42.5524019980439,
-215.269012080392));
#218211=CARTESIAN_POINT('Ctrl Pts',(61.7719995865043,-42.7563620955974,
-215.28594567536));
#218212=CARTESIAN_POINT('Ctrl Pts',(61.773404874694,-42.959953962892,-215.307419583956));
#218213=CARTESIAN_POINT('Ctrl Pts',(61.7745274697019,-43.1629057175116,
-215.33385125057));
#218214=CARTESIAN_POINT('Ctrl Pts',(61.7756179114226,-43.3600445422469,
-215.359525863247));
#218215=CARTESIAN_POINT('Ctrl Pts',(61.7764416279693,-43.5565795724041,
-215.389878433321));
#218216=CARTESIAN_POINT('Ctrl Pts',(61.776979990947,-43.7522133493642,-215.425304673598));
#218217=CARTESIAN_POINT('Ctrl Pts',(61.7772599446031,-43.8539446967897,
-215.443726641489));
#218218=CARTESIAN_POINT('Ctrl Pts',(61.7774630868531,-43.9554311411284,
-215.463520493776));
#218219=CARTESIAN_POINT('Ctrl Pts',(61.7775694692765,-44.0566083899622,
-215.484773367159));
#218220=CARTESIAN_POINT('Ctrl Pts',(61.7776616631061,-44.1442912770964,
-215.503191670874));
#218221=CARTESIAN_POINT('Ctrl Pts',(61.7776812199491,-44.2317418789998,
-215.522705760019));
#218222=CARTESIAN_POINT('Ctrl Pts',(61.7776158976463,-44.3189153994202,
-215.543372349475));
#218223=CARTESIAN_POINT('Ctrl Pts',(61.7774793872847,-44.5010903732092,
-215.586561329047));
#218224=CARTESIAN_POINT('Ctrl Pts',(61.776971632175,-44.6820611556678,-215.634785515999));
#218225=CARTESIAN_POINT('Ctrl Pts',(61.7762981534219,-44.861601675134,-215.688054278203));
#218226=CARTESIAN_POINT('Ctrl Pts',(61.7758058406997,-44.9928457291807,
-215.726993723886));
#218227=CARTESIAN_POINT('Ctrl Pts',(61.7752246785357,-45.1233178082053,
-215.76862450638));
#218228=CARTESIAN_POINT('Ctrl Pts',(61.7741149286305,-45.2524961979307,
-215.813816197241));
#218229=CARTESIAN_POINT('Ctrl Pts',(61.7737518188742,-45.2947633190072,
-215.828602901684));
#218230=CARTESIAN_POINT('Ctrl Pts',(61.7733322304229,-45.3368915425888,
-215.84377083554));
#218231=CARTESIAN_POINT('Ctrl Pts',(61.7728410789541,-45.3788614114542,
-215.85935045978));
#218232=CARTESIAN_POINT('Ctrl Pts',(61.7716501647156,-45.4806273993207,
-215.897126985992));
#218233=CARTESIAN_POINT('Ctrl Pts',(61.770039058637,-45.5814837181052,-215.937335255004));
#218234=CARTESIAN_POINT('Ctrl Pts',(61.7687805957718,-45.6818729518896,
-215.97872923867));
#218235=CARTESIAN_POINT('Ctrl Pts',(61.7679957127754,-45.7444840982349,
-216.004545998808));
#218236=CARTESIAN_POINT('Ctrl Pts',(61.7673475935058,-45.8069144706641,
-216.030823980101));
#218237=CARTESIAN_POINT('Ctrl Pts',(61.7670197730423,-45.8692809645529,
-216.057260894206));
#218238=CARTESIAN_POINT('',(62.0596235416337,-26.3318125162586,-215.724256795808));
#218239=CARTESIAN_POINT('Ctrl Pts',(62.0596235416336,-26.3318125162586,
-215.724256795808));
#218240=CARTESIAN_POINT('Ctrl Pts',(62.0577555696928,-26.4339470287308,
-215.753206765195));
#218241=CARTESIAN_POINT('Ctrl Pts',(62.0556509594839,-26.5309758697194,
-215.78008917588));
#218242=CARTESIAN_POINT('Ctrl Pts',(62.0535185542792,-26.6228963243231,
-215.804904027864));
#218243=CARTESIAN_POINT('Ctrl Pts',(62.0524523516769,-26.6688565516249,
-215.817311453857));
#218244=CARTESIAN_POINT('Ctrl Pts',(62.0513788550085,-26.7135398071411,
-215.829201990171));
#218245=CARTESIAN_POINT('Ctrl Pts',(62.0503220815731,-26.7569463787902,
-215.840575642485));
#218246=CARTESIAN_POINT('Ctrl Pts',(62.0497936948554,-26.7786496646148,
-215.846262468642));
#218247=CARTESIAN_POINT('Ctrl Pts',(62.0492694727596,-26.8000337816635,
-215.851820063874));
#218248=CARTESIAN_POINT('Ctrl Pts',(62.0487522794443,-26.8210987994165,
-215.857248440741));
#218249=CARTESIAN_POINT('Ctrl Pts',(62.0484936827866,-26.831631308293,-215.859962629175));
#218250=CARTESIAN_POINT('Ctrl Pts',(62.0482368423131,-26.8420840424851,
-215.862644512399));
#218251=CARTESIAN_POINT('Ctrl Pts',(62.0479821086777,-26.8524570116361,
-215.865294090431));
#218252=CARTESIAN_POINT('Ctrl Pts',(62.0477273750424,-26.8628299807872,
-215.867943668463));
#218253=CARTESIAN_POINT('Ctrl Pts',(62.0475055092753,-26.8718673652825,
-215.87024310001));
#218254=CARTESIAN_POINT('Ctrl Pts',(62.0472245741916,-26.8833366343711,
-215.873145907713));
#218255=CARTESIAN_POINT('Ctrl Pts',(62.044686460433,-26.9869559804883,-215.899371383265));
#218256=CARTESIAN_POINT('Ctrl Pts',(62.0420179406569,-27.0914557462519,
-215.92482563192));
#218257=CARTESIAN_POINT('Ctrl Pts',(62.0392255024341,-27.1958803121717,
-215.949297947245));
#218258=CARTESIAN_POINT('Ctrl Pts',(62.037072574512,-27.276390083844,-215.968165734741));
#218259=CARTESIAN_POINT('Ctrl Pts',(62.0348470483848,-27.3568551308637,
-215.986449843552));
#218260=CARTESIAN_POINT('Ctrl Pts',(62.0325730614187,-27.4368380736824,
-216.004053709611));
#218261=CARTESIAN_POINT('Ctrl Pts',(62.0273496175495,-27.6205622632014,
-216.044490531642));
#218262=CARTESIAN_POINT('Ctrl Pts',(62.0217447926267,-27.8051449629816,
-216.082146693372));
#218263=CARTESIAN_POINT('Ctrl Pts',(62.0157615800826,-27.9906023336393,
-216.117022203835));
#218264=CARTESIAN_POINT('Ctrl Pts',(62.0127699738106,-28.0833310189681,
-216.134459959066));
#218265=CARTESIAN_POINT('Ctrl Pts',(62.0096837379248,-28.1762783746767,
-216.151202530794));
#218266=CARTESIAN_POINT('Ctrl Pts',(62.0065029781599,-28.2694468745861,
-216.167249951255));
#218267=CARTESIAN_POINT('Ctrl Pts',(62.0045649202469,-28.326215056352,-216.17702775043));
#218268=CARTESIAN_POINT('Ctrl Pts',(62.0025715818842,-28.3837721485962,
-216.186658104095));
#218269=CARTESIAN_POINT('Ctrl Pts',(62.0005575197782,-28.440826636372,-216.195938775444));
#218270=CARTESIAN_POINT('Ctrl Pts',(61.999266083288,-28.4774105367535,-216.201889633464));
#218271=CARTESIAN_POINT('Ctrl Pts',(61.9979668951508,-28.5137878102374,
-216.207696719568));
#218272=CARTESIAN_POINT('Ctrl Pts',(61.9966772047599,-28.5496182363568,
-216.213306717361));
#218273=CARTESIAN_POINT('Ctrl Pts',(61.9834730873014,-28.916457563364,-216.270743037214));
#218274=CARTESIAN_POINT('Ctrl Pts',(61.9688293280833,-29.2870958911852,
-216.317548125342));
#218275=CARTESIAN_POINT('Ctrl Pts',(61.952786772668,-29.6616689192713,-216.353721981745));
#218276=CARTESIAN_POINT('Ctrl Pts',(61.9447654949604,-29.8489554333143,
-216.371808909947));
#218277=CARTESIAN_POINT('Ctrl Pts',(61.9363936787991,-30.0372261754395,
-216.387238030228));
#218278=CARTESIAN_POINT('Ctrl Pts',(61.927671271276,-30.2265006299287,-216.400009356926));
#218279=CARTESIAN_POINT('Ctrl Pts',(61.9233100675144,-30.3211378571733,
-216.406395020275));
#218280=CARTESIAN_POINT('Ctrl Pts',(61.918861178249,-30.416026012326,-216.412116210088));
#218281=CARTESIAN_POINT('Ctrl Pts',(61.9143242456229,-30.511167646582,-216.417172959074));
#218282=CARTESIAN_POINT('Ctrl Pts',(61.9122918465998,-30.5537880204005,
-216.419438219007));
#218283=CARTESIAN_POINT('Ctrl Pts',(61.9102417779571,-30.5964592611722,
-216.421570140067));
#218284=CARTESIAN_POINT('Ctrl Pts',(61.9081739949697,-30.6391815979838,
-216.423568722218));
#218285=CARTESIAN_POINT('Ctrl Pts',(61.9079338177601,-30.6441438845029,
-216.42380086161));
#218286=CARTESIAN_POINT('Ctrl Pts',(61.907693401551,-30.6491068603752,-216.424031202087));
#218287=CARTESIAN_POINT('Ctrl Pts',(61.9074527465505,-30.6540705259621,
-216.424259743649));
#218288=CARTESIAN_POINT('Ctrl Pts',(61.9062964708086,-30.6779194636387,
-216.425357817919));
#218289=CARTESIAN_POINT('Ctrl Pts',(61.9051346810113,-30.7017843234952,
-216.426414366295));
#218290=CARTESIAN_POINT('Ctrl Pts',(61.9039674023205,-30.7256651457048,
-216.427429384853));
#218291=CARTESIAN_POINT('Ctrl Pts',(61.9028001236297,-30.7495459679144,
-216.42844440341));
#218292=CARTESIAN_POINT('Ctrl Pts',(61.9015664443406,-30.774678958245,-216.429466072831));
#218293=CARTESIAN_POINT('Ctrl Pts',(61.9004491180021,-30.7973555397603,
-216.430349855778));
#218294=CARTESIAN_POINT('Ctrl Pts',(61.8821128244839,-31.1694978945224,
-216.444853499847));
#218295=CARTESIAN_POINT('Ctrl Pts',(61.8624992424722,-31.5454595353348,
-216.449238051427));
#218296=CARTESIAN_POINT('Ctrl Pts',(61.8416722272066,-31.9253979377884,
-216.443503510518));
#218297=CARTESIAN_POINT('Ctrl Pts',(61.8234061296913,-32.2586186043355,
-216.438474096456));
#218298=CARTESIAN_POINT('Ctrl Pts',(61.80420578693,-32.5948987249562,-216.425661108758));
#218299=CARTESIAN_POINT('Ctrl Pts',(61.7840819782534,-32.9343377021117,
-216.405064547423));
#218300=CARTESIAN_POINT('Ctrl Pts',(61.7608750372752,-33.3257815105432,
-216.381312424209));
#218301=CARTESIAN_POINT('Ctrl Pts',(61.736440544479,-33.7214276748005,-216.347209011029));
#218302=CARTESIAN_POINT('Ctrl Pts',(61.710868892887,-34.1214456828077,-216.302754307884));
#218303=CARTESIAN_POINT('Ctrl Pts',(61.6852972412951,-34.5214636908148,
-216.258299604738));
#218304=CARTESIAN_POINT('Ctrl Pts',(61.6585878780578,-34.9258545898999,
-216.203493611628));
#218305=CARTESIAN_POINT('Ctrl Pts',(61.6307906445938,-35.3347454916144,
-216.138336328552));
#218306=CARTESIAN_POINT('',(61.9835319875972,-17.519732572983,-215.952954107728));
#218307=CARTESIAN_POINT('Ctrl Pts',(61.9835319875972,-17.519732572983,-215.952954107728));
#218308=CARTESIAN_POINT('Ctrl Pts',(61.9836423128332,-17.5314237398636,
-215.949884435609));
#218309=CARTESIAN_POINT('Ctrl Pts',(61.9839561888802,-17.5486136892257,
-215.94516693725));
#218310=CARTESIAN_POINT('Ctrl Pts',(61.9846242057265,-17.5694505236489,
-215.939058207716));
#218311=CARTESIAN_POINT('Ctrl Pts',(61.9850106576282,-17.5789972212952,
-215.936149795196));
#218312=CARTESIAN_POINT('Ctrl Pts',(61.9852497232006,-17.5844090820673,
-215.934473721412));
#218313=CARTESIAN_POINT('Ctrl Pts',(61.985366427141,-17.5869458954142,-215.933681710066));
#218314=CARTESIAN_POINT('Ctrl Pts',(61.985432903138,-17.5883703075193,-215.933235701669));
#218315=CARTESIAN_POINT('Ctrl Pts',(61.9856070518024,-17.594619343813,-215.931447708497));
#218316=CARTESIAN_POINT('Ctrl Pts',(61.9860546172725,-17.6114739051512,
-215.92667840684));
#218317=CARTESIAN_POINT('Ctrl Pts',(61.9863253289469,-17.6217716024391,
-215.923771928037));
#218318=CARTESIAN_POINT('Ctrl Pts',(61.9867299233137,-17.6370620065691,
-215.919467837146));
#218319=CARTESIAN_POINT('Ctrl Pts',(61.9869232851332,-17.6443175804049,
-215.917427541273));
#218320=CARTESIAN_POINT('Ctrl Pts',(61.9870567406185,-17.6493108036505,
-215.91602385836));
#218321=CARTESIAN_POINT('Ctrl Pts',(61.9871592737459,-17.6531325304696,
-215.914949912397));
#218322=CARTESIAN_POINT('Ctrl Pts',(61.9884067096461,-17.6995234326739,
-215.901916052651));
#218323=CARTESIAN_POINT('Ctrl Pts',(61.9896013562167,-17.7444613163572,
-215.889465407473));
#218324=CARTESIAN_POINT('Ctrl Pts',(61.9931612274189,-17.8798611362945,
-215.852478094865));
#218325=CARTESIAN_POINT('Ctrl Pts',(61.9954673813378,-17.9696252699092,
-215.828653542303));
#218326=CARTESIAN_POINT('Ctrl Pts',(62.0023087939979,-18.2421350443946,
-215.758452964092));
#218327=CARTESIAN_POINT('Ctrl Pts',(62.0066123618738,-18.4220229695549,
-215.714899340256));
#218328=CARTESIAN_POINT('Ctrl Pts',(62.0149533931261,-18.7884597836193,
-215.631916484355));
#218329=CARTESIAN_POINT('Ctrl Pts',(62.0208820386822,-19.0631041231828,
-215.574032320922));
#218330=CARTESIAN_POINT('Ctrl Pts',(62.0263304049722,-19.337211649177,-215.522677625229));
#218331=CARTESIAN_POINT('Ctrl Pts',(62.0298564228196,-19.5198018772034,
-215.489892154265));
#218332=CARTESIAN_POINT('Ctrl Pts',(62.0315368963012,-19.6094031181495,
-215.474490491189));
#218333=CARTESIAN_POINT('Ctrl Pts',(62.0399691054701,-20.0731650506289,
-215.398453897984));
#218334=CARTESIAN_POINT('Ctrl Pts',(62.0458406539154,-20.4430189247693,
-215.349605146099));
#218335=CARTESIAN_POINT('Ctrl Pts',(62.053384096181,-20.9946381408474,-215.294302802292));
#218336=CARTESIAN_POINT('Ctrl Pts',(62.0568388647613,-21.2696575934642,
-215.271144326393));
#218337=CARTESIAN_POINT('Ctrl Pts',(62.0603145156397,-21.5888204107672,
-215.25198832252));
#218338=CARTESIAN_POINT('Ctrl Pts',(62.0619127847657,-21.7479398050394,
-215.244375875086));
#218339=CARTESIAN_POINT('Ctrl Pts',(62.0625677447133,-21.8160306805066,
-215.241534587864));
#218340=CARTESIAN_POINT('Ctrl Pts',(62.0629977011145,-21.8614012144509,
-215.239733994217));
#218341=CARTESIAN_POINT('Ctrl Pts',(62.0631962788612,-21.8826539937182,
-215.23893107315));
#218342=CARTESIAN_POINT('Ctrl Pts',(62.0775837642522,-23.4480132314265,
-215.183208144136));
#218343=CARTESIAN_POINT('Ctrl Pts',(62.0768822737846,-24.9479678284623,
-215.345269143632));
#218344=CARTESIAN_POINT('Ctrl Pts',(62.0596235416337,-26.3318125162586,
-215.724256795808));
#218345=CARTESIAN_POINT('',(62.0301313496079,-8.32556739006806,-215.882447372551));
#218346=CARTESIAN_POINT('Ctrl Pts',(62.030115892062,-8.32556237289759,-215.882468962491));
#218347=CARTESIAN_POINT('Ctrl Pts',(62.0303011812704,-8.34626436240946,
-215.88753471463));
#218348=CARTESIAN_POINT('Ctrl Pts',(62.030989541129,-8.38035489028408,-215.895278718971));
#218349=CARTESIAN_POINT('Ctrl Pts',(62.0325396354948,-8.45153820976076,
-215.910912103787));
#218350=CARTESIAN_POINT('Ctrl Pts',(62.0334411715356,-8.49214135874183,
-215.919733140771));
#218351=CARTESIAN_POINT('Ctrl Pts',(62.0346319766011,-8.54826989225757,
-215.931781953593));
#218352=CARTESIAN_POINT('Ctrl Pts',(62.035249580053,-8.57852190021065,-215.938245760757));
#218353=CARTESIAN_POINT('Ctrl Pts',(62.035517626716,-8.59195564672906,-215.941110121131));
#218354=CARTESIAN_POINT('Ctrl Pts',(62.035696909637,-8.60101558787812,-215.943040618559));
#218355=CARTESIAN_POINT('Ctrl Pts',(62.0358192267169,-8.60726231337101,
-215.944370592652));
#218356=CARTESIAN_POINT('Ctrl Pts',(62.0377253709339,-8.70525149376917,
-215.965223593057));
#218357=CARTESIAN_POINT('Ctrl Pts',(62.0394990136822,-8.80024742224131,
-215.984787334564));
#218358=CARTESIAN_POINT('Ctrl Pts',(62.0446069194413,-9.08616302923329,
-216.041699399449));
#218359=CARTESIAN_POINT('Ctrl Pts',(62.0477024749532,-9.27634345079324,
-216.076945388547));
#218360=CARTESIAN_POINT('Ctrl Pts',(62.0561197654603,-9.85181203919491,
-216.175621086794));
#218361=CARTESIAN_POINT('Ctrl Pts',(62.0604994716209,-10.2371764573657,
-216.231000261074));
#218362=CARTESIAN_POINT('Ctrl Pts',(62.0666464852748,-11.0056304231739,
-216.320132465571));
#218363=CARTESIAN_POINT('Ctrl Pts',(62.0684180957827,-11.3899288480629,
-216.354110109381));
#218364=CARTESIAN_POINT('Ctrl Pts',(62.0691637284138,-11.9674718683663,
-216.38919388744));
#218365=CARTESIAN_POINT('Ctrl Pts',(62.0690573031364,-12.2565170460506,
-216.402765104555));
#218366=CARTESIAN_POINT('Ctrl Pts',(62.0682218034411,-12.546158239528,-216.410380313799));
#218367=CARTESIAN_POINT('Ctrl Pts',(62.0675010132409,-12.7394054961317,
-216.414133562656));
#218368=CARTESIAN_POINT('Ctrl Pts',(62.0670521567137,-12.8373278964512,
-216.415355334398));
#218369=CARTESIAN_POINT('Ctrl Pts',(62.064459531591,-13.3151375449165,-216.418086040195));
#218370=CARTESIAN_POINT('Ctrl Pts',(62.0611113064883,-13.6974629887201,
-216.409927510236));
#218371=CARTESIAN_POINT('Ctrl Pts',(62.0542476848807,-14.2720292606053,
-216.382175073402));
#218372=CARTESIAN_POINT('Ctrl Pts',(62.0516520094611,-14.4637308422343,
-216.370338487474));
#218373=CARTESIAN_POINT('Ctrl Pts',(62.0458415981264,-14.8476509075169,
-216.341493768322));
#218374=CARTESIAN_POINT('Ctrl Pts',(62.0425860803387,-15.0420961048042,
-216.32425904904));
#218375=CARTESIAN_POINT('Ctrl Pts',(62.0251468210422,-15.9937435603833,
-216.227422444945));
#218376=CARTESIAN_POINT('Ctrl Pts',(62.0064818380416,-16.7545321493873,
-216.110109904781));
#218377=CARTESIAN_POINT('Ctrl Pts',(61.9835319875972,-17.519732572983,-215.952954107728));
#218378=CARTESIAN_POINT('',(62.0174953884411,0.438808195154074,-215.788045995909));
#218379=CARTESIAN_POINT('Ctrl Pts',(62.0174993799523,0.438809887676684,
-215.78803981657));
#218380=CARTESIAN_POINT('Ctrl Pts',(62.0175199857004,0.437737880397535,
-215.787745494507));
#218381=CARTESIAN_POINT('Ctrl Pts',(62.0175417397146,0.436720607586659,
-215.787462636701));
#218382=CARTESIAN_POINT('Ctrl Pts',(62.0175648395666,0.435767459872816,
-215.787193239101));
#218383=CARTESIAN_POINT('Ctrl Pts',(62.0180184663837,0.417049878348607,
-215.781902903222));
#218384=CARTESIAN_POINT('Ctrl Pts',(62.0184685135507,0.398079840556354,
-215.776592465129));
#218385=CARTESIAN_POINT('Ctrl Pts',(62.0189140804213,0.3789318657975,-215.771283693546));
#218386=CARTESIAN_POINT('Ctrl Pts',(62.0200362972047,0.330705258177559,
-215.757912877713));
#218387=CARTESIAN_POINT('Ctrl Pts',(62.0211298298166,0.281349530773877,
-215.744556209106));
#218388=CARTESIAN_POINT('Ctrl Pts',(62.0221829382759,0.232059213442546,
-215.731526094723));
#218389=CARTESIAN_POINT('Ctrl Pts',(62.0232455199048,0.182325508223198,
-215.718378768783));
#218390=CARTESIAN_POINT('Ctrl Pts',(62.0242669515709,0.132658426088991,
-215.705563865472));
#218391=CARTESIAN_POINT('Ctrl Pts',(62.0252391344941,0.0842905961880013,
-215.693349192722));
#218392=CARTESIAN_POINT('Ctrl Pts',(62.0262580962381,0.0335954367315529,
-215.680546782854));
#218393=CARTESIAN_POINT('Ctrl Pts',(62.0272229739792,-0.01567238529281,
-215.668403547226));
#218394=CARTESIAN_POINT('Ctrl Pts',(62.0281286510849,-0.0620880344041088,
-215.657170900034));
#218395=CARTESIAN_POINT('Ctrl Pts',(62.028226837897,-0.0671200757225747,
-215.655953139518));
#218396=CARTESIAN_POINT('Ctrl Pts',(62.0283243325486,-0.0721185899463497,
-215.654746031811));
#218397=CARTESIAN_POINT('Ctrl Pts',(62.0284211310589,-0.0770817583052276,
-215.653549862627));
#218398=CARTESIAN_POINT('Ctrl Pts',(62.0286398303158,-0.088295166749099,
-215.650847328145));
#218399=CARTESIAN_POINT('Ctrl Pts',(62.0288550016787,-0.0993281296954822,
-215.648200444206));
#218400=CARTESIAN_POINT('Ctrl Pts',(62.0290666028553,-0.110159665422851,
-215.64561242937));
#218401=CARTESIAN_POINT('Ctrl Pts',(62.0293620204162,-0.125281631738813,
-215.641999287692));
#218402=CARTESIAN_POINT('Ctrl Pts',(62.0296517907571,-0.140209428581813,
-215.638457495469));
#218403=CARTESIAN_POINT('Ctrl Pts',(62.0299360452298,-0.154942260830281,
-215.634985279954));
#218404=CARTESIAN_POINT('Ctrl Pts',(62.0300059984789,-0.158567918766427,
-215.634130789417));
#218405=CARTESIAN_POINT('Ctrl Pts',(62.0300756176579,-0.162181769268651,
-215.633280512819));
#218406=CARTESIAN_POINT('Ctrl Pts',(62.0301449046902,-0.165783800560488,
-215.632434424177));
#218407=CARTESIAN_POINT('Ctrl Pts',(62.0301647249564,-0.166814198551956,
-215.632192391844));
#218408=CARTESIAN_POINT('Ctrl Pts',(62.0301845180428,-0.167843629372059,
-215.631950702214));
#218409=CARTESIAN_POINT('Ctrl Pts',(62.0302042839942,-0.168872092745587,
-215.631709354683));
#218410=CARTESIAN_POINT('Ctrl Pts',(62.0302210196731,-0.169742884768136,
-215.631505007586));
#218411=CARTESIAN_POINT('Ctrl Pts',(62.0302377586917,-0.170614166281166,
-215.631300627362));
#218412=CARTESIAN_POINT('Ctrl Pts',(62.0302547273007,-0.171497727936975,
-215.631093451879));
#218413=CARTESIAN_POINT('Ctrl Pts',(62.0305332898224,-0.186002579968649,
-215.627692387902));
#218414=CARTESIAN_POINT('Ctrl Pts',(62.030856381188,-0.202924818300808,
-215.623750049934));
#218415=CARTESIAN_POINT('Ctrl Pts',(62.0311751486078,-0.219750316957847,
-215.619863638711));
#218416=CARTESIAN_POINT('Ctrl Pts',(62.0312538679905,-0.223905361629116,
-215.618903892283));
#218417=CARTESIAN_POINT('Ctrl Pts',(62.0313323354895,-0.228054487912501,
-215.617947396967));
#218418=CARTESIAN_POINT('Ctrl Pts',(62.0314098394012,-0.232159795046044,
-215.617002821984));
#218419=CARTESIAN_POINT('Ctrl Pts',(62.031458562176,-0.234740593235482,
-215.616409015643));
#218420=CARTESIAN_POINT('Ctrl Pts',(62.0315067944369,-0.237298224911199,
-215.615821256297));
#218421=CARTESIAN_POINT('Ctrl Pts',(62.0315550744332,-0.239861171708681,
-215.615232983426));
#218422=CARTESIAN_POINT('Ctrl Pts',(62.0323343763903,-0.281230467590438,
-215.605737493905));
#218423=CARTESIAN_POINT('Ctrl Pts',(62.0331009888089,-0.322656164563466,
-215.596414500743));
#218424=CARTESIAN_POINT('Ctrl Pts',(62.0338548909205,-0.364136660223962,
-215.587264567044));
#218425=CARTESIAN_POINT('Ctrl Pts',(62.0340165521309,-0.373031431884385,
-215.585302522723));
#218426=CARTESIAN_POINT('Ctrl Pts',(62.0341776604944,-0.381930442620933,
-215.583348052048));
#218427=CARTESIAN_POINT('Ctrl Pts',(62.0343383387091,-0.390840585373911,
-215.581399672612));
#218428=CARTESIAN_POINT('Ctrl Pts',(62.0354513689017,-0.45256182073756,
-215.567903100327));
#218429=CARTESIAN_POINT('Ctrl Pts',(62.0365412856687,-0.514694904346594,
-215.554729173333));
#218430=CARTESIAN_POINT('Ctrl Pts',(62.0375948581298,-0.576467803200393,
-215.542038436149));
#218431=CARTESIAN_POINT('Ctrl Pts',(62.0378614395503,-0.592097964134217,
-215.538827347335));
#218432=CARTESIAN_POINT('Ctrl Pts',(62.0381257087559,-0.607705042805249,
-215.535646994792));
#218433=CARTESIAN_POINT('Ctrl Pts',(62.0383874809175,-0.623276488100884,
-215.532499578114));
#218434=CARTESIAN_POINT('Ctrl Pts',(62.0385111622365,-0.630633637468982,
-215.531012496203));
#218435=CARTESIAN_POINT('Ctrl Pts',(62.0386342476484,-0.637980515719275,
-215.529533228673));
#218436=CARTESIAN_POINT('Ctrl Pts',(62.038756844207,-0.645323326956518,
-215.528060485936));
#218437=CARTESIAN_POINT('Ctrl Pts',(62.0411798407565,-0.790446538305592,
-215.498953220549));
#218438=CARTESIAN_POINT('Ctrl Pts',(62.0434488356458,-0.936202892943907,
-215.471950926648));
#218439=CARTESIAN_POINT('Ctrl Pts',(62.0455635795042,-1.08252171004957,
-215.4470693343));
#218440=CARTESIAN_POINT('Ctrl Pts',(62.0460443920013,-1.11578905613439,
-215.441412204478));
#218441=CARTESIAN_POINT('Ctrl Pts',(62.0465172330842,-1.14908547288418,
-215.435864670581));
#218442=CARTESIAN_POINT('Ctrl Pts',(62.0469821039688,-1.18241012093648,
-215.430426863699));
#218443=CARTESIAN_POINT('Ctrl Pts',(62.0471750188093,-1.19623937843347,
-215.428170250771));
#218444=CARTESIAN_POINT('Ctrl Pts',(62.0473666820277,-1.2100821617595,-215.425931119288));
#218445=CARTESIAN_POINT('Ctrl Pts',(62.0475571027041,-1.22393946910655,
-215.423709384899));
#218446=CARTESIAN_POINT('Ctrl Pts',(62.0487854491708,-1.31332878778413,
-215.409377645093));
#218447=CARTESIAN_POINT('Ctrl Pts',(62.0499611329979,-1.40327519821237,
-215.395781629928));
#218448=CARTESIAN_POINT('Ctrl Pts',(62.0510753972293,-1.49309213594665,
-215.383025488572));
#218449=CARTESIAN_POINT('Ctrl Pts',(62.0520503784318,-1.57168195646414,
-215.371863864886));
#218450=CARTESIAN_POINT('Ctrl Pts',(62.0529783941484,-1.65017255152723,
-215.361344478395));
#218451=CARTESIAN_POINT('Ctrl Pts',(62.0538558009956,-1.728101006012,-215.351506437208));
#218452=CARTESIAN_POINT('Ctrl Pts',(62.053961526629,-1.73749121676863,-215.350320974456));
#218453=CARTESIAN_POINT('Ctrl Pts',(62.0540665752971,-1.74687815347842,
-215.34914474847));
#218454=CARTESIAN_POINT('Ctrl Pts',(62.0541710336924,-1.75626947748911,
-215.347976789977));
#218455=CARTESIAN_POINT('Ctrl Pts',(62.0568806618616,-1.99987839011803,
-215.317680199397));
#218456=CARTESIAN_POINT('Ctrl Pts',(62.0591750307562,-2.24486471169071,
-215.29315003336));
#218457=CARTESIAN_POINT('Ctrl Pts',(62.0610585920148,-2.49090725646128,
-215.274384720384));
#218458=CARTESIAN_POINT('Ctrl Pts',(62.0629666027971,-2.74014355084581,
-215.255375824693));
#218459=CARTESIAN_POINT('Ctrl Pts',(62.064453075031,-2.99046152215792,-215.242282398062));
#218460=CARTESIAN_POINT('Ctrl Pts',(62.0655265978205,-3.24153013486207,
-215.235049704537));
#218461=CARTESIAN_POINT('Ctrl Pts',(62.06572580812,-3.28812015981675,-215.233707555998));
#218462=CARTESIAN_POINT('Ctrl Pts',(62.0659108088742,-3.33473606268537,
-215.232567081462));
#218463=CARTESIAN_POINT('Ctrl Pts',(62.0660816687505,-3.38137573845494,
-215.231627742877));
#218464=CARTESIAN_POINT('Ctrl Pts',(62.0664200834408,-3.47375290608351,
-215.229767235991));
#218465=CARTESIAN_POINT('Ctrl Pts',(62.0667030200249,-3.56622340514867,
-215.228695834708));
#218466=CARTESIAN_POINT('Ctrl Pts',(62.0669311442066,-3.65877138252441,
-215.228408582734));
#218467=CARTESIAN_POINT('Ctrl Pts',(62.0670291451991,-3.69852952464318,
-215.228285180741));
#218468=CARTESIAN_POINT('Ctrl Pts',(62.0671176862561,-3.73860300807162,
-215.228306525401));
#218469=CARTESIAN_POINT('Ctrl Pts',(62.0671957931192,-3.77860267586971,
-215.228474317159));
#218470=CARTESIAN_POINT('Ctrl Pts',(62.0672995013967,-3.83171320269179,
-215.228697106725));
#218471=CARTESIAN_POINT('Ctrl Pts',(62.0673846537059,-3.8846939386638,-215.229179757501));
#218472=CARTESIAN_POINT('Ctrl Pts',(62.0674508958752,-3.93663220814274,
-215.229897227125));
#218473=CARTESIAN_POINT('Ctrl Pts',(62.0677838568108,-4.19769574163658,
-215.233503530476));
#218474=CARTESIAN_POINT('Ctrl Pts',(62.0676791696996,-4.45960993311365,
-215.243348814244));
#218475=CARTESIAN_POINT('Ctrl Pts',(62.0671218812092,-4.72202625183822,
-215.259534787271));
#218476=CARTESIAN_POINT('Ctrl Pts',(62.0665693752761,-4.98219055725087,
-215.275581854964));
#218477=CARTESIAN_POINT('Ctrl Pts',(62.0655719913671,-5.24284830173915,
-215.297861274943));
#218478=CARTESIAN_POINT('Ctrl Pts',(62.0641187349921,-5.50365673697162,
-215.326421191673));
#218479=CARTESIAN_POINT('Ctrl Pts',(62.06267127947,-5.76342412301369,-215.354867107956));
#218480=CARTESIAN_POINT('Ctrl Pts',(62.0607715710024,-6.02334089753718,
-215.389543527112));
#218481=CARTESIAN_POINT('Ctrl Pts',(62.0584124940865,-6.28306684796035,
-215.430446656303));
#218482=CARTESIAN_POINT('Ctrl Pts',(62.056064416915,-6.54158176576643,-215.471159065147));
#218483=CARTESIAN_POINT('Ctrl Pts',(62.0532612348401,-6.79990753681709,
-215.518040271634));
#218484=CARTESIAN_POINT('Ctrl Pts',(62.0499998217298,-7.0577086353118,-215.571035080249));
#218485=CARTESIAN_POINT('Ctrl Pts',(62.0479865133785,-7.21685226019025,
-215.603749393695));
#218486=CARTESIAN_POINT('Ctrl Pts',(62.0457986624207,-7.37579595113682,
-215.638792426276));
#218487=CARTESIAN_POINT('Ctrl Pts',(62.0434363036247,-7.53446101372002,
-215.676141298899));
#218488=CARTESIAN_POINT('Ctrl Pts',(62.0410955413965,-7.69167556812021,
-215.713148729969));
#218489=CARTESIAN_POINT('Ctrl Pts',(62.0385792907942,-7.8486307341177,-215.752453819732));
#218490=CARTESIAN_POINT('Ctrl Pts',(62.0358856150351,-8.00521067750114,
-215.794042233454));
#218491=CARTESIAN_POINT('Ctrl Pts',(62.0356705839639,-8.01771015998553,
-215.797362158328));
#218492=CARTESIAN_POINT('Ctrl Pts',(62.0354544772225,-8.03020406724771,
-215.800695783931));
#218493=CARTESIAN_POINT('Ctrl Pts',(62.0352372951836,-8.04269236432169,
-215.804043085035));
#218494=CARTESIAN_POINT('Ctrl Pts',(62.0340910376763,-8.10860391184118,
-215.821709688772));
#218495=CARTESIAN_POINT('Ctrl Pts',(62.0329135938924,-8.17442996315404,
-215.839776233286));
#218496=CARTESIAN_POINT('Ctrl Pts',(62.0317048636879,-8.24016300281515,
-215.858240914477));
#218497=CARTESIAN_POINT('Ctrl Pts',(62.0313454521133,-8.25970848550308,
-215.863731320951));
#218498=CARTESIAN_POINT('Ctrl Pts',(62.0309832742987,-8.27924574457128,
-215.869256928137));
#218499=CARTESIAN_POINT('Ctrl Pts',(62.0306183276176,-8.2987745826764,-215.87481768646));
#218500=CARTESIAN_POINT('Ctrl Pts',(62.0304520445045,-8.30767263864652,
-215.877351372209));
#218501=CARTESIAN_POINT('Ctrl Pts',(62.0299989413369,-8.31437631353327,
-215.87976001137));
#218502=CARTESIAN_POINT('Ctrl Pts',(62.0301313496079,-8.32556739006806,
-215.882447372551));
#218503=CARTESIAN_POINT('',(61.6795265634691,9.54487894167559,-216.064116268519));
#218504=CARTESIAN_POINT('Ctrl Pts',(61.6795265634691,9.54487894167559,-216.064116268519));
#218505=CARTESIAN_POINT('Ctrl Pts',(61.6802430723727,9.521532518164,-216.069164370748));
#218506=CARTESIAN_POINT('Ctrl Pts',(61.6858191140444,9.43596373115034,-216.083872747801));
#218507=CARTESIAN_POINT('Ctrl Pts',(61.6957728249672,9.26950019496731,-216.11128748116));
#218508=CARTESIAN_POINT('Ctrl Pts',(61.6969269211031,9.25002898428,-216.114484504439));
#218509=CARTESIAN_POINT('Ctrl Pts',(61.6987217468774,9.21935845937455,-216.119506452048));
#218510=CARTESIAN_POINT('Ctrl Pts',(61.6990332190503,9.21399578439662,-216.120382944374));
#218511=CARTESIAN_POINT('Ctrl Pts',(61.6997227074585,9.20216114842476,-216.122313163012));
#218512=CARTESIAN_POINT('Ctrl Pts',(61.7014452264265,9.17257711291344,-216.127127572639));
#218513=CARTESIAN_POINT('Ctrl Pts',(61.7031617251547,9.1430058402448,-216.131886297433));
#218514=CARTESIAN_POINT('Ctrl Pts',(61.707269685065,9.07205921748622,-216.143200322058));
#218515=CARTESIAN_POINT('Ctrl Pts',(61.7099772069086,9.02506624388822,-216.150558627133));
#218516=CARTESIAN_POINT('Ctrl Pts',(61.7181461990841,8.88255125425903,-216.172456831843));
#218517=CARTESIAN_POINT('Ctrl Pts',(61.7235262896899,8.78772837399376,-216.186468897908));
#218518=CARTESIAN_POINT('Ctrl Pts',(61.7341541864233,8.59845357840604,-216.21331955589));
#218519=CARTESIAN_POINT('Ctrl Pts',(61.7393293185008,8.50532389398001,-216.225986299975));
#218520=CARTESIAN_POINT('Ctrl Pts',(61.7550912725796,8.21855250979642,-216.263257408001));
#218521=CARTESIAN_POINT('Ctrl Pts',(61.7704389797822,7.9330281740466,-216.296891034172));
#218522=CARTESIAN_POINT('Ctrl Pts',(61.7876193646635,7.6020550716402,-216.329764671456));
#218523=CARTESIAN_POINT('Ctrl Pts',(61.7948263815603,7.46066243116414,-216.342489317454));
#218524=CARTESIAN_POINT('Ctrl Pts',(61.7995963088469,7.36650073122957,-216.350669291297));
#218525=CARTESIAN_POINT('Ctrl Pts',(61.8019009783335,7.32072772463824,-216.354506331839));
#218526=CARTESIAN_POINT('Ctrl Pts',(61.8236187514576,6.88657756038332,-216.389500564472));
#218527=CARTESIAN_POINT('Ctrl Pts',(61.841685773179,6.50361036801132,-216.410524462369));
#218528=CARTESIAN_POINT('Ctrl Pts',(61.8669476828372,5.93336384123643,-216.426937179217));
#218529=CARTESIAN_POINT('Ctrl Pts',(61.8791181718381,5.6492911840457,-216.431362755141));
#218530=CARTESIAN_POINT('Ctrl Pts',(61.8925037732819,5.31966138595964,-216.429909557678));
#218531=CARTESIAN_POINT('Ctrl Pts',(61.89806457218,5.17876916430307,-216.427868965328));
#218532=CARTESIAN_POINT('Ctrl Pts',(61.9017324838976,5.08492433768665,-216.42619350522));
#218533=CARTESIAN_POINT('Ctrl Pts',(61.9034768601047,5.03986902103991,-216.425243169568));
#218534=CARTESIAN_POINT('Ctrl Pts',(61.965005265824,3.43392956880248,-216.385718336118));
#218535=CARTESIAN_POINT('Ctrl Pts',(62.0024632855742,1.91945558740173,-216.173720582219));
#218536=CARTESIAN_POINT('Ctrl Pts',(62.0174913965262,0.438806542391791,
-215.788052185604));
#218537=CARTESIAN_POINT('Ctrl Pts',(61.7131038227345,20.0389506617863,-216.160137831703));
#218538=CARTESIAN_POINT('Ctrl Pts',(61.7323346392832,19.2987667715537,-215.83025492416));
#218539=CARTESIAN_POINT('Ctrl Pts',(61.7438969106769,18.4794569854656,-215.58734776891));
#218540=CARTESIAN_POINT('Ctrl Pts',(61.7532854409784,17.1629064376784,-215.353450664475));
#218541=CARTESIAN_POINT('Ctrl Pts',(61.7550394001384,16.7094538020103,-215.29722890107));
#218542=CARTESIAN_POINT('Ctrl Pts',(61.7556514218488,16.011209030212,-215.245512163072));
#218543=CARTESIAN_POINT('Ctrl Pts',(61.7554491649581,15.657569560302,-215.227807770851));
#218544=CARTESIAN_POINT('Ctrl Pts',(61.7542962920732,15.2379182467459,-215.221422105953));
#218545=CARTESIAN_POINT('Ctrl Pts',(61.7534832401325,15.0264285229173,-215.221796638344));
#218546=CARTESIAN_POINT('Ctrl Pts',(61.7529831735412,14.91269863981,-215.22295282485));
#218547=CARTESIAN_POINT('Ctrl Pts',(61.7527320896283,14.8595090355654,-215.223752498906));
#218548=CARTESIAN_POINT('Ctrl Pts',(61.7525842430511,14.8290869986268,-215.224273158453));
#218549=CARTESIAN_POINT('Ctrl Pts',(61.7525410952316,14.8203036414675,-215.224430378052));
#218550=CARTESIAN_POINT('Ctrl Pts',(61.7443507875376,13.1665996145072,-215.255022606964));
#218551=CARTESIAN_POINT('Ctrl Pts',(61.720909381464,11.3762073620345,-215.53487822515));
#218552=CARTESIAN_POINT('Ctrl Pts',(61.6795265634691,9.54487894167559,-216.064116268519));
#218553=CARTESIAN_POINT('Ctrl Pts',(61.6907486315906,20.6657286340102,-216.300532529068));
#218554=CARTESIAN_POINT('Ctrl Pts',(61.7321110912357,20.3496658649069,-216.247078381677));
#218555=CARTESIAN_POINT('Ctrl Pts',(61.713103822739,20.0389506617614,-216.160137831685));
#218556=CARTESIAN_POINT('Ctrl Pts',(61.9064790936528,20.7060595729952,-215.92903923894));
#218557=CARTESIAN_POINT('Ctrl Pts',(61.9373844794568,20.4413798330517,-215.880084558757));
#218558=CARTESIAN_POINT('Ctrl Pts',(61.9252463833055,20.1793980393595,-215.812042320923));
#218559=CARTESIAN_POINT('Ctrl Pts',(62.0699842872639,20.7460043187545,-215.538658319552));
#218560=CARTESIAN_POINT('Ctrl Pts',(62.0914940184093,20.5335632238432,-215.496856996578));
#218561=CARTESIAN_POINT('Ctrl Pts',(62.0850713031281,20.3222903717942,-215.445236972404));
#218562=CARTESIAN_POINT('Ctrl Pts',(62.2967890390184,20.824939865421,-214.721940813782));
#218563=CARTESIAN_POINT('Ctrl Pts',(62.3035607512221,20.7183157084577,-214.699282243487));
#218564=CARTESIAN_POINT('Ctrl Pts',(62.3043696537349,20.611682425576,-214.675676922536));
#218565=CARTESIAN_POINT('Ctrl Pts',(62.3587717320579,20.8641365401031,-214.2924597236));
#218566=CARTESIAN_POINT('Ctrl Pts',(62.36063660277,20.8116268449194,-214.281171503343));
#218567=CARTESIAN_POINT('Ctrl Pts',(62.3625010497726,20.7591101230298,-214.269920324208));
#218568=CARTESIAN_POINT('Ctrl Pts',(62.3650472056256,20.9007985863674,-213.86644416092));
#218569=CARTESIAN_POINT('Ctrl Pts',(62.3650472056256,20.9007985863674,-213.86644416092));
#218570=CARTESIAN_POINT('Ctrl Pts',(62.3650472056256,20.9007985863674,-213.86644416092));
#218571=CARTESIAN_POINT('',(61.6907486315871,20.6657286340098,-216.300532529074));
#218572=CARTESIAN_POINT('Origin',(59.1013738165116,20.5826972454933,-214.78783829177));
#218573=CARTESIAN_POINT('Ctrl Pts',(61.6907486315871,20.66572863401,-216.300532529074));
#218574=CARTESIAN_POINT('Ctrl Pts',(61.9064790936528,20.7060595729952,-215.92903923894));
#218575=CARTESIAN_POINT('Ctrl Pts',(62.0699842872639,20.7460043187545,-215.538658319552));
#218576=CARTESIAN_POINT('Ctrl Pts',(62.296781831605,20.8249373570031,-214.721966767474));
#218577=CARTESIAN_POINT('Ctrl Pts',(62.358763853093,20.864131557726,-214.292514315806));
#218578=CARTESIAN_POINT('Ctrl Pts',(62.3650460084164,20.9007915960462,-213.866525388642));
#218579=CARTESIAN_POINT('Ctrl Pts',(61.4993881814496,20.607119072182,-216.605481304304));
#218580=CARTESIAN_POINT('Ctrl Pts',(61.6055583132372,20.2909606839731,-216.465410556121));
#218581=CARTESIAN_POINT('Ctrl Pts',(61.6377935655235,19.9815886122025,-216.280755810352));
#218582=CARTESIAN_POINT('Ctrl Pts',(61.5691908701343,20.635935030248,-216.502281627828));
#218583=CARTESIAN_POINT('Ctrl Pts',(61.6507949119074,20.3194192931332,-216.390568004056));
#218584=CARTESIAN_POINT('Ctrl Pts',(61.6652027952701,20.0090334790708,-216.239468240025));
#218585=CARTESIAN_POINT('Ctrl Pts',(61.6387815649058,20.6575029215218,-216.391600777272));
#218586=CARTESIAN_POINT('Ctrl Pts',(61.6967727624802,20.3410293418688,-216.311297779665));
#218587=CARTESIAN_POINT('Ctrl Pts',(61.6926044944813,20.0301302514676,-216.195652941674));
#218588=CARTESIAN_POINT('Ctrl Pts',(61.7080768938388,20.6687713493157,-216.270467388273));
#218589=CARTESIAN_POINT('Ctrl Pts',(61.7438559996883,20.3528222220489,-216.225852774312));
#218590=CARTESIAN_POINT('Ctrl Pts',(61.7199387591126,20.0421410735254,-216.14839440092));
#218591=CARTESIAN_POINT('',(61.5168384358791,20.6141575017552,-216.579518431174));
#218592=CARTESIAN_POINT('',(61.6446456814072,19.9883159925442,-216.270380726959));
#218593=CARTESIAN_POINT('Origin',(59.0326817073425,20.5344053061246,-214.899457439615));
#218594=CARTESIAN_POINT('Ctrl Pts',(61.516838435851,20.614157501844,-216.579518431211));
#218595=CARTESIAN_POINT('Ctrl Pts',(61.5771479675576,20.6380049970577,-216.489212055522));
#218596=CARTESIAN_POINT('Ctrl Pts',(61.6351552038294,20.6553354111624,-216.396265812028));
#218597=CARTESIAN_POINT('Ctrl Pts',(61.6907486315871,20.66572863401,-216.300532529074));
#218598=CARTESIAN_POINT('Ctrl Pts',(61.6446456814073,19.9883159925441,-216.270380726959));
#218599=CARTESIAN_POINT('Ctrl Pts',(61.6589899518011,20.0021161053552,-216.248548270214));
#218600=CARTESIAN_POINT('Ctrl Pts',(61.6733754048797,20.0141614257302,-216.225936038732));
#218601=CARTESIAN_POINT('Ctrl Pts',(61.6878163906252,20.0240270541524,-216.202356324519));
#218602=CARTESIAN_POINT('Ctrl Pts',(61.6962258005136,20.0297720991703,-216.188625164793));
#218603=CARTESIAN_POINT('Ctrl Pts',(61.7046540333319,20.034777214613,-216.174565637229));
#218604=CARTESIAN_POINT('Ctrl Pts',(61.7131038227239,20.038950661781,-216.160137831721));
#218605=CARTESIAN_POINT('Ctrl Pts',(62.0998335778874,28.4197995297673,-213.858707258037));
#218606=CARTESIAN_POINT('Ctrl Pts',(62.0737483304577,28.4205138141115,-215.350417820742));
#218607=CARTESIAN_POINT('Ctrl Pts',(61.235107328202,28.3894013135675,-216.583947161644));
#218608=CARTESIAN_POINT('Ctrl Pts',(62.2010617731482,25.8108994796242,-213.861712475947));
#218609=CARTESIAN_POINT('Ctrl Pts',(62.1750190192639,25.812006950141,-215.350359724743));
#218610=CARTESIAN_POINT('Ctrl Pts',(61.3394317178725,25.7825379828778,-216.58230034997));
#218611=CARTESIAN_POINT('Ctrl Pts',(62.2927210668524,23.2015642400677,-213.864398964149));
#218612=CARTESIAN_POINT('Ctrl Pts',(62.2667395005803,23.2024779691081,-215.350312870121));
#218613=CARTESIAN_POINT('Ctrl Pts',(61.4338508567495,23.1751069333097,-216.580828347939));
#218614=CARTESIAN_POINT('Ctrl Pts',(62.3748047396227,20.5920154834281,-213.866720382044));
#218615=CARTESIAN_POINT('Ctrl Pts',(62.3488810204336,20.5925259779214,-215.350234406272));
#218616=CARTESIAN_POINT('Ctrl Pts',(61.5183514407949,20.5675003107738,-216.579494546858));
#218617=CARTESIAN_POINT('',(61.2351073280272,28.3894013125172,-216.583947161963));
#218618=CARTESIAN_POINT('Origin',(-967.060476622167,-12.7722155952905,-232.807288933329));
#218619=CARTESIAN_POINT('',(62.099833577893,28.4197995297552,-213.858707258032));
#218620=CARTESIAN_POINT('Origin',(57.1043579940171,28.2258690560256,-213.771445225846));
#218621=CARTESIAN_POINT('Origin',(-1003.25098428815,-12.9621320438613,-174.780968069139));
#218622=CARTESIAN_POINT('Ctrl Pts',(62.0688011703024,29.2457316556486,-213.781328275569));
#218623=CARTESIAN_POINT('Ctrl Pts',(62.0289469563781,29.5310768106848,-215.415988103393));
#218624=CARTESIAN_POINT('Ctrl Pts',(61.0052807181397,29.7205356651696,-216.708851684624));
#218625=CARTESIAN_POINT('Ctrl Pts',(62.0742729941045,29.0960629819322,-213.807353032748));
#218626=CARTESIAN_POINT('Ctrl Pts',(62.0368058273153,29.3327506759839,-215.417932437979));
#218627=CARTESIAN_POINT('Ctrl Pts',(61.0493770342224,29.4859232929652,-216.703260974786));
#218628=CARTESIAN_POINT('Ctrl Pts',(62.0798211066684,28.9461456833678,-213.82776792667));
#218629=CARTESIAN_POINT('Ctrl Pts',(62.0445308741403,29.1383495067355,-215.415821866988));
#218630=CARTESIAN_POINT('Ctrl Pts',(61.0888241268935,29.2581335927935,-216.69312078545));
#218631=CARTESIAN_POINT('Ctrl Pts',(62.0911177663954,28.645756714799,-213.854728078229));
#218632=CARTESIAN_POINT('Ctrl Pts',(62.0608777530688,28.7334658375517,-215.390288011995));
#218633=CARTESIAN_POINT('Ctrl Pts',(61.1729733940828,28.7720316195816,-216.645653415601));
#218634=CARTESIAN_POINT('Ctrl Pts',(62.0968756241727,28.4952634919339,-213.860788934278));
#218635=CARTESIAN_POINT('Ctrl Pts',(62.0695770660397,28.5216890337278,-215.365176615215));
#218636=CARTESIAN_POINT('Ctrl Pts',(61.2182542009739,28.5113092167426,-216.605776792465));
#218637=CARTESIAN_POINT('Ctrl Pts',(62.1027691607293,28.3443970744867,-213.858075427907));
#218638=CARTESIAN_POINT('Ctrl Pts',(62.0779510070526,28.3183576151588,-215.336592494545));
#218639=CARTESIAN_POINT('Ctrl Pts',(61.2532962738455,28.2653275536711,-216.563073912214));
#218640=CARTESIAN_POINT('',(61.0271214515743,29.6036708476852,-216.705447812142));
#218641=CARTESIAN_POINT('',(62.0715435503803,29.170876467827,-213.793867031503));
#218642=CARTESIAN_POINT('Origin',(57.0762058255522,28.9734268472959,-213.706604999317));
#218643=CARTESIAN_POINT('Ctrl Pts',(62.0998335778932,28.4197995297553,-213.858707258032));
#218644=CARTESIAN_POINT('Ctrl Pts',(62.0949496006365,28.5456716573274,-213.858562269111));
#218645=CARTESIAN_POINT('Ctrl Pts',(62.0901675429832,28.6710240626335,-213.852460313436));
#218646=CARTESIAN_POINT('Ctrl Pts',(62.0854694365319,28.7959511990833,-213.84124800245));
#218647=CARTESIAN_POINT('Ctrl Pts',(62.0807548271212,28.9213171649822,-213.829996306167));
#218648=CARTESIAN_POINT('Ctrl Pts',(62.0761182844882,29.0462698189248,-213.813935251642));
#218649=CARTESIAN_POINT('Ctrl Pts',(62.0715435503805,29.1708764678268,-213.793867031503));
#218650=CARTESIAN_POINT('Ctrl Pts',(61.0271214515743,29.6036708476852,-216.705447812142));
#218651=CARTESIAN_POINT('Ctrl Pts',(61.0473497691228,29.4934302108373,-216.701965843739));
#218652=CARTESIAN_POINT('Ctrl Pts',(61.0662258246735,29.3872447406964,-216.697037564987));
#218653=CARTESIAN_POINT('Ctrl Pts',(61.092939107741,29.234817073613,-216.687475681334));
#218654=CARTESIAN_POINT('Ctrl Pts',(61.1015764034094,29.1851490360971,-216.683926809195));
#218655=CARTESIAN_POINT('Ctrl Pts',(61.1141822136387,29.1124498685452,-216.678061134607));
#218656=CARTESIAN_POINT('Ctrl Pts',(61.1203973405399,29.0765540137621,-216.674992705717));
#218657=CARTESIAN_POINT('Ctrl Pts',(61.1264920221608,29.0413270583538,-216.671720889435));
#218658=CARTESIAN_POINT('Ctrl Pts',(61.1305296762386,29.01798876909,-216.669494481381));
#218659=CARTESIAN_POINT('Ctrl Pts',(61.1328731847041,29.0044428970592,-216.668162653334));
#218660=CARTESIAN_POINT('Ctrl Pts',(61.1610345826342,28.8416940907171,-216.651802264667));
#218661=CARTESIAN_POINT('Ctrl Pts',(61.1982120890333,28.6316301319716,-216.62405122618));
#218662=CARTESIAN_POINT('Ctrl Pts',(61.2351073279234,28.3894013132814,-216.583947162069));
#218663=CARTESIAN_POINT('Ctrl Pts',(61.0265937502316,29.6037608952923,-216.706123999504));
#218664=CARTESIAN_POINT('Ctrl Pts',(62.0328659203364,29.432086372265,-215.416932921719));
#218665=CARTESIAN_POINT('Ctrl Pts',(62.0715435503799,29.1708764678276,-213.793867031504));
#218666=CARTESIAN_POINT('Ctrl Pts',(60.9825645796766,29.8436221509486,-216.713705040631));
#218667=CARTESIAN_POINT('Ctrl Pts',(62.0158262438435,29.7028146280762,-215.414349655834));
#218668=CARTESIAN_POINT('Ctrl Pts',(62.0610597588847,29.4471784511516,-213.768820140554));
#218669=CARTESIAN_POINT('Ctrl Pts',(60.9251255281948,30.093369550312,-216.724290200207));
#218670=CARTESIAN_POINT('Ctrl Pts',(61.9883890041931,29.9794001400379,-215.414675965098));
#218671=CARTESIAN_POINT('Ctrl Pts',(62.0405226886033,29.7223719581141,-213.744683753048));
#218672=CARTESIAN_POINT('Ctrl Pts',(60.8090550311091,30.5582447334237,-216.734083503021));
#218673=CARTESIAN_POINT('Ctrl Pts',(61.9158847636691,30.513005122286,-215.407737544432));
#218674=CARTESIAN_POINT('Ctrl Pts',(61.9794688757528,30.270714507063,-213.698186104728));
#218675=CARTESIAN_POINT('Ctrl Pts',(60.7468471946344,30.7826875211125,-216.737055032757));
#218676=CARTESIAN_POINT('Ctrl Pts',(61.8707136570867,30.7753294640716,-215.403383061571));
#218677=CARTESIAN_POINT('Ctrl Pts',(61.9389263175003,30.5439708219921,-213.676343773128));
#218678=CARTESIAN_POINT('Ctrl Pts',(60.5974728457365,31.2445885019563,-216.748323533354));
#218679=CARTESIAN_POINT('Ctrl Pts',(61.7592263865063,31.3084059968012,-215.399922850299));
#218680=CARTESIAN_POINT('Ctrl Pts',(61.8376360324932,31.0884065479068,-213.634598566576));
#218681=CARTESIAN_POINT('Ctrl Pts',(60.5132484754513,31.4761990764113,-216.754202271862));
#218682=CARTESIAN_POINT('Ctrl Pts',(61.6932218885361,31.5756441252082,-215.398886644252));
#218683=CARTESIAN_POINT('Ctrl Pts',(61.7769096374107,31.3595164244255,-213.614424841559));
#218684=CARTESIAN_POINT('Ctrl Pts',(60.3353787972406,31.9258725276716,-216.761796156373));
#218685=CARTESIAN_POINT('Ctrl Pts',(61.5426514848983,32.1020838962177,-215.394244475031));
#218686=CARTESIAN_POINT('Ctrl Pts',(61.6347983988382,31.8994507060226,-213.575433990375));
#218687=CARTESIAN_POINT('Ctrl Pts',(60.2431411074621,32.1425438899593,-216.763259486997));
#218688=CARTESIAN_POINT('Ctrl Pts',(61.4584458415044,32.3604872290325,-215.390415183932));
#218689=CARTESIAN_POINT('Ctrl Pts',(61.553185886347,32.168827114668,-213.55678698258));
#218690=CARTESIAN_POINT('Ctrl Pts',(60.0922775089899,32.4653895464032,-216.76679570928));
#218691=CARTESIAN_POINT('Ctrl Pts',(61.3177123000692,32.7449914243882,-215.386464661929));
#218692=CARTESIAN_POINT('Ctrl Pts',(61.4159587545684,32.5674954665497,-213.530743809026));
#218693=CARTESIAN_POINT('Ctrl Pts',(60.0397836500009,32.5728382848651,-216.768161995858));
#218694=CARTESIAN_POINT('Ctrl Pts',(61.2682557637607,32.8729588341924,-215.3854110548));
#218695=CARTESIAN_POINT('Ctrl Pts',(61.367676762258,32.699721268844,-213.52234238551));
#218696=CARTESIAN_POINT('Ctrl Pts',(59.9288125178118,32.7888250337031,-216.771641849425));
#218697=CARTESIAN_POINT('Ctrl Pts',(61.1639802174555,33.1287940399443,-215.384139008864));
#218698=CARTESIAN_POINT('Ctrl Pts',(61.2664764446162,32.9616854374291,-213.505934868453));
#218699=CARTESIAN_POINT('Ctrl Pts',(59.8686110761104,32.8993820177949,-216.774231175379));
#218700=CARTESIAN_POINT('Ctrl Pts',(61.1085304672864,33.2580306163176,-215.384328545335));
#218701=CARTESIAN_POINT('Ctrl Pts',(61.2135447672982,33.0914831455605,-213.497857516741));
#218702=CARTESIAN_POINT('Ctrl Pts',(59.6957162986054,33.2125071669439,-216.777043804247));
#218703=CARTESIAN_POINT('Ctrl Pts',(60.9396247822756,33.6325165068372,-215.38088449035));
#218704=CARTESIAN_POINT('Ctrl Pts',(61.0478125873327,33.4773667644598,-213.474082387732));
#218705=CARTESIAN_POINT('Ctrl Pts',(59.5851327557243,33.4043691267079,-216.775410250767));
#218706=CARTESIAN_POINT('Ctrl Pts',(60.8222645138006,33.8692180996893,-215.375922515872));
#218707=CARTESIAN_POINT('Ctrl Pts',(60.928044089869,33.730020614473,-213.459385328775));
#218708=CARTESIAN_POINT('Ctrl Pts',(59.401265962428,33.6968854804001,-216.776684954411));
#218709=CARTESIAN_POINT('Ctrl Pts',(60.6302585737573,34.2248518898603,-215.372298465673));
#218710=CARTESIAN_POINT('Ctrl Pts',(60.7344672841328,34.1022007074189,-213.439632708163));
#218711=CARTESIAN_POINT('Ctrl Pts',(59.3355992902892,33.7965187512738,-216.777959065008));
#218712=CARTESIAN_POINT('Ctrl Pts',(60.5629578125134,34.3444556219022,-215.371922956317));
#218713=CARTESIAN_POINT('Ctrl Pts',(60.6676250274774,34.2251152633889,-213.433348725254));
#218714=CARTESIAN_POINT('Ctrl Pts',(59.1992609912169,33.9957058462152,-216.780349347581));
#218715=CARTESIAN_POINT('Ctrl Pts',(60.4230592905929,34.5826912965888,-215.371180244526));
#218716=CARTESIAN_POINT('Ctrl Pts',(60.5293279501712,34.4685916589618,-213.420959244596));
#218717=CARTESIAN_POINT('Ctrl Pts',(59.1288052942883,34.0949722689346,-216.781320682795));
#218718=CARTESIAN_POINT('Ctrl Pts',(60.3505196458902,34.7011122420226,-215.370684459066));
#218719=CARTESIAN_POINT('Ctrl Pts',(60.45787721928,34.5891494282615,-213.414818675447));
#218720=CARTESIAN_POINT('Ctrl Pts',(59.03102591712,34.2324713614236,-216.780298741043));
#218721=CARTESIAN_POINT('Ctrl Pts',(60.2427003997968,34.8702746739671,-215.367852804425));
#218722=CARTESIAN_POINT('Ctrl Pts',(60.3471832550309,34.7682519438017,-213.406087731129));
#218723=CARTESIAN_POINT('Ctrl Pts',(59.0007435323251,34.2754518704397,-216.779359734745));
#218724=CARTESIAN_POINT('Ctrl Pts',(60.2073665276868,34.9246098826991,-215.366397395166));
#218725=CARTESIAN_POINT('Ctrl Pts',(60.3096963328381,34.8276667087864,-213.40328205755));
#218726=CARTESIAN_POINT('Ctrl Pts',(58.9378339843495,34.3626721170424,-216.778074064536));
#218727=CARTESIAN_POINT('Ctrl Pts',(60.1349754818777,35.0339069140606,-215.36407541824));
#218728=CARTESIAN_POINT('Ctrl Pts',(60.2335269589271,34.945932810391,-213.397980978203));
#218729=CARTESIAN_POINT('Ctrl Pts',(58.9053639383789,34.4067399736955,-216.777661739873));
#218730=CARTESIAN_POINT('Ctrl Pts',(60.0979756928914,35.088748275143,-215.363147491525));
#218731=CARTESIAN_POINT('Ctrl Pts',(60.1948462339725,35.0047819102636,-213.395467604646));
#218732=CARTESIAN_POINT('Ctrl Pts',(58.8053491301352,34.5398396001192,-216.776857332426));
#218733=CARTESIAN_POINT('Ctrl Pts',(59.9846859375433,35.2535081898727,-215.360820730381));
#218734=CARTESIAN_POINT('Ctrl Pts',(60.0770110939915,35.1804605606286,-213.388255279851));
#218735=CARTESIAN_POINT('Ctrl Pts',(58.7349881372357,34.6298757701064,-216.776911998089));
#218736=CARTESIAN_POINT('Ctrl Pts',(59.9060137786903,35.3637066384188,-215.359888334169));
#218737=CARTESIAN_POINT('Ctrl Pts',(59.9960526306669,35.2964118100118,-213.383856689816));
#218738=CARTESIAN_POINT('Ctrl Pts',(58.6659957159662,34.7166003426006,-216.776374027644));
#218739=CARTESIAN_POINT('Ctrl Pts',(59.8268160252816,35.4705884119597,-215.358542412566));
#218740=CARTESIAN_POINT('Ctrl Pts',(59.9134443065885,35.4101621769243,-213.379883144536));
#218741=CARTESIAN_POINT('',(58.6665914736623,34.7169872964315,-216.775646223556));
#218742=CARTESIAN_POINT('',(59.9134443065973,35.4101621769153,-213.379883144535));
#218743=CARTESIAN_POINT('Origin',(55.8698139418538,32.470529749032,-213.292621112349));
#218744=CARTESIAN_POINT('Ctrl Pts',(62.0715435503799,29.1708764678276,-213.793867031504));
#218745=CARTESIAN_POINT('Ctrl Pts',(62.0643014392995,29.3617434510075,-213.776564859235));
#218746=CARTESIAN_POINT('Ctrl Pts',(62.0522600475002,29.5519971941426,-213.759753107678));
#218747=CARTESIAN_POINT('Ctrl Pts',(62.0354890800171,29.7414131526144,-213.743402541702));
#218748=CARTESIAN_POINT('Ctrl Pts',(62.0279429432301,29.8266413145379,-213.736045565575));
#218749=CARTESIAN_POINT('Ctrl Pts',(62.0194399620359,29.9116999236011,-213.728781830163));
#218750=CARTESIAN_POINT('Ctrl Pts',(62.0099898554776,29.9965687797107,-213.721608053805));
#218751=CARTESIAN_POINT('Ctrl Pts',(61.9889706914869,30.1853362177545,-213.705651960531));
#218752=CARTESIAN_POINT('Ctrl Pts',(61.9632502648204,30.373215364858,-213.690387208237));
#218753=CARTESIAN_POINT('Ctrl Pts',(61.9329235309347,30.5599217016399,-213.675635343783));
#218754=CARTESIAN_POINT('Ctrl Pts',(61.9190056872795,30.6456068141406,-213.668865272733));
#218755=CARTESIAN_POINT('Ctrl Pts',(61.904118389167,30.73104504063,-213.66220316716));
#218756=CARTESIAN_POINT('Ctrl Pts',(61.8882744453593,30.8162093827887,-213.655631541451));
#218757=CARTESIAN_POINT('Ctrl Pts',(61.8865583969754,30.8254334833975,-213.654919772474));
#218758=CARTESIAN_POINT('Ctrl Pts',(61.884831153,30.8346542910449,-213.654208753614));
#218759=CARTESIAN_POINT('Ctrl Pts',(61.8830927250357,30.8438717751564,-213.653498479181));
#218760=CARTESIAN_POINT('Ctrl Pts',(61.8486303829777,31.0265978339227,-213.639418102558));
#218761=CARTESIAN_POINT('Ctrl Pts',(61.8097530423276,31.20808602447,-213.625773220073));
#218762=CARTESIAN_POINT('Ctrl Pts',(61.7665678010779,31.3880986014977,-213.612525374102));
#218763=CARTESIAN_POINT('Ctrl Pts',(61.747192030664,31.4688642117661,-213.606581509611));
#218764=CARTESIAN_POINT('Ctrl Pts',(61.7269497583691,31.54933287442,-213.600717484172));
#218765=CARTESIAN_POINT('Ctrl Pts',(61.7058540178194,31.6294835659502,-213.594929422224));
#218766=CARTESIAN_POINT('Ctrl Pts',(61.7034089471228,31.6387733136466,-213.59425856544));
#218767=CARTESIAN_POINT('Ctrl Pts',(61.7009521439872,31.6480594437296,-213.593588930303));
#218768=CARTESIAN_POINT('Ctrl Pts',(61.6984836689592,31.6573418016004,-213.592920528782));
#218769=CARTESIAN_POINT('Ctrl Pts',(61.6606248428338,31.7997046647723,-213.582669302148));
#218770=CARTESIAN_POINT('Ctrl Pts',(61.6200524091205,31.941077973338,-213.572715378021));
#218771=CARTESIAN_POINT('Ctrl Pts',(61.5768449470309,32.0813729523784,-213.563091155333));
#218772=CARTESIAN_POINT('Ctrl Pts',(61.5412940675433,32.1968069457527,-213.555172393981));
#218773=CARTESIAN_POINT('Ctrl Pts',(61.5039582038038,32.3115108548697,-213.547476866768));
#218774=CARTESIAN_POINT('Ctrl Pts',(61.4648558996718,32.4254280494983,-213.540024838124));
#218775=CARTESIAN_POINT('Ctrl Pts',(61.4637643495236,32.4286080751626,-213.539816812967));
#218776=CARTESIAN_POINT('Ctrl Pts',(61.4627391435221,32.4315904138355,-213.539621864181));
#218777=CARTESIAN_POINT('Ctrl Pts',(61.4617011316131,32.4346060163256,-213.539424870969));
#218778=CARTESIAN_POINT('Ctrl Pts',(61.4600818133902,32.4393104132821,-213.539117557831));
#218779=CARTESIAN_POINT('Ctrl Pts',(61.4584315246665,32.4440961213275,-213.538805189393));
#218780=CARTESIAN_POINT('Ctrl Pts',(61.4564456905764,32.4498387425552,-213.538430823349));
#218781=CARTESIAN_POINT('Ctrl Pts',(61.4168161144555,32.5644392755033,-213.530959923492));
#218782=CARTESIAN_POINT('Ctrl Pts',(61.3757353289488,32.6772777468317,-213.52379011113));
#218783=CARTESIAN_POINT('Ctrl Pts',(61.3334684629503,32.7880141235003,-213.516853234189));
#218784=CARTESIAN_POINT('Ctrl Pts',(61.3280232273835,32.8022802783837,-213.515959557117));
#218785=CARTESIAN_POINT('Ctrl Pts',(61.3225582818976,32.8165116104594,-213.515069754931));
#218786=CARTESIAN_POINT('Ctrl Pts',(61.317074171808,32.8307074509615,-213.514183689717));
#218787=CARTESIAN_POINT('Ctrl Pts',(61.2657604929994,32.963534981416,-213.505892961587));
#218788=CARTESIAN_POINT('Ctrl Pts',(61.2127553614539,33.0933166559663,-213.497856596317));
#218789=CARTESIAN_POINT('Ctrl Pts',(61.1582925442941,33.2201235367584,-213.490078204233));
#218790=CARTESIAN_POINT('Ctrl Pts',(61.0707863518123,33.423865977882,-213.477580549678));
#218791=CARTESIAN_POINT('Ctrl Pts',(60.9794973350864,33.6199773638123,-213.466093247516));
#218792=CARTESIAN_POINT('Ctrl Pts',(60.8853140442522,33.8087163473985,-213.455630952108));
#218793=CARTESIAN_POINT('Ctrl Pts',(60.8567940840068,33.8658690361711,-213.452462829116));
#218794=CARTESIAN_POINT('Ctrl Pts',(60.8280087145055,33.9223456729049,-213.449388335299));
#218795=CARTESIAN_POINT('Ctrl Pts',(60.7989825602443,33.9781533043984,-213.446406949198));
#218796=CARTESIAN_POINT('Ctrl Pts',(60.7789255400534,34.0167162770057,-213.444346816784));
#218797=CARTESIAN_POINT('Ctrl Pts',(60.758753934641,34.0549586516216,-213.44232317516));
#218798=CARTESIAN_POINT('Ctrl Pts',(60.7384761670337,34.0928815999144,-213.440328492273));
#218799=CARTESIAN_POINT('Ctrl Pts',(60.6923105839104,34.179219260726,-213.43578727746));
#218800=CARTESIAN_POINT('Ctrl Pts',(60.645609474611,34.2638723253871,-213.431435301927));
#218801=CARTESIAN_POINT('Ctrl Pts',(60.5984740490749,34.3468561605459,-213.427198972163));
#218802=CARTESIAN_POINT('Ctrl Pts',(60.5325838024229,34.4628586216366,-213.421277039564));
#218803=CARTESIAN_POINT('Ctrl Pts',(60.465847821872,34.5755963690338,-213.415555332432));
#218804=CARTESIAN_POINT('Ctrl Pts',(60.3984978653644,34.6851586013184,-213.410238215137));
#218805=CARTESIAN_POINT('Ctrl Pts',(60.3936934720552,34.6929741973935,-213.409858919825));
#218806=CARTESIAN_POINT('Ctrl Pts',(60.3888859574889,34.7007736311751,-213.409481661815));
#218807=CARTESIAN_POINT('Ctrl Pts',(60.3840754072371,34.7085569334586,-213.409106505425));
#218808=CARTESIAN_POINT('Ctrl Pts',(60.366977631822,34.7362205368859,-213.407773115403));
#218809=CARTESIAN_POINT('Ctrl Pts',(60.3498409473359,34.7636809861284,-213.406471589833));
#218810=CARTESIAN_POINT('Ctrl Pts',(60.3326688897114,34.7909397659281,-213.405206193258));
#218811=CARTESIAN_POINT('Ctrl Pts',(60.3123511070016,34.8231920432625,-213.403708990464));
#218812=CARTESIAN_POINT('Ctrl Pts',(60.2919954872675,34.8551439920857,-213.402249242024));
#218813=CARTESIAN_POINT('Ctrl Pts',(60.2716012226596,34.8868093488113,-213.400835331901));
#218814=CARTESIAN_POINT('Ctrl Pts',(60.233057341349,34.9466548874837,-213.398163130427));
#218815=CARTESIAN_POINT('Ctrl Pts',(60.1943775602019,35.0054745948108,-213.395635650738));
#218816=CARTESIAN_POINT('Ctrl Pts',(60.1555597569617,35.0633482773578,-213.393230682939));
#218817=CARTESIAN_POINT('Ctrl Pts',(60.1054112893713,35.1381149115123,-213.390123720679));
#218818=CARTESIAN_POINT('Ctrl Pts',(60.0550310847817,35.2112955200002,-213.387210565911));
#218819=CARTESIAN_POINT('Ctrl Pts',(60.0045837464213,35.2828198922257,-213.384513350095));
#218820=CARTESIAN_POINT('Ctrl Pts',(59.9742196990514,35.3258701203834,-213.382889906887));
#218821=CARTESIAN_POINT('Ctrl Pts',(59.9438303909373,35.3683210152462,-213.381344746419));
#218822=CARTESIAN_POINT('Ctrl Pts',(59.9134443065957,35.4101621769143,-213.379883144536));
#218823=CARTESIAN_POINT('Ctrl Pts',(58.6665914736623,34.7169872964315,-216.775646223557));
#218824=CARTESIAN_POINT('Ctrl Pts',(58.6670681057105,34.7163534317084,-216.775672326265));
#218825=CARTESIAN_POINT('Ctrl Pts',(58.6694802109214,34.7133058321613,-216.775702228632));
#218826=CARTESIAN_POINT('Ctrl Pts',(58.6738398478374,34.7078154007888,-216.77573593066));
#218827=CARTESIAN_POINT('Ctrl Pts',(58.6779611895904,34.7026250731325,-216.775767790554));
#218828=CARTESIAN_POINT('Ctrl Pts',(58.6838228717898,34.6952517669432,-216.775803046086));
#218829=CARTESIAN_POINT('Ctrl Pts',(58.6914531347878,34.6856286956792,-216.775841697255));
#218830=CARTESIAN_POINT('Ctrl Pts',(58.6946762133137,34.6815638404636,-216.77585802379));
#218831=CARTESIAN_POINT('Ctrl Pts',(58.6982150950876,34.6770970184521,-216.775874956201));
#218832=CARTESIAN_POINT('Ctrl Pts',(58.7020730820553,34.6722205751115,-216.775892494489));
#218833=CARTESIAN_POINT('Ctrl Pts',(58.7104004168453,34.6616949365798,-216.775930350291));
#218834=CARTESIAN_POINT('Ctrl Pts',(58.7202130485412,34.6492638479551,-216.775971028858));
#218835=CARTESIAN_POINT('Ctrl Pts',(58.7315582160844,34.6348202407144,-216.776014530189));
#218836=CARTESIAN_POINT('Ctrl Pts',(58.7356441068596,34.6296184663589,-216.776030196919));
#218837=CARTESIAN_POINT('Ctrl Pts',(58.7399289731632,34.624155238461,-216.776046229773));
#218838=CARTESIAN_POINT('Ctrl Pts',(58.7444157618656,34.6184240118923,-216.776062628748));
#218839=CARTESIAN_POINT('Ctrl Pts',(58.752888320475,34.6076015381303,-216.776093595502));
#218840=CARTESIAN_POINT('Ctrl Pts',(58.7599936864881,34.5984905903666,-216.77611896689));
#218841=CARTESIAN_POINT('Ctrl Pts',(58.766363196952,34.5903053720178,-216.776141810194));
#218842=CARTESIAN_POINT('Ctrl Pts',(58.7727327074159,34.582120153669,-216.776164653498));
#218843=CARTESIAN_POINT('Ctrl Pts',(58.7783668410405,34.5748594774657,-216.776184968719));
#218844=CARTESIAN_POINT('Ctrl Pts',(58.7839180023781,34.5676893598984,-216.776205823138));
#218845=CARTESIAN_POINT('Ctrl Pts',(58.7981566088431,34.5492981663918,-216.776259314263));
#218846=CARTESIAN_POINT('Ctrl Pts',(58.8103680803945,34.5334124046094,-216.776308259613));
#218847=CARTESIAN_POINT('Ctrl Pts',(58.8204666936249,34.5202243498463,-216.776352659188));
#218848=CARTESIAN_POINT('Ctrl Pts',(58.8261165404609,34.5128460605926,-216.776377499311));
#218849=CARTESIAN_POINT('Ctrl Pts',(58.831105290415,34.5063115020565,-216.776400916589));
#218850=CARTESIAN_POINT('Ctrl Pts',(58.8354207734538,34.5006474105254,-216.776422911022));
#218851=CARTESIAN_POINT('Ctrl Pts',(58.8430653672725,34.4906138456338,-216.776461872709));
#218852=CARTESIAN_POINT('Ctrl Pts',(58.8509803426121,34.4801753925234,-216.776514330255));
#218853=CARTESIAN_POINT('Ctrl Pts',(58.859576729319,34.4687645990523,-216.77659066946));
#218854=CARTESIAN_POINT('Ctrl Pts',(58.8645070583051,34.4622201091727,-216.776634452669));
#218855=CARTESIAN_POINT('Ctrl Pts',(58.8696618519958,34.4553550877796,-216.776686091569));
#218856=CARTESIAN_POINT('Ctrl Pts',(58.8751220460667,34.4480552757866,-216.776747545545));
#218857=CARTESIAN_POINT('Ctrl Pts',(58.8887140285765,34.4298839588616,-216.776900522043));
#218858=CARTESIAN_POINT('Ctrl Pts',(58.9035417976025,34.4099025757787,-216.777103008302));
#218859=CARTESIAN_POINT('Ctrl Pts',(58.9196893653339,34.3879363985254,-216.777355004323));
#218860=CARTESIAN_POINT('Ctrl Pts',(58.9350478981359,34.3670435768017,-216.777594686807));
#218861=CARTESIAN_POINT('Ctrl Pts',(58.9516002919803,34.344355360868,-216.777879158776));
#218862=CARTESIAN_POINT('Ctrl Pts',(58.9694406023619,34.3196790386863,-216.778208420229));
#218863=CARTESIAN_POINT('Ctrl Pts',(58.9741892585224,34.3131108026612,-216.778296061609));
#218864=CARTESIAN_POINT('Ctrl Pts',(58.9790292925856,34.3064014597548,-216.778386876301));
#218865=CARTESIAN_POINT('Ctrl Pts',(58.9839627723711,34.2995468089717,-216.778480864304));
#218866=CARTESIAN_POINT('Ctrl Pts',(58.9886303649067,34.2930615859201,-216.778569786874));
#218867=CARTESIAN_POINT('Ctrl Pts',(58.9937888639037,34.2858763757545,-216.778670966967));
#218868=CARTESIAN_POINT('Ctrl Pts',(58.9986503973408,34.2790909006063,-216.778766669489));
#218869=CARTESIAN_POINT('Ctrl Pts',(59.0011878457208,34.275549262326,-216.77881662085));
#218870=CARTESIAN_POINT('Ctrl Pts',(59.0036439919825,34.2721173577295,-216.77886507998));
#218871=CARTESIAN_POINT('Ctrl Pts',(59.0059043510499,34.2689566585687,-216.778909525111));
#218872=CARTESIAN_POINT('Ctrl Pts',(59.0092769019573,34.2642407623304,-216.778975839117));
#218873=CARTESIAN_POINT('Ctrl Pts',(59.0122136252413,34.2601285170381,-216.779033217198));
#218874=CARTESIAN_POINT('Ctrl Pts',(59.0143297408352,34.2571655299183,-216.779073283126));
#218875=CARTESIAN_POINT('Ctrl Pts',(59.0205814042945,34.2484119446414,-216.779191650335));
#218876=CARTESIAN_POINT('Ctrl Pts',(59.0269902590843,34.2394421233898,-216.779297323683));
#218877=CARTESIAN_POINT('Ctrl Pts',(59.0335603692097,34.230245789034,-216.779390226452));
#218878=CARTESIAN_POINT('Ctrl Pts',(59.0467005894606,34.2118531203223,-216.779576031989));
#218879=CARTESIAN_POINT('Ctrl Pts',(59.0604859975106,34.1925545204065,-216.779710952715));
#218880=CARTESIAN_POINT('Ctrl Pts',(59.0749542980427,34.1722521293946,-216.779794966433));
#218881=CARTESIAN_POINT('Ctrl Pts',(59.0928834858082,34.1470933085825,-216.779899076638));
#218882=CARTESIAN_POINT('Ctrl Pts',(59.1118608905283,34.1203946818412,-216.779925012753));
#218883=CARTESIAN_POINT('Ctrl Pts',(59.1319699799244,34.0919293325671,-216.779872774776));
#218884=CARTESIAN_POINT('Ctrl Pts',(59.1515521564952,34.0642098528504,-216.779821905577));
#218885=CARTESIAN_POINT('Ctrl Pts',(59.1722074420135,34.034815269011,-216.779696905362));
#218886=CARTESIAN_POINT('Ctrl Pts',(59.1940260470494,34.00348904357,-216.77949777413));
#218887=CARTESIAN_POINT('Ctrl Pts',(59.2150912904043,33.9732444627997,-216.779305518583));
#218888=CARTESIAN_POINT('Ctrl Pts',(59.2372408851721,33.9411994683062,-216.779044162892));
#218889=CARTESIAN_POINT('Ctrl Pts',(59.2605688679621,33.9070761502832,-216.778713707057));
#218890=CARTESIAN_POINT('Ctrl Pts',(59.2683576234456,33.8956830442971,-216.778603374341));
#218891=CARTESIAN_POINT('Ctrl Pts',(59.2762778514711,33.8840578464883,-216.77848533861));
#218892=CARTESIAN_POINT('Ctrl Pts',(59.2843333938043,33.8721889432235,-216.778359599865));
#218893=CARTESIAN_POINT('Ctrl Pts',(59.2946877417116,33.8569330177253,-216.778197979125));
#218894=CARTESIAN_POINT('Ctrl Pts',(59.3052656351694,33.8412745138219,-216.778023631672));
#218895=CARTESIAN_POINT('Ctrl Pts',(59.3160756783319,33.825187105161,-216.777836559618));
#218896=CARTESIAN_POINT('Ctrl Pts',(59.3214806999131,33.8171434008306,-216.777743023591));
#218897=CARTESIAN_POINT('Ctrl Pts',(59.3269437546586,33.8089924675107,-216.777646301599));
#218898=CARTESIAN_POINT('Ctrl Pts',(59.3324659843164,33.8007307931777,-216.777546401141));
#218899=CARTESIAN_POINT('Ctrl Pts',(59.336148956312,33.7952207877831,-216.777479773962));
#218900=CARTESIAN_POINT('Ctrl Pts',(59.3386313887352,33.7914980545715,-216.77743462791));
#218901=CARTESIAN_POINT('Ctrl Pts',(59.3409419466165,33.788029764492,-216.777393081159));
#218902=CARTESIAN_POINT('Ctrl Pts',(59.3420958275834,33.7862977178972,-216.777372332921));
#218903=CARTESIAN_POINT('Ctrl Pts',(59.3432071719571,33.7846282449242,-216.777352482332));
#218904=CARTESIAN_POINT('Ctrl Pts',(59.3444056335457,33.7828262864623,-216.777331302268));
#218905=CARTESIAN_POINT('Ctrl Pts',(59.3587987884887,33.7611853197513,-216.777076936214));
#218906=CARTESIAN_POINT('Ctrl Pts',(59.3733313547227,33.7391229883341,-216.776840546535));
#218907=CARTESIAN_POINT('Ctrl Pts',(59.3880081141125,33.7166181250504,-216.776622133232));
#218908=CARTESIAN_POINT('Ctrl Pts',(59.3968408863624,33.7030742406942,-216.776490687664));
#218909=CARTESIAN_POINT('Ctrl Pts',(59.4057258834763,33.689370076979,-216.776365752919));
#218910=CARTESIAN_POINT('Ctrl Pts',(59.414664146579,33.6755010224523,-216.776247328996));
#218911=CARTESIAN_POINT('Ctrl Pts',(59.4354299748332,33.6432797283332,-216.775972200504));
#218912=CARTESIAN_POINT('Ctrl Pts',(59.4564833090992,33.6101684309622,-216.775732214143));
#218913=CARTESIAN_POINT('Ctrl Pts',(59.4777543001217,33.5762439212329,-216.775527369912));
#218914=CARTESIAN_POINT('Ctrl Pts',(59.5386076841382,33.4791905579952,-216.7749413387));
#218915=CARTESIAN_POINT('Ctrl Pts',(59.6012426021026,33.3754811362627,-216.774642929323));
#218916=CARTESIAN_POINT('Ctrl Pts',(59.6640221266443,33.2669168310396,-216.774632140179));
#218917=CARTESIAN_POINT('Ctrl Pts',(59.6954118889152,33.2126346784281,-216.774626745607));
#218918=CARTESIAN_POINT('Ctrl Pts',(59.7268378070652,33.1571388073496,-216.774693260578));
#218919=CARTESIAN_POINT('Ctrl Pts',(59.7580951362872,33.1006547607048,-216.774831677976));
#218920=CARTESIAN_POINT('Ctrl Pts',(59.7624935951323,33.0927064567148,-216.774851155751));
#218921=CARTESIAN_POINT('Ctrl Pts',(59.7675147142201,33.0835960625502,-216.774877767774));
#218922=CARTESIAN_POINT('Ctrl Pts',(59.771546136366,33.0762626462417,-216.77489833135));
#218923=CARTESIAN_POINT('Ctrl Pts',(59.7746769665955,33.0705674645828,-216.774914301164));
#218924=CARTESIAN_POINT('Ctrl Pts',(59.7772112214269,33.0659462300852,-216.774926623049));
#218925=CARTESIAN_POINT('Ctrl Pts',(59.7783965726506,33.0637901480713,-216.774929122416));
#218926=CARTESIAN_POINT('Ctrl Pts',(59.7811082446338,33.0588577811293,-216.774934840101));
#218927=CARTESIAN_POINT('Ctrl Pts',(59.7843039578434,33.0530748594205,-216.774921261397));
#218928=CARTESIAN_POINT('Ctrl Pts',(59.787982068665,33.0464338395745,-216.774888013666));
#218929=CARTESIAN_POINT('Ctrl Pts',(59.7953382903084,33.0331517998827,-216.774821518205));
#218930=CARTESIAN_POINT('Ctrl Pts',(59.8046250197526,33.016437872032,-216.77467730494));
#218931=CARTESIAN_POINT('Ctrl Pts',(59.8158139222979,32.9962087252168,-216.774455267294));
#218932=CARTESIAN_POINT('Ctrl Pts',(59.8273746215905,32.9753073828081,-216.774225851545));
#218933=CARTESIAN_POINT('Ctrl Pts',(59.8409673874441,32.9506520965263,-216.773913353466));
#218934=CARTESIAN_POINT('Ctrl Pts',(59.8565272281041,32.9221349455562,-216.773517773058));
#218935=CARTESIAN_POINT('Ctrl Pts',(59.8668775326413,32.9031655226989,-216.77325463555));
#218936=CARTESIAN_POINT('Ctrl Pts',(59.8780975533821,32.8824869344996,-216.772954735577));
#218937=CARTESIAN_POINT('Ctrl Pts',(59.890155046688,32.86006864128,-216.772618073137));
#218938=CARTESIAN_POINT('Ctrl Pts',(59.8950579505909,32.8509527550394,-216.772481177056));
#218939=CARTESIAN_POINT('Ctrl Pts',(59.9000991622126,32.8415492682111,-216.772338202461));
#218940=CARTESIAN_POINT('Ctrl Pts',(59.905276601872,32.8318558217261,-216.772189149354));
#218941=CARTESIAN_POINT('Ctrl Pts',(59.923802279304,32.7971711755308,-216.771655814354));
#218942=CARTESIAN_POINT('Ctrl Pts',(59.9440745976445,32.7587734499515,-216.771044655015));
#218943=CARTESIAN_POINT('Ctrl Pts',(59.9659784543963,32.7165579454281,-216.770355671337));
#218944=CARTESIAN_POINT('Ctrl Pts',(59.9785736797882,32.6922830517175,-216.769959489751));
#218945=CARTESIAN_POINT('Ctrl Pts',(59.9897140153398,32.6705908525983,-216.769604001407));
#218946=CARTESIAN_POINT('Ctrl Pts',(60.0001226521558,32.6501730512935,-216.769272192519));
#218947=CARTESIAN_POINT('Ctrl Pts',(60.0078152626543,32.6350830644442,-216.769026965734));
#218948=CARTESIAN_POINT('Ctrl Pts',(60.0151073907883,32.6206878929927,-216.768794672909));
#218949=CARTESIAN_POINT('Ctrl Pts',(60.0222799414978,32.6064454485188,-216.768568445878));
#218950=CARTESIAN_POINT('Ctrl Pts',(60.0440128353844,32.5632907122228,-216.767882975919));
#218951=CARTESIAN_POINT('Ctrl Pts',(60.0636456592396,32.5235387638354,-216.767272561604));
#218952=CARTESIAN_POINT('Ctrl Pts',(60.0812847352957,32.4873272570907,-216.766737202934));
#218953=CARTESIAN_POINT('Ctrl Pts',(60.0910422583728,32.4672959010496,-216.766441055077));
#218954=CARTESIAN_POINT('Ctrl Pts',(60.1001895698892,32.4483469042561,-216.766167874568));
#218955=CARTESIAN_POINT('Ctrl Pts',(60.1087433600541,32.4304970192806,-216.765917661409));
#218956=CARTESIAN_POINT('Ctrl Pts',(60.120751774401,32.4054380909345,-216.765566394517));
#218957=CARTESIAN_POINT('Ctrl Pts',(60.1315907220463,32.3825457742647,-216.765260392976));
#218958=CARTESIAN_POINT('Ctrl Pts',(60.1413019208989,32.3618542151778,-216.764999703275));
#218959=CARTESIAN_POINT('Ctrl Pts',(60.1461575203253,32.3515084356343,-216.764869358425));
#218960=CARTESIAN_POINT('Ctrl Pts',(60.1507310984236,32.34171280714,-216.764750259777));
#218961=CARTESIAN_POINT('Ctrl Pts',(60.1550272753044,32.3324703279183,-216.764642510907));
#218962=CARTESIAN_POINT('Ctrl Pts',(60.1571753637447,32.3278490883075,-216.764588636472));
#218963=CARTESIAN_POINT('Ctrl Pts',(60.1592540966846,32.3233661336264,-216.764537594417));
#218964=CARTESIAN_POINT('Ctrl Pts',(60.1612640098706,32.3190218110534,-216.764489384796));
#218965=CARTESIAN_POINT('Ctrl Pts',(60.1632739230566,32.3146774884804,-216.764441175175));
#218966=CARTESIAN_POINT('Ctrl Pts',(60.1643981239921,32.3122456819017,-216.764414355239));
#218967=CARTESIAN_POINT('Ctrl Pts',(60.1670878018744,32.3064050638589,-216.764353243169));
#218968=CARTESIAN_POINT('Ctrl Pts',(60.2018664146461,32.2308835322313,-216.763563039623));
#218969=CARTESIAN_POINT('Ctrl Pts',(60.2364926227202,32.1536653398071,-216.762652288959));
#218970=CARTESIAN_POINT('Ctrl Pts',(60.2707822025251,32.0749362568614,-216.761620991176));
#218971=CARTESIAN_POINT('Ctrl Pts',(60.2901586062156,32.030447916613,-216.761038223984));
#218972=CARTESIAN_POINT('Ctrl Pts',(60.3094271217391,31.9854779357794,-216.760416964048));
#218973=CARTESIAN_POINT('Ctrl Pts',(60.3285512744986,31.9400665097129,-216.75975721137));
#218974=CARTESIAN_POINT('Ctrl Pts',(60.3668652508642,31.8490877182901,-216.758435440475));
#218975=CARTESIAN_POINT('Ctrl Pts',(60.4045983421644,31.7563428873234,-216.756959169431));
#218976=CARTESIAN_POINT('Ctrl Pts',(60.4416544436433,31.6615857304821,-216.755328398239));
#218977=CARTESIAN_POINT('Ctrl Pts',(60.478078104031,31.5684458058176,-216.753725459621));
#218978=CARTESIAN_POINT('Ctrl Pts',(60.513847627481,31.4733618155951,-216.751973249597));
#218979=CARTESIAN_POINT('Ctrl Pts',(60.5488797035791,31.3760505696478,-216.750071768167));
#218980=CARTESIAN_POINT('Ctrl Pts',(60.5831095211231,31.2809678179308,-216.748213831966));
#218981=CARTESIAN_POINT('Ctrl Pts',(60.6166352373989,31.183758742476,-216.746213382909));
#218982=CARTESIAN_POINT('Ctrl Pts',(60.649387527739,31.0841099747386,-216.744070420997));
#218983=CARTESIAN_POINT('Ctrl Pts',(60.6594381189747,31.0535310741102,-216.743412817086));
#218984=CARTESIAN_POINT('Ctrl Pts',(60.6694159421373,31.0227220726697,-216.742741793132));
#218985=CARTESIAN_POINT('Ctrl Pts',(60.6793191674292,30.9916729347315,-216.742057349136));
#218986=CARTESIAN_POINT('Ctrl Pts',(60.704438687947,30.9129168290677,-216.740321257659));
#218987=CARTESIAN_POINT('Ctrl Pts',(60.7290793248211,30.8326114173318,-216.738498823948));
#218988=CARTESIAN_POINT('Ctrl Pts',(60.7531045634047,30.7510497143758,-216.736590048002));
#218989=CARTESIAN_POINT('Ctrl Pts',(60.7768402186365,30.6704710989022,-216.734704279101));
#218990=CARTESIAN_POINT('Ctrl Pts',(60.7999752420945,30.5886661793071,-216.732734236839));
#218991=CARTESIAN_POINT('Ctrl Pts',(60.8223658568759,30.505966038184,-216.730679921216));
#218992=CARTESIAN_POINT('Ctrl Pts',(60.8443315930004,30.424835194073,-216.728664587767));
#218993=CARTESIAN_POINT('Ctrl Pts',(60.8655809084215,30.3428427332773,-216.726568148913));
#218994=CARTESIAN_POINT('Ctrl Pts',(60.8859661387063,30.2603493499802,-216.724390604653));
#218995=CARTESIAN_POINT('Ctrl Pts',(60.905775148304,30.1801877722767,-216.722274612115));
#218996=CARTESIAN_POINT('Ctrl Pts',(60.924768216205,30.0995532287051,-216.720082034513));
#218997=CARTESIAN_POINT('Ctrl Pts',(60.9427985975151,30.018822490257,-216.717812871847));
#218998=CARTESIAN_POINT('Ctrl Pts',(60.9628078301142,29.929231477415,-216.715294666445));
#218999=CARTESIAN_POINT('Ctrl Pts',(60.981629326843,29.8395226647074,-216.712682142926));
#219000=CARTESIAN_POINT('Ctrl Pts',(60.9992577262092,29.7501026756727,-216.709975301288));
#219001=CARTESIAN_POINT('Ctrl Pts',(61.0089023416902,29.7011804001644,-216.70849437008));
#219002=CARTESIAN_POINT('Ctrl Pts',(61.0181900345037,29.6523454397984,-216.706985207031));
#219003=CARTESIAN_POINT('Ctrl Pts',(61.0271214515743,29.6036708476852,-216.705447812141));
#219004=CARTESIAN_POINT('Ctrl Pts',(59.4999643211654,35.9450057402374,-213.371639708519));
#219005=CARTESIAN_POINT('Ctrl Pts',(59.4820528027665,35.9125166648153,-215.346308247144));
#219006=CARTESIAN_POINT('Ctrl Pts',(58.4265182736836,35.031835198701,-216.764384131257));
#219007=CARTESIAN_POINT('Ctrl Pts',(59.6440986517757,35.7696968033851,-213.370755972398));
#219008=CARTESIAN_POINT('Ctrl Pts',(59.6013542567595,35.7669646494558,-215.346152352702));
#219009=CARTESIAN_POINT('Ctrl Pts',(58.510163538665,34.9284713760201,-216.764533686556));
#219010=CARTESIAN_POINT('Ctrl Pts',(59.7818407313688,35.5913782362947,-213.373552880528));
#219011=CARTESIAN_POINT('Ctrl Pts',(59.7162237024563,35.619624715777,-215.350089533734));
#219012=CARTESIAN_POINT('Ctrl Pts',(58.5901397589686,34.8235003567024,-216.76833687912));
#219013=CARTESIAN_POINT('Ctrl Pts',(59.9134443065991,35.4101621769129,-213.379883144535));
#219014=CARTESIAN_POINT('Ctrl Pts',(59.8268417476681,35.4705704696998,-215.357954892849));
#219015=CARTESIAN_POINT('Ctrl Pts',(58.6665914736623,34.7169872964315,-216.775646223556));
#219016=CARTESIAN_POINT('',(58.4265182736835,35.0318351987012,-216.764384131257));
#219017=CARTESIAN_POINT('',(59.4999643211654,35.9450057402376,-213.371639708519));
#219018=CARTESIAN_POINT('Origin',(55.6381166865346,32.7703375395218,-213.284377676332));
#219019=CARTESIAN_POINT('Origin',(52.7506200812507,30.3721960348575,-218.064222059651));
#219020=CARTESIAN_POINT('Origin',(55.6093041609777,32.7570348813246,-220.18888881869));
#219021=CARTESIAN_POINT('Ctrl Pts',(58.4265182736835,35.0318351987011,-216.764384131257));
#219022=CARTESIAN_POINT('Ctrl Pts',(59.4820528027664,35.9125166648155,-215.346308247144));
#219023=CARTESIAN_POINT('Ctrl Pts',(59.4999643211654,35.9450057402375,-213.371639708519));
#219024=CARTESIAN_POINT('Ctrl Pts',(57.5486529224426,36.1166487545749,-216.76281454263));
#219025=CARTESIAN_POINT('Ctrl Pts',(58.5785030826818,37.0120312881232,-215.346864153326));
#219026=CARTESIAN_POINT('Ctrl Pts',(58.5926451028776,37.0484655333588,-213.380920503252));
#219027=CARTESIAN_POINT('Ctrl Pts',(56.6223825642191,37.1990499756784,-216.761500614409));
#219028=CARTESIAN_POINT('Ctrl Pts',(57.6304520413514,38.1023651317007,-215.347861259707));
#219029=CARTESIAN_POINT('Ctrl Pts',(57.6483853099758,38.1336349814895,-213.391180664313));
#219030=CARTESIAN_POINT('Ctrl Pts',(55.6813080372829,38.2352492592495,-216.760202274403));
#219031=CARTESIAN_POINT('Ctrl Pts',(56.6650296771562,39.1519706625638,-215.348455523392));
#219032=CARTESIAN_POINT('Ctrl Pts',(56.682191157046,39.1835711849515,-213.399142265953));
#219033=CARTESIAN_POINT('Ctrl Pts',(59.4999643211654,35.9450057402376,-213.371639708519));
#219034=CARTESIAN_POINT('Ctrl Pts',(59.3530691590842,36.1236561004343,-213.373142271034));
#219035=CARTESIAN_POINT('Ctrl Pts',(59.2112226056842,36.2945126600292,-213.374608432805));
#219036=CARTESIAN_POINT('Ctrl Pts',(59.0746685317258,36.4576720204601,-213.376021791858));
#219037=CARTESIAN_POINT('Ctrl Pts',(58.9328872802121,36.6270769869141,-213.377489253132));
#219038=CARTESIAN_POINT('Ctrl Pts',(58.796811282469,36.7881845701405,-213.378899850635));
#219039=CARTESIAN_POINT('Ctrl Pts',(58.6666613429046,36.9411232025734,-213.380242059925));
#219040=CARTESIAN_POINT('Ctrl Pts',(58.5286621778041,37.1032854260672,-213.381665216648));
#219041=CARTESIAN_POINT('Ctrl Pts',(58.3973253842116,37.2562640920389,-213.383011540957));
#219042=CARTESIAN_POINT('Ctrl Pts',(58.2728579280455,37.4002283770448,-213.384273976912));
#219043=CARTESIAN_POINT('Ctrl Pts',(58.1439265508173,37.5493558205486,-213.385581689076));
#219044=CARTESIAN_POINT('Ctrl Pts',(58.0223657791532,37.6888112780918,-213.386799480846));
#219045=CARTESIAN_POINT('Ctrl Pts',(57.9083499192908,37.8187915053139,-213.387925278214));
#219046=CARTESIAN_POINT('Ctrl Pts',(57.7890456668349,37.9548005996757,-213.389103293391));
#219047=CARTESIAN_POINT('Ctrl Pts',(57.6780022225769,38.080435763234,-213.390180681546));
#219048=CARTESIAN_POINT('Ctrl Pts',(57.5753634650057,38.1959220404739,-213.391159767909));
#219049=CARTESIAN_POINT('Ctrl Pts',(57.5666424872746,38.205734642223,-213.391242958612));
#219050=CARTESIAN_POINT('Ctrl Pts',(57.5579821567034,38.2154739702272,-213.391325441773));
#219051=CARTESIAN_POINT('Ctrl Pts',(57.54938254494,38.2251401600279,-213.391407219936));
#219052=CARTESIAN_POINT('Ctrl Pts',(57.4434126431882,38.3442531167146,-213.392414942629));
#219053=CARTESIAN_POINT('Ctrl Pts',(57.3467222359999,38.4521993238965,-213.393315003254));
#219054=CARTESIAN_POINT('Ctrl Pts',(57.2595019988215,38.5491319021046,-213.394112818152));
#219055=CARTESIAN_POINT('Ctrl Pts',(57.1707868735558,38.6477258304891,-213.394924306987));
#219056=CARTESIAN_POINT('Ctrl Pts',(57.0918688820637,38.7349261105185,-213.395630140928));
#219057=CARTESIAN_POINT('Ctrl Pts',(57.0229004219518,38.8108710912233,-213.396237430413));
#219058=CARTESIAN_POINT('Ctrl Pts',(56.9539806056297,38.8867625075645,-213.396844291575));
#219059=CARTESIAN_POINT('Ctrl Pts',(56.8949958287087,38.9514150403455,-213.39735285088));
#219060=CARTESIAN_POINT('Ctrl Pts',(56.846057438065,39.0049345300186,-213.397769859768));
#219061=CARTESIAN_POINT('Ctrl Pts',(56.7974487746849,39.0580934268187,-213.398184059017));
#219062=CARTESIAN_POINT('Ctrl Pts',(56.758751223571,39.1002691381783,-213.398508007919));
#219063=CARTESIAN_POINT('Ctrl Pts',(56.7300398301481,39.1315270272855,-213.398746686664));
#219064=CARTESIAN_POINT('Ctrl Pts',(56.718140259053,39.1444820054098,-213.398845608184));
#219065=CARTESIAN_POINT('Ctrl Pts',(56.7079556605156,39.1555611147679,-213.398929857286));
#219066=CARTESIAN_POINT('Ctrl Pts',(56.6994898314762,39.1647668800231,-213.398999668388));
#219067=CARTESIAN_POINT('Origin',(55.9211377566494,34.484843995799,-216.774150960848));
#219068=CARTESIAN_POINT('Ctrl Pts',(-33.195117167568,-74.788972786398,-216.360364163614));
#219069=CARTESIAN_POINT('Ctrl Pts',(-33.5111161912263,-75.4317844535893,
-215.275130706023));
#219070=CARTESIAN_POINT('Ctrl Pts',(-33.8499480590156,-75.4429517542805,
-214.019797229742));
#219071=CARTESIAN_POINT('Ctrl Pts',(-32.6155847805473,-74.7878402293263,
-216.243940775302));
#219072=CARTESIAN_POINT('Ctrl Pts',(-32.8892442190157,-75.4538060704667,
-215.132352055413));
#219073=CARTESIAN_POINT('Ctrl Pts',(-33.1824288617165,-75.4672690607831,
-213.840684379537));
#219074=CARTESIAN_POINT('Ctrl Pts',(-32.0212270237052,-74.7863264493868,
-216.159798603417));
#219075=CARTESIAN_POINT('Ctrl Pts',(-32.2560519535044,-75.4749926756692,
-215.02671038484));
#219076=CARTESIAN_POINT('Ctrl Pts',(-32.5054567082896,-75.490529408973,
-213.70327768978));
#219077=CARTESIAN_POINT('Ctrl Pts',(-30.8096077807694,-74.7834423664695,
-216.044618097811));
#219078=CARTESIAN_POINT('Ctrl Pts',(-30.9708520272369,-75.5157273627552,
-214.874910704589));
#219079=CARTESIAN_POINT('Ctrl Pts',(-31.1363635597063,-75.5350116089517,
-213.495389670921));
#219080=CARTESIAN_POINT('Ctrl Pts',(-30.1906743701442,-74.7820017193782,
-216.013777891697));
#219081=CARTESIAN_POINT('Ctrl Pts',(-30.3169577787275,-75.5353200743763,
-214.829020724472));
#219082=CARTESIAN_POINT('Ctrl Pts',(-30.4420278504982,-75.5562948594353,
-213.424911104697));
#219083=CARTESIAN_POINT('Ctrl Pts',(-28.3231908545672,-74.7775797475947,
-215.993570943196));
#219084=CARTESIAN_POINT('Ctrl Pts',(-28.3468574989069,-75.5911225591905,
-214.770729972352));
#219085=CARTESIAN_POINT('Ctrl Pts',(-28.3564670829161,-75.6166161717328,
-213.301750622476));
#219086=CARTESIAN_POINT('Ctrl Pts',(-27.0679344027315,-74.7746484451523,
-216.074360875667));
#219087=CARTESIAN_POINT('Ctrl Pts',(-27.0307252020175,-75.6241519763574,
-214.8360616272));
#219088=CARTESIAN_POINT('Ctrl Pts',(-26.9668397448124,-75.6520766916683,
-213.334864912836));
#219089=CARTESIAN_POINT('Ctrl Pts',(-25.4972121053677,-74.7680761663345,
-216.277655442628));
#219090=CARTESIAN_POINT('Ctrl Pts',(-25.3875902558758,-75.660467613276,
-215.025917676458));
#219091=CARTESIAN_POINT('Ctrl Pts',(-25.2304946712801,-75.69095341109,-213.493045368148));
#219092=CARTESIAN_POINT('Ctrl Pts',(-25.1829211564315,-74.7666138888157,
-216.323526964491));
#219093=CARTESIAN_POINT('Ctrl Pts',(-25.0584884038483,-75.667492051274,
-215.069507359353));
#219094=CARTESIAN_POINT('Ctrl Pts',(-24.8832331864634,-75.6984545252065,
-213.530658916364));
#219095=CARTESIAN_POINT('Ctrl Pts',(-24.7112938709068,-74.7641811379905,
-216.400031379012));
#219096=CARTESIAN_POINT('Ctrl Pts',(-24.5649041979751,-75.677656913773,
-215.143052185656));
#219097=CARTESIAN_POINT('Ctrl Pts',(-24.3623518852465,-75.7092984574834,
-213.595842802549));
#219098=CARTESIAN_POINT('Ctrl Pts',(-24.5540530570477,-74.7633303755955,
-216.426816063351));
#219099=CARTESIAN_POINT('Ctrl Pts',(-24.4003337914636,-75.6809842523408,
-215.168937491766));
#219100=CARTESIAN_POINT('Ctrl Pts',(-24.1887266067715,-75.7128451348644,
-213.619031941073));
#219101=CARTESIAN_POINT('Ctrl Pts',(-24.3771247109268,-74.7623270196362,
-216.458383475085));
#219102=CARTESIAN_POINT('Ctrl Pts',(-24.2152221662776,-75.6846576265878,
-215.199574868406));
#219103=CARTESIAN_POINT('Ctrl Pts',(-23.993400190719,-75.7167589553957,
-213.646748365346));
#219104=CARTESIAN_POINT('Ctrl Pts',(-24.3524265920656,-74.7640480279028,
-216.460210032117));
#219105=CARTESIAN_POINT('Ctrl Pts',(-24.1918224422937,-75.685150167527,
-215.201759610203));
#219106=CARTESIAN_POINT('Ctrl Pts',(-23.971697273502,-75.7171928640745,
-213.64984499144));
#219107=CARTESIAN_POINT('Ctrl Pts',(-24.3044381111283,-74.7669661611978,
-216.464262972695));
#219108=CARTESIAN_POINT('Ctrl Pts',(-24.145811351019,-75.686111198423,-215.206400261357));
#219109=CARTESIAN_POINT('Ctrl Pts',(-23.9282912658856,-75.7180607732476,
-213.655957300462));
#219110=CARTESIAN_POINT('Ctrl Pts',(-24.2804399390943,-74.768422067462,
-216.466265094574));
#219111=CARTESIAN_POINT('Ctrl Pts',(-24.122804155314,-75.6865914263234,
-215.208696671395));
#219112=CARTESIAN_POINT('Ctrl Pts',(-23.9065882035168,-75.7184945038463,
-213.65898840561));
#219113=CARTESIAN_POINT('Ctrl Pts',(-24.2084335919611,-74.7727802747408,
-216.472197988386));
#219114=CARTESIAN_POINT('Ctrl Pts',(-24.0537812020154,-75.6880311791424,
-215.215513350447));
#219115=CARTESIAN_POINT('Ctrl Pts',(-23.8414788399347,-75.7197950312437,
-213.668006138953));
#219116=CARTESIAN_POINT('Ctrl Pts',(-24.1604135896905,-74.7756730640264,
-216.476055288949));
#219117=CARTESIAN_POINT('Ctrl Pts',(-24.007756858606,-75.6889899241308,
-215.21996181218));
#219118=CARTESIAN_POINT('Ctrl Pts',(-23.7980723622357,-75.7206611636291,
-213.673917185906));
#219119=CARTESIAN_POINT('Ctrl Pts',(-24.0163059872845,-74.7843131366596,
-216.487329869079));
#219120=CARTESIAN_POINT('Ctrl Pts',(-23.8696780681879,-75.6918624958728,
-215.233013550851));
#219121=CARTESIAN_POINT('Ctrl Pts',(-23.6678522169305,-75.7232569640359,
-213.691344507444));
#219122=CARTESIAN_POINT('Ctrl Pts',(-23.9201708060206,-74.790022125549,
-216.494449836486));
#219123=CARTESIAN_POINT('Ctrl Pts',(-23.7775889862671,-75.693773263006,
-215.24132615917));
#219124=CARTESIAN_POINT('Ctrl Pts',(-23.5810378370742,-75.7249840351277,
-213.702554973155));
#219125=CARTESIAN_POINT('Ctrl Pts',(-23.0543761384816,-74.8409373246843,
-216.55487821878));
#219126=CARTESIAN_POINT('Ctrl Pts',(-22.9496972317124,-75.7109072613411,
-215.31244750849));
#219127=CARTESIAN_POINT('Ctrl Pts',(-22.7996997171921,-75.7404979925406,
-213.799694500261));
#219128=CARTESIAN_POINT('Ctrl Pts',(-22.2802129953757,-74.8830149514975,
-216.582469365009));
#219129=CARTESIAN_POINT('Ctrl Pts',(-22.2105077358072,-75.7258946484434,
-215.350200325304));
#219130=CARTESIAN_POINT('Ctrl Pts',(-22.1051150671109,-75.7540771354417,
-213.859339381341));
#219131=CARTESIAN_POINT('Ctrl Pts',(-19.9480374324794,-74.9971174078387,
-216.573710635787));
#219132=CARTESIAN_POINT('Ctrl Pts',(-19.9923615170938,-75.7701462160935,
-215.372355885965));
#219133=CARTESIAN_POINT('Ctrl Pts',(-20.0211481644292,-75.7944435076961,
-213.943127994586));
#219134=CARTESIAN_POINT('Ctrl Pts',(-18.3784534462325,-75.0569932128216,
-216.444004457652));
#219135=CARTESIAN_POINT('Ctrl Pts',(-18.5026050448183,-75.7989293347893,
-215.264664590274));
#219136=CARTESIAN_POINT('Ctrl Pts',(-18.6315506331755,-75.820882116255,
-213.870845873572));
#219137=CARTESIAN_POINT('Ctrl Pts',(-16.4159929405093,-75.1060693071363,
-216.099784138263));
#219138=CARTESIAN_POINT('Ctrl Pts',(-16.6428565698784,-75.8341980922607,
-214.945032036074));
#219139=CARTESIAN_POINT('Ctrl Pts',(-16.8941304191336,-75.8539663905531,
-213.584247821028));
#219140=CARTESIAN_POINT('Ctrl Pts',(-16.0234311669877,-75.1146217816123,
-216.021999801869));
#219141=CARTESIAN_POINT('Ctrl Pts',(-16.2709049660166,-75.8412164523101,
-214.872036381481));
#219142=CARTESIAN_POINT('Ctrl Pts',(-16.5465119853673,-75.8605843548391,
-213.517253116689));
#219143=CARTESIAN_POINT('Ctrl Pts',(-15.5821111183439,-75.1228293554344,
-215.924370829589));
#219144=CARTESIAN_POINT('Ctrl Pts',(-15.8527737534803,-75.8490693606545,
-214.779617569726));
#219145=CARTESIAN_POINT('Ctrl Pts',(-16.1557115150513,-75.8680259655566,
-213.430908966255));
#219146=CARTESIAN_POINT('Ctrl Pts',(-15.5330836643943,-75.1237216024415,
-215.913383521458));
#219147=CARTESIAN_POINT('Ctrl Pts',(-15.80632185682,-75.8499412604403,-214.76920653716));
#219148=CARTESIAN_POINT('Ctrl Pts',(-16.1122963714596,-75.8688526965665,
-213.421163614009));
#219149=CARTESIAN_POINT('Ctrl Pts',(-15.4595543784234,-75.1250304693475,
-215.89669284964));
#219150=CARTESIAN_POINT('Ctrl Pts',(-15.7366548093111,-75.8512481475662,
-214.753376392039));
#219151=CARTESIAN_POINT('Ctrl Pts',(-16.0471843630155,-75.8700926288146,
-213.406318025322));
#219152=CARTESIAN_POINT('Ctrl Pts',(-15.4428346873128,-75.1249802811429,
-215.893460636911));
#219153=CARTESIAN_POINT('Ctrl Pts',(-15.717616990686,-75.8515973969198,
-214.749400339868));
#219154=CARTESIAN_POINT('Ctrl Pts',(-16.0254808327191,-75.8705054473464,
-213.40135933222));
#219155=CARTESIAN_POINT('Ctrl Pts',(-15.4044488780932,-75.1251858633582,
-215.885607154577));
#219156=CARTESIAN_POINT('Ctrl Pts',(-15.6768826779187,-75.8523475797937,
-214.740718555761));
#219157=CARTESIAN_POINT('Ctrl Pts',(-15.9820686541031,-75.8713279510056,
-213.391549918843));
#219158=CARTESIAN_POINT('Ctrl Pts',(-15.3852505461376,-75.125287706196,
-215.881710069587));
#219159=CARTESIAN_POINT('Ctrl Pts',(-15.6565119316422,-75.8527215830931,
-214.736409774352));
#219160=CARTESIAN_POINT('Ctrl Pts',(-15.9603609089925,-75.8717379561663,
-213.386680086228));
#219161=CARTESIAN_POINT('Ctrl Pts',(-15.2892320910633,-75.1257922165004,
-215.862372207289));
#219162=CARTESIAN_POINT('Ctrl Pts',(-15.554636473512,-75.8545862406554,
-214.71502472581));
#219163=CARTESIAN_POINT('Ctrl Pts',(-15.8518139508743,-75.8737817636487,
-213.362504307539));
#219164=CARTESIAN_POINT('Ctrl Pts',(-15.2123315921028,-75.1261807769495,
-215.84737406594));
#219165=CARTESIAN_POINT('Ctrl Pts',(-15.4730825113387,-75.8560605251818,
-214.698428383582));
#219166=CARTESIAN_POINT('Ctrl Pts',(-15.7649500436515,-75.8753969121213,
-213.343718445522));
#219167=CARTESIAN_POINT('Ctrl Pts',(-14.9813854912302,-75.1273026315548,
-215.803769736317));
#219168=CARTESIAN_POINT('Ctrl Pts',(-15.228245061749,-75.8604317832489,
-214.650138423064));
#219169=CARTESIAN_POINT('Ctrl Pts',(-15.5042810069002,-75.8801832140909,
-213.288988999601));
#219170=CARTESIAN_POINT('Ctrl Pts',(-14.8270954714867,-75.1279921494453,
-215.776553069533));
#219171=CARTESIAN_POINT('Ctrl Pts',(-15.0648116368335,-75.8632766913161,
-214.619948856185));
#219172=CARTESIAN_POINT('Ctrl Pts',(-15.3303985992444,-75.8832952367866,
-213.254672773818));
#219173=CARTESIAN_POINT('Ctrl Pts',(-14.0541706789573,-75.1311620007791,
-215.649419407507));
#219174=CARTESIAN_POINT('Ctrl Pts',(-14.246396511414,-75.8771638537659,
-214.478590791259));
#219175=CARTESIAN_POINT('Ctrl Pts',(-14.4604916971159,-75.8984676315696,
-213.093510431314));
#219176=CARTESIAN_POINT('Ctrl Pts',(-13.431184632244,-75.132817249281,-215.576219198929));
#219177=CARTESIAN_POINT('Ctrl Pts',(-13.5887407903827,-75.8871770758808,
-214.396239991641));
#219178=CARTESIAN_POINT('Ctrl Pts',(-13.7629914808672,-75.909367896352,
-212.997732926983));
#219179=CARTESIAN_POINT('Ctrl Pts',(-11.5527066094476,-75.1354056675812,
-215.433716025809));
#219180=CARTESIAN_POINT('Ctrl Pts',(-11.6081515883783,-75.914047646435,
-214.231144849336));
#219181=CARTESIAN_POINT('Ctrl Pts',(-11.6663094461884,-75.9385232689356,
-212.798366319057));
#219182=CARTESIAN_POINT('Ctrl Pts',(-10.2877799376859,-75.1340135603591,
-215.440539106394));
#219183=CARTESIAN_POINT('Ctrl Pts',(-10.2793458601892,-75.927717636071,
-214.229655494057));
#219184=CARTESIAN_POINT('Ctrl Pts',(-10.2630041028497,-75.9532535042689,
-212.78151870618));
#219185=CARTESIAN_POINT('Ctrl Pts',(-8.38347923240153,-75.126649730628,
-215.593193327535));
#219186=CARTESIAN_POINT('Ctrl Pts',(-8.28003450179184,-75.941922781162,
-214.376965965048));
#219187=CARTESIAN_POINT('Ctrl Pts',(-8.15049526818619,-75.9684568916159,
-212.91497169383));
#219188=CARTESIAN_POINT('Ctrl Pts',(-7.74635347447534,-75.1232850699231,
-215.668279738107));
#219189=CARTESIAN_POINT('Ctrl Pts',(-7.61095052122154,-75.9456083422809,
-214.451585639128));
#219190=CARTESIAN_POINT('Ctrl Pts',(-7.44371915288171,-75.9723750977203,
-212.986447448666));
#219191=CARTESIAN_POINT('Ctrl Pts',(-6.7941630494427,-75.1167245643831,
-215.8171218942));
#219192=CARTESIAN_POINT('Ctrl Pts',(-6.61073165231177,-75.949511555175,
-214.601581194446));
#219193=CARTESIAN_POINT('Ctrl Pts',(-6.38618665189478,-75.9764782937961,
-213.134044386266));
#219194=CARTESIAN_POINT('Ctrl Pts',(-6.47794571480321,-75.1142884671426,
-215.872668348987));
#219195=CARTESIAN_POINT('Ctrl Pts',(-6.27842297660572,-75.9505402725157,
-214.657841670266));
#219196=CARTESIAN_POINT('Ctrl Pts',(-6.03476907566787,-75.97754871877,-213.189871250874));
#219197=CARTESIAN_POINT('Ctrl Pts',(-6.00556655574115,-75.1102319614325,
-215.964906904596));
#219198=CARTESIAN_POINT('Ctrl Pts',(-5.78184694432798,-75.9516786620228,
-214.751620845591));
#219199=CARTESIAN_POINT('Ctrl Pts',(-5.50928664215075,-75.978712818264,
-213.283577816478));
#219200=CARTESIAN_POINT('Ctrl Pts',(-5.84843151319126,-75.1088126744791,
-215.997140440631));
#219201=CARTESIAN_POINT('Ctrl Pts',(-5.61661283811424,-75.9519906782163,
-214.784451666501));
#219202=CARTESIAN_POINT('Ctrl Pts',(-5.33440000717681,-75.9790272405617,
-213.316475520459));
#219203=CARTESIAN_POINT('Ctrl Pts',(-5.65243869966684,-75.1069512163146,
-216.039300200532));
#219204=CARTESIAN_POINT('Ctrl Pts',(-5.4104807172672,-75.9522966621249,
-214.827456690397));
#219205=CARTESIAN_POINT('Ctrl Pts',(-5.1161362621178,-75.9793285596488,
-213.359686451246));
#219206=CARTESIAN_POINT('Ctrl Pts',(-5.61326165750729,-75.1065745592821,
-216.04782548518));
#219207=CARTESIAN_POINT('Ctrl Pts',(-5.36927136766082,-75.9523536622172,
-214.836156753581));
#219208=CARTESIAN_POINT('Ctrl Pts',(-5.07250098499984,-75.9793842386791,
-213.368433019225));
#219209=CARTESIAN_POINT('Ctrl Pts',(-5.55450205387992,-75.1060026905412,
-216.060759634097));
#219210=CARTESIAN_POINT('Ctrl Pts',(-5.30746024813262,-75.9524328958794,
-214.849360730742));
#219211=CARTESIAN_POINT('Ctrl Pts',(-5.00704455769206,-75.979460913428,
-213.381715900943));
#219212=CARTESIAN_POINT('Ctrl Pts',(-5.53491761156424,-75.1058109307596,
-216.065095153168));
#219213=CARTESIAN_POINT('Ctrl Pts',(-5.28685781194929,-75.9524582612829,
-214.85378754548));
#219214=CARTESIAN_POINT('Ctrl Pts',(-4.9852263867816,-75.9794853292611,
-213.386170460015));
#219215=CARTESIAN_POINT('Ctrl Pts',(-5.50554413451951,-75.1055215751752,
-216.071634702396));
#219216=CARTESIAN_POINT('Ctrl Pts',(-5.2559566454412,-75.952494739044,-214.860465953734));
#219217=CARTESIAN_POINT('Ctrl Pts',(-4.95250008958594,-75.9795202381749,
-213.392892775367));
#219218=CARTESIAN_POINT('Ctrl Pts',(-5.49575350661914,-75.1054248373341,
-216.073820597239));
#219219=CARTESIAN_POINT('Ctrl Pts',(-5.24565657882127,-75.9525066366783,
-214.862698474386));
#219220=CARTESIAN_POINT('Ctrl Pts',(-4.94159148370997,-75.9795315886736,
-213.395140293282));
#219221=CARTESIAN_POINT('Ctrl Pts',(-5.47617332109849,-75.1052307878912,
-216.078204488416));
#219222=CARTESIAN_POINT('Ctrl Pts',(-5.22505721795924,-75.9525299083859,
-214.867176270342));
#219223=CARTESIAN_POINT('Ctrl Pts',(-4.91977459201134,-75.9795537178522,
-213.399648834811));
#219224=CARTESIAN_POINT('Ctrl Pts',(-5.46775998763707,-75.1049040600624,
-216.080458414741));
#219225=CARTESIAN_POINT('Ctrl Pts',(-5.21551613357834,-75.9525365950561,
-214.869490968336));
#219226=CARTESIAN_POINT('Ctrl Pts',(-4.90886637668479,-75.979564444277,
-213.401912833547));
#219227=CARTESIAN_POINT('Ctrl Pts',(-5.35883349107929,-75.1074979249758,
-216.099458947456));
#219228=CARTESIAN_POINT('Ctrl Pts',(-5.11136656618359,-75.9527073582981,
-214.888713509689));
#219229=CARTESIAN_POINT('Ctrl Pts',(-4.81069244996574,-75.9796594680882,
-213.422289301941));
#219230=CARTESIAN_POINT('Ctrl Pts',(-5.26196254924258,-75.109746081089,
-216.115929091618));
#219231=CARTESIAN_POINT('Ctrl Pts',(-5.01875445567398,-75.9528546760428,
-214.905377832462));
#219232=CARTESIAN_POINT('Ctrl Pts',(-4.72341604058447,-75.9797411532712,
-213.43995044954));
#219233=CARTESIAN_POINT('Ctrl Pts',(-4.38966212112596,-75.129464412617,
-216.260333501036));
#219234=CARTESIAN_POINT('Ctrl Pts',(-4.1856409578542,-75.9541400040838,
-215.05137059809));
#219235=CARTESIAN_POINT('Ctrl Pts',(-3.93783085851934,-75.9804521342285,
-213.594787559664));
#219236=CARTESIAN_POINT('Ctrl Pts',(-3.61066071653182,-75.143382837027,
-216.361345807815));
#219237=CARTESIAN_POINT('Ctrl Pts',(-3.44231755118432,-75.9550058719466,
-215.153647449945));
#219238=CARTESIAN_POINT('Ctrl Pts',(-3.2388370683562,-75.9809140489,-213.703064133886));
#219239=CARTESIAN_POINT('Ctrl Pts',(-2.43793380877736,-75.158324347106,
-216.467698922128));
#219240=CARTESIAN_POINT('Ctrl Pts',(-2.32497867688892,-75.9559405053742,
-215.261362555356));
#219241=CARTESIAN_POINT('Ctrl Pts',(-2.18920489796754,-75.9814176712845,
-213.817320721562));
#219242=CARTESIAN_POINT('Ctrl Pts',(-2.04653708635396,-75.1623004098586,
-216.495634771282));
#219243=CARTESIAN_POINT('Ctrl Pts',(-1.95228850104495,-75.956191020554,
-215.289675834488));
#219244=CARTESIAN_POINT('Ctrl Pts',(-1.83913744423942,-75.9815538586382,
-213.847387631165));
#219245=CARTESIAN_POINT('Ctrl Pts',(-1.26261892289813,-75.1682023804309,
-216.536118946838));
#219246=CARTESIAN_POINT('Ctrl Pts',(-1.20625878776482,-75.956574549768,
-215.330747400307));
#219247=CARTESIAN_POINT('Ctrl Pts',(-1.13861344723909,-75.9817683431745,
-213.891105902662));
#219248=CARTESIAN_POINT('Ctrl Pts',(-0.870690610263053,-75.1700713359302,
-216.548458769496));
#219249=CARTESIAN_POINT('Ctrl Pts',(-0.8331611987563,-75.9567099274067,
-215.34331728403));
#219250=CARTESIAN_POINT('Ctrl Pts',(-0.788152053854913,-75.9818502107287,
-213.904552602819));
#219251=CARTESIAN_POINT('Ctrl Pts',(-0.0946346290956796,-75.1716828999797,
-216.55940101613));
#219252=CARTESIAN_POINT('Ctrl Pts',(-0.0911222846775505,-75.9568355718726,
-215.354479378076));
#219253=CARTESIAN_POINT('Ctrl Pts',(-0.0868749634279395,-75.9819292803481,
-213.916498075924));
#219254=CARTESIAN_POINT('Ctrl Pts',(0.289821995872756,-75.1715354727665,
-216.558387830722));
#219255=CARTESIAN_POINT('Ctrl Pts',(0.278068638204925,-75.956821763788,
-215.353439573327));
#219256=CARTESIAN_POINT('Ctrl Pts',(0.263931643533207,-75.9819197939239,
-213.91538037431));
#219257=CARTESIAN_POINT('Ctrl Pts',(1.06864077654397,-75.1692292709605,
-216.542760365914));
#219258=CARTESIAN_POINT('Ctrl Pts',(1.0219251337563,-75.9566479467771,-215.337513737709));
#219259=CARTESIAN_POINT('Ctrl Pts',(0.965895527519129,-75.9818124764925,
-213.898350217505));
#219260=CARTESIAN_POINT('Ctrl Pts',(1.46241230485478,-75.1669596440325,
-216.527770436365));
#219261=CARTESIAN_POINT('Ctrl Pts',(1.39635237112926,-75.9564918800891,
-215.322268188682));
#219262=CARTESIAN_POINT('Ctrl Pts',(1.31706165436456,-75.9817211615821,
-213.882064332672));
#219263=CARTESIAN_POINT('Ctrl Pts',(2.64158476672795,-75.157028128614,-216.458935843592));
#219264=CARTESIAN_POINT('Ctrl Pts',(2.518920939202,-75.9558541077429,-215.25245869547));
#219265=CARTESIAN_POINT('Ctrl Pts',(2.37116135636138,-75.9813684091457,
-213.807836336228));
#219266=CARTESIAN_POINT('Ctrl Pts',(3.42746352318773,-75.1462601427746,
-216.381942172347));
#219267=CARTESIAN_POINT('Ctrl Pts',(3.26785428161275,-75.9551914419494,
-215.174452709293));
#219268=CARTESIAN_POINT('Ctrl Pts',(3.07468059463055,-75.9810166072727,
-213.725184571819));
#219269=CARTESIAN_POINT('Ctrl Pts',(4.60404126994595,-75.1242840669289,
-216.222415136132));
#219270=CARTESIAN_POINT('Ctrl Pts',(4.39015023062561,-75.9537982622651,
-215.013097647576));
#219271=CARTESIAN_POINT('Ctrl Pts',(4.13107556051587,-75.9802608955334,
-213.554116576666));
#219272=CARTESIAN_POINT('Ctrl Pts',(4.99546403484811,-75.1160271457934,
-216.161939532443));
#219273=CARTESIAN_POINT('Ctrl Pts',(4.76410117541733,-75.9532672027339,
-214.951901043922));
#219274=CARTESIAN_POINT('Ctrl Pts',(4.48326091718761,-75.9799705283094,
-213.489291039963));
#219275=CARTESIAN_POINT('Ctrl Pts',(5.41027241482983,-75.1062699534614,
-216.09046397724));
#219276=CARTESIAN_POINT('Ctrl Pts',(5.16054567878141,-75.9526264884405,
-214.879614360294));
#219277=CARTESIAN_POINT('Ctrl Pts',(4.85705526974492,-75.9796144475554,
-213.412642866388));
#219278=CARTESIAN_POINT('Ctrl Pts',(5.4346695038882,-75.1056923633818,-216.086232887577));
#219279=CARTESIAN_POINT('Ctrl Pts',(5.18387402798683,-75.952588500194,-214.875333406559));
#219280=CARTESIAN_POINT('Ctrl Pts',(4.87904219608802,-75.9795933268261,
-213.408105477469));
#219281=CARTESIAN_POINT('Ctrl Pts',(5.4712601362539,-75.1048205145248,-216.079846427648));
#219282=CARTESIAN_POINT('Ctrl Pts',(5.21886319527768,-75.9525310919893,
-214.868871767276));
#219283=CARTESIAN_POINT('Ctrl Pts',(4.91202112514165,-75.9795613813585,
-213.40125652354));
#219284=CARTESIAN_POINT('Ctrl Pts',(5.4790807817468,-75.1052596530533,-216.077552452273));
#219285=CARTESIAN_POINT('Ctrl Pts',(5.22811604565769,-75.9525264981582,
-214.866510233269));
#219286=CARTESIAN_POINT('Ctrl Pts',(4.92301425681121,-75.9795504814768,
-213.398978166736));
#219287=CARTESIAN_POINT('Ctrl Pts',(5.49881361376608,-75.1054550956631,
-216.073136911307));
#219288=CARTESIAN_POINT('Ctrl Pts',(5.24887592608961,-75.9525029380811,
-214.862000190262));
#219289=CARTESIAN_POINT('Ctrl Pts',(4.94500105373396,-75.9795280629415,
-213.394437292551));
#219290=CARTESIAN_POINT('Ctrl Pts',(5.5086806337521,-75.1055525263003,-216.070935271933));
#219291=CARTESIAN_POINT('Ctrl Pts',(5.25925632234409,-75.9524908921101,
-214.859751631201));
#219292=CARTESIAN_POINT('Ctrl Pts',(4.95599468254889,-75.9795165632374,
-213.392173699146));
#219293=CARTESIAN_POINT('Ctrl Pts',(5.55801873311596,-75.1060382306792,
-216.05995770291));
#219294=CARTESIAN_POINT('Ctrl Pts',(5.31115963401093,-75.9524293340583,
-214.848541320831));
#219295=CARTESIAN_POINT('Ctrl Pts',(5.01096397729203,-75.9794576130073,
-213.380889917595));
#219296=CARTESIAN_POINT('Ctrl Pts',(5.59749880870147,-75.1064221580628,
-216.051273655991));
#219297=CARTESIAN_POINT('Ctrl Pts',(5.35269029216777,-75.9523758332619,
-214.839676206352));
#219298=CARTESIAN_POINT('Ctrl Pts',(5.05494309510992,-75.9794058073811,
-213.371972284299));
#219299=CARTESIAN_POINT('Ctrl Pts',(5.7159670297233,-75.1075602019096,-216.025514511917));
#219300=CARTESIAN_POINT('Ctrl Pts',(5.47730056979923,-75.9522025875599,
-214.813390278519));
#219301=CARTESIAN_POINT('Ctrl Pts',(5.18689145327219,-75.9792364716388,
-213.345546335821));
#219302=CARTESIAN_POINT('Ctrl Pts',(5.79498316352783,-75.1083005814153,
-216.008732396227));
#219303=CARTESIAN_POINT('Ctrl Pts',(5.56040450116008,-75.9520700938053,
-214.796277534812));
#219304=CARTESIAN_POINT('Ctrl Pts',(5.27487169751627,-75.9791050230153,
-213.328364951587));
#219305=CARTESIAN_POINT('Ctrl Pts',(6.03213727287012,-75.1104680783436,
-215.959550347728));
#219306=CARTESIAN_POINT('Ctrl Pts',(5.80978587963131,-75.9516217475982,
-214.746168419211));
#219307=CARTESIAN_POINT('Ctrl Pts',(5.53885614015153,-75.9786551294951,
-213.278119496813));
#219308=CARTESIAN_POINT('Ctrl Pts',(6.1903809047475,-75.1118415742934,-215.928314470138));
#219309=CARTESIAN_POINT('Ctrl Pts',(5.97615687411766,-75.9512550103054,
-214.71439558984));
#219310=CARTESIAN_POINT('Ctrl Pts',(5.71490403776887,-75.9782811424582,
-213.246353807529));
#219311=CARTESIAN_POINT('Ctrl Pts',(6.98222284448457,-75.1183676778219,
-215.779809027149));
#219312=CARTESIAN_POINT('Ctrl Pts',(6.80827192600329,-75.9490838436669,
-214.563656651227));
#219313=CARTESIAN_POINT('Ctrl Pts',(6.59543144166356,-75.9760422697398,
-213.096080563456));
#219314=CARTESIAN_POINT('Ctrl Pts',(7.61766362532376,-75.1225044545407,
-215.685484989009));
#219315=CARTESIAN_POINT('Ctrl Pts',(7.47572460167024,-75.9462668204644,
-214.468784151763));
#219316=CARTESIAN_POINT('Ctrl Pts',(7.30077147419061,-75.9730722423746,
-213.003143500855));
#219317=CARTESIAN_POINT('Ctrl Pts',(9.52720981831856,-75.1321158303546,
-215.474464687372));
#219318=CARTESIAN_POINT('Ctrl Pts',(9.48054159649718,-75.9345906696201,
-214.260062974152));
#219319=CARTESIAN_POINT('Ctrl Pts',(9.4194934943534,-75.960636334928,-212.804632346833));
#219320=CARTESIAN_POINT('Ctrl Pts',(10.8047815872151,-75.1348247966243,
-215.428648443105));
#219321=CARTESIAN_POINT('Ctrl Pts',(10.8218971913187,-75.9225254849928,
-214.220488336749));
#219322=CARTESIAN_POINT('Ctrl Pts',(10.8355301758809,-75.9476698821379,
-212.777963649677));
#219323=CARTESIAN_POINT('Ctrl Pts',(12.7172077249894,-75.1340707842268,
-215.513470836751));
#219324=CARTESIAN_POINT('Ctrl Pts',(12.8359348263178,-75.8977553183569,
-214.324390406467));
#219325=CARTESIAN_POINT('Ctrl Pts',(12.9654496957873,-75.9208595381148,
-212.912174558945));
#219326=CARTESIAN_POINT('Ctrl Pts',(13.3539693845637,-75.1330093149386,
-215.567557023935));
#219327=CARTESIAN_POINT('Ctrl Pts',(13.5071520281508,-75.8883911745511,
-214.386405940268));
#219328=CARTESIAN_POINT('Ctrl Pts',(13.6764103124011,-75.9106906578871,
-212.986243267424));
#219329=CARTESIAN_POINT('Ctrl Pts',(14.3064153442316,-75.1300979705268,
-215.691855458681));
#219330=CARTESIAN_POINT('Ctrl Pts',(14.5136752922168,-75.8725932457468,
-214.525772201742));
#219331=CARTESIAN_POINT('Ctrl Pts',(14.7445314576483,-75.8934744325803,
-213.147223427492));
#219332=CARTESIAN_POINT('Ctrl Pts',(14.623689531781,-75.1289051437049,-215.740556702165));
#219333=CARTESIAN_POINT('Ctrl Pts',(14.8492851726867,-75.8670321534769,
-214.580010009994));
#219334=CARTESIAN_POINT('Ctrl Pts',(15.1011378555104,-75.8874026004125,
-213.209291022116));
#219335=CARTESIAN_POINT('Ctrl Pts',(15.0973358826677,-75.1267587770309,
-215.825039956629));
#219336=CARTESIAN_POINT('Ctrl Pts',(15.3511219071714,-75.8582618484975,
-214.673710136175));
#219337=CARTESIAN_POINT('Ctrl Pts',(15.6350705546162,-75.8778081087278,
-213.315738009231));
#219338=CARTESIAN_POINT('Ctrl Pts',(15.2548567752318,-75.125983673237,-215.855107341301));
#219339=CARTESIAN_POINT('Ctrl Pts',(15.5181282247503,-75.8552673104085,
-214.706995901577));
#219340=CARTESIAN_POINT('Ctrl Pts',(15.8129038281666,-75.8745286185941,
-213.353446581077));
#219341=CARTESIAN_POINT('Ctrl Pts',(15.4218002487273,-75.1250930170855,
-215.889154542325));
#219342=CARTESIAN_POINT('Ctrl Pts',(15.6952956461322,-75.8520085747563,
-214.744640182935));
#219343=CARTESIAN_POINT('Ctrl Pts',(16.0016916963461,-75.8709562729166,
-213.395980975865));
#219344=CARTESIAN_POINT('Ctrl Pts',(15.4316188990632,-75.1250403784937,
-215.891165045285));
#219345=CARTESIAN_POINT('Ctrl Pts',(15.7057151340514,-75.8518166215729,
-214.746862695126));
#219346=CARTESIAN_POINT('Ctrl Pts',(16.0127962765676,-75.8707458117443,
-213.398492081262));
#219347=CARTESIAN_POINT('Ctrl Pts',(15.4512530718343,-75.1249346051803,
-215.895201541308));
#219348=CARTESIAN_POINT('Ctrl Pts',(15.7265519313712,-75.8514321507501,
-214.75132449253));
#219349=CARTESIAN_POINT('Ctrl Pts',(16.0350042567052,-75.8703242422743,
-213.403532508095));
#219350=CARTESIAN_POINT('Ctrl Pts',(15.459740253059,-75.1249637297094,-215.896828454245));
#219351=CARTESIAN_POINT('Ctrl Pts',(15.7362557047496,-75.8512542699721,
-214.753340594192));
#219352=CARTESIAN_POINT('Ctrl Pts',(16.0461076394828,-75.8701131295941,
-213.406062095362));
#219353=CARTESIAN_POINT('Ctrl Pts',(15.4820248334799,-75.1246924436737,
-215.901694128387));
#219354=CARTESIAN_POINT('Ctrl Pts',(15.7585152623914,-75.8508393951058,
-214.758282360298));
#219355=CARTESIAN_POINT('Ctrl Pts',(16.0683132899191,-75.8696902738925,
-213.411138474507));
#219356=CARTESIAN_POINT('Ctrl Pts',(15.4959535248115,-75.1243825850165,
-215.904955531531));
#219357=CARTESIAN_POINT('Ctrl Pts',(15.7711420877953,-75.8506012003567,
-214.761213105418));
#219358=CARTESIAN_POINT('Ctrl Pts',(16.0794167111148,-75.86947882605,-213.413667362903));
#219359=CARTESIAN_POINT('Ctrl Pts',(15.521032584694,-75.123932842705,-215.910624249774));
#219360=CARTESIAN_POINT('Ctrl Pts',(15.7949037776395,-75.8501553676149,
-214.766587894379));
#219361=CARTESIAN_POINT('Ctrl Pts',(16.101624858776,-75.8690559192528,-213.418704779072));
#219362=CARTESIAN_POINT('Ctrl Pts',(15.5335728237211,-75.1237066808223,
-215.913449505672));
#219363=CARTESIAN_POINT('Ctrl Pts',(15.8067852660439,-75.8499324059612,
-214.769266012297));
#219364=CARTESIAN_POINT('Ctrl Pts',(16.1127295663156,-75.8688444554581,
-213.421213600409));
#219365=CARTESIAN_POINT('Ctrl Pts',(15.596277579428,-75.1225694141948,-215.927530278499));
#219366=CARTESIAN_POINT('Ctrl Pts',(15.866195871248,-75.8488173718676,-214.78261021411));
#219367=CARTESIAN_POINT('Ctrl Pts',(16.1682562721183,-75.8677870840726,
-213.433708281287));
#219368=CARTESIAN_POINT('Ctrl Pts',(15.6464527782837,-75.1216389380232,
-215.93864927566));
#219369=CARTESIAN_POINT('Ctrl Pts',(15.9137348084119,-75.8479246157398,
-214.793137208678));
#219370=CARTESIAN_POINT('Ctrl Pts',(16.2126877745262,-75.8669410192569,
-213.443545863115));
#219371=CARTESIAN_POINT('Ctrl Pts',(15.7970131172075,-75.1187853774811,
-215.971569760114));
#219372=CARTESIAN_POINT('Ctrl Pts',(16.0563828683782,-75.8452441451922,
-214.824273352458));
#219373=CARTESIAN_POINT('Ctrl Pts',(16.3460126749685,-75.8644023051579,
-213.472584430655));
#219374=CARTESIAN_POINT('Ctrl Pts',(15.8974330079295,-75.1168001636331,
-215.992934742601));
#219375=CARTESIAN_POINT('Ctrl Pts',(16.1515241770282,-75.8434542111259,
-214.844437852363));
#219376=CARTESIAN_POINT('Ctrl Pts',(16.4349364663841,-75.8627091362929,
-213.491311234129));
#219377=CARTESIAN_POINT('Ctrl Pts',(17.6053820959646,-75.0816362045942,
-216.346260837099));
#219378=CARTESIAN_POINT('Ctrl Pts',(17.7698966769832,-75.8129696618018,
-215.177219033293));
#219379=CARTESIAN_POINT('Ctrl Pts',(17.9473288709126,-75.8339127266394,
-213.798933624518));
#219380=CARTESIAN_POINT('Ctrl Pts',(19.2277908337019,-75.0263499924907,
-216.527622591312));
#219381=CARTESIAN_POINT('Ctrl Pts',(19.3086934863095,-75.7834585100956,
-215.336116175665));
#219382=CARTESIAN_POINT('Ctrl Pts',(19.3813247221325,-75.8066729690042,
-213.923601542428));
#219383=CARTESIAN_POINT('Ctrl Pts',(21.6558359806902,-74.9150494601847,
-216.590897359445));
#219384=CARTESIAN_POINT('Ctrl Pts',(21.6153500443125,-75.7378479315545,
-215.366882072238));
#219385=CARTESIAN_POINT('Ctrl Pts',(21.5462509158658,-75.7649417071187,
-213.893044878855));
#219386=CARTESIAN_POINT('Ctrl Pts',(22.4648784248499,-74.8731903210939,
-216.578042999207));
#219387=CARTESIAN_POINT('Ctrl Pts',(22.3867384863216,-75.7223537446655,
-215.343224536461));
#219388=CARTESIAN_POINT('Ctrl Pts',(22.2701738627727,-75.7508758505917,
-213.84723891686));
#219389=CARTESIAN_POINT('Ctrl Pts',(23.4728708240175,-74.816161830225,-216.524453677946));
#219390=CARTESIAN_POINT('Ctrl Pts',(23.3494355632829,-75.7026196357405,
-215.276919328278));
#219391=CARTESIAN_POINT('Ctrl Pts',(23.177540032039,-75.732985743614,-213.751482920168));
#219392=CARTESIAN_POINT('Ctrl Pts',(23.6743655621636,-74.8045134968797,
-216.511872971906));
#219393=CARTESIAN_POINT('Ctrl Pts',(23.5422576362207,-75.6986468679756,
-215.261803887036));
#219394=CARTESIAN_POINT('Ctrl Pts',(23.3591731636709,-75.7293914716431,
-213.730409932309));
#219395=CARTESIAN_POINT('Ctrl Pts',(23.9762017683036,-74.7867010048439,
-216.490346610853));
#219396=CARTESIAN_POINT('Ctrl Pts',(23.8312594277273,-75.6926601948462,
-215.236527096512));
#219397=CARTESIAN_POINT('Ctrl Pts',(23.6316298755007,-75.7239779322202,
-213.696069266785));
#219398=CARTESIAN_POINT('Ctrl Pts',(24.0767465863703,-74.7807068465897,
-216.48272879554));
#219399=CARTESIAN_POINT('Ctrl Pts',(23.9275870343842,-75.690659379697,-215.227664419223));
#219400=CARTESIAN_POINT('Ctrl Pts',(23.7224502835782,-75.7221697265246,
-213.684167363404));
#219401=CARTESIAN_POINT('Ctrl Pts',(24.2274640600537,-74.7716317815129,
-216.470654320984));
#219402=CARTESIAN_POINT('Ctrl Pts',(24.0720224749929,-75.687650992375,-215.213735619942));
#219403=CARTESIAN_POINT('Ctrl Pts',(23.858683087999,-75.7194515985814,-213.665648035631));
#219404=CARTESIAN_POINT('Ctrl Pts',(24.2776865884637,-74.7685927882663,
-216.466521534823));
#219405=CARTESIAN_POINT('Ctrl Pts',(24.1201662478945,-75.6866468359805,
-215.208986051363));
#219406=CARTESIAN_POINT('Ctrl Pts',(23.9040943881952,-75.7185445860867,
-213.659363844575));
#219407=CARTESIAN_POINT('Ctrl Pts',(24.3529955852829,-74.7640134807405,
-216.460162360007));
#219408=CARTESIAN_POINT('Ctrl Pts',(24.1923680699484,-75.6851387760389,
-215.201704952376));
#219409=CARTESIAN_POINT('Ctrl Pts',(23.9722118786887,-75.7171825779668,
-213.649772915152));
#219410=CARTESIAN_POINT('Ctrl Pts',(24.3784994717427,-74.7623348648064,
-216.458136672852));
#219411=CARTESIAN_POINT('Ctrl Pts',(24.2166607054916,-75.6846291537297,
-215.199335161605));
#219412=CARTESIAN_POINT('Ctrl Pts',(23.9949178673861,-75.7167286261278,
-213.64653127887));
#219413=CARTESIAN_POINT('Ctrl Pts',(24.4196337599662,-74.7625680326348,
-216.450800742114));
#219414=CARTESIAN_POINT('Ctrl Pts',(24.259705887401,-75.6837748047058,-215.192214283183));
#219415=CARTESIAN_POINT('Ctrl Pts',(24.0403296350762,-75.7158185240332,
-213.640091106598));
#219416=CARTESIAN_POINT('Ctrl Pts',(24.4402002771278,-74.762683912951,-216.447154613061));
#219417=CARTESIAN_POINT('Ctrl Pts',(24.2812282571141,-75.6833465808423,
-215.188677021339));
#219418=CARTESIAN_POINT('Ctrl Pts',(24.0630354011898,-75.715362317608,-213.636895804635));
#219419=CARTESIAN_POINT('Ctrl Pts',(24.7898203708446,-74.764641964529,-216.385541888145));
#219420=CARTESIAN_POINT('Ctrl Pts',(24.6469467821791,-75.6760520799882,
-215.128963778829));
#219421=CARTESIAN_POINT('Ctrl Pts',(24.4490314221452,-75.7075871592492,
-213.582997463384));
#219422=CARTESIAN_POINT('Ctrl Pts',(25.1187116623081,-74.7663052298968,
-216.333145267762));
#219423=CARTESIAN_POINT('Ctrl Pts',(24.9912410172876,-75.6689153385714,
-215.078669907208));
#219424=CARTESIAN_POINT('Ctrl Pts',(24.812291644422,-75.6999735317664,-213.538617767255));
#219425=CARTESIAN_POINT('Ctrl Pts',(26.7622290318585,-74.7737857064687,
-216.099514369437));
#219426=CARTESIAN_POINT('Ctrl Pts',(26.7099624617689,-75.6319318195073,
-214.857743429527));
#219427=CARTESIAN_POINT('Ctrl Pts',(26.6284393652984,-75.6604150064864,
-213.3491278222));
#219428=CARTESIAN_POINT('Ctrl Pts',(28.075080877613,-74.7769924622541,-216.001871476478));
#219429=CARTESIAN_POINT('Ctrl Pts',(28.0859463587902,-75.5980221249252,
-214.775154563847));
#219430=CARTESIAN_POINT('Ctrl Pts',(28.0808759169087,-75.6240391544431,
-213.29892337729));
#219431=CARTESIAN_POINT('Ctrl Pts',(30.0270254090569,-74.7816141294705,
-216.00764859601));
#219432=CARTESIAN_POINT('Ctrl Pts',(30.1441281348009,-75.5404095409703,
-214.819104347431));
#219433=CARTESIAN_POINT('Ctrl Pts',(30.2586772078354,-75.5618154664653,
-213.408748577776));
#219434=CARTESIAN_POINT('Ctrl Pts',(30.6746003481513,-74.783131073334,-216.03519912743));
#219435=CARTESIAN_POINT('Ctrl Pts',(30.8278988046784,-75.5201201036592,
-214.861853605089));
#219436=CARTESIAN_POINT('Ctrl Pts',(30.9844671541994,-75.5397907755024,
-213.476605004965));
#219437=CARTESIAN_POINT('Ctrl Pts',(31.9599958800107,-74.7861720113306,
-216.151048029206));
#219438=CARTESIAN_POINT('Ctrl Pts',(32.1907307647438,-75.477181336842,-215.015719242188));
#219439=CARTESIAN_POINT('Ctrl Pts',(32.435703007658,-75.4929295570714,-213.689014761762));
#219440=CARTESIAN_POINT('Ctrl Pts',(32.6006286165977,-74.7878210783825,
-216.24000664944));
#219441=CARTESIAN_POINT('Ctrl Pts',(32.872988366941,-75.4544140916729,-215.127572191219));
#219442=CARTESIAN_POINT('Ctrl Pts',(33.1649378192402,-75.46794300932,-213.834823319187));
#219443=CARTESIAN_POINT('Ctrl Pts',(33.2168085208362,-74.7890149970872,
-216.36473842254));
#219444=CARTESIAN_POINT('Ctrl Pts',(33.5343686210915,-75.4309604638016,
-215.280488076331));
#219445=CARTESIAN_POINT('Ctrl Pts',(33.8749380667978,-75.4420407256794,
-214.026523605855));
#219446=CARTESIAN_POINT('',(24.3802580872756,-74.7628322230906,-216.457148834596));
#219447=CARTESIAN_POINT('',(15.4710515403103,-75.1252154310809,-215.898655568186));
#219448=CARTESIAN_POINT('Ctrl Pts',(24.3802580872756,-74.7628322230906,
-216.457148834596));
#219449=CARTESIAN_POINT('Ctrl Pts',(23.6057867097546,-74.8100705737294,
-216.52370992462));
#219450=CARTESIAN_POINT('Ctrl Pts',(22.8447074397333,-74.8532777187265,
-216.562969013006));
#219451=CARTESIAN_POINT('Ctrl Pts',(21.7246656382609,-74.9110314666933,
-216.58090464313));
#219452=CARTESIAN_POINT('Ctrl Pts',(21.3548976004719,-74.9291197144322,
-216.580057686095));
#219453=CARTESIAN_POINT('Ctrl Pts',(20.805828082717,-74.9545797369581,-216.568548999929));
#219454=CARTESIAN_POINT('Ctrl Pts',(20.5326875016302,-74.9668922756974,
-216.560235094192));
#219455=CARTESIAN_POINT('Ctrl Pts',(20.2164959770152,-74.9805477557225,
-216.546056302856));
#219456=CARTESIAN_POINT('Ctrl Pts',(20.0815178427006,-74.9862507373229,
-216.539019842002));
#219457=CARTESIAN_POINT('Ctrl Pts',(19.9916510399144,-74.9900198259762,
-216.534115571212));
#219458=CARTESIAN_POINT('Ctrl Pts',(19.9487412234712,-74.9918067539723,
-216.531673616063));
#219459=CARTESIAN_POINT('Ctrl Pts',(18.4050368468729,-75.0555944587559,
-216.439859003958));
#219460=CARTESIAN_POINT('Ctrl Pts',(16.9264817129947,-75.0994115785442,
-216.229780408324));
#219461=CARTESIAN_POINT('Ctrl Pts',(15.4710515403103,-75.1252154310809,
-215.898655568186));
#219462=CARTESIAN_POINT('',(32.8638454863375,-74.7886392304488,-216.296979356602));
#219463=CARTESIAN_POINT('Ctrl Pts',(32.863845486296,-74.788639230448,-216.296979356596));
#219464=CARTESIAN_POINT('Ctrl Pts',(32.2178333387358,-74.7872541619425,
-216.181772728121));
#219465=CARTESIAN_POINT('Ctrl Pts',(31.5389214686617,-74.7860747654139,
-216.100629599085));
#219466=CARTESIAN_POINT('Ctrl Pts',(30.4747208094706,-74.7835574505676,
-216.030010154687));
#219467=CARTESIAN_POINT('Ctrl Pts',(30.1123332242519,-74.7826192987842,
-216.014986214748));
#219468=CARTESIAN_POINT('Ctrl Pts',(29.5576378729449,-74.7811432549687,
-216.005224117128));
#219469=CARTESIAN_POINT('Ctrl Pts',(29.2775116904412,-74.7803894360587,
-216.00353652139));
#219470=CARTESIAN_POINT('Ctrl Pts',(28.9459188512441,-74.7795141404412,
-216.007156202572));
#219471=CARTESIAN_POINT('Ctrl Pts',(28.7789380649846,-74.7790835460274,
-216.010363178883));
#219472=CARTESIAN_POINT('Ctrl Pts',(28.6951526914092,-74.7788711619761,
-216.012315950968));
#219473=CARTESIAN_POINT('Ctrl Pts',(28.6591815979652,-74.7787808680542,
-216.013227699846));
#219474=CARTESIAN_POINT('Ctrl Pts',(28.6351868666064,-74.7787208463327,
-216.013852165));
#219475=CARTESIAN_POINT('Ctrl Pts',(28.6219205756486,-74.7786877885733,
-216.014207264721));
#219476=CARTESIAN_POINT('Ctrl Pts',(27.2352432404576,-74.7752439591572,
-216.052173807495));
#219477=CARTESIAN_POINT('Ctrl Pts',(25.8185917312215,-74.7709950882897,
-216.199722892692));
#219478=CARTESIAN_POINT('Ctrl Pts',(24.3802580872756,-74.7628322230906,
-216.457148834596));
#219479=CARTESIAN_POINT('',(33.3513892243221,-75.4608554610386,-213.894117162909));
#219480=CARTESIAN_POINT('Ctrl Pts',(32.863845486296,-74.788639230448,-216.296979356596));
#219481=CARTESIAN_POINT('Ctrl Pts',(32.9410850039213,-74.999970347199,-215.939487466059));
#219482=CARTESIAN_POINT('Ctrl Pts',(33.0236138935975,-75.1681413467096,
-215.548509757113));
#219483=CARTESIAN_POINT('Ctrl Pts',(33.1895226861483,-75.3962354831127,
-214.734437839155));
#219484=CARTESIAN_POINT('Ctrl Pts',(33.2727909348202,-75.4560174753842,
-214.311772816012));
#219485=CARTESIAN_POINT('Ctrl Pts',(33.3513899426336,-75.4608558287546,
-213.894117302352));
#219486=CARTESIAN_POINT('Ctrl Pts',(-33.3513928247577,-75.4608558931301,
-213.894101966659));
#219487=CARTESIAN_POINT('Ctrl Pts',(-32.8873496662889,-75.4772841921233,
-213.784425468418));
#219488=CARTESIAN_POINT('Ctrl Pts',(-32.4201892950423,-75.4931733089948,
-213.693836888586));
#219489=CARTESIAN_POINT('Ctrl Pts',(-31.9507721192534,-75.5085355661565,
-213.619497087055));
#219490=CARTESIAN_POINT('Ctrl Pts',(-31.9075027906416,-75.5099516084055,
-213.612644689088));
#219491=CARTESIAN_POINT('Ctrl Pts',(-31.8642143022296,-75.5113631741533,
-213.605930383152));
#219492=CARTESIAN_POINT('Ctrl Pts',(-31.8209073365556,-75.5127702730643,
-213.599351966943));
#219493=CARTESIAN_POINT('Ctrl Pts',(-31.657104814835,-75.51809242728,-213.574470030579));
#219494=CARTESIAN_POINT('Ctrl Pts',(-31.4929112225694,-75.5233541895962,
-213.551532319841));
#219495=CARTESIAN_POINT('Ctrl Pts',(-31.3284605632087,-75.5285525767555,
-213.530477412274));
#219496=CARTESIAN_POINT('Ctrl Pts',(-30.9340514163604,-75.5410200940794,
-213.479980514525));
#219497=CARTESIAN_POINT('Ctrl Pts',(-30.5375718139143,-75.5531426206814,
-213.440194218096));
#219498=CARTESIAN_POINT('Ctrl Pts',(-30.1405091673275,-75.5648865535421,
-213.410317899452));
#219499=CARTESIAN_POINT('Ctrl Pts',(-30.0093310829785,-75.5687664113645,
-213.400447622606));
#219500=CARTESIAN_POINT('Ctrl Pts',(-29.8780892162955,-75.5726049379618,
-213.391659383122));
#219501=CARTESIAN_POINT('Ctrl Pts',(-29.7468368704954,-75.5764008912256,
-213.383925473857));
#219502=CARTESIAN_POINT('Ctrl Pts',(-29.5908035364721,-75.5809135362373,
-213.37473137039));
#219503=CARTESIAN_POINT('Ctrl Pts',(-29.4348076545751,-75.5853653973002,
-213.366996066073));
#219504=CARTESIAN_POINT('Ctrl Pts',(-29.2788373795595,-75.5897573793404,
-213.360688865401));
#219505=CARTESIAN_POINT('Ctrl Pts',(-28.587495913932,-75.6092249304514,
-213.332732068141));
#219506=CARTESIAN_POINT('Ctrl Pts',(-27.8963404060334,-75.6275309381467,
-213.332477866803));
#219507=CARTESIAN_POINT('Ctrl Pts',(-27.2053257342637,-75.6447219136339,
-213.35739210847));
#219508=CARTESIAN_POINT('Ctrl Pts',(-26.6627179145517,-75.6582208422514,
-213.376955603868));
#219509=CARTESIAN_POINT('Ctrl Pts',(-26.120198033493,-75.6710321930194,
-213.412038537932));
#219510=CARTESIAN_POINT('Ctrl Pts',(-25.5777648626619,-75.683177813424,
-213.461422194978));
#219511=CARTESIAN_POINT('Ctrl Pts',(-25.4434846238148,-75.6861844820729,
-213.473647201891));
#219512=CARTESIAN_POINT('Ctrl Pts',(-25.3092057560598,-75.689150084866,
-213.48676925098));
#219513=CARTESIAN_POINT('Ctrl Pts',(-25.1749285663624,-75.692074732042,
-213.50078176889));
#219514=CARTESIAN_POINT('Ctrl Pts',(-24.9619426474422,-75.6967137080862,
-213.523007949004));
#219515=CARTESIAN_POINT('Ctrl Pts',(-24.7489594890241,-75.7012498838473,
-213.547462664372));
#219516=CARTESIAN_POINT('Ctrl Pts',(-24.5359790241656,-75.7056838071389,
-213.574115147839));
#219517=CARTESIAN_POINT('Ctrl Pts',(-24.4070995903422,-75.7083668772684,
-213.590243185599));
#219518=CARTESIAN_POINT('Ctrl Pts',(-24.2782211440055,-75.7110124995285,
-213.607176310471));
#219519=CARTESIAN_POINT('Ctrl Pts',(-24.1493436789706,-75.713620770764,
-213.62490909452));
#219520=CARTESIAN_POINT('Ctrl Pts',(-24.1045967081316,-75.714526377007,
-213.631066015519));
#219521=CARTESIAN_POINT('Ctrl Pts',(-24.0598498586817,-75.7154274806628,
-213.637319324643));
#219522=CARTESIAN_POINT('Ctrl Pts',(-24.0151031302881,-75.7163240858007,
-213.643668793969));
#219523=CARTESIAN_POINT('Ctrl Pts',(-23.9934001948624,-75.7167589547645,
-213.646748396159));
#219524=CARTESIAN_POINT('Ctrl Pts',(-23.9716972776745,-75.7171928634372,
-213.649845022571));
#219525=CARTESIAN_POINT('Ctrl Pts',(-23.9499942742991,-75.7176268179877,
-213.652901178597));
#219526=CARTESIAN_POINT('Ctrl Pts',(-23.9282912704726,-75.7180607725472,
-213.655957334687));
#219527=CARTESIAN_POINT('Ctrl Pts',(-23.9065882084806,-75.7184945030891,
-213.658988442607));
#219528=CARTESIAN_POINT('Ctrl Pts',(-23.8848850880541,-75.7189280121292,
-213.661994358033));
#219529=CARTESIAN_POINT('Ctrl Pts',(-23.8414788461836,-75.7197950302298,
-213.668006189026));
#219530=CARTESIAN_POINT('Ctrl Pts',(-23.7980723705685,-75.7206611623083,
-213.673917250899));
#219531=CARTESIAN_POINT('Ctrl Pts',(-23.7546656590397,-75.7215264286156,
-213.679726381899));
#219532=CARTESIAN_POINT('Ctrl Pts',(-23.6678522342647,-75.7232569612644,
-213.691344644129));
#219533=CARTESIAN_POINT('Ctrl Pts',(-23.581037865851,-75.7249840306461,
-213.702555193327));
#219534=CARTESIAN_POINT('Ctrl Pts',(-23.4942225353474,-75.7267078008841,
-213.713348614776));
#219535=CARTESIAN_POINT('Ctrl Pts',(-23.3707348340602,-75.7291597229468,
-213.72870137328));
#219536=CARTESIAN_POINT('Ctrl Pts',(-23.2472451863123,-75.7316049709933,
-213.743210120025));
#219537=CARTESIAN_POINT('Ctrl Pts',(-23.1237535338497,-75.7340440351597,
-213.75684673174));
#219538=CARTESIAN_POINT('Ctrl Pts',(-22.5526996859888,-75.7453228297144,
-213.819905565566));
#219539=CARTESIAN_POINT('Ctrl Pts',(-21.9816053178851,-75.7564694844777,
-213.864306970363));
#219540=CARTESIAN_POINT('Ctrl Pts',(-21.4104614756218,-75.7675316609456,
-213.88731993422));
#219541=CARTESIAN_POINT('Ctrl Pts',(-21.2977418163553,-75.7697148671187,
-213.891861720812));
#219542=CARTESIAN_POINT('Ctrl Pts',(-21.1850201592615,-75.7718949319907,
-213.895561976977));
#219543=CARTESIAN_POINT('Ctrl Pts',(-21.0722963627658,-75.7740721183519,
-213.898405686423));
#219544=CARTESIAN_POINT('Ctrl Pts',(-20.3101280724893,-75.7887929001041,
-213.917633083245));
#219545=CARTESIAN_POINT('Ctrl Pts',(-19.5478296370527,-75.8033869760415,
-213.897455950411));
#219546=CARTESIAN_POINT('Ctrl Pts',(-18.7854746599048,-75.8179333033253,
-213.833237968256));
#219547=CARTESIAN_POINT('Ctrl Pts',(-18.2708779812001,-75.8277522091264,
-213.789890234823));
#219548=CARTESIAN_POINT('Ctrl Pts',(-17.7562545676338,-75.8375493971014,
-213.72647578556));
#219549=CARTESIAN_POINT('Ctrl Pts',(-17.241613757919,-75.8473494730384,
-213.641571672275));
#219550=CARTESIAN_POINT('Ctrl Pts',(-17.1504453664671,-75.8490855521491,
-213.626530946219));
#219551=CARTESIAN_POINT('Ctrl Pts',(-17.059268607012,-75.8508216747552,
-213.610825285784));
#219552=CARTESIAN_POINT('Ctrl Pts',(-16.96809027621,-75.8525577589421,-213.594453482362));
#219553=CARTESIAN_POINT('Ctrl Pts',(-16.7970429357528,-75.8558145917923,
-213.563740555186));
#219554=CARTESIAN_POINT('Ctrl Pts',(-16.6259904766021,-75.8590713549408,
-213.530679591711));
#219555=CARTESIAN_POINT('Ctrl Pts',(-16.4549329472469,-75.8623283920597,
-213.495250367538));
#219556=CARTESIAN_POINT('Ctrl Pts',(-16.3696536621392,-75.8639521603797,
-213.477587427353));
#219557=CARTESIAN_POINT('Ctrl Pts',(-16.2843852368415,-75.865575760016,
-213.459338620813));
#219558=CARTESIAN_POINT('Ctrl Pts',(-16.1991337604474,-75.8671991180785,
-213.440502891606));
#219559=CARTESIAN_POINT('Ctrl Pts',(-16.1557108260507,-75.8680259773147,
-213.430908891968));
#219560=CARTESIAN_POINT('Ctrl Pts',(-16.1122956661453,-75.868852709237,
-213.421163496792));
#219561=CARTESIAN_POINT('Ctrl Pts',(-16.0688883605895,-75.8696793177453,
-213.411266577736));
#219562=CARTESIAN_POINT('Ctrl Pts',(-16.0471841769452,-75.8700926321087,
-213.40631799717));
#219563=CARTESIAN_POINT('Ctrl Pts',(-16.0254806449976,-75.8705054507595,
-213.401359298027));
#219564=CARTESIAN_POINT('Ctrl Pts',(-16.0037747424049,-75.8709166991138,
-213.396454629959));
#219565=CARTESIAN_POINT('Ctrl Pts',(-15.9831651900046,-75.871307175597,
-213.391797693296));
#219566=CARTESIAN_POINT('Ctrl Pts',(-15.9625543147019,-75.8716965249299,
-213.387172236819));
#219567=CARTESIAN_POINT('Ctrl Pts',(-15.9419421324393,-75.8720847496106,
-213.382578090849));
#219568=CARTESIAN_POINT('Ctrl Pts',(-15.9408452649187,-75.8721054088032,
-213.382333615547));
#219569=CARTESIAN_POINT('Ctrl Pts',(-15.9397483932213,-75.87212606482,-213.382089228799));
#219570=CARTESIAN_POINT('Ctrl Pts',(-15.9386515173484,-75.8721467176615,
-213.381844930582));
#219571=CARTESIAN_POINT('Ctrl Pts',(-15.851813756867,-75.8737817672998,
-213.362504264434));
#219572=CARTESIAN_POINT('Ctrl Pts',(-15.7649498283845,-75.8753969160326,
-213.343718402895));
#219573=CARTESIAN_POINT('Ctrl Pts',(-15.6780603215635,-75.8769923431775,
-213.325475501279));
#219574=CARTESIAN_POINT('Ctrl Pts',(-15.5042797865617,-75.8801832254017,
-213.288989378631));
#219575=CARTESIAN_POINT('Ctrl Pts',(-15.3303969644586,-75.883295232643,
-213.25467435116));
#219576=CARTESIAN_POINT('Ctrl Pts',(-15.1564162069293,-75.8863296353476,
-213.222445734065));
#219577=CARTESIAN_POINT('Ctrl Pts',(-15.0759336740236,-75.8877333331991,
-213.207536954653));
#219578=CARTESIAN_POINT('Ctrl Pts',(-14.9954303042051,-75.8891204649254,
-213.193072142904));
#219579=CARTESIAN_POINT('Ctrl Pts',(-14.9149064146963,-75.8904911137141,
-213.179045535909));
#219580=CARTESIAN_POINT('Ctrl Pts',(-14.2991321754372,-75.9009726021306,
-213.071782668898));
#219581=CARTESIAN_POINT('Ctrl Pts',(-13.6821528490865,-75.9104918796616,
-212.990053078907));
#219582=CARTESIAN_POINT('Ctrl Pts',(-13.0640933699476,-75.9190856566173,
-212.931320199254));
#219583=CARTESIAN_POINT('Ctrl Pts',(-12.9941535614473,-75.9200581311684,
-212.924673967792));
#219584=CARTESIAN_POINT('Ctrl Pts',(-12.9242001019972,-75.9210188053301,
-212.918319156356));
#219585=CARTESIAN_POINT('Ctrl Pts',(-12.8542330789119,-75.9219676899831,
-212.912254648701));
#219586=CARTESIAN_POINT('Ctrl Pts',(-12.103744918449,-75.932145723381,-212.847204843899));
#219587=CARTESIAN_POINT('Ctrl Pts',(-11.3516069380129,-75.9409718595207,
-212.815352430239));
#219588=CARTESIAN_POINT('Ctrl Pts',(-10.5980291929577,-75.9484605685429,
-212.815191307246));
#219589=CARTESIAN_POINT('Ctrl Pts',(-10.0177252773204,-75.9542273619457,
-212.815067232053));
#219590=CARTESIAN_POINT('Ctrl Pts',(-9.43656819308798,-75.9592010864688,
-212.833735208245));
#219591=CARTESIAN_POINT('Ctrl Pts',(-8.85466502499123,-75.9633890545989,
-212.870489657771));
#219592=CARTESIAN_POINT('Ctrl Pts',(-8.80621265809307,-75.9637377672018,
-212.873550029619));
#219593=CARTESIAN_POINT('Ctrl Pts',(-8.7577487416815,-75.9640810280511,
-212.876738332401));
#219594=CARTESIAN_POINT('Ctrl Pts',(-8.70927474202254,-75.9644188262203,
-212.880054548429));
#219595=CARTESIAN_POINT('Ctrl Pts',(-8.16802284443195,-75.9681906193745,
-212.917082815758));
#219596=CARTESIAN_POINT('Ctrl Pts',(-7.62521966310781,-75.9712836556175,
-212.970057781598));
#219597=CARTESIAN_POINT('Ctrl Pts',(-7.08306476118715,-75.9736810365594,
-213.038940050712));
#219598=CARTESIAN_POINT('Ctrl Pts',(-6.96823963948708,-75.9741887873101,
-213.053528897748));
#219599=CARTESIAN_POINT('Ctrl Pts',(-6.85344360943193,-75.9746653412367,
-213.06883110778));
#219600=CARTESIAN_POINT('Ctrl Pts',(-6.73869756970069,-75.9751105507597,
-213.084846007434));
#219601=CARTESIAN_POINT('Ctrl Pts',(-6.70123227716741,-75.9752559144258,
-213.090074971343));
#219602=CARTESIAN_POINT('Ctrl Pts',(-6.66377970851828,-75.9753979183016,
-213.095378751942));
#219603=CARTESIAN_POINT('Ctrl Pts',(-6.62633993925021,-75.9755365658722,
-213.10075735341));
#219604=CARTESIAN_POINT('Ctrl Pts',(-6.31150977816634,-75.9767024501139,
-213.145985889793));
#219605=CARTESIAN_POINT('Ctrl Pts',(-5.99754483591358,-75.9776311781919,
-213.196509446686));
#219606=CARTESIAN_POINT('Ctrl Pts',(-5.68444746635923,-75.9783247837595,
-213.252342367387));
#219607=CARTESIAN_POINT('Ctrl Pts',(-5.65269333611006,-75.9783951287822,
-213.258004905653));
#219608=CARTESIAN_POINT('Ctrl Pts',(-5.62094813600815,-75.9784630546653,
-213.263722092798));
#219609=CARTESIAN_POINT('Ctrl Pts',(-5.5892118753693,-75.9785285627877,
-213.269493984429));
#219610=CARTESIAN_POINT('Ctrl Pts',(-5.4458894272464,-75.9788244005545,
-213.295560118943));
#219611=CARTESIAN_POINT('Ctrl Pts',(-5.30273879712366,-75.9790709489129,
-213.322743719392));
#219612=CARTESIAN_POINT('Ctrl Pts',(-5.15978901555836,-75.9792682954213,
-213.351044287356));
#219613=CARTESIAN_POINT('Ctrl Pts',(-5.13085816823248,-75.9793082353333,
-213.35677188905));
#219614=CARTESIAN_POINT('Ctrl Pts',(-5.1019356538566,-75.9793461604998,
-213.362545209928));
#219615=CARTESIAN_POINT('Ctrl Pts',(-5.07301593827139,-75.9793820774016,
-213.368365449668));
#219616=CARTESIAN_POINT('Ctrl Pts',(-5.05829718990994,-75.9794003573822,
-213.37132767258));
#219617=CARTESIAN_POINT('Ctrl Pts',(-5.04358000194555,-75.9794181161351,
-213.374301880288));
#219618=CARTESIAN_POINT('Ctrl Pts',(-5.02886336884999,-75.9794353549927,
-213.377288283786));
#219619=CARTESIAN_POINT('Ctrl Pts',(-5.00704302178793,-75.9794609150413,
-213.381716223271));
#219620=CARTESIAN_POINT('Ctrl Pts',(-4.98522511827338,-75.9794853303841,
-213.386170733756));
#219621=CARTESIAN_POINT('Ctrl Pts',(-4.96340885953034,-75.9795086014944,
-213.390652023996));
#219622=CARTESIAN_POINT('Ctrl Pts',(-4.9524998768548,-75.9795202379597,
-213.392892844394));
#219623=CARTESIAN_POINT('Ctrl Pts',(-4.94159130543411,-75.979531588317,
-213.39514036091));
#219624=CARTESIAN_POINT('Ctrl Pts',(-4.93068304543216,-75.9795426525913,
-213.397394600517));
#219625=CARTESIAN_POINT('Ctrl Pts',(-4.91977448336048,-75.9795537171721,
-213.399648902548));
#219626=CARTESIAN_POINT('Ctrl Pts',(-4.9088663032563,-75.9795644433992,
-213.401912903139));
#219627=CARTESIAN_POINT('Ctrl Pts',(-4.89795817571377,-75.9795750013207,
-213.404176948458));
#219628=CARTESIAN_POINT('Ctrl Pts',(-4.8107062930038,-75.9796594519766,
-213.422286584224));
#219629=CARTESIAN_POINT('Ctrl Pts',(-4.72344700942351,-75.9797411185036,
-213.439944730912));
#219630=CARTESIAN_POINT('Ctrl Pts',(-4.63612898071532,-75.9798201342666,
-213.457155494977));
#219631=CARTESIAN_POINT('Ctrl Pts',(-4.60996385918782,-75.9798438115881,
-213.462312754481));
#219632=CARTESIAN_POINT('Ctrl Pts',(-4.5837934588528,-75.9798672535015,
-213.467429677896));
#219633=CARTESIAN_POINT('Ctrl Pts',(-4.5576163974065,-75.9798904631868,
-213.472506347965));
#219634=CARTESIAN_POINT('Ctrl Pts',(-4.07663947765109,-75.9803169175844,
-213.565785004833));
#219635=CARTESIAN_POINT('Ctrl Pts',(-3.59417252100192,-75.9806646032663,
-213.645311443452));
#219636=CARTESIAN_POINT('Ctrl Pts',(-3.11009598855904,-75.9809468066053,
-213.709986409894));
#219637=CARTESIAN_POINT('Ctrl Pts',(-2.92000878015336,-75.9810576222332,
-213.735382980479));
#219638=CARTESIAN_POINT('Ctrl Pts',(-2.72967334665686,-75.9811583442642,
-213.758488932177));
#219639=CARTESIAN_POINT('Ctrl Pts',(-2.53908232066754,-75.9812497918801,
-213.77923549017));
#219640=CARTESIAN_POINT('Ctrl Pts',(-2.52097369221552,-75.981258480594,
-213.781206683244));
#219641=CARTESIAN_POINT('Ctrl Pts',(-2.50286275684531,-75.9812670852011,
-213.783156596776));
#219642=CARTESIAN_POINT('Ctrl Pts',(-2.4847495087102,-75.9812756060268,
-213.785085192613));
#219643=CARTESIAN_POINT('Ctrl Pts',(-2.15358059177547,-75.9814313943545,
-213.820346178928));
#219644=CARTESIAN_POINT('Ctrl Pts',(-1.82162137854988,-75.9815590179761,
-213.848492418773));
#219645=CARTESIAN_POINT('Ctrl Pts',(-1.48887673016169,-75.9816607414808,
-213.86926725327));
#219646=CARTESIAN_POINT('Ctrl Pts',(-1.13928261377975,-75.9817676160432,
-213.891094080371));
#219647=CARTESIAN_POINT('Ctrl Pts',(-0.788816617423684,-75.9818494936408,
-213.90457805642));
#219648=CARTESIAN_POINT('Ctrl Pts',(-0.437513953977255,-75.9818892910274,
-213.91055136394));
#219649=CARTESIAN_POINT('Ctrl Pts',(-0.422238919642044,-75.9818910214625,
-213.910811090059));
#219650=CARTESIAN_POINT('Ctrl Pts',(-0.406962321199802,-75.9818926595883,
-213.911057348003));
#219651=CARTESIAN_POINT('Ctrl Pts',(-0.391684159219294,-75.9818942057822,
-213.911290104531));
#219652=CARTESIAN_POINT('Ctrl Pts',(-0.106400275277922,-75.9819230773301,
-213.915636287441));
#219653=CARTESIAN_POINT('Ctrl Pts',(0.179082832830468,-75.9819195513841,
-213.915281542));
#219654=CARTESIAN_POINT('Ctrl Pts',(0.464388804013359,-75.98188633428,-213.910069992462));
#219655=CARTESIAN_POINT('Ctrl Pts',(0.514569929607294,-75.9818804918797,
-213.909153357522));
#219656=CARTESIAN_POINT('Ctrl Pts',(0.564745571523509,-75.9818737317438,
-213.908086604403));
#219657=CARTESIAN_POINT('Ctrl Pts',(0.614913677116972,-75.9818660695581,
-213.906869053894));
#219658=CARTESIAN_POINT('Ctrl Pts',(0.883836747769246,-75.981824996879,
-213.90034244864));
#219659=CARTESIAN_POINT('Ctrl Pts',(1.15254856945707,-75.9817618231612,
-213.889259482589));
#219660=CARTESIAN_POINT('Ctrl Pts',(1.42073621839167,-75.9816819480231,
-213.873375461236));
#219661=CARTESIAN_POINT('Ctrl Pts',(1.50335308767494,-75.9816573419912,
-213.868482289903));
#219662=CARTESIAN_POINT('Ctrl Pts',(1.58592020389488,-75.9816311515161,
-213.86313387284));
#219663=CARTESIAN_POINT('Ctrl Pts',(1.66842839174222,-75.9816035352139,
-213.857324070858));
#219664=CARTESIAN_POINT('Ctrl Pts',(1.68217044445011,-75.9815989356136,
-213.856356426227));
#219665=CARTESIAN_POINT('Ctrl Pts',(1.69591085645726,-75.9815942920412,
-213.855376236483));
#219666=CARTESIAN_POINT('Ctrl Pts',(1.70964958405473,-75.9815896042878,
-213.854383528651));
#219667=CARTESIAN_POINT('Ctrl Pts',(2.19610545981022,-75.98142362202,-213.819234090393));
#219668=CARTESIAN_POINT('Ctrl Pts',(2.68121874436983,-75.9812020443835,
-213.76833459995));
#219669=CARTESIAN_POINT('Ctrl Pts',(3.16507275796152,-75.9809144082949,
-213.702579531751));
#219670=CARTESIAN_POINT('Ctrl Pts',(3.36992000515139,-75.9807926330087,
-213.674741083932));
#219671=CARTESIAN_POINT('Ctrl Pts',(3.57454157170993,-75.980659021922,-213.644239294627));
#219672=CARTESIAN_POINT('Ctrl Pts',(3.77894390642551,-75.980512799313,-213.611139249122));
#219673=CARTESIAN_POINT('Ctrl Pts',(3.78445653335865,-75.9805088557636,
-213.610246557742));
#219674=CARTESIAN_POINT('Ctrl Pts',(3.78996896840898,-75.9805049029287,
-213.609351987569));
#219675=CARTESIAN_POINT('Ctrl Pts',(3.79548121007169,-75.9805009407858,
-213.608455540887));
#219676=CARTESIAN_POINT('Ctrl Pts',(4.06858712343268,-75.9803046350508,
-213.56404078103));
#219677=CARTESIAN_POINT('Ctrl Pts',(4.34137765120749,-75.9800854014844,
-213.514997391923));
#219678=CARTESIAN_POINT('Ctrl Pts',(4.61403589949818,-75.9798400767937,
-213.461499221038));
#219679=CARTESIAN_POINT('Ctrl Pts',(4.68714478617817,-75.9797742969571,
-213.447154554271));
#219680=CARTESIAN_POINT('Ctrl Pts',(4.76024416353237,-75.979706639818,-213.432489315292));
#219681=CARTESIAN_POINT('Ctrl Pts',(4.83333754839952,-75.9796370409594,
-213.417506229945));
#219682=CARTESIAN_POINT('Ctrl Pts',(4.83391415551471,-75.9796364919194,
-213.417388033837));
#219683=CARTESIAN_POINT('Ctrl Pts',(4.8344907616134,-75.9796359427591,-213.41726981808));
#219684=CARTESIAN_POINT('Ctrl Pts',(4.83506736669369,-75.9796353934785,
-213.417151582676));
#219685=CARTESIAN_POINT('Ctrl Pts',(4.85705527089062,-75.9796144475508,
-213.412642866356));
#219686=CARTESIAN_POINT('Ctrl Pts',(4.87904219752034,-75.979593326817,-213.408105477613));
#219687=CARTESIAN_POINT('Ctrl Pts',(4.90102814896698,-75.9795720298321,
-213.40353950903));
#219688=CARTESIAN_POINT('Ctrl Pts',(4.91202112578867,-75.9795613813386,
-213.40125652451));
#219689=CARTESIAN_POINT('Ctrl Pts',(4.92301425754122,-75.9795504814521,
-213.398978167959));
#219690=CARTESIAN_POINT('Ctrl Pts',(4.93400765560909,-75.9795392721793,
-213.396707731265));
#219691=CARTESIAN_POINT('Ctrl Pts',(4.94500105464879,-75.9795280629055,
-213.39443729437));
#219692=CARTESIAN_POINT('Ctrl Pts',(4.95599468356498,-75.9795165631949,
-213.392173701309));
#219693=CARTESIAN_POINT('Ctrl Pts',(4.96698854204686,-75.9795047731424,
-213.3899169455));
#219694=CARTESIAN_POINT('Ctrl Pts',(5.01096398928681,-75.9794576129176,
-213.38088991953));
#219695=CARTESIAN_POINT('Ctrl Pts',(5.05494310946406,-75.9794058072462,
-213.371972288104));
#219696=CARTESIAN_POINT('Ctrl Pts',(5.09892588297217,-75.9793493619682,
-213.363163643794));
#219697=CARTESIAN_POINT('Ctrl Pts',(5.18689153127894,-75.9792364712821,
-213.345546334888));
#219698=CARTESIAN_POINT('Ctrl Pts',(5.27487179213221,-75.9791050224788,
-213.328364955098));
#219699=CARTESIAN_POINT('Ctrl Pts',(5.36286651682885,-75.9789550580173,
-213.31161649334));
#219700=CARTESIAN_POINT('Ctrl Pts',(5.53216176684228,-75.9786665376417,
-213.279393709186));
#219701=CARTESIAN_POINT('Ctrl Pts',(5.70151054468751,-75.9783094868255,
-213.248773074071));
#219702=CARTESIAN_POINT('Ctrl Pts',(5.8709119085587,-75.9778841486961,-213.219736583428));
#219703=CARTESIAN_POINT('Ctrl Pts',(5.87761103143291,-75.9778673283334,
-213.218588310391));
#219704=CARTESIAN_POINT('Ctrl Pts',(5.88431023694467,-75.9778504011683,
-213.217442515181));
#219705=CARTESIAN_POINT('Ctrl Pts',(5.89100952505437,-75.977833367216,-213.216299196671));
#219706=CARTESIAN_POINT('Ctrl Pts',(6.57648381222072,-75.9760904452671,
-213.099314313008));
#219707=CARTESIAN_POINT('Ctrl Pts',(7.26281953055674,-75.9732311015326,
-213.008169089905));
#219708=CARTESIAN_POINT('Ctrl Pts',(7.95000030915388,-75.9692589748972,
-212.942376327843));
#219709=CARTESIAN_POINT('Ctrl Pts',(7.96900370297949,-75.969149129149,-212.940556885554));
#219710=CARTESIAN_POINT('Ctrl Pts',(7.98800774705063,-75.96903843191,-212.938756857887));
#219711=CARTESIAN_POINT('Ctrl Pts',(8.00701244074232,-75.9689268832679,
-212.936976234005));
#219712=CARTESIAN_POINT('Ctrl Pts',(9.01669616134442,-75.9630005131925,
-212.842375027793));
#219713=CARTESIAN_POINT('Ctrl Pts',(10.0281851201039,-75.954683893227,-212.80183031115));
#219714=CARTESIAN_POINT('Ctrl Pts',(11.0415920643372,-75.9438949943452,
-212.819044947185));
#219715=CARTESIAN_POINT('Ctrl Pts',(11.4021166221425,-75.9400567899391,
-212.825169139525));
#219716=CARTESIAN_POINT('Ctrl Pts',(11.7628843913312,-75.9359056873238,
-212.838603457441));
#219717=CARTESIAN_POINT('Ctrl Pts',(12.1239020500588,-75.9314379745397,
-212.859514796659));
#219718=CARTESIAN_POINT('Ctrl Pts',(12.1677558321591,-75.9308952694997,
-212.862054953051));
#219719=CARTESIAN_POINT('Ctrl Pts',(12.2116133487246,-75.9303478845685,
-212.864705871123));
#219720=CARTESIAN_POINT('Ctrl Pts',(12.2554746014879,-75.9297958135096,
-212.86746783182));
#219721=CARTESIAN_POINT('Ctrl Pts',(12.9091879304763,-75.9215676807724,
-212.90863242261));
#219722=CARTESIAN_POINT('Ctrl Pts',(13.5637374768946,-75.9122941099966,
-212.974714278678));
#219723=CARTESIAN_POINT('Ctrl Pts',(14.2192120561195,-75.9019172187269,
-213.068681012528));
#219724=CARTESIAN_POINT('Ctrl Pts',(14.2756314127241,-75.9010240375913,
-213.076769110578));
#219725=CARTESIAN_POINT('Ctrl Pts',(14.3320574272743,-75.9001226764094,
-213.085064287729));
#219726=CARTESIAN_POINT('Ctrl Pts',(14.3884903026081,-75.8992130957741,
-213.093568472595));
#219727=CARTESIAN_POINT('Ctrl Pts',(14.6818682279193,-75.894484453505,-213.137779229139));
#219728=CARTESIAN_POINT('Ctrl Pts',(14.9756256940205,-75.8895296456064,
-213.187702769479));
#219729=CARTESIAN_POINT('Ctrl Pts',(15.2691013315942,-75.8843532160818,
-213.243611744504));
#219730=CARTESIAN_POINT('Ctrl Pts',(15.3317819141186,-75.8832476332788,
-213.25555279403));
#219731=CARTESIAN_POINT('Ctrl Pts',(15.3944477533609,-75.882131973196,-213.267766562248));
#219732=CARTESIAN_POINT('Ctrl Pts',(15.4570929624156,-75.8810062707486,
-213.280255808989));
#219733=CARTESIAN_POINT('Ctrl Pts',(15.56931266771,-75.8789897398949,-213.302628463016));
#219734=CARTESIAN_POINT('Ctrl Pts',(15.6814735367602,-75.87694090377,-213.325885882819));
#219735=CARTESIAN_POINT('Ctrl Pts',(15.7935782943546,-75.8748593371064,
-213.350053261412));
#219736=CARTESIAN_POINT('Ctrl Pts',(15.8592678329298,-75.8736396105169,
-213.364214515426));
#219737=CARTESIAN_POINT('Ctrl Pts',(15.9249374177143,-75.8724086568486,
-213.378688144354));
#219738=CARTESIAN_POINT('Ctrl Pts',(15.9905865115854,-75.8711664099023,
-213.393479023437));
#219739=CARTESIAN_POINT('Ctrl Pts',(16.0016916798719,-75.8709562720226,
-213.395981041236));
#219740=CARTESIAN_POINT('Ctrl Pts',(16.0127962614987,-75.8707458109113,
-213.39849214194));
#219741=CARTESIAN_POINT('Ctrl Pts',(16.0239002537432,-75.8705350262171,
-213.401012351154));
#219742=CARTESIAN_POINT('Ctrl Pts',(16.0350042443252,-75.8703242415545,
-213.403532559989));
#219743=CARTESIAN_POINT('Ctrl Pts',(16.0461076283636,-75.870113128927,-213.406062143155));
#219744=CARTESIAN_POINT('Ctrl Pts',(16.0572104545953,-75.8699017011283,
-213.408600328877));
#219745=CARTESIAN_POINT('Ctrl Pts',(16.068313281294,-75.8696902733207,-213.411138514705));
#219746=CARTESIAN_POINT('Ctrl Pts',(16.0794167037132,-75.8694788255209,
-213.413667399603));
#219747=CARTESIAN_POINT('Ctrl Pts',(16.0905207773752,-75.8692673721864,
-213.416186104166));
#219748=CARTESIAN_POINT('Ctrl Pts',(16.1016248536337,-75.8690559188024,
-213.418704809319));
#219749=CARTESIAN_POINT('Ctrl Pts',(16.1127295622337,-75.8688444550433,
-213.421213627703));
#219750=CARTESIAN_POINT('Ctrl Pts',(16.1238349020251,-75.868632980843,-213.423712560667));
#219751=CARTESIAN_POINT('Ctrl Pts',(16.1682563297534,-75.8677870827362,
-213.43370830795));
#219752=CARTESIAN_POINT('Ctrl Pts',(16.2126878564162,-75.8669410175819,
-213.44354588758));
#219753=CARTESIAN_POINT('Ctrl Pts',(16.2571294072557,-75.8660947811755,
-213.453225389057));
#219754=CARTESIAN_POINT('Ctrl Pts',(16.2772265474938,-75.8657121002966,
-213.45760260576));
#219755=CARTESIAN_POINT('Ctrl Pts',(16.2973257376673,-75.8653293844006,
-213.461947495525));
#219756=CARTESIAN_POINT('Ctrl Pts',(16.3174269708162,-75.8649466330907,
-213.466260067273));
#219757=CARTESIAN_POINT('Ctrl Pts',(16.3862275772071,-75.8636365879792,
-213.481020731416));
#219758=CARTESIAN_POINT('Ctrl Pts',(16.4550519918267,-75.8623261155969,
-213.495403612882));
#219759=CARTESIAN_POINT('Ctrl Pts',(16.5239002432807,-75.8610151961749,
-213.509409025261));
#219760=CARTESIAN_POINT('Ctrl Pts',(17.2221321564218,-75.8477203665076,
-213.651446414345));
#219761=CARTESIAN_POINT('Ctrl Pts',(17.9228698040644,-75.8343918984152,
-213.753884770493));
#219762=CARTESIAN_POINT('Ctrl Pts',(18.6259929002108,-75.8209788271971,
-213.818960489682));
#219763=CARTESIAN_POINT('Ctrl Pts',(19.2618685562882,-75.8088485963633,
-213.877812297936));
#219764=CARTESIAN_POINT('Ctrl Pts',(19.8996944331453,-75.7966491630361,
-213.906106594897));
#219765=CARTESIAN_POINT('Ctrl Pts',(20.5393478070102,-75.7843436373544,
-213.905482499602));
#219766=CARTESIAN_POINT('Ctrl Pts',(20.6343955077762,-75.7825151283986,
-213.905389763715));
#219767=CARTESIAN_POINT('Ctrl Pts',(20.7294829484021,-75.780684194172,-213.904663931103));
#219768=CARTESIAN_POINT('Ctrl Pts',(20.8246099557498,-75.7788507122291,
-213.903310241351));
#219769=CARTESIAN_POINT('Ctrl Pts',(21.4384220517384,-75.7670200720597,
-213.894575485918));
#219770=CARTESIAN_POINT('Ctrl Pts',(22.0538553854744,-75.7550759076376,
-213.860164387392));
#219771=CARTESIAN_POINT('Ctrl Pts',(22.6707441337976,-75.742964226742,-213.802911549687));
#219772=CARTESIAN_POINT('Ctrl Pts',(22.7791427338394,-75.7408359835915,
-213.792851182282));
#219773=CARTESIAN_POINT('Ctrl Pts',(22.8875828374366,-75.738702595359,-213.782088145393));
#219774=CARTESIAN_POINT('Ctrl Pts',(22.9960671998898,-75.7365636899579,
-213.770637922095));
#219775=CARTESIAN_POINT('Ctrl Pts',(23.1775336789479,-75.7329858505033,
-213.751484638991));
#219776=CARTESIAN_POINT('Ctrl Pts',(23.3591607784853,-75.729391712817,-213.730411774765));
#219777=CARTESIAN_POINT('Ctrl Pts',(23.5408109811078,-75.7257824438295,
-213.707516230951));
#219778=CARTESIAN_POINT('Ctrl Pts',(23.6074556822628,-75.7244582578413,
-213.699116203572));
#219779=CARTESIAN_POINT('Ctrl Pts',(23.6741036716134,-75.7231320329098,
-213.690470919469));
#219780=CARTESIAN_POINT('Ctrl Pts',(23.7407558015218,-75.7218036786003,
-213.681584355796));
#219781=CARTESIAN_POINT('Ctrl Pts',(23.7649272860614,-75.7213219491238,
-213.67836163153));
#219782=CARTESIAN_POINT('Ctrl Pts',(23.7890994558372,-75.7208399367944,
-213.675107155865));
#219783=CARTESIAN_POINT('Ctrl Pts',(23.8132721536629,-75.7203576411583,
-213.671821148346));
#219784=CARTESIAN_POINT('Ctrl Pts',(23.8586819366496,-75.719451621469,-213.665648196968));
#219785=CARTESIAN_POINT('Ctrl Pts',(23.9040935831152,-75.7185446020397,
-213.659363966219));
#219786=CARTESIAN_POINT('Ctrl Pts',(23.9495060511029,-75.7176365802963,
-213.652969909908));
#219787=CARTESIAN_POINT('Ctrl Pts',(23.9722118101336,-75.7171825789216,
-213.649772948628));
#219788=CARTESIAN_POINT('Ctrl Pts',(23.9949178430555,-75.7167286260788,
-213.646531313061));
#219789=CARTESIAN_POINT('Ctrl Pts',(24.0176237567913,-75.716273574272,-213.64331123187));
#219790=CARTESIAN_POINT('Ctrl Pts',(24.040329699698,-75.7158185218806,-213.640091146543));
#219791=CARTESIAN_POINT('Ctrl Pts',(24.0630355105879,-75.715362314347,-213.636895849934));
#219792=CARTESIAN_POINT('Ctrl Pts',(24.0857410597618,-75.7149049538362,
-213.63372538747));
#219793=CARTESIAN_POINT('Ctrl Pts',(24.149226200756,-75.7136261652772,-213.624860715005));
#219794=CARTESIAN_POINT('Ctrl Pts',(24.2127092960951,-75.7123383647039,
-213.616190085964));
#219795=CARTESIAN_POINT('Ctrl Pts',(24.2761875099214,-75.7110415995584,
-213.60771456582));
#219796=CARTESIAN_POINT('Ctrl Pts',(24.4546501076116,-75.707395875104,-213.583886495517));
#219797=CARTESIAN_POINT('Ctrl Pts',(24.6330855092358,-75.7036790698468,
-213.561598684543));
#219798=CARTESIAN_POINT('Ctrl Pts',(24.811493481113,-75.6998909745234,-213.540865649074));
#219799=CARTESIAN_POINT('Ctrl Pts',(24.9328485812406,-75.6973142696687,
-213.526762806198));
#219800=CARTESIAN_POINT('Ctrl Pts',(25.0541916184914,-75.694704503639,-213.51338286188));
#219801=CARTESIAN_POINT('Ctrl Pts',(25.1755222227724,-75.6920616293237,
-213.500729684749));
#219802=CARTESIAN_POINT('Ctrl Pts',(25.9054256855671,-75.6761625647317,
-213.42461040835));
#219803=CARTESIAN_POINT('Ctrl Pts',(26.6348775042369,-75.6590755014285,
-213.374208344441));
#219804=CARTESIAN_POINT('Ctrl Pts',(27.3638191453224,-75.6407602143513,
-213.352071040965));
#219805=CARTESIAN_POINT('Ctrl Pts',(27.9388020795704,-75.6263132724952,
-213.334609325251));
#219806=CARTESIAN_POINT('Ctrl Pts',(28.5134684250624,-75.6111021500901,
-213.334733221256));
#219807=CARTESIAN_POINT('Ctrl Pts',(29.0878122600391,-75.5951066404747,
-213.353691247444));
#219808=CARTESIAN_POINT('Ctrl Pts',(29.2361430259429,-75.5909756199121,
-213.358587371287));
#219809=CARTESIAN_POINT('Ctrl Pts',(29.3844524585103,-75.5867919458944,
-213.364758607598));
#219810=CARTESIAN_POINT('Ctrl Pts',(29.5327391727653,-75.5825553544812,
-213.372223725378));
#219811=CARTESIAN_POINT('Ctrl Pts',(30.095996724499,-75.5664629343402,-213.400579495384));
#219812=CARTESIAN_POINT('Ctrl Pts',(30.6589214000291,-75.5496030053619,
-213.447840466442));
#219813=CARTESIAN_POINT('Ctrl Pts',(31.2214620547992,-75.5319252870199,
-213.517061341304));
#219814=CARTESIAN_POINT('Ctrl Pts',(31.3845113472357,-75.5268014982891,
-213.537124628415));
#219815=CARTESIAN_POINT('Ctrl Pts',(31.5473250535973,-75.5216152683976,
-213.559016745048));
#219816=CARTESIAN_POINT('Ctrl Pts',(31.7100818423904,-75.5163598790567,
-213.582831843075));
#219817=CARTESIAN_POINT('Ctrl Pts',(31.9201729023719,-75.5095760740589,
-213.613573044256));
#219818=CARTESIAN_POINT('Ctrl Pts',(32.1304868253325,-75.5026645193156,
-213.647621648096));
#219819=CARTESIAN_POINT('Ctrl Pts',(32.3408536996831,-75.4956277389932,
-213.685202481806));
#219820=CARTESIAN_POINT('Ctrl Pts',(32.5391806661271,-75.4889936940697,
-213.720632455128));
#219821=CARTESIAN_POINT('Ctrl Pts',(32.7375557017912,-75.4822483051993,
-213.759202024971));
#219822=CARTESIAN_POINT('Ctrl Pts',(32.9358259199764,-75.4753925207355,
-213.801143310705));
#219823=CARTESIAN_POINT('Ctrl Pts',(33.0744170048196,-75.470600320399,-213.830460312233));
#219824=CARTESIAN_POINT('Ctrl Pts',(33.2129566775175,-75.4657541566474,
-213.861425618706));
#219825=CARTESIAN_POINT('Ctrl Pts',(33.3513856130173,-75.4608541370173,
-213.894132075576));
#219826=CARTESIAN_POINT('',(-24.3802580872756,-74.7628322230906,-216.457148834596));
#219827=CARTESIAN_POINT('Ctrl Pts',(-32.863845486296,-74.788639230448,-216.296979356596));
#219828=CARTESIAN_POINT('Ctrl Pts',(-32.3897890127524,-74.7876292350666,
-216.21237071581));
#219829=CARTESIAN_POINT('Ctrl Pts',(-31.9064151032494,-74.7864231071773,
-216.148265135018));
#219830=CARTESIAN_POINT('Ctrl Pts',(-30.8096937949103,-74.783832940506,
-216.043994115321));
#219831=CARTESIAN_POINT('Ctrl Pts',(-30.1907416630467,-74.7824030861366,
-216.013146550001));
#219832=CARTESIAN_POINT('Ctrl Pts',(-28.3232034263091,-74.7780118788819,
-215.992921294503));
#219833=CARTESIAN_POINT('Ctrl Pts',(-27.0679146701128,-74.7750988404896,
-216.073704234167));
#219834=CARTESIAN_POINT('Ctrl Pts',(-25.4971541039145,-74.7685482393304,
-216.276993162089));
#219835=CARTESIAN_POINT('Ctrl Pts',(-25.1828553480248,-74.7670902389161,
-216.322863772022));
#219836=CARTESIAN_POINT('Ctrl Pts',(-24.7112165018673,-74.7646638286032,
-216.399367062212));
#219837=CARTESIAN_POINT('Ctrl Pts',(-24.5539718322166,-74.7638151669929,
-216.426151417743));
#219838=CARTESIAN_POINT('Ctrl Pts',(-24.3915131858716,-74.7628960486129,
-216.455136152234));
#219839=CARTESIAN_POINT('Ctrl Pts',(-24.3859775141005,-74.7629941311872,
-216.455944332801));
#219840=CARTESIAN_POINT('Ctrl Pts',(-24.3802580872756,-74.7628322230906,
-216.457148834596));
#219841=CARTESIAN_POINT('',(-15.4710514507746,-75.1252161784242,-215.898656021024));
#219842=CARTESIAN_POINT('Ctrl Pts',(-24.3802580872756,-74.7628322230906,
-216.457148834596));
#219843=CARTESIAN_POINT('Ctrl Pts',(-24.3593193041524,-74.7638570105243,
-216.459291035607));
#219844=CARTESIAN_POINT('Ctrl Pts',(-24.3356346771204,-74.7655513238598,
-216.460962733904));
#219845=CARTESIAN_POINT('Ctrl Pts',(-24.2899211502609,-74.7683276680052,
-216.464803183085));
#219846=CARTESIAN_POINT('Ctrl Pts',(-24.2213401559703,-74.7724835783518,
-216.470497497242));
#219847=CARTESIAN_POINT('Ctrl Pts',(-24.0612427007151,-74.7821202755749,
-216.483317127563));
#219848=CARTESIAN_POINT('Ctrl Pts',(-23.9238868015989,-74.7902760704183,
-216.493495745774));
#219849=CARTESIAN_POINT('Ctrl Pts',(-23.6490005011524,-74.8064468993936,
-216.512749384951));
#219850=CARTESIAN_POINT('Ctrl Pts',(-23.0984533463628,-74.8382473041046,
-216.546816326886));
#219851=CARTESIAN_POINT('Ctrl Pts',(-22.5457350571009,-74.8683220564567,
-216.56702542312));
#219852=CARTESIAN_POINT('Ctrl Pts',(-21.4378390571114,-74.9258908205721,
-216.587544672568));
#219853=CARTESIAN_POINT('Ctrl Pts',(-20.6958771255011,-74.9607892729635,
-216.574455021372));
#219854=CARTESIAN_POINT('Ctrl Pts',(-19.207074977151,-75.0225411715837,
-216.488342549631));
#219855=CARTESIAN_POINT('Ctrl Pts',(-18.4604021561735,-75.0494131998981,
-216.415548765925));
#219856=CARTESIAN_POINT('Ctrl Pts',(-17.3393212995558,-75.0829993251798,
-216.258218186126));
#219857=CARTESIAN_POINT('Ctrl Pts',(-16.965457286696,-75.0930660264359,
-216.197703030854));
#219858=CARTESIAN_POINT('Ctrl Pts',(-16.3111878076399,-75.1086524189823,
-216.077446851186));
#219859=CARTESIAN_POINT('Ctrl Pts',(-16.0307837607371,-75.1146887137984,
-216.021340208994));
#219860=CARTESIAN_POINT('Ctrl Pts',(-15.7037899646612,-75.1209827194714,
-215.950528672311));
#219861=CARTESIAN_POINT('Ctrl Pts',(-15.6570792202537,-75.1218640593031,
-215.940285071964));
#219862=CARTESIAN_POINT('Ctrl Pts',(-15.5870218132984,-75.123159310396,
-215.924728992095));
#219863=CARTESIAN_POINT('Ctrl Pts',(-15.5636711778655,-75.1235865944026,
-215.91951195042));
#219864=CARTESIAN_POINT('Ctrl Pts',(-15.5169735358771,-75.124432237608,
-215.90901446866));
#219865=CARTESIAN_POINT('Ctrl Pts',(-15.4919351428462,-75.1249550271076,
-215.903217577102));
#219866=CARTESIAN_POINT('Ctrl Pts',(-15.4710515403103,-75.1252154310809,
-215.898655568186));
#219867=CARTESIAN_POINT('',(-5.46041973257396,-75.1055542085046,-216.081029782323));
#219868=CARTESIAN_POINT('Ctrl Pts',(-15.4710513612508,-75.1252169257673,
-215.898656473865));
#219869=CARTESIAN_POINT('Ctrl Pts',(-15.4532848117673,-75.1254395973537,
-215.894776408977));
#219870=CARTESIAN_POINT('Ctrl Pts',(-15.4393547346688,-75.1254225509925,
-215.892050193159));
#219871=CARTESIAN_POINT('Ctrl Pts',(-15.4238009726903,-75.1255059168102,
-215.888868014377));
#219872=CARTESIAN_POINT('Ctrl Pts',(-15.4139021823397,-75.125558972833,
-215.886842798828));
#219873=CARTESIAN_POINT('Ctrl Pts',(-15.4040019487999,-75.1256117765925,
-215.884825471668));
#219874=CARTESIAN_POINT('Ctrl Pts',(-15.3941002813744,-75.1256643291047,
-215.882816013199));
#219875=CARTESIAN_POINT('Ctrl Pts',(-15.3848027542714,-75.125713675178,
-215.880929159826));
#219876=CARTESIAN_POINT('Ctrl Pts',(-15.3755039630117,-75.1257627998731,
-215.879049244014));
#219877=CARTESIAN_POINT('Ctrl Pts',(-15.3662039151108,-75.1258117037368,
-215.877176249902));
#219878=CARTESIAN_POINT('Ctrl Pts',(-15.3500371100749,-75.1258967161193,
-215.87392031714));
#219879=CARTESIAN_POINT('Ctrl Pts',(-15.3338665084111,-75.1259810613781,
-215.870685298734));
#219880=CARTESIAN_POINT('Ctrl Pts',(-15.3176921482388,-75.1260647420003,
-215.867471115233));
#219881=CARTESIAN_POINT('Ctrl Pts',(-15.2667346398205,-75.1263283787665,
-215.857344793014));
#219882=CARTESIAN_POINT('Ctrl Pts',(-15.2157398292535,-75.126585424701,
-215.84742526286));
#219883=CARTESIAN_POINT('Ctrl Pts',(-15.1647089702132,-75.1268360572174,
-215.837709888246));
#219884=CARTESIAN_POINT('Ctrl Pts',(-15.1549733482384,-75.1268838726663,
-215.835856397704));
#219885=CARTESIAN_POINT('Ctrl Pts',(-15.1452364133038,-75.1269314532125,
-215.834010339996));
#219886=CARTESIAN_POINT('Ctrl Pts',(-15.1354981739144,-75.1269787997638,
-215.832171697309));
#219887=CARTESIAN_POINT('Ctrl Pts',(-15.0431472560069,-75.1274278026377,
-215.814735245702));
#219888=CARTESIAN_POINT('Ctrl Pts',(-14.9506790955974,-75.1278557796285,
-215.797965447865));
#219889=CARTESIAN_POINT('Ctrl Pts',(-14.8581003871648,-75.1282633600128,
-215.781848690665));
#219890=CARTESIAN_POINT('Ctrl Pts',(-14.7963296830584,-75.1285353072859,
-215.771095209039));
#219891=CARTESIAN_POINT('Ctrl Pts',(-14.7345097643979,-75.1287981742431,
-215.760632452894));
#219892=CARTESIAN_POINT('Ctrl Pts',(-14.6726426166134,-75.1290521427022,
-215.750456386401));
#219893=CARTESIAN_POINT('Ctrl Pts',(-14.0542810189402,-75.1315905552163,
-215.648746691346));
#219894=CARTESIAN_POINT('Ctrl Pts',(-13.4312745436638,-75.133248132206,
-215.575545102645));
#219895=CARTESIAN_POINT('Ctrl Pts',(-12.8050954815233,-75.1341130418415,
-215.528043650926));
#219896=CARTESIAN_POINT('Ctrl Pts',(-11.5527373572422,-75.1358428611124,
-215.433040747489));
#219897=CARTESIAN_POINT('Ctrl Pts',(-10.2877748918477,-75.1344540393816,
-215.439867099146));
#219898=CARTESIAN_POINT('Ctrl Pts',(-9.0182067883447,-75.1295474748707,
-215.541642492796));
#219899=CARTESIAN_POINT('Ctrl Pts',(-8.38342273659319,-75.1270941926152,
-215.592530189621));
#219900=CARTESIAN_POINT('Ctrl Pts',(-7.74627999058338,-75.123730716052,
-215.66762028791));
#219901=CARTESIAN_POINT('Ctrl Pts',(-7.11146965938098,-75.119358125502,
-215.766852735003));
#219902=CARTESIAN_POINT('Ctrl Pts',(-6.79406449377977,-75.117171830227,
-215.81646895855));
#219903=CARTESIAN_POINT('Ctrl Pts',(-6.47783883753869,-75.1147362439731,
-215.87201775923));
#219904=CARTESIAN_POINT('Ctrl Pts',(-6.1629111324363,-75.1120324006556,
-215.933512637504));
#219905=CARTESIAN_POINT('Ctrl Pts',(-6.03250386903793,-75.1109127760498,
-215.95897682709));
#219906=CARTESIAN_POINT('Ctrl Pts',(-5.90231929343371,-75.1097471139405,
-215.985461175739));
#219907=CARTESIAN_POINT('Ctrl Pts',(-5.77236656503421,-75.108533846862,
-216.012969613053));
#219908=CARTESIAN_POINT('Ctrl Pts',(-5.74540428172294,-75.1082821210914,
-216.018676998265));
#219909=CARTESIAN_POINT('Ctrl Pts',(-5.71845197873014,-75.1080283460713,
-216.024428467385));
#219910=CARTESIAN_POINT('Ctrl Pts',(-5.69150973786122,-75.1077725078021,
-216.03022405551));
#219911=CARTESIAN_POINT('Ctrl Pts',(-5.66646960728471,-75.1075347316017,
-216.035610477676));
#219912=CARTESIAN_POINT('Ctrl Pts',(-5.64143825767027,-75.1072951740359,
-216.041034985145));
#219913=CARTESIAN_POINT('Ctrl Pts',(-5.61641111550247,-75.1070537769128,
-216.046498659192));
#219914=CARTESIAN_POINT('Ctrl Pts',(-5.60225899656066,-75.1069172738804,
-216.049588207509));
#219915=CARTESIAN_POINT('Ctrl Pts',(-5.5881082229804,-75.1067801826414,
-216.052690279619));
#219916=CARTESIAN_POINT('Ctrl Pts',(-5.57395797348773,-75.1066424926987,
-216.055805069817));
#219917=CARTESIAN_POINT('Ctrl Pts',(-5.56213395055293,-75.106527438258,
-216.058407804897));
#219918=CARTESIAN_POINT('Ctrl Pts',(-5.5503106939716,-75.1064119695425,
-216.061019334865));
#219919=CARTESIAN_POINT('Ctrl Pts',(-5.5384882141471,-75.1062960850126,
-216.06363966873));
#219920=CARTESIAN_POINT('Ctrl Pts',(-5.53072620436407,-75.1062200014103,
-216.065360040209));
#219921=CARTESIAN_POINT('Ctrl Pts',(-5.52296450117121,-75.1061437384122,
-216.067084212726));
#219922=CARTESIAN_POINT('Ctrl Pts',(-5.51520313283029,-75.1060672957268,
-216.068812183402));
#219923=CARTESIAN_POINT('Ctrl Pts',(-5.50998013296097,-75.1060158537493,
-216.069975018384));
#219924=CARTESIAN_POINT('Ctrl Pts',(-5.50475728473136,-75.1059643304001,
-216.071139573398));
#219925=CARTESIAN_POINT('Ctrl Pts',(-5.49953459675603,-75.1059127255892,
-216.072305847558));
#219926=CARTESIAN_POINT('Ctrl Pts',(-5.4949664419899,-75.1058675881496,
-216.073325958444));
#219927=CARTESIAN_POINT('Ctrl Pts',(-5.49039840272466,-75.1058223886675,
-216.074347385634));
#219928=CARTESIAN_POINT('Ctrl Pts',(-5.48583047998682,-75.1057771267157,
-216.075370130076));
#219929=CARTESIAN_POINT('Ctrl Pts',(-5.47741546935228,-75.1056937453129,
-216.077254226161));
#219930=CARTESIAN_POINT('Ctrl Pts',(-5.47001733418767,-75.1054407487899,
-216.079184123322));
#219931=CARTESIAN_POINT('Ctrl Pts',(-5.46041973163172,-75.1055542085157,
-216.081029782504));
#219932=CARTESIAN_POINT('',(-2.08228321273563E-9,-75.1718294574641,-216.556685219365));
#219933=CARTESIAN_POINT('Ctrl Pts',(-5.46041973163172,-75.1055542085157,
-216.081029782504));
#219934=CARTESIAN_POINT('Ctrl Pts',(-5.45885110379661,-75.1055727671836,
-216.081331414038));
#219935=CARTESIAN_POINT('Ctrl Pts',(-5.45722372289247,-75.1056011148421,
-216.08163079528));
#219936=CARTESIAN_POINT('Ctrl Pts',(-5.45552354686627,-75.1056415918994,
-216.081927358492));
#219937=CARTESIAN_POINT('Ctrl Pts',(-5.42896346001207,-75.1062739229874,
-216.086560258006));
#219938=CARTESIAN_POINT('Ctrl Pts',(-5.4023997922979,-75.1069019363042,
-216.091161602676));
#219939=CARTESIAN_POINT('Ctrl Pts',(-5.37583248801623,-75.1075256256449,
-216.095731281078));
#219940=CARTESIAN_POINT('Ctrl Pts',(-5.34756454570321,-75.1081892388635,
-216.100593475754));
#219941=CARTESIAN_POINT('Ctrl Pts',(-5.31929239183766,-75.1088479905342,
-216.105419789335));
#219942=CARTESIAN_POINT('Ctrl Pts',(-5.29101614121995,-75.109501813166,
-216.110210140245));
#219943=CARTESIAN_POINT('Ctrl Pts',(-5.24899125576366,-75.1104735410511,
-216.117329682048));
#219944=CARTESIAN_POINT('Ctrl Pts',(-5.2069570409512,-75.1114344776116,
-216.124369701056));
#219945=CARTESIAN_POINT('Ctrl Pts',(-5.16491312624508,-75.1123846717332,
-216.131329677671));
#219946=CARTESIAN_POINT('Ctrl Pts',(-5.15037893222956,-75.1127131450881,
-216.133735677474));
#219947=CARTESIAN_POINT('Ctrl Pts',(-5.13584345917987,-75.1130403536024,
-216.136132065221));
#219948=CARTESIAN_POINT('Ctrl Pts',(-5.12130671024801,-75.1133662960798,
-216.138518821461));
#219949=CARTESIAN_POINT('Ctrl Pts',(-5.00813060145967,-75.1159039268427,
-216.157100953211));
#219950=CARTESIAN_POINT('Ctrl Pts',(-4.89487775170335,-75.1183645441208,
-216.17509957011));
#219951=CARTESIAN_POINT('Ctrl Pts',(-4.7815505844652,-75.1207471055566,
-216.192506042143));
#219952=CARTESIAN_POINT('Ctrl Pts',(-4.13290185680472,-75.1343841308309,
-216.292135162081));
#219953=CARTESIAN_POINT('Ctrl Pts',(-3.48181844620929,-75.1454639977537,
-216.372365290844));
#219954=CARTESIAN_POINT('Ctrl Pts',(-2.82877069498839,-75.1537838320299,
-216.431585941174));
#219955=CARTESIAN_POINT('Ctrl Pts',(-2.4378715048134,-75.1587638912597,
-216.467034044643));
#219956=CARTESIAN_POINT('Ctrl Pts',(-2.04648484597347,-75.1627399695325,
-216.49496695171));
#219957=CARTESIAN_POINT('Ctrl Pts',(-1.6545361090901,-75.1656914643869,
-216.51520608631));
#219958=CARTESIAN_POINT('Ctrl Pts',(-1.55726525698595,-75.1664239438987,
-216.520228880576));
#219959=CARTESIAN_POINT('Ctrl Pts',(-1.45999630524016,-75.1670898141191,
-216.524764978152));
#219960=CARTESIAN_POINT('Ctrl Pts',(-1.36278838454174,-75.1676893633231,
-216.528830176404));
#219961=CARTESIAN_POINT('Ctrl Pts',(-1.0683010862481,-75.1695056723644,
-216.541145523156));
#219962=CARTESIAN_POINT('Ctrl Pts',(-0.774374080750881,-75.1707133120289,
-216.549139133372));
#219963=CARTESIAN_POINT('Ctrl Pts',(-0.482651045412875,-75.1713202986035,
-216.553250233342));
#219964=CARTESIAN_POINT('Ctrl Pts',(-0.32135449366988,-75.1716559074844,
-216.55552330118));
#219965=CARTESIAN_POINT('Ctrl Pts',(-0.160674879972797,-75.1718268822641,
-216.556675869296));
#219966=CARTESIAN_POINT('Ctrl Pts',(-2.08390146224025E-9,-75.1718294574641,
-216.556685219365));
#219967=CARTESIAN_POINT('',(5.46042745654276,-75.1055279660516,-216.081066924971));
#219968=CARTESIAN_POINT('Ctrl Pts',(5.46042745578382,-75.1055279660664,
-216.081066925108));
#219969=CARTESIAN_POINT('Ctrl Pts',(5.45993480282964,-75.1055396823069,
-216.08115292583));
#219970=CARTESIAN_POINT('Ctrl Pts',(5.45943508011546,-75.105552577858,-216.081238659116));
#219971=CARTESIAN_POINT('Ctrl Pts',(5.45892782922234,-75.1055667291498,
-216.081324107006));
#219972=CARTESIAN_POINT('Ctrl Pts',(5.43445808519729,-75.106249386377,-216.08544610666));
#219973=CARTESIAN_POINT('Ctrl Pts',(5.41003401191501,-75.1069218819067,
-216.089540658102));
#219974=CARTESIAN_POINT('Ctrl Pts',(5.38565413548417,-75.1075845285616,
-216.093607913568));
#219975=CARTESIAN_POINT('Ctrl Pts',(5.18349069268347,-75.1130793443166,
-216.127334514682));
#219976=CARTESIAN_POINT('Ctrl Pts',(4.98432744151869,-75.1178998244099,
-216.159195131404));
#219977=CARTESIAN_POINT('Ctrl Pts',(4.7873988108972,-75.1222097067706,-216.189233242711));
#219978=CARTESIAN_POINT('Ctrl Pts',(4.59346686514457,-75.1264540051721,
-216.218814260739));
#219979=CARTESIAN_POINT('Ctrl Pts',(4.40170187503902,-75.1302028561389,
-216.246627797542));
#219980=CARTESIAN_POINT('Ctrl Pts',(4.2113748109516,-75.133596771578,-216.272668667851));
#219981=CARTESIAN_POINT('Ctrl Pts',(4.02263252030788,-75.1369624273102,
-216.29849270678));
#219982=CARTESIAN_POINT('Ctrl Pts',(3.83539560876742,-75.1399698220657,
-216.322564617354));
#219983=CARTESIAN_POINT('Ctrl Pts',(3.64894511433005,-75.1427408218472,
-216.344863570406));
#219984=CARTESIAN_POINT('Ctrl Pts',(3.46350264848808,-75.1454968404561,
-216.367041966081));
#219985=CARTESIAN_POINT('Ctrl Pts',(3.27883802569263,-75.1480189080841,
-216.387466521769));
#219986=CARTESIAN_POINT('Ctrl Pts',(3.0942537415948,-75.1504164842619,-216.406067479382));
#219987=CARTESIAN_POINT('Ctrl Pts',(2.97606961646031,-75.1519515848497,
-216.417977149335));
#219988=CARTESIAN_POINT('Ctrl Pts',(2.8579186272538,-75.1534354475146,-216.429138253026));
#219989=CARTESIAN_POINT('Ctrl Pts',(2.73962012210223,-75.1548947920788,
-216.439521688862));
#219990=CARTESIAN_POINT('Ctrl Pts',(2.47563199262865,-75.1581513813423,
-216.462692766133));
#219991=CARTESIAN_POINT('Ctrl Pts',(2.20960587740754,-75.1609796487111,
-216.482597308869));
#219992=CARTESIAN_POINT('Ctrl Pts',(1.94119260980385,-75.1633477206973,
-216.499030144061));
#219993=CARTESIAN_POINT('Ctrl Pts',(1.91262982784451,-75.1635997154083,
-216.500778818755));
#219994=CARTESIAN_POINT('Ctrl Pts',(1.88404001758171,-75.16384649255,-216.502488132198));
#219995=CARTESIAN_POINT('Ctrl Pts',(1.85542276083298,-75.1640880090813,
-216.504157802307));
#219996=CARTESIAN_POINT('Ctrl Pts',(1.6615865500581,-75.1657238978628,-216.515467150717));
#219997=CARTESIAN_POINT('Ctrl Pts',(1.46632769852334,-75.167117630478,-216.524914581302));
#219998=CARTESIAN_POINT('Ctrl Pts',(1.27012448174892,-75.1682493321424,
-216.532526663344));
#219999=CARTESIAN_POINT('Ctrl Pts',(1.0739212649745,-75.1693810338068,-216.540138745386));
#220000=CARTESIAN_POINT('Ctrl Pts',(0.876772908783234,-75.1702507211618,
-216.545915388321));
#220001=CARTESIAN_POINT('Ctrl Pts',(0.679214520499131,-75.1708359333832,
-216.549878882062));
#220002=CARTESIAN_POINT('Ctrl Pts',(0.514175265018196,-75.1713248166453,
-216.553189964228));
#220003=CARTESIAN_POINT('Ctrl Pts',(0.348963760683292,-75.1716349551876,
-216.555303266427));
#220004=CARTESIAN_POINT('Ctrl Pts',(0.182855563317092,-75.1717627023986,
-216.556196336037));
#220005=CARTESIAN_POINT('Ctrl Pts',(0.122036851785086,-75.1718094756518,
-216.556523323771));
#220006=CARTESIAN_POINT('Ctrl Pts',(0.0610974427796169,-75.17183179282,
-216.556686693538));
#220007=CARTESIAN_POINT('Ctrl Pts',(-2.08228314334659E-9,-75.1718294574641,
-216.556685219365));
#220008=CARTESIAN_POINT('Ctrl Pts',(15.4710515403117,-75.1252154310692,
-215.898655568178));
#220009=CARTESIAN_POINT('Ctrl Pts',(15.4710444072622,-75.1252155180421,
-215.898654010539));
#220010=CARTESIAN_POINT('Ctrl Pts',(15.4710372753328,-75.1252156049439,
-215.898652453234));
#220011=CARTESIAN_POINT('Ctrl Pts',(15.4710301445247,-75.1252156917747,
-215.898650896265));
#220012=CARTESIAN_POINT('Ctrl Pts',(15.4632205313114,-75.1253107882393,
-215.89694571343));
#220013=CARTESIAN_POINT('Ctrl Pts',(15.4566954720675,-75.1253250136118,
-215.895632435197));
#220014=CARTESIAN_POINT('Ctrl Pts',(15.4500821771012,-75.1253433777805,
-215.894298660203));
#220015=CARTESIAN_POINT('Ctrl Pts',(15.4473001599164,-75.1253511030419,
-215.893737580594));
#220016=CARTESIAN_POINT('Ctrl Pts',(15.4445019222413,-75.1253595982398,
-215.89317269173));
#220017=CARTESIAN_POINT('Ctrl Pts',(15.4415826360871,-75.1253753548161,
-215.892572501974));
#220018=CARTESIAN_POINT('Ctrl Pts',(15.431805521493,-75.1254281258855,-215.890562379049));
#220019=CARTESIAN_POINT('Ctrl Pts',(15.4219863172516,-75.125480885207,-215.888551578341));
#220020=CARTESIAN_POINT('Ctrl Pts',(15.4121257804215,-75.1255336230737,
-215.886540432606));
#220021=CARTESIAN_POINT('Ctrl Pts',(15.3125359516136,-75.1260662670059,
-215.866228185619));
#220022=CARTESIAN_POINT('Ctrl Pts',(15.2087290430498,-75.1265966180202,
-215.845884352904));
#220023=CARTESIAN_POINT('Ctrl Pts',(15.1014911451759,-75.1271154275382,
-215.825827329062));
#220024=CARTESIAN_POINT('Ctrl Pts',(15.0483340175637,-75.1273725980377,
-215.815885192961));
#220025=CARTESIAN_POINT('Ctrl Pts',(14.994334045534,-75.1276269586628,-215.806012782418));
#220026=CARTESIAN_POINT('Ctrl Pts',(14.9395881264798,-75.1278775432677,
-215.796244204861));
#220027=CARTESIAN_POINT('Ctrl Pts',(14.8328496966638,-75.1283661094974,
-215.777198353628));
#220028=CARTESIAN_POINT('Ctrl Pts',(14.7232666795004,-75.1288402890429,
-215.758549615031));
#220029=CARTESIAN_POINT('Ctrl Pts',(14.6116090761272,-75.1292936107873,
-215.740523436667));
#220030=CARTESIAN_POINT('Ctrl Pts',(14.4998196734473,-75.1297474676273,
-215.722475980418));
#220031=CARTESIAN_POINT('Ctrl Pts',(14.3859511729408,-75.1301804134914,
-215.705052733827));
#220032=CARTESIAN_POINT('Ctrl Pts',(14.2707946954948,-75.1305875112326,
-215.688430822599));
#220033=CARTESIAN_POINT('Ctrl Pts',(14.1775809961871,-75.1309170375196,
-215.674976174892));
#220034=CARTESIAN_POINT('Ctrl Pts',(14.08352386201,-75.1312296577405,-215.662045641129));
#220035=CARTESIAN_POINT('Ctrl Pts',(13.9890487123067,-75.131523511689,-215.649708842601));
#220036=CARTESIAN_POINT('Ctrl Pts',(13.8706173590175,-75.1318918786183,
-215.634243783804));
#220037=CARTESIAN_POINT('Ctrl Pts',(13.7514956746712,-75.1322310618388,
-215.619703035971));
#220038=CARTESIAN_POINT('Ctrl Pts',(13.6324649705354,-75.1325385051961,
-215.606174570825));
#220039=CARTESIAN_POINT('Ctrl Pts',(13.5110600892106,-75.1328520807948,
-215.592376267964));
#220040=CARTESIAN_POINT('Ctrl Pts',(13.3897499113001,-75.1331326371434,
-215.579631007093));
#220041=CARTESIAN_POINT('Ctrl Pts',(13.269366485729,-75.1333791353553,-215.567977329651));
#220042=CARTESIAN_POINT('Ctrl Pts',(13.1857541228561,-75.1335503408002,
-215.559883262694));
#220043=CARTESIAN_POINT('Ctrl Pts',(13.1025888908574,-75.1337051523037,
-215.552314606038));
#220044=CARTESIAN_POINT('Ctrl Pts',(13.0201501679703,-75.1338436762563,
-215.545269564757));
#220045=CARTESIAN_POINT('Ctrl Pts',(12.74793949394,-75.1343010790058,-215.522007008418));
#220046=CARTESIAN_POINT('Ctrl Pts',(12.4736131226656,-75.1346118390224,
-215.503567904302));
#220047=CARTESIAN_POINT('Ctrl Pts',(12.1974965686788,-75.1347541683181,
-215.489955494028));
#220048=CARTESIAN_POINT('Ctrl Pts',(12.158295281145,-75.1347743753341,-215.488022889838));
#220049=CARTESIAN_POINT('Ctrl Pts',(12.1190579304802,-75.1347911879743,
-215.486187491866));
#220050=CARTESIAN_POINT('Ctrl Pts',(12.079785468434,-75.134804544487,-215.484449227347));
#220051=CARTESIAN_POINT('Ctrl Pts',(11.9686573435008,-75.1348423390162,
-215.479530511623));
#220052=CARTESIAN_POINT('Ctrl Pts',(11.8572498437104,-75.1348526804321,
-215.475382902043));
#220053=CARTESIAN_POINT('Ctrl Pts',(11.745583751326,-75.1348334804312,-215.472014693408));
#220054=CARTESIAN_POINT('Ctrl Pts',(11.531040929044,-75.1347965916827,-215.465543391591));
#220055=CARTESIAN_POINT('Ctrl Pts',(11.3155447321185,-75.134682579359,-215.461900568881));
#220056=CARTESIAN_POINT('Ctrl Pts',(11.0992457878686,-75.1344846717163,
-215.461123426466));
#220057=CARTESIAN_POINT('Ctrl Pts',(10.9910963157436,-75.134385717895,-215.460734855258));
#220058=CARTESIAN_POINT('Ctrl Pts',(10.8827460955464,-75.1342626066487,
-215.46106738632));
#220059=CARTESIAN_POINT('Ctrl Pts',(10.7742145999442,-75.1341148057718,
-215.462123878904));
#220060=CARTESIAN_POINT('Ctrl Pts',(10.719948852143,-75.1340409053334,-215.462652125196));
#220061=CARTESIAN_POINT('Ctrl Pts',(10.665637788193,-75.1339608327989,-215.463361348184));
#220062=CARTESIAN_POINT('Ctrl Pts',(10.6112838593016,-75.1338745235653,
-215.464251823122));
#220063=CARTESIAN_POINT('Ctrl Pts',(10.5841068948558,-75.1338313689484,
-215.464697060592));
#220064=CARTESIAN_POINT('Ctrl Pts',(10.5569192142964,-75.1337866551771,
-215.465187610195));
#220065=CARTESIAN_POINT('Ctrl Pts',(10.5297211268796,-75.1337403743035,
-215.465723501161));
#220066=CARTESIAN_POINT('Ctrl Pts',(10.5025230394628,-75.1336940934299,
-215.466259392128));
#220067=CARTESIAN_POINT('Ctrl Pts',(10.4739383472588,-75.1336437465829,
-215.466872305924));
#220068=CARTESIAN_POINT('Ctrl Pts',(10.448095954022,-75.1335968225131,-215.467467223928));
#220069=CARTESIAN_POINT('Ctrl Pts',(10.1462333405878,-75.1330487067788,
-215.474416406298));
#220070=CARTESIAN_POINT('Ctrl Pts',(9.84329653499747,-75.1323073858502,
-215.486945485866));
#220071=CARTESIAN_POINT('Ctrl Pts',(9.53971836891024,-75.1313633897806,
-215.505042608647));
#220072=CARTESIAN_POINT('Ctrl Pts',(9.2333624588946,-75.1304107561355,-215.523305320322));
#220073=CARTESIAN_POINT('Ctrl Pts',(8.9263535402191,-75.1292517076195,-215.54723840805));
#220074=CARTESIAN_POINT('Ctrl Pts',(8.61913837793364,-75.1278781119617,
-215.576776604102));
#220075=CARTESIAN_POINT('Ctrl Pts',(8.49748869591185,-75.1273342017141,
-215.588473006488));
#220076=CARTESIAN_POINT('Ctrl Pts',(8.37580668504316,-75.1267566698495,
-215.601047692491));
#220077=CARTESIAN_POINT('Ctrl Pts',(8.25412008964395,-75.1261450871463,
-215.614494361863));
#220078=CARTESIAN_POINT('Ctrl Pts',(7.93597421378264,-75.1245461229043,
-215.649650267003));
#220079=CARTESIAN_POINT('Ctrl Pts',(7.6177819932054,-75.1227121680132,-215.690837597706));
#220080=CARTESIAN_POINT('Ctrl Pts',(7.30003766104192,-75.1206257462514,
-215.738083374911));
#220081=CARTESIAN_POINT('Ctrl Pts',(6.98229332887844,-75.1185393244897,
-215.785329152116));
#220082=CARTESIAN_POINT('Ctrl Pts',(6.66499706338629,-75.1162004058076,
-215.838633471389));
#220083=CARTESIAN_POINT('Ctrl Pts',(6.34863921534703,-75.1135939732195,
-215.897965001334));
#220084=CARTESIAN_POINT('Ctrl Pts',(6.19013846044381,-75.1122881054013,
-215.92769112428));
#220085=CARTESIAN_POINT('Ctrl Pts',(6.03187496724258,-75.110914607648,-215.95893405755));
#220086=CARTESIAN_POINT('Ctrl Pts',(5.87391202237455,-75.1094709993413,
-215.99169380274));
#220087=CARTESIAN_POINT('Ctrl Pts',(5.85986277650748,-75.1093426046216,
-215.994607458946));
#220088=CARTESIAN_POINT('Ctrl Pts',(5.84581590807222,-75.1092136552757,
-215.997533113053));
#220089=CARTESIAN_POINT('Ctrl Pts',(5.83177146177245,-75.1090841494548,
-216.000470765675));
#220090=CARTESIAN_POINT('Ctrl Pts',(5.76675282097511,-75.1084846033941,
-216.014070602686));
#220091=CARTESIAN_POINT('Ctrl Pts',(5.70178675789727,-75.1078733517838,
-216.027927095996));
#220092=CARTESIAN_POINT('Ctrl Pts',(5.63685944095259,-75.1072499409931,
-216.042044479373));
#220093=CARTESIAN_POINT('Ctrl Pts',(5.59736507119977,-75.1068707290152,
-216.050631884263));
#220094=CARTESIAN_POINT('Ctrl Pts',(5.55788503954139,-75.1064870172208,
-216.059315834801));
#220095=CARTESIAN_POINT('Ctrl Pts',(5.51841624616035,-75.1060986971487,
-216.068097395342));
#220096=CARTESIAN_POINT('Ctrl Pts',(5.50854826989078,-75.106001609477,-216.07029295856));
#220097=CARTESIAN_POINT('Ctrl Pts',(5.49868099617033,-75.1059042337217,
-216.072494623766));
#220098=CARTESIAN_POINT('Ctrl Pts',(5.48881437665547,-75.1058065681362,
-216.074702408412));
#220099=CARTESIAN_POINT('Ctrl Pts',(5.47935752456062,-75.1057129586689,
-216.07681850226));
#220100=CARTESIAN_POINT('Ctrl Pts',(5.47177960667182,-75.105305864689,-216.079013797392));
#220101=CARTESIAN_POINT('Ctrl Pts',(5.46042745654277,-75.1055279660516,
-216.081066924971));
#220102=CARTESIAN_POINT('Ctrl Pts',(33.2001189077142,-74.6413232806246,
-216.55743652807));
#220103=CARTESIAN_POINT('Ctrl Pts',(33.006978144415,-74.6583015829289,-216.5409993187));
#220104=CARTESIAN_POINT('Ctrl Pts',(32.8147762212939,-74.654089681431,-216.510956849065));
#220105=CARTESIAN_POINT('Ctrl Pts',(33.2543277379907,-75.1597676010536,
-215.769699247187));
#220106=CARTESIAN_POINT('Ctrl Pts',(33.1208674957723,-75.1687053141157,
-215.755692348251));
#220107=CARTESIAN_POINT('Ctrl Pts',(32.9875388545361,-75.1686237089069,
-215.738022261266));
#220108=CARTESIAN_POINT('Ctrl Pts',(33.3072722515331,-75.4457401389311,
-214.838681123811));
#220109=CARTESIAN_POINT('Ctrl Pts',(33.2414347818499,-75.4479382330087,
-214.830721324794));
#220110=CARTESIAN_POINT('Ctrl Pts',(33.1755313708028,-75.45012854121,-214.823325453787));
#220111=CARTESIAN_POINT('Ctrl Pts',(33.3513928282978,-75.4608560063641,
-213.894101968638));
#220112=CARTESIAN_POINT('Ctrl Pts',(33.3513928282978,-75.4608560063641,
-213.894101968638));
#220113=CARTESIAN_POINT('Ctrl Pts',(33.3513928282978,-75.4608560063641,
-213.894101968638));
#220114=CARTESIAN_POINT('',(33.2148661077881,-74.776924583375,-216.339144130369));
#220115=CARTESIAN_POINT('Origin',(33.132841491033,-72.1913959359691,-214.819830610287));
#220116=CARTESIAN_POINT('Origin',(33.2007176148554,-71.2835629216187,-214.037774394011));
#220117=CARTESIAN_POINT('Ctrl Pts',(33.1752262860966,-74.6372704537069,
-216.564961398279));
#220118=CARTESIAN_POINT('Ctrl Pts',(32.9990492150883,-74.6974990623407,
-216.482388336084));
#220119=CARTESIAN_POINT('Ctrl Pts',(32.8237598256931,-74.7342241033955,
-216.385388039321));
#220120=CARTESIAN_POINT('Ctrl Pts',(33.1949631872882,-74.6820694401112,
-216.496303691397));
#220121=CARTESIAN_POINT('Ctrl Pts',(33.0186275335319,-74.7272821064536,
-216.433478854616));
#220122=CARTESIAN_POINT('Ctrl Pts',(32.8430811295252,-74.7517232841479,
-216.358132577342));
#220123=CARTESIAN_POINT('Ctrl Pts',(33.2094670740371,-74.7292736488378,
-216.420526748278));
#220124=CARTESIAN_POINT('Ctrl Pts',(33.0332084422046,-74.7590740423288,
-216.380020841619));
#220125=CARTESIAN_POINT('Ctrl Pts',(32.8576392292869,-74.7701076430367,
-216.328432913941));
#220126=CARTESIAN_POINT('Ctrl Pts',(33.214866107803,-74.776924583857,-216.339144130663));
#220127=CARTESIAN_POINT('Ctrl Pts',(33.039029721468,-74.791820591591,-216.32328753345));
#220128=CARTESIAN_POINT('Ctrl Pts',(32.8638454862961,-74.788639230448,-216.296979356596));
#220129=CARTESIAN_POINT('',(33.1752262860962,-74.6372704537073,-216.564961398278));
#220130=CARTESIAN_POINT('',(32.8237598256931,-74.7342241033955,-216.385388039321));
#220131=CARTESIAN_POINT('Origin',(33.095784450501,-72.1361943004091,-214.910178309726));
#220132=CARTESIAN_POINT('Origin',(32.1378319467103,-74.4550490573172,-216.331724193165));
#220133=CARTESIAN_POINT('Origin',(31.688241471423,-74.6383695133239,-216.347659411481));
#220134=CARTESIAN_POINT('Ctrl Pts',(40.9503927122327,-75.196232348644,-213.885776709122));
#220135=CARTESIAN_POINT('Ctrl Pts',(40.9511754288092,-75.170618016806,-215.350418326104));
#220136=CARTESIAN_POINT('Ctrl Pts',(40.9214983009156,-74.3592730501824,
-216.569709261874));
#220137=CARTESIAN_POINT('Ctrl Pts',(38.3512480421664,-75.2960131239162,
-213.888896036206));
#220138=CARTESIAN_POINT('Ctrl Pts',(38.3524464105013,-75.2704427058848,
-215.35035620914));
#220139=CARTESIAN_POINT('Ctrl Pts',(38.3243446255555,-74.4622360886798,
-216.567950322327));
#220140=CARTESIAN_POINT('Ctrl Pts',(35.7515873189136,-75.386298205372,-213.891764703899));
#220141=CARTESIAN_POINT('Ctrl Pts',(35.7526446696784,-75.3607900951698,
-215.350336416166));
#220142=CARTESIAN_POINT('Ctrl Pts',(35.7265937516153,-74.5554064323997,
-216.566381833318));
#220143=CARTESIAN_POINT('Ctrl Pts',(33.1518661790638,-75.4670741746135,
-213.89429696046));
#220144=CARTESIAN_POINT('Ctrl Pts',(33.1525004164731,-75.4416278685769,
-215.350281850594));
#220145=CARTESIAN_POINT('Ctrl Pts',(33.1287433582894,-74.6387629869627,
-216.564935505388));
#220146=CARTESIAN_POINT('',(40.9214982998565,-74.3592730496089,-216.569709262804));
#220147=CARTESIAN_POINT('Origin',(-0.00331736233953883,957.648657693644,
-233.042565174374));
#220148=CARTESIAN_POINT('',(40.9503927122327,-75.1962323486441,-213.885776709122));
#220149=CARTESIAN_POINT('Origin',(40.758509388043,-70.2006777120066,-213.798514676938));
#220150=CARTESIAN_POINT('Origin',(-0.00137743448293204,990.512730862347,
-181.064274177303));
#220151=CARTESIAN_POINT('Ctrl Pts',(41.9926628230245,-75.1580153204876,
-213.752528187964));
#220152=CARTESIAN_POINT('Ctrl Pts',(42.3889675192146,-75.111938779609,-215.496580546143));
#220153=CARTESIAN_POINT('Ctrl Pts',(42.6506409244545,-73.9423397713714,
-216.824911934325));
#220154=CARTESIAN_POINT('Ctrl Pts',(41.9066793323699,-75.1610610934851,
-213.772054913982));
#220155=CARTESIAN_POINT('Ctrl Pts',(42.2773680112949,-75.116350496584,-215.497499167852));
#220156=CARTESIAN_POINT('Ctrl Pts',(42.5223146433776,-73.9743057102176,
-216.821387777151));
#220157=CARTESIAN_POINT('Ctrl Pts',(41.8205323433655,-75.1641318505835,
-213.789924116914));
#220158=CARTESIAN_POINT('Ctrl Pts',(42.1584887885637,-75.1211304958163,
-215.492781710638));
#220159=CARTESIAN_POINT('Ctrl Pts',(42.3813794284652,-74.0123061097281,
-216.810485774879));
#220160=CARTESIAN_POINT('Ctrl Pts',(41.6477999581399,-75.1703415381605,
-213.821539718001));
#220161=CARTESIAN_POINT('Ctrl Pts',(41.9257553840235,-75.1304773990168,
-215.482136500692));
#220162=CARTESIAN_POINT('Ctrl Pts',(42.1071714177053,-74.0810920561211,
-216.786773384908));
#220163=CARTESIAN_POINT('Ctrl Pts',(41.5612314342482,-75.1734777382289,
-213.835404439881));
#220164=CARTESIAN_POINT('Ctrl Pts',(41.8102296619885,-75.1351214208437,
-215.47561143684));
#220165=CARTESIAN_POINT('Ctrl Pts',(41.9710574680702,-74.1134796538391,
-216.773245626094));
#220166=CARTESIAN_POINT('Ctrl Pts',(41.3876518834424,-75.1798203744341,
-213.858883738274));
#220167=CARTESIAN_POINT('Ctrl Pts',(41.5763451014607,-75.1445888151757,
-215.456563678652));
#220168=CARTESIAN_POINT('Ctrl Pts',(41.6930958560081,-74.1786675398504,
-216.738185296849));
#220169=CARTESIAN_POINT('Ctrl Pts',(41.3006463902351,-75.1830256709096,
-213.868551556963));
#220170=CARTESIAN_POINT('Ctrl Pts',(41.457783462217,-75.1494218955781,-215.443955718151));
#220171=CARTESIAN_POINT('Ctrl Pts',(41.5508831144746,-74.211785746889,-216.716530930378));
#220172=CARTESIAN_POINT('Ctrl Pts',(41.1260290982083,-75.1895400074134,
-213.882061105842));
#220173=CARTESIAN_POINT('Ctrl Pts',(41.2077086857337,-75.1598056161679,
-215.404074252971));
#220174=CARTESIAN_POINT('Ctrl Pts',(41.2425985226721,-74.2859889767733,
-216.652644382816));
#220175=CARTESIAN_POINT('Ctrl Pts',(41.0384011165223,-75.1928537189715,
-213.885671097949));
#220176=CARTESIAN_POINT('Ctrl Pts',(41.0764186050639,-75.1653524051027,
-215.376453037444));
#220177=CARTESIAN_POINT('Ctrl Pts',(41.0767448130875,-74.3265280313286,
-216.609717214812));
#220178=CARTESIAN_POINT('Ctrl Pts',(40.9503927097337,-75.1962323487394,
-213.885776709126));
#220179=CARTESIAN_POINT('Ctrl Pts',(40.9511754272533,-75.1706180168537,
-215.350418326773));
#220180=CARTESIAN_POINT('Ctrl Pts',(40.9214983001298,-74.3592730495305,
-216.569709262898));
#220181=CARTESIAN_POINT('',(42.6506409244548,-73.9423397713703,-216.824911934326));
#220182=CARTESIAN_POINT('',(41.992662823025,-75.1580153204871,-213.752528187964));
#220183=CARTESIAN_POINT('Origin',(41.7958961124187,-70.1626506491805,-213.665266155779));
#220184=CARTESIAN_POINT('Ctrl Pts',(40.9503927122327,-75.1962323486435,
-213.885776709123));
#220185=CARTESIAN_POINT('Ctrl Pts',(41.0384742514642,-75.1928509113328,
-213.885671010119));
#220186=CARTESIAN_POINT('Ctrl Pts',(41.1260976159393,-75.1895374500536,
-213.882055874302));
#220187=CARTESIAN_POINT('Ctrl Pts',(41.2133377538246,-75.1862828366109,
-213.875306456167));
#220188=CARTESIAN_POINT('Ctrl Pts',(41.3007070197978,-75.183023405867,-213.868547047912));
#220189=CARTESIAN_POINT('Ctrl Pts',(41.3877081322076,-75.1798183151621,
-213.858876354802));
#220190=CARTESIAN_POINT('Ctrl Pts',(41.474441679009,-75.1766490529394,-213.847144238358));
#220191=CARTESIAN_POINT('Ctrl Pts',(41.5612776272786,-75.1734760489453,
-213.835398270459));
#220192=CARTESIAN_POINT('Ctrl Pts',(41.6478454293564,-75.1703399027889,
-213.821531434952));
#220193=CARTESIAN_POINT('Ctrl Pts',(41.7341661542895,-75.167236693896,-213.805731936783));
#220194=CARTESIAN_POINT('Ctrl Pts',(41.8205769752921,-75.1641302460715,
-213.789915948105));
#220195=CARTESIAN_POINT('Ctrl Pts',(41.9067233040927,-75.1610595358851,
-213.772044928068));
#220196=CARTESIAN_POINT('Ctrl Pts',(41.9926628230246,-75.1580153204876,
-213.752528187964));
#220197=CARTESIAN_POINT('Ctrl Pts',(42.6506409244545,-73.9423397713714,
-216.824911934325));
#220198=CARTESIAN_POINT('Ctrl Pts',(42.6307622877728,-73.9472915225057,
-216.824366012901));
#220199=CARTESIAN_POINT('Ctrl Pts',(42.6093064459885,-73.9527355471689,
-216.823572622786));
#220200=CARTESIAN_POINT('Ctrl Pts',(42.5862580487576,-73.9586516704412,
-216.822521533163));
#220201=CARTESIAN_POINT('Ctrl Pts',(42.5651297238504,-73.9640749444952,
-216.821558005729));
#220202=CARTESIAN_POINT('Ctrl Pts',(42.5426629131741,-73.9698950400132,
-216.820377807274));
#220203=CARTESIAN_POINT('Ctrl Pts',(42.5188810740907,-73.9760752302692,
-216.818985181213));
#220204=CARTESIAN_POINT('Ctrl Pts',(42.5012061616511,-73.9806684125396,
-216.817950166907));
#220205=CARTESIAN_POINT('Ctrl Pts',(42.4828055171911,-73.9854601121619,
-216.816798032545));
#220206=CARTESIAN_POINT('Ctrl Pts',(42.4637042950621,-73.9904260452816,
-216.815536054635));
#220207=CARTESIAN_POINT('Ctrl Pts',(42.4404178110658,-73.9964800622099,
-216.813997565203));
#220208=CARTESIAN_POINT('Ctrl Pts',(42.4160776169921,-74.0027995026238,
-216.812291477255));
#220209=CARTESIAN_POINT('Ctrl Pts',(42.3906990643268,-74.0093570496853,
-216.810412585741));
#220210=CARTESIAN_POINT('Ctrl Pts',(42.3763863042646,-74.0130553140792,
-216.809352945983));
#220211=CARTESIAN_POINT('Ctrl Pts',(42.3617439418181,-74.0168288938945,
-216.808238554472));
#220212=CARTESIAN_POINT('Ctrl Pts',(42.3467808471404,-74.0206690551345,
-216.807070477435));
#220213=CARTESIAN_POINT('Ctrl Pts',(42.3260334557344,-74.0259937108977,
-216.805450855826));
#220214=CARTESIAN_POINT('Ctrl Pts',(42.3046653349005,-74.0314489113354,
-216.803726144206));
#220215=CARTESIAN_POINT('Ctrl Pts',(42.282693951358,-74.0370140073013,-216.801893254208));
#220216=CARTESIAN_POINT('Ctrl Pts',(42.2717082595868,-74.0397965552843,
-216.80097680921));
#220217=CARTESIAN_POINT('Ctrl Pts',(42.2605717445896,-74.0426065375714,
-216.80003328781));
#220218=CARTESIAN_POINT('Ctrl Pts',(42.2492868609298,-74.0454417000548,
-216.799061210825));
#220219=CARTESIAN_POINT('Ctrl Pts',(42.2476466472937,-74.0458537798162,
-216.798919923243));
#220220=CARTESIAN_POINT('Ctrl Pts',(42.2459714240578,-74.0462743143251,
-216.79877538963));
#220221=CARTESIAN_POINT('Ctrl Pts',(42.2442753061012,-74.0466997068187,
-216.798628821829));
#220222=CARTESIAN_POINT('Ctrl Pts',(42.2343019113844,-74.0492010701416,
-216.797766984048));
#220223=CARTESIAN_POINT('Ctrl Pts',(42.2235917525255,-74.0518770861086,
-216.796829303334));
#220224=CARTESIAN_POINT('Ctrl Pts',(42.2149915568324,-74.0540196533554,
-216.796068609183));
#220225=CARTESIAN_POINT('Ctrl Pts',(42.1706803715226,-74.0650589014953,
-216.79214924959));
#220226=CARTESIAN_POINT('Ctrl Pts',(42.1275668081456,-74.0756321880183,
-216.788126946768));
#220227=CARTESIAN_POINT('Ctrl Pts',(42.0856601792248,-74.0857924220622,
-216.783988160757));
#220228=CARTESIAN_POINT('Ctrl Pts',(42.0514330282735,-74.0940907718287,
-216.780607815995));
#220229=CARTESIAN_POINT('Ctrl Pts',(42.0180116994635,-74.1021132445813,
-216.777150281193));
#220230=CARTESIAN_POINT('Ctrl Pts',(41.9854208969419,-74.1098785765232,
-216.773621645226));
#220231=CARTESIAN_POINT('Ctrl Pts',(41.9491739275612,-74.1185150545277,
-216.769697152734));
#220232=CARTESIAN_POINT('Ctrl Pts',(41.9139454439493,-74.1268379755528,
-216.765680926037));
#220233=CARTESIAN_POINT('Ctrl Pts',(41.8797446980124,-74.1348830668482,
-216.76157559263));
#220234=CARTESIAN_POINT('Ctrl Pts',(41.8636268779551,-74.1386744851431,
-216.759640868012));
#220235=CARTESIAN_POINT('Ctrl Pts',(41.8477367980506,-74.1424044857841,
-216.757686077121));
#220236=CARTESIAN_POINT('Ctrl Pts',(41.8320763341616,-74.1460759416482,
-216.755712418611));
#220237=CARTESIAN_POINT('Ctrl Pts',(41.8311216619832,-74.1462997560124,
-216.75559210309));
#220238=CARTESIAN_POINT('Ctrl Pts',(41.8301678262242,-74.1465233676039,
-216.755471711903));
#220239=CARTESIAN_POINT('Ctrl Pts',(41.8292148259921,-74.146746777301,-216.755351244198));
#220240=CARTESIAN_POINT('Ctrl Pts',(41.8209218072531,-74.1486908909979,
-216.754302932876));
#220241=CARTESIAN_POINT('Ctrl Pts',(41.8126931811236,-74.150619097667,-216.753249433925));
#220242=CARTESIAN_POINT('Ctrl Pts',(41.8045289047161,-74.1525319178485,
-216.752190218595));
#220243=CARTESIAN_POINT('Ctrl Pts',(41.7971876354883,-74.154251914482,-216.751237778412));
#220244=CARTESIAN_POINT('Ctrl Pts',(41.7908759595339,-74.155730666367,-216.750410022281));
#220245=CARTESIAN_POINT('Ctrl Pts',(41.7829568743593,-74.1575858560275,
-216.749357771845));
#220246=CARTESIAN_POINT('Ctrl Pts',(41.7820690900058,-74.157793835651,-216.749239807276));
#220247=CARTESIAN_POINT('Ctrl Pts',(41.7811610687575,-74.1580065539296,
-216.749118981173));
#220248=CARTESIAN_POINT('Ctrl Pts',(41.780229065532,-74.158224887783,-216.748994768089));
#220249=CARTESIAN_POINT('Ctrl Pts',(41.7432469728695,-74.166888423037,-216.74406596565));
#220250=CARTESIAN_POINT('Ctrl Pts',(41.7064247994052,-74.1755267166944,
-216.738833576768));
#220251=CARTESIAN_POINT('Ctrl Pts',(41.6698363362772,-74.1841324671723,
-216.733270467841));
#220252=CARTESIAN_POINT('Ctrl Pts',(41.6357861761109,-74.1921411988071,
-216.728093296301));
#220253=CARTESIAN_POINT('Ctrl Pts',(41.6019383182243,-74.2001218266649,
-216.722629698114));
#220254=CARTESIAN_POINT('Ctrl Pts',(41.5683888997643,-74.2080560005233,
-216.716887710817));
#220255=CARTESIAN_POINT('Ctrl Pts',(41.5658879250897,-74.208647461383,-216.716459668678));
#220256=CARTESIAN_POINT('Ctrl Pts',(41.5633886271414,-74.2092386577173,
-216.716030094091));
#220257=CARTESIAN_POINT('Ctrl Pts',(41.5608910547313,-74.209829578775,-216.715598997537));
#220258=CARTESIAN_POINT('Ctrl Pts',(41.5248897036665,-74.218347432497,-216.709384940102));
#220259=CARTESIAN_POINT('Ctrl Pts',(41.4892213917955,-74.2268154997241,
-216.702847269723));
#220260=CARTESIAN_POINT('Ctrl Pts',(41.4539047110238,-74.2352388213443,
-216.695991911182));
#220261=CARTESIAN_POINT('Ctrl Pts',(41.436246370638,-74.2394504821544,-216.692564231912));
#220262=CARTESIAN_POINT('Ctrl Pts',(41.4186759422659,-74.2436510576244,
-216.689057198583));
#220263=CARTESIAN_POINT('Ctrl Pts',(41.4011954472694,-74.2478417983752,
-216.685471738462));
#220264=CARTESIAN_POINT('Ctrl Pts',(41.3997093795187,-74.2481980654421,
-216.685166928062));
#220265=CARTESIAN_POINT('Ctrl Pts',(41.3982239689329,-74.248554247276,-216.684861570055));
#220266=CARTESIAN_POINT('Ctrl Pts',(41.3967391882741,-74.2489103603681,
-216.684555646867));
#220267=CARTESIAN_POINT('Ctrl Pts',(41.3894912914141,-74.2506487120545,
-216.683062295171));
#220268=CARTESIAN_POINT('Ctrl Pts',(41.3822589060392,-74.2523842115382,
-216.681553953867));
#220269=CARTESIAN_POINT('Ctrl Pts',(41.3750419560604,-74.2541173315647,
-216.680030625044));
#220270=CARTESIAN_POINT('Ctrl Pts',(41.3706942605806,-74.2551614122536,
-216.679112928531));
#220271=CARTESIAN_POINT('Ctrl Pts',(41.3663519670483,-74.2562081204571,
-216.678184906664));
#220272=CARTESIAN_POINT('Ctrl Pts',(41.3620153797659,-74.2572535870782,
-216.677252080092));
#220273=CARTESIAN_POINT('Ctrl Pts',(41.3597115677721,-74.2578089912207,
-216.676756515976));
#220274=CARTESIAN_POINT('Ctrl Pts',(41.357083273891,-74.2584426661523,-216.67618918604));
#220275=CARTESIAN_POINT('Ctrl Pts',(41.3546498070752,-74.2590293918546,
-216.675661945151));
#220276=CARTESIAN_POINT('Ctrl Pts',(41.3534710965864,-74.2593135871167,
-216.675406562845));
#220277=CARTESIAN_POINT('Ctrl Pts',(41.3523381619096,-74.2595867503155,
-216.675160651369));
#220278=CARTESIAN_POINT('Ctrl Pts',(41.3513103446013,-74.2598345701721,
-216.674937249552));
#220279=CARTESIAN_POINT('Ctrl Pts',(41.3507823355832,-74.2599618798779,
-216.674822483851));
#220280=CARTESIAN_POINT('Ctrl Pts',(41.3502820707845,-74.2600825005792,
-216.67471366168));
#220281=CARTESIAN_POINT('Ctrl Pts',(41.3498176099809,-74.260194488636,-216.674612565794));
#220282=CARTESIAN_POINT('Ctrl Pts',(41.3495507065253,-74.2602588428271,
-216.674554470813));
#220283=CARTESIAN_POINT('Ctrl Pts',(41.349295626601,-74.2603203462675,-216.6744989274));
#220284=CARTESIAN_POINT('Ctrl Pts',(41.3490539004976,-74.2603786299418,
-216.674446274729));
#220285=CARTESIAN_POINT('Ctrl Pts',(41.3488409954975,-74.2604299644295,
-216.674399899858));
#220286=CARTESIAN_POINT('Ctrl Pts',(41.3486297325562,-74.26048090302,-216.674353868862));
#220287=CARTESIAN_POINT('Ctrl Pts',(41.3484171089924,-74.260532169689,-216.674307527587));
#220288=CARTESIAN_POINT('Ctrl Pts',(41.332256670365,-74.2644286891677,-216.670785362304));
#220289=CARTESIAN_POINT('Ctrl Pts',(41.313866979032,-74.2688638131955,-216.666696381376));
#220290=CARTESIAN_POINT('Ctrl Pts',(41.2933719087617,-74.2737953734653,
-216.662018990123));
#220291=CARTESIAN_POINT('Ctrl Pts',(41.2715055234229,-74.2790569020066,
-216.657028636922));
#220292=CARTESIAN_POINT('Ctrl Pts',(41.2472462603474,-74.2848832608977,
-216.651368281838));
#220293=CARTESIAN_POINT('Ctrl Pts',(41.2207831869297,-74.2911945272362,
-216.645041682585));
#220294=CARTESIAN_POINT('Ctrl Pts',(41.2075516502209,-74.2943501604055,
-216.641878382958));
#220295=CARTESIAN_POINT('Ctrl Pts',(41.193769728485,-74.2976265312604,-216.638549076509));
#220296=CARTESIAN_POINT('Ctrl Pts',(41.1794634363018,-74.3010106466872,
-216.635057733616));
#220297=CARTESIAN_POINT('Ctrl Pts',(41.175886863256,-74.3018566755439,-216.634184897892));
#220298=CARTESIAN_POINT('Ctrl Pts',(41.1722775197716,-74.3027094288298,
-216.633301946298));
#220299=CARTESIAN_POINT('Ctrl Pts',(41.1686358540257,-74.303568675218,-216.632408973159));
#220300=CARTESIAN_POINT('Ctrl Pts',(41.1678188235789,-74.3037614525099,
-216.63220862906));
#220301=CARTESIAN_POINT('Ctrl Pts',(41.1670023237384,-74.3039540472148,
-216.632008309053));
#220302=CARTESIAN_POINT('Ctrl Pts',(41.166193024558,-74.3041448868624,-216.631809653647));
#220303=CARTESIAN_POINT('Ctrl Pts',(41.1561807058362,-74.3065058769922,
-216.629351970152));
#220304=CARTESIAN_POINT('Ctrl Pts',(41.146902295185,-74.3086873866522,-216.627062103609));
#220305=CARTESIAN_POINT('Ctrl Pts',(41.1349991103359,-74.3114709450446,
-216.624104235142));
#220306=CARTESIAN_POINT('Ctrl Pts',(41.1124558837132,-74.316742675968,-216.618502381518));
#220307=CARTESIAN_POINT('Ctrl Pts',(41.0914762557644,-74.3215964004882,
-216.61322223478));
#220308=CARTESIAN_POINT('Ctrl Pts',(41.0720298933579,-74.3260478784422,
-216.608296677193));
#220309=CARTESIAN_POINT('Ctrl Pts',(41.0490622752251,-74.3313054090608,
-216.602479222835));
#220310=CARTESIAN_POINT('Ctrl Pts',(41.0282329838513,-74.3360021895108,
-216.597156269549));
#220311=CARTESIAN_POINT('Ctrl Pts',(41.009435971611,-74.3401861457994,-216.59233766627));
#220312=CARTESIAN_POINT('Ctrl Pts',(40.9866694566912,-74.3452536587665,
-216.586501483263));
#220313=CARTESIAN_POINT('Ctrl Pts',(40.9668825400494,-74.3495699488692,
-216.581404474632));
#220314=CARTESIAN_POINT('Ctrl Pts',(40.9498286058995,-74.3532377994501,
-216.577010383348));
#220315=CARTESIAN_POINT('Ctrl Pts',(40.9393802972515,-74.355484954541,-216.574318287696));
#220316=CARTESIAN_POINT('Ctrl Pts',(40.9299569023606,-74.357488938127,-216.571889095025));
#220317=CARTESIAN_POINT('Ctrl Pts',(40.9214983001327,-74.359273049609,-216.56970926278));
#220318=CARTESIAN_POINT('Ctrl Pts',(42.378985830374,-74.0076928996301,-216.816073769133));
#220319=CARTESIAN_POINT('Ctrl Pts',(42.0789070994075,-75.1309710808869,
-215.501557062395));
#220320=CARTESIAN_POINT('Ctrl Pts',(41.6783348544084,-75.1653401212506,
-213.793428390226));
#220321=CARTESIAN_POINT('Ctrl Pts',(42.695627452923,-73.9307974382047,-216.831927633052));
#220322=CARTESIAN_POINT('Ctrl Pts',(42.436365014004,-75.113727280111,-215.499981515909));
#220323=CARTESIAN_POINT('Ctrl Pts',(42.0353813628522,-75.1619567754401,
-213.74615836671));
#220324=CARTESIAN_POINT('Ctrl Pts',(42.9815174465389,-73.8601470375395,
-216.832053666316));
#220325=CARTESIAN_POINT('Ctrl Pts',(42.7754409185831,-75.0814850954717,
-215.487452688235));
#220326=CARTESIAN_POINT('Ctrl Pts',(42.390949946975,-75.141795992121,-213.701832784708));
#220327=CARTESIAN_POINT('Ctrl Pts',(43.472508493266,-73.7123523458651,-216.83864882647));
#220328=CARTESIAN_POINT('Ctrl Pts',(43.3576044403188,-74.9997256985912,
-215.473802374509));
#220329=CARTESIAN_POINT('Ctrl Pts',(42.9950456425551,-75.0789259129395,
-213.631395393593));
#220330=CARTESIAN_POINT('Ctrl Pts',(43.6784848417686,-73.6416002218129,
-216.843674394851));
#220331=CARTESIAN_POINT('Ctrl Pts',(43.6010750190848,-74.9575939227159,
-215.470830714392));
#220332=CARTESIAN_POINT('Ctrl Pts',(43.2442829554274,-75.0445859118627,
-213.603599246343));
#220333=CARTESIAN_POINT('Ctrl Pts',(44.0840990697417,-73.4894561004303,
-216.851382274181));
#220334=CARTESIAN_POINT('Ctrl Pts',(44.0850213450697,-74.8573500503074,
-215.464209987895));
#220335=CARTESIAN_POINT('Ctrl Pts',(43.7407999450918,-74.95923489871,-213.549700262593));
#220336=CARTESIAN_POINT('Ctrl Pts',(44.2823423460514,-73.4093259654149,
-216.853445535287));
#220337=CARTESIAN_POINT('Ctrl Pts',(44.3244805372772,-74.7994341803878,
-215.459998179187));
#220338=CARTESIAN_POINT('Ctrl Pts',(43.9880896419911,-74.9082283395985,
-213.523624316504));
#220339=CARTESIAN_POINT('Ctrl Pts',(44.6663395277273,-73.2455758099323,
-216.853514051937));
#220340=CARTESIAN_POINT('Ctrl Pts',(44.7957647856255,-74.6691872475075,
-215.448954698364));
#220341=CARTESIAN_POINT('Ctrl Pts',(44.4808857844433,-74.7891870797359,
-213.473791302964));
#220342=CARTESIAN_POINT('Ctrl Pts',(44.8545941767413,-73.160040525945,-216.852689496172));
#220343=CARTESIAN_POINT('Ctrl Pts',(45.0293409228867,-74.5964823667737,
-215.443148236746));
#220344=CARTESIAN_POINT('Ctrl Pts',(44.7267891898549,-74.721020944827,-213.450088190065));
#220345=CARTESIAN_POINT('Ctrl Pts',(45.1403300017806,-73.0164913703724,
-216.854408324069));
#220346=CARTESIAN_POINT('Ctrl Pts',(45.3818326897387,-74.4739715465294,
-215.437873869065));
#220347=CARTESIAN_POINT('Ctrl Pts',(45.0928291473828,-74.6060271525094,
-213.416036405783));
#220348=CARTESIAN_POINT('Ctrl Pts',(45.2374002351368,-72.9646875296883,
-216.856056355454));
#220349=CARTESIAN_POINT('Ctrl Pts',(45.5006825021446,-74.4305046217021,
-215.437245699608));
#220350=CARTESIAN_POINT('Ctrl Pts',(45.214226071449,-74.5656241151966,-213.404928397068));
#220351=CARTESIAN_POINT('Ctrl Pts',(45.4284787286636,-72.8598153097967,
-216.858166103866));
#220352=CARTESIAN_POINT('Ctrl Pts',(45.7360618860342,-74.3398903326153,
-215.435132674419));
#220353=CARTESIAN_POINT('Ctrl Pts',(45.4557176198574,-74.4806914809447,
-213.382939645023));
#220354=CARTESIAN_POINT('Ctrl Pts',(45.5194683717665,-72.8099576191881,
-216.85739628503));
#220355=CARTESIAN_POINT('Ctrl Pts',(45.8503038319864,-74.2936199432179,
-215.432466908975));
#220356=CARTESIAN_POINT('Ctrl Pts',(45.5757446359314,-74.4361813329111,
-213.372122623236));
#220357=CARTESIAN_POINT('Ctrl Pts',(45.7858192096191,-72.661331939478,-216.853747605829));
#220358=CARTESIAN_POINT('Ctrl Pts',(46.1875371987659,-74.1507296656985,
-215.423451267174));
#220359=CARTESIAN_POINT('Ctrl Pts',(45.9328087573252,-74.2968675255568,
-213.340776903284));
#220360=CARTESIAN_POINT('Ctrl Pts',(45.9533357768491,-72.5652157418087,
-216.849067911601));
#220361=CARTESIAN_POINT('Ctrl Pts',(46.4038103241023,-74.0507287717429,
-215.415634323609));
#220362=CARTESIAN_POINT('Ctrl Pts',(46.1672258662471,-74.1961452862636,
-213.321432015392));
#220363=CARTESIAN_POINT('Ctrl Pts',(46.2126944376478,-72.3997852941367,
-216.847762456798));
#220364=CARTESIAN_POINT('Ctrl Pts',(46.7326853185615,-73.8858310589856,
-215.40996726368));
#220365=CARTESIAN_POINT('Ctrl Pts',(46.5133864112302,-74.0333951638931,
-213.294382252724));
#220366=CARTESIAN_POINT('Ctrl Pts',(46.3017762942777,-72.3394642981084,
-216.848685723507));
#220367=CARTESIAN_POINT('Ctrl Pts',(46.8441430626577,-73.827734396332,-215.409501019432));
#220368=CARTESIAN_POINT('Ctrl Pts',(46.6278478339237,-73.9772067981799,
-213.285618874283));
#220369=CARTESIAN_POINT('Ctrl Pts',(46.4779428408734,-72.2168840934957,
-216.849684972937));
#220370=CARTESIAN_POINT('Ctrl Pts',(47.0649879674724,-73.7078522436265,
-215.407953880452));
#220371=CARTESIAN_POINT('Ctrl Pts',(46.854860842577,-73.860987309113,-213.268274976754));
#220372=CARTESIAN_POINT('Ctrl Pts',(46.563987673213,-72.1558719051303,-216.84929201614));
#220373=CARTESIAN_POINT('Ctrl Pts',(47.1735256569728,-73.6464646449198,
-215.406402005381));
#220374=CARTESIAN_POINT('Ctrl Pts',(46.9674078998239,-73.8009605735783,
-213.259666405972));
#220375=CARTESIAN_POINT('Ctrl Pts',(46.6792210572178,-72.0788709964896,
-216.844067134084));
#220376=CARTESIAN_POINT('Ctrl Pts',(47.3251236075319,-73.5574882456331,
-215.399499935695));
#220377=CARTESIAN_POINT('Ctrl Pts',(47.1348908421815,-73.7079618268763,
-213.247450860241));
#220378=CARTESIAN_POINT('Ctrl Pts',(46.7161187190905,-72.054648443314,-216.841899297837));
#220379=CARTESIAN_POINT('Ctrl Pts',(47.3744063047614,-73.5280295183312,
-215.39678689924));
#220380=CARTESIAN_POINT('Ctrl Pts',(47.1904997834325,-73.6764658823414,
-213.243519901449));
#220381=CARTESIAN_POINT('Ctrl Pts',(46.7914227504076,-72.0034439643619,
-216.838436648525));
#220382=CARTESIAN_POINT('Ctrl Pts',(47.4739959337873,-73.4674961130268,
-215.392271721982));
#220383=CARTESIAN_POINT('Ctrl Pts',(47.3012779793222,-73.6124762223558,
-213.23594003108));
#220384=CARTESIAN_POINT('Ctrl Pts',(46.8291605334885,-71.9772975723057,
-216.836877529182));
#220385=CARTESIAN_POINT('Ctrl Pts',(47.5237795851717,-73.4367153932032,
-215.390203908609));
#220386=CARTESIAN_POINT('Ctrl Pts',(47.3564465383167,-73.5799829806061,
-213.232287185903));
#220387=CARTESIAN_POINT('Ctrl Pts',(47.0047959981998,-71.8539654157978,
-216.829930772006));
#220388=CARTESIAN_POINT('Ctrl Pts',(47.7552986345005,-73.2910829611759,
-215.380974273969));
#220389=CARTESIAN_POINT('Ctrl Pts',(47.6127233872645,-73.4260937179139,
-213.215858918559));
#220390=CARTESIAN_POINT('Ctrl Pts',(47.1416754793996,-71.7530639275421,
-216.825332946412));
#220391=CARTESIAN_POINT('Ctrl Pts',(47.9349954979552,-73.1707886047709,
-215.374842476235));
#220392=CARTESIAN_POINT('Ctrl Pts',(47.8110561400091,-73.2984848189965,
-213.204657242929));
#220393=CARTESIAN_POINT('Ctrl Pts',(47.2645314954405,-71.6680428481242,
-216.815412755198));
#220394=CARTESIAN_POINT('Ctrl Pts',(48.1016743030229,-73.0519933533766,
-215.363909661586));
#220395=CARTESIAN_POINT('Ctrl Pts',(48.0063773132287,-73.1639317249219,
-213.195676583529));
#220396=CARTESIAN_POINT('',(47.0905557676078,-71.7934728593479,-216.824560386716));
#220397=CARTESIAN_POINT('',(47.738383176916,-73.3429891884109,-213.20923907124));
#220398=CARTESIAN_POINT('Origin',(45.0170666017296,-69.1493247484068,-213.121977039054));
#220399=CARTESIAN_POINT('Ctrl Pts',(41.9926628230251,-75.158015320487,-213.752528187964));
#220400=CARTESIAN_POINT('Ctrl Pts',(42.2254656098299,-75.1493651193979,
-213.722768055243));
#220401=CARTESIAN_POINT('Ctrl Pts',(42.4681215167616,-75.1331685973929,
-213.693142558933));
#220402=CARTESIAN_POINT('Ctrl Pts',(42.7199965340293,-75.1075199128603,
-213.663651669654));
#220403=CARTESIAN_POINT('Ctrl Pts',(42.7283364387217,-75.1066706520372,
-213.662675188507));
#220404=CARTESIAN_POINT('Ctrl Pts',(42.7366864637874,-75.105811021856,-213.661698964705));
#220405=CARTESIAN_POINT('Ctrl Pts',(42.7450465875749,-75.1049409518136,
-213.660723025752));
#220406=CARTESIAN_POINT('Ctrl Pts',(42.8629292927521,-75.092672448034,-213.646961707528));
#220407=CARTESIAN_POINT('Ctrl Pts',(42.9828102619913,-75.0783292984929,
-213.633222439322));
#220408=CARTESIAN_POINT('Ctrl Pts',(43.1046068311246,-75.061707483384,-213.619516336771));
#220409=CARTESIAN_POINT('Ctrl Pts',(43.1698239612476,-75.0528071745612,
-213.61217727394));
#220410=CARTESIAN_POINT('Ctrl Pts',(43.2355897416449,-75.0432535660333,
-213.60484662163));
#220411=CARTESIAN_POINT('Ctrl Pts',(43.3018892782285,-75.0330153825397,
-213.597524382064));
#220412=CARTESIAN_POINT('Ctrl Pts',(43.3350390465203,-75.0278962907928,
-213.593863262281));
#220413=CARTESIAN_POINT('Ctrl Pts',(43.3683222534951,-75.0226060529535,
-213.590204245643));
#220414=CARTESIAN_POINT('Ctrl Pts',(43.4017369013796,-75.0171407709502,
-213.586547333187));
#220415=CARTESIAN_POINT('Ctrl Pts',(43.4257091389091,-75.0132198845532,
-213.583923801904));
#220416=CARTESIAN_POINT('Ctrl Pts',(43.4506713130679,-75.0090536411257,
-213.581201064996));
#220417=CARTESIAN_POINT('Ctrl Pts',(43.4746375299073,-75.0049733307183,
-213.578595150767));
#220418=CARTESIAN_POINT('Ctrl Pts',(43.4806793653705,-75.003944692603,-213.577938204988));
#220419=CARTESIAN_POINT('Ctrl Pts',(43.4866579344334,-75.0029217746917,
-213.577288656496));
#220420=CARTESIAN_POINT('Ctrl Pts',(43.492541479833,-75.0019103973164,-213.576649914173));
#220421=CARTESIAN_POINT('Ctrl Pts',(43.4958506536986,-75.001341552623,-213.576290656402));
#220422=CARTESIAN_POINT('Ctrl Pts',(43.4991297695187,-75.0007763630848,
-213.575934821562));
#220423=CARTESIAN_POINT('Ctrl Pts',(43.5023731804519,-75.0002158902631,
-213.575583015162));
#220424=CARTESIAN_POINT('Ctrl Pts',(43.6789624549774,-74.9697006422707,
-213.556428724122));
#220425=CARTESIAN_POINT('Ctrl Pts',(43.8536594409741,-74.9352051779825,
-213.537945346085));
#220426=CARTESIAN_POINT('Ctrl Pts',(44.0262846068755,-74.8969298990303,
-213.5201354507));
#220427=CARTESIAN_POINT('Ctrl Pts',(44.0960369712285,-74.8814640705733,
-213.512939035824));
#220428=CARTESIAN_POINT('Ctrl Pts',(44.1654511141014,-74.8653816412826,
-213.505852312176));
#220429=CARTESIAN_POINT('Ctrl Pts',(44.2345154218962,-74.8486979706476,
-213.498874379054));
#220430=CARTESIAN_POINT('Ctrl Pts',(44.2414195724209,-74.8470301544189,
-213.498176816127));
#220431=CARTESIAN_POINT('Ctrl Pts',(44.2483205387897,-74.8453562275326,
-213.497480382308));
#220432=CARTESIAN_POINT('Ctrl Pts',(44.2552182767284,-74.8436762135253,
-213.496785065357));
#220433=CARTESIAN_POINT('Ctrl Pts',(44.3785490214338,-74.8136377602704,
-213.484352879892));
#220434=CARTESIAN_POINT('Ctrl Pts',(44.5007688078792,-74.7816740241074,
-213.472271040558));
#220435=CARTESIAN_POINT('Ctrl Pts',(44.6218268047523,-74.7478698888918,
-213.460539666428));
#220436=CARTESIAN_POINT('Ctrl Pts',(44.6823558031889,-74.730967821284,-213.454673979364));
#220437=CARTESIAN_POINT('Ctrl Pts',(44.7425943156762,-74.7136054349217,
-213.448895904716));
#220438=CARTESIAN_POINT('Ctrl Pts',(44.8025361239107,-74.6957920070001,
-213.443205432122));
#220439=CARTESIAN_POINT('Ctrl Pts',(44.832507028028,-74.6868852930393,-213.440360195825));
#220440=CARTESIAN_POINT('Ctrl Pts',(44.862403752144,-74.6778658069359,-213.437536859826));
#220441=CARTESIAN_POINT('Ctrl Pts',(44.8922255056854,-74.6687346377144,
-213.434735421505));
#220442=CARTESIAN_POINT('Ctrl Pts',(44.9071363824561,-74.6641690531036,
-213.433334702345));
#220443=CARTESIAN_POINT('Ctrl Pts',(44.9220285163037,-74.659575547045,-213.431939457592));
#220444=CARTESIAN_POINT('Ctrl Pts',(44.9369018081516,-74.6549542512991,
-213.430549686832));
#220445=CARTESIAN_POINT('Ctrl Pts',(44.9443384540756,-74.6526436034261,
-213.429854801452));
#220446=CARTESIAN_POINT('Ctrl Pts',(44.951770389481,-74.6503260080913,-213.42916128457));
#220447=CARTESIAN_POINT('Ctrl Pts',(44.9591976019665,-74.648001481498,-213.428469136128));
#220448=CARTESIAN_POINT('Ctrl Pts',(44.9632239542959,-74.6467413367153,
-213.428093916826));
#220449=CARTESIAN_POINT('Ctrl Pts',(44.9669164143748,-74.6455834371407,
-213.42775004086));
#220450=CARTESIAN_POINT('Ctrl Pts',(44.9708158520873,-74.6443584060741,
-213.427387164341));
#220451=CARTESIAN_POINT('Ctrl Pts',(44.9741095137599,-74.6433236830783,
-213.427080660539));
#220452=CARTESIAN_POINT('Ctrl Pts',(44.9775507366128,-74.6422410785831,
-213.426760598811));
#220453=CARTESIAN_POINT('Ctrl Pts',(44.9814650631701,-74.6410071371356,
-213.426396801056));
#220454=CARTESIAN_POINT('Ctrl Pts',(45.1029661757967,-74.6027054633773,
-213.415104480054));
#220455=CARTESIAN_POINT('Ctrl Pts',(45.2207505984801,-74.5633287619067,
-213.404380114071));
#220456=CARTESIAN_POINT('Ctrl Pts',(45.3349856468011,-74.5231510781069,
-213.394033506047));
#220457=CARTESIAN_POINT('Ctrl Pts',(45.4338636380008,-74.4883746349437,
-213.385077832353));
#220458=CARTESIAN_POINT('Ctrl Pts',(45.5300341549536,-74.4530118326486,
-213.376452280864));
#220459=CARTESIAN_POINT('Ctrl Pts',(45.6234911871441,-74.4172713854539,
-213.368201767278));
#220460=CARTESIAN_POINT('Ctrl Pts',(45.647438567939,-74.4081132720548,-213.366087660015));
#220461=CARTESIAN_POINT('Ctrl Pts',(45.6712079590872,-74.3989302024541,
-213.363998049609));
#220462=CARTESIAN_POINT('Ctrl Pts',(45.6947996061161,-74.3897253635627,
-213.361933438076));
#220463=CARTESIAN_POINT('Ctrl Pts',(45.7122545962654,-74.3829148864485,
-213.36040587309));
#220464=CARTESIAN_POINT('Ctrl Pts',(45.7296144252457,-74.3760917616531,
-213.358892409563));
#220465=CARTESIAN_POINT('Ctrl Pts',(45.7468800576082,-74.3692569240176,
-213.35739252679));
#220466=CARTESIAN_POINT('Ctrl Pts',(45.8653228670678,-74.3223697116205,
-213.347103281331));
#220467=CARTESIAN_POINT('Ctrl Pts',(45.9792491168717,-74.2749665555787,
-213.337419776965));
#220468=CARTESIAN_POINT('Ctrl Pts',(46.0887466065047,-74.227432345403,-213.328341976054));
#220469=CARTESIAN_POINT('Ctrl Pts',(46.1434953513212,-74.2036652403152,
-213.323803075599));
#220470=CARTESIAN_POINT('Ctrl Pts',(46.1971371799208,-74.1798649863958,
-213.319415602941));
#220471=CARTESIAN_POINT('Ctrl Pts',(46.2496845193491,-74.1560772358378,
-213.315179562423));
#220472=CARTESIAN_POINT('Ctrl Pts',(46.2759581890632,-74.1441833605588,
-213.313061542164));
#220473=CARTESIAN_POINT('Ctrl Pts',(46.3019582288627,-74.1322925940271,
-213.310981379613));
#220474=CARTESIAN_POINT('Ctrl Pts',(46.3276862909874,-74.1204104680073,
-213.308939076144));
#220475=CARTESIAN_POINT('Ctrl Pts',(46.3405503220498,-74.1144694049973,
-213.307917924409));
#220476=CARTESIAN_POINT('Ctrl Pts',(46.3533463581902,-74.1085305009325,
-213.306906237422));
#220477=CARTESIAN_POINT('Ctrl Pts',(46.3660746062855,-74.1025944385409,
-213.305904015303));
#220478=CARTESIAN_POINT('Ctrl Pts',(46.3724387303331,-74.0996264073452,
-213.305402904244));
#220479=CARTESIAN_POINT('Ctrl Pts',(46.3787859073362,-74.0966590864933,
-213.3049041594));
#220480=CARTESIAN_POINT('Ctrl Pts',(46.3851161634271,-74.0936925606538,
-213.304407780787));
#220481=CARTESIAN_POINT('Ctrl Pts',(46.3882812914726,-74.0922092977341,
-213.304159591481));
#220482=CARTESIAN_POINT('Ctrl Pts',(46.3914421892879,-74.0907262335627,
-213.303911993733));
#220483=CARTESIAN_POINT('Ctrl Pts',(46.3945988601571,-74.0892433786806,
-213.303664987544));
#220484=CARTESIAN_POINT('Ctrl Pts',(46.3958585478266,-74.0886516369096,
-213.303566418304));
#220485=CARTESIAN_POINT('Ctrl Pts',(46.3969087996539,-74.0881580320819,
-213.303484260743));
#220486=CARTESIAN_POINT('Ctrl Pts',(46.3979995769197,-74.0876451955363,
-213.303398971659));
#220487=CARTESIAN_POINT('Ctrl Pts',(46.3996421953226,-74.0868729070281,
-213.303270533503));
#220488=CARTESIAN_POINT('Ctrl Pts',(46.401376773792,-74.0860571311396,-213.303134964987));
#220489=CARTESIAN_POINT('Ctrl Pts',(46.4040561947953,-74.0847954504982,
-213.30292574716));
#220490=CARTESIAN_POINT('Ctrl Pts',(46.5066049547341,-74.0365074864015,
-213.294918409471));
#220491=CARTESIAN_POINT('Ctrl Pts',(46.6048557467194,-73.9883693144774,
-213.28738335352));
#220492=CARTESIAN_POINT('Ctrl Pts',(46.6989248687914,-73.9407068034154,
-213.280190704557));
#220493=CARTESIAN_POINT('Ctrl Pts',(46.7131637398907,-73.9334923175529,
-213.27910198172));
#220494=CARTESIAN_POINT('Ctrl Pts',(46.7273067980788,-73.9262886830176,
-213.278021188919));
#220495=CARTESIAN_POINT('Ctrl Pts',(46.7413544421108,-73.9190969799375,
-213.276947964261));
#220496=CARTESIAN_POINT('Ctrl Pts',(46.8219064532499,-73.877858310642,-213.270793878609));
#220497=CARTESIAN_POINT('Ctrl Pts',(46.8993200983177,-73.8370145004555,
-213.264878976843));
#220498=CARTESIAN_POINT('Ctrl Pts',(46.9736981082125,-73.7967395376575,
-213.259314339676));
#220499=CARTESIAN_POINT('Ctrl Pts',(47.0095207926616,-73.7773419054064,
-213.256634243213));
#220500=CARTESIAN_POINT('Ctrl Pts',(47.0446390884701,-73.7580761615461,
-213.254034615544));
#220501=CARTESIAN_POINT('Ctrl Pts',(47.0790632952255,-73.7389613310804,
-213.25152381406));
#220502=CARTESIAN_POINT('Ctrl Pts',(47.1365946196497,-73.7070157434696,
-213.247327646642));
#220503=CARTESIAN_POINT('Ctrl Pts',(47.1921917917575,-73.6754884956987,
-213.243405092136));
#220504=CARTESIAN_POINT('Ctrl Pts',(47.2458889523972,-73.6444709939159,
-213.239730824515));
#220505=CARTESIAN_POINT('Ctrl Pts',(47.3032098578872,-73.6113602806669,
-213.235808599493));
#220506=CARTESIAN_POINT('Ctrl Pts',(47.3583648958864,-73.5788310316487,
-213.232164844058));
#220507=CARTESIAN_POINT('Ctrl Pts',(47.4113921142577,-73.546989220601,-213.228765490142));
#220508=CARTESIAN_POINT('Ctrl Pts',(47.5006757254644,-73.4933761523499,
-213.223041890023));
#220509=CARTESIAN_POINT('Ctrl Pts',(47.5839277861292,-73.4417153369978,
-213.218003707915));
#220510=CARTESIAN_POINT('Ctrl Pts',(47.6613227244206,-73.3924652818581,
-213.213567309774));
#220511=CARTESIAN_POINT('Ctrl Pts',(47.6876873451025,-73.3756882283325,
-213.212056048744));
#220512=CARTESIAN_POINT('Ctrl Pts',(47.7133720810526,-73.3591905530428,
-213.210614503331));
#220513=CARTESIAN_POINT('Ctrl Pts',(47.7383831769159,-73.3429891884108,
-213.20923907124));
#220514=CARTESIAN_POINT('Ctrl Pts',(47.0905557676078,-71.7934728593479,
-216.824560386716));
#220515=CARTESIAN_POINT('Ctrl Pts',(47.0153154861726,-71.8474340839192,
-216.828160153995));
#220516=CARTESIAN_POINT('Ctrl Pts',(46.9368040133168,-71.9030117484293,
-216.831773097603));
#220517=CARTESIAN_POINT('Ctrl Pts',(46.8105116370282,-71.9908582593833,
-216.837212277512));
#220518=CARTESIAN_POINT('Ctrl Pts',(46.7669927040833,-72.020887478965,-216.839028631564));
#220519=CARTESIAN_POINT('Ctrl Pts',(46.6991242326024,-72.0673122522426,
-216.841758103766));
#220520=CARTESIAN_POINT('Ctrl Pts',(46.6760717227842,-72.0830169115032,
-216.842668751354));
#220521=CARTESIAN_POINT('Ctrl Pts',(46.6407809462547,-72.106953442936,-216.844035958017));
#220522=CARTESIAN_POINT('Ctrl Pts',(46.6199834046119,-72.121027909888,-216.844833855528));
#220523=CARTESIAN_POINT('Ctrl Pts',(46.5987769248733,-72.1353112488642,
-216.845632383546));
#220524=CARTESIAN_POINT('Ctrl Pts',(46.5865515833884,-72.1435268361654,
-216.846088839681));
#220525=CARTESIAN_POINT('Ctrl Pts',(46.5819665060498,-72.1466049757675,
-216.846259389817));
#220526=CARTESIAN_POINT('Ctrl Pts',(46.555537766819,-72.1643384243489,-216.847240570889));
#220527=CARTESIAN_POINT('Ctrl Pts',(46.5231938316714,-72.1867724289952,
-216.847819543089));
#220528=CARTESIAN_POINT('Ctrl Pts',(46.4606822267319,-72.2303448318372,
-216.848171262885));
#220529=CARTESIAN_POINT('Ctrl Pts',(46.4374915718699,-72.246531469105,-216.848202379732));
#220530=CARTESIAN_POINT('Ctrl Pts',(46.3856103030984,-72.2825820153409,
-216.848092367259));
#220531=CARTESIAN_POINT('Ctrl Pts',(46.3558503353891,-72.3031801798479,
-216.847943622513));
#220532=CARTESIAN_POINT('Ctrl Pts',(46.2631145147534,-72.3667848726466,
-216.847284711573));
#220533=CARTESIAN_POINT('Ctrl Pts',(46.208151407488,-72.4033115039303,-216.847007932495));
#220534=CARTESIAN_POINT('Ctrl Pts',(46.1416458441078,-72.4467401169996,
-216.846836506201));
#220535=CARTESIAN_POINT('Ctrl Pts',(46.1221295340369,-72.4593269700902,
-216.846819987823));
#220536=CARTESIAN_POINT('Ctrl Pts',(46.0974082219484,-72.4751244180359,
-216.846856145838));
#220537=CARTESIAN_POINT('Ctrl Pts',(46.0861848140159,-72.4822527182994,
-216.84688945874));
#220538=CARTESIAN_POINT('Ctrl Pts',(46.0751835275252,-72.4891763075989,
-216.846954983109));
#220539=CARTESIAN_POINT('Ctrl Pts',(46.0709255770755,-72.4918415808474,
-216.846988777692));
#220540=CARTESIAN_POINT('Ctrl Pts',(46.0681893543815,-72.4935509553511,
-216.847012576906));
#220541=CARTESIAN_POINT('Ctrl Pts',(46.0680823775556,-72.4936192985686,
-216.847012518365));
#220542=CARTESIAN_POINT('Ctrl Pts',(45.986400536202,-72.544427560482,-216.847862664063));
#220543=CARTESIAN_POINT('Ctrl Pts',(45.8584635249158,-72.6215820396233,
-216.849534490042));
#220544=CARTESIAN_POINT('Ctrl Pts',(45.6967296702545,-72.714040109495,-216.852246641916));
#220545=CARTESIAN_POINT('Ctrl Pts',(45.6042304529531,-72.7654497464509,
-216.853958836125));
#220546=CARTESIAN_POINT('Ctrl Pts',(45.5586484610098,-72.7903262952877,
-216.85485107458));
#220547=CARTESIAN_POINT('Ctrl Pts',(45.5341488619496,-72.8035792364326,
-216.855342803594));
#220548=CARTESIAN_POINT('Ctrl Pts',(45.5294717188307,-72.8061050271169,
-216.855437120383));
#220549=CARTESIAN_POINT('Ctrl Pts',(45.5046882376694,-72.8194776935945,
-216.855938034955));
#220550=CARTESIAN_POINT('Ctrl Pts',(45.470715692922,-72.8383454154814,-216.856101554138));
#220551=CARTESIAN_POINT('Ctrl Pts',(45.4028375426769,-72.8758731489928,
-216.855884938175));
#220552=CARTESIAN_POINT('Ctrl Pts',(45.3773872318471,-72.8899169068841,
-216.855735750397));
#220553=CARTESIAN_POINT('Ctrl Pts',(45.3348444051485,-72.9132059925027,
-216.855396495046));
#220554=CARTESIAN_POINT('Ctrl Pts',(45.3124812465956,-72.9254056289433,
-216.855197998949));
#220555=CARTESIAN_POINT('Ctrl Pts',(45.2884584929797,-72.9384146386768,
-216.854956200221));
#220556=CARTESIAN_POINT('Ctrl Pts',(45.2720721122027,-72.9472642953749,
-216.854785378261));
#220557=CARTESIAN_POINT('Ctrl Pts',(45.2647205457611,-72.951225960519,-216.85470655318));
#220558=CARTESIAN_POINT('Ctrl Pts',(45.1783811276406,-72.9976001084211,
-216.853748673381));
#220559=CARTESIAN_POINT('Ctrl Pts',(45.1162386053219,-73.0296995672728,
-216.853096086082));
#220560=CARTESIAN_POINT('Ctrl Pts',(45.0467315615012,-73.0651255515261,
-216.852415497251));
#220561=CARTESIAN_POINT('Ctrl Pts',(45.0274969846771,-73.074811491286,-216.85223834966));
#220562=CARTESIAN_POINT('Ctrl Pts',(45.0046549590261,-73.0862425626378,
-216.852047201304));
#220563=CARTESIAN_POINT('Ctrl Pts',(44.9947354495031,-73.0911831765483,
-216.851970270382));
#220564=CARTESIAN_POINT('Ctrl Pts',(44.985805048694,-73.0956046027232,-216.851913143341));
#220565=CARTESIAN_POINT('Ctrl Pts',(44.9825450402972,-73.0972128634217,
-216.851895651545));
#220566=CARTESIAN_POINT('Ctrl Pts',(44.9804978794133,-73.0982214477538,
-216.851885543953));
#220567=CARTESIAN_POINT('Ctrl Pts',(44.9815296466787,-73.0977154089663,
-216.851889037914));
#220568=CARTESIAN_POINT('Ctrl Pts',(44.7937050256253,-73.1899692383285,
-216.851156413369));
#220569=CARTESIAN_POINT('Ctrl Pts',(44.6038221421328,-73.276007932375,-216.850981194006));
#220570=CARTESIAN_POINT('Ctrl Pts',(44.3891332656768,-73.3655067295875,
-216.851398473015));
#220571=CARTESIAN_POINT('Ctrl Pts',(44.3652648622609,-73.3753494207078,
-216.851453370693));
#220572=CARTESIAN_POINT('Ctrl Pts',(44.3354181459926,-73.3875229791999,
-216.851532659472));
#220573=CARTESIAN_POINT('Ctrl Pts',(44.3303128275422,-73.3895972284648,
-216.851547718566));
#220574=CARTESIAN_POINT('Ctrl Pts',(44.3241159589436,-73.3921189971362,
-216.851559824846));
#220575=CARTESIAN_POINT('Ctrl Pts',(44.3145787175221,-73.3960037439674,
-216.851569925362));
#220576=CARTESIAN_POINT('Ctrl Pts',(44.2769462497412,-73.4113612035586,
-216.851518312626));
#220577=CARTESIAN_POINT('Ctrl Pts',(44.2346656261212,-73.428647567988,-216.851202761778));
#220578=CARTESIAN_POINT('Ctrl Pts',(44.1176065965149,-73.4759833562347,
-216.849929669799));
#220579=CARTESIAN_POINT('Ctrl Pts',(44.0188557871459,-73.5153738373685,
-216.848393248556));
#220580=CARTESIAN_POINT('Ctrl Pts',(43.8384285616185,-73.5832970739191,
-216.845057076804));
#220581=CARTESIAN_POINT('Ctrl Pts',(43.7728881056669,-73.6074012984833,
-216.843773096239));
#220582=CARTESIAN_POINT('Ctrl Pts',(43.6928204059483,-73.6358421539148,
-216.842135204374));
#220583=CARTESIAN_POINT('Ctrl Pts',(43.6838358636326,-73.6390206080686,
-216.841950530088));
#220584=CARTESIAN_POINT('Ctrl Pts',(43.6656893389447,-73.6454130775643,
-216.841575808911));
#220585=CARTESIAN_POINT('Ctrl Pts',(43.6613867719329,-73.6469205732218,
-216.841486892913));
#220586=CARTESIAN_POINT('Ctrl Pts',(43.6432709423947,-73.6532597550245,
-216.841114816226));
#220587=CARTESIAN_POINT('Ctrl Pts',(43.6069988100621,-73.6658712095105,
-216.840375657652));
#220588=CARTESIAN_POINT('Ctrl Pts',(43.5706001821117,-73.6782836949642,
-216.839651483473));
#220589=CARTESIAN_POINT('Ctrl Pts',(43.4489677593928,-73.7192243136924,
-216.837270868198));
#220590=CARTESIAN_POINT('Ctrl Pts',(43.3505740698763,-73.7506204343719,
-216.835472931678));
#220591=CARTESIAN_POINT('Ctrl Pts',(43.052725368472,-73.8406182541426,-216.830398789216));
#220592=CARTESIAN_POINT('Ctrl Pts',(42.850988648335,-73.8949175961045,-216.827442250372));
#220593=CARTESIAN_POINT('Ctrl Pts',(42.6506409244548,-73.9423397713703,
-216.824911934326));
#220594=CARTESIAN_POINT('Ctrl Pts',(48.7454044931546,-72.6086641314349,
-213.184229057458));
#220595=CARTESIAN_POINT('Ctrl Pts',(48.7033558856732,-72.5944415704724,
-215.339600005589));
#220596=CARTESIAN_POINT('Ctrl Pts',(47.6826029798323,-71.3710801272352,
-216.791855002172));
#220597=CARTESIAN_POINT('Ctrl Pts',(48.4201758660447,-72.8745352082672,
-213.18165597563));
#220598=CARTESIAN_POINT('Ctrl Pts',(48.4312469413185,-72.8157272237703,
-215.339098369127));
#220599=CARTESIAN_POINT('Ctrl Pts',(47.4907935026806,-71.5238447201971,
-216.792044585111));
#220600=CARTESIAN_POINT('Ctrl Pts',(48.0843074405258,-73.1189108367609,
-213.190215709195));
#220601=CARTESIAN_POINT('Ctrl Pts',(48.1524733410718,-73.0220158932171,
-215.351128153903));
#220602=CARTESIAN_POINT('Ctrl Pts',(47.2933342139034,-71.6644126162231,
-216.803168697192));
#220603=CARTESIAN_POINT('Ctrl Pts',(47.7383831769152,-73.3429891884114,
-213.20923907124));
#220604=CARTESIAN_POINT('Ctrl Pts',(47.8674267413582,-73.2141877251378,
-215.374920075632));
#220605=CARTESIAN_POINT('Ctrl Pts',(47.0905557676078,-71.7934728593478,
-216.824560386716));
#220606=CARTESIAN_POINT('',(47.6826029798323,-71.3710801272351,-216.791855002172));
#220607=CARTESIAN_POINT('',(48.7454044931547,-72.6086641314348,-213.184229057458));
#220608=CARTESIAN_POINT('Origin',(45.5817163713881,-68.7378163165586,-213.096967025272));
#220609=CARTESIAN_POINT('Origin',(42.8925236218019,-65.4916988456017,-217.549100737884));
#220610=CARTESIAN_POINT('Ctrl Pts',(47.6826029798323,-71.3710801272352,
-216.791855002172));
#220611=CARTESIAN_POINT('Ctrl Pts',(47.5930241849003,-71.4424241948411,
-216.791943540537));
#220612=CARTESIAN_POINT('Ctrl Pts',(47.501770357419,-71.5114565096234,-216.794420184531));
#220613=CARTESIAN_POINT('Ctrl Pts',(47.4089903151591,-71.5780732065795,
-216.799270679234));
#220614=CARTESIAN_POINT('Ctrl Pts',(47.315016754119,-71.6455468580804,-216.804183570508));
#220615=CARTESIAN_POINT('Ctrl Pts',(47.2194774794399,-71.7105423809681,
-216.81153173483));
#220616=CARTESIAN_POINT('Ctrl Pts',(47.1225445112692,-71.7729893080334,
-216.821266633682));
#220617=CARTESIAN_POINT('Ctrl Pts',(47.1118983115526,-71.7798478874183,
-216.822335822828));
#220618=CARTESIAN_POINT('Ctrl Pts',(47.1012353169086,-71.7866757600782,
-216.823433769923));
#220619=CARTESIAN_POINT('Ctrl Pts',(47.0905557676078,-71.7934728593478,
-216.824560386716));
#220620=CARTESIAN_POINT('Ctrl Pts',(47.6826029798322,-71.3710801272353,
-216.791855002172));
#220621=CARTESIAN_POINT('Ctrl Pts',(48.7033558856732,-72.5944415704724,
-215.339600005589));
#220622=CARTESIAN_POINT('Ctrl Pts',(48.7454044931547,-72.6086641314348,
-213.184229057458));
#220623=CARTESIAN_POINT('Ctrl Pts',(48.7278636855945,-70.5385934818759,
-216.790821882089));
#220624=CARTESIAN_POINT('Ctrl Pts',(49.761732857596,-71.7299417527765,-215.340395531872));
#220625=CARTESIAN_POINT('Ctrl Pts',(49.8084038141043,-71.7395463911349,
-213.198257848046));
#220626=CARTESIAN_POINT('Ctrl Pts',(49.7727562910368,-69.6608348552492,
-216.790293600173));
#220627=CARTESIAN_POINT('Ctrl Pts',(50.8130965389874,-70.8232845236527,
-215.341943634334));
#220628=CARTESIAN_POINT('Ctrl Pts',(50.8549407258148,-70.835967150169,-213.213888016011));
#220629=CARTESIAN_POINT('Ctrl Pts',(50.7746555306532,-68.7687177611616,
-216.79041881877));
#220630=CARTESIAN_POINT('Ctrl Pts',(51.8269633350129,-69.9002951910831,
-215.34395680141));
#220631=CARTESIAN_POINT('Ctrl Pts',(51.8687937432179,-69.9121576054873,
-213.227785479717));
#220632=CARTESIAN_POINT('Origin',(46.9399934642734,-69.2345705942718,-216.824055271245));
#220633=CARTESIAN_POINT('Ctrl Pts',(48.7454044931547,-72.6086641314348,
-213.184229057458));
#220634=CARTESIAN_POINT('Ctrl Pts',(49.0966483416997,-72.3214805470352,
-213.189018754026));
#220635=CARTESIAN_POINT('Ctrl Pts',(49.445331300399,-72.0311663472331,-213.193869847133));
#220636=CARTESIAN_POINT('Ctrl Pts',(49.7914306652966,-71.7378094434948,
-213.198721048627));
#220637=CARTESIAN_POINT('Ctrl Pts',(50.1399413000144,-71.4424087259844,
-213.20360604838));
#220638=CARTESIAN_POINT('Ctrl Pts',(50.4858333869782,-71.1439217890174,
-213.208491419808));
#220639=CARTESIAN_POINT('Ctrl Pts',(50.8290574947046,-70.8423935581624,
-213.213315112328));
#220640=CARTESIAN_POINT('Ctrl Pts',(51.172281602431,-70.5408653273073,-213.218138804848));
#220641=CARTESIAN_POINT('Ctrl Pts',(51.5128390059467,-70.2362947052039,
-213.222901065645));
#220642=CARTESIAN_POINT('Ctrl Pts',(51.8506357777519,-69.9286975574418,
-213.227536544435));
#220643=CARTESIAN_POINT('Origin',(-7.03224757818595E-6,47.3239895493301,
-196.659261305123));
#220644=CARTESIAN_POINT('',(0.0473571427401393,53.3225154460666,-213.879539002147));
#220645=CARTESIAN_POINT('Origin',(0.46976145343121,53.0041184688829,-208.56971754274));
#220646=CARTESIAN_POINT('',(0.0544835933803345,52.4792219709059,-216.57221503382));
#220647=CARTESIAN_POINT('Origin',(0.0463362411570871,48.3232770745245,-213.79227696996));
#220648=CARTESIAN_POINT('Origin',(0.0318052213360498,52.469100728301,-216.511513110739));
#220649=CARTESIAN_POINT('Ctrl Pts',(0.0473571427401181,53.3225154460666,
-213.879539002147));
#220650=CARTESIAN_POINT('Ctrl Pts',(0.0513181061457815,53.2968418492561,
-215.350332007314));
#220651=CARTESIAN_POINT('Ctrl Pts',(0.0544853477938667,52.4787689033323,
-216.572892235108));
#220652=CARTESIAN_POINT('Ctrl Pts',(1.50078629177953,53.3222855571144,-213.875705279281));
#220653=CARTESIAN_POINT('Ctrl Pts',(1.62614544992748,53.2965621608307,-215.346507035678));
#220654=CARTESIAN_POINT('Ctrl Pts',(1.72636223391502,52.4781147405702,-216.56897010493));
#220655=CARTESIAN_POINT('Ctrl Pts',(2.92702243085717,53.3114912412646,-213.695947807356));
#220656=CARTESIAN_POINT('Ctrl Pts',(3.17360837162122,53.2833921337829,-215.166683249136));
#220657=CARTESIAN_POINT('Ctrl Pts',(3.36628637758863,52.4472954145725,-216.38513789576));
#220658=CARTESIAN_POINT('Ctrl Pts',(4.37281940663811,53.2905575229658,-213.348880503444));
#220659=CARTESIAN_POINT('Ctrl Pts',(4.73714801109632,53.2579878078057,-214.82094618417));
#220660=CARTESIAN_POINT('Ctrl Pts',(5.02417785496923,52.3884400051989,-216.030189424361));
#220661=CARTESIAN_POINT('Ctrl Pts',(4.4166077184939,53.289913868413,-213.338209943704));
#220662=CARTESIAN_POINT('Ctrl Pts',(4.78457700700934,53.2572054630635,-214.810300111701));
#220663=CARTESIAN_POINT('Ctrl Pts',(5.07438936223524,52.38663030623,-216.019276413929));
#220664=CARTESIAN_POINT('Ctrl Pts',(4.47131352346949,53.2890977177666,-213.324680435774));
#220665=CARTESIAN_POINT('Ctrl Pts',(4.84383217904547,53.2562134344238,-214.796802126739));
#220666=CARTESIAN_POINT('Ctrl Pts',(5.13712105476995,52.3843352406963,-216.005439190793));
#220667=CARTESIAN_POINT('Ctrl Pts',(4.48225430767143,53.2889337622212,-213.321972140265));
#220668=CARTESIAN_POINT('Ctrl Pts',(4.8530836264365,53.2560652079218,-214.794050223811));
#220669=CARTESIAN_POINT('Ctrl Pts',(5.14497267313242,52.3846620371662,-216.002795752475));
#220670=CARTESIAN_POINT('Ctrl Pts',(4.50414007083002,53.2886037420393,-213.316582951083));
#220671=CARTESIAN_POINT('Ctrl Pts',(4.87325651228538,53.2557343778721,-214.788605124326));
#220672=CARTESIAN_POINT('Ctrl Pts',(5.16368704978722,52.384808931647,-215.997453930094));
#220673=CARTESIAN_POINT('Ctrl Pts',(4.51508431353993,53.2884377751688,-213.313897267951));
#220674=CARTESIAN_POINT('Ctrl Pts',(4.88334426763236,53.2555681292117,-214.785891301654));
#220675=CARTESIAN_POINT('Ctrl Pts',(5.17304536586829,52.3848811302304,-215.994791426239));
#220676=CARTESIAN_POINT('Ctrl Pts',(4.54792112758205,53.2879370021236,-213.30586696962));
#220677=CARTESIAN_POINT('Ctrl Pts',(4.91361107625039,53.2550668868734,-214.777776140093));
#220678=CARTESIAN_POINT('Ctrl Pts',(5.20112370349652,52.3850939761974,-215.986829153085));
#220679=CARTESIAN_POINT('Ctrl Pts',(4.56981778483334,53.2875993235168,-213.300549105442));
#220680=CARTESIAN_POINT('Ctrl Pts',(4.93379446859988,53.2547293838989,-214.77240089122));
#220681=CARTESIAN_POINT('Ctrl Pts',(5.21984711401021,52.3852308738026,-215.981554622283));
#220682=CARTESIAN_POINT('Ctrl Pts',(4.67932834463653,53.2858917529309,-213.274138348232));
#220683=CARTESIAN_POINT('Ctrl Pts',(5.03472988581075,53.2530252892833,-214.745701624089));
#220684=CARTESIAN_POINT('Ctrl Pts',(5.31348684546282,52.3858903127237,-215.955350443654));
#220685=CARTESIAN_POINT('Ctrl Pts',(4.76702406700707,53.2844643286532,-213.253581139957));
#220686=CARTESIAN_POINT('Ctrl Pts',(5.11556895614656,53.2516084370936,-214.724900005178));
#220687=CARTESIAN_POINT('Ctrl Pts',(5.38847118038393,52.3863377057957,-215.934926221979));
#220688=CARTESIAN_POINT('Ctrl Pts',(5.03037439102468,53.2799968687426,-213.193632432861));
#220689=CARTESIAN_POINT('Ctrl Pts',(5.35831561743065,53.247196875607,-214.664189566484));
#220690=CARTESIAN_POINT('Ctrl Pts',(5.61364510061675,52.3874374899134,-215.875279476601));
#220691=CARTESIAN_POINT('Ctrl Pts',(5.20629213894649,53.2767716505112,-213.155963782957));
#220692=CARTESIAN_POINT('Ctrl Pts',(5.52050447418381,53.2440403454911,-214.625960795307));
#220693=CARTESIAN_POINT('Ctrl Pts',(5.76405550081911,52.3878474698,-215.837682829783));
#220694=CARTESIAN_POINT('Ctrl Pts',(5.7351090490271,53.2663464299268,-213.049921731156));
#220695=CARTESIAN_POINT('Ctrl Pts',(6.00800931507342,53.2339186236173,-214.518122615114));
#220696=CARTESIAN_POINT('Ctrl Pts',(6.21619890377965,52.3880929077652,-215.731466854287));
#220697=CARTESIAN_POINT('Ctrl Pts',(6.08932836962055,53.2583903798102,-212.988474563998));
#220698=CARTESIAN_POINT('Ctrl Pts',(6.33470802101544,53.2262917188763,-214.455267165325));
#220699=CARTESIAN_POINT('Ctrl Pts',(6.51906256367254,52.3869415830987,-215.669383233572));
#220700=CARTESIAN_POINT('Ctrl Pts',(7.15467547994453,53.2314932970166,-212.832839779496));
#220701=CARTESIAN_POINT('Ctrl Pts',(7.31721137313374,53.2007743525897,-214.294930171996));
#220702=CARTESIAN_POINT('Ctrl Pts',(7.4301490293476,52.3794528536415,-215.510259917988));
#220703=CARTESIAN_POINT('Ctrl Pts',(7.86408306340235,53.2096427750673,-212.767811172676));
#220704=CARTESIAN_POINT('Ctrl Pts',(7.9719989895612,53.1803473395072,-214.22594561548));
#220705=CARTESIAN_POINT('Ctrl Pts',(8.03673212095718,52.3691912963031,-215.440813554609));
#220706=CARTESIAN_POINT('Ctrl Pts',(9.98981135051243,53.1323666949439,-212.690409355922));
#220707=CARTESIAN_POINT('Ctrl Pts',(9.93185501850042,53.1089544676763,-214.134581778742));
#220708=CARTESIAN_POINT('Ctrl Pts',(9.85169968539593,52.3227594953376,-215.343739708831));
#220709=CARTESIAN_POINT('Ctrl Pts',(11.4039030907724,53.0652276040225,-212.794256396978));
#220710=CARTESIAN_POINT('Ctrl Pts',(11.2367879874246,53.0477230606374,-214.22619279686));
#220711=CARTESIAN_POINT('Ctrl Pts',(11.0567236931827,52.271013981524,-215.426125580955));
#220712=CARTESIAN_POINT('Ctrl Pts',(13.1664443333411,52.9616798229974,-213.138287858329));
#220713=CARTESIAN_POINT('Ctrl Pts',(12.8547213220072,52.9546856753362,-214.549698418581));
#220714=CARTESIAN_POINT('Ctrl Pts',(12.54724214411,52.1791590921482,-215.730009700032));
#220715=CARTESIAN_POINT('Ctrl Pts',(13.5182905195363,52.9400113359771,-213.217839110357));
#220716=CARTESIAN_POINT('Ctrl Pts',(13.1775056939578,52.9352623790446,-214.624917702853));
#220717=CARTESIAN_POINT('Ctrl Pts',(12.8442482944742,52.1594335681189,-215.800867210821));
#220718=CARTESIAN_POINT('Ctrl Pts',(13.8914034372555,52.9159732378538,-213.314153161469));
#220719=CARTESIAN_POINT('Ctrl Pts',(13.519416343042,52.91377595379,-214.716322291134));
#220720=CARTESIAN_POINT('Ctrl Pts',(13.1586925435442,52.137008372533,-215.887205379916));
#220721=CARTESIAN_POINT('Ctrl Pts',(13.9133485948345,52.9145554991731,-213.319862053585));
#220722=CARTESIAN_POINT('Ctrl Pts',(13.5395282183867,52.9125087139671,-214.721742162107));
#220723=CARTESIAN_POINT('Ctrl Pts',(13.1771851227051,52.1356838534725,-215.892324735676));
#220724=CARTESIAN_POINT('Ctrl Pts',(13.9572335779744,52.9117125575511,-213.331366738556));
#220725=CARTESIAN_POINT('Ctrl Pts',(13.5797448109807,52.9099679570789,-214.732666696408));
#220726=CARTESIAN_POINT('Ctrl Pts',(13.2141620165421,52.1330240247262,-215.90264489138));
#220727=CARTESIAN_POINT('Ctrl Pts',(13.9791751707466,52.910287801062,-213.337130942172));
#220728=CARTESIAN_POINT('Ctrl Pts',(13.6053354404193,52.9083470662355,-214.739112678143));
#220729=CARTESIAN_POINT('Ctrl Pts',(13.2427576996845,52.1315237651408,-215.909751051737));
#220730=CARTESIAN_POINT('Ctrl Pts',(14.0450114907337,52.906007261992,-213.354204614102));
#220731=CARTESIAN_POINT('Ctrl Pts',(13.67719453886,52.9037874808928,-214.757359487488));
#220732=CARTESIAN_POINT('Ctrl Pts',(13.3194789666303,52.1271448577845,-215.929109421424));
#220733=CARTESIAN_POINT('Ctrl Pts',(14.0889121696723,52.9031437987804,-213.36539506595));
#220734=CARTESIAN_POINT('Ctrl Pts',(13.7251035033336,52.9007361441998,-214.769331200397));
#220735=CARTESIAN_POINT('Ctrl Pts',(13.3706237530771,52.1241944637679,-215.941816004742));
#220736=CARTESIAN_POINT('Ctrl Pts',(14.2206434120527,52.8945239974864,-213.398393774553));
#220737=CARTESIAN_POINT('Ctrl Pts',(13.8688369510683,52.8915473464146,-214.804670640288));
#220738=CARTESIAN_POINT('Ctrl Pts',(13.5240519748989,52.1152502744402,-215.979342795789));
#220739=CARTESIAN_POINT('Ctrl Pts',(14.3085031783526,52.8887382469479,-213.419629432868));
#220740=CARTESIAN_POINT('Ctrl Pts',(13.9646727465828,52.8853747963935,-214.827463939186));
#220741=CARTESIAN_POINT('Ctrl Pts',(13.6263292941939,52.1091634838073,-216.003570107382));
#220742=CARTESIAN_POINT('Ctrl Pts',(14.5721978639792,52.8712625751263,-213.481070862543));
#220743=CARTESIAN_POINT('Ctrl Pts',(14.252217261359,52.8667166406394,-214.893568804806));
#220744=CARTESIAN_POINT('Ctrl Pts',(13.9331521185388,52.0905335590214,-216.073910240701));
#220745=CARTESIAN_POINT('Ctrl Pts',(14.7481481313963,52.8594542225811,-213.519011772404));
#220746=CARTESIAN_POINT('Ctrl Pts',(14.4439820930866,52.8540893087314,-214.934610621538));
#220747=CARTESIAN_POINT('Ctrl Pts',(14.1376887958124,52.0776210286607,-216.117682146349));
#220748=CARTESIAN_POINT('Ctrl Pts',(15.6286519779478,52.799613377426,-213.693903709884));
#220749=CARTESIAN_POINT('Ctrl Pts',(15.4031772187442,52.7899993081263,-215.12497225672));
#220750=CARTESIAN_POINT('Ctrl Pts',(15.1604959234659,52.0106176596974,-216.321274261672));
#220751=CARTESIAN_POINT('Ctrl Pts',(16.3354684203193,52.7491845407321,-213.786320807185));
#220752=CARTESIAN_POINT('Ctrl Pts',(16.1726687571268,52.7356086885058,-215.229790369045));
#220753=CARTESIAN_POINT('Ctrl Pts',(15.9799531666696,51.9491102505506,-216.435321014709));
#220754=CARTESIAN_POINT('Ctrl Pts',(18.4626009435542,52.5898921039226,-213.93074044221));
#220755=CARTESIAN_POINT('Ctrl Pts',(18.4831256320861,52.5630943102473,-215.41083522379));
#220756=CARTESIAN_POINT('Ctrl Pts',(18.4346796935493,51.7426456517123,-216.639808829428));
#220757=CARTESIAN_POINT('Ctrl Pts',(19.889576854664,52.4730122776555,-213.850322288953));
#220758=CARTESIAN_POINT('Ctrl Pts',(20.0303223005475,52.4352353701873,-215.353938852772));
#220759=CARTESIAN_POINT('Ctrl Pts',(20.0708290034904,51.5750773518433,-216.593838971602));
#220760=CARTESIAN_POINT('Ctrl Pts',(21.6827252055215,52.3125514421363,-213.558099210805));
#220761=CARTESIAN_POINT('Ctrl Pts',(21.9611240710592,52.2595696821476,-215.091433587878));
#220762=CARTESIAN_POINT('Ctrl Pts',(22.10701332157,51.3339336809999,-216.337638892853));
#220763=CARTESIAN_POINT('Ctrl Pts',(22.0420804380365,52.2797161015951,-213.490009648216));
#220764=CARTESIAN_POINT('Ctrl Pts',(22.3484158142329,52.2235225648504,-215.02913808195));
#220765=CARTESIAN_POINT('Ctrl Pts',(22.5140828494934,51.2840959663516,-216.276412274292));
#220766=CARTESIAN_POINT('Ctrl Pts',(22.489685929986,52.237965427953,-213.393843363054));
#220767=CARTESIAN_POINT('Ctrl Pts',(22.830297685778,52.1776606940211,-214.940224931789));
#220768=CARTESIAN_POINT('Ctrl Pts',(23.0202154747916,51.2201134032129,-216.188409850374));
#220769=CARTESIAN_POINT('Ctrl Pts',(22.5791527085523,52.2295777954778,-213.374053497722));
#220770=CARTESIAN_POINT('Ctrl Pts',(22.9266518936637,52.1684397634174,-214.92187419643));
#220771=CARTESIAN_POINT('Ctrl Pts',(23.1213352805328,51.2072292399456,-216.170232433021));
#220772=CARTESIAN_POINT('Ctrl Pts',(22.6909190277613,52.2190463850868,-213.348628685159));
#220773=CARTESIAN_POINT('Ctrl Pts',(23.0469943568649,52.156860007596,-214.898249234479));
#220774=CARTESIAN_POINT('Ctrl Pts',(23.2476077584572,51.1910139587644,-216.146798480699));
#220775=CARTESIAN_POINT('Ctrl Pts',(22.7132689336663,52.2169377595729,-213.343509345961));
#220776=CARTESIAN_POINT('Ctrl Pts',(23.0710617306981,52.1545410005613,-214.893489132397));
#220777=CARTESIAN_POINT('Ctrl Pts',(23.2728558874527,51.1877653983752,-216.142076078541));
#220778=CARTESIAN_POINT('Ctrl Pts',(22.7467887689231,52.2137713063516,-213.335778919634));
#220779=CARTESIAN_POINT('Ctrl Pts',(23.1071557559864,52.1510584252376,-214.886297549121));
#220780=CARTESIAN_POINT('Ctrl Pts',(23.3107186471497,51.1828842897498,-216.134939216676));
#220781=CARTESIAN_POINT('Ctrl Pts',(22.7579612100689,52.2127152361209,-213.333193541222));
#220782=CARTESIAN_POINT('Ctrl Pts',(23.1191863165467,52.1498968514716,-214.883891703835));
#220783=CARTESIAN_POINT('Ctrl Pts',(23.3233379945114,51.1812558755664,-216.132551386277));
#220784=CARTESIAN_POINT('Ctrl Pts',(22.7803044200105,52.2106019240513,-213.328005669353));
#220785=CARTESIAN_POINT('Ctrl Pts',(23.1432453661066,52.147572322968,-214.879062842723));
#220786=CARTESIAN_POINT('Ctrl Pts',(23.3485735632596,51.1779962891938,-216.127757998687));
#220787=CARTESIAN_POINT('Ctrl Pts',(22.7914750239802,52.2095447316332,-213.325401286812));
#220788=CARTESIAN_POINT('Ctrl Pts',(23.1566284527116,52.1462704833645,-214.87692670199));
#220789=CARTESIAN_POINT('Ctrl Pts',(23.3635425140041,51.1754974311187,-216.125669225138));
#220790=CARTESIAN_POINT('Ctrl Pts',(22.8473256024037,52.2042553206975,-213.312356521225));
#220791=CARTESIAN_POINT('Ctrl Pts',(23.2084106565659,52.1413088528524,-214.863000994536));
#220792=CARTESIAN_POINT('Ctrl Pts',(23.4121150904848,51.1726824854318,-216.111643547468));
#220793=CARTESIAN_POINT('Ctrl Pts',(22.8920158443536,52.2000074805641,-213.302049206934));
#220794=CARTESIAN_POINT('Ctrl Pts',(23.2498473184699,52.1373250721395,-214.851985232895));
#220795=CARTESIAN_POINT('Ctrl Pts',(23.450976928624,51.1704115507272,-216.100543254307));
#220796=CARTESIAN_POINT('Ctrl Pts',(23.1155161868957,52.1786865508133,-213.251157958149));
#220797=CARTESIAN_POINT('Ctrl Pts',(23.4570203439368,52.117339881761,-214.797550367366));
#220798=CARTESIAN_POINT('Ctrl Pts',(23.6453045375155,51.1589619023911,-216.045645542894));
#220799=CARTESIAN_POINT('Ctrl Pts',(23.2944736580684,52.1613682854172,-213.212509671947));
#220800=CARTESIAN_POINT('Ctrl Pts',(23.6229334914969,52.1011197585585,-214.756006577968));
#220801=CARTESIAN_POINT('Ctrl Pts',(23.8008254618619,51.1494982987292,-216.003659147808));
#220802=CARTESIAN_POINT('Ctrl Pts',(24.1900632291311,52.0734578840137,-213.02978559012));
#220803=CARTESIAN_POINT('Ctrl Pts',(24.4523439445286,52.0189511941718,-214.558750653319));
#220804=CARTESIAN_POINT('Ctrl Pts',(24.5786925763469,51.1006544733309,-215.803557774365));
#220805=CARTESIAN_POINT('Ctrl Pts',(24.9090934498498,51.9989121398747,-212.917162893799));
#220806=CARTESIAN_POINT('Ctrl Pts',(25.1186944050463,51.9494811141712,-214.433449924263));
#220807=CARTESIAN_POINT('Ctrl Pts',(25.2018288175531,51.0567050281331,-215.674851310126));
#220808=CARTESIAN_POINT('Ctrl Pts',(26.3528137916526,51.8410386164222,-212.765468959133));
#220809=CARTESIAN_POINT('Ctrl Pts',(26.4549358636402,51.803024530226,-214.254620439179));
#220810=CARTESIAN_POINT('Ctrl Pts',(26.4489097601866,50.9587713152296,-215.485839368666));
#220811=CARTESIAN_POINT('Ctrl Pts',(27.0774998386423,51.757712611848,-212.726350374933));
#220812=CARTESIAN_POINT('Ctrl Pts',(27.1250938204043,51.7260245846545,-214.200855802869));
#220813=CARTESIAN_POINT('Ctrl Pts',(27.0728462116736,50.9047968613094,-215.425489070919));
#220814=CARTESIAN_POINT('Ctrl Pts',(28.1693846366643,51.6257897144361,-212.730030329923));
#220815=CARTESIAN_POINT('Ctrl Pts',(28.133153944658,51.6046668429049,-214.180734173614));
#220816=CARTESIAN_POINT('Ctrl Pts',(28.0085132019179,50.8158988470028,-215.392519511646));
#220817=CARTESIAN_POINT('Ctrl Pts',(28.5341580010441,51.5806587005877,-212.741678726248));
#220818=CARTESIAN_POINT('Ctrl Pts',(28.4694894459954,51.5632588178081,-214.184116855442));
#220819=CARTESIAN_POINT('Ctrl Pts',(28.320362539182,50.7849405015155,-215.391147109929));
#220820=CARTESIAN_POINT('Ctrl Pts',(29.2654690940375,51.4880085266914,-212.787471470535));
#220821=CARTESIAN_POINT('Ctrl Pts',(29.1429594857087,51.4784684902285,-214.212632134674));
#220822=CARTESIAN_POINT('Ctrl Pts',(28.9438185512427,50.7202631028992,-215.409064536584));
#220823=CARTESIAN_POINT('Ctrl Pts',(29.6331976033025,51.4403305324129,-212.821772692263));
#220824=CARTESIAN_POINT('Ctrl Pts',(29.4812293665496,51.4349376880746,-214.237876571198));
#220825=CARTESIAN_POINT('Ctrl Pts',(29.2564302637446,50.6864303950653,-215.42845818016));
#220826=CARTESIAN_POINT('Ctrl Pts',(31.462411304102,51.1976497020186,-213.05276291922));
#220827=CARTESIAN_POINT('Ctrl Pts',(31.1598855435033,51.2141722963552,-214.421574027106));
#220828=CARTESIAN_POINT('Ctrl Pts',(30.8062875514217,50.5113774631636,-215.58023710365));
#220829=CARTESIAN_POINT('Ctrl Pts',(32.8718379544085,50.9930622692497,-213.421070504589));
#220830=CARTESIAN_POINT('Ctrl Pts',(32.4486765378635,51.0294768386726,-214.747355725967));
#220831=CARTESIAN_POINT('Ctrl Pts',(31.9841321905945,50.3552367741408,-215.87179911295));
#220832=CARTESIAN_POINT('Ctrl Pts',(34.2185104850841,50.7818638678805,-214.004031647198));
#220833=CARTESIAN_POINT('Ctrl Pts',(33.6642034707759,50.8420733856997,-215.278241777324));
#220834=CARTESIAN_POINT('Ctrl Pts',(33.0835570625902,50.1833829144682,-216.356884220228));
#220835=CARTESIAN_POINT('',(5.13104565674618,52.3850329666526,-216.006074884366));
#220836=CARTESIAN_POINT('',(13.2064798588263,52.1340212825562,-215.899800104744));
#220837=CARTESIAN_POINT('Ctrl Pts',(5.13104565674618,52.3850329666526,-216.006074884366));
#220838=CARTESIAN_POINT('Ctrl Pts',(5.1522723863429,52.3849119363674,-216.000415561109));
#220839=CARTESIAN_POINT('Ctrl Pts',(5.18369007136552,52.3849388776591,-215.991787544618));
#220840=CARTESIAN_POINT('Ctrl Pts',(5.2221706225626,52.3853576829994,-215.98074183974));
#220841=CARTESIAN_POINT('Ctrl Pts',(5.23991278899162,52.3856572015947,-215.975516213414));
#220842=CARTESIAN_POINT('Ctrl Pts',(5.24999842259676,52.3858537036521,-215.972512762277));
#220843=CARTESIAN_POINT('Ctrl Pts',(5.25431824827715,52.3859432179003,-215.971219626002));
#220844=CARTESIAN_POINT('Ctrl Pts',(5.26070648918049,52.3860788494767,-215.96930321972));
#220845=CARTESIAN_POINT('Ctrl Pts',(5.27389209107745,52.3861808482352,-215.965609200379));
#220846=CARTESIAN_POINT('Ctrl Pts',(5.30493951670919,52.3863517352301,-215.957082350732));
#220847=CARTESIAN_POINT('Ctrl Pts',(5.32328062740663,52.3864424667375,-215.95207247075));
#220848=CARTESIAN_POINT('Ctrl Pts',(5.34961236428572,52.3865761864417,-215.944921314242));
#220849=CARTESIAN_POINT('Ctrl Pts',(5.36195508675722,52.3866420092958,-215.941576612198));
#220850=CARTESIAN_POINT('Ctrl Pts',(5.37041866445846,52.3866880806414,-215.939284606238));
#220851=CARTESIAN_POINT('Ctrl Pts',(5.3766407570771,52.3867228499403,-215.937600959149));
#220852=CARTESIAN_POINT('Ctrl Pts',(5.46224792408119,52.387209238623,-215.914445988889));
#220853=CARTESIAN_POINT('Ctrl Pts',(5.54481645278234,52.3875795430898,-215.892793204776));
#220854=CARTESIAN_POINT('Ctrl Pts',(5.79534687511541,52.3884036177798,-215.829175878375));
#220855=CARTESIAN_POINT('Ctrl Pts',(5.96055636587489,52.3885516848245,-215.789947269247));
#220856=CARTESIAN_POINT('Ctrl Pts',(6.2979554273082,52.3880338386774,-215.715495695431));
#220857=CARTESIAN_POINT('Ctrl Pts',(6.4666575859569,52.3873610716747,-215.681107141238));
#220858=CARTESIAN_POINT('Ctrl Pts',(6.80397794650947,52.3851945176741,-215.618004498281));
#220859=CARTESIAN_POINT('Ctrl Pts',(6.97119969975367,52.3837164893957,-215.589504826742));
#220860=CARTESIAN_POINT('Ctrl Pts',(7.48099337258852,52.3779565382077,-215.511231006924));
#220861=CARTESIAN_POINT('Ctrl Pts',(7.82010832743786,52.3724788185414,-215.470605457691));
#220862=CARTESIAN_POINT('Ctrl Pts',(8.32716511723021,52.3618554631322,-215.427002629812));
#220863=CARTESIAN_POINT('Ctrl Pts',(8.58029034720757,52.3559412520016,-215.409535089865));
#220864=CARTESIAN_POINT('Ctrl Pts',(8.8747949213488,52.347988683421,-215.396740572747));
#220865=CARTESIAN_POINT('Ctrl Pts',(9.00082715023796,52.3443544942176,-215.392882411015));
#220866=CARTESIAN_POINT('Ctrl Pts',(9.08480653626051,52.3418814354433,-215.390671459359));
#220867=CARTESIAN_POINT('Ctrl Pts',(9.12559907967593,52.3406558542846,-215.389767430667));
#220868=CARTESIAN_POINT('Ctrl Pts',(10.5486606647616,52.2969998804139,-215.364516209537));
#220869=CARTESIAN_POINT('Ctrl Pts',(11.9026484148537,52.2279542766091,-215.534782163801));
#220870=CARTESIAN_POINT('Ctrl Pts',(13.2064798588263,52.1340212825562,-215.899800104744));
#220871=CARTESIAN_POINT('Ctrl Pts',(0.0544835933803345,52.4792219709059,
-216.57221503382));
#220872=CARTESIAN_POINT('Ctrl Pts',(0.911160817479643,52.4788868661666,
-216.570205286074));
#220873=CARTESIAN_POINT('Ctrl Pts',(1.76241895715707,52.4706614931604,-216.520914925994));
#220874=CARTESIAN_POINT('Ctrl Pts',(3.03147279341818,52.4469055640949,-216.37863656052));
#220875=CARTESIAN_POINT('Ctrl Pts',(3.45317987983679,52.437124954073,-216.319765648019));
#220876=CARTESIAN_POINT('Ctrl Pts',(4.08382026129649,52.4196309296523,-216.214709957797));
#220877=CARTESIAN_POINT('Ctrl Pts',(4.29371035972386,52.4133485556671,-216.176866822026));
#220878=CARTESIAN_POINT('Ctrl Pts',(4.71285393159547,52.3998755739423,-216.095622991724));
#220879=CARTESIAN_POINT('Ctrl Pts',(4.92331707557612,52.3926407185815,-216.051954867598));
#220880=CARTESIAN_POINT('Ctrl Pts',(5.13104565674618,52.3850329666526,-216.006074884366));
#220881=CARTESIAN_POINT('',(33.8288256031492,50.8425198063061,-213.842075047864));
#220882=CARTESIAN_POINT('Ctrl Pts',(33.8288255478891,50.842519431512,-213.842075041244));
#220883=CARTESIAN_POINT('Ctrl Pts',(33.4284854188798,50.9043645576862,-213.682497552222));
#220884=CARTESIAN_POINT('Ctrl Pts',(33.0234151108197,50.9655031314903,-213.541601722254));
#220885=CARTESIAN_POINT('Ctrl Pts',(32.6138910800848,51.0258461372266,-213.418284882882));
#220886=CARTESIAN_POINT('Ctrl Pts',(32.331432047247,51.0674662272815,-213.333230154545));
#220887=CARTESIAN_POINT('Ctrl Pts',(32.0468531911046,51.1087080507273,-213.256538359194));
#220888=CARTESIAN_POINT('Ctrl Pts',(31.760231540292,51.1495445945205,-213.187851585035));
#220889=CARTESIAN_POINT('Ctrl Pts',(31.409874876356,51.1994618119026,-213.103891182943));
#220890=CARTESIAN_POINT('Ctrl Pts',(31.0565047178319,51.2487669147299,-213.031971634751));
#220891=CARTESIAN_POINT('Ctrl Pts',(30.7001071569706,51.2974289024419,-212.971577841718));
#220892=CARTESIAN_POINT('Ctrl Pts',(30.4677048343532,51.3291607665437,-212.932195816379));
#220893=CARTESIAN_POINT('Ctrl Pts',(30.2340152891889,51.3606190839795,-212.897715883105));
#220894=CARTESIAN_POINT('Ctrl Pts',(29.9990356615501,51.3917943388598,-212.868006986073));
#220895=CARTESIAN_POINT('Ctrl Pts',(29.8721559397073,51.4086277456846,-212.851965354593));
#220896=CARTESIAN_POINT('Ctrl Pts',(29.7450788398527,51.425353889665,-212.837366281459));
#220897=CARTESIAN_POINT('Ctrl Pts',(29.6179629924412,51.4419530974048,-212.824189892595));
#220898=CARTESIAN_POINT('Ctrl Pts',(29.3784059472776,51.4732352486014,-212.799358238269));
#220899=CARTESIAN_POINT('Ctrl Pts',(29.1386589563805,51.5040741022767,-212.779534675732));
#220900=CARTESIAN_POINT('Ctrl Pts',(28.8998133411101,51.5343335838555,-212.76457826505));
#220901=CARTESIAN_POINT('Ctrl Pts',(28.5341328392157,51.5806618465631,-212.7416795078));
#220902=CARTESIAN_POINT('Ctrl Pts',(28.1693740007316,51.6257909648341,-212.73003226545));
#220903=CARTESIAN_POINT('Ctrl Pts',(27.8054230251458,51.6697639760348,-212.728805896947));
#220904=CARTESIAN_POINT('Ctrl Pts',(27.2316173468697,51.7390918943822,-212.726872402443));
#220905=CARTESIAN_POINT('Ctrl Pts',(26.6598134037606,51.8055490660031,-212.750767890064));
#220906=CARTESIAN_POINT('Ctrl Pts',(26.0896436282477,51.8692665869875,-212.798150768092));
#220907=CARTESIAN_POINT('Ctrl Pts',(25.9366320432575,51.8863659130062,-212.810866505719));
#220908=CARTESIAN_POINT('Ctrl Pts',(25.7837381711085,51.9032678997162,-212.825274048008));
#220909=CARTESIAN_POINT('Ctrl Pts',(25.6309549566012,51.9199750044334,-212.8413287466));
#220910=CARTESIAN_POINT('Ctrl Pts',(25.5252626824047,51.9315326346253,-212.8524350557));
#220911=CARTESIAN_POINT('Ctrl Pts',(25.4196234520893,51.9429969636597,-212.864330645356));
#220912=CARTESIAN_POINT('Ctrl Pts',(25.3140353742927,51.9543686087815,-212.877005898441));
#220913=CARTESIAN_POINT('Ctrl Pts',(24.6986753884516,52.0206417669555,-212.950876393313));
#220914=CARTESIAN_POINT('Ctrl Pts',(24.085246551812,52.0837464971781,-213.05117739929));
#220915=CARTESIAN_POINT('Ctrl Pts',(23.4735918363912,52.1437861556349,-213.17596614546));
#220916=CARTESIAN_POINT('Ctrl Pts',(23.3778558249152,52.1531835448581,-213.195498042353));
#220917=CARTESIAN_POINT('Ctrl Pts',(23.2821634538006,52.1625057785251,-213.215631611061));
#220918=CARTESIAN_POINT('Ctrl Pts',(23.186514300368,52.1717531873607,-213.236361158368));
#220919=CARTESIAN_POINT('Ctrl Pts',(23.1032160300043,52.1798065065351,-213.254413962539));
#220920=CARTESIAN_POINT('Ctrl Pts',(23.0199493662686,52.187803195851,-213.27291866346));
#220921=CARTESIAN_POINT('Ctrl Pts',(22.9367159200592,52.195743293347,-213.291870988623));
#220922=CARTESIAN_POINT('Ctrl Pts',(22.8920159948606,52.2000074657477,-213.302049198894));
#220923=CARTESIAN_POINT('Ctrl Pts',(22.8473256517277,52.2042553156829,-213.312356529244));
#220924=CARTESIAN_POINT('Ctrl Pts',(22.8026451428263,52.2084868488976,-213.322792347156));
#220925=CARTESIAN_POINT('Ctrl Pts',(22.7914750218758,52.209544731607,-213.325401300168));
#220926=CARTESIAN_POINT('Ctrl Pts',(22.780304416052,52.2106019242221,-213.328005681876));
#220927=CARTESIAN_POINT('Ctrl Pts',(22.769132817356,52.2116585796836,-213.330599615209));
#220928=CARTESIAN_POINT('Ctrl Pts',(22.7579612024781,52.2127152366756,-213.333193552299));
#220929=CARTESIAN_POINT('Ctrl Pts',(22.7467887595399,52.2137713070928,-213.335778930073));
#220930=CARTESIAN_POINT('Ctrl Pts',(22.7356154921252,52.2148267904764,-213.3383557354));
#220931=CARTESIAN_POINT('Ctrl Pts',(22.7132688713518,52.2169377653624,-213.343509365876));
#220932=CARTESIAN_POINT('Ctrl Pts',(22.6909189526696,52.2190463920882,-213.348628706468));
#220933=CARTESIAN_POINT('Ctrl Pts',(22.6685657646965,52.2211526670291,-213.353713651068));
#220934=CARTESIAN_POINT('Ctrl Pts',(22.6646488913269,52.2215217424485,-213.354604668677));
#220935=CARTESIAN_POINT('Ctrl Pts',(22.6607319175832,52.2218907456562,-213.35549463026));
#220936=CARTESIAN_POINT('Ctrl Pts',(22.656814843617,52.2222596766334,-213.356383535222));
#220937=CARTESIAN_POINT('Ctrl Pts',(22.571309563035,52.2303130212968,-213.37578732203));
#220938=CARTESIAN_POINT('Ctrl Pts',(22.4857590592471,52.2383317076776,-213.394687120906));
#220939=CARTESIAN_POINT('Ctrl Pts',(22.400164917909,52.2463155472972,-213.413077019702));
#220940=CARTESIAN_POINT('Ctrl Pts',(22.3089921278352,52.2548197383814,-213.432665491017));
#220941=CARTESIAN_POINT('Ctrl Pts',(22.2177437865542,52.2632866458112,-213.451679464809));
#220942=CARTESIAN_POINT('Ctrl Pts',(22.1264553921399,52.2717131158806,-213.470105691494));
#220943=CARTESIAN_POINT('Ctrl Pts',(21.8592067817213,52.2963817764615,-213.524048840656));
#220944=CARTESIAN_POINT('Ctrl Pts',(21.5914443578931,52.320719710873,-213.572977568712));
#220945=CARTESIAN_POINT('Ctrl Pts',(21.3240957724509,52.3446435619465,-213.616545275377));
#220946=CARTESIAN_POINT('Ctrl Pts',(21.2373298036592,52.3524078675335,-213.63068484627));
#220947=CARTESIAN_POINT('Ctrl Pts',(21.1505925461993,52.3601300382443,-213.644263375919));
#220948=CARTESIAN_POINT('Ctrl Pts',(21.0638877077022,52.367809951321,-213.657275547301));
#220949=CARTESIAN_POINT('Ctrl Pts',(19.9403638201412,52.4673264944071,-213.825887652807));
#220950=CARTESIAN_POINT('Ctrl Pts',(18.8213013409432,52.5598362291047,-213.899469470177));
#220951=CARTESIAN_POINT('Ctrl Pts',(17.707326389879,52.6457198325126,-213.866672048325));
#220952=CARTESIAN_POINT('Ctrl Pts',(17.4861860769682,52.6627689833156,-213.860161280624));
#220953=CARTESIAN_POINT('Ctrl Pts',(17.2652462240557,52.6795570130793,-213.849458152787));
#220954=CARTESIAN_POINT('Ctrl Pts',(17.0445116841478,52.6960869022234,-213.834473635931));
#220955=CARTESIAN_POINT('Ctrl Pts',(16.9763221692139,52.7011933306197,-213.829844605348));
#220956=CARTESIAN_POINT('Ctrl Pts',(16.9081523016037,52.7062751479288,-213.824806041847));
#220957=CARTESIAN_POINT('Ctrl Pts',(16.840002239673,52.711332452689,-213.819355050373));
#220958=CARTESIAN_POINT('Ctrl Pts',(16.1996233055684,52.7588539272113,-213.768134258916));
#220959=CARTESIAN_POINT('Ctrl Pts',(15.5609952943595,52.8042113945009,-213.68046926394));
#220960=CARTESIAN_POINT('Ctrl Pts',(14.924248781074,52.8474860509722,-213.553990748347));
#220961=CARTESIAN_POINT('Ctrl Pts',(14.8649438022416,52.8515165443199,-213.542210855511));
#220962=CARTESIAN_POINT('Ctrl Pts',(14.805655093962,52.8555289645469,-213.530094945451));
#220963=CARTESIAN_POINT('Ctrl Pts',(14.7463827693231,52.8595233836131,-213.517640823919));
#220964=CARTESIAN_POINT('Ctrl Pts',(14.6296583420206,52.8673895552329,-213.49311504039));
#220965=CARTESIAN_POINT('Ctrl Pts',(14.5129975854129,52.8751859177491,-213.467277078932));
#220966=CARTESIAN_POINT('Ctrl Pts',(14.3964014059857,52.8829130229972,-213.440109913241));
#220967=CARTESIAN_POINT('Ctrl Pts',(14.3392716131961,52.8866991498142,-213.426798546143));
#220968=CARTESIAN_POINT('Ctrl Pts',(14.2821573282399,52.8904686504836,-213.413167990813));
#220969=CARTESIAN_POINT('Ctrl Pts',(14.2250586750738,52.8942215948612,-213.399215938865));
#220970=CARTESIAN_POINT('Ctrl Pts',(14.194308849405,52.8962427000706,-213.391702221092));
#220971=CARTESIAN_POINT('Ctrl Pts',(14.1635634419795,52.8982590111407,-213.384095232764));
#220972=CARTESIAN_POINT('Ctrl Pts',(14.1328225823492,52.9002705316719,-213.376394641145));
#220973=CARTESIAN_POINT('Ctrl Pts',(14.0889125166806,52.9031437759365,-213.365395160722));
#220974=CARTESIAN_POINT('Ctrl Pts',(14.04501173063,52.9060072461916,-213.354204687974));
#220975=CARTESIAN_POINT('Ctrl Pts',(14.0011206054638,52.9088609546765,-213.342822186056));
#220976=CARTESIAN_POINT('Ctrl Pts',(13.9791751851707,52.9102877996675,-213.337130971998));
#220977=CARTESIAN_POINT('Ctrl Pts',(13.9572335774877,52.9117125570174,-213.331366770806));
#220978=CARTESIAN_POINT('Ctrl Pts',(13.9352910762429,52.9131340283108,-213.325614433984));
#220979=CARTESIAN_POINT('Ctrl Pts',(13.9133485638354,52.9145555003274,-213.319862094235));
#220980=CARTESIAN_POINT('Ctrl Pts',(13.8914033905367,52.9159732398363,-213.314153208262));
#220981=CARTESIAN_POINT('Ctrl Pts',(13.8694556009263,52.9173872435139,-213.308487695886));
#220982=CARTESIAN_POINT('Ctrl Pts',(13.8144534891343,52.9209307980008,-213.294289676376));
#220983=CARTESIAN_POINT('Ctrl Pts',(13.7594349499713,52.9244508908472,-213.280363986675));
#220984=CARTESIAN_POINT('Ctrl Pts',(13.7044006823105,52.9279474706966,-213.266709421035));
#220985=CARTESIAN_POINT('Ctrl Pts',(13.4080399531756,52.9467766292863,-213.193179287882));
#220986=CARTESIAN_POINT('Ctrl Pts',(13.111238199284,52.9649231366537,-213.127512319222));
#220987=CARTESIAN_POINT('Ctrl Pts',(12.8139330465279,52.9823892815607,-213.069496767474));
#220988=CARTESIAN_POINT('Ctrl Pts',(12.7628798586912,52.9853885648508,-213.059534347269));
#220989=CARTESIAN_POINT('Ctrl Pts',(12.7118203984046,52.9883673151377,-213.049796876756));
#220990=CARTESIAN_POINT('Ctrl Pts',(12.6607543476393,52.9913255531845,-213.040283642667));
#220991=CARTESIAN_POINT('Ctrl Pts',(11.9341251305787,53.033418923704,-212.904917900964));
#220992=CARTESIAN_POINT('Ctrl Pts',(11.2065836165116,53.0713381586144,-212.814853696238));
#220993=CARTESIAN_POINT('Ctrl Pts',(10.4781609695859,53.1051019822928,-212.767914897224));
#220994=CARTESIAN_POINT('Ctrl Pts',(9.84365029734438,53.1345128010667,-212.727027688346));
#220995=CARTESIAN_POINT('Ctrl Pts',(9.20847145458215,53.1607704757915,-212.71886382913));
#220996=CARTESIAN_POINT('Ctrl Pts',(8.57265926894805,53.1838840251076,-212.742013573981));
#220997=CARTESIAN_POINT('Ctrl Pts',(8.53829774072219,53.1851331626599,-212.743264667667));
#220998=CARTESIAN_POINT('Ctrl Pts',(8.50393420974303,53.186373110042,-212.744608085481));
#220999=CARTESIAN_POINT('Ctrl Pts',(8.46956866922752,53.1876038661027,-212.746043776936));
#221000=CARTESIAN_POINT('Ctrl Pts',(8.05134105999121,53.2025821308736,-212.76351609939));
#221001=CARTESIAN_POINT('Ctrl Pts',(7.63294373529608,53.2161951626094,-212.794632608455));
#221002=CARTESIAN_POINT('Ctrl Pts',(7.21417793555096,53.2284476001673,-212.839302228769));
#221003=CARTESIAN_POINT('Ctrl Pts',(6.95775348625815,53.2359501816942,-212.866654946675));
#221004=CARTESIAN_POINT('Ctrl Pts',(6.7011908579688,53.2429425029055,-212.899090463672));
#221005=CARTESIAN_POINT('Ctrl Pts',(6.44444424425754,53.2494246606916,-212.936597453296));
#221006=CARTESIAN_POINT('Ctrl Pts',(6.41857408693467,53.2500778122144,-212.940376711407));
#221007=CARTESIAN_POINT('Ctrl Pts',(6.39270791173976,53.2507256250243,-212.944206865458));
#221008=CARTESIAN_POINT('Ctrl Pts',(6.36684597343843,53.2513681007524,-212.948087807708));
#221009=CARTESIAN_POINT('Ctrl Pts',(6.07745447788328,53.2585573148641,-212.991515012155));
#221010=CARTESIAN_POINT('Ctrl Pts',(5.78889207385616,53.2650712745851,-213.041253048807));
#221011=CARTESIAN_POINT('Ctrl Pts',(5.50128323027576,53.270919363331,-213.097172229243));
#221012=CARTESIAN_POINT('Ctrl Pts',(5.46169210968322,53.2717243886004,-213.10486984726));
#221013=CARTESIAN_POINT('Ctrl Pts',(5.42211906881833,53.272516787632,-213.112684672594));
#221014=CARTESIAN_POINT('Ctrl Pts',(5.38256444434729,53.2732965767615,-213.120616442334));
#221015=CARTESIAN_POINT('Ctrl Pts',(5.3611025543334,53.273719681487,-213.124920130514));
#221016=CARTESIAN_POINT('Ctrl Pts',(5.3396451356634,53.2741390978143,-213.129258387298));
#221017=CARTESIAN_POINT('Ctrl Pts',(5.31819206008386,53.2745548325864,-213.133631201848));
#221018=CARTESIAN_POINT('Ctrl Pts',(5.16346960690728,53.2775531674208,-213.165168525801));
#221019=CARTESIAN_POINT('Ctrl Pts',(5.00900884763755,53.2803593125375,-213.198496059741));
#221020=CARTESIAN_POINT('Ctrl Pts',(4.8548075087274,53.282975175313,-213.233598239233));
#221021=CARTESIAN_POINT('Ctrl Pts',(4.83548667519224,53.2833029328383,-213.237996407053));
#221022=CARTESIAN_POINT('Ctrl Pts',(4.81616991445747,53.2836277030468,-213.242422436058));
#221023=CARTESIAN_POINT('Ctrl Pts',(4.79685722222972,53.2839494896213,-213.246876296775));
#221024=CARTESIAN_POINT('Ctrl Pts',(4.72842778016165,53.2850896556584,-213.262657380027));
#221025=CARTESIAN_POINT('Ctrl Pts',(4.66004791848346,53.2861923861431,-213.278788317342));
#221026=CARTESIAN_POINT('Ctrl Pts',(4.59171994251606,53.2872578052511,-213.295267139758));
#221027=CARTESIAN_POINT('Ctrl Pts',(4.5698179350381,53.2875993171566,-213.300549299616));
#221028=CARTESIAN_POINT('Ctrl Pts',(4.54792125858747,53.2879369954791,-213.305867203353));
#221029=CARTESIAN_POINT('Ctrl Pts',(4.5260299888062,53.2882708445054,-213.311220784634));
#221030=CARTESIAN_POINT('Ctrl Pts',(4.51508439514893,53.2884377683898,-213.313897565191));
#221031=CARTESIAN_POINT('Ctrl Pts',(4.50414015314406,53.2886037349587,-213.316583265061));
#221032=CARTESIAN_POINT('Ctrl Pts',(4.49319727224048,53.2887687447573,-213.319277875874));
#221033=CARTESIAN_POINT('Ctrl Pts',(4.48225439119639,53.288933754558,-213.321972486721));
#221034=CARTESIAN_POINT('Ctrl Pts',(4.47131360771932,53.2890977098182,-213.324680797967));
#221035=CARTESIAN_POINT('Ctrl Pts',(4.46037245702231,53.2892609395381,-213.327386711909));
#221036=CARTESIAN_POINT('Ctrl Pts',(4.41660743854964,53.2899138646194,-213.338210470483));
#221037=CARTESIAN_POINT('Ctrl Pts',(4.37281891468805,53.2905575212915,-213.348881124149));
#221038=CARTESIAN_POINT('Ctrl Pts',(4.32900749630779,53.2911918673437,-213.359398181113));
#221039=CARTESIAN_POINT('Ctrl Pts',(4.3117489870416,53.2914417535064,-213.36354113589));
#221040=CARTESIAN_POINT('Ctrl Pts',(4.29448693048927,53.2916901975378,-213.367660294877));
#221041=CARTESIAN_POINT('Ctrl Pts',(4.27722136169741,53.2919371969757,-213.371755612804));
#221042=CARTESIAN_POINT('Ctrl Pts',(3.34936233526414,53.3052110520531,-213.591839743872));
#221043=CARTESIAN_POINT('Ctrl Pts',(2.41131193878792,53.31431299312,-213.743095767745));
#221044=CARTESIAN_POINT('Ctrl Pts',(1.46228217016154,53.3189491272516,-213.820197476168));
#221045=CARTESIAN_POINT('Ctrl Pts',(0.993352427694286,53.3212399101715,
-213.858294578567));
#221046=CARTESIAN_POINT('Ctrl Pts',(0.521742197153976,53.3224404125564,
-213.878287712818));
#221047=CARTESIAN_POINT('Ctrl Pts',(0.0473571427401393,53.3225154460666,
-213.879539002147));
#221048=CARTESIAN_POINT('',(32.9259571996587,50.2082406705958,-216.288179546259));
#221049=CARTESIAN_POINT('Ctrl Pts',(33.8288256585371,50.8425201819751,-213.84207505449));
#221050=CARTESIAN_POINT('Ctrl Pts',(33.8195965630401,50.8433616845868,-213.871510133232));
#221051=CARTESIAN_POINT('Ctrl Pts',(33.8091847500211,50.8440238380756,-213.904584950093));
#221052=CARTESIAN_POINT('Ctrl Pts',(33.7975369080429,50.8442737231641,-213.941293234272));
#221053=CARTESIAN_POINT('Ctrl Pts',(33.7860605485555,50.8445199293808,-213.977461089759));
#221054=CARTESIAN_POINT('Ctrl Pts',(33.7733837057459,50.8443657685501,-214.017156701474));
#221055=CARTESIAN_POINT('Ctrl Pts',(33.7594592797241,50.8435407324466,-214.060358070837));
#221056=CARTESIAN_POINT('Ctrl Pts',(33.7574531295846,50.8434218660538,-214.066582272325));
#221057=CARTESIAN_POINT('Ctrl Pts',(33.7554210983262,50.8432889943485,-214.072879209069));
#221058=CARTESIAN_POINT('Ctrl Pts',(33.7533630630681,50.8431412280489,-214.079248777559));
#221059=CARTESIAN_POINT('Ctrl Pts',(33.743082867682,50.8424031131771,-214.111065729359));
#221060=CARTESIAN_POINT('Ctrl Pts',(33.7321506472359,50.8412946106023,-214.144698787172));
#221061=CARTESIAN_POINT('Ctrl Pts',(33.7205438950311,50.839697062375,-214.180141701911));
#221062=CARTESIAN_POINT('Ctrl Pts',(33.7050682254247,50.8375669980719,-214.227398921562));
#221063=CARTESIAN_POINT('Ctrl Pts',(33.6883933898817,50.8345693205334,-214.277874335582));
#221064=CARTESIAN_POINT('Ctrl Pts',(33.6704630953645,50.8303840566376,-214.3315457339));
#221065=CARTESIAN_POINT('Ctrl Pts',(33.6535595541392,50.8264384560377,-214.382143714498));
#221066=CARTESIAN_POINT('Ctrl Pts',(33.6355453144694,50.8214386172029,-214.435562374112));
#221067=CARTESIAN_POINT('Ctrl Pts',(33.616381403873,50.8150836718686,-214.491738971497));
#221068=CARTESIAN_POINT('Ctrl Pts',(33.5979822127623,50.8089823152004,-214.54567388974));
#221069=CARTESIAN_POINT('Ctrl Pts',(33.5785230926711,50.8016316349254,-214.60215137588));
#221070=CARTESIAN_POINT('Ctrl Pts',(33.5579782849136,50.7927360421654,-214.661078169069));
#221071=CARTESIAN_POINT('Ctrl Pts',(33.5545247916949,50.7912407315431,-214.670983507833));
#221072=CARTESIAN_POINT('Ctrl Pts',(33.5510406454633,50.7897017020583,-214.68095795797));
#221073=CARTESIAN_POINT('Ctrl Pts',(33.5475257550617,50.7881174703285,-214.691000955107));
#221074=CARTESIAN_POINT('Ctrl Pts',(33.5276567606859,50.7791621153292,-214.747772071938));
#221075=CARTESIAN_POINT('Ctrl Pts',(33.5068038044279,50.7687640806476,-214.806738808839));
#221076=CARTESIAN_POINT('Ctrl Pts',(33.4849539835288,50.7566390582463,-214.867785259312));
#221077=CARTESIAN_POINT('Ctrl Pts',(33.4813986178706,50.7546660952435,-214.877718633804));
#221078=CARTESIAN_POINT('Ctrl Pts',(33.4778168848558,50.752647352948,-214.887706978624));
#221079=CARTESIAN_POINT('Ctrl Pts',(33.474208761572,50.7505815441923,-214.897749680414));
#221080=CARTESIAN_POINT('Ctrl Pts',(33.4613176761033,50.7432008326319,-214.93363019694));
#221081=CARTESIAN_POINT('Ctrl Pts',(33.4480895339613,50.7352195121941,-214.970205208588));
#221082=CARTESIAN_POINT('Ctrl Pts',(33.4345241362373,50.7265767845305,-215.007444068341));
#221083=CARTESIAN_POINT('Ctrl Pts',(33.4277414373753,50.7222554206986,-215.026063498218));
#221084=CARTESIAN_POINT('Ctrl Pts',(33.420874423949,50.7177686428876,-215.044848868558));
#221085=CARTESIAN_POINT('Ctrl Pts',(33.4139232666345,50.7131085754662,-215.063795757132));
#221086=CARTESIAN_POINT('Ctrl Pts',(33.4104476879772,50.7107785417556,-215.073269201418));
#221087=CARTESIAN_POINT('Ctrl Pts',(33.4069510734007,50.7084051816795,-215.082783023661));
#221088=CARTESIAN_POINT('Ctrl Pts',(33.4034334518911,50.7059874903625,-215.092336644895));
#221089=CARTESIAN_POINT('Ctrl Pts',(33.4006142359874,50.7040498191854,-215.099993443913));
#221090=CARTESIAN_POINT('Ctrl Pts',(33.3974201203686,50.7018312093553,-215.108655100518));
#221091=CARTESIAN_POINT('Ctrl Pts',(33.3947200356436,50.6999375550647,-215.115966490004));
#221092=CARTESIAN_POINT('Ctrl Pts',(33.3941967810423,50.6995705801652,-215.117383378206));
#221093=CARTESIAN_POINT('Ctrl Pts',(33.3936920899953,50.6992159596698,-215.118749616727));
#221094=CARTESIAN_POINT('Ctrl Pts',(33.3932122995932,50.6988783027811,-215.120048145458));
#221095=CARTESIAN_POINT('Ctrl Pts',(33.3930787584929,50.698784322009,-215.120409567768));
#221096=CARTESIAN_POINT('Ctrl Pts',(33.3929471464134,50.6986916573888,-215.120765745917));
#221097=CARTESIAN_POINT('Ctrl Pts',(33.3928176000307,50.6986004087735,-215.121116312229));
#221098=CARTESIAN_POINT('Ctrl Pts',(33.3296193541769,50.6540854458574,-215.292137497787));
#221099=CARTESIAN_POINT('Ctrl Pts',(33.269750414294,50.6027332408916,-215.448578025303));
#221100=CARTESIAN_POINT('Ctrl Pts',(33.213875240217,50.5483631417154,-215.590759975443));
#221101=CARTESIAN_POINT('Ctrl Pts',(33.1849670106321,50.520233595177,-215.664320881971));
#221102=CARTESIAN_POINT('Ctrl Pts',(33.157127397143,50.4912973997056,-215.734065604051));
#221103=CARTESIAN_POINT('Ctrl Pts',(33.130445480466,50.4620814546802,-215.800037964159));
#221104=CARTESIAN_POINT('Ctrl Pts',(33.1027008264358,50.4317018422744,-215.868637994993));
#221105=CARTESIAN_POINT('Ctrl Pts',(33.076200305561,50.4010143910844,-215.933180065315));
#221106=CARTESIAN_POINT('Ctrl Pts',(33.0509711670511,50.3705041612344,-215.993871545003));
#221107=CARTESIAN_POINT('Ctrl Pts',(33.0258539400521,50.340129268781,-216.054293809189));
#221108=CARTESIAN_POINT('Ctrl Pts',(33.0019968128992,50.3099300470371,-216.110899575011));
#221109=CARTESIAN_POINT('Ctrl Pts',(32.9794222099075,50.2803372957559,-216.163874712886));
#221110=CARTESIAN_POINT('Ctrl Pts',(32.9607164963076,50.2558162208868,-216.207770845074));
#221111=CARTESIAN_POINT('Ctrl Pts',(32.9428912873839,50.2317107069135,-216.249173830476));
#221112=CARTESIAN_POINT('Ctrl Pts',(32.9259571994407,50.208240670622,-216.288179546181));
#221113=CARTESIAN_POINT('',(23.3713075575292,51.175583428683,-216.122695209519));
#221114=CARTESIAN_POINT('Ctrl Pts',(23.3713098772595,51.175574422021,-216.122706729219));
#221115=CARTESIAN_POINT('Ctrl Pts',(23.3842461965447,51.1745227766932,-216.1193823466));
#221116=CARTESIAN_POINT('Ctrl Pts',(23.4031827800646,51.173197367639,-216.114240118892));
#221117=CARTESIAN_POINT('Ctrl Pts',(23.4259755039501,51.172009386705,-216.10752048342));
#221118=CARTESIAN_POINT('Ctrl Pts',(23.4363729991939,51.171582118472,-216.104305205249));
#221119=CARTESIAN_POINT('Ctrl Pts',(23.4422558498776,51.1713690087708,-216.102448446714));
#221120=CARTESIAN_POINT('Ctrl Pts',(23.4450357599012,51.1712750486653,-216.10156219481));
#221121=CARTESIAN_POINT('Ctrl Pts',(23.4463575991215,51.1712315234358,-216.101139270919));
#221122=CARTESIAN_POINT('Ctrl Pts',(23.4531000314565,51.1708420894904,-216.099209074551));
#221123=CARTESIAN_POINT('Ctrl Pts',(23.4715714957454,51.1697457853851,-216.093982383968));
#221124=CARTESIAN_POINT('Ctrl Pts',(23.4828968517328,51.1690699569358,-216.090786189668));
#221125=CARTESIAN_POINT('Ctrl Pts',(23.4997698432704,51.1680649377872,-216.086037310555));
#221126=CARTESIAN_POINT('Ctrl Pts',(23.5077858872702,51.1675887931229,-216.083783508271));
#221127=CARTESIAN_POINT('Ctrl Pts',(23.5133043622529,51.1672613852725,-216.082232402665));
#221128=CARTESIAN_POINT('Ctrl Pts',(23.5175432944616,51.1670102829937,-216.081041398148));
#221129=CARTESIAN_POINT('Ctrl Pts',(23.5684041867088,51.1640002556831,-216.066753810042));
#221130=CARTESIAN_POINT('Ctrl Pts',(23.617522122373,51.1610630770063,-216.053151092884));
#221131=CARTESIAN_POINT('Ctrl Pts',(23.765876757628,51.1521012881781,-216.012658976564));
#221132=CARTESIAN_POINT('Ctrl Pts',(23.8636871351588,51.1460726566935,-215.986741705726));
#221133=CARTESIAN_POINT('Ctrl Pts',(24.0625051787286,51.1335736717109,-215.935672011281));
#221134=CARTESIAN_POINT('Ctrl Pts',(24.1616902419922,51.127214610338,-215.911003826816));
#221135=CARTESIAN_POINT('Ctrl Pts',(24.3595824477507,51.1142829433766,-215.863400783403));
#221136=CARTESIAN_POINT('Ctrl Pts',(24.4562741336651,51.1078470209333,-215.84091768686));
#221137=CARTESIAN_POINT('Ctrl Pts',(24.757680353937,51.0874063464124,-215.773357811072));
#221138=CARTESIAN_POINT('Ctrl Pts',(25.0576479162834,51.0662997370015,-215.711186730808));
#221139=CARTESIAN_POINT('Ctrl Pts',(25.4047677167914,51.0405701572308,-215.648084196));
#221140=CARTESIAN_POINT('Ctrl Pts',(25.5775768522701,51.0274352005315,-215.618890526638));
#221141=CARTESIAN_POINT('Ctrl Pts',(25.6514727371838,51.0217486675082,-215.606884153634));
#221142=CARTESIAN_POINT('Ctrl Pts',(25.7006994792023,51.0179449857611,-215.598992171539));
#221143=CARTESIAN_POINT('Ctrl Pts',(25.7241069658211,51.0161293054655,-215.595287525604));
#221144=CARTESIAN_POINT('Ctrl Pts',(26.1620821414063,50.9820110096248,-215.526965608493));
#221145=CARTESIAN_POINT('Ctrl Pts',(26.5699068021216,50.9480387215192,-215.478347477118));
#221146=CARTESIAN_POINT('Ctrl Pts',(27.173438244869,50.8946136997262,-215.428947554207));
#221147=CARTESIAN_POINT('Ctrl Pts',(27.4731530412198,50.8672827350125,-215.41012941129));
#221148=CARTESIAN_POINT('Ctrl Pts',(27.8188791896975,50.834366423916,-215.398468093662));
#221149=CARTESIAN_POINT('Ctrl Pts',(27.9907131851713,50.8176558576065,-215.395210730458));
#221150=CARTESIAN_POINT('Ctrl Pts',(28.0763674429529,50.809238077671,-215.394225372759));
#221151=CARTESIAN_POINT('Ctrl Pts',(28.1130195236067,50.805617126528,-215.393940931724));
#221152=CARTESIAN_POINT('Ctrl Pts',(28.137441537465,50.8032002031682,-215.393781938839));
#221153=CARTESIAN_POINT('Ctrl Pts',(28.1484568678156,50.8021083756591,-215.393722523643));
#221154=CARTESIAN_POINT('Ctrl Pts',(29.8754561237135,50.6305994564353,-215.386804771997));
#221155=CARTESIAN_POINT('Ctrl Pts',(31.4945003627672,50.4284988051297,-215.684974988241));
#221156=CARTESIAN_POINT('Ctrl Pts',(32.9259571993476,50.2082406704928,-216.288179546395));
#221157=CARTESIAN_POINT('Ctrl Pts',(13.206503688621,52.1340678863284,-215.899726709711));
#221158=CARTESIAN_POINT('Ctrl Pts',(13.21434555531,52.1335848677323,-215.90178674226));
#221159=CARTESIAN_POINT('Ctrl Pts',(13.2231507448613,52.1330862366278,-215.904029229699));
#221160=CARTESIAN_POINT('Ctrl Pts',(13.2322895587349,52.1325819238806,-215.906330078911));
#221161=CARTESIAN_POINT('Ctrl Pts',(13.2421441100756,52.1320381141556,-215.908811126998));
#221162=CARTESIAN_POINT('Ctrl Pts',(13.2523869533356,52.1314876923625,-215.911360109152));
#221163=CARTESIAN_POINT('Ctrl Pts',(13.2622878817901,52.1309421505403,-215.913833109968));
#221164=CARTESIAN_POINT('Ctrl Pts',(13.2644020884909,52.1308256576092,-215.914361185181));
#221165=CARTESIAN_POINT('Ctrl Pts',(13.2665008919367,52.1307093841564,-215.914885832636));
#221166=CARTESIAN_POINT('Ctrl Pts',(13.268577468265,52.1305934374337,-215.915405707262));
#221167=CARTESIAN_POINT('Ctrl Pts',(13.3206494413752,52.1276859716487,-215.92844201957));
#221168=CARTESIAN_POINT('Ctrl Pts',(13.3712586349829,52.1247839437585,-215.940981499432));
#221169=CARTESIAN_POINT('Ctrl Pts',(13.4220397900242,52.1218170785976,-215.953412057766));
#221170=CARTESIAN_POINT('Ctrl Pts',(13.4721084324292,52.1188918416532,-215.965668202386));
#221171=CARTESIAN_POINT('Ctrl Pts',(13.5223442093494,52.1159035600009,-215.977818360123));
#221172=CARTESIAN_POINT('Ctrl Pts',(13.5743125134382,52.1127772956712,-215.990186103883));
#221173=CARTESIAN_POINT('Ctrl Pts',(13.6237866881243,52.1098010710228,-216.001960279046));
#221174=CARTESIAN_POINT('Ctrl Pts',(13.6748310589708,52.106699798131,-216.01393169343));
#221175=CARTESIAN_POINT('Ctrl Pts',(13.7287953846035,52.1034020067022,-216.026336308893));
#221176=CARTESIAN_POINT('Ctrl Pts',(13.7581476789267,52.1016082708685,-216.033083431548));
#221177=CARTESIAN_POINT('Ctrl Pts',(13.7883638330608,52.0997562789374,-216.039957977688));
#221178=CARTESIAN_POINT('Ctrl Pts',(13.8196609440104,52.0978335624414,-216.046991805997));
#221179=CARTESIAN_POINT('Ctrl Pts',(13.8490469338718,52.0960282543556,-216.053596121894));
#221180=CARTESIAN_POINT('Ctrl Pts',(13.8789171341203,52.0941830434785,-216.060245085436));
#221181=CARTESIAN_POINT('Ctrl Pts',(13.9092735522173,52.0922980630924,-216.066930897808));
#221182=CARTESIAN_POINT('Ctrl Pts',(13.9325325762528,52.0908537950643,-216.072053553259));
#221183=CARTESIAN_POINT('Ctrl Pts',(13.9518947805123,52.0896438292969,-216.076285734692));
#221184=CARTESIAN_POINT('Ctrl Pts',(13.9714301061238,52.0884198382981,-216.080530595315));
#221185=CARTESIAN_POINT('Ctrl Pts',(13.9773912291603,52.0880463425559,-216.081825896809));
#221186=CARTESIAN_POINT('Ctrl Pts',(13.9833684716841,52.0876714833885,-216.083122015781));
#221187=CARTESIAN_POINT('Ctrl Pts',(13.9894774736147,52.0872880602886,-216.08444370039));
#221188=CARTESIAN_POINT('Ctrl Pts',(14.0417353629624,52.0840081657732,-216.095749712219));
#221189=CARTESIAN_POINT('Ctrl Pts',(14.0940361976639,52.080693570248,-216.10686308862));
#221190=CARTESIAN_POINT('Ctrl Pts',(14.1463794799969,52.0773442814346,-216.117783727481));
#221191=CARTESIAN_POINT('Ctrl Pts',(14.2116086830721,52.0731704614059,-216.131392819961));
#221192=CARTESIAN_POINT('Ctrl Pts',(14.2770368470204,52.0689342305803,-216.144729384953));
#221193=CARTESIAN_POINT('Ctrl Pts',(14.3424131370686,52.0646515126906,-216.157742539444));
#221194=CARTESIAN_POINT('Ctrl Pts',(14.3819594720578,52.0620608824145,-216.165614239817));
#221195=CARTESIAN_POINT('Ctrl Pts',(14.4214887322589,52.0594530513133,-216.173367856955));
#221196=CARTESIAN_POINT('Ctrl Pts',(14.4609448354491,52.0568318528244,-216.180993676633));
#221197=CARTESIAN_POINT('Ctrl Pts',(14.6703112873129,52.0429229519732,-216.221458666319));
#221198=CARTESIAN_POINT('Ctrl Pts',(14.8802278373797,52.0284671787079,-216.258828965844));
#221199=CARTESIAN_POINT('Ctrl Pts',(15.0906678685067,52.0134661474936,-216.29311301509));
#221200=CARTESIAN_POINT('Ctrl Pts',(15.2048442057614,52.0053271884281,-216.311714167866));
#221201=CARTESIAN_POINT('Ctrl Pts',(15.3196612788897,51.9969923389717,-216.329481780615));
#221202=CARTESIAN_POINT('Ctrl Pts',(15.4343240930968,51.9885185807898,-216.346290289808));
#221203=CARTESIAN_POINT('Ctrl Pts',(15.4912716221164,51.9843100708792,-216.354638271424));
#221204=CARTESIAN_POINT('Ctrl Pts',(15.5481810921433,51.9800674264624,-216.362750478828));
#221205=CARTESIAN_POINT('Ctrl Pts',(15.6049550958312,51.9757983834695,-216.37061622704));
#221206=CARTESIAN_POINT('Ctrl Pts',(15.6432593674605,51.972918146534,-216.375923088218));
#221207=CARTESIAN_POINT('Ctrl Pts',(15.6815019757728,51.9700259035013,-216.381117827339));
#221208=CARTESIAN_POINT('Ctrl Pts',(15.7196530119027,51.9671241561828,-216.386197949282));
#221209=CARTESIAN_POINT('Ctrl Pts',(15.7321491591731,51.9661737059327,-216.387861913316));
#221210=CARTESIAN_POINT('Ctrl Pts',(15.7446430517792,51.9652216618178,-216.38951459821));
#221211=CARTESIAN_POINT('Ctrl Pts',(15.757141562356,51.964267500545,-216.391156918244));
#221212=CARTESIAN_POINT('Ctrl Pts',(16.1023878232211,51.9379107110961,-216.436522711827));
#221213=CARTESIAN_POINT('Ctrl Pts',(16.4495094479191,51.9100635699139,-216.473758372625));
#221214=CARTESIAN_POINT('Ctrl Pts',(16.7982755207299,51.8807308388097,-216.502811102886));
#221215=CARTESIAN_POINT('Ctrl Pts',(16.9356744178246,51.8691749989024,-216.514256634452));
#221216=CARTESIAN_POINT('Ctrl Pts',(17.0733636198955,51.8573836148247,-216.524441248057));
#221217=CARTESIAN_POINT('Ctrl Pts',(17.2113121006742,51.8453591541769,-216.533361219666));
#221218=CARTESIAN_POINT('Ctrl Pts',(17.3873312366818,51.8300162148257,-216.544742901341));
#221219=CARTESIAN_POINT('Ctrl Pts',(17.563780758969,51.8142931202842,-216.554066374654));
#221220=CARTESIAN_POINT('Ctrl Pts',(17.740651385583,51.798190546547,-216.561329640317));
#221221=CARTESIAN_POINT('Ctrl Pts',(17.82908669889,51.7901392596783,-216.564961273148));
#221222=CARTESIAN_POINT('Ctrl Pts',(17.9176273123319,51.7819931029086,-216.568077867492));
#221223=CARTESIAN_POINT('Ctrl Pts',(18.0062721385295,51.7737521657921,-216.57067924594));
#221224=CARTESIAN_POINT('Ctrl Pts',(18.0284333450789,51.771691931513,-216.571329590552));
#221225=CARTESIAN_POINT('Ctrl Pts',(18.0506010648767,51.7696257735029,-216.571947734384));
#221226=CARTESIAN_POINT('Ctrl Pts',(18.0727752807906,51.767553693247,-216.572533675092));
#221227=CARTESIAN_POINT('Ctrl Pts',(18.0826472293756,51.7666312042702,-216.572794535568));
#221228=CARTESIAN_POINT('Ctrl Pts',(18.0925204655065,51.7657075414897,-216.573049013306));
#221229=CARTESIAN_POINT('Ctrl Pts',(18.1023949876674,51.7647827050386,-216.573297108109));
#221230=CARTESIAN_POINT('Ctrl Pts',(18.1081226892839,51.7642462550566,-216.573441015123));
#221231=CARTESIAN_POINT('Ctrl Pts',(18.1138457806533,51.7637098836875,-216.573582655078));
#221232=CARTESIAN_POINT('Ctrl Pts',(18.1195929857986,51.763170895431,-216.573722717714));
#221233=CARTESIAN_POINT('Ctrl Pts',(18.1603576817877,51.7593478733078,-216.574716176378));
#221234=CARTESIAN_POINT('Ctrl Pts',(18.2020533295113,51.7554188871131,-216.575618681072));
#221235=CARTESIAN_POINT('Ctrl Pts',(18.2422451882278,51.7516141613284,-216.576382388678));
#221236=CARTESIAN_POINT('Ctrl Pts',(18.2524463154636,51.750648480888,-216.576576225905));
#221237=CARTESIAN_POINT('Ctrl Pts',(18.2625505722048,51.7496908479096,-216.576761383499));
#221238=CARTESIAN_POINT('Ctrl Pts',(18.2725181564702,51.748745111455,-216.576937599951));
#221239=CARTESIAN_POINT('Ctrl Pts',(18.7428983089622,51.7041148734871,-216.585253428466));
#221240=CARTESIAN_POINT('Ctrl Pts',(19.216369753222,51.6568224052065,-216.57911957981));
#221241=CARTESIAN_POINT('Ctrl Pts',(19.6931266362225,51.6068304012012,-216.55847565067));
#221242=CARTESIAN_POINT('Ctrl Pts',(20.1859350419897,51.555155258852,-216.537136678604));
#221243=CARTESIAN_POINT('Ctrl Pts',(20.6822542104159,51.5005957234902,-216.500293855085));
#221244=CARTESIAN_POINT('Ctrl Pts',(21.182281606225,51.4431025697233,-216.447827972626));
#221245=CARTESIAN_POINT('Ctrl Pts',(21.3543133005346,51.4233223642053,-216.429777372342));
#221246=CARTESIAN_POINT('Ctrl Pts',(21.5267837552778,51.4031948498831,-216.409877098555));
#221247=CARTESIAN_POINT('Ctrl Pts',(21.6997004409249,51.38271782281,-216.388121030837));
#221248=CARTESIAN_POINT('Ctrl Pts',(21.9953744771053,51.3477037047621,-216.350919853117));
#221249=CARTESIAN_POINT('Ctrl Pts',(22.2925066862195,51.3116541950269,-216.308265698683));
#221250=CARTESIAN_POINT('Ctrl Pts',(22.5903904274446,51.2746319829009,-216.260299999768));
#221251=CARTESIAN_POINT('Ctrl Pts',(22.6888701076597,51.2623925246612,-216.244442649947));
#221252=CARTESIAN_POINT('Ctrl Pts',(22.7874315150287,51.2500467878896,-216.228004830549));
#221253=CARTESIAN_POINT('Ctrl Pts',(22.8860478603066,51.2375971391525,-216.21099182717));
#221254=CARTESIAN_POINT('Ctrl Pts',(22.8969925217376,51.2362154494338,-216.209103686199));
#221255=CARTESIAN_POINT('Ctrl Pts',(22.9079381323242,51.2348324777314,-216.207208369015));
#221256=CARTESIAN_POINT('Ctrl Pts',(22.9188844817569,51.233448249318,-216.205305911946));
#221257=CARTESIAN_POINT('Ctrl Pts',(23.0199556227651,51.2206672262,-216.187739918103));
#221258=CARTESIAN_POINT('Ctrl Pts',(23.1211180993683,51.2077756142702,-216.169561242903));
#221259=CARTESIAN_POINT('Ctrl Pts',(23.2222432186999,51.1947893198607,-216.150796397354));
#221260=CARTESIAN_POINT('Ctrl Pts',(23.2474937923346,51.1915466894895,-216.14611088383));
#221261=CARTESIAN_POINT('Ctrl Pts',(23.2727420420805,51.1882981597227,-216.141388850273));
#221262=CARTESIAN_POINT('Ctrl Pts',(23.2979859748199,51.1850439859153,-216.136630762429));
#221263=CARTESIAN_POINT('Ctrl Pts',(23.310606184657,51.1834171254447,-216.134252049585));
#221264=CARTESIAN_POINT('Ctrl Pts',(23.3232253155973,51.1817888544157,-216.131864325995));
#221265=CARTESIAN_POINT('Ctrl Pts',(23.3358431189853,51.180159205015,-216.129467651824));
#221266=CARTESIAN_POINT('Ctrl Pts',(23.3476893197676,51.1786292117656,-216.127217538822));
#221267=CARTESIAN_POINT('Ctrl Pts',(23.3616078199705,51.1763334684996,-216.125238790202));
#221268=CARTESIAN_POINT('Ctrl Pts',(23.3713052124462,51.1755924372823,-216.1226836965));
#221269=CARTESIAN_POINT('Ctrl Pts',(32.9259571993474,50.2082406704929,-216.288179546395));
#221270=CARTESIAN_POINT('Ctrl Pts',(33.2211981697202,50.1902923385546,-216.363964513646));
#221271=CARTESIAN_POINT('Ctrl Pts',(33.5148860377456,50.119298258903,-216.408010072973));
#221272=CARTESIAN_POINT('Ctrl Pts',(33.085259856697,50.4290321519905,-215.921237668862));
#221273=CARTESIAN_POINT('Ctrl Pts',(33.3343836373402,50.4107015464113,-215.980471424072));
#221274=CARTESIAN_POINT('Ctrl Pts',(33.5814103734301,50.3541144443598,-216.021456775784));
#221275=CARTESIAN_POINT('Ctrl Pts',(33.241157299543,50.5918672086098,-215.531581018364));
#221276=CARTESIAN_POINT('Ctrl Pts',(33.4420534427606,50.5741543933337,-215.576409379719));
#221277=CARTESIAN_POINT('Ctrl Pts',(33.6410713756206,50.5314895370126,-215.611814434793));
#221278=CARTESIAN_POINT('Ctrl Pts',(33.5452672954357,50.8058893973708,-214.708515271655));
#221279=CARTESIAN_POINT('Ctrl Pts',(33.6463864491617,50.7933600420917,-214.728899815191));
#221280=CARTESIAN_POINT('Ctrl Pts',(33.74687298472,50.7754606859937,-214.748374319679));
#221281=CARTESIAN_POINT('Ctrl Pts',(33.6935058134431,50.8548585528471,-214.273661258903));
#221282=CARTESIAN_POINT('Ctrl Pts',(33.7431496001434,50.8473673908384,-214.28335774542));
#221283=CARTESIAN_POINT('Ctrl Pts',(33.7927859204527,50.839876592974,-214.293095991117));
#221284=CARTESIAN_POINT('Ctrl Pts',(33.8288256585371,50.8425201819751,-213.84207505449));
#221285=CARTESIAN_POINT('Ctrl Pts',(33.8288256585371,50.8425201819751,-213.84207505449));
#221286=CARTESIAN_POINT('Ctrl Pts',(33.8288256585371,50.8425201819751,-213.84207505449));
#221287=CARTESIAN_POINT('',(33.5148860365099,50.1192982504877,-216.408010067648));
#221288=CARTESIAN_POINT('Ctrl Pts',(33.828825603085,50.8425198058687,-213.84207504786));
#221289=CARTESIAN_POINT('Ctrl Pts',(33.8203599637206,50.8418988523823,-213.948018702658));
#221290=CARTESIAN_POINT('Ctrl Pts',(33.8113602728046,50.8379426869151,-214.054203876756));
#221291=CARTESIAN_POINT('Ctrl Pts',(33.801851649264,50.8306220685841,-214.160265521188));
#221292=CARTESIAN_POINT('Ctrl Pts',(33.7923627726763,50.8233166532847,-214.266106903004));
#221293=CARTESIAN_POINT('Ctrl Pts',(33.782367072251,50.8126607033274,-214.371824659818));
#221294=CARTESIAN_POINT('Ctrl Pts',(33.7718970641518,50.7986764690415,-214.477053509786));
#221295=CARTESIAN_POINT('Ctrl Pts',(33.7614327641875,50.7846998588086,-214.582224990125));
#221296=CARTESIAN_POINT('Ctrl Pts',(33.7504946875091,50.7673986651718,-214.686907490459));
#221297=CARTESIAN_POINT('Ctrl Pts',(33.739122769926,50.7468461932371,-214.790742945814));
#221298=CARTESIAN_POINT('Ctrl Pts',(33.7277363195123,50.726267456111,-214.894711098498));
#221299=CARTESIAN_POINT('Ctrl Pts',(33.7159149485736,50.7024293080928,-214.997829456524));
#221300=CARTESIAN_POINT('Ctrl Pts',(33.7037059133141,50.6754546714005,-215.099754179867));
#221301=CARTESIAN_POINT('Ctrl Pts',(33.7004879085736,50.6683448132581,-215.126619057879));
#221302=CARTESIAN_POINT('Ctrl Pts',(33.6972430090231,50.6610173127084,-215.153401121628));
#221303=CARTESIAN_POINT('Ctrl Pts',(33.6939721578997,50.6534749601291,-215.180094331735));
#221304=CARTESIAN_POINT('Ctrl Pts',(33.680746959044,50.6229785819881,-215.288024347028));
#221305=CARTESIAN_POINT('Ctrl Pts',(33.6670909984717,50.5889646595794,-215.394538656221));
#221306=CARTESIAN_POINT('Ctrl Pts',(33.6530129144354,50.5514703365522,-215.499660268446));
#221307=CARTESIAN_POINT('Ctrl Pts',(33.6390782603778,50.5143580122358,-215.603710883327));
#221308=CARTESIAN_POINT('Ctrl Pts',(33.62472996409,50.4738353334169,-215.706398080906));
#221309=CARTESIAN_POINT('Ctrl Pts',(33.6099691795183,50.4298895667813,-215.807726784846));
#221310=CARTESIAN_POINT('Ctrl Pts',(33.5949804948845,50.3852652967167,-215.910619959686));
#221311=CARTESIAN_POINT('Ctrl Pts',(33.5795664055371,50.337110875308,-216.012113461442));
#221312=CARTESIAN_POINT('Ctrl Pts',(33.5637217734253,50.2853700999101,-216.112178111571));
#221313=CARTESIAN_POINT('Ctrl Pts',(33.5478771413135,50.2336293245122,-216.2122427617));
#221314=CARTESIAN_POINT('Ctrl Pts',(33.5316018373211,50.1783013178955,-216.310879445869));
#221315=CARTESIAN_POINT('Ctrl Pts',(33.5148860340386,50.1192982336575,-216.408010056999));
#221316=CARTESIAN_POINT('Origin',(33.1454591002416,47.6034469977721,-214.816150729402));
#221317=CARTESIAN_POINT('Ctrl Pts',(42.4267736782988,48.5085693923201,-216.591605848694));
#221318=CARTESIAN_POINT('Ctrl Pts',(42.583706717545,49.3531444934432,-215.348104479787));
#221319=CARTESIAN_POINT('Ctrl Pts',(42.5875626890161,49.379257463449,-213.836967828456));
#221320=CARTESIAN_POINT('Ctrl Pts',(39.4353118162483,49.0695244129458,-216.590608342213));
#221321=CARTESIAN_POINT('Ctrl Pts',(39.5811128234,49.9141052314507,-215.348112574353));
#221322=CARTESIAN_POINT('Ctrl Pts',(39.5843350108959,49.9402879854258,-213.83895548199));
#221323=CARTESIAN_POINT('Ctrl Pts',(36.428830517738,49.5716582570521,-216.58986415622));
#221324=CARTESIAN_POINT('Ctrl Pts',(36.5632179392288,50.4163761404316,-215.34823479602));
#221325=CARTESIAN_POINT('Ctrl Pts',(36.5662930978424,50.4425286599252,-213.840777099111));
#221326=CARTESIAN_POINT('Ctrl Pts',(33.4195851394632,50.0130984955555,-216.589106829638));
#221327=CARTESIAN_POINT('Ctrl Pts',(33.542491458609,50.8579889698439,-215.348218150781));
#221328=CARTESIAN_POINT('Ctrl Pts',(33.5455787101075,50.8841045229765,-213.842210502424));
#221329=CARTESIAN_POINT('',(33.4734406969954,50.0051916611406,-216.589120383859));
#221330=CARTESIAN_POINT('',(42.426773677794,48.5085693922785,-216.591605848887));
#221331=CARTESIAN_POINT('Ctrl Pts',(33.4734406957278,50.0051916525032,-216.589120377853));
#221332=CARTESIAN_POINT('Ctrl Pts',(34.6872050562177,49.8268448619461,-216.589425787482));
#221333=CARTESIAN_POINT('Ctrl Pts',(35.900785979965,49.6385891008449,-216.589729376108));
#221334=CARTESIAN_POINT('Ctrl Pts',(37.1141764064761,49.4403902132283,-216.590048882378));
#221335=CARTESIAN_POINT('Ctrl Pts',(38.3138694840402,49.2444286923036,-216.590364781903));
#221336=CARTESIAN_POINT('Ctrl Pts',(39.5133769998352,49.038747081503,-216.590696227305));
#221337=CARTESIAN_POINT('Ctrl Pts',(40.7126774431349,48.8232639614083,-216.591060621883));
#221338=CARTESIAN_POINT('Ctrl Pts',(41.2840915331536,48.720595700364,-216.591234239927));
#221339=CARTESIAN_POINT('Ctrl Pts',(41.8554583384076,48.6157016985461,-216.591415342921));
#221340=CARTESIAN_POINT('Ctrl Pts',(42.4267736778188,48.5085693924101,-216.591605848693));
#221341=CARTESIAN_POINT('Origin',(31.3861213810748,49.6296476280943,-215.743606971984));
#221342=CARTESIAN_POINT('',(42.5875626890161,49.379257463449,-213.836967828456));
#221343=CARTESIAN_POINT('Origin',(32.5120060875395,16.8401705115765,-213.68691157036));
#221344=CARTESIAN_POINT('Origin',(41.6694842675319,44.465041620637,-213.749705796269));
#221345=CARTESIAN_POINT('Ctrl Pts',(32.8943360433596,50.1648136138274,-216.360311415042));
#221346=CARTESIAN_POINT('Ctrl Pts',(33.1846932575851,50.1143213461432,-216.493132115846));
#221347=CARTESIAN_POINT('Ctrl Pts',(33.4734406974176,50.0051916640201,-216.589120385861));
#221348=CARTESIAN_POINT('Ctrl Pts',(32.9074380702227,50.1790964451624,-216.336991557183));
#221349=CARTESIAN_POINT('Ctrl Pts',(33.1995861132115,50.1392297940232,-216.451282693355));
#221350=CARTESIAN_POINT('Ctrl Pts',(33.4901672823063,50.0432442151984,-216.530872105694));
#221351=CARTESIAN_POINT('Ctrl Pts',(32.9180956124805,50.1935640066324,-216.312978006505));
#221352=CARTESIAN_POINT('Ctrl Pts',(33.2118808797868,50.1645315900617,-216.408280615883));
#221353=CARTESIAN_POINT('Ctrl Pts',(33.5041153010624,50.0812800820291,-216.470595425695));
#221354=CARTESIAN_POINT('Ctrl Pts',(32.9259571993478,50.2082406704929,-216.288179546395));
#221355=CARTESIAN_POINT('Ctrl Pts',(33.2211981697207,50.1902923385545,-216.363964513646));
#221356=CARTESIAN_POINT('Ctrl Pts',(33.514886037746,50.1192982589029,-216.408010072973));
#221357=CARTESIAN_POINT('',(32.8943360433598,50.1648136138275,-216.360311415042));
#221358=CARTESIAN_POINT('Origin',(33.114566694526,47.5599010752717,-214.888601821826));
#221359=CARTESIAN_POINT('Ctrl Pts',(32.9259571993478,50.2082406704928,-216.288179546395));
#221360=CARTESIAN_POINT('Ctrl Pts',(32.9213942089986,50.1997220625292,-216.302573035724));
#221361=CARTESIAN_POINT('Ctrl Pts',(32.9158742467131,50.1912547814121,-216.316733684137));
#221362=CARTESIAN_POINT('Ctrl Pts',(32.9095161990492,50.1828980465912,-216.330573580559));
#221363=CARTESIAN_POINT('Ctrl Pts',(32.9048796509347,50.1768039741453,-216.340666198458));
#221364=CARTESIAN_POINT('Ctrl Pts',(32.8997987066436,50.1707685930943,-216.350588604011));
#221365=CARTESIAN_POINT('Ctrl Pts',(32.8943360433598,50.1648136138274,-216.360311415041));
#221366=CARTESIAN_POINT('Ctrl Pts',(43.8236246153786,48.0167834579706,-216.751202893194));
#221367=CARTESIAN_POINT('Ctrl Pts',(43.7824688833554,49.1245550970912,-215.437118008003));
#221368=CARTESIAN_POINT('Ctrl Pts',(43.4788788509402,49.2125323561774,-213.747150416911));
#221369=CARTESIAN_POINT('Ctrl Pts',(43.7070375561973,48.0584796180488,-216.749598999916));
#221370=CARTESIAN_POINT('Ctrl Pts',(43.6780057882132,49.1445743904358,-215.439141898609));
#221371=CARTESIAN_POINT('Ctrl Pts',(43.3960890720396,49.2280611496102,-213.762531770702));
#221372=CARTESIAN_POINT('Ctrl Pts',(43.5769822704868,48.1075829537179,-216.741403895083));
#221373=CARTESIAN_POINT('Ctrl Pts',(43.5654977323301,49.1661436865509,-215.436130708587));
#221374=CARTESIAN_POINT('Ctrl Pts',(43.3131689559366,49.2435966472704,-213.776308010994));
#221375=CARTESIAN_POINT('Ctrl Pts',(43.3411495534845,48.1931491450329,-216.723561139181));
#221376=CARTESIAN_POINT('Ctrl Pts',(43.360551859855,49.2053294166112,-215.42835185675));
#221377=CARTESIAN_POINT('Ctrl Pts',(43.1590773754414,49.2724456764506,-213.798159517638));
#221378=CARTESIAN_POINT('Ctrl Pts',(43.2329881782316,48.2313298419848,-216.7140760013));
#221379=CARTESIAN_POINT('Ctrl Pts',(43.2666405269032,49.2232479005123,-215.423740216265));
#221380=CARTESIAN_POINT('Ctrl Pts',(43.0879593352497,49.2857509575947,-213.806842606535));
#221381=CARTESIAN_POINT('Ctrl Pts',(43.0131869934634,48.3080252308524,-216.690346042172));
#221382=CARTESIAN_POINT('Ctrl Pts',(43.0771008479443,49.25936156653,-215.41076207127));
#221383=CARTESIAN_POINT('Ctrl Pts',(42.9454754544989,49.3123914274194,-213.82126574075));
#221384=CARTESIAN_POINT('Ctrl Pts',(42.9009214691654,48.3469469661758,-216.675816338558));
#221385=CARTESIAN_POINT('Ctrl Pts',(42.9810968950835,49.2776314124782,-215.402200104636));
#221386=CARTESIAN_POINT('Ctrl Pts',(42.8741106150282,49.325726212528,-213.827018288817));
#221387=CARTESIAN_POINT('Ctrl Pts',(42.6462982590026,48.4352161716465,-216.634760492906));
#221388=CARTESIAN_POINT('Ctrl Pts',(42.7667553785484,49.3184005119929,-215.376486525154));
#221389=CARTESIAN_POINT('Ctrl Pts',(42.7188997255464,49.3547228975728,-213.835548827928));
#221390=CARTESIAN_POINT('Ctrl Pts',(42.5029768685179,48.4845286599184,-216.606768911376));
#221391=CARTESIAN_POINT('Ctrl Pts',(42.6479264611755,49.3409861001092,-215.358258220572));
#221392=CARTESIAN_POINT('Ctrl Pts',(42.6349927775592,49.3703969686686,-213.837560447468));
#221393=CARTESIAN_POINT('Ctrl Pts',(42.3669756126708,48.5277324522344,-216.579923496877));
#221394=CARTESIAN_POINT('Ctrl Pts',(42.5335765527017,49.3626423449188,-215.340343539781));
#221395=CARTESIAN_POINT('Ctrl Pts',(42.5508500423968,49.3861157519262,-213.836818243375));
#221396=CARTESIAN_POINT('',(43.4427334535923,49.2193110042465,-213.753761106585));
#221397=CARTESIAN_POINT('',(43.7719279964152,48.0354975596111,-216.750009718968));
#221398=CARTESIAN_POINT('Origin',(42.506225613034,44.3085739513886,-213.666499074398));
#221399=CARTESIAN_POINT('Ctrl Pts',(42.4267736781731,48.508569392226,-216.591605848995));
#221400=CARTESIAN_POINT('Ctrl Pts',(42.5057689245607,48.4828880590072,-216.607095809672));
#221401=CARTESIAN_POINT('Ctrl Pts',(42.575038200036,48.4597022300457,-216.619925307791));
#221402=CARTESIAN_POINT('Ctrl Pts',(42.6601019032662,48.4307995702034,-216.635178861068));
#221403=CARTESIAN_POINT('Ctrl Pts',(42.6853248155618,48.4221459310976,-216.639598263176));
#221404=CARTESIAN_POINT('Ctrl Pts',(42.7180424554192,48.4108740731269,-216.645229692863));
#221405=CARTESIAN_POINT('Ctrl Pts',(42.733123554025,48.4056646763262,-216.647795989338));
#221406=CARTESIAN_POINT('Ctrl Pts',(42.7484073760464,48.4003773583356,-216.650353519746));
#221407=CARTESIAN_POINT('Ctrl Pts',(42.754455589884,48.3982847882281,-216.651356072319));
#221408=CARTESIAN_POINT('Ctrl Pts',(42.75837545544,48.396928711148,-216.652003655836));
#221409=CARTESIAN_POINT('Ctrl Pts',(42.758272534821,48.396964146891,-216.651987901739));
#221410=CARTESIAN_POINT('Ctrl Pts',(42.8237908566439,48.3743057303187,-216.662734627152));
#221411=CARTESIAN_POINT('Ctrl Pts',(42.883124963599,48.3536052295174,-216.671690111223));
#221412=CARTESIAN_POINT('Ctrl Pts',(42.9675591338409,48.324082926417,-216.683384715795));
#221413=CARTESIAN_POINT('Ctrl Pts',(42.9949458054802,48.3144969358278,-216.686993147063));
#221414=CARTESIAN_POINT('Ctrl Pts',(43.0479583477075,48.2959547366843,-216.693630469087));
#221415=CARTESIAN_POINT('Ctrl Pts',(43.0723486758755,48.2874289836569,-216.69652208628));
#221416=CARTESIAN_POINT('Ctrl Pts',(43.1499857554147,48.2603817225497,-216.705151268472));
#221417=CARTESIAN_POINT('Ctrl Pts',(43.2040029954931,48.2414864744923,-216.710625663544));
#221418=CARTESIAN_POINT('Ctrl Pts',(43.2882855452362,48.211708547662,-216.718419666566));
#221419=CARTESIAN_POINT('Ctrl Pts',(43.3312401528149,48.1964607001404,-216.722212270681));
#221420=CARTESIAN_POINT('Ctrl Pts',(43.3753820418788,48.1806472701165,-216.725848278702));
#221421=CARTESIAN_POINT('Ctrl Pts',(43.4050695940576,48.169976191394,-216.728237484917));
#221422=CARTESIAN_POINT('Ctrl Pts',(43.4180564137545,48.1652953793453,-216.729262098874));
#221423=CARTESIAN_POINT('Ctrl Pts',(43.5718487752363,48.10963028015,-216.741073640917));
#221424=CARTESIAN_POINT('Ctrl Pts',(43.6853875967172,48.0669209671252,-216.747552049762));
#221425=CARTESIAN_POINT('Ctrl Pts',(43.7719279964152,48.0354975596111,-216.750009718968));
#221426=CARTESIAN_POINT('Ctrl Pts',(43.4427334535923,49.2193110042462,-213.753761106585));
#221427=CARTESIAN_POINT('Ctrl Pts',(43.3719706400381,49.2325796186167,-213.766495780037));
#221428=CARTESIAN_POINT('Ctrl Pts',(43.3010945110738,49.2458572251103,-213.778020270751));
#221429=CARTESIAN_POINT('Ctrl Pts',(43.2300784559227,49.2591528525595,-213.788090955962));
#221430=CARTESIAN_POINT('Ctrl Pts',(43.1590933274703,49.2724426899114,-213.798157255503));
#221431=CARTESIAN_POINT('Ctrl Pts',(43.0879758381644,49.2857478720148,-213.806840936004));
#221432=CARTESIAN_POINT('Ctrl Pts',(43.0167173948743,49.2990711925071,-213.814054173643));
#221433=CARTESIAN_POINT('Ctrl Pts',(42.9454929340351,49.3123881592388,-213.821263971359));
#221434=CARTESIAN_POINT('Ctrl Pts',(42.8741286599837,49.3257228413477,-213.827017297049));
#221435=CARTESIAN_POINT('Ctrl Pts',(42.8025937883447,49.3390870721022,-213.830948922094));
#221436=CARTESIAN_POINT('Ctrl Pts',(42.731095982805,49.3524443781234,-213.83487850995));
#221437=CARTESIAN_POINT('Ctrl Pts',(42.6594242987748,49.3658330544367,-213.836920272795));
#221438=CARTESIAN_POINT('Ctrl Pts',(42.5875626890161,49.3792574634491,-213.836967828456));
#221439=CARTESIAN_POINT('Ctrl Pts',(47.064076521496,46.1934774086348,-216.786882195125));
#221440=CARTESIAN_POINT('Ctrl Pts',(47.7234387387225,47.4080545337851,-215.373546262479));
#221441=CARTESIAN_POINT('Ctrl Pts',(47.6028228022501,47.5293656571523,-213.40423171224));
#221442=CARTESIAN_POINT('Ctrl Pts',(46.9484052815617,46.2805028601163,-216.790124036479));
#221443=CARTESIAN_POINT('Ctrl Pts',(47.5766388725972,47.508813370891,-215.37845116732));
#221444=CARTESIAN_POINT('Ctrl Pts',(47.4422878419382,47.6357207591759,-213.413415509028));
#221445=CARTESIAN_POINT('Ctrl Pts',(46.8302467814474,46.3687247217733,-216.791504353852));
#221446=CARTESIAN_POINT('Ctrl Pts',(47.4263946384086,47.6067406666075,-215.382015347526));
#221447=CARTESIAN_POINT('Ctrl Pts',(47.2794655898102,47.7377048300804,-213.423678997697));
#221448=CARTESIAN_POINT('Ctrl Pts',(46.5987178641575,46.5304722851862,-216.79905959227));
#221449=CARTESIAN_POINT('Ctrl Pts',(47.129483939867,47.7906773992089,-215.393854083401));
#221450=CARTESIAN_POINT('Ctrl Pts',(46.9524663169082,47.931159795535,-213.446422385028));
#221451=CARTESIAN_POINT('Ctrl Pts',(46.4620556574027,46.6321591428633,-216.795250645318));
#221452=CARTESIAN_POINT('Ctrl Pts',(46.9655757003049,47.8868672070918,-215.393231131327));
#221453=CARTESIAN_POINT('Ctrl Pts',(46.7883227793212,48.0228296206497,-213.458567219471));
#221454=CARTESIAN_POINT('Ctrl Pts',(46.2017839218346,46.8104888208194,-216.792669267422));
#221455=CARTESIAN_POINT('Ctrl Pts',(46.6457795593283,48.0640235510291,-215.396870081809));
#221456=CARTESIAN_POINT('Ctrl Pts',(46.4554564500058,48.1980381642128,-213.483257157301));
#221457=CARTESIAN_POINT('Ctrl Pts',(46.0766700563314,46.8895585675527,-216.794042256812));
#221458=CARTESIAN_POINT('Ctrl Pts',(46.4887913192792,48.1462000233379,-215.401238442915));
#221459=CARTESIAN_POINT('Ctrl Pts',(46.2867982818209,48.281531361307,-213.496222696252));
#221460=CARTESIAN_POINT('Ctrl Pts',(45.87994004771,47.0109902272891,-216.794160241211));
#221461=CARTESIAN_POINT('Ctrl Pts',(46.2457858413235,48.2661200717717,-215.40646574203));
#221462=CARTESIAN_POINT('Ctrl Pts',(46.0305084677243,48.4005429744946,-213.516940454076));
#221463=CARTESIAN_POINT('Ctrl Pts',(45.8130083614259,47.0517196539655,-216.793924557511));
#221464=CARTESIAN_POINT('Ctrl Pts',(46.1636642989778,48.3054420800928,-215.408029222597));
#221465=CARTESIAN_POINT('Ctrl Pts',(45.9444636232077,48.4392026490444,-213.524043423009));
#221466=CARTESIAN_POINT('Ctrl Pts',(45.6738275139891,47.1362504084184,-216.791429029715));
#221467=CARTESIAN_POINT('Ctrl Pts',(45.9955390217945,48.3833415744636,-215.409524793596));
#221468=CARTESIAN_POINT('Ctrl Pts',(45.7716909901163,48.5142583186283,-213.538427044985));
#221469=CARTESIAN_POINT('Ctrl Pts',(45.6014941600616,47.1800522287631,-216.789086099185));
#221470=CARTESIAN_POINT('Ctrl Pts',(45.909487227893,48.4219032984012,-215.409390457658));
#221471=CARTESIAN_POINT('Ctrl Pts',(45.6849221753667,48.5506755813471,-213.545667919355));
#221472=CARTESIAN_POINT('Ctrl Pts',(45.3906864148211,47.3015955364168,-216.784924808343));
#221473=CARTESIAN_POINT('Ctrl Pts',(45.6556189845464,48.5320404250428,-215.41161214138));
#221474=CARTESIAN_POINT('Ctrl Pts',(45.4234990388784,48.656600479725,-213.567641621079));
#221475=CARTESIAN_POINT('Ctrl Pts',(45.2524205018182,47.3757252143881,-216.78361659133));
#221476=CARTESIAN_POINT('Ctrl Pts',(45.4876266651675,48.6001390907726,-215.414568111945));
#221477=CARTESIAN_POINT('Ctrl Pts',(45.2477531990456,48.72277066996,-213.582727977839));
#221478=CARTESIAN_POINT('Ctrl Pts',(44.9704029731687,47.5202017602144,-216.780193800645));
#221479=CARTESIAN_POINT('Ctrl Pts',(45.1474130999697,48.7286782833904,-215.420341153695));
#221480=CARTESIAN_POINT('Ctrl Pts',(44.8934628220207,48.8462330088366,-213.614222279602));
#221481=CARTESIAN_POINT('Ctrl Pts',(44.8252346194533,47.5917409614306,-216.777410227236));
#221482=CARTESIAN_POINT('Ctrl Pts',(44.9742728080524,48.7893969151401,-215.42260502614));
#221483=CARTESIAN_POINT('Ctrl Pts',(44.7149101065309,48.9035307364313,-213.630594481039));
#221484=CARTESIAN_POINT('Ctrl Pts',(44.5266344343995,47.7322552775795,-216.769106033588));
#221485=CARTESIAN_POINT('Ctrl Pts',(44.6220976077485,48.9031595903168,-215.425477584854));
#221486=CARTESIAN_POINT('Ctrl Pts',(44.3548749879417,49.0092996064572,-213.664137638348));
#221487=CARTESIAN_POINT('Ctrl Pts',(44.3737726429906,47.8005581457219,-216.763841197291));
#221488=CARTESIAN_POINT('Ctrl Pts',(44.4434408439288,48.9560287134227,-215.426312574315));
#221489=CARTESIAN_POINT('Ctrl Pts',(44.1732412416258,49.0577948170598,-213.681295718708));
#221490=CARTESIAN_POINT('Ctrl Pts',(44.0708469448104,47.925010686338,-216.756464337538));
#221491=CARTESIAN_POINT('Ctrl Pts',(44.0869468343345,49.052302299606,-215.431212914185));
#221492=CARTESIAN_POINT('Ctrl Pts',(43.8055081380661,49.1462823788298,-213.716921533579));
#221493=CARTESIAN_POINT('Ctrl Pts',(43.9199928553144,47.9817986673754,-216.754308697682));
#221494=CARTESIAN_POINT('Ctrl Pts',(43.9084710831663,49.0958794298658,-215.435250774665));
#221495=CARTESIAN_POINT('Ctrl Pts',(43.6192098223546,49.1861560840058,-213.735550650933));
#221496=CARTESIAN_POINT('Ctrl Pts',(43.7631348840936,48.0386758038654,-216.749772686363));
#221497=CARTESIAN_POINT('Ctrl Pts',(43.7261216974267,49.135628774228,-215.437783134142));
#221498=CARTESIAN_POINT('Ctrl Pts',(43.4322454110891,49.2212868218137,-213.754842699038));
#221499=CARTESIAN_POINT('',(47.5938143592265,47.5353276146283,-213.404748058676));
#221500=CARTESIAN_POINT('',(47.0575921287078,46.1983743823903,-216.787046295788));
#221501=CARTESIAN_POINT('Origin',(44.8332438581234,43.3673981711062,-213.31748602649));
#221502=CARTESIAN_POINT('Ctrl Pts',(43.7719279964153,48.0354975596113,-216.750009718968));
#221503=CARTESIAN_POINT('Ctrl Pts',(43.7999682355946,48.025315958121,-216.750806036441));
#221504=CARTESIAN_POINT('Ctrl Pts',(43.8324552729532,48.0134635334545,-216.75163878995));
#221505=CARTESIAN_POINT('Ctrl Pts',(43.869389236841,47.9997974421566,-216.752507979496));
#221506=CARTESIAN_POINT('Ctrl Pts',(43.887856218785,47.9929643965077,-216.752942574269));
#221507=CARTESIAN_POINT('Ctrl Pts',(43.907434250537,47.9856775685499,-216.753386278009));
#221508=CARTESIAN_POINT('Ctrl Pts',(43.9281174324963,47.9779175176578,-216.753839100978));
#221509=CARTESIAN_POINT('Ctrl Pts',(43.9384590234759,47.9740374922117,-216.754065512463));
#221510=CARTESIAN_POINT('Ctrl Pts',(43.9490768944605,47.9700391399423,-216.75429418598));
#221511=CARTESIAN_POINT('Ctrl Pts',(43.9599697070893,47.9659199939512,-216.754525143987));
#221512=CARTESIAN_POINT('Ctrl Pts',(43.9654161134037,47.9638604209556,-216.75464062299));
#221513=CARTESIAN_POINT('Ctrl Pts',(43.970931254658,47.9617706482002,-216.754756671998));
#221514=CARTESIAN_POINT('Ctrl Pts',(43.9765149348169,47.9596503652226,-216.754873291075));
#221515=CARTESIAN_POINT('Ctrl Pts',(43.9820986149759,47.957530082245,-216.754989910151));
#221516=CARTESIAN_POINT('Ctrl Pts',(43.986323611751,47.95592358258,-216.755077719017));
#221517=CARTESIAN_POINT('Ctrl Pts',(43.9934713819637,47.9531976722309,-216.755224856242));
#221518=CARTESIAN_POINT('Ctrl Pts',(44.0285940305662,47.9398031186203,-216.755947857807));
#221519=CARTESIAN_POINT('Ctrl Pts',(44.0598368421922,47.9276795028024,-216.756596414032));
#221520=CARTESIAN_POINT('Ctrl Pts',(44.0871926282956,47.916949837956,-216.757170524919));
#221521=CARTESIAN_POINT('Ctrl Pts',(44.1043740011675,47.9102108478271,-216.757531107254));
#221522=CARTESIAN_POINT('Ctrl Pts',(44.1200230264987,47.9040208116318,-216.757862322909));
#221523=CARTESIAN_POINT('Ctrl Pts',(44.1341440632014,47.8984021424213,-216.758164171885));
#221524=CARTESIAN_POINT('Ctrl Pts',(44.1524461762284,47.8911198499724,-216.758555394866));
#221525=CARTESIAN_POINT('Ctrl Pts',(44.1681816696013,47.8847977496136,-216.758897286368));
#221526=CARTESIAN_POINT('Ctrl Pts',(44.1813646140109,47.8794715426646,-216.75918984639));
#221527=CARTESIAN_POINT('Ctrl Pts',(44.1879560862157,47.8768084391901,-216.759336126401));
#221528=CARTESIAN_POINT('Ctrl Pts',(44.1939094622523,47.8743940914731,-216.759470073542));
#221529=CARTESIAN_POINT('Ctrl Pts',(44.1992265052247,47.8722317355578,-216.759591691156));
#221530=CARTESIAN_POINT('Ctrl Pts',(44.2018850267109,47.8711505576002,-216.759652499962));
#221531=CARTESIAN_POINT('Ctrl Pts',(44.204384462322,47.8701323708537,-216.759710220538));
#221532=CARTESIAN_POINT('Ctrl Pts',(44.2067250158902,47.8691775029316,-216.759764860289));
#221533=CARTESIAN_POINT('Ctrl Pts',(44.2078952926744,47.8687000689706,-216.759792180164));
#221534=CARTESIAN_POINT('Ctrl Pts',(44.2090258474261,47.8682384623275,-216.759818729464));
#221535=CARTESIAN_POINT('Ctrl Pts',(44.2100969163324,47.8678007420343,-216.759844122804));
#221536=CARTESIAN_POINT('Ctrl Pts',(44.2111679852387,47.8673630217411,-216.759869516143));
#221537=CARTESIAN_POINT('Ctrl Pts',(44.2122192840712,47.8669333446112,-216.75989452408));
#221538=CARTESIAN_POINT('Ctrl Pts',(44.2144806688504,47.8660075143691,-216.759948709947));
#221539=CARTESIAN_POINT('Ctrl Pts',(44.2449761228487,47.8535224150545,-216.760679422656));
#221540=CARTESIAN_POINT('Ctrl Pts',(44.2755711243667,47.8408061684401,-216.761443377949));
#221541=CARTESIAN_POINT('Ctrl Pts',(44.3061404540436,47.8279027716419,-216.762238392159));
#221542=CARTESIAN_POINT('Ctrl Pts',(44.3481107408968,47.8101869999606,-216.763329910186));
#221543=CARTESIAN_POINT('Ctrl Pts',(44.3900317972361,47.7921181966764,-216.764479974366));
#221544=CARTESIAN_POINT('Ctrl Pts',(44.4317077200863,47.7737754898824,-216.765682933317));
#221545=CARTESIAN_POINT('Ctrl Pts',(44.4677231453878,47.7579241219657,-216.766722504256));
#221546=CARTESIAN_POINT('Ctrl Pts',(44.5035561515456,47.7418688288015,-216.767801577222));
#221547=CARTESIAN_POINT('Ctrl Pts',(44.5392322306382,47.7255991325106,-216.768920152147));
#221548=CARTESIAN_POINT('Ctrl Pts',(44.5570702701845,47.7174642843651,-216.76947943961));
#221549=CARTESIAN_POINT('Ctrl Pts',(44.5748690780222,47.7092758355722,-216.770048602683));
#221550=CARTESIAN_POINT('Ctrl Pts',(44.5926318406004,47.7010324781867,-216.770627641213));
#221551=CARTESIAN_POINT('Ctrl Pts',(44.605953912534,47.6948499601476,-216.77106192011));
#221552=CARTESIAN_POINT('Ctrl Pts',(44.6192557090139,47.6886365560366,-216.771501753962));
#221553=CARTESIAN_POINT('Ctrl Pts',(44.6325385743512,47.6823917143765,-216.771947142795));
#221554=CARTESIAN_POINT('Ctrl Pts',(44.6369661961303,47.6803101004898,-216.772095605739));
#221555=CARTESIAN_POINT('Ctrl Pts',(44.6432770207651,47.6773348113996,-216.772308487795));
#221556=CARTESIAN_POINT('Ctrl Pts',(44.6458151790926,47.6761363731342,-216.772394383283));
#221557=CARTESIAN_POINT('Ctrl Pts',(44.667735113507,47.6657864718322,-216.773136190224));
#221558=CARTESIAN_POINT('Ctrl Pts',(44.6940783900531,47.6533905421585,-216.773881695209));
#221559=CARTESIAN_POINT('Ctrl Pts',(44.7248101335922,47.6388298667565,-216.774630898238));
#221560=CARTESIAN_POINT('Ctrl Pts',(44.7510143492991,47.6264143304045,-216.775269725571));
#221561=CARTESIAN_POINT('Ctrl Pts',(44.7804087087902,47.6124243901338,-216.775911241589));
#221562=CARTESIAN_POINT('Ctrl Pts',(44.8129802196091,47.5967576098995,-216.776555446292));
#221563=CARTESIAN_POINT('Ctrl Pts',(44.8483655605272,47.5797373874492,-216.777255303391));
#221564=CARTESIAN_POINT('Ctrl Pts',(44.8874993594066,47.5607390605947,-216.777958333788));
#221565=CARTESIAN_POINT('Ctrl Pts',(44.9303902108242,47.5395897055685,-216.778664537483));
#221566=CARTESIAN_POINT('Ctrl Pts',(44.951835636533,47.5290150280554,-216.77901763933));
#221567=CARTESIAN_POINT('Ctrl Pts',(44.9742208346179,47.517901876086,-216.779371534503));
#221568=CARTESIAN_POINT('Ctrl Pts',(44.9975507822766,47.5062239777693,-216.779726222999));
#221569=CARTESIAN_POINT('Ctrl Pts',(44.9983644784359,47.5058166789126,-216.779738593737));
#221570=CARTESIAN_POINT('Ctrl Pts',(44.9991793241654,47.5054086927271,-216.77975096544));
#221571=CARTESIAN_POINT('Ctrl Pts',(44.9999953197465,47.5050000180245,-216.779763338108));
#221572=CARTESIAN_POINT('Ctrl Pts',(45.0108772620136,47.4995500197372,-216.77992833736));
#221573=CARTESIAN_POINT('Ctrl Pts',(45.0219637216991,47.4939775693251,-216.78009350826));
#221574=CARTESIAN_POINT('Ctrl Pts',(45.0332532520402,47.4882807840264,-216.780258851139));
#221575=CARTESIAN_POINT('Ctrl Pts',(45.0393212967433,47.4852188012147,-216.780347721796));
#221576=CARTESIAN_POINT('Ctrl Pts',(45.0454480117016,47.4821208957931,-216.780436641231));
#221577=CARTESIAN_POINT('Ctrl Pts',(45.0516331238869,47.4789867866292,-216.780525610852));
#221578=CARTESIAN_POINT('Ctrl Pts',(45.0578182360722,47.4758526774653,-216.780614580473));
#221579=CARTESIAN_POINT('Ctrl Pts',(45.062340348357,47.4735583574169,-216.780679268952));
#221580=CARTESIAN_POINT('Ctrl Pts',(45.0703633822198,47.469475560477,-216.780792668464));
#221581=CARTESIAN_POINT('Ctrl Pts',(45.1106116695992,47.4489938340672,-216.781361547544));
#221582=CARTESIAN_POINT('Ctrl Pts',(45.1479437072911,47.4296838782679,-216.781890800055));
#221583=CARTESIAN_POINT('Ctrl Pts',(45.1823388278365,47.4116798480988,-216.782380425997));
#221584=CARTESIAN_POINT('Ctrl Pts',(45.2210852171756,47.391398158384,-216.782931993692));
#221585=CARTESIAN_POINT('Ctrl Pts',(45.2561053197537,47.3727738991893,-216.783433274439));
#221586=CARTESIAN_POINT('Ctrl Pts',(45.2874192254577,47.3559454252637,-216.783884268239));
#221587=CARTESIAN_POINT('Ctrl Pts',(45.3169652113322,47.3400670529649,-216.78430979984));
#221588=CARTESIAN_POINT('Ctrl Pts',(45.3432132151396,47.3257864069596,-216.784690562402));
#221589=CARTESIAN_POINT('Ctrl Pts',(45.3662022526885,47.3131837743999,-216.785026555925));
#221590=CARTESIAN_POINT('Ctrl Pts',(45.3945609497833,47.297637484626,-216.785441029064));
#221591=CARTESIAN_POINT('Ctrl Pts',(45.4179621298102,47.284645416901,-216.785787376854));
#221592=CARTESIAN_POINT('Ctrl Pts',(45.4364877857767,47.2743030919902,-216.786065599295));
#221593=CARTESIAN_POINT('Ctrl Pts',(45.4404938146909,47.2720666447244,-216.786125762733));
#221594=CARTESIAN_POINT('Ctrl Pts',(45.4442718252743,47.2699539101085,-216.786182740581));
#221595=CARTESIAN_POINT('Ctrl Pts',(45.4478225530286,47.2679655548132,-216.786236532841));
#221596=CARTESIAN_POINT('Ctrl Pts',(45.4578079875536,47.2623738584096,-216.786387808615));
#221597=CARTESIAN_POINT('Ctrl Pts',(45.4659962721697,47.2577662199214,-216.786513890861));
#221598=CARTESIAN_POINT('Ctrl Pts',(45.4724009492202,47.2541536209048,-216.786614810403));
#221599=CARTESIAN_POINT('Ctrl Pts',(45.4756032877455,47.2523473213965,-216.786665270174));
#221600=CARTESIAN_POINT('Ctrl Pts',(45.4783596950982,47.2507897283842,-216.786709385351));
#221601=CARTESIAN_POINT('Ctrl Pts',(45.4806713295795,47.2494816957264,-216.786747224623));
#221602=CARTESIAN_POINT('Ctrl Pts',(45.4818271468202,47.2488276793975,-216.78676614426));
#221603=CARTESIAN_POINT('Ctrl Pts',(45.482871769002,47.2482360497932,-216.786783491525));
#221604=CARTESIAN_POINT('Ctrl Pts',(45.4838053126926,47.2477068917666,-216.786799265584));
#221605=CARTESIAN_POINT('Ctrl Pts',(45.4842720845379,47.2474423127533,-216.786807152614));
#221606=CARTESIAN_POINT('Ctrl Pts',(45.4847110860037,47.2471933509791,-216.786814646129));
#221607=CARTESIAN_POINT('Ctrl Pts',(45.4851084672805,47.2469678398215,-216.786821549312));
#221608=CARTESIAN_POINT('Ctrl Pts',(45.4855058485574,47.2467423286638,-216.786828452496));
#221609=CARTESIAN_POINT('Ctrl Pts',(45.4858895864854,47.2465247922921,-216.786835158855));
#221610=CARTESIAN_POINT('Ctrl Pts',(45.4879940552358,47.2453288536159,-216.78687250758));
#221611=CARTESIAN_POINT('Ctrl Pts',(45.5247478018735,47.2244422393148,-216.787524788859));
#221612=CARTESIAN_POINT('Ctrl Pts',(45.5620119202703,47.2028903192636,-216.788266723893));
#221613=CARTESIAN_POINT('Ctrl Pts',(45.5989423960054,47.1811378446028,-216.789080931354));
#221614=CARTESIAN_POINT('Ctrl Pts',(45.6258353862223,47.165297564276,-216.789673842029));
#221615=CARTESIAN_POINT('Ctrl Pts',(45.6525518901226,47.1493516911605,-216.790305077603));
#221616=CARTESIAN_POINT('Ctrl Pts',(45.6787817315062,47.1334878263734,-216.790967926176));
#221617=CARTESIAN_POINT('Ctrl Pts',(45.6825303096061,47.1312206782328,-216.791062655672));
#221618=CARTESIAN_POINT('Ctrl Pts',(45.6862689755748,47.1289552138267,-216.791158030833));
#221619=CARTESIAN_POINT('Ctrl Pts',(45.6899967965639,47.1266920637689,-216.791254032068));
#221620=CARTESIAN_POINT('Ctrl Pts',(45.7228131866165,47.1067693219689,-216.792099140777));
#221621=CARTESIAN_POINT('Ctrl Pts',(45.7561216578679,47.0864990412011,-216.792755263244));
#221622=CARTESIAN_POINT('Ctrl Pts',(45.7898044813981,47.065949222955,-216.793222399469));
#221623=CARTESIAN_POINT('Ctrl Pts',(45.8066458931633,47.0556743138319,-216.793455967582));
#221624=CARTESIAN_POINT('Ctrl Pts',(45.8235805995987,47.0453297617529,-216.793642289121));
#221625=CARTESIAN_POINT('Ctrl Pts',(45.8405920420434,47.0349255859399,-216.793781363054));
#221626=CARTESIAN_POINT('Ctrl Pts',(45.8490977632657,47.0297234980334,-216.79385090002));
#221627=CARTESIAN_POINT('Ctrl Pts',(45.8576226695517,47.0245065059502,-216.793908626949));
#221628=CARTESIAN_POINT('Ctrl Pts',(45.8661645460346,47.0192759789475,-216.793954541448));
#221629=CARTESIAN_POINT('Ctrl Pts',(45.870435484276,47.0166607154462,-216.793977498697));
#221630=CARTESIAN_POINT('Ctrl Pts',(45.8747106651369,47.0140420683319,-216.793997502963));
#221631=CARTESIAN_POINT('Ctrl Pts',(45.8789898076483,47.0114202126398,-216.79401455427));
#221632=CARTESIAN_POINT('Ctrl Pts',(45.8811293789039,47.0101092847938,-216.794023079923));
#221633=CARTESIAN_POINT('Ctrl Pts',(45.8832699405766,47.0087975548103,-216.794030867345));
#221634=CARTESIAN_POINT('Ctrl Pts',(45.8854114570194,47.0074850449998,-216.794037916534));
#221635=CARTESIAN_POINT('Ctrl Pts',(45.8875529734622,47.0061725351893,-216.794044965722));
#221636=CARTESIAN_POINT('Ctrl Pts',(45.8907066610453,47.0042392997017,-216.794053905808));
#221637=CARTESIAN_POINT('Ctrl Pts',(45.8918388348603,47.0035451985448,-216.794056849418));
#221638=CARTESIAN_POINT('Ctrl Pts',(45.9017349656741,46.9974781832549,-216.794082578986));
#221639=CARTESIAN_POINT('Ctrl Pts',(45.9140558641918,46.9899297596758,-216.794091079011));
#221640=CARTESIAN_POINT('Ctrl Pts',(45.9287146500497,46.9809163219443,-216.794082349493));
#221641=CARTESIAN_POINT('Ctrl Pts',(45.9408886437017,46.9734307406152,-216.794075099704));
#221642=CARTESIAN_POINT('Ctrl Pts',(45.9546746901182,46.9649346626169,-216.794055966429));
#221643=CARTESIAN_POINT('Ctrl Pts',(45.9699974444731,46.9554476628383,-216.794024949666));
#221644=CARTESIAN_POINT('Ctrl Pts',(45.9868839363196,46.9449924835213,-216.793990767541));
#221645=CARTESIAN_POINT('Ctrl Pts',(46.0056380469337,46.9333329342966,-216.793942152665));
#221646=CARTESIAN_POINT('Ctrl Pts',(46.026117443191,46.9205161485541,-216.793879105039));
#221647=CARTESIAN_POINT('Ctrl Pts',(46.0363571413196,46.9141077556829,-216.793847581226));
#221648=CARTESIAN_POINT('Ctrl Pts',(46.0470274212995,46.9074104503921,-216.793812449226));
#221649=CARTESIAN_POINT('Ctrl Pts',(46.0581055216702,46.9004329827126,-216.793773709038));
#221650=CARTESIAN_POINT('Ctrl Pts',(46.0655876516163,46.8957204130368,-216.793747543982));
#221651=CARTESIAN_POINT('Ctrl Pts',(46.0738521325161,46.890503370826,-216.793717443146));
#221652=CARTESIAN_POINT('Ctrl Pts',(46.0816805652799,46.8855491135382,-216.79368804623));
#221653=CARTESIAN_POINT('Ctrl Pts',(46.0854429715589,46.8831680585699,-216.793673917841));
#221654=CARTESIAN_POINT('Ctrl Pts',(46.0891054119841,46.8808474685615,-216.793659952046));
#221655=CARTESIAN_POINT('Ctrl Pts',(46.0925367545552,46.8786711564055,-216.793646663912));
#221656=CARTESIAN_POINT('Ctrl Pts',(46.1249973118812,46.8580832075096,-216.79352095794));
#221657=CARTESIAN_POINT('Ctrl Pts',(46.1545286634281,46.8390961398004,-216.79344153441));
#221658=CARTESIAN_POINT('Ctrl Pts',(46.1813384366676,46.8216767497614,-216.793408393323));
#221659=CARTESIAN_POINT('Ctrl Pts',(46.1894515732713,46.8164053179713,-216.793398364213));
#221660=CARTESIAN_POINT('Ctrl Pts',(46.1973156706764,46.8112771226396,-216.793392573558));
#221661=CARTESIAN_POINT('Ctrl Pts',(46.2049368905182,46.8062904844855,-216.793391021358));
#221662=CARTESIAN_POINT('Ctrl Pts',(46.2213396202164,46.7955580191531,-216.793387680643));
#221663=CARTESIAN_POINT('Ctrl Pts',(46.2366172731346,46.7854815518693,-216.793403973138));
#221664=CARTESIAN_POINT('Ctrl Pts',(46.2508323842425,46.7760404634134,-216.793439914088));
#221665=CARTESIAN_POINT('Ctrl Pts',(46.2579399397965,46.7713199191855,-216.793457884563));
#221666=CARTESIAN_POINT('Ctrl Pts',(46.2647818439802,46.7667581956347,-216.793480740381));
#221667=CARTESIAN_POINT('Ctrl Pts',(46.2713659264824,46.7623523087817,-216.793508515375));
#221668=CARTESIAN_POINT('Ctrl Pts',(46.2746579677335,46.7601493653551,-216.793522402872));
#221669=CARTESIAN_POINT('Ctrl Pts',(46.2778855526769,46.7579853797555,-216.793537518667));
#221670=CARTESIAN_POINT('Ctrl Pts',(46.2810496433213,46.7558599741858,-216.793553862528));
#221671=CARTESIAN_POINT('Ctrl Pts',(46.2815161385684,46.755546616666,-216.793556272173));
#221672=CARTESIAN_POINT('Ctrl Pts',(46.2819516748022,46.7552540000806,-216.79355852675));
#221673=CARTESIAN_POINT('Ctrl Pts',(46.2823694031142,46.7549732901716,-216.793560706644));
#221674=CARTESIAN_POINT('Ctrl Pts',(46.2845577700535,46.7535027260118,-216.793572126526));
#221675=CARTESIAN_POINT('Ctrl Pts',(46.2862606393729,46.7523574370574,-216.793581496779));
#221676=CARTESIAN_POINT('Ctrl Pts',(46.2893451131554,46.75027822677,-216.793600374501));
#221677=CARTESIAN_POINT('Ctrl Pts',(46.2896653831733,46.7500623362282,-216.793602334631));
#221678=CARTESIAN_POINT('Ctrl Pts',(46.2900005062908,46.7498363964486,-216.793604397263));
#221679=CARTESIAN_POINT('Ctrl Pts',(46.2903525372648,46.7495990142202,-216.793606575336));
#221680=CARTESIAN_POINT('Ctrl Pts',(46.3125906116356,46.7346033915579,-216.793744165901));
#221681=CARTESIAN_POINT('Ctrl Pts',(46.3339221814183,46.7199958452874,-216.793972420847));
#221682=CARTESIAN_POINT('Ctrl Pts',(46.3546813907234,46.7056150358813,-216.794248529204));
#221683=CARTESIAN_POINT('Ctrl Pts',(46.3762392929501,46.6906809370646,-216.794535260595));
#221684=CARTESIAN_POINT('Ctrl Pts',(46.3971796363455,46.6759914456177,-216.794873598471));
#221685=CARTESIAN_POINT('Ctrl Pts',(46.4178247858721,46.6613900474904,-216.795215597964));
#221686=CARTESIAN_POINT('Ctrl Pts',(46.4397055789028,46.6459147335447,-216.795578066646));
#221687=CARTESIAN_POINT('Ctrl Pts',(46.4612546635803,46.630538341508,-216.795944648367));
#221688=CARTESIAN_POINT('Ctrl Pts',(46.4828018122461,46.6151008458368,-216.796258264017));
#221689=CARTESIAN_POINT('Ctrl Pts',(46.5052220656438,46.5990378126186,-216.796584587581));
#221690=CARTESIAN_POINT('Ctrl Pts',(46.5276398302866,46.5829086656922,-216.796853565667));
#221691=CARTESIAN_POINT('Ctrl Pts',(46.5503739020283,46.566560657057,-216.797000895555));
#221692=CARTESIAN_POINT('Ctrl Pts',(46.5760029895584,46.5481308505086,-216.797166986814));
#221693=CARTESIAN_POINT('Ctrl Pts',(46.602033725843,46.529422623157,-216.797178475217));
#221694=CARTESIAN_POINT('Ctrl Pts',(46.628861222937,46.5102540599383,-216.79694323161));
#221695=CARTESIAN_POINT('Ctrl Pts',(46.6442602233249,46.4992512924642,-216.796808201629));
#221696=CARTESIAN_POINT('Ctrl Pts',(46.6599206127002,46.4880975557103,-216.796591879193));
#221697=CARTESIAN_POINT('Ctrl Pts',(46.6759114459435,46.4767631089541,-216.796276840848));
#221698=CARTESIAN_POINT('Ctrl Pts',(46.6906059672228,46.4663474998038,-216.795987341383));
#221699=CARTESIAN_POINT('Ctrl Pts',(46.7050820297943,46.4560666092541,-216.795679810554));
#221700=CARTESIAN_POINT('Ctrl Pts',(46.7193659094848,46.4459104620005,-216.795354248359));
#221701=CARTESIAN_POINT('Ctrl Pts',(46.7382039925211,46.4325161777138,-216.794924885483));
#221702=CARTESIAN_POINT('Ctrl Pts',(46.7567078125574,46.4193388589338,-216.794464160181));
#221703=CARTESIAN_POINT('Ctrl Pts',(46.7749052518499,46.4063621036006,-216.793972072453));
#221704=CARTESIAN_POINT('Ctrl Pts',(46.7909030289276,46.3949539468994,-216.793539467093));
#221705=CARTESIAN_POINT('Ctrl Pts',(46.8066640171603,46.3837007972895,-216.793082623085));
#221706=CARTESIAN_POINT('Ctrl Pts',(46.8222071071304,46.3725915476252,-216.792601540443));
#221707=CARTESIAN_POINT('Ctrl Pts',(46.8299786521155,46.367036922793,-216.792360999121));
#221708=CARTESIAN_POINT('Ctrl Pts',(46.8376957225221,46.3615182729302,-216.792114398121));
#221709=CARTESIAN_POINT('Ctrl Pts',(46.8453606733607,46.3560342140465,-216.791861737467));
#221710=CARTESIAN_POINT('Ctrl Pts',(46.8511093864896,46.3519211698836,-216.791672241976));
#221711=CARTESIAN_POINT('Ctrl Pts',(46.8568287823605,46.3478275831453,-216.791479337929));
#221712=CARTESIAN_POINT('Ctrl Pts',(46.8625198537008,46.3437528704933,-216.79128302532));
#221713=CARTESIAN_POINT('Ctrl Pts',(46.8641769268255,46.3425664336306,-216.791225864844));
#221714=CARTESIAN_POINT('Ctrl Pts',(46.8672064496826,46.3403971424021,-216.791120311155));
#221715=CARTESIAN_POINT('Ctrl Pts',(46.8680054423642,46.3398248670299,-216.791092423137));
#221716=CARTESIAN_POINT('Ctrl Pts',(46.8681211396226,46.3397419993226,-216.791088384843));
#221717=CARTESIAN_POINT('Ctrl Pts',(46.8681901367227,46.3396925799012,-216.791085975056));
#221718=CARTESIAN_POINT('Ctrl Pts',(46.868201520183,46.3396844276801,-216.791085576526));
#221719=CARTESIAN_POINT('Ctrl Pts',(46.8685685936507,46.3394215494343,-216.791072725425));
#221720=CARTESIAN_POINT('Ctrl Pts',(46.8709671673915,46.3376639117433,-216.791022665875));
#221721=CARTESIAN_POINT('Ctrl Pts',(46.875368288887,46.334427330707,-216.790935397876));
#221722=CARTESIAN_POINT('Ctrl Pts',(46.8795994466559,46.331315740852,-216.790851500016));
#221723=CARTESIAN_POINT('Ctrl Pts',(46.8856808427705,46.326837585854,-216.790733212068));
#221724=CARTESIAN_POINT('Ctrl Pts',(46.8935467207944,46.3210286787986,-216.790580534032));
#221725=CARTESIAN_POINT('Ctrl Pts',(46.90157058323,46.3151031011362,-216.790424789491));
#221726=CARTESIAN_POINT('Ctrl Pts',(46.9114507502922,46.3077931236649,-216.790233259554));
#221727=CARTESIAN_POINT('Ctrl Pts',(46.9230833813073,46.2991549282109,-216.790005944221));
#221728=CARTESIAN_POINT('Ctrl Pts',(46.9288996968149,46.2948358304839,-216.789892286554));
#221729=CARTESIAN_POINT('Ctrl Pts',(46.9351536534424,46.2901849284473,-216.789769682536));
#221730=CARTESIAN_POINT('Ctrl Pts',(46.9418300414805,46.285210383585,-216.789638133061));
#221731=CARTESIAN_POINT('Ctrl Pts',(46.9451682354996,46.2827231111539,-216.789572358324));
#221732=CARTESIAN_POINT('Ctrl Pts',(46.9486120361007,46.2801549263655,-216.789504345222));
#221733=CARTESIAN_POINT('Ctrl Pts',(46.9521594324836,46.2775069041238,-216.789434096866));
#221734=CARTESIAN_POINT('Ctrl Pts',(46.9550814801921,46.2753256854247,-216.789376232159));
#221735=CARTESIAN_POINT('Ctrl Pts',(46.9589745467844,46.2724170025407,-216.789298950658));
#221736=CARTESIAN_POINT('Ctrl Pts',(46.9616112445893,46.2704454910704,-216.789246484071));
#221737=CARTESIAN_POINT('Ctrl Pts',(46.9621755254093,46.2700235670612,-216.789235255674));
#221738=CARTESIAN_POINT('Ctrl Pts',(46.9626824488577,46.2696444664173,-216.789225163812));
#221739=CARTESIAN_POINT('Ctrl Pts',(46.9631104211035,46.2693243772486,-216.789216642034));
#221740=CARTESIAN_POINT('Ctrl Pts',(46.980514184376,46.2563077478473,-216.788870098506));
#221741=CARTESIAN_POINT('Ctrl Pts',(46.9963445219175,46.2444288905238,-216.788533594325));
#221742=CARTESIAN_POINT('Ctrl Pts',(47.0107402837605,46.2336120791181,-216.788207129489));
#221743=CARTESIAN_POINT('Ctrl Pts',(47.0261770769916,46.2220130485903,-216.787857056307));
#221744=CARTESIAN_POINT('Ctrl Pts',(47.0399639945659,46.2116354196435,-216.787518526964));
#221745=CARTESIAN_POINT('Ctrl Pts',(47.0522206527176,46.2024148717456,-216.787191541462));
#221746=CARTESIAN_POINT('Ctrl Pts',(47.0540450260366,46.2010424159454,-216.787142870477));
#221747=CARTESIAN_POINT('Ctrl Pts',(47.0558354138571,46.19969564163,-216.787094455252));
#221748=CARTESIAN_POINT('Ctrl Pts',(47.0575921287077,46.1983743823902,-216.787046295788));
#221749=CARTESIAN_POINT('Ctrl Pts',(47.5938143592254,47.5353276146289,-213.404748058676));
#221750=CARTESIAN_POINT('Ctrl Pts',(47.4864021701981,47.6063414465537,-213.410916600681));
#221751=CARTESIAN_POINT('Ctrl Pts',(47.3727955180169,47.6788238138538,-213.41786320449));
#221752=CARTESIAN_POINT('Ctrl Pts',(47.2527927928078,47.7521475639727,-213.425781542233));
#221753=CARTESIAN_POINT('Ctrl Pts',(47.2075811278853,47.7797726767813,-213.428764818089));
#221754=CARTESIAN_POINT('Ctrl Pts',(47.161461484639,47.8075168510272,-213.431886395367));
#221755=CARTESIAN_POINT('Ctrl Pts',(47.1144227976596,47.8353452540809,-213.435158020616));
#221756=CARTESIAN_POINT('Ctrl Pts',(47.0214662420634,47.8903389765197,-213.441623316181));
#221757=CARTESIAN_POINT('Ctrl Pts',(46.9249056173264,47.945674409168,-213.448583307771));
#221758=CARTESIAN_POINT('Ctrl Pts',(46.8246139149985,48.0010896024748,-213.455937351587));
#221759=CARTESIAN_POINT('Ctrl Pts',(46.7880174307094,48.0213106297797,-213.458620845263));
#221760=CARTESIAN_POINT('Ctrl Pts',(46.7509240118438,48.0415422237553,-213.461356338266));
#221761=CARTESIAN_POINT('Ctrl Pts',(46.7133270224978,48.0617714853602,-213.464137256222));
#221762=CARTESIAN_POINT('Ctrl Pts',(46.6831717520134,48.0779966902505,-213.466367736232));
#221763=CARTESIAN_POINT('Ctrl Pts',(46.6526943629849,48.0942192315053,-213.468635888902));
#221764=CARTESIAN_POINT('Ctrl Pts',(46.6218917752265,48.110432305252,-213.470934821448));
#221765=CARTESIAN_POINT('Ctrl Pts',(46.4984211243293,48.1754216101847,-213.480149978956));
#221766=CARTESIAN_POINT('Ctrl Pts',(46.3697617304992,48.2402352763643,-213.490086744041));
#221767=CARTESIAN_POINT('Ctrl Pts',(46.2357652584914,48.304370847364,-213.500726997951));
#221768=CARTESIAN_POINT('Ctrl Pts',(46.219639872116,48.3120890420842,-213.502007466032));
#221769=CARTESIAN_POINT('Ctrl Pts',(46.2034371774102,48.3197973951656,-213.503298178144));
#221770=CARTESIAN_POINT('Ctrl Pts',(46.1871569030505,48.327495013277,-213.504599149635));
#221771=CARTESIAN_POINT('Ctrl Pts',(46.1635870781003,48.3386392672011,-213.506482635727));
#221772=CARTESIAN_POINT('Ctrl Pts',(46.1398591423213,48.3497589583645,-213.508384553586));
#221773=CARTESIAN_POINT('Ctrl Pts',(46.1159688146372,48.3608529964996,-213.510307882609));
#221774=CARTESIAN_POINT('Ctrl Pts',(46.0459424972984,48.393371371521,-213.515945463234));
#221775=CARTESIAN_POINT('Ctrl Pts',(45.9744755547282,48.4256892487927,-213.521758156206));
#221776=CARTESIAN_POINT('Ctrl Pts',(45.9016170264935,48.4577050961598,-213.527740501239));
#221777=CARTESIAN_POINT('Ctrl Pts',(45.8871630536565,48.4640565309117,-213.528927303315));
#221778=CARTESIAN_POINT('Ctrl Pts',(45.8726527968879,48.470396704033,-213.530121292051));
#221779=CARTESIAN_POINT('Ctrl Pts',(45.8580875854649,48.4767243421701,-213.531322368788));
#221780=CARTESIAN_POINT('Ctrl Pts',(45.8234192369333,48.4917854873846,-213.534181190795));
#221781=CARTESIAN_POINT('Ctrl Pts',(45.7884329611125,48.5067790279182,-213.537073745386));
#221782=CARTESIAN_POINT('Ctrl Pts',(45.7531297470218,48.5216957329351,-213.540007556183));
#221783=CARTESIAN_POINT('Ctrl Pts',(45.7280621712483,48.5322875626859,-213.542090752468));
#221784=CARTESIAN_POINT('Ctrl Pts',(45.7028344378474,48.5428408361259,-213.544193292514));
#221785=CARTESIAN_POINT('Ctrl Pts',(45.6774461022642,48.553352630891,-213.546315176312));
#221786=CARTESIAN_POINT('Ctrl Pts',(45.6647519344726,48.5586085282736,-213.547376118211));
#221787=CARTESIAN_POINT('Ctrl Pts',(45.6520176160559,48.5638540557922,-213.548441896045));
#221788=CARTESIAN_POINT('Ctrl Pts',(45.6392430948086,48.5690888454429,-213.549512509832));
#221789=CARTESIAN_POINT('Ctrl Pts',(45.6276157176962,48.5738535542092,-213.55048698316));
#221790=CARTESIAN_POINT('Ctrl Pts',(45.6145896480273,48.5791640088112,-213.55158016601));
#221791=CARTESIAN_POINT('Ctrl Pts',(45.6038931400742,48.5835053146679,-213.552478890456));
#221792=CARTESIAN_POINT('Ctrl Pts',(45.6028378344585,48.5839336230905,-213.552567557613));
#221793=CARTESIAN_POINT('Ctrl Pts',(45.6018052171491,48.5843525379327,-213.552654329039));
#221794=CARTESIAN_POINT('Ctrl Pts',(45.6007988765239,48.584760628636,-213.552738902164));
#221795=CARTESIAN_POINT('Ctrl Pts',(45.5997929733645,48.5851685419385,-213.552823438524));
#221796=CARTESIAN_POINT('Ctrl Pts',(45.5987870597672,48.5855762915489,-213.552907982691));
#221797=CARTESIAN_POINT('Ctrl Pts',(45.5977811357529,48.5859838775069,-213.552992534718));
#221798=CARTESIAN_POINT('Ctrl Pts',(45.4223180751081,48.6570789887088,-213.567740922417));
#221799=CARTESIAN_POINT('Ctrl Pts',(45.2465642771724,48.723184982287,-213.582833694045));
#221800=CARTESIAN_POINT('Ctrl Pts',(45.0706080135195,48.7845018379456,-213.598475150732));
#221801=CARTESIAN_POINT('Ctrl Pts',(44.8922650990797,48.8466503884742,-213.614328766362));
#221802=CARTESIAN_POINT('Ctrl Pts',(44.7137050712026,48.9038847439255,-213.630706762686));
#221803=CARTESIAN_POINT('Ctrl Pts',(44.5348925487863,48.9564151707958,-213.64736607016));
#221804=CARTESIAN_POINT('Ctrl Pts',(44.3782619231994,49.0024291384522,-213.661958771589));
#221805=CARTESIAN_POINT('Ctrl Pts',(44.2213274321021,49.0448507637341,-213.676759131991));
#221806=CARTESIAN_POINT('Ctrl Pts',(44.0648182073631,49.0836230166911,-213.691823145796));
#221807=CARTESIAN_POINT('Ctrl Pts',(44.0402375397782,49.0897124204502,-213.694189035196));
#221808=CARTESIAN_POINT('Ctrl Pts',(44.0156672588303,49.0957118208884,-213.696561420079));
#221809=CARTESIAN_POINT('Ctrl Pts',(43.9911100751508,49.1016210123337,-213.698940508622));
#221810=CARTESIAN_POINT('Ctrl Pts',(43.8077580917296,49.1457409727519,-213.716703563573));
#221811=CARTESIAN_POINT('Ctrl Pts',(43.6249609203382,49.1848928448817,-213.734979503089));
#221812=CARTESIAN_POINT('Ctrl Pts',(43.4427334535923,49.2193110042465,-213.753761106585));
#221813=CARTESIAN_POINT('Ctrl Pts',(47.5746165801345,45.8238283676803,-216.758537654376));
#221814=CARTESIAN_POINT('Ctrl Pts',(48.4386236174112,46.8746099006705,-215.343430354514));
#221815=CARTESIAN_POINT('Ctrl Pts',(48.4710160211071,46.8924605148108,-213.380827300298));
#221816=CARTESIAN_POINT('Ctrl Pts',(47.406334611411,45.9580463783691,-216.758691640524));
#221817=CARTESIAN_POINT('Ctrl Pts',(48.202043344371,47.0656079993358,-215.343093772686));
#221818=CARTESIAN_POINT('Ctrl Pts',(48.1862070583782,47.1231145402161,-213.379368669215));
#221819=CARTESIAN_POINT('Ctrl Pts',(47.2339088845731,46.082710612235,-216.768384423925));
#221820=CARTESIAN_POINT('Ctrl Pts',(47.960805927557,47.2450787050191,-215.353433308566));
#221821=CARTESIAN_POINT('Ctrl Pts',(47.8936638370752,47.3370869807142,-213.387528102992));
#221822=CARTESIAN_POINT('Ctrl Pts',(47.0575921287078,46.1983743823903,-216.787046295788));
#221823=CARTESIAN_POINT('Ctrl Pts',(47.7151968771192,47.4137062867165,-215.373807350724));
#221824=CARTESIAN_POINT('Ctrl Pts',(47.5938143592261,47.5353276146285,-213.404748058676));
#221825=CARTESIAN_POINT('',(48.4710160211073,46.8924605148106,-213.380827300298));
#221826=CARTESIAN_POINT('',(47.5746165801346,45.8238283676801,-216.758537654376));
#221827=CARTESIAN_POINT('Origin',(45.3249961798233,43.0072392217583,-213.293565268111));
#221828=CARTESIAN_POINT('Ctrl Pts',(47.0575921287078,46.1983743823903,-216.787046295788));
#221829=CARTESIAN_POINT('Ctrl Pts',(47.1206620655918,46.1575511266546,-216.779921519949));
#221830=CARTESIAN_POINT('Ctrl Pts',(47.1845910131245,46.1142804480577,-216.774132275845));
#221831=CARTESIAN_POINT('Ctrl Pts',(47.2492989402458,46.068604399768,-216.769677997844));
#221832=CARTESIAN_POINT('Ctrl Pts',(47.2701598994296,46.0538790605176,-216.768241998953));
#221833=CARTESIAN_POINT('Ctrl Pts',(47.2911021053937,46.0389034482834,-216.766944780022));
#221834=CARTESIAN_POINT('Ctrl Pts',(47.3121237178813,46.0236781569863,-216.765786424972));
#221835=CARTESIAN_POINT('Ctrl Pts',(47.3752706746417,45.9779428066763,-216.7623068348));
#221836=CARTESIAN_POINT('Ctrl Pts',(47.4391323549421,45.9299570309712,-216.760079358312));
#221837=CARTESIAN_POINT('Ctrl Pts',(47.5036335622899,45.8797589197311,-216.759104615009));
#221838=CARTESIAN_POINT('Ctrl Pts',(47.5272094638708,45.861410957285,-216.758748335598));
#221839=CARTESIAN_POINT('Ctrl Pts',(47.5508712124359,45.8427671528649,-216.758559382341));
#221840=CARTESIAN_POINT('Ctrl Pts',(47.5746165801345,45.8238283676803,-216.758537654376));
#221841=CARTESIAN_POINT('Origin',(42.9552659882971,40.1115177027145,-218.083290145329));
#221842=CARTESIAN_POINT('Ctrl Pts',(50.7984099663005,43.0953291376929,-216.756961257354));
#221843=CARTESIAN_POINT('Ctrl Pts',(51.7004178351441,44.0801543735299,-215.34722316631));
#221844=CARTESIAN_POINT('Ctrl Pts',(51.7300796834961,44.0990078745203,-213.405670914582));
#221845=CARTESIAN_POINT('Ctrl Pts',(49.7561440689262,44.0321489495818,-216.756606633388));
#221846=CARTESIAN_POINT('Ctrl Pts',(50.6433589272998,45.038170309669,-215.345619228189));
#221847=CARTESIAN_POINT('Ctrl Pts',(50.6732101690724,45.0571976655732,-213.399273427567));
#221848=CARTESIAN_POINT('Ctrl Pts',(48.6689534025382,44.9510092870779,-216.757536292366));
#221849=CARTESIAN_POINT('Ctrl Pts',(49.5465852939469,45.977756673802,-215.344527068798));
#221850=CARTESIAN_POINT('Ctrl Pts',(49.5810652140745,45.9933960278872,-213.390312554365));
#221851=CARTESIAN_POINT('Ctrl Pts',(47.5746165801346,45.82382836768,-216.758537654376));
#221852=CARTESIAN_POINT('Ctrl Pts',(48.4386236174113,46.8746099006704,-215.343430354514));
#221853=CARTESIAN_POINT('Ctrl Pts',(48.4710160211072,46.8924605148107,-213.380827300298));
#221854=CARTESIAN_POINT('Ctrl Pts',(47.5746165801346,45.82382836768,-216.758537654376));
#221855=CARTESIAN_POINT('Ctrl Pts',(47.7452087461311,45.6877677925128,-216.758381555714));
#221856=CARTESIAN_POINT('Ctrl Pts',(47.9124683327338,45.5531103788107,-216.758230158611));
#221857=CARTESIAN_POINT('Ctrl Pts',(48.0767469921133,45.4196924030786,-216.758087000702));
#221858=CARTESIAN_POINT('Ctrl Pts',(48.2545046554837,45.2753275311754,-216.757932096738));
#221859=CARTESIAN_POINT('Ctrl Pts',(48.4287726329384,45.1324137879986,-216.757786825112));
#221860=CARTESIAN_POINT('Ctrl Pts',(48.6000196954607,44.990687035835,-216.757654799907));
#221861=CARTESIAN_POINT('Ctrl Pts',(48.786492574132,44.8363591596576,-216.757511036156));
#221862=CARTESIAN_POINT('Ctrl Pts',(48.9693842428768,44.6834386251299,-216.757382955664));
#221863=CARTESIAN_POINT('Ctrl Pts',(49.1493163534013,44.5315208113952,-216.757274540693));
#221864=CARTESIAN_POINT('Ctrl Pts',(49.3151698180586,44.3914896870029,-216.757174608567));
#221865=CARTESIAN_POINT('Ctrl Pts',(49.4785095089783,44.2523092521545,-216.757091358214));
#221866=CARTESIAN_POINT('Ctrl Pts',(49.6398237993626,44.113623656301,-216.757027743289));
#221867=CARTESIAN_POINT('Ctrl Pts',(51.7111509599702,44.1161634567458,-213.405556126747));
#221868=CARTESIAN_POINT('Ctrl Pts',(51.5538775663418,44.2586564036198,-213.404600680556));
#221869=CARTESIAN_POINT('Ctrl Pts',(51.3882561727022,44.4075223032268,-213.403542288886));
#221870=CARTESIAN_POINT('Ctrl Pts',(51.2140278838009,44.5626338811098,-213.40237201694));
#221871=CARTESIAN_POINT('Ctrl Pts',(51.0473579435284,44.7110164289977,-213.401252513577));
#221872=CARTESIAN_POINT('Ctrl Pts',(50.872811270086,44.8651146889509,-213.400030584105));
#221873=CARTESIAN_POINT('Ctrl Pts',(50.6901748034305,45.0247715567893,-213.398701013203));
#221874=CARTESIAN_POINT('Ctrl Pts',(50.5184166713263,45.1749188187229,-213.397450635232));
#221875=CARTESIAN_POINT('Ctrl Pts',(50.339503487995,45.3299822316343,-213.396105033313));
#221876=CARTESIAN_POINT('Ctrl Pts',(50.1532748754427,45.489788841628,-213.394662671329));
#221877=CARTESIAN_POINT('Ctrl Pts',(49.9727593666554,45.6446929195525,-213.393264557989));
#221878=CARTESIAN_POINT('Ctrl Pts',(49.7853700957918,45.8040538101684,-213.391775498415));
#221879=CARTESIAN_POINT('Ctrl Pts',(49.5909813482879,45.9676714965567,-213.390197223026));
#221880=CARTESIAN_POINT('Ctrl Pts',(49.4054192875547,46.1238597299213,-213.388690613012));
#221881=CARTESIAN_POINT('Ctrl Pts',(49.2134787906277,46.2839269881764,-213.387102687596));
#221882=CARTESIAN_POINT('Ctrl Pts',(49.0150726319924,46.4476586616144,-213.385438187813));
#221883=CARTESIAN_POINT('Ctrl Pts',(48.8388362262783,46.5930950826748,-213.383959677967));
#221884=CARTESIAN_POINT('Ctrl Pts',(48.6574984947564,46.7414223711376,-213.382420773499));
#221885=CARTESIAN_POINT('Ctrl Pts',(48.4710160211073,46.8924605148106,-213.380827300298));
#221886=CARTESIAN_POINT('Ctrl Pts',(32.8237598256933,-74.7342241033955,
-216.385388039321));
#221887=CARTESIAN_POINT('Ctrl Pts',(32.9990492150882,-74.6974990623407,
-216.482388336084));
#221888=CARTESIAN_POINT('Ctrl Pts',(33.1752262860961,-74.6372704537072,
-216.564961398279));
#221889=CARTESIAN_POINT('Ctrl Pts',(30.6715671894371,-72.7849850406464,
-219.42138468029));
#221890=CARTESIAN_POINT('Ctrl Pts',(30.8686320743566,-72.7455847913414,
-219.534693600851));
#221891=CARTESIAN_POINT('Ctrl Pts',(31.0696428925502,-72.6787836312099,
-219.626145751152));
#221892=CARTESIAN_POINT('Ctrl Pts',(28.5222070452525,-70.8331480683141,
-222.457793536072));
#221893=CARTESIAN_POINT('Ctrl Pts',(28.74408228947,-70.7922628748654,-222.589726795606));
#221894=CARTESIAN_POINT('Ctrl Pts',(28.9728528878395,-70.717730574095,-222.691719005855));
#221895=CARTESIAN_POINT('Ctrl Pts',(24.22299709402,-66.9233834882713,-228.527077755974));
#221896=CARTESIAN_POINT('Ctrl Pts',(24.5031890807173,-66.8863601198576,
-228.700118508997));
#221897=CARTESIAN_POINT('Ctrl Pts',(24.7931301396491,-66.7918626783751,
-228.829883596514));
#221898=CARTESIAN_POINT('Ctrl Pts',(22.0732081844572,-64.9654158172774,
-231.5599598492));
#221899=CARTESIAN_POINT('Ctrl Pts',(22.3840010183804,-64.9310042721652,
-231.75981083814));
#221900=CARTESIAN_POINT('Ctrl Pts',(22.7103354655404,-64.8270019993908,
-231.902532738117));
#221901=CARTESIAN_POINT('Ctrl Pts',(19.9239651248057,-63.0021267267442,
-234.590483038352));
#221902=CARTESIAN_POINT('Ctrl Pts',(20.2743464925947,-62.9804444339628,
-234.812766684068));
#221903=CARTESIAN_POINT('Ctrl Pts',(20.6355201207023,-62.8599765985421,
-234.979164865714));
#221904=CARTESIAN_POINT('Ctrl Pts',(20.0008767612649,-63.072381322781,-234.482033952692));
#221905=CARTESIAN_POINT('Ctrl Pts',(20.8043363234604,-63.8062709127761,
-233.349112874569));
#221906=CARTESIAN_POINT('Ctrl Pts',(21.6389257523856,-64.5677853736611,
-232.172066819715));
#221907=CARTESIAN_POINT('Ctrl Pts',(22.5046052525514,-65.3568774568241,
-230.950881057122));
#221908=CARTESIAN_POINT('Ctrl Pts',(22.6909951274677,-65.5267772576743,
-230.687946955649));
#221909=CARTESIAN_POINT('Ctrl Pts',(22.8788262188055,-65.6979556905867,
-230.422966630293));
#221910=CARTESIAN_POINT('Ctrl Pts',(23.0680980001634,-65.8704125801202,
-230.15593998937));
#221911=CARTESIAN_POINT('Ctrl Pts',(23.892776251857,-66.6218264735841,-228.992475146313));
#221912=CARTESIAN_POINT('Ctrl Pts',(24.7448045778254,-67.3975073430028,
-227.790160920506));
#221913=CARTESIAN_POINT('Ctrl Pts',(25.6241174401257,-68.1974604163476,
-226.549006038147));
#221914=CARTESIAN_POINT('Ctrl Pts',(25.871454308192,-68.4224746248779,-226.199888705114));
#221915=CARTESIAN_POINT('Ctrl Pts',(26.1209497924506,-68.6494095067943,
-225.847698406426));
#221916=CARTESIAN_POINT('Ctrl Pts',(26.3726020696362,-68.8782657782927,
-225.492435646023));
#221917=CARTESIAN_POINT('Ctrl Pts',(26.3807555168343,-68.8856806427496,
-225.480925254817));
#221918=CARTESIAN_POINT('Ctrl Pts',(26.388911227222,-68.8930975247752,-225.469411638228));
#221919=CARTESIAN_POINT('Ctrl Pts',(26.3970692009449,-68.9005164243056,
-225.457894796357));
#221920=CARTESIAN_POINT('Ctrl Pts',(26.4015990100156,-68.9046358539004,
-225.451499936978));
#221921=CARTESIAN_POINT('Ctrl Pts',(26.4072298854293,-68.9097565796957,
-225.443550657396));
#221922=CARTESIAN_POINT('Ctrl Pts',(26.4106607344689,-68.9128765773254,
-225.438707242511));
#221923=CARTESIAN_POINT('Ctrl Pts',(26.9376257303311,-69.3920960122429,
-224.694777656712));
#221924=CARTESIAN_POINT('Ctrl Pts',(27.4987696124221,-69.9022318817608,
-223.902462772249));
#221925=CARTESIAN_POINT('Ctrl Pts',(28.0941798074988,-70.4432427576873,
-223.06172624895));
#221926=CARTESIAN_POINT('Ctrl Pts',(28.6593592576155,-70.9567849037433,
-222.263676417321));
#221927=CARTESIAN_POINT('Ctrl Pts',(29.2554133760404,-71.4981462944317,
-221.42199684022));
#221928=CARTESIAN_POINT('Ctrl Pts',(29.8824557852991,-72.0672894473805,
-220.536679862955));
#221929=CARTESIAN_POINT('Ctrl Pts',(30.4700178601725,-72.6005977641848,
-219.707104905343));
#221930=CARTESIAN_POINT('Ctrl Pts',(31.0847886949289,-73.1582994545215,
-218.839214470805));
#221931=CARTESIAN_POINT('Ctrl Pts',(31.7269003069944,-73.7403633058953,
-217.933026378428));
#221932=CARTESIAN_POINT('Ctrl Pts',(32.0840513618251,-74.0641149942168,
-217.428992458178));
#221933=CARTESIAN_POINT('Ctrl Pts',(32.449661634212,-74.3954036850947,-216.913110714144));
#221934=CARTESIAN_POINT('Ctrl Pts',(32.8237598256933,-74.7342241033955,
-216.385388039321));
#221935=CARTESIAN_POINT('Ctrl Pts',(33.175226286096,-74.6372704537073,-216.564961398278));
#221936=CARTESIAN_POINT('Ctrl Pts',(31.0696461168607,-72.6787866302694,
-219.626141063516));
#221937=CARTESIAN_POINT('Ctrl Pts',(28.9728566674875,-70.7177341241867,
-222.691713455223));
#221938=CARTESIAN_POINT('Ctrl Pts',(26.8829915137443,-68.7547966262351,
-225.760801301184));
#221939=CARTESIAN_POINT('Ctrl Pts',(24.8618782440303,-66.8564353766477,
-228.728923029172));
#221940=CARTESIAN_POINT('Ctrl Pts',(22.8473703065303,-64.9562682465909,
-231.700386777838));
#221941=CARTESIAN_POINT('Ctrl Pts',(20.8402917354589,-63.0540784607098,
-234.675571320208));
#221942=CARTESIAN_POINT('Ctrl Pts',(49.585934372064,-31.4593264371528,-234.588572160238));
#221943=CARTESIAN_POINT('Ctrl Pts',(49.5518743118955,-31.8037460359236,
-234.831813626471));
#221944=CARTESIAN_POINT('Ctrl Pts',(49.4157810444631,-32.1591416363978,
-235.016540311968));
#221945=CARTESIAN_POINT('Ctrl Pts',(53.6191877437562,-36.2386826179501,
-228.465030977459));
#221946=CARTESIAN_POINT('Ctrl Pts',(53.577029434305,-36.5620211523723,-228.699571716257));
#221947=CARTESIAN_POINT('Ctrl Pts',(53.4511949264874,-36.9037628342018,
-228.868965623418));
#221948=CARTESIAN_POINT('Ctrl Pts',(57.647776611751,-41.0147938695427,-222.337140791317));
#221949=CARTESIAN_POINT('Ctrl Pts',(57.6060482975282,-41.3304581550816,
-222.559407848575));
#221950=CARTESIAN_POINT('Ctrl Pts',(57.4820653937753,-41.6584214713118,
-222.726315285231));
#221951=CARTESIAN_POINT('Ctrl Pts',(61.6760242364039,-45.7878268313144,
-216.206690793878));
#221952=CARTESIAN_POINT('Ctrl Pts',(61.634703071674,-46.0974912749688,-216.419279621934));
#221953=CARTESIAN_POINT('Ctrl Pts',(61.5121276273783,-46.4145707939142,
-216.584292819143));
#221954=CARTESIAN_POINT('Ctrl Pts',(49.628292885354,-32.4090157027691,-234.692796608792));
#221955=CARTESIAN_POINT('Ctrl Pts',(50.3968964627269,-33.3128002682304,
-233.521887849703));
#221956=CARTESIAN_POINT('Ctrl Pts',(51.2000586009216,-34.2576769533107,
-232.298264219454));
#221957=CARTESIAN_POINT('Ctrl Pts',(52.0377754118614,-35.2438971802995,
-231.021914190803));
#221958=CARTESIAN_POINT('Ctrl Pts',(52.1772574460439,-35.4081054206212,
-230.809398581709));
#221959=CARTESIAN_POINT('Ctrl Pts',(52.3176974834605,-35.5734597351558,
-230.595421181564));
#221960=CARTESIAN_POINT('Ctrl Pts',(52.4590955550812,-35.7399611653641,
-230.379981875082));
#221961=CARTESIAN_POINT('Ctrl Pts',(52.9544067724006,-36.3232083421935,
-229.625307473028));
#221962=CARTESIAN_POINT('Ctrl Pts',(53.4614885013061,-36.9204792537099,
-228.852675067089));
#221963=CARTESIAN_POINT('Ctrl Pts',(53.9803314191105,-37.5317625649504,
-228.062098198908));
#221964=CARTESIAN_POINT('Ctrl Pts',(54.3046082427385,-37.9138146344759,
-227.567987656295));
#221965=CARTESIAN_POINT('Ctrl Pts',(54.6334770682644,-38.3013448755334,
-227.066870608985));
#221966=CARTESIAN_POINT('Ctrl Pts',(54.9669330063277,-38.694346084446,-226.558754472118));
#221967=CARTESIAN_POINT('Ctrl Pts',(55.1128199792304,-38.8662841133452,
-226.336453662239));
#221968=CARTESIAN_POINT('Ctrl Pts',(55.2595849207926,-39.0392692670975,
-226.112813235058));
#221969=CARTESIAN_POINT('Ctrl Pts',(55.4072272930583,-39.2133007270977,
-225.887834013941));
#221970=CARTESIAN_POINT('Ctrl Pts',(55.4418309740581,-39.2540893505352,
-225.835104508991));
#221971=CARTESIAN_POINT('Ctrl Pts',(55.4764828535101,-39.294935448816,-225.782301462303));
#221972=CARTESIAN_POINT('Ctrl Pts',(55.5111829239329,-39.3358390104245,
-225.729424885354));
#221973=CARTESIAN_POINT('Ctrl Pts',(55.5197223943885,-39.3459051212891,
-225.716412290246));
#221974=CARTESIAN_POINT('Ctrl Pts',(55.5282647833905,-39.3559747122528,
-225.703395241991));
#221975=CARTESIAN_POINT('Ctrl Pts',(55.5368100908256,-39.3660477831409,
-225.690373740763));
#221976=CARTESIAN_POINT('Ctrl Pts',(55.5410660544895,-39.3710646446184,
-225.683888422768));
#221977=CARTESIAN_POINT('Ctrl Pts',(55.5453227420728,-39.3760823692935,
-225.677402000211));
#221978=CARTESIAN_POINT('Ctrl Pts',(55.5495801535614,-39.3811009571446,
-225.670914473112));
#221979=CARTESIAN_POINT('Ctrl Pts',(55.5517047016773,-39.3836053501054,
-225.667677045038));
#221980=CARTESIAN_POINT('Ctrl Pts',(55.5538294300633,-39.3861099580181,
-225.664439341906));
#221981=CARTESIAN_POINT('Ctrl Pts',(55.5559543387177,-39.38861478088,-225.66120136372));
#221982=CARTESIAN_POINT('Ctrl Pts',(55.5570799677375,-39.3899416620601,
-225.65948610777));
#221983=CARTESIAN_POINT('Ctrl Pts',(55.5582056473433,-39.3912686035581,
-225.657770774635));
#221984=CARTESIAN_POINT('Ctrl Pts',(55.5593313775347,-39.3925956053735,
-225.656055364317));
#221985=CARTESIAN_POINT('Ctrl Pts',(55.5596938325846,-39.3930228645097,
-225.655503048018));
#221986=CARTESIAN_POINT('Ctrl Pts',(55.5600602415825,-39.3934547845997,
-225.654944706604));
#221987=CARTESIAN_POINT('Ctrl Pts',(55.5604310504557,-39.3938918913041,
-225.654379660559));
#221988=CARTESIAN_POINT('Ctrl Pts',(55.56260151923,-39.3964504235328,-225.651072256439));
#221989=CARTESIAN_POINT('Ctrl Pts',(55.5649034761736,-39.3991639557866,
-225.647564487588));
#221990=CARTESIAN_POINT('Ctrl Pts',(55.567076907099,-39.4017259849979,-225.644252568918));
#221991=CARTESIAN_POINT('Ctrl Pts',(55.5681625613162,-39.4030057486127,
-225.64259822673));
#221992=CARTESIAN_POINT('Ctrl Pts',(55.5692161467671,-39.4042477103806,
-225.640992751492));
#221993=CARTESIAN_POINT('Ctrl Pts',(55.5702052568722,-39.4054136694099,
-225.639485525041));
#221994=CARTESIAN_POINT('Ctrl Pts',(55.5707995144804,-39.4061141778977,
-225.638579982998));
#221995=CARTESIAN_POINT('Ctrl Pts',(55.5713704990073,-39.4067872523628,
-225.637709904929));
#221996=CARTESIAN_POINT('Ctrl Pts',(55.5719111825918,-39.4074246083393,
-225.636886000043));
#221997=CARTESIAN_POINT('Ctrl Pts',(55.5721274114958,-39.4076794982383,
-225.636556505944));
#221998=CARTESIAN_POINT('Ctrl Pts',(55.5723390474855,-39.4079289740502,
-225.63623401062));
#221999=CARTESIAN_POINT('Ctrl Pts',(55.5725523044745,-39.4081803607153,
-225.63590904518));
#222000=CARTESIAN_POINT('Ctrl Pts',(56.480606911226,-40.4785922629171,-224.252196527753));
#222001=CARTESIAN_POINT('Ctrl Pts',(57.4295918931899,-41.5977057670165,
-222.806047408064));
#222002=CARTESIAN_POINT('Ctrl Pts',(58.41951461835,-42.7654653352818,-221.297452480847));
#222003=CARTESIAN_POINT('Ctrl Pts',(59.3138922525458,-43.8205154047766,
-219.9344637064));
#222004=CARTESIAN_POINT('Ctrl Pts',(60.2416866050878,-44.9152741778433,
-218.520501594197));
#222005=CARTESIAN_POINT('Ctrl Pts',(61.2029208033956,-46.0496598975624,
-217.055538740336));
#222006=CARTESIAN_POINT('Ctrl Pts',(61.305608086042,-46.1708447110407,-216.899038841658));
#222007=CARTESIAN_POINT('Ctrl Pts',(61.4086770135913,-46.292481719804,-216.741956884158));
#222008=CARTESIAN_POINT('Ctrl Pts',(61.512127627378,-46.4145707939139,-216.584292819143));
#222009=CARTESIAN_POINT('Ctrl Pts',(61.6760242364037,-45.7878268313144,
-216.206690793879));
#222010=CARTESIAN_POINT('Ctrl Pts',(60.5637265567327,-44.4698757063932,
-217.899457957883));
#222011=CARTESIAN_POINT('Ctrl Pts',(59.5069823263366,-43.2175506185294,
-219.507438028199));
#222012=CARTESIAN_POINT('Ctrl Pts',(58.5057724458651,-42.0309753379664,
-221.030605568401));
#222013=CARTESIAN_POINT('Ctrl Pts',(58.0051675056294,-41.4376876976849,
-221.792189338502));
#222014=CARTESIAN_POINT('Ctrl Pts',(57.5184463076789,-40.8608379362804,
-222.532571676405));
#222015=CARTESIAN_POINT('Ctrl Pts',(57.0456083644949,-40.3004320974512,
-223.251750990183));
#222016=CARTESIAN_POINT('Ctrl Pts',(56.8091893929029,-40.0202291780366,
-223.611340647071));
#222017=CARTESIAN_POINT('Ctrl Pts',(56.5762412683301,-39.7441372317215,
-223.965629563901));
#222018=CARTESIAN_POINT('Ctrl Pts',(56.3467639682679,-39.4721564367441,
-224.314617689053));
#222019=CARTESIAN_POINT('Ctrl Pts',(56.2320253182368,-39.3361660392554,
-224.489111751629));
#222020=CARTESIAN_POINT('Ctrl Pts',(56.118154376098,-39.2012034292329,-224.662280617158));
#222021=CARTESIAN_POINT('Ctrl Pts',(56.0051511455154,-39.0672686087644,
-224.834124283574));
#222022=CARTESIAN_POINT('Ctrl Pts',(55.948649530224,-39.0003011985301,-224.920046116782));
#222023=CARTESIAN_POINT('Ctrl Pts',(55.8923648429232,-38.9335907356627,
-225.005636650262));
#222024=CARTESIAN_POINT('Ctrl Pts',(55.8362970842186,-38.8671372180928,
-225.090895883975));
#222025=CARTESIAN_POINT('Ctrl Pts',(55.783733560433,-38.804837045371,-225.170826415581));
#222026=CARTESIAN_POINT('Ctrl Pts',(55.7313606965502,-38.7427627034764,
-225.250465765753));
#222027=CARTESIAN_POINT('Ctrl Pts',(55.6791784931789,-38.6809141896789,
-225.329813934577));
#222028=CARTESIAN_POINT('Ctrl Pts',(55.6756996796209,-38.6767909554257,
-225.335103812498));
#222029=CARTESIAN_POINT('Ctrl Pts',(55.6731827947325,-38.6738078386652,
-225.338930980825));
#222030=CARTESIAN_POINT('Ctrl Pts',(55.6687445946432,-38.6685474979491,
-225.345679685923));
#222031=CARTESIAN_POINT('Ctrl Pts',(54.483867468869,-37.2641814795681,-227.147397981386));
#222032=CARTESIAN_POINT('Ctrl Pts',(53.3720416758563,-35.9463663620178,
-228.837390453384));
#222033=CARTESIAN_POINT('Ctrl Pts',(52.3333167239498,-34.7152710364236,
-230.415667378188));
#222034=CARTESIAN_POINT('Ctrl Pts',(51.3799740041157,-33.5853706100183,
-231.864211396874));
#222035=CARTESIAN_POINT('Ctrl Pts',(50.4882100328808,-32.5285192791855,
-233.21865145119));
#222036=CARTESIAN_POINT('Ctrl Pts',(49.6580997553206,-31.5448418376796,
-234.479004906517));
#222037=CARTESIAN_POINT('Ctrl Pts',(61.6446456814074,19.9883159925443,-216.270380726959));
#222038=CARTESIAN_POINT('Ctrl Pts',(61.616890721367,20.2979288461104,-216.446591335266));
#222039=CARTESIAN_POINT('Ctrl Pts',(61.5168384358512,20.6141575018442,-216.579518431211));
#222040=CARTESIAN_POINT('Ctrl Pts',(57.6234673266503,16.1196899878155,-222.390750665928));
#222041=CARTESIAN_POINT('Ctrl Pts',(57.5955705123416,16.4361291341491,-222.575565676854));
#222042=CARTESIAN_POINT('Ctrl Pts',(57.494494092276,16.762978594578,-222.709815956689));
#222043=CARTESIAN_POINT('Ctrl Pts',(53.6019508938474,12.2476417326856,-228.50878407383));
#222044=CARTESIAN_POINT('Ctrl Pts',(53.5738347736258,12.5726920250932,-228.704663275299));
#222045=CARTESIAN_POINT('Ctrl Pts',(53.4715033219665,12.9130963103019,-228.840508302186));
#222046=CARTESIAN_POINT('Ctrl Pts',(49.5760442618401,8.3708766333566,-234.622127004475));
#222047=CARTESIAN_POINT('Ctrl Pts',(49.5561728047784,8.71705005588278,-234.825566445945));
#222048=CARTESIAN_POINT('Ctrl Pts',(49.444665056238,9.07318219289785,-234.975080467413));
#222049=CARTESIAN_POINT('Ctrl Pts',(49.6480781836462,8.44024209637808,-234.512742074857));
#222050=CARTESIAN_POINT('Ctrl Pts',(50.5108389786845,9.27104318303506,-233.202606649067));
#222051=CARTESIAN_POINT('Ctrl Pts',(51.4422122349174,10.1678939238171,-231.787674256305));
#222052=CARTESIAN_POINT('Ctrl Pts',(52.942166373959,11.6122001294847,-229.508080216706));
#222053=CARTESIAN_POINT('Ctrl Pts',(53.4592996669872,12.1101370188218,-228.722016295096));
#222054=CARTESIAN_POINT('Ctrl Pts',(54.2607151734181,12.8817572829805,-227.503621550068));
#222055=CARTESIAN_POINT('Ctrl Pts',(54.6678517734159,13.273745816856,-226.8845994619));
#222056=CARTESIAN_POINT('Ctrl Pts',(55.1540928798677,13.7418663231132,-226.14521377331));
#222057=CARTESIAN_POINT('Ctrl Pts',(55.4307667843284,14.0082198307574,-225.724473721243));
#222058=CARTESIAN_POINT('Ctrl Pts',(55.5679131202823,14.1402470759619,-225.515906191076));
#222059=CARTESIAN_POINT('Ctrl Pts',(55.6389493534834,14.2086309446081,-225.407874655615));
#222060=CARTESIAN_POINT('Ctrl Pts',(55.6443683020085,14.2138475540897,-225.399633534663));
#222061=CARTESIAN_POINT('Ctrl Pts',(57.4212558731114,15.9243864082124,-222.697345395563));
#222062=CARTESIAN_POINT('Ctrl Pts',(59.4202299305932,17.8482884045604,-219.656016999063));
#222063=CARTESIAN_POINT('Ctrl Pts',(61.6446456814072,19.9883159925442,-216.270380726959));
#222064=CARTESIAN_POINT('Ctrl Pts',(61.5168384358511,20.614157501844,-216.579518431211));
#222065=CARTESIAN_POINT('Ctrl Pts',(60.509204282799,19.6494018606037,-218.115214191548));
#222066=CARTESIAN_POINT('Ctrl Pts',(59.5377925343497,18.7194149348883,-219.595668877975));
#222067=CARTESIAN_POINT('Ctrl Pts',(58.6026020527902,17.8244138442871,-221.020869980282));
#222068=CARTESIAN_POINT('Ctrl Pts',(58.5427562442271,17.7671398824708,-221.112073124469));
#222069=CARTESIAN_POINT('Ctrl Pts',(58.4830587721403,17.710009176867,-221.203049992023));
#222070=CARTESIAN_POINT('Ctrl Pts',(58.4235096385423,17.6530217783262,-221.293800577196));
#222071=CARTESIAN_POINT('Ctrl Pts',(57.9284578513069,17.1792665480993,-222.048240426577));
#222072=CARTESIAN_POINT('Ctrl Pts',(57.4436640563974,16.715388786722,-222.787033765522));
#222073=CARTESIAN_POINT('Ctrl Pts',(56.9691198749181,16.2614050505997,-223.510192149142));
#222074=CARTESIAN_POINT('Ctrl Pts',(56.6725297614939,15.9776652155236,-223.962166138905));
#222075=CARTESIAN_POINT('Ctrl Pts',(56.3799432813792,15.6977900414939,-224.408032920716));
#222076=CARTESIAN_POINT('Ctrl Pts',(56.091358153519,15.4217789157186,-224.847795942265));
#222077=CARTESIAN_POINT('Ctrl Pts',(55.9651021600802,15.3010240481919,-225.040192264193));
#222078=CARTESIAN_POINT('Ctrl Pts',(55.8396120364535,15.1810087617059,-225.231420310576));
#222079=CARTESIAN_POINT('Ctrl Pts',(55.7148875380785,15.0617329150462,-225.421480456045));
#222080=CARTESIAN_POINT('Ctrl Pts',(55.6856552337718,15.0337776384854,-225.466025802639));
#222081=CARTESIAN_POINT('Ctrl Pts',(55.6564649864125,15.0058629803695,-225.510506994689));
#222082=CARTESIAN_POINT('Ctrl Pts',(55.6273167926219,14.9779889384813,-225.554924037388));
#222083=CARTESIAN_POINT('Ctrl Pts',(55.6201436043062,14.9711293109853,-225.56585479399));
#222084=CARTESIAN_POINT('Ctrl Pts',(55.6129729628437,14.9642721432938,-225.576781665572));
#222085=CARTESIAN_POINT('Ctrl Pts',(55.6058048681833,14.9574174353723,-225.587704652211));
#222086=CARTESIAN_POINT('Ctrl Pts',(55.6022348210379,14.954003469513,-225.593144811573));
#222087=CARTESIAN_POINT('Ctrl Pts',(55.5986654056286,14.9505901138013,-225.598584007272));
#222088=CARTESIAN_POINT('Ctrl Pts',(55.595096621949,14.947177368233,-225.604022239318));
#222089=CARTESIAN_POINT('Ctrl Pts',(55.5933157152495,14.9454743282082,-225.606736044567));
#222090=CARTESIAN_POINT('Ctrl Pts',(55.5915349658661,14.943771440124,-225.609449609844));
#222091=CARTESIAN_POINT('Ctrl Pts',(55.589754373798,14.9420687039798,-225.612162935149));
#222092=CARTESIAN_POINT('Ctrl Pts',(55.5887986781916,14.9411547959146,-225.613619255841));
#222093=CARTESIAN_POINT('Ctrl Pts',(55.5878430279043,14.94024093162,-225.615075507402));
#222094=CARTESIAN_POINT('Ctrl Pts',(55.586887422936,14.9393271110959,-225.616531689833));
#222095=CARTESIAN_POINT('Ctrl Pts',(55.5865850402481,14.9390379502863,-225.616992470565));
#222096=CARTESIAN_POINT('Ctrl Pts',(55.5862873065917,14.9387532352696,-225.617446166943));
#222097=CARTESIAN_POINT('Ctrl Pts',(55.5859935256647,14.9384723001864,-225.617893840014));
#222098=CARTESIAN_POINT('Ctrl Pts',(55.584266632255,14.9368209167942,-225.62052533718));
#222099=CARTESIAN_POINT('Ctrl Pts',(55.5826696508247,14.9352937661347,-225.622958869973));
#222100=CARTESIAN_POINT('Ctrl Pts',(55.5809424055013,14.9336420489766,-225.625590902938));
#222101=CARTESIAN_POINT('Ctrl Pts',(55.5800796262211,14.9328169969,-225.626905634248));
#222102=CARTESIAN_POINT('Ctrl Pts',(55.5791843445349,14.9319608640104,-225.628269893732));
#222103=CARTESIAN_POINT('Ctrl Pts',(55.578224133597,14.9310426415477,-225.629733094454));
#222104=CARTESIAN_POINT('Ctrl Pts',(55.5776368070909,14.9304809978822,-225.630628081727));
#222105=CARTESIAN_POINT('Ctrl Pts',(55.5770251884148,14.929896124466,-225.631560086172));
#222106=CARTESIAN_POINT('Ctrl Pts',(55.5763818568836,14.92928092516,-225.632540415665));
#222107=CARTESIAN_POINT('Ctrl Pts',(55.5761254152632,14.9290356974675,-225.632931189739));
#222108=CARTESIAN_POINT('Ctrl Pts',(55.5758654862487,14.9287871349127,-225.633327278013));
#222109=CARTESIAN_POINT('Ctrl Pts',(55.5756069918427,14.9285399442642,-225.633721180178));
#222110=CARTESIAN_POINT('Ctrl Pts',(54.6009073193254,13.9964631235507,-227.119000174852));
#222111=CARTESIAN_POINT('Ctrl Pts',(53.6642063037329,13.101179913745,-228.546300112712));
#222112=CARTESIAN_POINT('Ctrl Pts',(52.7655077853552,12.2427220677471,-229.915616611674));
#222113=CARTESIAN_POINT('Ctrl Pts',(51.8033650152148,11.323660788456,-231.381600968574));
#222114=CARTESIAN_POINT('Ctrl Pts',(50.8847798806897,10.4468075147946,-232.781126025169));
#222115=CARTESIAN_POINT('Ctrl Pts',(50.0097760330178,9.61214928592863,-234.114165364083));
#222116=CARTESIAN_POINT('Ctrl Pts',(49.8830780335951,9.49129321417494,-234.307185563756));
#222117=CARTESIAN_POINT('Ctrl Pts',(49.7572937961925,9.37132173405822,-234.498811779421));
#222118=CARTESIAN_POINT('Ctrl Pts',(49.6324234200406,9.25223473081225,-234.689043900262));
#222119=CARTESIAN_POINT('Ctrl Pts',(23.3435674340446,39.0028315981393,-234.685329588431));
#222120=CARTESIAN_POINT('Ctrl Pts',(23.6220011219804,38.9711607503308,-234.795474514856));
#222121=CARTESIAN_POINT('Ctrl Pts',(23.9003793742244,38.8880062428325,-234.874538682189));
#222122=CARTESIAN_POINT('Ctrl Pts',(24.8211107939746,40.877797860099,-231.583566767888));
#222123=CARTESIAN_POINT('Ctrl Pts',(25.0911477353951,40.8413970872541,-231.693486415051));
#222124=CARTESIAN_POINT('Ctrl Pts',(25.3613763065334,40.7570726336726,-231.772074584151));
#222125=CARTESIAN_POINT('Ctrl Pts',(26.3601379756881,42.7472614109061,-228.507926237645));
#222126=CARTESIAN_POINT('Ctrl Pts',(26.6294910045101,42.7083687308544,-228.618918190678));
#222127=CARTESIAN_POINT('Ctrl Pts',(26.8976008468902,42.6201313634466,-228.700804952979));
#222128=CARTESIAN_POINT('Ctrl Pts',(29.5673202653105,46.4871525231188,-222.371256086851));
#222129=CARTESIAN_POINT('Ctrl Pts',(29.8423301360257,46.4421792512365,-222.490600959002));
#222130=CARTESIAN_POINT('Ctrl Pts',(30.1156268744464,46.3449292397562,-222.578666771697));
#222131=CARTESIAN_POINT('Ctrl Pts',(31.2349886649714,48.357017195617,-219.311797960276));
#222132=CARTESIAN_POINT('Ctrl Pts',(31.5173957493039,48.3097394640464,-219.436505895139));
#222133=CARTESIAN_POINT('Ctrl Pts',(31.7969999993534,48.2062302604519,-219.529408809912));
#222134=CARTESIAN_POINT('Ctrl Pts',(32.9442943454133,50.2193438073887,-216.27126917285));
#222135=CARTESIAN_POINT('Ctrl Pts',(33.2349457782287,50.1687782395761,-216.404317351376));
#222136=CARTESIAN_POINT('Ctrl Pts',(33.5239821027453,50.0594436315753,-216.500446897106));
#222137=CARTESIAN_POINT('Ctrl Pts',(23.9972286658434,39.0117605909834,-234.669151698811));
#222138=CARTESIAN_POINT('Ctrl Pts',(24.3327345456529,39.4399669118617,-233.958598804035));
#222139=CARTESIAN_POINT('Ctrl Pts',(24.6854969464168,39.8847826332992,-233.221626122003));
#222140=CARTESIAN_POINT('Ctrl Pts',(25.2417823256465,40.576961386451,-232.076537418069));
#222141=CARTESIAN_POINT('Ctrl Pts',(25.4317384457601,40.8118462958157,-231.688236236611));
#222142=CARTESIAN_POINT('Ctrl Pts',(25.723657541265,41.1704115471192,-231.095877044201));
#222143=CARTESIAN_POINT('Ctrl Pts',(25.8713636961786,41.3512535867699,-230.797220592941));
#222144=CARTESIAN_POINT('Ctrl Pts',(26.0467904156662,41.564964282497,-230.444453570124));
#222145=CARTESIAN_POINT('Ctrl Pts',(26.1416066636588,41.6801828126252,-230.254310210665));
#222146=CARTESIAN_POINT('Ctrl Pts',(26.1860831699019,41.7341503401857,-230.165260585893));
#222147=CARTESIAN_POINT('Ctrl Pts',(26.2115545459155,41.7650376285435,-230.114297684302));
#222148=CARTESIAN_POINT('Ctrl Pts',(26.2187586061939,41.7737714214641,-230.099887554133));
#222149=CARTESIAN_POINT('Ctrl Pts',(26.5792284479624,42.210703138559,-229.378993935433));
#222150=CARTESIAN_POINT('Ctrl Pts',(26.9502784517109,42.6554480634503,-228.645975349437));
#222151=CARTESIAN_POINT('Ctrl Pts',(27.5320846287234,43.3443938192852,-227.511624012913));
#222152=CARTESIAN_POINT('Ctrl Pts',(27.8292992959109,43.6943231798319,-226.935742480268));
#222153=CARTESIAN_POINT('Ctrl Pts',(28.187363035252,44.1121215812652,-226.248645429514));
#222154=CARTESIAN_POINT('Ctrl Pts',(28.3692597182274,44.3234069165231,-225.90128808847));
#222155=CARTESIAN_POINT('Ctrl Pts',(28.4674767065592,44.4372345141931,-225.714183580142));
#222156=CARTESIAN_POINT('Ctrl Pts',(28.5135222374433,44.4905279982249,-225.626590416781));
#222157=CARTESIAN_POINT('Ctrl Pts',(28.5398857549393,44.5210240112345,-225.576469166008));
#222158=CARTESIAN_POINT('Ctrl Pts',(28.5472959748104,44.5295939877615,-225.562384320267));
#222159=CARTESIAN_POINT('Ctrl Pts',(28.9232877526146,44.9643580741901,-224.847853406652));
#222160=CARTESIAN_POINT('Ctrl Pts',(29.3098036855485,45.4068161964465,-224.121210421383));
#222161=CARTESIAN_POINT('Ctrl Pts',(29.9147542901699,46.0921360058483,-222.996588661072));
#222162=CARTESIAN_POINT('Ctrl Pts',(30.223526374801,46.4402036354049,-222.425613460314));
#222163=CARTESIAN_POINT('Ctrl Pts',(30.594963504495,46.8557539570813,-221.744313165042));
#222164=CARTESIAN_POINT('Ctrl Pts',(30.7835078386655,47.0658975627284,-221.399872377143));
#222165=CARTESIAN_POINT('Ctrl Pts',(30.8852740454166,47.1791089645397,-221.214335176413));
#222166=CARTESIAN_POINT('Ctrl Pts',(30.9329723885077,47.2321136761852,-221.127474748553));
#222167=CARTESIAN_POINT('Ctrl Pts',(30.9602794753431,47.2624443837978,-221.077772528342));
#222168=CARTESIAN_POINT('Ctrl Pts',(30.9679432262936,47.2709552412231,-221.063826154286));
#222169=CARTESIAN_POINT('Ctrl Pts',(31.7422680026501,48.1307494830713,-219.654932201219));
#222170=CARTESIAN_POINT('Ctrl Pts',(32.5743824792101,49.0398372611993,-218.167004164594));
#222171=CARTESIAN_POINT('Ctrl Pts',(33.473440697418,50.0051916640197,-216.589120385862));
#222172=CARTESIAN_POINT('Ctrl Pts',(32.8943360433598,50.1648136138275,-216.360311415042));
#222173=CARTESIAN_POINT('Ctrl Pts',(31.9457996056765,49.1307894599697,-218.048583135007));
#222174=CARTESIAN_POINT('Ctrl Pts',(31.0649583664921,48.1537646198439,-219.645964150516));
#222175=CARTESIAN_POINT('Ctrl Pts',(29.839374049799,46.7731472080332,-221.905699617094));
#222176=CARTESIAN_POINT('Ctrl Pts',(29.4468033566793,46.3270986719498,-222.636222096506));
#222177=CARTESIAN_POINT('Ctrl Pts',(28.8812510347518,45.6792205773753,-223.697921801452));
#222178=CARTESIAN_POINT('Ctrl Pts',(28.6043018556398,45.3605804968602,-224.220250650383));
#222179=CARTESIAN_POINT('Ctrl Pts',(28.2912644925847,44.998100764893,-224.814722551268));
#222180=CARTESIAN_POINT('Ctrl Pts',(28.1372482450597,44.8191770801532,-225.108230562661));
#222181=CARTESIAN_POINT('Ctrl Pts',(28.0526798290621,44.7207710516647,-225.269676371552));
#222182=CARTESIAN_POINT('Ctrl Pts',(28.0119681642909,44.6733490752071,-225.347483262868));
#222183=CARTESIAN_POINT('Ctrl Pts',(27.990307112259,44.6481055978128,-225.388902606174));
#222184=CARTESIAN_POINT('Ctrl Pts',(27.9883067709655,44.6457743250737,-225.39272775696));
#222185=CARTESIAN_POINT('Ctrl Pts',(26.2378764098086,42.6055670942602,-228.740321770674));
#222186=CARTESIAN_POINT('Ctrl Pts',(24.7202894771203,40.7480003447697,-231.798693741316));
#222187=CARTESIAN_POINT('Ctrl Pts',(23.3965311730097,39.0699180251917,-234.574369193282));
#222188=CARTESIAN_POINT('Origin',(7.99493453126772,-4.92182388367686,-192.281986444803));
#222189=CARTESIAN_POINT('',(7.45184924284871,-4.40456343718705,-229.35005));
#222190=CARTESIAN_POINT('',(8.57396770167424,-4.44514727677342,-229.35005));
#222191=CARTESIAN_POINT('Origin',(7.99493453126772,-4.92182388367686,-229.35005));
#222192=CARTESIAN_POINT('',(7.45184924284871,-4.40456343718705,-192.281986444803));
#222193=CARTESIAN_POINT('',(8.57396770167424,-4.44514727677342,-192.281986444803));
#222194=CARTESIAN_POINT('Origin',(1.25,-20.2703558849778,-192.281986444803));
#222195=CARTESIAN_POINT('',(0.5,-20.2703558849778,-229.35005));
#222196=CARTESIAN_POINT('',(0.5,-20.2703558849778,-235.35005));
#222197=CARTESIAN_POINT('',(1.14413406213993,-19.5278652094801,-229.35005));
#222198=CARTESIAN_POINT('',(1.14413406213993,-19.5278652094801,-192.281986444803));
#222199=CARTESIAN_POINT('Origin',(1.25,-20.2703558849778,-229.35005));
#222200=CARTESIAN_POINT('Origin',(10.2798200094577,-12.7534818258363,-192.281986444803));
#222201=CARTESIAN_POINT('',(10.2798200094577,-12.0034818258363,-229.35005));
#222202=CARTESIAN_POINT('',(10.2798200094577,-12.0034818258363,-229.35005));
#222203=CARTESIAN_POINT('',(11.0243360211906,-12.844013081618,-229.35005));
#222204=CARTESIAN_POINT('',(11.0243360211906,-12.844013081618,-192.281986444803));
#222205=CARTESIAN_POINT('Origin',(10.2798200094577,-12.7534818258363,-229.35005));
#222206=CARTESIAN_POINT('Origin',(8.76687405914144,-12.7534818258363,-192.281986444803));
#222207=CARTESIAN_POINT('',(8.02438338364376,-12.6476158879763,-229.35005));
#222208=CARTESIAN_POINT('',(8.02438338364376,-12.6476158879763,-192.281986444803));
#222209=CARTESIAN_POINT('',(8.76687405914144,-12.0034818258363,-229.35005));
#222210=CARTESIAN_POINT('',(8.76687405914144,-12.0034818258363,-235.35005));
#222211=CARTESIAN_POINT('Origin',(8.76687405914144,-12.7534818258363,-229.35005));
#222212=CARTESIAN_POINT('Origin',(8.76687405914145,-10.2534818258363,-192.281986444803));
#222213=CARTESIAN_POINT('',(8.76687405914145,-11.0034818258363,-229.35005));
#222214=CARTESIAN_POINT('',(8.76687405914145,-11.0034818258363,-229.35005));
#222215=CARTESIAN_POINT('',(8.02438338364376,-10.3593477636964,-229.35005));
#222216=CARTESIAN_POINT('',(8.02438338364376,-10.3593477636964,-192.281986444803));
#222217=CARTESIAN_POINT('Origin',(8.76687405914145,-10.2534818258363,-229.35005));
#222218=CARTESIAN_POINT('Origin',(10.2798200094577,-10.2534818258363,-192.281986444803));
#222219=CARTESIAN_POINT('',(11.0243360211906,-10.1629505700546,-229.35005));
#222220=CARTESIAN_POINT('',(11.0243360211906,-10.1629505700546,-192.281986444803));
#222221=CARTESIAN_POINT('',(10.2798200094577,-11.0034818258363,-229.35005));
#222222=CARTESIAN_POINT('',(10.2798200094577,-11.0034818258363,-229.35005));
#222223=CARTESIAN_POINT('Origin',(10.2798200094577,-10.2534818258363,-229.35005));
#222224=CARTESIAN_POINT('Origin',(6.95148506756697,-6.01736880073006,-192.281986444803));
#222225=CARTESIAN_POINT('',(6.36274467860838,-6.48200280121742,-229.35005));
#222226=CARTESIAN_POINT('',(6.36274467860838,-6.48200280121742,-192.281986444803));
#222227=CARTESIAN_POINT('',(6.40839977914796,-5.50010835424024,-229.35005));
#222228=CARTESIAN_POINT('',(6.40839977914796,-5.50010835424024,-235.35005));
#222229=CARTESIAN_POINT('Origin',(6.95148506756697,-6.01736880073006,-229.35005));
#222230=CARTESIAN_POINT('Origin',(5.14120077283694,-4.29316731243069,-192.281986444803));
#222231=CARTESIAN_POINT('',(5.68428606125595,-4.81042775892049,-229.35005));
#222232=CARTESIAN_POINT('',(5.68428606125595,-4.81042775892049,-229.35005));
#222233=CARTESIAN_POINT('',(4.70577833960231,-4.90382867901287,-229.35005));
#222234=CARTESIAN_POINT('',(4.70577833960231,-4.90382867901288,-192.281986444803));
#222235=CARTESIAN_POINT('Origin',(5.14120077283694,-4.29316731243068,-229.35005));
#222236=CARTESIAN_POINT('Origin',(1.25,-2.73660776669488,-192.281986444803));
#222237=CARTESIAN_POINT('',(1.14413406213993,-3.47909844219256,-229.35005));
#222238=CARTESIAN_POINT('',(1.14413406213993,-3.47909844219257,-192.281986444803));
#222239=CARTESIAN_POINT('',(0.5,-2.73660776669487,-229.35005));
#222240=CARTESIAN_POINT('',(0.5,-2.73660776669487,-235.35005));
#222241=CARTESIAN_POINT('Origin',(1.25,-2.73660776669487,-229.35005));
#222242=CARTESIAN_POINT('Origin',(8.87499999999985,-23.3741205625531,-192.281986444803));
#222243=CARTESIAN_POINT('',(8.83216440217218,-22.6253448207192,-229.35005));
#222244=CARTESIAN_POINT('',(9.62499999999985,-23.3741205625531,-229.35005));
#222245=CARTESIAN_POINT('Origin',(8.87499999999985,-23.3741205625531,-229.35005));
#222246=CARTESIAN_POINT('',(8.83216440217218,-22.6253448207192,-192.281986444803));
#222247=CARTESIAN_POINT('',(9.62499999999985,-23.3741205625531,-235.35005));
#222248=CARTESIAN_POINT('Origin',(12.7946237611812,-12.7534818258363,-192.281986444803));
#222249=CARTESIAN_POINT('',(12.0481776255232,-12.6805560652209,-229.35005));
#222250=CARTESIAN_POINT('',(12.0481776255232,-12.6805560652209,-192.281986444803));
#222251=CARTESIAN_POINT('',(12.7946237611812,-12.0034818258363,-229.35005));
#222252=CARTESIAN_POINT('',(12.7946237611812,-12.0034818258363,-235.35005));
#222253=CARTESIAN_POINT('Origin',(12.7946237611812,-12.7534818258363,-229.35005));
#222254=CARTESIAN_POINT('Origin',(11.3749999999999,-20.8590213785032,-229.35005));
#222255=CARTESIAN_POINT('',(11.3749999999999,-21.6090213785032,-229.35005));
#222256=CARTESIAN_POINT('',(11.3749999999999,-21.6090213785032,-229.35005));
#222257=CARTESIAN_POINT('',(10.6249999999999,-20.8590213785032,-229.35005));
#222258=CARTESIAN_POINT('',(10.6249999999999,-20.8590213785032,-235.35005));
#222259=CARTESIAN_POINT('Origin',(11.3749999999999,-20.8590213785032,-229.35005));
#222260=CARTESIAN_POINT('Origin',(19.,-20.8590213785032,-229.35005));
#222261=CARTESIAN_POINT('',(19.75,-20.8590213785032,-229.35005));
#222262=CARTESIAN_POINT('',(19.75,-20.8590213785032,-235.35005));
#222263=CARTESIAN_POINT('',(19.,-21.6090213785031,-229.35005));
#222264=CARTESIAN_POINT('',(19.,-21.6090213785031,-229.35005));
#222265=CARTESIAN_POINT('Origin',(19.,-20.8590213785032,-229.35005));
#222266=CARTESIAN_POINT('Origin',(19.,-12.7534818258363,-229.35005));
#222267=CARTESIAN_POINT('',(19.,-12.0034818258363,-229.35005));
#222268=CARTESIAN_POINT('',(19.,-12.0034818258363,-229.35005));
#222269=CARTESIAN_POINT('',(19.75,-12.7534818258363,-229.35005));
#222270=CARTESIAN_POINT('',(19.75,-12.7534818258363,-235.35005));
#222271=CARTESIAN_POINT('Origin',(19.,-12.7534818258363,-229.35005));
#222272=CARTESIAN_POINT('Origin',(12.7946237611812,-10.2534818258363,-192.281986444803));
#222273=CARTESIAN_POINT('',(12.7946237611812,-11.0034818258363,-229.35005));
#222274=CARTESIAN_POINT('',(12.7946237611812,-11.0034818258363,-229.35005));
#222275=CARTESIAN_POINT('',(12.0481776255232,-10.3264075864518,-229.35005));
#222276=CARTESIAN_POINT('',(12.0481776255232,-10.3264075864518,-192.281986444803));
#222277=CARTESIAN_POINT('Origin',(12.7946237611812,-10.2534818258363,-229.35005));
#222278=CARTESIAN_POINT('Origin',(19.,-10.2534818258363,-229.35005));
#222279=CARTESIAN_POINT('',(19.75,-10.2534818258363,-229.35005));
#222280=CARTESIAN_POINT('',(19.75,-10.2534818258363,-235.35005));
#222281=CARTESIAN_POINT('',(19.,-11.0034818258363,-229.35005));
#222282=CARTESIAN_POINT('',(19.,-11.0034818258363,-229.35005));
#222283=CARTESIAN_POINT('Origin',(19.,-10.2534818258363,-229.35005));
#222284=CARTESIAN_POINT('Origin',(19.,-2.14794227316951,-229.35005));
#222285=CARTESIAN_POINT('',(19.,-1.39794227316951,-229.35005));
#222286=CARTESIAN_POINT('',(19.,-1.39794227316951,-229.35005));
#222287=CARTESIAN_POINT('',(19.75,-2.14794227316951,-229.35005));
#222288=CARTESIAN_POINT('',(19.75,-2.14794227316951,-235.35005));
#222289=CARTESIAN_POINT('Origin',(19.,-2.14794227316951,-229.35005));
#222290=CARTESIAN_POINT('Origin',(11.3749999999999,-2.14794227316951,-229.35005));
#222291=CARTESIAN_POINT('',(10.6249999999999,-2.14794227316951,-229.35005));
#222292=CARTESIAN_POINT('',(10.6249999999999,-2.14794227316951,-235.35005));
#222293=CARTESIAN_POINT('',(11.3749999999999,-1.3979422731695,-229.35005));
#222294=CARTESIAN_POINT('',(11.3749999999999,-1.3979422731695,-229.35005));
#222295=CARTESIAN_POINT('Origin',(11.3749999999999,-2.14794227316951,-229.35005));
#222296=CARTESIAN_POINT('Origin',(8.87499999999985,0.367156910880378,-192.281986444803));
#222297=CARTESIAN_POINT('',(9.62499999999985,0.367156910880385,-229.35005));
#222298=CARTESIAN_POINT('',(9.62499999999985,0.367156910880383,-229.35005));
#222299=CARTESIAN_POINT('',(8.83216440217218,-0.38161883095341,-229.35005));
#222300=CARTESIAN_POINT('',(8.83216440217218,-0.381618830953416,-192.281986444803));
#222301=CARTESIAN_POINT('Origin',(8.87499999999985,0.367156910880383,-229.35005));
#222302=CARTESIAN_POINT('Origin',(8.87499999999986,8.45759727949731,-229.35005));
#222303=CARTESIAN_POINT('',(8.87499999999986,9.20759727949731,-229.35005));
#222304=CARTESIAN_POINT('',(8.87499999999986,9.20759727949731,-229.35005));
#222305=CARTESIAN_POINT('',(9.62499999999986,8.45759727949731,-229.35005));
#222306=CARTESIAN_POINT('',(9.62499999999986,8.45759727949731,-235.35005));
#222307=CARTESIAN_POINT('Origin',(8.87499999999986,8.45759727949731,-229.35005));
#222308=CARTESIAN_POINT('Origin',(1.25,8.45759727949731,-229.35005));
#222309=CARTESIAN_POINT('',(0.5,8.45759727949731,-229.35005));
#222310=CARTESIAN_POINT('',(0.5,8.45759727949731,-235.35005));
#222311=CARTESIAN_POINT('',(1.25,9.20759727949731,-229.35005));
#222312=CARTESIAN_POINT('',(1.25,9.20759727949731,-229.35005));
#222313=CARTESIAN_POINT('Origin',(1.25,8.45759727949731,-229.35005));
#222314=CARTESIAN_POINT('Origin',(1.25,2.29555713691451,-192.281986444803));
#222315=CARTESIAN_POINT('',(1.18233753211584,1.54861551239502,-229.35005));
#222316=CARTESIAN_POINT('',(1.18233753211584,1.54861551239501,-192.281986444803));
#222317=CARTESIAN_POINT('',(0.5,2.29555713691451,-229.35005));
#222318=CARTESIAN_POINT('',(0.5,2.29555713691451,-235.35005));
#222319=CARTESIAN_POINT('Origin',(1.25,2.29555713691451,-229.35005));
#222320=CARTESIAN_POINT('Origin',(1.25,-25.3025207885872,-192.281986444803));
#222321=CARTESIAN_POINT('',(0.5,-25.3025207885872,-229.35005));
#222322=CARTESIAN_POINT('',(0.5,-25.3025207885872,-235.35005));
#222323=CARTESIAN_POINT('',(1.18233753211584,-24.5555791640676,-229.35005));
#222324=CARTESIAN_POINT('',(1.18233753211584,-24.5555791640676,-192.281986444803));
#222325=CARTESIAN_POINT('Origin',(1.25,-25.3025207885872,-229.35005));
#222326=CARTESIAN_POINT('Origin',(1.25,-31.46456093117,-229.35005));
#222327=CARTESIAN_POINT('',(1.25,-32.21456093117,-229.35005));
#222328=CARTESIAN_POINT('',(1.25,-32.21456093117,-229.35005));
#222329=CARTESIAN_POINT('',(0.5,-31.46456093117,-229.35005));
#222330=CARTESIAN_POINT('',(0.5,-31.46456093117,-235.35005));
#222331=CARTESIAN_POINT('Origin',(1.25,-31.46456093117,-229.35005));
#222332=CARTESIAN_POINT('Origin',(8.87499999999984,-31.46456093117,-229.35005));
#222333=CARTESIAN_POINT('',(9.62499999999984,-31.46456093117,-229.35005));
#222334=CARTESIAN_POINT('',(9.62499999999984,-31.46456093117,-235.35005));
#222335=CARTESIAN_POINT('',(8.87499999999984,-32.21456093117,-229.35005));
#222336=CARTESIAN_POINT('',(8.87499999999984,-32.21456093117,-229.35005));
#222337=CARTESIAN_POINT('Origin',(8.87499999999984,-31.46456093117,-229.35005));
#222338=CARTESIAN_POINT('Origin',(31.625,21.5631368321642,-229.35005));
#222339=CARTESIAN_POINT('',(31.625,20.8131368321642,-229.35005));
#222340=CARTESIAN_POINT('',(31.625,20.8131368321642,-229.35005));
#222341=CARTESIAN_POINT('',(30.875,21.5631368321642,-229.35005));
#222342=CARTESIAN_POINT('',(30.875,21.5631368321642,-235.35005));
#222343=CARTESIAN_POINT('Origin',(31.625,21.5631368321642,-229.35005));
#222344=CARTESIAN_POINT('Origin',(33.751462642771,21.5631368321642,-229.35005));
#222345=CARTESIAN_POINT('',(34.2872001450371,22.0880037949896,-229.35005));
#222346=CARTESIAN_POINT('',(34.2872001450371,22.0880037949896,-229.35005));
#222347=CARTESIAN_POINT('',(33.751462642771,20.8131368321642,-229.35005));
#222348=CARTESIAN_POINT('',(33.751462642771,20.8131368321642,-229.35005));
#222349=CARTESIAN_POINT('Origin',(33.751462642771,21.5631368321642,-229.35005));
#222350=CARTESIAN_POINT('Origin',(31.625,23.6023848491226,-229.35005));
#222351=CARTESIAN_POINT('',(30.875,23.6023848491226,-229.35005));
#222352=CARTESIAN_POINT('',(32.1269841269841,24.1596208280901,-229.35005));
#222353=CARTESIAN_POINT('Origin',(31.625,23.6023848491226,-229.35005));
#222354=CARTESIAN_POINT('',(30.875,23.6023848491226,-229.35005));
#222355=CARTESIAN_POINT('',(32.1269841269841,24.1596208280901,-229.35005));
#222356=CARTESIAN_POINT('Origin',(29.125,19.0631368321642,-229.35005));
#222357=CARTESIAN_POINT('',(29.125,19.8131368321642,-229.35005));
#222358=CARTESIAN_POINT('',(29.125,19.8131368321642,-229.35005));
#222359=CARTESIAN_POINT('',(29.875,19.0631368321642,-229.35005));
#222360=CARTESIAN_POINT('',(29.875,19.0631368321642,-235.35005));
#222361=CARTESIAN_POINT('Origin',(29.125,19.0631368321642,-229.35005));
#222362=CARTESIAN_POINT('Origin',(21.5,19.0631368321642,-229.35005));
#222363=CARTESIAN_POINT('',(20.75,19.0631368321642,-229.35005));
#222364=CARTESIAN_POINT('',(20.75,19.0631368321642,-235.35005));
#222365=CARTESIAN_POINT('',(21.5,19.8131368321642,-229.35005));
#222366=CARTESIAN_POINT('',(21.5,19.8131368321642,-229.35005));
#222367=CARTESIAN_POINT('Origin',(21.5,19.0631368321642,-229.35005));
#222368=CARTESIAN_POINT('Origin',(21.5,10.9575972794973,-229.35005));
#222369=CARTESIAN_POINT('',(21.5,10.2075972794973,-229.35005));
#222370=CARTESIAN_POINT('',(21.5,10.2075972794973,-229.35005));
#222371=CARTESIAN_POINT('',(20.75,10.9575972794973,-229.35005));
#222372=CARTESIAN_POINT('',(20.75,10.9575972794973,-235.35005));
#222373=CARTESIAN_POINT('Origin',(21.5,10.9575972794973,-229.35005));
#222374=CARTESIAN_POINT('Origin',(29.125,10.9575972794973,-229.35005));
#222375=CARTESIAN_POINT('',(29.875,10.9575972794973,-229.35005));
#222376=CARTESIAN_POINT('',(29.875,10.9575972794973,-235.35005));
#222377=CARTESIAN_POINT('',(29.125,10.2075972794973,-229.35005));
#222378=CARTESIAN_POINT('',(29.125,10.2075972794973,-229.35005));
#222379=CARTESIAN_POINT('Origin',(29.125,10.9575972794973,-229.35005));
#222380=CARTESIAN_POINT('Origin',(29.125,8.45759727949731,-229.35005));
#222381=CARTESIAN_POINT('',(29.125,9.20759727949731,-229.35005));
#222382=CARTESIAN_POINT('',(29.125,9.20759727949731,-229.35005));
#222383=CARTESIAN_POINT('',(29.875,8.45759727949731,-229.35005));
#222384=CARTESIAN_POINT('',(29.875,8.45759727949731,-235.35005));
#222385=CARTESIAN_POINT('Origin',(29.125,8.45759727949731,-229.35005));
#222386=CARTESIAN_POINT('Origin',(21.5,8.45759727949731,-229.35005));
#222387=CARTESIAN_POINT('',(20.75,8.45759727949731,-229.35005));
#222388=CARTESIAN_POINT('',(20.75,8.45759727949731,-235.35005));
#222389=CARTESIAN_POINT('',(21.5,9.20759727949731,-229.35005));
#222390=CARTESIAN_POINT('',(21.5,9.20759727949731,-229.35005));
#222391=CARTESIAN_POINT('Origin',(21.5,8.45759727949731,-229.35005));
#222392=CARTESIAN_POINT('Origin',(21.5,0.35205772683049,-229.35005));
#222393=CARTESIAN_POINT('',(21.5,-0.39794227316951,-229.35005));
#222394=CARTESIAN_POINT('',(21.5,-0.39794227316951,-229.35005));
#222395=CARTESIAN_POINT('',(20.75,0.352057726830487,-229.35005));
#222396=CARTESIAN_POINT('',(20.75,0.352057726830487,-235.35005));
#222397=CARTESIAN_POINT('Origin',(21.5,0.35205772683049,-229.35005));
#222398=CARTESIAN_POINT('Origin',(29.125,0.352057726830493,-229.35005));
#222399=CARTESIAN_POINT('',(29.875,0.352057726830494,-229.35005));
#222400=CARTESIAN_POINT('',(29.875,0.352057726830494,-235.35005));
#222401=CARTESIAN_POINT('',(29.125,-0.397942273169507,-229.35005));
#222402=CARTESIAN_POINT('',(29.125,-0.397942273169507,-229.35005));
#222403=CARTESIAN_POINT('Origin',(29.125,0.352057726830493,-229.35005));
#222404=CARTESIAN_POINT('Origin',(29.125,-44.5701004838368,-229.35005));
#222405=CARTESIAN_POINT('',(29.125,-43.8201004838368,-229.35005));
#222406=CARTESIAN_POINT('',(29.125,-43.8201004838368,-229.35005));
#222407=CARTESIAN_POINT('',(29.875,-44.5701004838368,-229.35005));
#222408=CARTESIAN_POINT('',(29.875,-44.5701004838368,-235.35005));
#222409=CARTESIAN_POINT('Origin',(29.125,-44.5701004838368,-229.35005));
#222410=CARTESIAN_POINT('Origin',(21.5,-44.5701004838368,-229.35005));
#222411=CARTESIAN_POINT('',(20.75,-44.5701004838368,-229.35005));
#222412=CARTESIAN_POINT('',(20.75,-44.5701004838368,-235.35005));
#222413=CARTESIAN_POINT('',(21.5,-43.8201004838368,-229.35005));
#222414=CARTESIAN_POINT('',(21.5,-43.8201004838368,-229.35005));
#222415=CARTESIAN_POINT('Origin',(21.5,-44.5701004838368,-229.35005));
#222416=CARTESIAN_POINT('Origin',(21.5,-52.8339989151841,-229.35005));
#222417=CARTESIAN_POINT('',(21.5238294101153,-53.5836202590728,-229.35005));
#222418=CARTESIAN_POINT('',(21.5238294101154,-53.5836202590729,-229.35005));
#222419=CARTESIAN_POINT('',(20.75,-52.8339989151841,-229.35005));
#222420=CARTESIAN_POINT('',(20.75,-52.8339989151841,-235.35005));
#222421=CARTESIAN_POINT('Origin',(21.5,-52.8339989151841,-229.35005));
#222422=CARTESIAN_POINT('Origin',(29.125,-48.7096221120845,-229.35005));
#222423=CARTESIAN_POINT('',(29.875,-48.7096221120845,-229.35005));
#222424=CARTESIAN_POINT('',(29.875,-48.7096221120845,-229.35005));
#222425=CARTESIAN_POINT('',(29.5873015873016,-49.3001957674217,-229.35005));
#222426=CARTESIAN_POINT('',(29.5873015873016,-49.3001957674217,-229.35005));
#222427=CARTESIAN_POINT('Origin',(29.125,-48.7096221120845,-229.35005));
#222428=CARTESIAN_POINT('Origin',(31.625,-42.0701004838368,-229.35005));
#222429=CARTESIAN_POINT('',(31.625,-42.8201004838368,-229.35005));
#222430=CARTESIAN_POINT('',(31.625,-42.8201004838368,-229.35005));
#222431=CARTESIAN_POINT('',(30.875,-42.0701004838368,-229.35005));
#222432=CARTESIAN_POINT('',(30.875,-42.0701004838368,-235.35005));
#222433=CARTESIAN_POINT('Origin',(31.625,-42.0701004838368,-229.35005));
#222434=CARTESIAN_POINT('Origin',(36.0311576807678,-42.0701004838368,-229.35005));
#222435=CARTESIAN_POINT('',(36.6030808185578,-42.5552849069797,-229.35005));
#222436=CARTESIAN_POINT('',(36.6030808185578,-42.5552849069797,-229.35005));
#222437=CARTESIAN_POINT('',(36.0311576807678,-42.8201004838368,-229.35005));
#222438=CARTESIAN_POINT('',(36.0311576807678,-42.8201004838368,-229.35005));
#222439=CARTESIAN_POINT('Origin',(36.0311576807678,-42.0701004838368,-229.35005));
#222440=CARTESIAN_POINT('Origin',(39.3771239584772,-33.96456093117,-229.35005));
#222441=CARTESIAN_POINT('',(39.3771239584772,-33.21456093117,-229.35005));
#222442=CARTESIAN_POINT('',(39.3771239584772,-33.21456093117,-229.35005));
#222443=CARTESIAN_POINT('',(40.1267106833091,-33.9894555481763,-229.35005));
#222444=CARTESIAN_POINT('',(40.1267106833092,-33.9894555481763,-229.35005));
#222445=CARTESIAN_POINT('Origin',(39.3771239584772,-33.96456093117,-229.35005));
#222446=CARTESIAN_POINT('Origin',(31.625,-33.96456093117,-229.35005));
#222447=CARTESIAN_POINT('',(30.875,-33.96456093117,-229.35005));
#222448=CARTESIAN_POINT('',(30.875,-33.96456093117,-235.35005));
#222449=CARTESIAN_POINT('',(31.625,-33.21456093117,-229.35005));
#222450=CARTESIAN_POINT('',(31.625,-33.21456093117,-229.35005));
#222451=CARTESIAN_POINT('Origin',(31.625,-33.96456093117,-229.35005));
#222452=CARTESIAN_POINT('Origin',(29.125,-2.14794227316952,-229.35005));
#222453=CARTESIAN_POINT('',(29.125,-1.39794227316951,-229.35005));
#222454=CARTESIAN_POINT('',(29.125,-1.39794227316951,-229.35005));
#222455=CARTESIAN_POINT('',(29.875,-2.14794227316951,-229.35005));
#222456=CARTESIAN_POINT('',(29.875,-2.14794227316951,-235.35005));
#222457=CARTESIAN_POINT('Origin',(29.125,-2.14794227316952,-229.35005));
#222458=CARTESIAN_POINT('Origin',(21.5,-2.14794227316951,-229.35005));
#222459=CARTESIAN_POINT('',(20.75,-2.14794227316951,-229.35005));
#222460=CARTESIAN_POINT('',(20.75,-2.14794227316951,-235.35005));
#222461=CARTESIAN_POINT('',(21.5,-1.39794227316951,-229.35005));
#222462=CARTESIAN_POINT('',(21.5,-1.39794227316951,-229.35005));
#222463=CARTESIAN_POINT('Origin',(21.5,-2.14794227316951,-229.35005));
#222464=CARTESIAN_POINT('Origin',(21.5,-10.2534818258363,-229.35005));
#222465=CARTESIAN_POINT('',(21.5,-11.0034818258363,-229.35005));
#222466=CARTESIAN_POINT('',(21.5,-11.0034818258363,-229.35005));
#222467=CARTESIAN_POINT('',(20.75,-10.2534818258363,-229.35005));
#222468=CARTESIAN_POINT('',(20.75,-10.2534818258363,-235.35005));
#222469=CARTESIAN_POINT('Origin',(21.5,-10.2534818258363,-229.35005));
#222470=CARTESIAN_POINT('Origin',(29.125,-10.2534818258363,-229.35005));
#222471=CARTESIAN_POINT('',(29.875,-10.2534818258363,-229.35005));
#222472=CARTESIAN_POINT('',(29.875,-10.2534818258363,-235.35005));
#222473=CARTESIAN_POINT('',(29.125,-11.0034818258363,-229.35005));
#222474=CARTESIAN_POINT('',(29.125,-11.0034818258363,-229.35005));
#222475=CARTESIAN_POINT('Origin',(29.125,-10.2534818258363,-229.35005));
#222476=CARTESIAN_POINT('Origin',(29.125,-12.7534818258363,-229.35005));
#222477=CARTESIAN_POINT('',(29.125,-12.0034818258363,-229.35005));
#222478=CARTESIAN_POINT('',(29.125,-12.0034818258363,-229.35005));
#222479=CARTESIAN_POINT('',(29.875,-12.7534818258363,-229.35005));
#222480=CARTESIAN_POINT('',(29.875,-12.7534818258363,-235.35005));
#222481=CARTESIAN_POINT('Origin',(29.125,-12.7534818258363,-229.35005));
#222482=CARTESIAN_POINT('Origin',(21.5,-12.7534818258363,-229.35005));
#222483=CARTESIAN_POINT('',(20.75,-12.7534818258363,-229.35005));
#222484=CARTESIAN_POINT('',(20.75,-12.7534818258363,-235.35005));
#222485=CARTESIAN_POINT('',(21.5,-12.0034818258363,-229.35005));
#222486=CARTESIAN_POINT('',(21.5,-12.0034818258363,-229.35005));
#222487=CARTESIAN_POINT('Origin',(21.5,-12.7534818258363,-229.35005));
#222488=CARTESIAN_POINT('Origin',(21.5,-20.8590213785032,-229.35005));
#222489=CARTESIAN_POINT('',(21.5,-21.6090213785031,-229.35005));
#222490=CARTESIAN_POINT('',(21.5,-21.6090213785031,-229.35005));
#222491=CARTESIAN_POINT('',(20.75,-20.8590213785032,-229.35005));
#222492=CARTESIAN_POINT('',(20.75,-20.8590213785032,-235.35005));
#222493=CARTESIAN_POINT('Origin',(21.5,-20.8590213785032,-229.35005));
#222494=CARTESIAN_POINT('Origin',(29.125,-20.8590213785032,-229.35005));
#222495=CARTESIAN_POINT('',(29.875,-20.8590213785032,-229.35005));
#222496=CARTESIAN_POINT('',(29.875,-20.8590213785032,-235.35005));
#222497=CARTESIAN_POINT('',(29.125,-21.6090213785031,-229.35005));
#222498=CARTESIAN_POINT('',(29.125,-21.6090213785031,-229.35005));
#222499=CARTESIAN_POINT('Origin',(29.125,-20.8590213785032,-229.35005));
#222500=CARTESIAN_POINT('Origin',(29.125,-23.3590213785032,-229.35005));
#222501=CARTESIAN_POINT('',(29.125,-22.6090213785032,-229.35005));
#222502=CARTESIAN_POINT('',(29.125,-22.6090213785032,-229.35005));
#222503=CARTESIAN_POINT('',(29.875,-23.3590213785032,-229.35005));
#222504=CARTESIAN_POINT('',(29.875,-23.3590213785032,-235.35005));
#222505=CARTESIAN_POINT('Origin',(29.125,-23.3590213785032,-229.35005));
#222506=CARTESIAN_POINT('Origin',(21.5,-23.3590213785032,-229.35005));
#222507=CARTESIAN_POINT('',(20.75,-23.3590213785032,-229.35005));
#222508=CARTESIAN_POINT('',(20.75,-23.3590213785032,-235.35005));
#222509=CARTESIAN_POINT('',(21.5,-22.6090213785032,-229.35005));
#222510=CARTESIAN_POINT('',(21.5,-22.6090213785032,-229.35005));
#222511=CARTESIAN_POINT('Origin',(21.5,-23.3590213785032,-229.35005));
#222512=CARTESIAN_POINT('Origin',(21.5,-31.46456093117,-229.35005));
#222513=CARTESIAN_POINT('',(21.5,-32.21456093117,-229.35005));
#222514=CARTESIAN_POINT('',(21.5,-32.21456093117,-229.35005));
#222515=CARTESIAN_POINT('',(20.75,-31.46456093117,-229.35005));
#222516=CARTESIAN_POINT('',(20.75,-31.46456093117,-235.35005));
#222517=CARTESIAN_POINT('Origin',(21.5,-31.46456093117,-229.35005));
#222518=CARTESIAN_POINT('Origin',(29.125,-31.46456093117,-229.35005));
#222519=CARTESIAN_POINT('',(29.875,-31.46456093117,-229.35005));
#222520=CARTESIAN_POINT('',(29.875,-31.46456093117,-235.35005));
#222521=CARTESIAN_POINT('',(29.125,-32.21456093117,-229.35005));
#222522=CARTESIAN_POINT('',(29.125,-32.21456093117,-229.35005));
#222523=CARTESIAN_POINT('Origin',(29.125,-31.46456093117,-229.35005));
#222524=CARTESIAN_POINT('Origin',(31.625,-44.5701004838368,-229.35005));
#222525=CARTESIAN_POINT('',(30.875,-44.5701004838368,-229.35005));
#222526=CARTESIAN_POINT('',(30.875,-44.5701004838368,-235.35005));
#222527=CARTESIAN_POINT('',(31.625,-43.8201004838368,-229.35005));
#222528=CARTESIAN_POINT('',(31.625,-43.8201004838368,-229.35005));
#222529=CARTESIAN_POINT('Origin',(31.625,-44.5701004838368,-229.35005));
#222530=CARTESIAN_POINT('Origin',(31.625,-46.609348500795,-229.35005));
#222531=CARTESIAN_POINT('',(32.1269841269841,-47.1665844797626,-229.35005));
#222532=CARTESIAN_POINT('',(32.1269841269841,-47.1665844797626,-229.35005));
#222533=CARTESIAN_POINT('',(30.875,-46.609348500795,-229.35005));
#222534=CARTESIAN_POINT('',(30.875,-46.609348500795,-235.35005));
#222535=CARTESIAN_POINT('Origin',(31.625,-46.609348500795,-229.35005));
#222536=CARTESIAN_POINT('Origin',(33.7514626427707,-44.5701004838368,-229.35005));
#222537=CARTESIAN_POINT('',(33.7514626427707,-43.8201004838368,-229.35005));
#222538=CARTESIAN_POINT('',(33.7514626427707,-43.8201004838368,-229.35005));
#222539=CARTESIAN_POINT('',(34.2872001450369,-45.0949674466622,-229.35005));
#222540=CARTESIAN_POINT('',(34.2872001450369,-45.0949674466622,-229.35005));
#222541=CARTESIAN_POINT('Origin',(33.7514626427707,-44.5701004838368,-229.35005));
#222542=CARTESIAN_POINT('Origin',(29.125,-42.0701004838368,-229.35005));
#222543=CARTESIAN_POINT('',(29.875,-42.0701004838368,-229.35005));
#222544=CARTESIAN_POINT('',(29.875,-42.0701004838368,-235.35005));
#222545=CARTESIAN_POINT('',(29.125,-42.8201004838368,-229.35005));
#222546=CARTESIAN_POINT('',(29.125,-42.8201004838368,-229.35005));
#222547=CARTESIAN_POINT('Origin',(29.125,-42.0701004838368,-229.35005));
#222548=CARTESIAN_POINT('Origin',(29.125,-33.96456093117,-229.35005));
#222549=CARTESIAN_POINT('',(29.125,-33.21456093117,-229.35005));
#222550=CARTESIAN_POINT('',(29.125,-33.21456093117,-229.35005));
#222551=CARTESIAN_POINT('',(29.875,-33.96456093117,-229.35005));
#222552=CARTESIAN_POINT('',(29.875,-33.96456093117,-235.35005));
#222553=CARTESIAN_POINT('Origin',(29.125,-33.96456093117,-229.35005));
#222554=CARTESIAN_POINT('Origin',(21.5,-33.96456093117,-229.35005));
#222555=CARTESIAN_POINT('',(20.75,-33.96456093117,-229.35005));
#222556=CARTESIAN_POINT('',(20.75,-33.96456093117,-235.35005));
#222557=CARTESIAN_POINT('',(21.5,-33.21456093117,-229.35005));
#222558=CARTESIAN_POINT('',(21.5,-33.21456093117,-229.35005));
#222559=CARTESIAN_POINT('Origin',(21.5,-33.96456093117,-229.35005));
#222560=CARTESIAN_POINT('Origin',(21.5,-42.0701004838368,-229.35005));
#222561=CARTESIAN_POINT('',(21.5,-42.8201004838368,-229.35005));
#222562=CARTESIAN_POINT('',(21.5,-42.8201004838368,-229.35005));
#222563=CARTESIAN_POINT('',(20.75,-42.0701004838368,-229.35005));
#222564=CARTESIAN_POINT('',(20.75,-42.0701004838368,-235.35005));
#222565=CARTESIAN_POINT('Origin',(21.5,-42.0701004838368,-229.35005));
#222566=CARTESIAN_POINT('Origin',(31.625,-23.3590213785032,-229.35005));
#222567=CARTESIAN_POINT('',(30.875,-23.3590213785032,-229.35005));
#222568=CARTESIAN_POINT('',(30.875,-23.3590213785032,-235.35005));
#222569=CARTESIAN_POINT('',(31.625,-22.6090213785032,-229.35005));
#222570=CARTESIAN_POINT('',(31.625,-22.6090213785032,-229.35005));
#222571=CARTESIAN_POINT('Origin',(31.625,-23.3590213785032,-229.35005));
#222572=CARTESIAN_POINT('Origin',(31.625,-31.46456093117,-229.35005));
#222573=CARTESIAN_POINT('',(31.625,-32.21456093117,-229.35005));
#222574=CARTESIAN_POINT('',(31.625,-32.21456093117,-229.35005));
#222575=CARTESIAN_POINT('',(30.875,-31.46456093117,-229.35005));
#222576=CARTESIAN_POINT('',(30.875,-31.46456093117,-235.35005));
#222577=CARTESIAN_POINT('Origin',(31.625,-31.46456093117,-229.35005));
#222578=CARTESIAN_POINT('Origin',(39.4555265729267,-31.46456093117,-229.35005));
#222579=CARTESIAN_POINT('',(40.2052001948773,-31.486684686535,-229.35005));
#222580=CARTESIAN_POINT('',(40.2052001948774,-31.486684686535,-229.35005));
#222581=CARTESIAN_POINT('',(39.4555265729267,-32.21456093117,-229.35005));
#222582=CARTESIAN_POINT('',(39.4555265729267,-32.21456093117,-229.35005));
#222583=CARTESIAN_POINT('Origin',(39.4555265729267,-31.46456093117,-229.35005));
#222584=CARTESIAN_POINT('Origin',(39.6461373136998,-23.3590213785032,-229.35005));
#222585=CARTESIAN_POINT('',(39.6461373136998,-22.6090213785032,-229.35005));
#222586=CARTESIAN_POINT('',(39.6461373136998,-22.6090213785032,-229.35005));
#222587=CARTESIAN_POINT('',(40.3960221980464,-23.3721614024167,-229.35005));
#222588=CARTESIAN_POINT('',(40.3960221980465,-23.3721614024167,-229.35005));
#222589=CARTESIAN_POINT('Origin',(39.6461373136998,-23.3590213785032,-229.35005));
#222590=CARTESIAN_POINT('Origin',(31.625,-12.7534818258363,-229.35005));
#222591=CARTESIAN_POINT('',(30.875,-12.7534818258363,-229.35005));
#222592=CARTESIAN_POINT('',(30.875,-12.7534818258363,-235.35005));
#222593=CARTESIAN_POINT('',(31.625,-12.0034818258363,-229.35005));
#222594=CARTESIAN_POINT('',(31.625,-12.0034818258363,-229.35005));
#222595=CARTESIAN_POINT('Origin',(31.625,-12.7534818258363,-229.35005));
#222596=CARTESIAN_POINT('Origin',(31.625,-20.8590213785032,-229.35005));
#222597=CARTESIAN_POINT('',(31.625,-21.6090213785031,-229.35005));
#222598=CARTESIAN_POINT('',(31.625,-21.6090213785031,-229.35005));
#222599=CARTESIAN_POINT('',(30.875,-20.8590213785032,-229.35005));
#222600=CARTESIAN_POINT('',(30.875,-20.8590213785032,-235.35005));
#222601=CARTESIAN_POINT('Origin',(31.625,-20.8590213785032,-229.35005));
#222602=CARTESIAN_POINT('Origin',(39.6853241707135,-20.8590213785032,-229.35005));
#222603=CARTESIAN_POINT('',(40.4352524876037,-20.8693905407753,-229.35005));
#222604=CARTESIAN_POINT('',(40.4352524876037,-20.8693905407753,-229.35005));
#222605=CARTESIAN_POINT('',(39.6853241707135,-21.6090213785031,-229.35005));
#222606=CARTESIAN_POINT('',(39.6853241707135,-21.6090213785031,-229.35005));
#222607=CARTESIAN_POINT('Origin',(39.6853241707135,-20.8590213785032,-229.35005));
#222608=CARTESIAN_POINT('Origin',(39.7488454733312,-12.7534818258363,-229.35005));
#222609=CARTESIAN_POINT('',(39.7488454733312,-12.0034818258363,-229.35005));
#222610=CARTESIAN_POINT('',(39.7488454733312,-12.0034818258363,-229.35005));
#222611=CARTESIAN_POINT('',(40.4988441937178,-12.754867256657,-229.35005));
#222612=CARTESIAN_POINT('',(40.4988441937178,-12.754867256657,-229.35005));
#222613=CARTESIAN_POINT('Origin',(39.7488454733312,-12.7534818258363,-229.35005));
#222614=CARTESIAN_POINT('Origin',(31.625,-2.14794227316952,-229.35005));
#222615=CARTESIAN_POINT('',(30.875,-2.14794227316951,-229.35005));
#222616=CARTESIAN_POINT('',(30.875,-2.14794227316951,-235.35005));
#222617=CARTESIAN_POINT('',(31.625,-1.39794227316951,-229.35005));
#222618=CARTESIAN_POINT('',(31.625,-1.39794227316951,-229.35005));
#222619=CARTESIAN_POINT('Origin',(31.625,-2.14794227316952,-229.35005));
#222620=CARTESIAN_POINT('Origin',(31.625,-10.2534818258363,-229.35005));
#222621=CARTESIAN_POINT('',(31.625,-11.0034818258363,-229.35005));
#222622=CARTESIAN_POINT('',(31.625,-11.0034818258363,-229.35005));
#222623=CARTESIAN_POINT('',(30.875,-10.2534818258363,-229.35005));
#222624=CARTESIAN_POINT('',(30.875,-10.2534818258363,-235.35005));
#222625=CARTESIAN_POINT('Origin',(31.625,-10.2534818258363,-229.35005));
#222626=CARTESIAN_POINT('Origin',(39.7488454733312,-10.2534818258363,-229.35005));
#222627=CARTESIAN_POINT('',(40.4988441937178,-10.2520963950157,-229.35005));
#222628=CARTESIAN_POINT('',(40.4988441937178,-10.2520963950157,-229.35005));
#222629=CARTESIAN_POINT('',(39.7488454733312,-11.0034818258363,-229.35005));
#222630=CARTESIAN_POINT('',(39.7488454733312,-11.0034818258363,-229.35005));
#222631=CARTESIAN_POINT('Origin',(39.7488454733312,-10.2534818258363,-229.35005));
#222632=CARTESIAN_POINT('Origin',(39.6853241707135,-2.14794227316952,-229.35005));
#222633=CARTESIAN_POINT('',(39.6853241707135,-1.39794227316952,-229.35005));
#222634=CARTESIAN_POINT('',(39.6853241707135,-1.39794227316952,-229.35005));
#222635=CARTESIAN_POINT('',(40.4352524876037,-2.13757311089736,-229.35005));
#222636=CARTESIAN_POINT('',(40.4352524876037,-2.13757311089736,-229.35005));
#222637=CARTESIAN_POINT('Origin',(39.6853241707135,-2.14794227316952,-229.35005));
#222638=CARTESIAN_POINT('Origin',(31.625,8.45759727949731,-229.35005));
#222639=CARTESIAN_POINT('',(30.875,8.45759727949731,-229.35005));
#222640=CARTESIAN_POINT('',(30.875,8.45759727949731,-235.35005));
#222641=CARTESIAN_POINT('',(31.625,9.20759727949731,-229.35005));
#222642=CARTESIAN_POINT('',(31.625,9.20759727949731,-229.35005));
#222643=CARTESIAN_POINT('Origin',(31.625,8.45759727949731,-229.35005));
#222644=CARTESIAN_POINT('Origin',(31.625,0.352057726830494,-229.35005));
#222645=CARTESIAN_POINT('',(31.625,-0.397942273169506,-229.35005));
#222646=CARTESIAN_POINT('',(31.625,-0.397942273169506,-229.35005));
#222647=CARTESIAN_POINT('',(30.875,0.352057726830494,-229.35005));
#222648=CARTESIAN_POINT('',(30.875,0.352057726830494,-235.35005));
#222649=CARTESIAN_POINT('Origin',(31.625,0.352057726830494,-229.35005));
#222650=CARTESIAN_POINT('Origin',(39.6461373136998,0.352057726830498,-229.35005));
#222651=CARTESIAN_POINT('',(40.3960221980465,0.365197750743975,-229.35005));
#222652=CARTESIAN_POINT('',(40.3960221980464,0.365197750743973,-229.35005));
#222653=CARTESIAN_POINT('',(39.6461373136998,-0.397942273169503,-229.35005));
#222654=CARTESIAN_POINT('',(39.6461373136998,-0.397942273169503,-229.35005));
#222655=CARTESIAN_POINT('Origin',(39.6461373136998,0.352057726830498,-229.35005));
#222656=CARTESIAN_POINT('Origin',(39.4555265729267,8.45759727949731,-229.35005));
#222657=CARTESIAN_POINT('',(39.4555265729267,9.20759727949731,-229.35005));
#222658=CARTESIAN_POINT('',(39.4555265729267,9.20759727949731,-229.35005));
#222659=CARTESIAN_POINT('',(40.2052001948774,8.47972103486228,-229.35005));
#222660=CARTESIAN_POINT('',(40.2052001948774,8.47972103486227,-229.35005));
#222661=CARTESIAN_POINT('Origin',(39.4555265729267,8.45759727949731,-229.35005));
#222662=CARTESIAN_POINT('Origin',(31.625,19.0631368321642,-229.35005));
#222663=CARTESIAN_POINT('',(30.875,19.0631368321642,-229.35005));
#222664=CARTESIAN_POINT('',(30.875,19.0631368321642,-235.35005));
#222665=CARTESIAN_POINT('',(31.625,19.8131368321642,-229.35005));
#222666=CARTESIAN_POINT('',(31.625,19.8131368321642,-229.35005));
#222667=CARTESIAN_POINT('Origin',(31.625,19.0631368321642,-229.35005));
#222668=CARTESIAN_POINT('Origin',(31.625,10.9575972794973,-229.35005));
#222669=CARTESIAN_POINT('',(31.625,10.2075972794973,-229.35005));
#222670=CARTESIAN_POINT('',(31.625,10.2075972794973,-229.35005));
#222671=CARTESIAN_POINT('',(30.875,10.9575972794973,-229.35005));
#222672=CARTESIAN_POINT('',(30.875,10.9575972794973,-235.35005));
#222673=CARTESIAN_POINT('Origin',(31.625,10.9575972794973,-229.35005));
#222674=CARTESIAN_POINT('Origin',(39.3771239584772,10.9575972794973,-229.35005));
#222675=CARTESIAN_POINT('',(40.1267106833092,10.9824918965036,-229.35005));
#222676=CARTESIAN_POINT('',(40.1267106833092,10.9824918965036,-229.35005));
#222677=CARTESIAN_POINT('',(39.3771239584772,10.2075972794973,-229.35005));
#222678=CARTESIAN_POINT('',(39.3771239584772,10.2075972794973,-229.35005));
#222679=CARTESIAN_POINT('Origin',(39.3771239584772,10.9575972794973,-229.35005));
#222680=CARTESIAN_POINT('Origin',(36.0311576807679,19.0631368321642,-229.35005));
#222681=CARTESIAN_POINT('',(36.0311576807679,19.8131368321642,-229.35005));
#222682=CARTESIAN_POINT('',(36.0311576807679,19.8131368321642,-229.35005));
#222683=CARTESIAN_POINT('',(36.6030808185579,19.548321255307,-229.35005));
#222684=CARTESIAN_POINT('',(36.6030808185579,19.548321255307,-229.35005));
#222685=CARTESIAN_POINT('Origin',(36.0311576807679,19.0631368321642,-229.35005));
#222686=CARTESIAN_POINT('Origin',(29.125,21.5631368321642,-229.35005));
#222687=CARTESIAN_POINT('',(29.875,21.5631368321642,-229.35005));
#222688=CARTESIAN_POINT('',(29.875,21.5631368321642,-235.35005));
#222689=CARTESIAN_POINT('',(29.125,20.8131368321642,-229.35005));
#222690=CARTESIAN_POINT('',(29.125,20.8131368321642,-229.35005));
#222691=CARTESIAN_POINT('Origin',(29.125,21.5631368321642,-229.35005));
#222692=CARTESIAN_POINT('Origin',(29.125,25.702658460412,-229.35005));
#222693=CARTESIAN_POINT('',(29.5873015873016,26.2932321157492,-229.35005));
#222694=CARTESIAN_POINT('',(29.5873015873016,26.2932321157492,-229.35005));
#222695=CARTESIAN_POINT('',(29.875,25.702658460412,-229.35005));
#222696=CARTESIAN_POINT('',(29.875,25.702658460412,-235.35005));
#222697=CARTESIAN_POINT('Origin',(29.125,25.702658460412,-229.35005));
#222698=CARTESIAN_POINT('Origin',(21.5,29.0311209585238,-229.35005));
#222699=CARTESIAN_POINT('',(20.75,29.0311209585238,-229.35005));
#222700=CARTESIAN_POINT('',(21.5791427781145,29.776933549375,-229.35005));
#222701=CARTESIAN_POINT('Origin',(21.5,29.0311209585238,-229.35005));
#222702=CARTESIAN_POINT('',(20.75,29.0311209585238,-229.35005));
#222703=CARTESIAN_POINT('',(21.5791427781145,29.7769335493751,-229.35005));
#222704=CARTESIAN_POINT('Origin',(21.5,21.5631368321642,-229.35005));
#222705=CARTESIAN_POINT('',(21.5,20.8131368321642,-229.35005));
#222706=CARTESIAN_POINT('',(21.5,20.8131368321642,-229.35005));
#222707=CARTESIAN_POINT('',(20.75,21.5631368321642,-229.35005));
#222708=CARTESIAN_POINT('',(20.75,21.5631368321642,-235.35005));
#222709=CARTESIAN_POINT('Origin',(21.5,21.5631368321642,-229.35005));
#222710=CARTESIAN_POINT('Origin',(19.,-52.9088458284789,-229.35005));
#222711=CARTESIAN_POINT('',(19.75,-52.9088458284789,-229.35005));
#222712=CARTESIAN_POINT('',(19.75,-52.9088458284789,-229.35005));
#222713=CARTESIAN_POINT('',(19.021058548474,-53.658550128544,-229.35005));
#222714=CARTESIAN_POINT('',(19.021058548474,-53.6585501285442,-229.35005));
#222715=CARTESIAN_POINT('Origin',(19.,-52.9088458284789,-229.35005));
#222716=CARTESIAN_POINT('Origin',(19.,-44.5701004838368,-229.35005));
#222717=CARTESIAN_POINT('',(19.,-43.8201004838368,-229.35005));
#222718=CARTESIAN_POINT('',(19.,-43.8201004838368,-229.35005));
#222719=CARTESIAN_POINT('',(19.75,-44.5701004838368,-229.35005));
#222720=CARTESIAN_POINT('',(19.75,-44.5701004838368,-235.35005));
#222721=CARTESIAN_POINT('Origin',(19.,-44.5701004838368,-229.35005));
#222722=CARTESIAN_POINT('Origin',(11.3749999999999,-44.5701004838369,-229.35005));
#222723=CARTESIAN_POINT('',(10.6249999999999,-44.5701004838369,-229.35005));
#222724=CARTESIAN_POINT('',(10.6249999999999,-44.5701004838369,-235.35005));
#222725=CARTESIAN_POINT('',(11.3749999999999,-43.8201004838368,-229.35005));
#222726=CARTESIAN_POINT('',(11.3749999999999,-43.8201004838368,-229.35005));
#222727=CARTESIAN_POINT('Origin',(11.3749999999999,-44.5701004838369,-229.35005));
#222728=CARTESIAN_POINT('Origin',(11.3749999999999,-53.08002700974,-229.35005));
#222729=CARTESIAN_POINT('',(11.3876074204679,-53.8299210375528,-229.35005));
#222730=CARTESIAN_POINT('',(11.3876074204679,-53.8299210375529,-229.35005));
#222731=CARTESIAN_POINT('',(10.6249999999999,-53.08002700974,-229.35005));
#222732=CARTESIAN_POINT('',(10.6249999999999,-53.08002700974,-235.35005));
#222733=CARTESIAN_POINT('Origin',(11.3749999999999,-53.08002700974,-229.35005));
#222734=CARTESIAN_POINT('Origin',(19.,19.0631368321642,-229.35005));
#222735=CARTESIAN_POINT('',(19.,19.8131368321642,-229.35005));
#222736=CARTESIAN_POINT('',(19.,19.8131368321642,-229.35005));
#222737=CARTESIAN_POINT('',(19.75,19.0631368321642,-229.35005));
#222738=CARTESIAN_POINT('',(19.75,19.0631368321642,-235.35005));
#222739=CARTESIAN_POINT('Origin',(19.,19.0631368321642,-229.35005));
#222740=CARTESIAN_POINT('Origin',(11.3749999999999,19.0631368321642,-229.35005));
#222741=CARTESIAN_POINT('',(10.6249999999999,19.0631368321642,-229.35005));
#222742=CARTESIAN_POINT('',(10.6249999999999,19.0631368321642,-235.35005));
#222743=CARTESIAN_POINT('',(11.3749999999999,19.8131368321642,-229.35005));
#222744=CARTESIAN_POINT('',(11.3749999999999,19.8131368321642,-229.35005));
#222745=CARTESIAN_POINT('Origin',(11.3749999999999,19.0631368321642,-229.35005));
#222746=CARTESIAN_POINT('Origin',(11.3749999999999,10.9575972794973,-229.35005));
#222747=CARTESIAN_POINT('',(11.3749999999999,10.2075972794973,-229.35005));
#222748=CARTESIAN_POINT('',(11.3749999999999,10.2075972794973,-229.35005));
#222749=CARTESIAN_POINT('',(10.6249999999999,10.9575972794973,-229.35005));
#222750=CARTESIAN_POINT('',(10.6249999999999,10.9575972794973,-235.35005));
#222751=CARTESIAN_POINT('Origin',(11.3749999999999,10.9575972794973,-229.35005));
#222752=CARTESIAN_POINT('Origin',(19.,10.9575972794973,-229.35005));
#222753=CARTESIAN_POINT('',(19.75,10.9575972794973,-229.35005));
#222754=CARTESIAN_POINT('',(19.75,10.9575972794973,-235.35005));
#222755=CARTESIAN_POINT('',(19.,10.2075972794973,-229.35005));
#222756=CARTESIAN_POINT('',(19.,10.2075972794973,-229.35005));
#222757=CARTESIAN_POINT('Origin',(19.,10.9575972794973,-229.35005));
#222758=CARTESIAN_POINT('Origin',(19.,8.45759727949731,-229.35005));
#222759=CARTESIAN_POINT('',(19.,9.20759727949731,-229.35005));
#222760=CARTESIAN_POINT('',(19.,9.20759727949731,-229.35005));
#222761=CARTESIAN_POINT('',(19.75,8.45759727949731,-229.35005));
#222762=CARTESIAN_POINT('',(19.75,8.45759727949731,-235.35005));
#222763=CARTESIAN_POINT('Origin',(19.,8.45759727949731,-229.35005));
#222764=CARTESIAN_POINT('Origin',(11.3749999999999,8.45759727949731,-229.35005));
#222765=CARTESIAN_POINT('',(10.6249999999999,8.45759727949731,-229.35005));
#222766=CARTESIAN_POINT('',(10.6249999999999,8.45759727949731,-235.35005));
#222767=CARTESIAN_POINT('',(11.3749999999999,9.20759727949731,-229.35005));
#222768=CARTESIAN_POINT('',(11.3749999999999,9.20759727949731,-229.35005));
#222769=CARTESIAN_POINT('Origin',(11.3749999999999,8.45759727949731,-229.35005));
#222770=CARTESIAN_POINT('Origin',(11.3749999999999,0.352057726830486,-229.35005));
#222771=CARTESIAN_POINT('',(11.3749999999999,-0.397942273169514,-229.35005));
#222772=CARTESIAN_POINT('',(11.3749999999999,-0.397942273169514,-229.35005));
#222773=CARTESIAN_POINT('',(10.6249999999999,0.352057726830487,-229.35005));
#222774=CARTESIAN_POINT('',(10.6249999999999,0.352057726830487,-235.35005));
#222775=CARTESIAN_POINT('Origin',(11.3749999999999,0.352057726830486,-229.35005));
#222776=CARTESIAN_POINT('Origin',(19.,0.352057726830489,-229.35005));
#222777=CARTESIAN_POINT('',(19.75,0.352057726830487,-229.35005));
#222778=CARTESIAN_POINT('',(19.75,0.352057726830487,-235.35005));
#222779=CARTESIAN_POINT('',(19.,-0.397942273169511,-229.35005));
#222780=CARTESIAN_POINT('',(19.,-0.397942273169511,-229.35005));
#222781=CARTESIAN_POINT('Origin',(19.,0.352057726830489,-229.35005));
#222782=CARTESIAN_POINT('Origin',(19.,-23.3590213785032,-229.35005));
#222783=CARTESIAN_POINT('',(19.,-22.6090213785032,-229.35005));
#222784=CARTESIAN_POINT('',(19.,-22.6090213785032,-229.35005));
#222785=CARTESIAN_POINT('',(19.75,-23.3590213785032,-229.35005));
#222786=CARTESIAN_POINT('',(19.75,-23.3590213785032,-235.35005));
#222787=CARTESIAN_POINT('Origin',(19.,-23.3590213785032,-229.35005));
#222788=CARTESIAN_POINT('Origin',(11.3749999999999,-23.3590213785032,-229.35005));
#222789=CARTESIAN_POINT('',(10.6249999999999,-23.3590213785032,-229.35005));
#222790=CARTESIAN_POINT('',(10.6249999999999,-23.3590213785032,-235.35005));
#222791=CARTESIAN_POINT('',(11.3749999999999,-22.6090213785032,-229.35005));
#222792=CARTESIAN_POINT('',(11.3749999999999,-22.6090213785032,-229.35005));
#222793=CARTESIAN_POINT('Origin',(11.3749999999999,-23.3590213785032,-229.35005));
#222794=CARTESIAN_POINT('Origin',(11.3749999999999,-31.46456093117,-229.35005));
#222795=CARTESIAN_POINT('',(11.3749999999999,-32.21456093117,-229.35005));
#222796=CARTESIAN_POINT('',(11.3749999999999,-32.21456093117,-229.35005));
#222797=CARTESIAN_POINT('',(10.6249999999999,-31.46456093117,-229.35005));
#222798=CARTESIAN_POINT('',(10.6249999999999,-31.46456093117,-235.35005));
#222799=CARTESIAN_POINT('Origin',(11.3749999999999,-31.46456093117,-229.35005));
#222800=CARTESIAN_POINT('Origin',(19.,-31.46456093117,-229.35005));
#222801=CARTESIAN_POINT('',(19.75,-31.46456093117,-229.35005));
#222802=CARTESIAN_POINT('',(19.75,-31.46456093117,-235.35005));
#222803=CARTESIAN_POINT('',(19.,-32.21456093117,-229.35005));
#222804=CARTESIAN_POINT('',(19.,-32.21456093117,-229.35005));
#222805=CARTESIAN_POINT('Origin',(19.,-31.46456093117,-229.35005));
#222806=CARTESIAN_POINT('Origin',(19.,-42.0701004838368,-229.35005));
#222807=CARTESIAN_POINT('',(19.75,-42.0701004838368,-229.35005));
#222808=CARTESIAN_POINT('',(19.75,-42.0701004838368,-235.35005));
#222809=CARTESIAN_POINT('',(19.,-42.8201004838368,-229.35005));
#222810=CARTESIAN_POINT('',(19.,-42.8201004838368,-229.35005));
#222811=CARTESIAN_POINT('Origin',(19.,-42.0701004838368,-229.35005));
#222812=CARTESIAN_POINT('Origin',(19.,-33.96456093117,-229.35005));
#222813=CARTESIAN_POINT('',(19.,-33.21456093117,-229.35005));
#222814=CARTESIAN_POINT('',(19.,-33.21456093117,-229.35005));
#222815=CARTESIAN_POINT('',(19.75,-33.96456093117,-229.35005));
#222816=CARTESIAN_POINT('',(19.75,-33.96456093117,-235.35005));
#222817=CARTESIAN_POINT('Origin',(19.,-33.96456093117,-229.35005));
#222818=CARTESIAN_POINT('Origin',(11.3749999999999,-33.96456093117,-229.35005));
#222819=CARTESIAN_POINT('',(10.6249999999999,-33.96456093117,-229.35005));
#222820=CARTESIAN_POINT('',(10.6249999999999,-33.96456093117,-235.35005));
#222821=CARTESIAN_POINT('',(11.3749999999999,-33.21456093117,-229.35005));
#222822=CARTESIAN_POINT('',(11.3749999999999,-33.21456093117,-229.35005));
#222823=CARTESIAN_POINT('Origin',(11.3749999999999,-33.96456093117,-229.35005));
#222824=CARTESIAN_POINT('Origin',(11.3749999999999,-42.0701004838369,-229.35005));
#222825=CARTESIAN_POINT('',(11.3749999999999,-42.8201004838369,-229.35005));
#222826=CARTESIAN_POINT('',(11.3749999999999,-42.8201004838369,-229.35005));
#222827=CARTESIAN_POINT('',(10.6249999999999,-42.0701004838368,-229.35005));
#222828=CARTESIAN_POINT('',(10.6249999999999,-42.0701004838368,-235.35005));
#222829=CARTESIAN_POINT('Origin',(11.3749999999999,-42.0701004838369,-229.35005));
#222830=CARTESIAN_POINT('Origin',(19.,21.5631368321642,-229.35005));
#222831=CARTESIAN_POINT('',(19.75,21.5631368321642,-229.35005));
#222832=CARTESIAN_POINT('',(19.75,21.5631368321642,-235.35005));
#222833=CARTESIAN_POINT('',(19.,20.8131368321642,-229.35005));
#222834=CARTESIAN_POINT('',(19.,20.8131368321642,-229.35005));
#222835=CARTESIAN_POINT('Origin',(19.,21.5631368321642,-229.35005));
#222836=CARTESIAN_POINT('Origin',(19.,29.2808336449858,-229.35005));
#222837=CARTESIAN_POINT('',(19.0699401294965,30.0275654430807,-229.35005));
#222838=CARTESIAN_POINT('',(19.0699401294965,30.0275654430807,-229.35005));
#222839=CARTESIAN_POINT('',(19.75,29.2808336449858,-229.35005));
#222840=CARTESIAN_POINT('',(19.75,29.2808336449858,-235.35005));
#222841=CARTESIAN_POINT('Origin',(19.,29.2808336449858,-229.35005));
#222842=CARTESIAN_POINT('Origin',(11.3749999999999,29.8508988479304,-229.35005));
#222843=CARTESIAN_POINT('',(10.6249999999999,29.8508988479304,-229.35005));
#222844=CARTESIAN_POINT('',(11.4168720512116,30.5997290899261,-229.35005));
#222845=CARTESIAN_POINT('Origin',(11.3749999999999,29.8508988479304,-229.35005));
#222846=CARTESIAN_POINT('',(10.6249999999999,29.8508988479304,-229.35005));
#222847=CARTESIAN_POINT('',(11.4168720512116,30.5997290899261,-229.35005));
#222848=CARTESIAN_POINT('Origin',(11.3749999999999,21.5631368321642,-229.35005));
#222849=CARTESIAN_POINT('',(11.3749999999999,20.8131368321642,-229.35005));
#222850=CARTESIAN_POINT('',(11.3749999999999,20.8131368321642,-229.35005));
#222851=CARTESIAN_POINT('',(10.6249999999999,21.5631368321642,-229.35005));
#222852=CARTESIAN_POINT('',(10.6249999999999,21.5631368321642,-235.35005));
#222853=CARTESIAN_POINT('Origin',(11.3749999999999,21.5631368321642,-229.35005));
#222854=CARTESIAN_POINT('Origin',(8.87499999999984,-53.1174378937751,-229.35005));
#222855=CARTESIAN_POINT('',(9.62499999999984,-53.1174378937751,-229.35005));
#222856=CARTESIAN_POINT('',(9.62499999999984,-53.1174378937751,-229.35005));
#222857=CARTESIAN_POINT('',(8.88483655882654,-53.8673733857413,-229.35005));
#222858=CARTESIAN_POINT('',(8.88483655882654,-53.8673733857413,-229.35005));
#222859=CARTESIAN_POINT('Origin',(8.87499999999984,-53.1174378937751,-229.35005));
#222860=CARTESIAN_POINT('Origin',(8.87499999999984,-44.5701004838369,-229.35005));
#222861=CARTESIAN_POINT('',(8.87499999999984,-43.8201004838368,-229.35005));
#222862=CARTESIAN_POINT('',(8.87499999999984,-43.8201004838368,-229.35005));
#222863=CARTESIAN_POINT('',(9.62499999999984,-44.5701004838369,-229.35005));
#222864=CARTESIAN_POINT('',(9.62499999999984,-44.5701004838369,-235.35005));
#222865=CARTESIAN_POINT('Origin',(8.87499999999984,-44.5701004838369,-229.35005));
#222866=CARTESIAN_POINT('Origin',(1.25,-44.5701004838369,-229.35005));
#222867=CARTESIAN_POINT('',(0.5,-44.5701004838369,-229.35005));
#222868=CARTESIAN_POINT('',(0.5,-44.5701004838369,-235.35005));
#222869=CARTESIAN_POINT('',(1.25,-43.8201004838368,-229.35005));
#222870=CARTESIAN_POINT('',(1.25,-43.8201004838368,-229.35005));
#222871=CARTESIAN_POINT('Origin',(1.25,-44.5701004838369,-229.35005));
#222872=CARTESIAN_POINT('Origin',(1.25,-53.1744855098348,-229.35005));
#222873=CARTESIAN_POINT('',(1.25138543082066,-53.9244842302215,-229.35005));
#222874=CARTESIAN_POINT('',(1.25138543082066,-53.9244842302215,-229.35005));
#222875=CARTESIAN_POINT('',(0.5,-53.1744855098348,-229.35005));
#222876=CARTESIAN_POINT('',(0.5,-53.1744855098348,-235.35005));
#222877=CARTESIAN_POINT('Origin',(1.25,-53.1744855098348,-229.35005));
#222878=CARTESIAN_POINT('Origin',(8.87499999999986,19.0631368321642,-229.35005));
#222879=CARTESIAN_POINT('',(8.87499999999986,19.8131368321642,-229.35005));
#222880=CARTESIAN_POINT('',(8.87499999999986,19.8131368321642,-229.35005));
#222881=CARTESIAN_POINT('',(9.62499999999986,19.0631368321642,-229.35005));
#222882=CARTESIAN_POINT('',(9.62499999999986,19.0631368321642,-235.35005));
#222883=CARTESIAN_POINT('Origin',(8.87499999999986,19.0631368321642,-229.35005));
#222884=CARTESIAN_POINT('Origin',(1.25,19.0631368321642,-229.35005));
#222885=CARTESIAN_POINT('',(0.5,19.0631368321642,-229.35005));
#222886=CARTESIAN_POINT('',(0.5,19.0631368321642,-235.35005));
#222887=CARTESIAN_POINT('',(1.25,19.8131368321642,-229.35005));
#222888=CARTESIAN_POINT('',(1.25,19.8131368321642,-229.35005));
#222889=CARTESIAN_POINT('Origin',(1.25,19.0631368321642,-229.35005));
#222890=CARTESIAN_POINT('Origin',(1.25,10.9575972794973,-229.35005));
#222891=CARTESIAN_POINT('',(1.25,10.2075972794973,-229.35005));
#222892=CARTESIAN_POINT('',(1.25,10.2075972794973,-229.35005));
#222893=CARTESIAN_POINT('',(0.5,10.9575972794973,-229.35005));
#222894=CARTESIAN_POINT('',(0.5,10.9575972794973,-235.35005));
#222895=CARTESIAN_POINT('Origin',(1.25,10.9575972794973,-229.35005));
#222896=CARTESIAN_POINT('Origin',(8.87499999999986,10.9575972794973,-229.35005));
#222897=CARTESIAN_POINT('',(9.62499999999986,10.9575972794973,-229.35005));
#222898=CARTESIAN_POINT('',(9.62499999999986,10.9575972794973,-235.35005));
#222899=CARTESIAN_POINT('',(8.87499999999986,10.2075972794973,-229.35005));
#222900=CARTESIAN_POINT('',(8.87499999999986,10.2075972794973,-229.35005));
#222901=CARTESIAN_POINT('Origin',(8.87499999999986,10.9575972794973,-229.35005));
#222902=CARTESIAN_POINT('Origin',(8.87499999999984,-42.0701004838369,-229.35005));
#222903=CARTESIAN_POINT('',(9.62499999999984,-42.0701004838368,-229.35005));
#222904=CARTESIAN_POINT('',(9.62499999999984,-42.0701004838368,-235.35005));
#222905=CARTESIAN_POINT('',(8.87499999999984,-42.8201004838369,-229.35005));
#222906=CARTESIAN_POINT('',(8.87499999999984,-42.8201004838369,-229.35005));
#222907=CARTESIAN_POINT('Origin',(8.87499999999984,-42.0701004838369,-229.35005));
#222908=CARTESIAN_POINT('Origin',(8.87499999999984,-33.96456093117,-229.35005));
#222909=CARTESIAN_POINT('',(8.87499999999984,-33.21456093117,-229.35005));
#222910=CARTESIAN_POINT('',(8.87499999999984,-33.21456093117,-229.35005));
#222911=CARTESIAN_POINT('',(9.62499999999984,-33.96456093117,-229.35005));
#222912=CARTESIAN_POINT('',(9.62499999999984,-33.96456093117,-235.35005));
#222913=CARTESIAN_POINT('Origin',(8.87499999999984,-33.96456093117,-229.35005));
#222914=CARTESIAN_POINT('Origin',(1.25,-33.96456093117,-229.35005));
#222915=CARTESIAN_POINT('',(0.5,-33.96456093117,-229.35005));
#222916=CARTESIAN_POINT('',(0.5,-33.96456093117,-235.35005));
#222917=CARTESIAN_POINT('',(1.25,-33.21456093117,-229.35005));
#222918=CARTESIAN_POINT('',(1.25,-33.21456093117,-229.35005));
#222919=CARTESIAN_POINT('Origin',(1.25,-33.96456093117,-229.35005));
#222920=CARTESIAN_POINT('Origin',(1.25,-42.0701004838369,-229.35005));
#222921=CARTESIAN_POINT('',(1.25,-42.8201004838369,-229.35005));
#222922=CARTESIAN_POINT('',(1.25,-42.8201004838369,-229.35005));
#222923=CARTESIAN_POINT('',(0.5,-42.0701004838369,-229.35005));
#222924=CARTESIAN_POINT('',(0.5,-42.0701004838369,-235.35005));
#222925=CARTESIAN_POINT('Origin',(1.25,-42.0701004838369,-229.35005));
#222926=CARTESIAN_POINT('Origin',(8.87499999999986,21.5631368321642,-229.35005));
#222927=CARTESIAN_POINT('',(9.62499999999986,21.5631368321642,-229.35005));
#222928=CARTESIAN_POINT('',(9.62499999999986,21.5631368321642,-235.35005));
#222929=CARTESIAN_POINT('',(8.87499999999986,20.8131368321642,-229.35005));
#222930=CARTESIAN_POINT('',(8.87499999999986,20.8131368321642,-229.35005));
#222931=CARTESIAN_POINT('Origin',(8.87499999999986,21.5631368321642,-229.35005));
#222932=CARTESIAN_POINT('Origin',(8.87499999999986,29.9752906431998,-229.35005));
#222933=CARTESIAN_POINT('',(8.90766940259363,30.7245787787886,-229.35005));
#222934=CARTESIAN_POINT('',(8.90766940259363,30.7245787787886,-229.35005));
#222935=CARTESIAN_POINT('',(9.62499999999986,29.9752906431998,-229.35005));
#222936=CARTESIAN_POINT('',(9.62499999999986,29.9752906431998,-235.35005));
#222937=CARTESIAN_POINT('Origin',(8.87499999999986,29.9752906431998,-229.35005));
#222938=CARTESIAN_POINT('Origin',(1.25,30.1648419118246,-229.35005));
#222939=CARTESIAN_POINT('',(0.5,30.1648419118246,-229.35005));
#222940=CARTESIAN_POINT('',(1.25460132430898,30.9148277969016,-229.35005));
#222941=CARTESIAN_POINT('Origin',(1.25,30.1648419118246,-229.35005));
#222942=CARTESIAN_POINT('',(0.5,30.1648419118246,-229.35005));
#222943=CARTESIAN_POINT('',(1.25460132430898,30.9148277969016,-229.35005));
#222944=CARTESIAN_POINT('Origin',(1.25,21.5631368321642,-229.35005));
#222945=CARTESIAN_POINT('',(1.25,20.8131368321642,-229.35005));
#222946=CARTESIAN_POINT('',(1.25,20.8131368321642,-229.35005));
#222947=CARTESIAN_POINT('',(0.5,21.5631368321642,-229.35005));
#222948=CARTESIAN_POINT('',(0.5,21.5631368321642,-235.35005));
#222949=CARTESIAN_POINT('Origin',(1.25,21.5631368321642,-229.35005));
#222950=CARTESIAN_POINT('Origin',(7.99493453126771,-18.0851397679958,-192.281986444803));
#222951=CARTESIAN_POINT('',(8.57396770167423,-18.5618163748993,-229.35005));
#222952=CARTESIAN_POINT('',(8.57396770167423,-18.5618163748993,-192.281986444803));
#222953=CARTESIAN_POINT('',(7.4518492428487,-18.6024002144856,-229.35005));
#222954=CARTESIAN_POINT('',(7.4518492428487,-18.6024002144856,-235.35005));
#222955=CARTESIAN_POINT('Origin',(7.99493453126771,-18.0851397679958,-229.35005));
#222956=CARTESIAN_POINT('Origin',(6.18465023653768,-19.8093412562951,-192.281986444803));
#222957=CARTESIAN_POINT('',(6.72773552495669,-19.2920808098054,-229.35005));
#222958=CARTESIAN_POINT('',(6.72773552495669,-19.2920808098054,-229.35005));
#222959=CARTESIAN_POINT('',(6.63257355852516,-20.4108931639637,-229.35005));
#222960=CARTESIAN_POINT('',(6.63257355852516,-20.4108931639637,-192.281986444803));
#222961=CARTESIAN_POINT('Origin',(6.18465023653768,-19.8093412562951,-229.35005));
#222962=CARTESIAN_POINT('Origin',(6.18465023653769,-3.19762239537749,-192.281986444803));
#222963=CARTESIAN_POINT('',(6.63257355852517,-2.59607048770891,-229.35005));
#222964=CARTESIAN_POINT('',(6.63257355852517,-2.59607048770891,-192.281986444803));
#222965=CARTESIAN_POINT('',(6.7277355249567,-3.7148828418673,-229.35005));
#222966=CARTESIAN_POINT('',(6.7277355249567,-3.7148828418673,-192.281986444803));
#222967=CARTESIAN_POINT('Origin',(6.18465023653769,-3.19762239537748,-229.35005));
#222968=CARTESIAN_POINT('Origin',(1.25,-1.22366181637858,-192.281986444803));
#222969=CARTESIAN_POINT('',(0.5,-1.22366181637858,-229.35005));
#222970=CARTESIAN_POINT('',(1.3405312557817,-0.479145804645729,-229.35005));
#222971=CARTESIAN_POINT('Origin',(1.25,-1.22366181637858,-229.35005));
#222972=CARTESIAN_POINT('',(0.5,-1.22366181637858,-229.35005));
#222973=CARTESIAN_POINT('',(1.3405312557817,-0.479145804645732,-192.281986444803));
#222974=CARTESIAN_POINT('Origin',(1.25,-21.7833018352941,-192.281986444803));
#222975=CARTESIAN_POINT('',(1.3405312557817,-22.5278178470269,-229.35005));
#222976=CARTESIAN_POINT('',(1.3405312557817,-22.5278178470269,-192.281986444803));
#222977=CARTESIAN_POINT('',(0.5,-21.7833018352941,-229.35005));
#222978=CARTESIAN_POINT('',(0.5,-21.7833018352941,-235.35005));
#222979=CARTESIAN_POINT('Origin',(1.25,-21.7833018352941,-229.35005));
#222980=CARTESIAN_POINT('Origin',(5.14120077283693,-18.713796339242,-192.281986444803));
#222981=CARTESIAN_POINT('',(4.7057783396023,-18.1031349726598,-229.35005));
#222982=CARTESIAN_POINT('',(5.68428606125594,-18.1965358927522,-229.35005));
#222983=CARTESIAN_POINT('Origin',(5.14120077283693,-18.713796339242,-229.35005));
#222984=CARTESIAN_POINT('',(4.7057783396023,-18.1031349726598,-192.281986444803));
#222985=CARTESIAN_POINT('',(5.68428606125594,-18.1965358927522,-192.281986444803));
#222986=CARTESIAN_POINT('Origin',(6.95148506756696,-16.9895948509426,-192.281986444803));
#222987=CARTESIAN_POINT('',(6.40839977914796,-17.5068552974324,-229.35005));
#222988=CARTESIAN_POINT('',(6.40839977914795,-17.5068552974324,-192.281986444803));
#222989=CARTESIAN_POINT('',(6.36274467860837,-16.5249608504553,-229.35005));
#222990=CARTESIAN_POINT('',(6.36274467860837,-16.5249608504553,-192.281986444803));
#222991=CARTESIAN_POINT('Origin',(6.95148506756696,-16.9895948509426,-229.35005));
#222992=CARTESIAN_POINT('Origin',(20.625,-3.54959888009691,-192.281986444803));
#222993=CARTESIAN_POINT('',(11.294759518486,-7.14773903260897,-229.35005));
#222994=CARTESIAN_POINT('',(11.294759518486,-7.14773903260897,-192.281986444803));
#222995=CARTESIAN_POINT('',(10.6249999999999,-3.54959888009691,-229.35005));
#222996=CARTESIAN_POINT('',(10.6249999999999,-3.54959888009691,-235.35005));
#222997=CARTESIAN_POINT('Origin',(20.625,-3.54959888009691,-229.35005));
#222998=CARTESIAN_POINT('Origin',(20.625,-19.4573647715757,-192.281986444803));
#222999=CARTESIAN_POINT('',(10.6249999999999,-19.4573647715757,-229.35005));
#223000=CARTESIAN_POINT('',(10.6249999999999,-19.4573647715757,-235.35005));
#223001=CARTESIAN_POINT('',(11.294759518486,-15.8592246190636,-229.35005));
#223002=CARTESIAN_POINT('',(11.294759518486,-15.8592246190636,-192.281986444803));
#223003=CARTESIAN_POINT('Origin',(20.625,-19.4573647715757,-229.35005));
#223004=CARTESIAN_POINT('Origin',(9.40330570654103,-32.6090213785032,-192.281986444803));
#223005=CARTESIAN_POINT('',(5.33358654455951,-23.474614668563,-229.35005));
#223006=CARTESIAN_POINT('',(5.33358654455951,-23.474614668563,-192.281986444803));
#223007=CARTESIAN_POINT('Origin',(9.40330570654103,-32.6090213785032,-229.35005));
#223008=CARTESIAN_POINT('Origin',(9.40330570654115,9.60205772683048,-192.281986444803));
#223009=CARTESIAN_POINT('',(5.33358654455957,0.46765101689032,-229.35005));
#223010=CARTESIAN_POINT('',(5.33358654455957,0.467651016890315,-192.281986444803));
#223011=CARTESIAN_POINT('Origin',(9.40330570654115,9.60205772683049,-229.35005));
#223012=CARTESIAN_POINT('Origin',(0.,-11.5034818258363,-235.35005));
#223013=CARTESIAN_POINT('',(-5.66442007243621E-16,-16.1288318258363,-235.35005));
#223014=CARTESIAN_POINT('Origin',(0.,-11.5034818258363,-235.35005));
#223015=CARTESIAN_POINT('Origin',(0.,-11.5034818258363,-235.35005));
#223016=CARTESIAN_POINT('',(-5.66442007243621E-16,-16.1288318258363,-235.35005));
#223017=CARTESIAN_POINT('Origin',(0.,-11.5034818258363,-236.10005));
#223018=CARTESIAN_POINT('Origin',(0.,-11.5034818258363,-192.281986444803));
#223019=CARTESIAN_POINT('Origin',(0.,-11.5034818258363,-229.35005));
#223020=CARTESIAN_POINT('Origin',(0.,-11.5034818258363,-192.281986444803));
#223021=CARTESIAN_POINT('Origin',(0.,-11.5034818258363,-229.35005));
#223022=CARTESIAN_POINT('Origin',(0.,-11.5034818258363,-192.281986444803));
#223023=CARTESIAN_POINT('',(-9.92642306853573E-16,-19.6090213785032,-235.35005));
#223024=CARTESIAN_POINT('',(-9.92642306853574E-16,-19.6090213785032,-192.281986444803));
#223025=CARTESIAN_POINT('Origin',(0.,-11.5034818258363,-235.35005));
#223026=CARTESIAN_POINT('Origin',(0.,-11.5034818258363,-229.35005));
#223027=CARTESIAN_POINT('Origin',(0.,-11.5034818258363,-235.35005));
#223028=CARTESIAN_POINT('Origin',(0.,-11.5034818258363,-229.35005));
#223029=CARTESIAN_POINT('Origin',(0.,-11.5034818258363,-235.35005));
#223030=CARTESIAN_POINT('Origin',(0.,-11.5034818258363,-229.35005));
#223031=CARTESIAN_POINT('Origin',(0.,-11.5034818258363,-235.35005));
#223032=CARTESIAN_POINT('Origin',(0.,-11.5034818258363,-229.35005));
#223033=CARTESIAN_POINT('Origin',(0.,-11.5034818258363,-235.35005));
#223034=CARTESIAN_POINT('Origin',(0.,-11.5034818258363,-229.35005));
#223035=CARTESIAN_POINT('Origin',(0.,-11.5034818258363,-235.35005));
#223036=CARTESIAN_POINT('Origin',(0.,-11.5034818258363,-229.35005));
#223037=CARTESIAN_POINT('Origin',(0.,-11.5034818258363,-235.35005));
#223038=CARTESIAN_POINT('Origin',(0.,-11.5034818258363,-229.35005));
#223039=CARTESIAN_POINT('Origin',(0.,-11.5034818258363,-235.35005));
#223040=CARTESIAN_POINT('Origin',(0.,-11.5034818258363,-229.35005));
#223041=CARTESIAN_POINT('Origin',(0.,-11.5034818258363,-235.35005));
#223042=CARTESIAN_POINT('Origin',(0.,-11.5034818258363,-192.281986444803));
#223043=CARTESIAN_POINT('Origin',(0.,-11.5034818258363,-229.35005));
#223044=CARTESIAN_POINT('Origin',(-6.10697827817036,-5.81657868152891,-192.281986444803));
#223045=CARTESIAN_POINT('',(-6.10697827817036,-5.81657868152891,-229.35005));
#223046=CARTESIAN_POINT('Origin',(-5.38286456027835,-5.12689808620917,-192.281986444803));
#223047=CARTESIAN_POINT('',(-5.38286456027835,-5.12689808620916,-229.35005));
#223048=CARTESIAN_POINT('Origin',(0.,-11.5034818258363,-192.281986444803));
#223049=CARTESIAN_POINT('Origin',(0.,-11.5034818258363,-229.35005));
#223050=CARTESIAN_POINT('Origin',(0.,-11.5034818258363,-192.281986444803));
#223051=CARTESIAN_POINT('Origin',(0.,-11.5034818258363,-229.35005));
#223052=CARTESIAN_POINT('Origin',(0.,-11.5034818258363,-192.281986444803));
#223053=CARTESIAN_POINT('Origin',(0.,-11.5034818258363,-229.35005));
#223054=CARTESIAN_POINT('Origin',(5.38286456027834,-5.12689808620917,-192.281986444803));
#223055=CARTESIAN_POINT('',(5.38286456027834,-5.12689808620916,-229.35005));
#223056=CARTESIAN_POINT('Origin',(6.10697827817035,-5.81657868152891,-192.281986444803));
#223057=CARTESIAN_POINT('',(6.10697827817035,-5.81657868152891,-229.35005));
#223058=CARTESIAN_POINT('Origin',(0.,-11.5034818258363,-192.281986444803));
#223059=CARTESIAN_POINT('Origin',(0.,-11.5034818258363,-229.35005));
#223060=CARTESIAN_POINT('Origin',(0.,-11.5034818258363,-192.281986444803));
#223061=CARTESIAN_POINT('Origin',(0.,-11.5034818258363,-229.35005));
#223062=CARTESIAN_POINT('Origin',(29.875,26.0662450163965,-235.35005));
#223063=CARTESIAN_POINT('',(29.875,26.0662450163965,-229.35005));
#223064=CARTESIAN_POINT('Origin',(30.875,26.0662450163965,-235.35005));
#223065=CARTESIAN_POINT('',(30.875,26.0662450163965,-229.35005));
#223066=CARTESIAN_POINT('Origin',(30.875,26.0662450163965,-235.35005));
#223067=CARTESIAN_POINT('',(30.875,26.0662450163965,-229.35005));
#223068=CARTESIAN_POINT('Origin',(29.875,26.0662450163965,-235.35005));
#223069=CARTESIAN_POINT('',(29.875,26.0662450163965,-229.35005));
#223070=CARTESIAN_POINT('Origin',(30.875,26.0662450163965,-235.35005));
#223071=CARTESIAN_POINT('',(30.875,26.0662450163965,-229.35005));
#223072=CARTESIAN_POINT('Origin',(29.875,26.0662450163965,-235.35005));
#223073=CARTESIAN_POINT('',(29.875,26.0662450163965,-229.35005));
#223074=CARTESIAN_POINT('Origin',(30.875,26.0662450163965,-235.35005));
#223075=CARTESIAN_POINT('',(30.875,26.0662450163965,-229.35005));
#223076=CARTESIAN_POINT('Origin',(29.875,26.0662450163965,-235.35005));
#223077=CARTESIAN_POINT('',(29.875,26.0662450163965,-229.35005));
#223078=CARTESIAN_POINT('Origin',(30.875,26.0662450163965,-235.35005));
#223079=CARTESIAN_POINT('',(30.875,26.0662450163965,-229.35005));
#223080=CARTESIAN_POINT('Origin',(29.875,26.0662450163965,-235.35005));
#223081=CARTESIAN_POINT('',(29.875,26.0662450163965,-229.35005));
#223082=CARTESIAN_POINT('Origin',(30.875,26.0662450163965,-235.35005));
#223083=CARTESIAN_POINT('',(30.875,26.0662450163965,-229.35005));
#223084=CARTESIAN_POINT('Origin',(29.875,26.0662450163965,-235.35005));
#223085=CARTESIAN_POINT('',(29.875,26.0662450163965,-229.35005));
#223086=CARTESIAN_POINT('Origin',(30.875,26.0662450163965,-235.35005));
#223087=CARTESIAN_POINT('',(30.875,26.0662450163965,-229.35005));
#223088=CARTESIAN_POINT('Origin',(29.875,26.0662450163965,-235.35005));
#223089=CARTESIAN_POINT('',(29.875,26.0662450163965,-229.35005));
#223090=CARTESIAN_POINT('Origin',(30.875,26.0662450163965,-235.35005));
#223091=CARTESIAN_POINT('',(30.875,26.0662450163965,-229.35005));
#223092=CARTESIAN_POINT('Origin',(29.875,26.0662450163965,-235.35005));
#223093=CARTESIAN_POINT('',(29.875,26.0662450163965,-229.35005));
#223094=CARTESIAN_POINT('Origin',(19.75,32.818676384831,-235.35005));
#223095=CARTESIAN_POINT('',(19.75,32.818676384831,-229.35005));
#223096=CARTESIAN_POINT('Origin',(20.75,32.818676384831,-235.35005));
#223097=CARTESIAN_POINT('',(20.75,32.818676384831,-229.35005));
#223098=CARTESIAN_POINT('Origin',(20.75,32.818676384831,-235.35005));
#223099=CARTESIAN_POINT('',(20.75,32.818676384831,-229.35005));
#223100=CARTESIAN_POINT('Origin',(19.75,32.818676384831,-235.35005));
#223101=CARTESIAN_POINT('',(19.75,32.818676384831,-229.35005));
#223102=CARTESIAN_POINT('Origin',(20.75,32.818676384831,-235.35005));
#223103=CARTESIAN_POINT('',(20.75,32.818676384831,-229.35005));
#223104=CARTESIAN_POINT('Origin',(19.75,32.818676384831,-235.35005));
#223105=CARTESIAN_POINT('',(19.75,32.818676384831,-229.35005));
#223106=CARTESIAN_POINT('Origin',(20.75,32.818676384831,-235.35005));
#223107=CARTESIAN_POINT('',(20.75,32.818676384831,-229.35005));
#223108=CARTESIAN_POINT('Origin',(19.75,32.818676384831,-235.35005));
#223109=CARTESIAN_POINT('',(19.75,32.818676384831,-229.35005));
#223110=CARTESIAN_POINT('Origin',(20.75,32.818676384831,-235.35005));
#223111=CARTESIAN_POINT('',(20.75,32.818676384831,-229.35005));
#223112=CARTESIAN_POINT('Origin',(19.75,32.818676384831,-235.35005));
#223113=CARTESIAN_POINT('',(19.75,32.818676384831,-229.35005));
#223114=CARTESIAN_POINT('Origin',(20.75,32.818676384831,-235.35005));
#223115=CARTESIAN_POINT('',(20.75,32.818676384831,-229.35005));
#223116=CARTESIAN_POINT('Origin',(19.75,32.818676384831,-235.35005));
#223117=CARTESIAN_POINT('',(19.75,32.818676384831,-229.35005));
#223118=CARTESIAN_POINT('Origin',(20.75,32.818676384831,-235.35005));
#223119=CARTESIAN_POINT('',(20.75,32.818676384831,-229.35005));
#223120=CARTESIAN_POINT('Origin',(19.75,32.818676384831,-235.35005));
#223121=CARTESIAN_POINT('',(19.75,32.818676384831,-229.35005));
#223122=CARTESIAN_POINT('Origin',(20.75,32.818676384831,-235.35005));
#223123=CARTESIAN_POINT('',(20.75,32.818676384831,-229.35005));
#223124=CARTESIAN_POINT('Origin',(19.75,32.818676384831,-235.35005));
#223125=CARTESIAN_POINT('',(19.75,32.818676384831,-229.35005));
#223126=CARTESIAN_POINT('Origin',(20.75,32.818676384831,-235.35005));
#223127=CARTESIAN_POINT('',(20.75,32.818676384831,-232.25005));
#223128=CARTESIAN_POINT('',(20.75,32.818676384831,-229.35005));
#223129=CARTESIAN_POINT('',(20.75,32.818676384831,-235.35005));
#223130=CARTESIAN_POINT('',(19.75,32.818676384831,-232.25005));
#223131=CARTESIAN_POINT('',(11.4589044897296,32.818676384831,-232.25005));
#223132=CARTESIAN_POINT('',(19.75,32.818676384831,-229.35005));
#223133=CARTESIAN_POINT('',(19.75,32.818676384831,-235.35005));
#223134=CARTESIAN_POINT('',(20.75,32.818676384831,-229.35005));
#223135=CARTESIAN_POINT('Origin',(20.75,32.818676384831,-235.35005));
#223136=CARTESIAN_POINT('',(20.75,32.3760227311709,-232.25005));
#223137=CARTESIAN_POINT('',(20.75,32.3760227311709,-229.35005));
#223138=CARTESIAN_POINT('',(20.75,32.3760227311709,-229.35005));
#223139=CARTESIAN_POINT('',(20.75,-32.0203896799758,-232.25005));
#223140=CARTESIAN_POINT('',(20.75,32.818676384831,-229.35005));
#223141=CARTESIAN_POINT('Origin',(19.75,32.818676384831,-235.35005));
#223142=CARTESIAN_POINT('',(19.75,32.4743226583831,-232.25005));
#223143=CARTESIAN_POINT('',(19.75,-32.0203896799758,-232.25005));
#223144=CARTESIAN_POINT('',(19.75,32.4743226583832,-229.35005));
#223145=CARTESIAN_POINT('',(19.75,32.4743226583832,-229.35005));
#223146=CARTESIAN_POINT('',(19.75,32.818676384831,-229.35005));
#223147=CARTESIAN_POINT('Origin',(9.62499999999986,32.818676384831,-235.35005));
#223148=CARTESIAN_POINT('',(9.62499999999986,32.818676384831,-229.35005));
#223149=CARTESIAN_POINT('Origin',(10.6249999999999,32.818676384831,-235.35005));
#223150=CARTESIAN_POINT('',(10.6249999999999,32.818676384831,-229.35005));
#223151=CARTESIAN_POINT('Origin',(10.6249999999999,32.818676384831,-235.35005));
#223152=CARTESIAN_POINT('',(10.6249999999999,32.818676384831,-229.35005));
#223153=CARTESIAN_POINT('Origin',(9.62499999999986,32.818676384831,-235.35005));
#223154=CARTESIAN_POINT('',(9.62499999999986,32.818676384831,-229.35005));
#223155=CARTESIAN_POINT('Origin',(10.6249999999999,32.818676384831,-235.35005));
#223156=CARTESIAN_POINT('',(10.6249999999999,32.818676384831,-229.35005));
#223157=CARTESIAN_POINT('Origin',(9.62499999999986,32.818676384831,-235.35005));
#223158=CARTESIAN_POINT('',(9.62499999999986,32.818676384831,-229.35005));
#223159=CARTESIAN_POINT('Origin',(10.6249999999999,32.818676384831,-235.35005));
#223160=CARTESIAN_POINT('',(10.6249999999999,32.818676384831,-229.35005));
#223161=CARTESIAN_POINT('Origin',(9.62499999999986,32.818676384831,-235.35005));
#223162=CARTESIAN_POINT('',(9.62499999999986,32.818676384831,-229.35005));
#223163=CARTESIAN_POINT('Origin',(10.6249999999999,32.818676384831,-235.35005));
#223164=CARTESIAN_POINT('',(10.6249999999999,32.818676384831,-229.35005));
#223165=CARTESIAN_POINT('Origin',(10.6249999999999,32.818676384831,-235.35005));
#223166=CARTESIAN_POINT('',(10.6249999999999,32.818676384831,-229.35005));
#223167=CARTESIAN_POINT('Origin',(10.6249999999999,32.818676384831,-235.35005));
#223168=CARTESIAN_POINT('',(10.6249999999999,32.818676384831,-229.35005));
#223169=CARTESIAN_POINT('Origin',(9.62499999999986,32.818676384831,-235.35005));
#223170=CARTESIAN_POINT('',(9.62499999999986,32.818676384831,-229.35005));
#223171=CARTESIAN_POINT('Origin',(10.6249999999999,32.818676384831,-235.35005));
#223172=CARTESIAN_POINT('',(10.6249999999999,32.818676384831,-229.35005));
#223173=CARTESIAN_POINT('Origin',(9.62499999999986,32.818676384831,-235.35005));
#223174=CARTESIAN_POINT('',(9.62499999999986,32.818676384831,-229.35005));
#223175=CARTESIAN_POINT('Origin',(0.5,32.818676384831,-235.35005));
#223176=CARTESIAN_POINT('',(0.5,32.818676384831,-229.35005));
#223177=CARTESIAN_POINT('Origin',(0.5,32.818676384831,-235.35005));
#223178=CARTESIAN_POINT('',(0.5,32.818676384831,-229.35005));
#223179=CARTESIAN_POINT('Origin',(0.5,32.818676384831,-235.35005));
#223180=CARTESIAN_POINT('',(0.5,32.818676384831,-229.35005));
#223181=CARTESIAN_POINT('Origin',(0.5,32.818676384831,-235.35005));
#223182=CARTESIAN_POINT('',(0.5,32.818676384831,-229.35005));
#223183=CARTESIAN_POINT('Origin',(0.5,32.818676384831,-235.35005));
#223184=CARTESIAN_POINT('',(0.5,32.818676384831,-229.35005));
#223185=CARTESIAN_POINT('Origin',(0.5,32.818676384831,-235.35005));
#223186=CARTESIAN_POINT('',(0.5,32.818676384831,-229.35005));
#223187=CARTESIAN_POINT('Origin',(0.5,32.818676384831,-235.35005));
#223188=CARTESIAN_POINT('',(0.5,32.818676384831,-229.35005));
#223189=CARTESIAN_POINT('Origin',(0.5,32.818676384831,-235.35005));
#223190=CARTESIAN_POINT('',(0.5,32.818676384831,-229.35005));
#223191=CARTESIAN_POINT('Origin',(7.14692237356698E-14,623.509175991979,
-229.35005));
#223192=CARTESIAN_POINT('Origin',(-2.61456814389029E-14,-173.57701443073,
-229.35005));
#223193=CARTESIAN_POINT('',(23.0363900009079,-56.0352881775207,-229.35005));
#223194=CARTESIAN_POINT('Origin',(7.14692237356698E-14,623.509175991979,
-229.35005));
#223195=CARTESIAN_POINT('',(24.6244543289934,-55.593007214519,-229.35005));
#223196=CARTESIAN_POINT('Origin',(22.9178089794592,-52.5372975341153,-229.35005));
#223197=CARTESIAN_POINT('',(41.8942895912772,-39.701327481882,-229.35005));
#223198=CARTESIAN_POINT('Origin',(-6.29739814579425E-15,-11.5034818258363,
-229.35005));
#223199=CARTESIAN_POINT('',(42.4880898820538,-37.8828103193512,-229.35005));
#223200=CARTESIAN_POINT('Origin',(38.9907249661392,-37.7470213473046,-229.35005));
#223201=CARTESIAN_POINT('',(42.4880898820539,14.8758466676788,-229.35005));
#223202=CARTESIAN_POINT('Origin',(-636.934816028482,-11.5034818258361,-229.35005));
#223203=CARTESIAN_POINT('',(41.8942895912773,16.6943638302095,-229.35005));
#223204=CARTESIAN_POINT('Origin',(38.9907249661392,14.740057695632,-229.35005));
#223205=CARTESIAN_POINT('',(26.6879613405455,31.3684521110126,-229.35005));
#223206=CARTESIAN_POINT('Origin',(-6.29739814579425E-15,-11.5034818258363,
-229.35005));
#223207=CARTESIAN_POINT('',(25.2655040598954,31.8709602996399,-229.35005));
#223208=CARTESIAN_POINT('Origin',(24.838300653577,28.3971299569735,-229.35005));
#223209=CARTESIAN_POINT('Origin',(-2.61456814389029E-14,-173.57701443073,
-229.35005));
#223210=CARTESIAN_POINT('Origin',(7.14692237356698E-14,623.509175991979,
-229.35005));
#223211=CARTESIAN_POINT('',(-1.23757166668304E-15,-43.8201004838368,-229.35005));
#223212=CARTESIAN_POINT('',(-1.54373336646988E-15,19.8131368321642,-229.35005));
#223213=CARTESIAN_POINT('',(-2.53637567332344E-15,10.2075972794973,-229.35005));
#223214=CARTESIAN_POINT('',(-2.8425373731103E-15,9.20759727949731,-229.35005));
#223215=CARTESIAN_POINT('',(-1.11087130309497E-13,-0.397942273169518,-229.35005));
#223216=CARTESIAN_POINT('',(-3.33261390928491E-13,-22.6090213785032,-229.35005));
#223217=CARTESIAN_POINT('',(0.,-32.21456093117,-229.35005));
#223218=CARTESIAN_POINT('',(-1.54373336646987E-15,-42.8201004838369,-229.35005));
#223219=CARTESIAN_POINT('',(0.,-33.21456093117,-229.35005));
#223220=CARTESIAN_POINT('Origin',(-2.61456814389029E-14,-173.57701443073,
-229.35005));
#223221=CARTESIAN_POINT('',(-1.23757166668304E-15,20.8131368321642,-229.35005));
#223222=CARTESIAN_POINT('Origin',(-2.61456814389029E-14,-173.57701443073,
-229.35005));
#223223=CARTESIAN_POINT('',(-1.23757166668304E-15,20.8131368321642,-229.35005));
#223224=CARTESIAN_POINT('',(-1.54373336646987E-15,-42.8201004838369,-229.35005));
#223225=CARTESIAN_POINT('',(0.,-33.21456093117,-229.35005));
#223226=CARTESIAN_POINT('',(-1.54373336646988E-15,19.8131368321642,-229.35005));
#223227=CARTESIAN_POINT('',(-2.53637567332344E-15,10.2075972794973,-229.35005));
#223228=CARTESIAN_POINT('Origin',(7.14692237356698E-14,623.509175991979,
-229.35005));
#223229=CARTESIAN_POINT('',(-1.23757166668304E-15,-43.8201004838368,-229.35005));
#223230=CARTESIAN_POINT('',(-1.23757166668304E-15,20.8131368321642,-229.35005));
#223231=CARTESIAN_POINT('',(24.960358769668,29.3896529120211,-229.35005));
#223232=CARTESIAN_POINT('Origin',(-2.61456814389029E-14,-173.57701443073,
-229.35005));
#223233=CARTESIAN_POINT('',(25.366775135568,29.2460791438418,-229.35005));
#223234=CARTESIAN_POINT('Origin',(24.838300653577,28.3971299569735,-229.35005));
#223235=CARTESIAN_POINT('Origin',(-6.29739814579425E-15,-11.5034818258363,
-229.35005));
#223236=CARTESIAN_POINT('',(-2.53637567332344E-15,10.2075972794973,-229.35005));
#223237=CARTESIAN_POINT('',(-1.54373336646988E-15,19.8131368321642,-229.35005));
#223238=CARTESIAN_POINT('',(39.8203148590359,15.2984308769399,-229.35005));
#223239=CARTESIAN_POINT('Origin',(-6.29739814579425E-15,-11.5034818258363,
-229.35005));
#223240=CARTESIAN_POINT('',(39.989972084972,14.7788545447883,-229.35005));
#223241=CARTESIAN_POINT('Origin',(38.9907249661392,14.740057695632,-229.35005));
#223242=CARTESIAN_POINT('Origin',(-636.934816028482,-11.5034818258361,-229.35005));
#223243=CARTESIAN_POINT('',(-1.11087130309497E-13,-0.397942273169518,-229.35005));
#223244=CARTESIAN_POINT('',(-2.8425373731103E-15,9.20759727949731,-229.35005));
#223245=CARTESIAN_POINT('Origin',(-636.934816028482,-11.5034818258361,-229.35005));
#223246=CARTESIAN_POINT('',(-2.22174260618994E-13,-11.0034818258363,-229.35005));
#223247=CARTESIAN_POINT('',(-1.11087130309497E-13,-1.3979422731695,-229.35005));
#223248=CARTESIAN_POINT('Origin',(-636.934816028482,-11.5034818258361,-229.35005));
#223249=CARTESIAN_POINT('',(-3.33261390928491E-13,-21.6090213785032,-229.35005));
#223250=CARTESIAN_POINT('',(-2.22174260618994E-13,-12.0034818258363,-229.35005));
#223251=CARTESIAN_POINT('Origin',(-636.934816028482,-11.5034818258361,-229.35005));
#223252=CARTESIAN_POINT('',(0.,-32.21456093117,-229.35005));
#223253=CARTESIAN_POINT('',(-3.33261390928491E-13,-22.6090213785032,-229.35005));
#223254=CARTESIAN_POINT('Origin',(-636.934816028482,-11.5034818258361,-229.35005));
#223255=CARTESIAN_POINT('',(-1.54373336646987E-15,-42.8201004838369,-229.35005));
#223256=CARTESIAN_POINT('',(0.,-33.21456093117,-229.35005));
#223257=CARTESIAN_POINT('',(-1.23757166668304E-15,-43.8201004838368,-229.35005));
#223258=CARTESIAN_POINT('Origin',(-6.29739814579425E-15,-11.5034818258363,
-229.35005));
#223259=CARTESIAN_POINT('',(-3.33261390928491E-13,-22.6090213785032,-229.35005));
#223260=CARTESIAN_POINT('',(0.,-32.21456093117,-229.35005));
#223261=CARTESIAN_POINT('',(-2.22174260618994E-13,-12.0034818258363,-229.35005));
#223262=CARTESIAN_POINT('',(-3.33261390928491E-13,-21.6090213785032,-229.35005));
#223263=CARTESIAN_POINT('',(-1.11087130309497E-13,-1.3979422731695,-229.35005));
#223264=CARTESIAN_POINT('',(-2.22174260618994E-13,-11.0034818258363,-229.35005));
#223265=CARTESIAN_POINT('',(-1.54373336646987E-15,-42.8201004838369,-229.35005));
#223266=CARTESIAN_POINT('',(0.,-33.21456093117,-229.35005));
#223267=CARTESIAN_POINT('',(39.989972084972,-37.7858181964606,-229.35005));
#223268=CARTESIAN_POINT('Origin',(-636.934816028482,-11.5034818258361,-229.35005));
#223269=CARTESIAN_POINT('',(39.8203148590358,-38.3053945286125,-229.35005));
#223270=CARTESIAN_POINT('Origin',(38.9907249661392,-37.7470213473046,-229.35005));
#223271=CARTESIAN_POINT('Origin',(-6.29739814579425E-15,-11.5034818258363,
-229.35005));
#223272=CARTESIAN_POINT('',(-1.23757166668304E-15,-43.8201004838368,-229.35005));
#223273=CARTESIAN_POINT('',(23.4054219364689,-53.410357442802,-229.35005));
#223274=CARTESIAN_POINT('Origin',(-6.29739814579425E-15,-11.5034818258363,
-229.35005));
#223275=CARTESIAN_POINT('',(22.9516892713016,-53.5367234322311,-229.35005));
#223276=CARTESIAN_POINT('Origin',(22.9178089794592,-52.5372975341153,-229.35005));
#223277=CARTESIAN_POINT('Origin',(7.14692237356698E-14,623.509175991979,
-229.35005));
#223278=CARTESIAN_POINT('',(-2.8425373731103E-15,9.20759727949731,-229.35005));
#223279=CARTESIAN_POINT('',(-1.11087130309497E-13,-0.397942273169518,-229.35005));
#223280=CARTESIAN_POINT('',(-1.54373336646988E-15,19.8131368321642,-229.35005));
#223281=CARTESIAN_POINT('',(-2.53637567332344E-15,10.2075972794973,-229.35005));
#223282=CARTESIAN_POINT('',(-1.23757166668304E-15,20.8131368321642,-229.35005));
#223283=CARTESIAN_POINT('Origin',(-6.29739814579425E-15,-11.5034818258363,
-229.35005));
#223284=CARTESIAN_POINT('',(-2.22174260618994E-13,-11.0034818258363,-229.35005));
#223285=CARTESIAN_POINT('',(-1.11087130309497E-13,-1.3979422731695,-229.35005));
#223286=CARTESIAN_POINT('',(0.,-32.21456093117,-229.35005));
#223287=CARTESIAN_POINT('',(-2.22174260618994E-13,-12.0034818258363,-229.35005));
#223288=CARTESIAN_POINT('',(-2.8425373731103E-15,9.20759727949731,-229.35005));
#223289=CARTESIAN_POINT('',(-2.22174260618994E-13,-11.0034818258363,-229.35005));
#223290=CARTESIAN_POINT('',(-2.22174260618994E-13,-12.0034818258363,-229.35005));
#223291=CARTESIAN_POINT('',(-3.33261390928491E-13,-21.6090213785032,-229.35005));
#223292=CARTESIAN_POINT('Origin',(24.838300653577,28.3971299569735,-229.35005));
#223293=CARTESIAN_POINT('',(25.2655040598954,31.8709602996399,-232.25005));
#223294=CARTESIAN_POINT('',(25.2655040598954,31.8709602996399,-229.35005));
#223295=CARTESIAN_POINT('',(26.6879613405455,31.3684521110126,-232.25005));
#223296=CARTESIAN_POINT('',(26.6879613405455,31.3684521110126,-229.35005));
#223297=CARTESIAN_POINT('Origin',(24.838300653577,28.3971299569735,-232.25005));
#223298=CARTESIAN_POINT('Origin',(-6.29739814579425E-15,-11.5034818258363,
-229.35005));
#223299=CARTESIAN_POINT('',(41.8942895912773,16.6943638302095,-232.25005));
#223300=CARTESIAN_POINT('Origin',(-6.29739814579425E-15,-11.5034818258363,
-232.25005));
#223301=CARTESIAN_POINT('',(41.8942895912773,16.6943638302095,-229.35005));
#223302=CARTESIAN_POINT('Origin',(38.9907249661392,14.740057695632,-229.35005));
#223303=CARTESIAN_POINT('',(42.4880898820539,14.8758466676788,-232.25005));
#223304=CARTESIAN_POINT('',(42.4880898820538,14.8758466676788,-229.35005));
#223305=CARTESIAN_POINT('Origin',(38.9907249661392,14.740057695632,-232.25005));
#223306=CARTESIAN_POINT('Origin',(-636.934816028482,-11.5034818258361,-229.35005));
#223307=CARTESIAN_POINT('',(42.4880898820539,-37.8828103193509,-232.25005));
#223308=CARTESIAN_POINT('',(42.4880898820539,-37.8828103193507,-229.35005));
#223309=CARTESIAN_POINT('Origin',(-636.934816028482,-11.5034818258361,-232.25005));
#223310=CARTESIAN_POINT('Origin',(38.9907249661392,-37.7470213473046,-229.35005));
#223311=CARTESIAN_POINT('',(41.8942895912772,-39.701327481882,-232.25005));
#223312=CARTESIAN_POINT('',(41.8942895912772,-39.701327481882,-229.35005));
#223313=CARTESIAN_POINT('Origin',(38.9907249661392,-37.7470213473046,-232.25005));
#223314=CARTESIAN_POINT('Origin',(-6.29739814579425E-15,-11.5034818258363,
-229.35005));
#223315=CARTESIAN_POINT('',(24.6244543289934,-55.593007214519,-232.25005));
#223316=CARTESIAN_POINT('Origin',(-6.29739814579425E-15,-11.5034818258363,
-232.25005));
#223317=CARTESIAN_POINT('',(24.6244543289934,-55.593007214519,-229.35005));
#223318=CARTESIAN_POINT('Origin',(22.9178089794592,-52.5372975341153,-229.35005));
#223319=CARTESIAN_POINT('',(23.036390000908,-56.0352881775208,-232.25005));
#223320=CARTESIAN_POINT('',(23.036390000908,-56.0352881775208,-229.35005));
#223321=CARTESIAN_POINT('Origin',(22.9178089794592,-52.5372975341153,-232.25005));
#223322=CARTESIAN_POINT('Origin',(7.14692237356698E-14,623.509175991979,
-229.35005));
#223323=CARTESIAN_POINT('Origin',(7.14692237356698E-14,623.509175991979,
-232.25005));
#223324=CARTESIAN_POINT('Origin',(0.127542579976414,-12.8706479699377,-225.85005));
#223325=CARTESIAN_POINT('',(45.4582830719504,-55.6286991261908,-225.850049994059));
#223326=CARTESIAN_POINT('',(46.0196463796681,-56.2008156187296,-225.85005));
#223327=CARTESIAN_POINT('',(1.84775995058105,-11.1827640290625,-225.85005));
#223328=CARTESIAN_POINT('',(41.9650064389658,-58.9506113934371,-225.850044661983));
#223329=CARTESIAN_POINT('Ctrl Pts',(45.4582830570449,-55.6286991119449,
-225.85005));
#223330=CARTESIAN_POINT('Ctrl Pts',(44.9026972694785,-56.2100079876823,
-225.85005));
#223331=CARTESIAN_POINT('Ctrl Pts',(44.3324112171386,-56.7795949075102,
-225.85005));
#223332=CARTESIAN_POINT('Ctrl Pts',(43.1653582851246,-57.8895859697625,
-225.85005));
#223333=CARTESIAN_POINT('Ctrl Pts',(42.5695992766628,-58.4285233279616,
-225.85005));
#223334=CARTESIAN_POINT('Ctrl Pts',(41.9650009328216,-58.9506050170295,
-225.85005));
#223335=CARTESIAN_POINT('',(42.5792116384512,-59.576583500476,-225.85005));
#223336=CARTESIAN_POINT('',(-1.59267479062803,-14.5585319108126,-225.85005));
#223337=CARTESIAN_POINT('Origin',(48.1334350484927,-61.7961505568785,-225.85005));
#223338=CARTESIAN_POINT('Origin',(53.4203077633109,-63.7432454966418,-228.35005));
#223339=CARTESIAN_POINT('',(46.0300274667465,-56.2113955881677,-225.0730275154));
#223340=CARTESIAN_POINT('',(46.0300165430729,-56.2113851125247,-225.073041905978));
#223341=CARTESIAN_POINT('',(46.0300271011815,-56.2113951953429,-225.073057235855));
#223342=CARTESIAN_POINT('Origin',(0.128459562639233,-12.6359082483571,-225.85005));
#223343=CARTESIAN_POINT('',(43.3207863665692,34.1152634411122,-225.85005));
#223344=CARTESIAN_POINT('',(43.7661191575918,33.2092653454987,-225.850049986033));
#223345=CARTESIAN_POINT('Origin',(48.892180948596,36.2913696007177,-225.85005));
#223346=CARTESIAN_POINT('',(43.0713417429912,33.8649821651551,-225.850049999629));
#223347=CARTESIAN_POINT('',(50.4030915963197,41.2213231498315,-225.85005));
#223348=CARTESIAN_POINT('Ctrl Pts',(43.7661189696348,33.2092654883827,-225.85005));
#223349=CARTESIAN_POINT('Ctrl Pts',(43.6513378376322,33.3196167396708,-225.85005));
#223350=CARTESIAN_POINT('Ctrl Pts',(43.5360342857599,33.4294426438742,-225.85005));
#223351=CARTESIAN_POINT('Ctrl Pts',(43.3044413458354,33.6480087532319,-225.85005));
#223352=CARTESIAN_POINT('Ctrl Pts',(43.188133833512,33.7567661029554,-225.85005));
#223353=CARTESIAN_POINT('Ctrl Pts',(43.0713417424048,33.8649821645222,-225.85005));
#223354=CARTESIAN_POINT('Origin',(50.4030915963197,41.2213231498315,-228.35005));
#223355=CARTESIAN_POINT('',(43.3259173910555,34.120411675359,-225.468974352258));
#223356=CARTESIAN_POINT('Ctrl Pts',(43.325917391056,34.1204116753647,-225.468974352262));
#223357=CARTESIAN_POINT('Ctrl Pts',(43.2834889555987,34.0778409323755,-225.532489880709));
#223358=CARTESIAN_POINT('Ctrl Pts',(43.2410614099671,34.0352710821964,-225.596002003533));
#223359=CARTESIAN_POINT('Ctrl Pts',(43.1562018216867,33.9501268697379,-225.72302878886));
#223360=CARTESIAN_POINT('Ctrl Pts',(43.1137729118023,33.9075556507304,-225.786538761927));
#223361=CARTESIAN_POINT('Ctrl Pts',(43.0713417427678,33.8649821649953,-225.850049999372));
#223362=CARTESIAN_POINT('',(43.3259171707406,34.1204114543102,-225.468990713749));
#223363=CARTESIAN_POINT('Origin',(48.982196043432,-44.3222432618617,-167.906149834141));
#223364=CARTESIAN_POINT('',(54.2707699605536,-64.1721709500326,-208.192630912054));
#223365=CARTESIAN_POINT('',(54.238698329297,-64.0517945379221,-214.260116171494));
#223366=CARTESIAN_POINT('Ctrl Pts',(54.2707699605539,-64.1721709500341,
-208.192630912048));
#223367=CARTESIAN_POINT('Ctrl Pts',(54.2547227572974,-64.1119400013452,
-211.229354398965));
#223368=CARTESIAN_POINT('Ctrl Pts',(54.2386983294438,-64.051794536968,-214.260116171476));
#223369=CARTESIAN_POINT('',(53.7300151844417,-62.1425230012532,-215.85005));
#223370=CARTESIAN_POINT('Ctrl Pts',(53.7300151844416,-62.1425230012532,
-215.85005));
#223371=CARTESIAN_POINT('Ctrl Pts',(53.8150179700951,-62.4615691514925,
-215.58578405635));
#223372=CARTESIAN_POINT('Ctrl Pts',(53.8997787313547,-62.7797068967878,
-215.321544427173));
#223373=CARTESIAN_POINT('Ctrl Pts',(54.0694761933685,-63.4166427518271,
-214.791113982271));
#223374=CARTESIAN_POINT('Ctrl Pts',(54.153975481613,-63.7337990944663,-214.526290576087));
#223375=CARTESIAN_POINT('Ctrl Pts',(54.238698329735,-64.0517945380611,-214.260116171799));
#223376=CARTESIAN_POINT('',(54.2707699605536,-64.1721709500326,-215.85005));
#223377=CARTESIAN_POINT('',(53.272912245153,-60.426850603907,-215.85005));
#223378=CARTESIAN_POINT('',(54.2707699605536,-64.1721709500326,-208.192630912054));
#223379=CARTESIAN_POINT('Origin',(52.3809255634408,-67.7420224291304,-167.906149834141));
#223380=CARTESIAN_POINT('',(50.9302694872204,-67.3511117063321,-214.24934096818));
#223381=CARTESIAN_POINT('',(51.0503406624406,-67.3834674874005,-208.192630912054));
#223382=CARTESIAN_POINT('Ctrl Pts',(50.9302694862954,-67.35111170647,-214.249340968162));
#223383=CARTESIAN_POINT('Ctrl Pts',(50.9902625163406,-67.3672781287523,
-211.223956213722));
#223384=CARTESIAN_POINT('Ctrl Pts',(51.0503406624421,-67.3834674874009,
-208.192630912048));
#223385=CARTESIAN_POINT('',(51.0503406624406,-67.3834674874005,-215.85005));
#223386=CARTESIAN_POINT('',(51.0503406624406,-67.3834674874005,-208.192630912054));
#223387=CARTESIAN_POINT('',(48.9715866554311,-66.8233021636441,-215.85005));
#223388=CARTESIAN_POINT('',(52.3809255634408,-67.7420224291304,-215.85005));
#223389=CARTESIAN_POINT('Ctrl Pts',(50.930269487352,-67.3511117067547,-214.249340968478));
#223390=CARTESIAN_POINT('Ctrl Pts',(50.6138859321166,-67.2658553002478,
-214.510066201586));
#223391=CARTESIAN_POINT('Ctrl Pts',(50.2970498578574,-67.1804769526797,
-214.770075985769));
#223392=CARTESIAN_POINT('Ctrl Pts',(49.6441919995299,-67.0045502521929,
-215.303702766343));
#223393=CARTESIAN_POINT('Ctrl Pts',(49.308126257683,-66.9139900538979,-215.577233713243));
#223394=CARTESIAN_POINT('Ctrl Pts',(48.9715866554311,-66.8233021636442,
-215.85005));
#223395=CARTESIAN_POINT('Origin',(0.,-12.9675000200281,-167.906149834141));
#223396=CARTESIAN_POINT('Origin',(0.,-12.9675000200281,-208.192630912054));
#223397=CARTESIAN_POINT('Origin',(0.,-12.9675000200281,-215.85005));
#223398=CARTESIAN_POINT('Origin',(48.9106432152246,18.4987427374335,-167.906149834141));
#223399=CARTESIAN_POINT('',(54.1218033366501,38.2387592929899,-214.33352989342));
#223400=CARTESIAN_POINT('',(54.1539855075907,38.3606662320892,-208.192630912062));
#223401=CARTESIAN_POINT('Ctrl Pts',(54.1218033367874,38.2387592920601,-214.333529893402));
#223402=CARTESIAN_POINT('Ctrl Pts',(54.1378828568779,38.299668952361,-211.26613387672));
#223403=CARTESIAN_POINT('Ctrl Pts',(54.1539855075911,38.3606662320908,-208.192630912056));
#223404=CARTESIAN_POINT('',(54.1539855075907,38.3606662320892,-215.85005));
#223405=CARTESIAN_POINT('',(54.1539855075907,38.3606662320892,-208.192630912062));
#223406=CARTESIAN_POINT('',(53.6858060762413,36.5871897873468,-215.85005));
#223407=CARTESIAN_POINT('',(53.3004948454233,35.1276203445352,-215.85005));
#223408=CARTESIAN_POINT('Ctrl Pts',(54.1218033370754,38.2387592931511,-214.333529893716));
#223409=CARTESIAN_POINT('Ctrl Pts',(54.0493242413282,37.9642065032659,-214.587336490182));
#223410=CARTESIAN_POINT('Ctrl Pts',(53.9768175206474,37.6895490693776,-214.840391892315));
#223411=CARTESIAN_POINT('Ctrl Pts',(53.8314491180682,37.1388895988389,-215.346026703309));
#223412=CARTESIAN_POINT('Ctrl Pts',(53.7586988751255,36.8633096959893,-215.598218415187));
#223413=CARTESIAN_POINT('Ctrl Pts',(53.6858060762413,36.5871897873468,-215.85005));
#223414=CARTESIAN_POINT('Origin',(52.2560139340206,41.9262034053684,-167.906149834141));
#223415=CARTESIAN_POINT('',(50.9262492693411,41.5646183371225,-208.192630912063));
#223416=CARTESIAN_POINT('',(50.8045364442235,41.5315226009329,-214.335913275013));
#223417=CARTESIAN_POINT('Ctrl Pts',(50.9262492693426,41.5646183371229,-208.192630912057));
#223418=CARTESIAN_POINT('Ctrl Pts',(50.8653490995025,41.5480585708328,-211.267327940101));
#223419=CARTESIAN_POINT('Ctrl Pts',(50.8045364435665,41.5315226010249,-214.335913275001));
#223420=CARTESIAN_POINT('',(49.1680521502591,41.086535378401,-215.85005));
#223421=CARTESIAN_POINT('Ctrl Pts',(49.1680521502591,41.086535378401,-215.85005));
#223422=CARTESIAN_POINT('Ctrl Pts',(49.4414268426973,41.1608704915587,-215.598356099773));
#223423=CARTESIAN_POINT('Ctrl Pts',(49.7144017835735,41.2350969056362,-215.34641310643));
#223424=CARTESIAN_POINT('Ctrl Pts',(50.2599964077802,41.3834531333722,-214.841609804263));
#223425=CARTESIAN_POINT('Ctrl Pts',(50.5323141821189,41.4575008529682,-214.589028866932));
#223426=CARTESIAN_POINT('Ctrl Pts',(50.8045364443354,41.5315226012339,-214.335913275222));
#223427=CARTESIAN_POINT('',(50.9262492693411,41.5646183371225,-215.85005));
#223428=CARTESIAN_POINT('',(47.6970590536189,40.6865479570431,-215.85005));
#223429=CARTESIAN_POINT('',(50.9262492693411,41.5646183371225,-208.192630912063));
#223430=CARTESIAN_POINT('Origin',(0.,-12.9675000200281,-167.906149834141));
#223431=CARTESIAN_POINT('Origin',(0.,-12.9675000200281,-208.192630912063));
#223432=CARTESIAN_POINT('Origin',(0.,-12.9675000200281,-215.85005));
#223433=CARTESIAN_POINT('Ctrl Pts',(-34.6658396818824,-73.7171632516135,
-213.428100838228));
#223434=CARTESIAN_POINT('Ctrl Pts',(-32.4073514514297,-71.6005216742484,
-216.754800866966));
#223435=CARTESIAN_POINT('Ctrl Pts',(-30.1566827897054,-69.4835812050616,
-220.086775418501));
#223436=CARTESIAN_POINT('Ctrl Pts',(-27.9187794471678,-67.3680563271156,
-223.428575651002));
#223437=CARTESIAN_POINT('Ctrl Pts',(-25.6808761046303,-65.2525314491696,
-226.770375883505));
#223438=CARTESIAN_POINT('Ctrl Pts',(-23.4556914905361,-63.138057119071,
-230.121736209584));
#223439=CARTESIAN_POINT('Ctrl Pts',(-21.2513677279815,-61.0308575536349,
-233.492320591244));
#223440=CARTESIAN_POINT('Ctrl Pts',(-33.2915597883734,-73.6042889215327,
-213.3745249105));
#223441=CARTESIAN_POINT('Ctrl Pts',(-31.0883634812044,-71.468152600341,
-216.692012555656));
#223442=CARTESIAN_POINT('Ctrl Pts',(-28.8904868213221,-69.3312704464811,
-220.012578308794));
#223443=CARTESIAN_POINT('Ctrl Pts',(-26.7014864455845,-67.1937325026276,
-223.338673968425));
#223444=CARTESIAN_POINT('Ctrl Pts',(-24.5124860698469,-65.056194558774,
-226.664769628057));
#223445=CARTESIAN_POINT('Ctrl Pts',(-22.3321348006857,-62.9178895928583,
-229.996164050332));
#223446=CARTESIAN_POINT('Ctrl Pts',(-20.1678151009491,-60.7799059276903,
-233.338582766127));
#223447=CARTESIAN_POINT('Ctrl Pts',(-31.9147855165948,-73.552107297594,
-213.332282575322));
#223448=CARTESIAN_POINT('Ctrl Pts',(-29.762790671335,-71.4048671987398,
-216.642517917955));
#223449=CARTESIAN_POINT('Ctrl Pts',(-27.614141519417,-69.2569201923722,
-219.954463723004));
#223450=CARTESIAN_POINT('Ctrl Pts',(-25.4710721309401,-67.1080216677693,
-223.269410149594));
#223451=CARTESIAN_POINT('Ctrl Pts',(-23.3280027424632,-64.9591231431663,
-226.584356576184));
#223452=CARTESIAN_POINT('Ctrl Pts',(-21.1903744149072,-62.8092567666832,
-229.902202966067));
#223453=CARTESIAN_POINT('Ctrl Pts',(-19.0627867609462,-60.6582241972154,
-233.225804571524));
#223454=CARTESIAN_POINT('Ctrl Pts',(-30.5241947376933,-73.5610723424068,
-213.298768106724));
#223455=CARTESIAN_POINT('Ctrl Pts',(-28.4276303246862,-71.4106207619995,
-216.603490576449));
#223456=CARTESIAN_POINT('Ctrl Pts',(-26.3326980553541,-69.2597735546543,
-219.908997954485));
#223457=CARTESIAN_POINT('Ctrl Pts',(-24.2404948075278,-67.1083375120315,
-223.215865028164));
#223458=CARTESIAN_POINT('Ctrl Pts',(-22.1482915597014,-64.9569014694087,
-226.522732101843));
#223459=CARTESIAN_POINT('Ctrl Pts',(-20.0587460707107,-62.8048792414949,
-229.830915083866));
#223460=CARTESIAN_POINT('Ctrl Pts',(-17.9741423861937,-60.651964437303,
-233.141673289924));
#223461=CARTESIAN_POINT('Ctrl Pts',(-29.1336039587916,-73.5700373872195,
-213.265253638125));
#223462=CARTESIAN_POINT('Ctrl Pts',(-27.0924699780375,-71.4163743252592,
-216.564463234942));
#223463=CARTESIAN_POINT('Ctrl Pts',(-25.0512545912912,-69.2626269169363,
-219.863532185965));
#223464=CARTESIAN_POINT('Ctrl Pts',(-23.0099174841155,-67.1086533562937,
-223.162319906734));
#223465=CARTESIAN_POINT('Ctrl Pts',(-20.9685803769398,-64.9546797956511,
-226.461107627501));
#223466=CARTESIAN_POINT('Ctrl Pts',(-18.9271177265143,-62.8005017163066,
-229.759627201665));
#223467=CARTESIAN_POINT('Ctrl Pts',(-16.8854980114412,-60.6457046773906,
-233.057542008323));
#223468=CARTESIAN_POINT('Ctrl Pts',(-27.7294536429032,-73.6399428041704,
-213.240474674736));
#223469=CARTESIAN_POINT('Ctrl Pts',(-25.7480542838189,-71.4909831817195,
-216.535913459003));
#223470=CARTESIAN_POINT('Ctrl Pts',(-23.7650962505812,-69.3425324796987,
-219.83072032752));
#223471=CARTESIAN_POINT('Ctrl Pts',(-21.7795474514592,-67.1949306447615,
-223.124474795611));
#223472=CARTESIAN_POINT('Ctrl Pts',(-19.7939986523371,-65.0473288098244,
-226.418229263703));
#223473=CARTESIAN_POINT('Ctrl Pts',(-17.8059306828216,-62.9005566886187,
-229.710963422664));
#223474=CARTESIAN_POINT('Ctrl Pts',(-15.8131699469721,-60.7552971507389,
-233.001768361203));
#223475=CARTESIAN_POINT('Ctrl Pts',(-26.2966554094194,-73.7792956476785,
-213.222281607897));
#223476=CARTESIAN_POINT('Ctrl Pts',(-24.3872303655785,-71.6390760412356,
-216.515494177504));
#223477=CARTESIAN_POINT('Ctrl Pts',(-22.4748413392017,-69.5000413221554,
-219.807779103235));
#223478=CARTESIAN_POINT('Ctrl Pts',(-20.557339302015,-67.3632863153304,
-223.098617135674));
#223479=CARTESIAN_POINT('Ctrl Pts',(-18.6398372648283,-65.2265313085053,
-226.389455168113));
#223480=CARTESIAN_POINT('Ctrl Pts',(-16.7173760151126,-63.0919383281561,
-229.678857882383));
#223481=CARTESIAN_POINT('Ctrl Pts',(-14.7853232876922,-60.962226893778,
-232.965939947977));
#223482=CARTESIAN_POINT('Ctrl Pts',(-25.9384558510484,-73.8141338585555,
-213.217733341187));
#223483=CARTESIAN_POINT('Ctrl Pts',(-24.0470243860184,-71.6760992561146,
-216.510389357129));
#223484=CARTESIAN_POINT('Ctrl Pts',(-22.1522776113568,-69.5394185327696,
-219.802043797164));
#223485=CARTESIAN_POINT('Ctrl Pts',(-20.251787264654,-67.4053752329726,
-223.09215272069));
#223486=CARTESIAN_POINT('Ctrl Pts',(-18.3512969179511,-65.2713319331756,
-226.382261644216));
#223487=CARTESIAN_POINT('Ctrl Pts',(-16.4452373481854,-63.1397837380405,
-229.670831497314));
#223488=CARTESIAN_POINT('Ctrl Pts',(-14.5283616228722,-61.0139593295377,
-232.95698284467));
#223489=CARTESIAN_POINT('Ctrl Pts',(-25.5784605350385,-73.8533601027436,
-213.213609922838));
#223490=CARTESIAN_POINT('Ctrl Pts',(-23.7057733627891,-71.7177470584876,
-216.50580220452));
#223491=CARTESIAN_POINT('Ctrl Pts',(-21.829424123399,-69.5836623243557,
-219.796931745576));
#223492=CARTESIAN_POINT('Ctrl Pts',(-19.9466959826127,-67.4525975067612,
-223.08644224016));
#223493=CARTESIAN_POINT('Ctrl Pts',(-18.0639678418265,-65.3215326891668,
-226.375952734745));
#223494=CARTESIAN_POINT('Ctrl Pts',(-16.1750566993381,-63.193316429139,
-229.663842850422));
#223495=CARTESIAN_POINT('Ctrl Pts',(-14.2740735233503,-61.0717557132381,
-232.949279321911));
#223496=CARTESIAN_POINT('Ctrl Pts',(-25.2164735434195,-73.8971500307606,
-213.209914643405));
#223497=CARTESIAN_POINT('Ctrl Pts',(-23.3633710413988,-71.7641197332807,
-216.501723891369));
#223498=CARTESIAN_POINT('Ctrl Pts',(-21.5062602068635,-69.6327963210957,
-219.792419393228));
#223499=CARTESIAN_POINT('Ctrl Pts',(-19.6421180325743,-67.5049019292708,
-223.081443379649));
#223500=CARTESIAN_POINT('Ctrl Pts',(-17.7779758582852,-65.3770075374459,
-226.370467366069));
#223501=CARTESIAN_POINT('Ctrl Pts',(-15.9070218020806,-63.2523352409497,
-229.657807174511));
#223502=CARTESIAN_POINT('Ctrl Pts',(-14.0226731406951,-61.135361514269,
-232.942719688923));
#223503=CARTESIAN_POINT('Ctrl Pts',(-25.1938493564434,-73.8998869012617,
-213.20968368844));
#223504=CARTESIAN_POINT('Ctrl Pts',(-23.341970896312,-71.7670180254552,
-216.501468996797));
#223505=CARTESIAN_POINT('Ctrl Pts',(-21.48606246208,-69.635867195892,-219.792137371206));
#223506=CARTESIAN_POINT('Ctrl Pts',(-19.6230819106969,-67.5081709556776,
-223.081130950866));
#223507=CARTESIAN_POINT('Ctrl Pts',(-17.7601013593138,-65.3804747154633,
-226.370124530527));
#223508=CARTESIAN_POINT('Ctrl Pts',(-15.8902696210019,-63.2560239166879,
-229.657429944766));
#223509=CARTESIAN_POINT('Ctrl Pts',(-14.0069606167792,-61.1393368768334,
-232.942309711862));
#223510=CARTESIAN_POINT('Ctrl Pts',(-25.1712173883496,-73.9026415976708,
-213.209454406389));
#223511=CARTESIAN_POINT('Ctrl Pts',(-23.3205662528727,-71.7699347734086,
-216.501216091021));
#223512=CARTESIAN_POINT('Ctrl Pts',(-21.4658635039096,-69.6389571726479,
-219.791857693934));
#223513=CARTESIAN_POINT('Ctrl Pts',(-19.6040477936697,-67.5114598348967,
-223.080821306009));
#223514=CARTESIAN_POINT('Ctrl Pts',(-17.7422320834297,-65.3839624971454,
-226.369784918083));
#223515=CARTESIAN_POINT('Ctrl Pts',(-15.8735258224357,-63.2597340257226,
-229.657056446399));
#223516=CARTESIAN_POINT('Ctrl Pts',(-13.9912593731559,-61.1433349412254,
-232.941904217913));
#223517=CARTESIAN_POINT('Ctrl Pts',(-25.1485775908401,-73.9054141624873,
-213.20922679825));
#223518=CARTESIAN_POINT('Ctrl Pts',(-23.2991570846963,-71.7728700013293,
-216.500965172342));
#223519=CARTESIAN_POINT('Ctrl Pts',(-21.4456633269945,-69.64206625697,-219.791580356527));
#223520=CARTESIAN_POINT('Ctrl Pts',(-19.585015694187,-67.5147685546799,
-223.080514436398));
#223521=CARTESIAN_POINT('Ctrl Pts',(-17.7243680613796,-65.3874708523898,
-226.369448516269));
#223522=CARTESIAN_POINT('Ctrl Pts',(-15.8567904524812,-63.2634655201407,
-229.656686662215));
#223523=CARTESIAN_POINT('Ctrl Pts',(-13.9755694621469,-61.1473556487506,
-232.94150318618));
#223524=CARTESIAN_POINT('Ctrl Pts',(-25.1372576920853,-73.9068004448956,
-213.209112994182));
#223525=CARTESIAN_POINT('Ctrl Pts',(-23.2884525006082,-71.7743376152897,
-216.500839713002));
#223526=CARTESIAN_POINT('Ctrl Pts',(-21.435563238537,-69.6436207991311,
-219.791441687824));
#223527=CARTESIAN_POINT('Ctrl Pts',(-19.5754996444458,-67.5164229145716,
-223.080361001593));
#223528=CARTESIAN_POINT('Ctrl Pts',(-17.7154360503545,-65.3892250300121,
-226.369280315361));
#223529=CARTESIAN_POINT('Ctrl Pts',(-15.848422767504,-63.2653312673498,
-229.656501770123));
#223530=CARTESIAN_POINT('Ctrl Pts',(-13.9677245066424,-61.1493660025132,
-232.941302670313));
#223531=CARTESIAN_POINT('Ctrl Pts',(-25.1275380438543,-73.9076291783905,
-213.20952316564));
#223532=CARTESIAN_POINT('Ctrl Pts',(-23.2795399985599,-71.7751646462399,
-216.501290127757));
#223533=CARTESIAN_POINT('Ctrl Pts',(-21.4274775737994,-69.6444332830956,
-219.791935697107));
#223534=CARTESIAN_POINT('Ctrl Pts',(-19.5682702013894,-67.5171959518095,
-223.080900090889));
#223535=CARTESIAN_POINT('Ctrl Pts',(-17.7090628289793,-65.3899586205233,
-226.369864484671));
#223536=CARTESIAN_POINT('Ctrl Pts',(-15.8429357037125,-63.2660013665179,
-229.657133322639));
#223537=CARTESIAN_POINT('Ctrl Pts',(-13.9631639616011,-61.1499215051536,
-232.941973404526));
#223538=CARTESIAN_POINT('Ctrl Pts',(-25.1172506902082,-73.9086491431425,
-213.209748447694));
#223539=CARTESIAN_POINT('Ctrl Pts',(-23.2699927375599,-71.7762117787703,
-216.501537340245));
#223540=CARTESIAN_POINT('Ctrl Pts',(-21.4186793651933,-69.6455012585658,
-219.79220648111));
#223541=CARTESIAN_POINT('Ctrl Pts',(-19.5602329485478,-67.5182732019455,
-223.081194907277));
#223542=CARTESIAN_POINT('Ctrl Pts',(-17.7017865319023,-65.3910451453252,
-226.370183333444));
#223543=CARTESIAN_POINT('Ctrl Pts',(-15.836432876535,-63.267085758858,-229.657477064394));
#223544=CARTESIAN_POINT('Ctrl Pts',(-13.9574463443376,-61.150982255238,
-232.942337206168));
#223545=CARTESIAN_POINT('Ctrl Pts',(-25.106963336562,-73.9096691078946,
-213.209973729747));
#223546=CARTESIAN_POINT('Ctrl Pts',(-23.2604454765599,-71.7772589113006,
-216.501784552733));
#223547=CARTESIAN_POINT('Ctrl Pts',(-21.4098811565871,-69.6465692340359,
-219.792477265113));
#223548=CARTESIAN_POINT('Ctrl Pts',(-19.5521956957062,-67.5193504520815,
-223.081489723665));
#223549=CARTESIAN_POINT('Ctrl Pts',(-17.6945102348253,-65.392131670127,
-226.370502182217));
#223550=CARTESIAN_POINT('Ctrl Pts',(-15.8299300493574,-63.2681701511981,
-229.657820806149));
#223551=CARTESIAN_POINT('Ctrl Pts',(-13.9517287270741,-61.1520430053224,
-232.94270100781));
#223552=CARTESIAN_POINT('Ctrl Pts',(-25.0966732952022,-73.9106854314293,
-213.210198877687));
#223553=CARTESIAN_POINT('Ctrl Pts',(-23.250895955041,-71.7783021244353,
-216.502031618963));
#223554=CARTESIAN_POINT('Ctrl Pts',(-21.4010811306241,-69.6476330262175,
-219.792747904445));
#223555=CARTESIAN_POINT('Ctrl Pts',(-19.5441571297629,-67.5204232646219,
-223.081784431703));
#223556=CARTESIAN_POINT('Ctrl Pts',(-17.6872331289017,-65.3932135030263,
-226.370820958961));
#223557=CARTESIAN_POINT('Ctrl Pts',(-15.8234269724959,-63.2692496127142,
-229.658164546835));
#223558=CARTESIAN_POINT('Ctrl Pts',(-13.9460116075155,-61.1530985453856,
-232.943064954014));
#223559=CARTESIAN_POINT('Ctrl Pts',(-25.0863805784975,-73.9116981070231,
-213.210423891692));
#223560=CARTESIAN_POINT('Ctrl Pts',(-23.2413441840141,-71.7793414134067,
-216.502278538958));
#223561=CARTESIAN_POINT('Ctrl Pts',(-21.3922792967099,-69.6486926323558,
-219.793018398825));
#223562=CARTESIAN_POINT('Ctrl Pts',(-19.5361172580706,-67.5214916392076,
-223.082079030658));
#223563=CARTESIAN_POINT('Ctrl Pts',(-17.6799552194313,-65.3942906460594,
-226.371139662492));
#223564=CARTESIAN_POINT('Ctrl Pts',(-15.8169236486442,-63.2703241481874,
-229.658508284608));
#223565=CARTESIAN_POINT('Ctrl Pts',(-13.9402949855656,-61.1541488842789,
-232.943429042643));
#223566=CARTESIAN_POINT('Ctrl Pts',(-25.045209711679,-73.9157488093984,
-213.211323947711));
#223567=CARTESIAN_POINT('Ctrl Pts',(-23.2031370999064,-71.7834985692924,
-216.503266218939));
#223568=CARTESIAN_POINT('Ctrl Pts',(-21.3570719610534,-69.6529310569089,
-219.794100376343));
#223569=CARTESIAN_POINT('Ctrl Pts',(-19.5039577713016,-67.5257651375503,
-223.083257426481));
#223570=CARTESIAN_POINT('Ctrl Pts',(-17.6508435815496,-65.3985992181917,
-226.372414476619));
#223571=CARTESIAN_POINT('Ctrl Pts',(-15.790910353237,-63.2746222900799,
-229.659883235697));
#223572=CARTESIAN_POINT('Ctrl Pts',(-13.917428497766,-61.1583502398519,
-232.944885397156));
#223573=CARTESIAN_POINT('Ctrl Pts',(-25.0039960393562,-73.9197411446691,
-213.212221860696));
#223574=CARTESIAN_POINT('Ctrl Pts',(-23.1648940236841,-71.7875929385222,
-216.504251559075));
#223575=CARTESIAN_POINT('Ctrl Pts',(-21.3218356981714,-69.6571025047546,
-219.795180034489));
#223576=CARTESIAN_POINT('Ctrl Pts',(-19.4717773925363,-67.5299676286889,
-223.084434076858));
#223577=CARTESIAN_POINT('Ctrl Pts',(-17.621719086901,-65.4028327526231,
-226.373688119226));
#223578=CARTESIAN_POINT('Ctrl Pts',(-15.764893105952,-63.2788416156206,
-229.661258140053));
#223579=CARTESIAN_POINT('Ctrl Pts',(-13.8945699719964,-61.1624683771664,
-232.946344030549));
#223580=CARTESIAN_POINT('Ctrl Pts',(-24.9627403530703,-73.923674682942,
-213.213117642504));
#223581=CARTESIAN_POINT('Ctrl Pts',(-23.1266156599325,-71.7916242163186,
-216.505234561518));
#223582=CARTESIAN_POINT('Ctrl Pts',(-21.2865711101685,-69.6612067996797,
-219.796257356156));
#223583=CARTESIAN_POINT('Ctrl Pts',(-19.4395765925336,-67.534099089021,
-223.085608935934));
#223584=CARTESIAN_POINT('Ctrl Pts',(-17.5925820748987,-65.4069913783622,
-226.374960515711));
#223585=CARTESIAN_POINT('Ctrl Pts',(-15.7388720794572,-63.2829824280842,
-229.662632880376));
#223586=CARTESIAN_POINT('Ctrl Pts',(-13.8717193997808,-61.1665038590062,
-232.947804805375));
#223587=CARTESIAN_POINT('Ctrl Pts',(-24.8802289804986,-73.9315417594878,
-213.214909206118));
#223588=CARTESIAN_POINT('Ctrl Pts',(-23.050058932429,-71.7996867719115,
-216.507200566404));
#223589=CARTESIAN_POINT('Ctrl Pts',(-21.2160419341625,-69.6694153895299,
-219.79841199949));
#223590=CARTESIAN_POINT('Ctrl Pts',(-19.3751749925283,-67.5423620096852,
-223.087958654085));
#223591=CARTESIAN_POINT('Ctrl Pts',(-17.534308050894,-65.4153086298405,
-226.37750530868));
#223592=CARTESIAN_POINT('Ctrl Pts',(-15.6868300264676,-63.2912640530112,
-229.665382361023));
#223593=CARTESIAN_POINT('Ctrl Pts',(-13.8260182553497,-61.1745748226858,
-232.950726355029));
#223594=CARTESIAN_POINT('Ctrl Pts',(-24.7975495521845,-73.9391736473788,
-213.216692244198));
#223595=CARTESIAN_POINT('Ctrl Pts',(-22.9733610549633,-71.8074969612026,
-216.509157219437));
#223596=CARTESIAN_POINT('Ctrl Pts',(-21.1453994575107,-69.6773553674969,
-219.800557295378));
#223597=CARTESIAN_POINT('Ctrl Pts',(-19.3106917073121,-67.5503408080304,
-223.090301205408));
#223598=CARTESIAN_POINT('Ctrl Pts',(-17.4759839571134,-65.4233262485639,
-226.380045115437));
#223599=CARTESIAN_POINT('Ctrl Pts',(-15.6347728560193,-63.2992316298716,
-229.668131184037));
#223600=CARTESIAN_POINT('Ctrl Pts',(-13.7803489284904,-61.1823151706218,
-232.953656471305));
#223601=CARTESIAN_POINT('Ctrl Pts',(-24.7147083990042,-73.9465669153705,
-213.218466861474));
#223602=CARTESIAN_POINT('Ctrl Pts',(-22.8965276622237,-71.8150523527114,
-216.511104550879));
#223603=CARTESIAN_POINT('Ctrl Pts',(-21.0746484989569,-69.6850253260783,
-219.802693125391));
#223604=CARTESIAN_POINT('Ctrl Pts',(-19.2461305058836,-67.5580352841057,
-223.092636242468));
#223605=CARTESIAN_POINT('Ctrl Pts',(-17.4176125128103,-65.431045242133,
-226.382579359545));
#223606=CARTESIAN_POINT('Ctrl Pts',(-15.5827019558309,-63.3068875335073,
-229.67087842819));
#223607=CARTESIAN_POINT('Ctrl Pts',(-13.7347113090203,-61.1897293326622,
-232.956594042948));
#223608=CARTESIAN_POINT('Ctrl Pts',(-24.5490260926436,-73.9613534513537,
-213.222016096024));
#223609=CARTESIAN_POINT('Ctrl Pts',(-22.7428608767445,-71.8301631357291,
-216.51499921376));
#223610=CARTESIAN_POINT('Ctrl Pts',(-20.9331465818493,-69.7003652432411,
-219.806964785417));
#223611=CARTESIAN_POINT('Ctrl Pts',(-19.1170081030267,-67.5734242362562,
-223.097306316589));
#223612=CARTESIAN_POINT('Ctrl Pts',(-17.3008696242042,-65.4464832292714,
-226.387647847762));
#223613=CARTESIAN_POINT('Ctrl Pts',(-15.478560155454,-63.3221993407787,
-229.676372916496));
#223614=CARTESIAN_POINT('Ctrl Pts',(-13.64343607008,-61.2045576567429,-232.962469186234));
#223615=CARTESIAN_POINT('Ctrl Pts',(-24.382696887998,-73.9751854967928,
-213.225531634411));
#223616=CARTESIAN_POINT('Ctrl Pts',(-22.5886520321449,-71.8442547181521,
-216.518856573352));
#223617=CARTESIAN_POINT('Ctrl Pts',(-20.79121073452,-69.7146250786933,-219.811198558066));
#223618=CARTESIAN_POINT('Ctrl Pts',(-18.987574030311,-67.5876759125815,
-223.101946307423));
#223619=CARTESIAN_POINT('Ctrl Pts',(-17.183937326102,-65.4607267464698,
-226.39269405678));
#223620=CARTESIAN_POINT('Ctrl Pts',(-15.3743634215613,-63.3362645204375,
-229.681861061496));
#223621=CARTESIAN_POINT('Ctrl Pts',(-13.5522877040622,-61.2180813417051,
-232.968374159806));
#223622=CARTESIAN_POINT('Ctrl Pts',(-24.2157714140078,-73.9880357308615,
-213.229014471039));
#223623=CARTESIAN_POINT('Ctrl Pts',(-22.4339461787348,-71.8573077591623,
-216.522677077293));
#223624=CARTESIAN_POINT('Ctrl Pts',(-20.6488795380216,-69.7277936159865,
-219.815393786219));
#223625=CARTESIAN_POINT('Ctrl Pts',(-18.8578584941732,-67.6007885459744,
-223.106553748693));
#223626=CARTESIAN_POINT('Ctrl Pts',(-17.0668374503248,-65.4737834759622,
-226.397713711166));
#223627=CARTESIAN_POINT('Ctrl Pts',(-15.2701229993362,-63.3491012702364,
-229.687335801966));
#223628=CARTESIAN_POINT('Ctrl Pts',(-13.4612647392615,-61.230334612939,
-232.974299931676));
#223629=CARTESIAN_POINT('Ctrl Pts',(-23.5480695180473,-74.0394366671362,
-213.24294581755));
#223630=CARTESIAN_POINT('Ctrl Pts',(-21.8151227650944,-71.9095199232031,
-216.537959093058));
#223631=CARTESIAN_POINT('Ctrl Pts',(-20.0795547520278,-69.7804677651596,
-219.832174698832));
#223632=CARTESIAN_POINT('Ctrl Pts',(-18.3389963496219,-67.6532390795458,
-223.124983513772));
#223633=CARTESIAN_POINT('Ctrl Pts',(-16.598437947216,-65.526010393932,-226.417792328712));
#223634=CARTESIAN_POINT('Ctrl Pts',(-14.8531613104359,-63.4004482694319,
-229.709234763845));
#223635=CARTESIAN_POINT('Ctrl Pts',(-13.0971728800584,-61.279347697875,
-232.998003019155));
#223636=CARTESIAN_POINT('Ctrl Pts',(-22.8709481805904,-74.0750232880782,
-213.256420242625));
#223637=CARTESIAN_POINT('Ctrl Pts',(-21.1884296153893,-71.9450395755471,
-216.552700075075));
#223638=CARTESIAN_POINT('Ctrl Pts',(-19.5039372878188,-69.8156379211665,
-219.84836591417));
#223639=CARTESIAN_POINT('Ctrl Pts',(-17.815594292309,-67.6874631000348,
-223.142892403823));
#223640=CARTESIAN_POINT('Ctrl Pts',(-16.1272512967992,-65.5592882789031,
-226.437418893476));
#223641=CARTESIAN_POINT('Ctrl Pts',(-14.4353045594034,-63.4322301175141,
-229.730858925088));
#223642=CARTESIAN_POINT('Ctrl Pts',(-12.7347707201458,-61.3081954246526,
-233.021942401312));
#223643=CARTESIAN_POINT('Ctrl Pts',(-22.1870742035844,-74.0934804397452,
-213.269235878432));
#223644=CARTESIAN_POINT('Ctrl Pts',(-20.5563486581325,-71.9629449474399,
-216.566743885946));
#223645=CARTESIAN_POINT('Ctrl Pts',(-18.9243205135762,-69.8327666793282,
-219.863841772444));
#223646=CARTESIAN_POINT('Ctrl Pts',(-17.2897176470888,-67.7033388994737,
-223.160157702189));
#223647=CARTESIAN_POINT('Ctrl Pts',(-15.6551147806014,-65.5739111196192,
-226.456473631933));
#223648=CARTESIAN_POINT('Ctrl Pts',(-14.0181153557779,-63.4451661048354,
-229.752051509661));
#223649=CARTESIAN_POINT('Ctrl Pts',(-12.3752611396659,-61.3182690712574,
-233.045942634108));
#223650=CARTESIAN_POINT('Ctrl Pts',(-20.8193262495723,-74.1303947430791,
-213.294867150045));
#223651=CARTESIAN_POINT('Ctrl Pts',(-19.292186743619,-71.9987556912256,
-216.594831507688));
#223652=CARTESIAN_POINT('Ctrl Pts',(-17.765086965091,-69.8670241956515,
-219.894793488995));
#223653=CARTESIAN_POINT('Ctrl Pts',(-16.2379643566484,-67.7350904983513,
-223.194688298921));
#223654=CARTESIAN_POINT('Ctrl Pts',(-14.7108417482059,-65.6031568010512,
-226.494583108848));
#223655=CARTESIAN_POINT('Ctrl Pts',(-13.183736948527,-63.471038079478,-229.794436678806));
#223656=CARTESIAN_POINT('Ctrl Pts',(-11.656241978706,-61.3384163644669,
-233.0939430997));
#223657=CARTESIAN_POINT('Ctrl Pts',(-19.42533001526,-74.0979893885821,-213.31813023739));
#223658=CARTESIAN_POINT('Ctrl Pts',(-18.0070778075469,-71.9634650061569,
-216.620336307912));
#223659=CARTESIAN_POINT('Ctrl Pts',(-16.5902654999009,-69.828635705168,
-219.92301297597));
#223660=CARTESIAN_POINT('Ctrl Pts',(-15.1764619582282,-67.6931640554203,
-223.226671478159));
#223661=CARTESIAN_POINT('Ctrl Pts',(-13.7626584165554,-65.5576924056727,
-226.53032998035));
#223662=CARTESIAN_POINT('Ctrl Pts',(-12.3515772232236,-63.4216427758456,
-229.834879431719));
#223663=CARTESIAN_POINT('Ctrl Pts',(-10.9479532026315,-61.283976471277,
-233.141846820839));
#223664=CARTESIAN_POINT('Ctrl Pts',(-18.0356123358475,-73.9925802279181,
-213.337833927419));
#223665=CARTESIAN_POINT('Ctrl Pts',(-16.7281499098072,-71.8547048439425,
-216.642247555954));
#223666=CARTESIAN_POINT('Ctrl Pts',(-15.4235797449757,-69.7165429992464,
-219.947634512311));
#223667=CARTESIAN_POINT('Ctrl Pts',(-14.1251185099843,-67.5779955815407,
-223.255219367307));
#223668=CARTESIAN_POINT('Ctrl Pts',(-12.8266572749929,-65.4394481638349,
-226.562804222303));
#223669=CARTESIAN_POINT('Ctrl Pts',(-11.5337362244292,-63.3004500825909,
-229.872316979927));
#223670=CARTESIAN_POINT('Ctrl Pts',(-10.2559925260515,-61.1612854472115,
-233.187802584486));
#223671=CARTESIAN_POINT('Ctrl Pts',(-17.6881829159944,-73.9662279377521,
-213.342759849927));
#223672=CARTESIAN_POINT('Ctrl Pts',(-16.4084179353722,-71.8275148033889,
-216.647725367964));
#223673=CARTESIAN_POINT('Ctrl Pts',(-15.1319083062445,-69.688519822766,
-219.953789896397));
#223674=CARTESIAN_POINT('Ctrl Pts',(-13.8622826479234,-67.5492034630707,
-223.262356339594));
#223675=CARTESIAN_POINT('Ctrl Pts',(-12.5926569896023,-65.4098871033754,
-226.570922782791));
#223676=CARTESIAN_POINT('Ctrl Pts',(-11.3292759747306,-63.2701519092773,
-229.881676366978));
#223677=CARTESIAN_POINT('Ctrl Pts',(-10.0830023569065,-61.1306126911951,
-233.199291525398));
#223678=CARTESIAN_POINT('Ctrl Pts',(-17.3409698674155,-73.935384443929,
-213.34743873701));
#223679=CARTESIAN_POINT('Ctrl Pts',(-16.0890297520637,-71.7957877789297,
-216.65295762787));
#223680=CARTESIAN_POINT('Ctrl Pts',(-14.8407142907582,-69.6559284272906,
-219.959704440269));
#223681=CARTESIAN_POINT('Ctrl Pts',(-13.6000677993871,-67.5158548561218,
-223.269270451958));
#223682=CARTESIAN_POINT('Ctrl Pts',(-12.3594213080159,-65.375781284953,
-226.578836463649));
#223683=CARTESIAN_POINT('Ctrl Pts',(-11.1257374792571,-63.2353536891053,
-229.890858807334));
#223684=CARTESIAN_POINT('Ctrl Pts',(-9.91109018312546,-61.0956375485126,
-233.210683839047));
#223685=CARTESIAN_POINT('Ctrl Pts',(-16.9945696080803,-73.9001081635259,
-213.351879630837));
#223686=CARTESIAN_POINT('Ctrl Pts',(-15.7705099053272,-71.7595755214746,
-216.657951790479));
#223687=CARTESIAN_POINT('Ctrl Pts',(-14.5504477647407,-69.6188149294866,
-219.965383361714));
#223688=CARTESIAN_POINT('Ctrl Pts',(-13.3388364480016,-67.4779925971457,
-223.275961013327));
#223689=CARTESIAN_POINT('Ctrl Pts',(-12.1272251312625,-65.3371702648048,
-226.586538664941));
#223690=CARTESIAN_POINT('Ctrl Pts',(-10.9233008549777,-63.1960951941825,
-229.899850654492));
#223691=CARTESIAN_POINT('Ctrl Pts',(-9.74027549479166,-61.0564003174778,
-233.221936356199));
#223692=CARTESIAN_POINT('Ctrl Pts',(-16.8213694784127,-73.8824700233243,
-213.35410007775));
#223693=CARTESIAN_POINT('Ctrl Pts',(-15.611249981959,-71.7414693927469,
-216.660448871784));
#223694=CARTESIAN_POINT('Ctrl Pts',(-14.4053145017319,-69.6002581805847,
-219.968222822436));
#223695=CARTESIAN_POINT('Ctrl Pts',(-13.2082207723089,-67.4590614676576,
-223.279306294012));
#223696=CARTESIAN_POINT('Ctrl Pts',(-12.0111270428858,-65.3178647547306,
-226.590389765587));
#223697=CARTESIAN_POINT('Ctrl Pts',(-10.822082542838,-63.1764659467212,
-229.904346578071));
#223698=CARTESIAN_POINT('Ctrl Pts',(-9.65486815062476,-61.0367817019604,
-233.227562614775));
#223699=CARTESIAN_POINT('Ctrl Pts',(-16.6483725774174,-73.8637237686103,
-213.356261096586));
#223700=CARTESIAN_POINT('Ctrl Pts',(-15.4522071799355,-71.7222420367263,
-216.662886513868));
#223701=CARTESIAN_POINT('Ctrl Pts',(-14.2604131527873,-69.5805709842817,
-219.971003481449));
#223702=CARTESIAN_POINT('Ctrl Pts',(-13.0778510032714,-67.4390019693148,
-223.282595807161));
#223703=CARTESIAN_POINT('Ctrl Pts',(-11.8952888537556,-65.297432954348,
-226.594188132872));
#223704=CARTESIAN_POINT('Ctrl Pts',(-10.7211396966759,-63.1557216095298,
-229.908795015727));
#223705=CARTESIAN_POINT('Ctrl Pts',(-9.5697351055252,-61.0160972517994,
-233.233154034774));
#223706=CARTESIAN_POINT('Ctrl Pts',(-16.475653681056,-73.8438772043605,
-213.358364250325));
#223707=CARTESIAN_POINT('Ctrl Pts',(-15.293447315483,-71.7019004243738,
-216.665266171061));
#223708=CARTESIAN_POINT('Ctrl Pts',(-14.1158002338706,-69.5597595986402,
-219.973726626617));
#223709=CARTESIAN_POINT('Ctrl Pts',(-12.9477726440157,-67.4178197482303,
-223.28583020421));
#223710=CARTESIAN_POINT('Ctrl Pts',(-11.7797450541607,-65.2758798978204,
-226.597933781803));
#223711=CARTESIAN_POINT('Ctrl Pts',(-10.6204947589615,-63.133867051308,
-229.913195248457));
#223712=CARTESIAN_POINT('Ctrl Pts',(-9.48487851766271,-60.9943501153288,
-233.238705966824));
#223713=CARTESIAN_POINT('Ctrl Pts',(-16.3892942328753,-73.8339539222356,
-213.359415827195));
#223714=CARTESIAN_POINT('Ctrl Pts',(-15.2140673832569,-71.6917296181976,
-216.666455999658));
#223715=CARTESIAN_POINT('Ctrl Pts',(-14.0434937744123,-69.5493539058194,
-219.9750881992));
#223716=CARTESIAN_POINT('Ctrl Pts',(-12.8827334643878,-67.407228637688,
-223.287447402734));
#223717=CARTESIAN_POINT('Ctrl Pts',(-11.7219731543633,-65.2651033695566,
-226.599806606268));
#223718=CARTESIAN_POINT('Ctrl Pts',(-10.5701722901042,-63.1229397721972,
-229.915395364823));
#223719=CARTESIAN_POINT('Ctrl Pts',(-9.44245022373146,-60.9834765470935,
-233.241481932849));
#223720=CARTESIAN_POINT('Ctrl Pts',(-16.3030042884726,-73.8237555680483,
-213.360452942392));
#223721=CARTESIAN_POINT('Ctrl Pts',(-15.1347581882095,-71.6812802533029,
-216.667631337573));
#223722=CARTESIAN_POINT('Ctrl Pts',(-13.9712594252062,-69.5386671710029,
-219.976435400044));
#223723=CARTESIAN_POINT('Ctrl Pts',(-12.8177671391991,-67.3963568497133,
-223.289050830054));
#223724=CARTESIAN_POINT('Ctrl Pts',(-11.664274853192,-65.2540465284237,
-226.601666260063));
#223725=CARTESIAN_POINT('Ctrl Pts',(-10.5199242971055,-63.1117349369396,
-229.917583440331));
#223726=CARTESIAN_POINT('Ctrl Pts',(-9.40009104247648,-60.9723372875069,
-233.244248035339));
#223727=CARTESIAN_POINT('Ctrl Pts',(-16.2167932117529,-73.8132831498086,
-213.361475819387));
#223728=CARTESIAN_POINT('Ctrl Pts',(-15.0555279749204,-71.6705532338771,
-216.66879240035));
#223729=CARTESIAN_POINT('Ctrl Pts',(-13.8991042674645,-69.5277002093067,
-219.977768430969));
#223730=CARTESIAN_POINT('Ctrl Pts',(-12.7528793682143,-67.3852051104264,
-223.290640615083));
#223731=CARTESIAN_POINT('Ctrl Pts',(-11.6066544689641,-65.242710011546,
-226.603512799196));
#223732=CARTESIAN_POINT('Ctrl Pts',(-10.4697535757229,-63.1002531490252,
-229.919759447508));
#223733=CARTESIAN_POINT('Ctrl Pts',(-9.35780123872676,-60.9609326117215,
-233.247003746217));
#223734=CARTESIAN_POINT('Ctrl Pts',(-16.1952404425729,-73.8106650452487,
-213.361731538637));
#223735=CARTESIAN_POINT('Ctrl Pts',(-15.0357204215981,-71.6678714790206,
-216.669082666044));
#223736=CARTESIAN_POINT('Ctrl Pts',(-13.8810654780291,-69.5249584688827,
-219.9781016887));
#223737=CARTESIAN_POINT('Ctrl Pts',(-12.7366574254681,-67.3824171756047,
-223.29103806134));
#223738=CARTESIAN_POINT('Ctrl Pts',(-11.5922493729072,-65.2398758823266,
-226.60397443398));
#223739=CARTESIAN_POINT('Ctrl Pts',(-10.4572108953772,-63.0973827020465,
-229.920303449302));
#223740=CARTESIAN_POINT('Ctrl Pts',(-9.34722878778933,-60.9580814427752,
-233.247692673936));
#223741=CARTESIAN_POINT('Ctrl Pts',(-16.1749279659312,-73.8079309222085,
-213.362368684823));
#223742=CARTESIAN_POINT('Ctrl Pts',(-15.0172739344155,-71.6650756920887,
-216.669799089985));
#223743=CARTESIAN_POINT('Ctrl Pts',(-13.8645330142372,-69.5221076454515,
-219.978916472587));
#223744=CARTESIAN_POINT('Ctrl Pts',(-12.7221372554057,-67.3795379414851,
-223.291998591574));
#223745=CARTESIAN_POINT('Ctrl Pts',(-11.5797414965742,-65.2369682375188,
-226.605080710561));
#223746=CARTESIAN_POINT('Ctrl Pts',(-10.4468084359715,-63.0944652668042,
-229.921596248607));
#223747=CARTESIAN_POINT('Ctrl Pts',(-9.33915242519547,-60.9552650705159,
-233.249310581749));
#223748=CARTESIAN_POINT('Ctrl Pts',(-16.1509595327512,-73.8054672009616,
-213.361871023763));
#223749=CARTESIAN_POINT('Ctrl Pts',(-14.9948134280635,-71.6625434043229,
-216.669248038006));
#223750=CARTESIAN_POINT('Ctrl Pts',(-13.8435558938145,-69.5195048912895,
-219.978299602301));
#223751=CARTESIAN_POINT('Ctrl Pts',(-12.702592770651,-67.376854004913,-223.291285721626));
#223752=CARTESIAN_POINT('Ctrl Pts',(-11.5616296474874,-65.2342031185365,
-226.60427184095));
#223753=CARTESIAN_POINT('Ctrl Pts',(-10.4300813444879,-63.0916122772293,
-229.920665266036));
#223754=CARTESIAN_POINT('Ctrl Pts',(-9.32369428622946,-60.9522734066326,
-233.248170744692));
#223755=CARTESIAN_POINT('Ctrl Pts',(-16.1269910995712,-73.8030034797147,
-213.361373362703));
#223756=CARTESIAN_POINT('Ctrl Pts',(-14.9723529217116,-71.660011116557,
-216.668696986026));
#223757=CARTESIAN_POINT('Ctrl Pts',(-13.8225787733917,-69.5169021371276,
-219.977682732017));
#223758=CARTESIAN_POINT('Ctrl Pts',(-12.6830482858962,-67.3741700683409,
-223.290572851677));
#223759=CARTESIAN_POINT('Ctrl Pts',(-11.5435177984007,-65.2314379995542,
-226.603462971339));
#223760=CARTESIAN_POINT('Ctrl Pts',(-10.4133542530044,-63.0887592876544,
-229.919734283464));
#223761=CARTESIAN_POINT('Ctrl Pts',(-9.30823614726345,-60.9492817427492,
-233.247030907634));
#223762=CARTESIAN_POINT('Ctrl Pts',(-16.103019054535,-73.8005584760351,
-213.360877925168));
#223763=CARTESIAN_POINT('Ctrl Pts',(-14.9498889438717,-71.6574980953291,
-216.668148455574));
#223764=CARTESIAN_POINT('Ctrl Pts',(-13.80159836519,-69.5143192404771,-219.977068760275));
#223765=CARTESIAN_POINT('Ctrl Pts',(-12.6635007640913,-67.3715067403955,
-223.289863459617));
#223766=CARTESIAN_POINT('Ctrl Pts',(-11.5254031629927,-65.2286942403139,
-226.602658158959));
#223767=CARTESIAN_POINT('Ctrl Pts',(-10.3966247242771,-63.0859285253037,
-229.918808118652));
#223768=CARTESIAN_POINT('Ctrl Pts',(-9.29277587349895,-60.9463138180459,
-233.245897218204));
#223769=CARTESIAN_POINT('Ctrl Pts',(-16.0790434247684,-73.7981321994186,
-213.360384703604));
#223770=CARTESIAN_POINT('Ctrl Pts',(-14.9274215266728,-71.6550043474074,
-216.66760243706));
#223771=CARTESIAN_POINT('Ctrl Pts',(-13.7806147058298,-69.5117562048794,
-219.976457674749));
#223772=CARTESIAN_POINT('Ctrl Pts',(-12.643950246094,-67.3688640192604,
-223.28915752863));
#223773=CARTESIAN_POINT('Ctrl Pts',(-11.5072857863581,-65.2259718336413,
-226.601857382511));
#223774=CARTESIAN_POINT('Ctrl Pts',(-10.379892806367,-63.0831199759327,
-229.917886743822));
#223775=CARTESIAN_POINT('Ctrl Pts',(-9.27731352151551,-60.9433696029743,
-233.244769639116));
#223776=CARTESIAN_POINT('Ctrl Pts',(-16.0310921652353,-73.7932796461856,
-213.359398260476));
#223777=CARTESIAN_POINT('Ctrl Pts',(-14.8824866922748,-71.6500168515638,
-216.666510400032));
#223778=CARTESIAN_POINT('Ctrl Pts',(-13.7386473871094,-69.5066301336839,
-219.975235503696));
#223779=CARTESIAN_POINT('Ctrl Pts',(-12.6048492100992,-67.36357857699,-223.287745666656));
#223780=CARTESIAN_POINT('Ctrl Pts',(-11.471051033089,-65.220527020296,-226.600255829615));
#223781=CARTESIAN_POINT('Ctrl Pts',(-10.3464289705466,-63.0775028771908,
-229.916043994163));
#223782=CARTESIAN_POINT('Ctrl Pts',(-9.24638881754862,-60.9374811728312,
-233.242514480938));
#223783=CARTESIAN_POINT('Ctrl Pts',(-15.9831265667899,-73.7885020011607,
-213.358420681147));
#223784=CARTESIAN_POINT('Ctrl Pts',(-14.8375381004534,-71.6451064488818,
-216.665428410643));
#223785=CARTESIAN_POINT('Ctrl Pts',(-13.6966670637724,-69.5015835066084,
-219.974024877362));
#223786=CARTESIAN_POINT('Ctrl Pts',(-12.565736189382,-67.3583755618043,
-223.286347648786));
#223787=CARTESIAN_POINT('Ctrl Pts',(-11.4348053149916,-65.2151676170003,
-226.598670420209));
#223788=CARTESIAN_POINT('Ctrl Pts',(-10.3129555781029,-63.0719746300436,
-229.914220404117));
#223789=CARTESIAN_POINT('Ctrl Pts',(-9.21545580106647,-60.9316875806773,
-233.24028376377));
#223790=CARTESIAN_POINT('Ctrl Pts',(-15.9351468463194,-73.7837993408402,
-213.357451906235));
#223791=CARTESIAN_POINT('Ctrl Pts',(-14.7925760080749,-71.6402731942684,
-216.664356393475));
#223792=CARTESIAN_POINT('Ctrl Pts',(-13.6546740285727,-69.496616353084,
-219.972825698813));
#223793=CARTESIAN_POINT('Ctrl Pts',(-12.5266115102174,-67.3532549610625,
-223.284963342766));
#223794=CARTESIAN_POINT('Ctrl Pts',(-11.3985489918621,-65.209893569041,
-226.597100986719));
#223795=CARTESIAN_POINT('Ctrl Pts',(-10.2794730121742,-63.066535124477,
-229.912415755275));
#223796=CARTESIAN_POINT('Ctrl Pts',(-9.18451492026534,-60.9259885966326,
-233.238077193559));
#223797=CARTESIAN_POINT('Ctrl Pts',(-15.1674713187905,-73.7085567757124,
-213.341951507641));
#223798=CARTESIAN_POINT('Ctrl Pts',(-14.0731825300186,-71.5629411204543,
-216.64720411878));
#223799=CARTESIAN_POINT('Ctrl Pts',(-12.9827854653765,-69.4171418966931,
-219.953638842029));
#223800=CARTESIAN_POINT('Ctrl Pts',(-11.9006166435836,-67.2713253491929,
-223.262814446454));
#223801=CARTESIAN_POINT('Ctrl Pts',(-10.8184478217907,-65.1255088016927,
-226.571990050878));
#223802=CARTESIAN_POINT('Ctrl Pts',(-9.74375195731604,-62.9795030354101,
-229.88354137378));
#223803=CARTESIAN_POINT('Ctrl Pts',(-8.68946082744711,-60.8348048519179,
-233.202772070185));
#223804=CARTESIAN_POINT('Ctrl Pts',(-14.3961811415349,-73.6525070500062,
-213.328697733291));
#223805=CARTESIAN_POINT('Ctrl Pts',(-13.3503336845521,-71.5053542835831,
-216.632595555745));
#223806=CARTESIAN_POINT('Ctrl Pts',(-12.3076436285635,-69.3580059281157,
-219.937370861218));
#223807=CARTESIAN_POINT('Ctrl Pts',(-11.2716399932958,-67.2104822157957,
-223.24415985318));
#223808=CARTESIAN_POINT('Ctrl Pts',(-10.2356363580282,-65.0629585034757,
-226.550948845142));
#223809=CARTESIAN_POINT('Ctrl Pts',(-9.20568876581819,-62.9151648957076,
-229.859489304317));
#223810=CARTESIAN_POINT('Ctrl Pts',(-8.19241564950965,-60.7677996422107,
-233.173615252749));
#223811=CARTESIAN_POINT('Ctrl Pts',(-13.6221605046832,-73.6159852550019,
-213.31749452838));
#223812=CARTESIAN_POINT('Ctrl Pts',(-12.6250760081642,-71.4677688674574,
-216.620281085237));
#223813=CARTESIAN_POINT('Ctrl Pts',(-11.6304405856088,-69.3193741723362,
-219.923700795082));
#223814=CARTESIAN_POINT('Ctrl Pts',(-10.640997887323,-67.1707515656038,
-223.228560662602));
#223815=CARTESIAN_POINT('Ctrl Pts',(-9.65155518903714,-65.0221289588714,
-226.533420530121));
#223816=CARTESIAN_POINT('Ctrl Pts',(-8.66680721407077,-62.8732305917486,
-229.839537084505));
#223817=CARTESIAN_POINT('Ctrl Pts',(-7.69505740665787,-60.7243047821025,
-233.149611908546));
#223818=CARTESIAN_POINT('Ctrl Pts',(-12.07411923098,-73.5429416649933,-213.295088118557));
#223819=CARTESIAN_POINT('Ctrl Pts',(-11.1745606553882,-71.392598035206,
-216.595652144222));
#223820=CARTESIAN_POINT('Ctrl Pts',(-10.2760344996993,-69.2421106607772,
-219.89636066281));
#223821=CARTESIAN_POINT('Ctrl Pts',(-9.37971367537722,-67.09129026522,-223.197362281445));
#223822=CARTESIAN_POINT('Ctrl Pts',(-8.48339285105508,-64.9404698696628,
-226.498363900081));
#223823=CARTESIAN_POINT('Ctrl Pts',(-7.58904411057593,-62.7893619838305,
-229.79963264488));
#223824=CARTESIAN_POINT('Ctrl Pts',(-6.70034092095431,-60.6373150618862,
-233.101605220139));
#223825=CARTESIAN_POINT('Ctrl Pts',(-10.5152913094354,-73.5480397670874,
-213.280876146804));
#223826=CARTESIAN_POINT('Ctrl Pts',(-9.71465477633019,-71.3974778260467,
-216.58020457724));
#223827=CARTESIAN_POINT('Ctrl Pts',(-8.91375512880964,-69.2469206315281,
-219.879431150906));
#223828=CARTESIAN_POINT('Ctrl Pts',(-8.11230379659613,-67.0963349552283,
-223.178417000718));
#223829=CARTESIAN_POINT('Ctrl Pts',(-7.31085246438261,-64.9457492789285,
-226.47740285053));
#223830=CARTESIAN_POINT('Ctrl Pts',(-6.50890496550992,-62.7951562480888,
-229.776184191023));
#223831=CARTESIAN_POINT('Ctrl Pts',(-5.70557348161402,-60.6443501137825,
-233.074265786289));
#223832=CARTESIAN_POINT('Ctrl Pts',(-8.95359233126488,-73.6335280557816,
-213.274065021079));
#223833=CARTESIAN_POINT('Ctrl Pts',(-8.25459642710867,-71.4837698867061,
-216.57292704644));
#223834=CARTESIAN_POINT('Ctrl Pts',(-7.5540771905589,-69.3342366336724,
-219.871616502806));
#223835=CARTESIAN_POINT('Ctrl Pts',(-6.8502996103062,-67.185240788125,-223.169973551181));
#223836=CARTESIAN_POINT('Ctrl Pts',(-6.1465220300535,-65.0362449425776,
-226.468330599556));
#223837=CARTESIAN_POINT('Ctrl Pts',(-5.43981664545391,-62.8877051452245,
-229.766371465045));
#223838=CARTESIAN_POINT('Ctrl Pts',(-4.72482964674679,-60.740737267561,
-233.063701736715));
#223839=CARTESIAN_POINT('Ctrl Pts',(-8.1727428421796,-73.6762722001287,
-213.270659458216));
#223840=CARTESIAN_POINT('Ctrl Pts',(-7.52456725249791,-71.5269159170358,
-216.569288281039));
#223841=CARTESIAN_POINT('Ctrl Pts',(-6.87423822143353,-69.3778946347445,
-219.867709178756));
#223842=CARTESIAN_POINT('Ctrl Pts',(-6.21929751716124,-67.2296937045733,
-223.165751826413));
#223843=CARTESIAN_POINT('Ctrl Pts',(-5.56435681288895,-65.0814927744022,
-226.463794474069));
#223844=CARTESIAN_POINT('Ctrl Pts',(-4.90527248542591,-62.9339795937923,
-229.761465102056));
#223845=CARTESIAN_POINT('Ctrl Pts',(-4.23445772931318,-60.7889308444503,
-233.058419711927));
#223846=CARTESIAN_POINT('Ctrl Pts',(-7.39116334463378,-73.7391136679641,
-213.269118043698));
#223847=CARTESIAN_POINT('Ctrl Pts',(-6.79447747105095,-71.5904135964271,
-216.567708642569));
#223848=CARTESIAN_POINT('Ctrl Pts',(-6.19501537235948,-69.4421777820088,
-219.866101050477));
#223849=CARTESIAN_POINT('Ctrl Pts',(-5.5895961783157,-67.2951158690107,
-223.164183697639));
#223850=CARTESIAN_POINT('Ctrl Pts',(-4.98417698427192,-65.1480539560125,
-226.462266344801));
#223851=CARTESIAN_POINT('Ctrl Pts',(-4.37340476876875,-63.0019608814007,
-229.760014474659));
#223852=CARTESIAN_POINT('Ctrl Pts',(-3.74746533531928,-60.8595124428614,
-233.057401329873));
#223853=CARTESIAN_POINT('Ctrl Pts',(-6.60994240840707,-73.8222558927847,
-213.269427912899));
#223854=CARTESIAN_POINT('Ctrl Pts',(-6.06557267238966,-71.6743247983103,
-216.568167153263));
#223855=CARTESIAN_POINT('Ctrl Pts',(-5.51780600976748,-69.5270045782123,
-219.866761419183));
#223856=CARTESIAN_POINT('Ctrl Pts',(-4.96273068554881,-67.3812822930865,
-223.165228588343));
#223857=CARTESIAN_POINT('Ctrl Pts',(-4.40765536133015,-65.2355600079607,
-226.463695757503));
#223858=CARTESIAN_POINT('Ctrl Pts',(-3.84600674946129,-63.0911343879048,
-229.761957061969));
#223859=CARTESIAN_POINT('Ctrl Pts',(-3.2657468262204,-60.9518397874746,
-233.060586757597));
#223860=CARTESIAN_POINT('Ctrl Pts',(-6.21933194029372,-73.863827005195,
-213.2695828475));
#223861=CARTESIAN_POINT('Ctrl Pts',(-5.70112027305902,-71.7162803992519,
-216.568396408611));
#223862=CARTESIAN_POINT('Ctrl Pts',(-5.17920132847148,-69.569417976314,
-219.867091603535));
#223863=CARTESIAN_POINT('Ctrl Pts',(-4.64929793916537,-67.4243655051244,
-223.165751033694));
#223864=CARTESIAN_POINT('Ctrl Pts',(-4.11939454985925,-65.2793130339348,
-226.464410463854));
#223865=CARTESIAN_POINT('Ctrl Pts',(-3.58230773980756,-63.1357211411568,
-229.762928355624));
#223866=CARTESIAN_POINT('Ctrl Pts',(-3.02488757167096,-60.9980034597812,
-233.062179471459));
#223867=CARTESIAN_POINT('Ctrl Pts',(-5.82880537803933,-73.9104727623473,
-213.27020061172));
#223868=CARTESIAN_POINT('Ctrl Pts',(-5.33695524072191,-71.7633387196078,
-216.56913509822));
#223869=CARTESIAN_POINT('Ctrl Pts',(-4.84108747043389,-69.6169666428243,
-219.86798871271));
#223870=CARTESIAN_POINT('Ctrl Pts',(-4.33655677660738,-67.4726345985374,
-223.16692657622));
#223871=CARTESIAN_POINT('Ctrl Pts',(-3.83202608278088,-65.3283025542505,
-226.465864439729));
#223872=CARTESIAN_POINT('Ctrl Pts',(-3.31969806921586,-63.1856069990699,
-229.764747958359));
#223873=CARTESIAN_POINT('Ctrl Pts',(-2.78530983748405,-61.0496071561033,
-233.064823984859));
#223874=CARTESIAN_POINT('Ctrl Pts',(-5.43848674342394,-73.9622193313154,
-213.27128471988));
#223875=CARTESIAN_POINT('Ctrl Pts',(-4.97321480130516,-71.8155087180245,
-216.570386574246));
#223876=CARTESIAN_POINT('Ctrl Pts',(-4.50361309768486,-69.6696426023929,
-219.869456114948));
#223877=CARTESIAN_POINT('Ctrl Pts',(-4.02466312854686,-67.526066627963,
-223.168760046202));
#223878=CARTESIAN_POINT('Ctrl Pts',(-3.54571315940887,-65.3824906535331,
-226.468063977456));
#223879=CARTESIAN_POINT('Ctrl Pts',(-3.05834355347626,-63.2407400353646,
-229.767424405843));
#223880=CARTESIAN_POINT('Ctrl Pts',(-2.54717478765636,-61.1065960304884,
-233.06853892423));
#223881=CARTESIAN_POINT('Ctrl Pts',(-5.4262892860922,-73.9638364115957,
-213.27131859826));
#223882=CARTESIAN_POINT('Ctrl Pts',(-4.96184791257339,-71.817139030475,
-216.570425682871));
#223883=CARTESIAN_POINT('Ctrl Pts',(-4.49306702353645,-69.6712887261295,
-219.869501971269));
#223884=CARTESIAN_POINT('Ctrl Pts',(-4.01491645204497,-67.5277363788826,
-223.168817342139));
#223885=CARTESIAN_POINT('Ctrl Pts',(-3.53676588055349,-65.3841840316357,
-226.468132713009));
#223886=CARTESIAN_POINT('Ctrl Pts',(-3.0501762248594,-63.2424629427488,
-229.767508044828));
#223887=CARTESIAN_POINT('Ctrl Pts',(-2.53973306734924,-61.1083769328129,
-233.068655016085));
#223888=CARTESIAN_POINT('Ctrl Pts',(-5.41409203184723,-73.9654584732471,
-213.271352932467));
#223889=CARTESIAN_POINT('Ctrl Pts',(-4.95048143852496,-71.8187743349515,
-216.570465292767));
#223890=CARTESIAN_POINT('Ctrl Pts',(-4.48252157393744,-69.6729398572013,
-219.869548385134));
#223891=CARTESIAN_POINT('Ctrl Pts',(-4.00517060326625,-67.5294111720907,
-223.168875281415));
#223892=CARTESIAN_POINT('Ctrl Pts',(-3.52781963259506,-65.3858824869801,
-226.468202177696));
#223893=CARTESIAN_POINT('Ctrl Pts',(-3.04201012206819,-63.2441909750325,
-229.767592521906));
#223894=CARTESIAN_POINT('Ctrl Pts',(-2.53229275617624,-61.1101630954175,
-233.068772155269));
#223895=CARTESIAN_POINT('Ctrl Pts',(-5.40189498448029,-73.9670855170893,
-213.27138772269));
#223896=CARTESIAN_POINT('Ctrl Pts',(-4.93911538335592,-71.8204146317568,
-216.570505404131));
#223897=CARTESIAN_POINT('Ctrl Pts',(-4.47197675343487,-69.6745959954063,
-219.869595356765));
#223898=CARTESIAN_POINT('Ctrl Pts',(-3.99542558698367,-67.5310910069568,
-223.168933864337));
#223899=CARTESIAN_POINT('Ctrl Pts',(-3.51887442053248,-65.3875860185073,
-226.468272371909));
#223900=CARTESIAN_POINT('Ctrl Pts',(-3.03384525018033,-63.2459241307671,
-229.767677837598));
#223901=CARTESIAN_POINT('Ctrl Pts',(-2.52485385910942,-61.1119545168846,
-233.068890342738));
#223902=CARTESIAN_POINT('Ctrl Pts',(-5.38969793711334,-73.9687125609316,
-213.271422512912));
#223903=CARTESIAN_POINT('Ctrl Pts',(-4.92774932818688,-71.8220549285621,
-216.570545515496));
#223904=CARTESIAN_POINT('Ctrl Pts',(-4.4614319329323,-69.6762521336113,
-219.869642328397));
#223905=CARTESIAN_POINT('Ctrl Pts',(-3.9856805707011,-67.5327708418229,
-223.16899244726));
#223906=CARTESIAN_POINT('Ctrl Pts',(-3.5099292084699,-65.3892895500345,
-226.468342566123));
#223907=CARTESIAN_POINT('Ctrl Pts',(-3.02568037829247,-63.2476572865017,
-229.767763153291));
#223908=CARTESIAN_POINT('Ctrl Pts',(-2.51741496204259,-61.1137459383516,
-233.069008530206));
#223909=CARTESIAN_POINT('Ctrl Pts',(-5.37672637028157,-73.9704678685259,
-213.271433929509));
#223910=CARTESIAN_POINT('Ctrl Pts',(-4.9155433526131,-71.8238395746452,
-216.570564049875));
#223911=CARTESIAN_POINT('Ctrl Pts',(-4.44996909929499,-69.6780729754426,
-219.869670623327));
#223912=CARTESIAN_POINT('Ctrl Pts',(-3.97491462260742,-67.5346472458208,
-223.169039474058));
#223913=CARTESIAN_POINT('Ctrl Pts',(-3.49986014591986,-65.3912215161989,
-226.468408324789));
#223914=CARTESIAN_POINT('Ctrl Pts',(-3.01626470944041,-63.2496602746465,
-229.767854189359));
#223915=CARTESIAN_POINT('Ctrl Pts',(-2.50854660210467,-61.1158851609529,
-233.069159596983));
#223916=CARTESIAN_POINT('Ctrl Pts',(-5.36570279694763,-73.9719187759859,
-213.271505747073));
#223917=CARTESIAN_POINT('Ctrl Pts',(-4.90545050752033,-71.8252794240533,
-216.570638631499));
#223918=CARTESIAN_POINT('Ctrl Pts',(-4.44081643235981,-69.6794979085229,
-219.869747875903));
#223919=CARTESIAN_POINT('Ctrl Pts',(-3.96671825976106,-67.536047760413,
-223.169117864674));
#223920=CARTESIAN_POINT('Ctrl Pts',(-3.49262008716231,-65.3925976123031,
-226.468487853445));
#223921=CARTESIAN_POINT('Ctrl Pts',(-3.00999783445047,-63.2510034927325,
-229.767933853275));
#223922=CARTESIAN_POINT('Ctrl Pts',(-2.50327678459181,-61.1171690939225,
-233.069231764379));
#223923=CARTESIAN_POINT('Ctrl Pts',(-5.34365565027976,-73.9748205909058,
-213.271649382202));
#223924=CARTESIAN_POINT('Ctrl Pts',(-4.88526481733479,-71.8281591228697,
-216.570787794748));
#223925=CARTESIAN_POINT('Ctrl Pts',(-4.42251109848946,-69.6823477746836,
-219.869902381056));
#223926=CARTESIAN_POINT('Ctrl Pts',(-3.95032553406833,-67.5388487895975,
-223.169274645906));
#223927=CARTESIAN_POINT('Ctrl Pts',(-3.4781399696472,-65.3953498045114,
-226.468646910757));
#223928=CARTESIAN_POINT('Ctrl Pts',(-2.99746408447056,-63.2536899289045,
-229.768093181107));
#223929=CARTESIAN_POINT('Ctrl Pts',(-2.4927371495661,-61.1197369598615,
-233.069376099171));
#223930=CARTESIAN_POINT('Ctrl Pts',(-5.32159500200748,-73.9777056883786,
-213.271792108186));
#223931=CARTESIAN_POINT('Ctrl Pts',(-4.86506777599914,-71.8310217620559,
-216.570936017706));
#223932=CARTESIAN_POINT('Ctrl Pts',(-4.40419656758946,-69.6851802994998,
-219.870055928012));
#223933=CARTESIAN_POINT('Ctrl Pts',(-3.93392595850568,-67.5416322892271,
-223.16943049385));
#223934=CARTESIAN_POINT('Ctrl Pts',(-3.4636553494219,-65.3980842789543,
-226.468805059689));
#223935=CARTESIAN_POINT('Ctrl Pts',(-2.98492828270904,-63.2563585875261,
-229.76825167595));
#223936=CARTESIAN_POINT('Ctrl Pts',(-2.48219900959581,-61.1222869643936,
-233.069519750154));
#223937=CARTESIAN_POINT('Ctrl Pts',(-5.29952110564376,-73.9805739848368,
-213.271933926145));
#223938=CARTESIAN_POINT('Ctrl Pts',(-4.84485958837554,-71.833867280769,
-216.571083300788));
#223939=CARTESIAN_POINT('Ctrl Pts',(-4.38587299316779,-69.6879954448049,
-219.870208515872));
#223940=CARTESIAN_POINT('Ctrl Pts',(-3.91751962681961,-67.5443982464756,
-223.169585405614));
#223941=CARTESIAN_POINT('Ctrl Pts',(-3.44916626047143,-65.4008010481464,
-226.468962295357));
#223942=CARTESIAN_POINT('Ctrl Pts',(-2.97239039461706,-63.2590095074215,
-229.768409329534));
#223943=CARTESIAN_POINT('Ctrl Pts',(-2.47166224167208,-61.1248191908138,
-233.069662708859));
#223944=CARTESIAN_POINT('Ctrl Pts',(-5.25537331291633,-73.9863105777533,
-213.272217562064));
#223945=CARTESIAN_POINT('Ctrl Pts',(-4.80444321312832,-71.8395583181952,
-216.571377866951));
#223946=CARTESIAN_POINT('Ctrl Pts',(-4.34922584432445,-69.693625735415,
-219.870513691592));
#223947=CARTESIAN_POINT('Ctrl Pts',(-3.88470696344747,-67.5499301609728,
-223.169895229143));
#223948=CARTESIAN_POINT('Ctrl Pts',(-3.42018808257049,-65.4062345865307,
-226.469276766693));
#223949=CARTESIAN_POINT('Ctrl Pts',(-2.9473146184331,-63.2643113472122,
-229.768724636701));
#223950=CARTESIAN_POINT('Ctrl Pts',(-2.45058870582462,-61.1298836436543,
-233.069948626269));
#223951=CARTESIAN_POINT('Ctrl Pts',(-5.21117252788928,-73.9919799664689,
-213.272497565759));
#223952=CARTESIAN_POINT('Ctrl Pts',(-4.7639822528083,-71.8451808736014,
-216.57166867345));
#223953=CARTESIAN_POINT('Ctrl Pts',(-4.3125425214412,-69.699186507887,-219.870815030722));
#223954=CARTESIAN_POINT('Ctrl Pts',(-3.85186727558167,-67.5553919059884,
-223.170201307704));
#223955=CARTESIAN_POINT('Ctrl Pts',(-3.39119202972214,-65.4115973040898,
-226.469587584685));
#223956=CARTESIAN_POINT('Ctrl Pts',(-2.92223049669452,-63.2695422325334,
-229.769036578502));
#223957=CARTESIAN_POINT('Ctrl Pts',(-2.42952065843729,-61.1348769849848,
-233.070231774323));
#223958=CARTESIAN_POINT('Ctrl Pts',(-5.16692077781557,-73.9975814841632,
-213.272773947677));
#223959=CARTESIAN_POINT('Ctrl Pts',(-4.72347834531912,-71.8507344617868,
-216.57195572551));
#223960=CARTESIAN_POINT('Ctrl Pts',(-4.27582425199423,-69.7046774580107,
-219.871112528569));
#223961=CARTESIAN_POINT('Ctrl Pts',(-3.81900131317034,-67.5607833783998,
-223.170503621156));
#223962=CARTESIAN_POINT('Ctrl Pts',(-3.36217837434646,-65.4168892987889,
-226.469894713743));
#223963=CARTESIAN_POINT('Ctrl Pts',(-2.89713775575502,-63.2747024686849,
-229.769345092714));
#223964=CARTESIAN_POINT('Ctrl Pts',(-2.40845711188386,-61.1397998699931,
-233.070512088159));
#223965=CARTESIAN_POINT('Ctrl Pts',(-5.07841727766817,-74.0087845195517,
-213.273326711516));
#223966=CARTESIAN_POINT('Ctrl Pts',(-4.64247053034076,-71.8618416381575,
-216.572529829629));
#223967=CARTESIAN_POINT('Ctrl Pts',(-4.2023877131003,-69.715659358258,-219.871707524263));
#223968=CARTESIAN_POINT('Ctrl Pts',(-3.7532693883477,-67.5715663232226,
-223.171108248061));
#223969=CARTESIAN_POINT('Ctrl Pts',(-3.30415106359509,-65.4274732881873,
-226.470508971858));
#223970=CARTESIAN_POINT('Ctrl Pts',(-2.84695227387601,-63.285022940988,
-229.769962121139));
#223971=CARTESIAN_POINT('Ctrl Pts',(-2.366330018777,-61.1496456400098,-233.07107271583));
#223972=CARTESIAN_POINT('Ctrl Pts',(-4.98970991817215,-74.0197160685976,
-213.273864986293));
#223973=CARTESIAN_POINT('Ctrl Pts',(-4.56129092778213,-71.8726729436333,
-216.573088913503));
#223974=CARTESIAN_POINT('Ctrl Pts',(-4.12881138864584,-69.7263619676298,
-219.872287151588));
#223975=CARTESIAN_POINT('Ctrl Pts',(-3.68743236529496,-67.5820681782785,
-223.171697810615));
#223976=CARTESIAN_POINT('Ctrl Pts',(-3.24605334194409,-65.4377743889271,
-226.471108469642));
#223977=CARTESIAN_POINT('Ctrl Pts',(-2.79673231139314,-63.2950608232797,
-229.770565433851));
#223978=CARTESIAN_POINT('Ctrl Pts',(-2.32422093228867,-61.1592096000228,
-233.071622002575));
#223979=CARTESIAN_POINT('Ctrl Pts',(-4.90081490576138,-74.0303708240067,
-213.274388879266));
#223980=CARTESIAN_POINT('Ctrl Pts',(-4.47995262653692,-71.8832245209659,
-216.573633049045));
#223981=CARTESIAN_POINT('Ctrl Pts',(-4.05510508965952,-69.7367828703165,
-219.872851412303));
#223982=CARTESIAN_POINT('Ctrl Pts',(-3.62149624377294,-67.5922881106059,
-223.172272195036));
#223983=CARTESIAN_POINT('Ctrl Pts',(-3.18788739788636,-65.4477933508953,
-226.471692977771));
#223984=CARTESIAN_POINT('Ctrl Pts',(-2.74647572406062,-63.3048184758955,
-229.77115459683));
#223985=CARTESIAN_POINT('Ctrl Pts',(-2.28212190434125,-61.1684968100619,
-233.072159477025));
#223986=CARTESIAN_POINT('Ctrl Pts',(-4.72302488093985,-74.051680334825,
-213.275436665212));
#223987=CARTESIAN_POINT('Ctrl Pts',(-4.3172760240465,-71.904327675631,-216.574721320128));
#223988=CARTESIAN_POINT('Ctrl Pts',(-3.90769249168688,-69.7576246756899,
-219.873979933731));
#223989=CARTESIAN_POINT('Ctrl Pts',(-3.48962400072889,-67.6127279752608,
-223.17342096388));
#223990=CARTESIAN_POINT('Ctrl Pts',(-3.0715555097709,-65.4678312748317,
-226.472861994029));
#223991=CARTESIAN_POINT('Ctrl Pts',(-2.64596254939558,-63.3243337811273,
-229.772332922788));
#223992=CARTESIAN_POINT('Ctrl Pts',(-2.19792384844641,-61.18707123014,-233.073234425924));
#223993=CARTESIAN_POINT('Ctrl Pts',(-4.54448425091446,-74.071882635413,
-213.276426893072));
#223994=CARTESIAN_POINT('Ctrl Pts',(-4.15396463899018,-71.9243118863183,
-216.57574975929));
#223995=CARTESIAN_POINT('Ctrl Pts',(-3.75976000462968,-69.7773396309741,
-219.87504693894));
#223996=CARTESIAN_POINT('Ctrl Pts',(-3.35735536122353,-67.6320401585041,
-223.174508959174));
#223997=CARTESIAN_POINT('Ctrl Pts',(-2.95495071781737,-65.486740686034,
-226.47397097941));
#223998=CARTESIAN_POINT('Ctrl Pts',(-2.54530281321105,-63.3427282647259,
-229.773454562434));
#223999=CARTESIAN_POINT('Ctrl Pts',(-2.11376604236526,-61.2045389007808,
-233.074262056417));
#224000=CARTESIAN_POINT('Ctrl Pts',(-4.36532254289751,-74.090935698542,
-213.277360794546));
#224001=CARTESIAN_POINT('Ctrl Pts',(-3.99012300028631,-71.9431466770906,
-216.576719412775));
#224002=CARTESIAN_POINT('Ctrl Pts',(-3.61138599425699,-69.7959086923527,
-219.876053052738));
#224003=CARTESIAN_POINT('Ctrl Pts',(-3.22473834211198,-67.6502178766122,
-223.175536013948));
#224004=CARTESIAN_POINT('Ctrl Pts',(-2.83809068996697,-65.5045270608717,
-226.475018975158));
#224005=CARTESIAN_POINT('Ctrl Pts',(-2.44448009833563,-63.3600195797742,
-229.774517081184));
#224006=CARTESIAN_POINT('Ctrl Pts',(-2.02958446470485,-61.2209373357876,
-233.075239398162));
#224007=CARTESIAN_POINT('Ctrl Pts',(-3.64867571082973,-74.1671479510582,
-213.281096400445));
#224008=CARTESIAN_POINT('Ctrl Pts',(-3.33475644547083,-72.0184858401796,
-216.580598026715));
#224009=CARTESIAN_POINT('Ctrl Pts',(-3.01788995276623,-69.8701849378668,
-219.880077507931));
#224010=CARTESIAN_POINT('Ctrl Pts',(-2.69427026566578,-67.7229287490447,
-223.179644233041));
#224011=CARTESIAN_POINT('Ctrl Pts',(-2.37065057856533,-65.5756725602225,
-226.479210958151));
#224012=CARTESIAN_POINT('Ctrl Pts',(-2.04118923883392,-63.4291848399676,
-229.778767156183));
#224013=CARTESIAN_POINT('Ctrl Pts',(-1.69285815406323,-61.2865310758151,
-233.079148765145));
#224014=CARTESIAN_POINT('Ctrl Pts',(-2.92179171700349,-74.2248568155794,
-213.283931439761));
#224015=CARTESIAN_POINT('Ctrl Pts',(-2.67067383150201,-72.0753567042848,
-216.583539105332));
#224016=CARTESIAN_POINT('Ctrl Pts',(-2.4171737530214,-69.9260843575689,
-219.883132378737));
#224017=CARTESIAN_POINT('Ctrl Pts',(-2.15816590409808,-67.7774746840945,
-223.182780825433));
#224018=CARTESIAN_POINT('Ctrl Pts',(-1.89915805517477,-65.6288650106202,
-226.48242927213));
#224019=CARTESIAN_POINT('Ctrl Pts',(-1.6354272504708,-63.4807382255424,
-229.782069599427));
#224020=CARTESIAN_POINT('Ctrl Pts',(-1.35605364503039,-61.3350668114237,
-233.08223904777));
#224021=CARTESIAN_POINT('Ctrl Pts',(-2.19241710279808,-74.2625655408562,
-213.285868033891));
#224022=CARTESIAN_POINT('Ctrl Pts',(-2.00425439386506,-72.1126446956918,
-216.585548495067));
#224023=CARTESIAN_POINT('Ctrl Pts',(-1.81427677031869,-69.9628615488284,
-219.885219900497));
#224024=CARTESIAN_POINT('Ctrl Pts',(-1.62009069259905,-67.8134811173994,
-223.184924670423));
#224025=CARTESIAN_POINT('Ctrl Pts',(-1.4259046148794,-65.6641006859703,
-226.484629440349));
#224026=CARTESIAN_POINT('Ctrl Pts',(-1.22812047595596,-63.5150120219902,
-229.784328496798));
#224027=CARTESIAN_POINT('Ctrl Pts',(-1.01831914241026,-61.36742518831,-233.084352143351));
#224028=CARTESIAN_POINT('Ctrl Pts',(-1.46304248859267,-74.3002742661329,
-213.287804628021));
#224029=CARTESIAN_POINT('Ctrl Pts',(-1.3378349562281,-72.1499326870988,
-216.587557884803));
#224030=CARTESIAN_POINT('Ctrl Pts',(-1.21137978761598,-69.999638740088,
-219.887307422256));
#224031=CARTESIAN_POINT('Ctrl Pts',(-1.08201548110001,-67.8494875507042,
-223.187068515412));
#224032=CARTESIAN_POINT('Ctrl Pts',(-0.952651174584045,-65.6993363613204,
-226.486829608568));
#224033=CARTESIAN_POINT('Ctrl Pts',(-0.820813701441127,-63.5492858184379,
-229.786587394169));
#224034=CARTESIAN_POINT('Ctrl Pts',(-0.680584639790125,-61.3997835651962,
-233.086465238933));
#224035=CARTESIAN_POINT('Ctrl Pts',(-0.731897203934337,-74.3172201941713,
-213.288876053933));
#224036=CARTESIAN_POINT('Ctrl Pts',(-0.669711243166844,-72.1670055479396,
-216.588673926417));
#224037=CARTESIAN_POINT('Ctrl Pts',(-0.606834169240839,-70.016790901708,
-219.888471798901));
#224038=CARTESIAN_POINT('Ctrl Pts',(-0.542375109003111,-67.8665762554763,
-223.188269671383));
#224039=CARTESIAN_POINT('Ctrl Pts',(-0.477916048765383,-65.7163616092447,
-226.488067543867));
#224040=CARTESIAN_POINT('Ctrl Pts',(-0.412094305693277,-63.566146963013,
-229.787865416351));
#224041=CARTESIAN_POINT('Ctrl Pts',(-0.341829933578211,-61.4159323167813,
-233.087663288834));
#224042=CARTESIAN_POINT('Ctrl Pts',(-6.84354621607228E-13,-74.3172201941715,
-213.288876053933));
#224043=CARTESIAN_POINT('Ctrl Pts',(-1.42776780017916E-12,-72.1670055479398,
-216.588673926417));
#224044=CARTESIAN_POINT('Ctrl Pts',(-2.08399076963921E-12,-70.0167909017082,
-219.8884717989));
#224045=CARTESIAN_POINT('Ctrl Pts',(-2.80926784707921E-12,-67.8665762554765,
-223.188269671383));
#224046=CARTESIAN_POINT('Ctrl Pts',(-3.53454492451921E-12,-65.7163616092449,
-226.488067543867));
#224047=CARTESIAN_POINT('Ctrl Pts',(-4.11012448022973E-12,-63.5661469630132,
-229.787865416351));
#224048=CARTESIAN_POINT('Ctrl Pts',(-4.66308425881617E-12,-61.4159323167815,
-233.087663288834));
#224049=CARTESIAN_POINT('Ctrl Pts',(0.731897203932968,-74.3172201941717,
-213.288876053933));
#224050=CARTESIAN_POINT('Ctrl Pts',(0.669711243163988,-72.16700554794,-216.588673926417));
#224051=CARTESIAN_POINT('Ctrl Pts',(0.606834169236671,-70.0167909017083,
-219.8884717989));
#224052=CARTESIAN_POINT('Ctrl Pts',(0.542375108997492,-67.8665762554767,
-223.188269671383));
#224053=CARTESIAN_POINT('Ctrl Pts',(0.477916048758314,-65.716361609245,
-226.488067543867));
#224054=CARTESIAN_POINT('Ctrl Pts',(0.412094305685056,-63.5661469630133,
-229.787865416351));
#224055=CARTESIAN_POINT('Ctrl Pts',(0.341829933568885,-61.4159323167817,
-233.087663288834));
#224056=CARTESIAN_POINT('Ctrl Pts',(1.4630412071525,-74.3002743777528,-213.287804633297));
#224057=CARTESIAN_POINT('Ctrl Pts',(1.33783407544282,-72.1499327874783,
-216.587557889776));
#224058=CARTESIAN_POINT('Ctrl Pts',(1.2113792856225,-69.9996388304174,-219.887307427019));
#224059=CARTESIAN_POINT('Ctrl Pts',(1.08201528753655,-67.8494876362415,
-223.187068521293));
#224060=CARTESIAN_POINT('Ctrl Pts',(0.952651289450599,-65.6993364420655,
-226.486829615567));
#224061=CARTESIAN_POINT('Ctrl Pts',(0.820814077178737,-63.5492858967185,
-229.786587402353));
#224062=CARTESIAN_POINT('Ctrl Pts',(0.680584991670135,-61.3997836690735,
-233.086465258331));
#224063=CARTESIAN_POINT('Ctrl Pts',(2.19241535457815,-74.2625656556727,
-213.285868034929));
#224064=CARTESIAN_POINT('Ctrl Pts',(2.00425272002901,-72.1126448113594,
-216.585548496058));
#224065=CARTESIAN_POINT('Ctrl Pts',(1.81427515642486,-69.96286166618,-219.885219901252));
#224066=CARTESIAN_POINT('Ctrl Pts',(1.62008907510343,-67.813481242547,-223.184924671597));
#224067=CARTESIAN_POINT('Ctrl Pts',(1.425902993782,-65.6641008189139,-226.484629441941));
#224068=CARTESIAN_POINT('Ctrl Pts',(1.2281188155361,-63.5150121637255,-229.784328497621));
#224069=CARTESIAN_POINT('Ctrl Pts',(1.01831713572084,-61.3674253807579,
-233.084352154385));
#224070=CARTESIAN_POINT('Ctrl Pts',(2.92178950200379,-74.2248569335925,
-213.28393143656));
#224071=CARTESIAN_POINT('Ctrl Pts',(2.6706713646152,-72.0753568352406,-216.583539102341));
#224072=CARTESIAN_POINT('Ctrl Pts',(2.41717102722723,-69.9260845019427,
-219.883132375486));
#224073=CARTESIAN_POINT('Ctrl Pts',(2.15816286267031,-67.7774748488525,
-223.182780821899));
#224074=CARTESIAN_POINT('Ctrl Pts',(1.8991546981134,-65.6288651957623,-226.482429268314));
#224075=CARTESIAN_POINT('Ctrl Pts',(1.63542355389346,-63.4807384307325,
-229.782069592889));
#224076=CARTESIAN_POINT('Ctrl Pts',(1.35604927977155,-61.3350670924422,
-233.082239050439));
#224077=CARTESIAN_POINT('Ctrl Pts',(3.64867763480066,-74.1671476563362,
-213.281096434137));
#224078=CARTESIAN_POINT('Ctrl Pts',(3.33475783198323,-72.0184856638598,
-216.580598059648));
#224079=CARTESIAN_POINT('Ctrl Pts',(3.01789082047128,-69.8701848769235,
-219.880077539642));
#224080=CARTESIAN_POINT('Ctrl Pts',(2.6942706773542,-67.7229287903462,-223.179644260014));
#224081=CARTESIAN_POINT('Ctrl Pts',(2.37065053423712,-65.5756727037689,
-226.479210980387));
#224082=CARTESIAN_POINT('Ctrl Pts',(2.04118878099155,-63.4291850796541,
-229.778767173092));
#224083=CARTESIAN_POINT('Ctrl Pts',(1.69285753982065,-61.2865313428857,
-233.079148752624));
#224084=CARTESIAN_POINT('Ctrl Pts',(4.36532376578682,-74.0909355242495,
-213.27736081295));
#224085=CARTESIAN_POINT('Ctrl Pts',(3.99012383085994,-71.9431465837745,
-216.576719427696));
#224086=CARTESIAN_POINT('Ctrl Pts',(3.61138642781057,-69.7959086820964,
-219.876053064671));
#224087=CARTESIAN_POINT('Ctrl Pts',(3.2247384017838,-67.6502179485229,-223.175536024031));
#224088=CARTESIAN_POINT('Ctrl Pts',(2.83809037575702,-65.5045272149494,
-226.47501898339));
#224089=CARTESIAN_POINT('Ctrl Pts',(2.44447941230847,-63.3600198215615,
-229.774517090706));
#224090=CARTESIAN_POINT('Ctrl Pts',(2.02958360100885,-61.2209376265333,
-233.07523940264));
#224091=CARTESIAN_POINT('Ctrl Pts',(4.54448529853335,-74.0718824912277,
-213.276426907653));
#224092=CARTESIAN_POINT('Ctrl Pts',(4.15396533057911,-71.9243118137532,
-216.575749769707));
#224093=CARTESIAN_POINT('Ctrl Pts',(3.75976032964539,-69.7773396333896,
-219.875046945928));
#224094=CARTESIAN_POINT('Ctrl Pts',(3.35735533289119,-67.632040238067,-223.174508965034));
#224095=CARTESIAN_POINT('Ctrl Pts',(2.95495033613699,-65.4867408427445,
-226.47397098414));
#224096=CARTESIAN_POINT('Ctrl Pts',(2.5453020701377,-63.3427285070384,-229.773454570109));
#224097=CARTESIAN_POINT('Ctrl Pts',(2.1137651163059,-61.2045391974451,-233.074262065144));
#224098=CARTESIAN_POINT('Ctrl Pts',(4.72302558275178,-74.0516802394771,
-213.275436674357));
#224099=CARTESIAN_POINT('Ctrl Pts',(4.31727644647028,-71.9043276347028,
-216.574721325169));
#224100=CARTESIAN_POINT('Ctrl Pts',(3.90769262251043,-69.7576246931073,
-219.873979935587));
#224101=CARTESIAN_POINT('Ctrl Pts',(3.48962384895622,-67.6127280546252,
-223.173420965523));
#224102=CARTESIAN_POINT('Ctrl Pts',(3.07155507540201,-65.4678314161431,
-226.472861995458));
#224103=CARTESIAN_POINT('Ctrl Pts',(2.64596182151007,-63.3243339939848,
-229.77233292858));
#224104=CARTESIAN_POINT('Ctrl Pts',(2.19792298970101,-61.1870714878141,
-233.073234436702));
#224105=CARTESIAN_POINT('Ctrl Pts',(4.90081532807169,-74.0303707671596,
-213.27438888447));
#224106=CARTESIAN_POINT('Ctrl Pts',(4.47995285021341,-71.8832245017814,
-216.573633050881));
#224107=CARTESIAN_POINT('Ctrl Pts',(4.05510510402121,-69.7367828923109,
-219.87285141164));
#224108=CARTESIAN_POINT('Ctrl Pts',(3.62149605519719,-67.5922881772786,
-223.172272194658));
#224109=CARTESIAN_POINT('Ctrl Pts',(3.18788700637317,-65.4477934622463,
-226.471692977676));
#224110=CARTESIAN_POINT('Ctrl Pts',(2.7464751198719,-63.3048186403858,-229.771154601106));
#224111=CARTESIAN_POINT('Ctrl Pts',(2.28212121845882,-61.1684970065069,
-233.072159487081));
#224112=CARTESIAN_POINT('Ctrl Pts',(4.98971020073165,-74.0197160310009,
-213.273864989526));
#224113=CARTESIAN_POINT('Ctrl Pts',(4.56129105208498,-71.8726729353207,
-216.573088913737));
#224114=CARTESIAN_POINT('Ctrl Pts',(4.1288113447766,-69.7263619919127,-219.872287149666));
#224115=CARTESIAN_POINT('Ctrl Pts',(3.68743215831767,-67.5820682386053,
-223.171697809226));
#224116=CARTESIAN_POINT('Ctrl Pts',(3.24605297185875,-65.4377744852979,
-226.471108468786));
#224117=CARTESIAN_POINT('Ctrl Pts',(2.79673176905281,-63.2950609635863,
-229.770565437369));
#224118=CARTESIAN_POINT('Ctrl Pts',(2.32422033283773,-61.1592097658532,
-233.071622012271));
#224119=CARTESIAN_POINT('Ctrl Pts',(5.07841743705022,-74.0087844985998,
-213.273326713143));
#224120=CARTESIAN_POINT('Ctrl Pts',(4.64247057287694,-71.8618416382213,
-216.572529828792));
#224121=CARTESIAN_POINT('Ctrl Pts',(4.20238763043668,-69.7156593822006,
-219.871707521718));
#224122=CARTESIAN_POINT('Ctrl Pts',(3.7532691846266,-67.5715663740637,-223.171108246189));
#224123=CARTESIAN_POINT('Ctrl Pts',(3.30415073881651,-65.4274733659267,
-226.47050897066));
#224124=CARTESIAN_POINT('Ctrl Pts',(2.84695182048441,-63.2850230523818,
-229.76996212396));
#224125=CARTESIAN_POINT('Ctrl Pts',(2.3663295321107,-61.149645769708,-233.071072724443));
#224126=CARTESIAN_POINT('Ctrl Pts',(5.1669208602018,-73.9975814734869,-213.272773948399));
#224127=CARTESIAN_POINT('Ctrl Pts',(4.72347834880175,-71.8507344649978,
-216.571955724444));
#224128=CARTESIAN_POINT('Ctrl Pts',(4.27582417043258,-69.704677477251,-219.871112526297));
#224129=CARTESIAN_POINT('Ctrl Pts',(3.81900114961728,-67.5607834159342,
-223.170503619482));
#224130=CARTESIAN_POINT('Ctrl Pts',(3.36217812880197,-65.4168893546174,
-226.469894712669));
#224131=CARTESIAN_POINT('Ctrl Pts',(2.89713742276365,-63.2747025478298,
-229.769345094758));
#224132=CARTESIAN_POINT('Ctrl Pts',(2.40845676115674,-61.1397999611404,
-233.070512094721));
#224133=CARTESIAN_POINT('Ctrl Pts',(5.21117257177759,-73.9919799609304,
-213.272497566026));
#224134=CARTESIAN_POINT('Ctrl Pts',(4.76398223676415,-71.8451808783859,
-216.571668672269));
#224135=CARTESIAN_POINT('Ctrl Pts',(4.31254244043052,-69.6991865247762,
-219.870815028586));
#224136=CARTESIAN_POINT('Ctrl Pts',(3.85186713211261,-67.5553919368695,
-223.17020130613));
#224137=CARTESIAN_POINT('Ctrl Pts',(3.3911918237947,-65.4115973489628,-226.469587583673));
#224138=CARTESIAN_POINT('Ctrl Pts',(2.92223022390326,-63.2695422955538,
-229.769036580157));
#224139=CARTESIAN_POINT('Ctrl Pts',(2.42952037567976,-61.1348770568567,
-233.070231779859));
#224140=CARTESIAN_POINT('Ctrl Pts',(5.25537332985224,-73.9863105757591,
-213.272217562053));
#224141=CARTESIAN_POINT('Ctrl Pts',(4.804443188236,-71.8395583232445,-216.571377865865));
#224142=CARTESIAN_POINT('Ctrl Pts',(4.34922577383909,-69.693625748861,-219.870513689814));
#224143=CARTESIAN_POINT('Ctrl Pts',(3.8847068492901,-67.5499301842444,-223.169895227836));
#224144=CARTESIAN_POINT('Ctrl Pts',(3.42018792474111,-65.4062346196278,
-226.469276765858));
#224145=CARTESIAN_POINT('Ctrl Pts',(2.94731441370204,-63.2643113932744,
-229.768724637945));
#224146=CARTESIAN_POINT('Ctrl Pts',(2.45058849682277,-61.1298836956491,
-233.069948630535));
#224147=CARTESIAN_POINT('Ctrl Pts',(5.29952111087686,-73.9805739843142,
-213.271933926068));
#224148=CARTESIAN_POINT('Ctrl Pts',(4.8448595684564,-71.8338672844239,-216.571083300041));
#224149=CARTESIAN_POINT('Ctrl Pts',(4.38587294574325,-69.6879954534902,
-219.870208514701));
#224150=CARTESIAN_POINT('Ctrl Pts',(3.91751955310888,-67.5443982610901,
-223.169585404755));
#224151=CARTESIAN_POINT('Ctrl Pts',(3.44916616047452,-65.4008010686901,
-226.46896229481));
#224152=CARTESIAN_POINT('Ctrl Pts',(2.97239026633894,-63.2590095358678,
-229.768409330315));
#224153=CARTESIAN_POINT('Ctrl Pts',(2.47166211180462,-61.1248192227346,
-233.069662711569));
#224154=CARTESIAN_POINT('Ctrl Pts',(5.32159500138917,-73.9777056885918,
-213.271792108075));
#224155=CARTESIAN_POINT('Ctrl Pts',(4.8650677585666,-71.8310217650135,-216.570936017129));
#224156=CARTESIAN_POINT('Ctrl Pts',(4.40419653169533,-69.6851803058048,
-219.870055927144));
#224157=CARTESIAN_POINT('Ctrl Pts',(3.93392590501828,-67.541632299513,-223.169430493215));
#224158=CARTESIAN_POINT('Ctrl Pts',(3.46365527834122,-65.3980842932212,
-226.468805059286));
#224159=CARTESIAN_POINT('Ctrl Pts',(2.98492819265739,-63.2563586071644,
-229.7682516765));
#224160=CARTESIAN_POINT('Ctrl Pts',(2.48219891929555,-61.1222869862773,
-233.069519752087));
#224161=CARTESIAN_POINT('Ctrl Pts',(5.34365564762243,-73.9748205913366,
-213.271649382111));
#224162=CARTESIAN_POINT('Ctrl Pts',(4.8852648058442,-71.8281591247152,-216.570787794402));
#224163=CARTESIAN_POINT('Ctrl Pts',(4.42251107725984,-69.6823477782787,
-219.869902380553));
#224164=CARTESIAN_POINT('Ctrl Pts',(3.95032550358819,-67.5388487952928,
-223.169274645539));
#224165=CARTESIAN_POINT('Ctrl Pts',(3.47813992991653,-65.395349812307,-226.468646910525));
#224166=CARTESIAN_POINT('Ctrl Pts',(2.99746403474337,-63.2536899395703,
-229.768093181413));
#224167=CARTESIAN_POINT('Ctrl Pts',(2.49273710017753,-61.119736971659,-233.069376100254));
#224168=CARTESIAN_POINT('Ctrl Pts',(5.36570279652679,-73.9719187760556,
-213.27150574706));
#224169=CARTESIAN_POINT('Ctrl Pts',(4.90545050582003,-71.8252794243274,
-216.570638631449));
#224170=CARTESIAN_POINT('Ctrl Pts',(4.44081642924868,-69.6794979090499,
-219.86974787583));
#224171=CARTESIAN_POINT('Ctrl Pts',(3.96671825530998,-67.5360477612441,
-223.16911786462));
#224172=CARTESIAN_POINT('Ctrl Pts',(3.49262008137128,-65.3925976134382,
-226.468487853411));
#224173=CARTESIAN_POINT('Ctrl Pts',(3.00999782721103,-63.2510034942836,
-229.76793385332));
#224174=CARTESIAN_POINT('Ctrl Pts',(2.50327677740755,-61.1171690956365,
-233.069231764537));
#224175=CARTESIAN_POINT('Ctrl Pts',(5.37672637097897,-73.9704678684151,
-213.271433929534));
#224176=CARTESIAN_POINT('Ctrl Pts',(4.91554335580794,-71.8238395741335,
-216.570564049972));
#224177=CARTESIAN_POINT('Ctrl Pts',(4.44996910524309,-69.6780729744356,
-219.869670623468));
#224178=CARTESIAN_POINT('Ctrl Pts',(3.97491463117087,-67.5346472442197,
-223.169039474161));
#224179=CARTESIAN_POINT('Ctrl Pts',(3.49986015709865,-65.3912215140038,
-226.468408324854));
#224180=CARTESIAN_POINT('Ctrl Pts',(3.01626472344486,-63.2496602716403,
-229.767854189273));
#224181=CARTESIAN_POINT('Ctrl Pts',(2.50854661602256,-61.1158851576253,
-233.069159596678));
#224182=CARTESIAN_POINT('Ctrl Pts',(5.38969793711063,-73.9687125609349,
-213.271422512912));
#224183=CARTESIAN_POINT('Ctrl Pts',(4.92774932818247,-71.8220549285655,
-216.570545515496));
#224184=CARTESIAN_POINT('Ctrl Pts',(4.46143193292641,-69.6762521336146,
-219.869642328397));
#224185=CARTESIAN_POINT('Ctrl Pts',(3.98568057069344,-67.5327708418263,
-223.16899244726));
#224186=CARTESIAN_POINT('Ctrl Pts',(3.50992920846046,-65.389289550038,-226.468342566122));
#224187=CARTESIAN_POINT('Ctrl Pts',(3.02568037828113,-63.2476572865054,
-229.767763153291));
#224188=CARTESIAN_POINT('Ctrl Pts',(2.51741496202948,-61.1137459383554,
-233.069008530206));
#224189=CARTESIAN_POINT('Ctrl Pts',(5.40189498447758,-73.9670855170926,
-213.27138772269));
#224190=CARTESIAN_POINT('Ctrl Pts',(4.93911538335151,-71.8204146317601,
-216.570505404131));
#224191=CARTESIAN_POINT('Ctrl Pts',(4.47197675342897,-69.6745959954096,
-219.869595356765));
#224192=CARTESIAN_POINT('Ctrl Pts',(3.995425586976,-67.5310910069602,-223.168933864337));
#224193=CARTESIAN_POINT('Ctrl Pts',(3.51887442052304,-65.3875860185108,
-226.468272371909));
#224194=CARTESIAN_POINT('Ctrl Pts',(3.03384525016898,-63.2459241307708,
-229.767677837598));
#224195=CARTESIAN_POINT('Ctrl Pts',(2.5248538590963,-61.1119545168883,-233.068890342738));
#224196=CARTESIAN_POINT('Ctrl Pts',(5.41409203184453,-73.9654584732504,
-213.271352932467));
#224197=CARTESIAN_POINT('Ctrl Pts',(4.95048143852055,-71.8187743349548,
-216.570465292767));
#224198=CARTESIAN_POINT('Ctrl Pts',(4.48252157393154,-69.6729398572046,
-219.869548385134));
#224199=CARTESIAN_POINT('Ctrl Pts',(4.00517060325858,-67.5294111720941,
-223.168875281415));
#224200=CARTESIAN_POINT('Ctrl Pts',(3.52781963258561,-65.3858824869837,
-226.468202177696));
#224201=CARTESIAN_POINT('Ctrl Pts',(3.04201012205683,-63.2441909750361,
-229.767592521906));
#224202=CARTESIAN_POINT('Ctrl Pts',(2.53229275616311,-61.1101630954213,
-233.068772155269));
#224203=CARTESIAN_POINT('Ctrl Pts',(5.42628928608951,-73.963836411599,-213.27131859826));
#224204=CARTESIAN_POINT('Ctrl Pts',(4.96184791256897,-71.8171390304783,
-216.570425682871));
#224205=CARTESIAN_POINT('Ctrl Pts',(4.49306702353044,-69.6712887261328,
-219.869501971269));
#224206=CARTESIAN_POINT('Ctrl Pts',(4.01491645203717,-67.527736378886,-223.168817342139));
#224207=CARTESIAN_POINT('Ctrl Pts',(3.5367658805439,-65.3841840316392,-226.468132713009));
#224208=CARTESIAN_POINT('Ctrl Pts',(3.05017622484798,-63.2424629427525,
-229.767508044828));
#224209=CARTESIAN_POINT('Ctrl Pts',(2.53973306733594,-61.1083769328167,
-233.068655016085));
#224210=CARTESIAN_POINT('Ctrl Pts',(5.43848674342124,-73.9622193313187,
-213.27128471988));
#224211=CARTESIAN_POINT('Ctrl Pts',(4.97321480130074,-71.8155087180278,
-216.570386574246));
#224212=CARTESIAN_POINT('Ctrl Pts',(4.50361309767885,-69.6696426023963,
-219.869456114948));
#224213=CARTESIAN_POINT('Ctrl Pts',(4.02466312853905,-67.5260666279664,
-223.168760046202));
#224214=CARTESIAN_POINT('Ctrl Pts',(3.54571315939927,-65.3824906535366,
-226.468063977456));
#224215=CARTESIAN_POINT('Ctrl Pts',(3.05834355346484,-63.2407400353682,
-229.767424405843));
#224216=CARTESIAN_POINT('Ctrl Pts',(2.54717478764305,-61.1065960304922,
-233.06853892423));
#224217=CARTESIAN_POINT('Ctrl Pts',(5.82880537803666,-73.9104727623503,
-213.27020061172));
#224218=CARTESIAN_POINT('Ctrl Pts',(5.33695524071748,-71.7633387196109,
-216.56913509822));
#224219=CARTESIAN_POINT('Ctrl Pts',(4.84108747042776,-69.6169666428275,
-219.86798871271));
#224220=CARTESIAN_POINT('Ctrl Pts',(4.33655677659942,-67.4726345985407,
-223.16692657622));
#224221=CARTESIAN_POINT('Ctrl Pts',(3.83202608277108,-65.3283025542538,
-226.465864439729));
#224222=CARTESIAN_POINT('Ctrl Pts',(3.31969806920419,-63.1856069990734,
-229.764747958359));
#224223=CARTESIAN_POINT('Ctrl Pts',(2.78530983747041,-61.049607156107,-233.064823984859));
#224224=CARTESIAN_POINT('Ctrl Pts',(6.2193319402912,-73.8638270051978,-213.2695828475));
#224225=CARTESIAN_POINT('Ctrl Pts',(5.70112027305471,-71.7162803992548,
-216.56839640861));
#224226=CARTESIAN_POINT('Ctrl Pts',(5.17920132846573,-69.5694179763168,
-219.867091603535));
#224227=CARTESIAN_POINT('Ctrl Pts',(4.64929793915769,-67.4243655051274,
-223.165751033694));
#224228=CARTESIAN_POINT('Ctrl Pts',(4.11939454984966,-65.2793130339379,
-226.464410463854));
#224229=CARTESIAN_POINT('Ctrl Pts',(3.58230773979595,-63.13572114116,-229.762928355624));
#224230=CARTESIAN_POINT('Ctrl Pts',(3.02488757165734,-60.9980034597846,
-233.062179471459));
#224231=CARTESIAN_POINT('Ctrl Pts',(6.60994240840454,-73.8222558927873,
-213.269427912899));
#224232=CARTESIAN_POINT('Ctrl Pts',(6.06557267238532,-71.6743247983129,
-216.568167153263));
#224233=CARTESIAN_POINT('Ctrl Pts',(5.51780600976152,-69.5270045782149,
-219.866761419183));
#224234=CARTESIAN_POINT('Ctrl Pts',(4.96273068554095,-67.3812822930893,
-223.165228588343));
#224235=CARTESIAN_POINT('Ctrl Pts',(4.40765536132037,-65.2355600079636,
-226.463695757503));
#224236=CARTESIAN_POINT('Ctrl Pts',(3.84600674944955,-63.0911343879077,
-229.761957061969));
#224237=CARTESIAN_POINT('Ctrl Pts',(3.26574682620663,-60.9518397874778,
-233.060586757597));
#224238=CARTESIAN_POINT('Ctrl Pts',(7.39116334463119,-73.7391136679663,
-213.269118043698));
#224239=CARTESIAN_POINT('Ctrl Pts',(6.79447747104655,-71.5904135964293,
-216.567708642569));
#224240=CARTESIAN_POINT('Ctrl Pts',(6.19501537235311,-69.4421777820111,
-219.866101050477));
#224241=CARTESIAN_POINT('Ctrl Pts',(5.58959617830746,-67.2951158690131,
-223.164183697639));
#224242=CARTESIAN_POINT('Ctrl Pts',(4.9841769842618,-65.148053956015,-226.462266344801));
#224243=CARTESIAN_POINT('Ctrl Pts',(4.37340476875675,-63.0019608814033,
-229.760014474658));
#224244=CARTESIAN_POINT('Ctrl Pts',(3.7474653353052,-60.8595124428641,-233.057401329873));
#224245=CARTESIAN_POINT('Ctrl Pts',(8.17274284217698,-73.6762722001305,
-213.270659458216));
#224246=CARTESIAN_POINT('Ctrl Pts',(7.52456725249353,-71.5269159170376,
-216.569288281038));
#224247=CARTESIAN_POINT('Ctrl Pts',(6.87423822142749,-69.3778946347463,
-219.867709178756));
#224248=CARTESIAN_POINT('Ctrl Pts',(6.2192975171534,-67.2296937045752,-223.165751826412));
#224249=CARTESIAN_POINT('Ctrl Pts',(5.56435681287931,-65.0814927744041,
-226.463794474068));
#224250=CARTESIAN_POINT('Ctrl Pts',(4.90527248541439,-62.9339795937943,
-229.761465102056));
#224251=CARTESIAN_POINT('Ctrl Pts',(4.23445772929978,-60.7889308444523,
-233.058419711927));
#224252=CARTESIAN_POINT('Ctrl Pts',(8.95359233126237,-73.6335280557829,
-213.274065021078));
#224253=CARTESIAN_POINT('Ctrl Pts',(8.25459642710441,-71.4837698867074,
-216.572927046439));
#224254=CARTESIAN_POINT('Ctrl Pts',(7.55407719055292,-69.3342366336737,
-219.871616502806));
#224255=CARTESIAN_POINT('Ctrl Pts',(6.85029961029843,-67.1852407881264,
-223.16997355118));
#224256=CARTESIAN_POINT('Ctrl Pts',(6.14652203004394,-65.036244942579,-226.468330599556));
#224257=CARTESIAN_POINT('Ctrl Pts',(5.43981664544253,-62.8877051452259,
-229.766371465045));
#224258=CARTESIAN_POINT('Ctrl Pts',(4.72482964673358,-60.7407372675625,
-233.063701736715));
#224259=CARTESIAN_POINT('Ctrl Pts',(10.5152913094331,-73.5480397670876,
-213.280876146803));
#224260=CARTESIAN_POINT('Ctrl Pts',(9.71465477632616,-71.397477826047,-216.58020457724));
#224261=CARTESIAN_POINT('Ctrl Pts',(8.91375512880376,-69.2469206315284,
-219.879431150906));
#224262=CARTESIAN_POINT('Ctrl Pts',(8.11230379658849,-67.0963349552287,
-223.178417000718));
#224263=CARTESIAN_POINT('Ctrl Pts',(7.31085246437322,-64.945749278929,-226.47740285053));
#224264=CARTESIAN_POINT('Ctrl Pts',(6.50890496549881,-62.7951562480893,
-229.776184191023));
#224265=CARTESIAN_POINT('Ctrl Pts',(5.70557348160117,-60.6443501137831,
-233.074265786289));
#224266=CARTESIAN_POINT('Ctrl Pts',(12.0741192309778,-73.5429416649928,
-213.295088118557));
#224267=CARTESIAN_POINT('Ctrl Pts',(11.174560655384,-71.3925980352056,-216.595652144222));
#224268=CARTESIAN_POINT('Ctrl Pts',(10.276034499693,-69.2421106607767,-219.89636066281));
#224269=CARTESIAN_POINT('Ctrl Pts',(9.37971367536872,-67.0912902652196,
-223.197362281445));
#224270=CARTESIAN_POINT('Ctrl Pts',(8.48339285104444,-64.9404698696625,
-226.498363900081));
#224271=CARTESIAN_POINT('Ctrl Pts',(7.58904411056311,-62.7893619838303,
-229.799632644879));
#224272=CARTESIAN_POINT('Ctrl Pts',(6.70034092093902,-60.637315061886,-233.101605220138));
#224273=CARTESIAN_POINT('Ctrl Pts',(13.6221605046809,-73.6159852550006,
-213.31749452838));
#224274=CARTESIAN_POINT('Ctrl Pts',(12.62507600816,-71.4677688674561,-216.620281085237));
#224275=CARTESIAN_POINT('Ctrl Pts',(11.6304405856027,-69.3193741723348,
-219.923700795081));
#224276=CARTESIAN_POINT('Ctrl Pts',(10.6409978873149,-67.1707515656024,
-223.228560662601));
#224277=CARTESIAN_POINT('Ctrl Pts',(9.65155518902709,-65.0221289588701,
-226.533420530121));
#224278=CARTESIAN_POINT('Ctrl Pts',(8.66680721405871,-62.8732305917473,
-229.839537084504));
#224279=CARTESIAN_POINT('Ctrl Pts',(7.69505740664371,-60.7243047821012,
-233.149611908545));
#224280=CARTESIAN_POINT('Ctrl Pts',(14.3961811415325,-73.6525070500044,
-213.32869773329));
#224281=CARTESIAN_POINT('Ctrl Pts',(13.3503336845479,-71.5053542835814,
-216.632595555744));
#224282=CARTESIAN_POINT('Ctrl Pts',(12.3076436285575,-69.3580059281139,
-219.937370861218));
#224283=CARTESIAN_POINT('Ctrl Pts',(11.271639993288,-67.2104822157939,-223.244159853179));
#224284=CARTESIAN_POINT('Ctrl Pts',(10.2356363580184,-65.0629585034738,
-226.550948845141));
#224285=CARTESIAN_POINT('Ctrl Pts',(9.20568876580652,-62.9151648957058,
-229.859489304316));
#224286=CARTESIAN_POINT('Ctrl Pts',(8.19241564949605,-60.7677996422088,
-233.173615252749));
#224287=CARTESIAN_POINT('Ctrl Pts',(15.1674713187882,-73.7085567757101,
-213.341951507641));
#224288=CARTESIAN_POINT('Ctrl Pts',(14.0731825300145,-71.562941120452,-216.647204118779));
#224289=CARTESIAN_POINT('Ctrl Pts',(12.9827854653705,-69.4171418966908,
-219.953638842029));
#224290=CARTESIAN_POINT('Ctrl Pts',(11.9006166435758,-67.2713253491906,
-223.262814446454));
#224291=CARTESIAN_POINT('Ctrl Pts',(10.818447821781,-65.1255088016904,-226.571990050878));
#224292=CARTESIAN_POINT('Ctrl Pts',(9.74375195730441,-62.9795030354078,
-229.883541373779));
#224293=CARTESIAN_POINT('Ctrl Pts',(8.68946082743354,-60.8348048519155,
-233.202772070184));
#224294=CARTESIAN_POINT('Ctrl Pts',(15.9351468463176,-73.7837993408375,
-213.357451906234));
#224295=CARTESIAN_POINT('Ctrl Pts',(14.7925760080712,-71.6402731942657,
-216.664356393474));
#224296=CARTESIAN_POINT('Ctrl Pts',(13.6546740285671,-69.4966163530812,
-219.972825698813));
#224297=CARTESIAN_POINT('Ctrl Pts',(12.5266115102098,-67.3532549610597,
-223.284963342766));
#224298=CARTESIAN_POINT('Ctrl Pts',(11.3985489918526,-65.2098935690382,
-226.597100986718));
#224299=CARTESIAN_POINT('Ctrl Pts',(10.2794730121625,-63.0665351244741,
-229.912415755274));
#224300=CARTESIAN_POINT('Ctrl Pts',(9.1845149202515,-60.9259885966297,-233.238077193558));
#224301=CARTESIAN_POINT('Ctrl Pts',(15.9831265667882,-73.788502001158,-213.358420681146));
#224302=CARTESIAN_POINT('Ctrl Pts',(14.8375381004497,-71.645106448879,-216.665428410643));
#224303=CARTESIAN_POINT('Ctrl Pts',(13.6966670637669,-69.5015835066056,
-219.974024877362));
#224304=CARTESIAN_POINT('Ctrl Pts',(12.5657361893745,-67.3583755618015,
-223.286347648785));
#224305=CARTESIAN_POINT('Ctrl Pts',(11.434805314982,-65.2151676169974,-226.598670420208));
#224306=CARTESIAN_POINT('Ctrl Pts',(10.3129555780911,-63.0719746300408,
-229.914220404117));
#224307=CARTESIAN_POINT('Ctrl Pts',(9.21545580105263,-60.9316875806744,
-233.240283763769));
#224308=CARTESIAN_POINT('Ctrl Pts',(16.0310921652337,-73.7932796461828,
-213.359398260476));
#224309=CARTESIAN_POINT('Ctrl Pts',(14.8824866922713,-71.6500168515611,
-216.666510400031));
#224310=CARTESIAN_POINT('Ctrl Pts',(13.7386473871037,-69.5066301336811,
-219.975235503695));
#224311=CARTESIAN_POINT('Ctrl Pts',(12.6048492100916,-67.3635785769872,
-223.287745666655));
#224312=CARTESIAN_POINT('Ctrl Pts',(11.4710510330794,-65.2205270202932,
-226.600255829615));
#224313=CARTESIAN_POINT('Ctrl Pts',(10.3464289705351,-63.077502877188,-229.916043994162));
#224314=CARTESIAN_POINT('Ctrl Pts',(9.24638881753499,-60.9374811728283,
-233.242514480938));
#224315=CARTESIAN_POINT('Ctrl Pts',(16.0790434247669,-73.7981321994158,
-213.360384703604));
#224316=CARTESIAN_POINT('Ctrl Pts',(14.9274215266693,-71.6550043474046,
-216.66760243706));
#224317=CARTESIAN_POINT('Ctrl Pts',(13.7806147058241,-69.5117562048766,
-219.976457674748));
#224318=CARTESIAN_POINT('Ctrl Pts',(12.6439502460863,-67.3688640192575,
-223.28915752863));
#224319=CARTESIAN_POINT('Ctrl Pts',(11.5072857863485,-65.2259718336384,
-226.60185738251));
#224320=CARTESIAN_POINT('Ctrl Pts',(10.3798928063555,-63.0831199759298,
-229.917886743821));
#224321=CARTESIAN_POINT('Ctrl Pts',(9.27731352150188,-60.9433696029714,
-233.244769639115));
#224322=CARTESIAN_POINT('Ctrl Pts',(16.1030190545335,-73.8005584760323,
-213.360877925168));
#224323=CARTESIAN_POINT('Ctrl Pts',(14.9498889438683,-71.6574980953263,
-216.668148455574));
#224324=CARTESIAN_POINT('Ctrl Pts',(13.8015983651843,-69.5143192404743,
-219.977068760275));
#224325=CARTESIAN_POINT('Ctrl Pts',(12.6635007640837,-67.3715067403927,
-223.289863459617));
#224326=CARTESIAN_POINT('Ctrl Pts',(11.5254031629831,-65.228694240311,-226.602658158959));
#224327=CARTESIAN_POINT('Ctrl Pts',(10.3966247242656,-63.0859285253007,
-229.918808118651));
#224328=CARTESIAN_POINT('Ctrl Pts',(9.29277587348532,-60.9463138180429,
-233.245897218204));
#224329=CARTESIAN_POINT('Ctrl Pts',(16.1269910995696,-73.8030034797118,
-213.361373362703));
#224330=CARTESIAN_POINT('Ctrl Pts',(14.972352921708,-71.6600111165541,-216.668696986025));
#224331=CARTESIAN_POINT('Ctrl Pts',(13.8225787733862,-69.5169021371247,
-219.977682732017));
#224332=CARTESIAN_POINT('Ctrl Pts',(12.6830482858887,-67.374170068338,-223.290572851677));
#224333=CARTESIAN_POINT('Ctrl Pts',(11.5435177983912,-65.2314379995513,
-226.603462971338));
#224334=CARTESIAN_POINT('Ctrl Pts',(10.4133542529928,-63.0887592876515,
-229.919734283464));
#224335=CARTESIAN_POINT('Ctrl Pts',(9.30823614724962,-60.9492817427462,
-233.247030907634));
#224336=CARTESIAN_POINT('Ctrl Pts',(16.1509595327496,-73.8054672009588,
-213.361871023762));
#224337=CARTESIAN_POINT('Ctrl Pts',(14.99481342806,-71.66254340432,-216.669248038005));
#224338=CARTESIAN_POINT('Ctrl Pts',(13.8435558938089,-69.5195048912867,
-219.978299602301));
#224339=CARTESIAN_POINT('Ctrl Pts',(12.7025927706434,-67.3768540049101,
-223.291285721626));
#224340=CARTESIAN_POINT('Ctrl Pts',(11.5616296474779,-65.2342031185336,
-226.60427184095));
#224341=CARTESIAN_POINT('Ctrl Pts',(10.4300813444763,-63.0916122772264,
-229.920665266035));
#224342=CARTESIAN_POINT('Ctrl Pts',(9.32369428621562,-60.9522734066295,
-233.248170744691));
#224343=CARTESIAN_POINT('Ctrl Pts',(16.1749279659296,-73.8079309222057,
-213.362368684823));
#224344=CARTESIAN_POINT('Ctrl Pts',(15.0172739344119,-71.6650756920859,
-216.669799089985));
#224345=CARTESIAN_POINT('Ctrl Pts',(13.8645330142317,-69.5221076454487,
-219.978916472587));
#224346=CARTESIAN_POINT('Ctrl Pts',(12.7221372553981,-67.3795379414822,
-223.291998591574));
#224347=CARTESIAN_POINT('Ctrl Pts',(11.5797414965646,-65.2369682375158,
-226.605080710561));
#224348=CARTESIAN_POINT('Ctrl Pts',(10.4468084359598,-63.0944652668013,
-229.921596248607));
#224349=CARTESIAN_POINT('Ctrl Pts',(9.33915242518163,-60.9552650705129,
-233.249310581748));
#224350=CARTESIAN_POINT('Ctrl Pts',(16.1952404425737,-73.8106650452457,
-213.361731538637));
#224351=CARTESIAN_POINT('Ctrl Pts',(15.0357204215971,-71.6678714790176,
-216.669082666045));
#224352=CARTESIAN_POINT('Ctrl Pts',(13.8810654780263,-69.5249584688797,
-219.978101688701));
#224353=CARTESIAN_POINT('Ctrl Pts',(12.7366574254637,-67.3824171756017,
-223.29103806134));
#224354=CARTESIAN_POINT('Ctrl Pts',(11.5922493729011,-65.2398758823236,
-226.60397443398));
#224355=CARTESIAN_POINT('Ctrl Pts',(10.4572108953697,-63.0973827020436,
-229.920303449303));
#224356=CARTESIAN_POINT('Ctrl Pts',(9.34722878778031,-60.9580814427723,
-233.247692673937));
#224357=CARTESIAN_POINT('Ctrl Pts',(16.2167932117536,-73.8132831498057,
-213.361475819388));
#224358=CARTESIAN_POINT('Ctrl Pts',(15.0555279749194,-71.6705532338741,
-216.66879240035));
#224359=CARTESIAN_POINT('Ctrl Pts',(13.8991042674617,-69.5277002093038,
-219.977768430969));
#224360=CARTESIAN_POINT('Ctrl Pts',(12.7528793682099,-67.3852051104234,
-223.290640615083));
#224361=CARTESIAN_POINT('Ctrl Pts',(11.606654468958,-65.2427100115431,-226.603512799197));
#224362=CARTESIAN_POINT('Ctrl Pts',(10.4697535757153,-63.1002531490222,
-229.919759447509));
#224363=CARTESIAN_POINT('Ctrl Pts',(9.35780123871772,-60.9609326117186,
-233.247003746218));
#224364=CARTESIAN_POINT('Ctrl Pts',(16.3030042884734,-73.8237555680453,
-213.360452942392));
#224365=CARTESIAN_POINT('Ctrl Pts',(15.1347581882085,-71.6812802533,-216.667631337573));
#224366=CARTESIAN_POINT('Ctrl Pts',(13.9712594252033,-69.538667171,-219.976435400044));
#224367=CARTESIAN_POINT('Ctrl Pts',(12.8177671391946,-67.3963568497104,
-223.289050830054));
#224368=CARTESIAN_POINT('Ctrl Pts',(11.6642748531859,-65.2540465284208,
-226.601666260063));
#224369=CARTESIAN_POINT('Ctrl Pts',(10.5199242970979,-63.1117349369367,
-229.917583440332));
#224370=CARTESIAN_POINT('Ctrl Pts',(9.40009104246739,-60.972337287504,-233.24424803534));
#224371=CARTESIAN_POINT('Ctrl Pts',(16.3892942328758,-73.8339539222327,
-213.359415827195));
#224372=CARTESIAN_POINT('Ctrl Pts',(15.2140673832556,-71.6917296181947,
-216.666455999658));
#224373=CARTESIAN_POINT('Ctrl Pts',(14.0434937744094,-69.5493539058165,
-219.975088199201));
#224374=CARTESIAN_POINT('Ctrl Pts',(12.8827334643832,-67.4072286376852,
-223.287447402735));
#224375=CARTESIAN_POINT('Ctrl Pts',(11.7219731543571,-65.2651033695538,
-226.599806606268));
#224376=CARTESIAN_POINT('Ctrl Pts',(10.5701722900963,-63.1229397721944,
-229.915395364823));
#224377=CARTESIAN_POINT('Ctrl Pts',(9.44245022372204,-60.9834765470907,
-233.24148193285));
#224378=CARTESIAN_POINT('Ctrl Pts',(16.4756536810565,-73.8438772043577,
-213.358364250326));
#224379=CARTESIAN_POINT('Ctrl Pts',(15.2934473154818,-71.701900424371,-216.665266171061));
#224380=CARTESIAN_POINT('Ctrl Pts',(14.1158002338677,-69.5597595986373,
-219.973726626617));
#224381=CARTESIAN_POINT('Ctrl Pts',(12.9477726440111,-67.4178197482275,
-223.28583020421));
#224382=CARTESIAN_POINT('Ctrl Pts',(11.7797450541545,-65.2758798978176,
-226.597933781804));
#224383=CARTESIAN_POINT('Ctrl Pts',(10.6204947589536,-63.1338670513053,
-229.913195248458));
#224384=CARTESIAN_POINT('Ctrl Pts',(9.48487851765326,-60.9943501153261,
-233.238705966825));
#224385=CARTESIAN_POINT('Ctrl Pts',(16.6483725774179,-73.8637237686076,
-213.356261096586));
#224386=CARTESIAN_POINT('Ctrl Pts',(15.4522071799342,-71.7222420367236,
-216.662886513868));
#224387=CARTESIAN_POINT('Ctrl Pts',(14.2604131527844,-69.5805709842789,
-219.97100348145));
#224388=CARTESIAN_POINT('Ctrl Pts',(13.0778510032668,-67.4390019693121,
-223.282595807161));
#224389=CARTESIAN_POINT('Ctrl Pts',(11.8952888537493,-65.2974329543453,
-226.594188132872));
#224390=CARTESIAN_POINT('Ctrl Pts',(10.721139696668,-63.1557216095271,-229.908795015729));
#224391=CARTESIAN_POINT('Ctrl Pts',(9.5697351055157,-61.0160972517968,-233.233154034775));
#224392=CARTESIAN_POINT('Ctrl Pts',(16.8213694784135,-73.8824700233217,
-213.354100077751));
#224393=CARTESIAN_POINT('Ctrl Pts',(15.6112499819579,-71.7414693927443,
-216.660448871784));
#224394=CARTESIAN_POINT('Ctrl Pts',(14.4053145017287,-69.6002581805821,
-219.968222822437));
#224395=CARTESIAN_POINT('Ctrl Pts',(13.2082207723041,-67.459061467655,-223.279306294012));
#224396=CARTESIAN_POINT('Ctrl Pts',(12.0111270428794,-65.317864754728,-226.590389765588));
#224397=CARTESIAN_POINT('Ctrl Pts',(10.8220825428301,-63.1764659467185,
-229.904346578072));
#224398=CARTESIAN_POINT('Ctrl Pts',(9.65486815061528,-61.0367817019578,
-233.227562614776));
#224399=CARTESIAN_POINT('Ctrl Pts',(16.994569608081,-73.9001081635233,-213.351879630837));
#224400=CARTESIAN_POINT('Ctrl Pts',(15.7705099053261,-71.759575521472,-216.657951790479));
#224401=CARTESIAN_POINT('Ctrl Pts',(14.5504477647375,-69.6188149294841,
-219.965383361714));
#224402=CARTESIAN_POINT('Ctrl Pts',(13.3388364479968,-67.4779925971432,
-223.275961013328));
#224403=CARTESIAN_POINT('Ctrl Pts',(12.1272251312561,-65.3371702648023,
-226.586538664941));
#224404=CARTESIAN_POINT('Ctrl Pts',(10.9233008549698,-63.19609519418,-229.899850654492));
#224405=CARTESIAN_POINT('Ctrl Pts',(9.74027549478214,-61.0564003174753,
-233.2219363562));
#224406=CARTESIAN_POINT('Ctrl Pts',(17.340969867416,-73.9353844439267,-213.347438737011));
#224407=CARTESIAN_POINT('Ctrl Pts',(16.0890297520624,-71.7957877789274,
-216.652957627871));
#224408=CARTESIAN_POINT('Ctrl Pts',(14.8407142907551,-69.6559284272883,
-219.959704440269));
#224409=CARTESIAN_POINT('Ctrl Pts',(13.6000677993823,-67.5158548561195,
-223.269270451959));
#224410=CARTESIAN_POINT('Ctrl Pts',(12.3594213080095,-65.3757812849507,
-226.578836463649));
#224411=CARTESIAN_POINT('Ctrl Pts',(11.125737479249,-63.235353689103,-229.890858807335));
#224412=CARTESIAN_POINT('Ctrl Pts',(9.91109018311586,-61.0956375485103,
-233.210683839047));
#224413=CARTESIAN_POINT('Ctrl Pts',(17.6881829159947,-73.96622793775,-213.342759849927));
#224414=CARTESIAN_POINT('Ctrl Pts',(16.4084179353708,-71.8275148033868,
-216.647725367964));
#224415=CARTESIAN_POINT('Ctrl Pts',(15.1319083062413,-69.6885198227639,
-219.953789896397));
#224416=CARTESIAN_POINT('Ctrl Pts',(13.8622826479186,-67.5492034630686,
-223.262356339594));
#224417=CARTESIAN_POINT('Ctrl Pts',(12.5926569895958,-65.4098871033733,
-226.570922782791));
#224418=CARTESIAN_POINT('Ctrl Pts',(11.3292759747224,-63.2701519092751,
-229.881676366979));
#224419=CARTESIAN_POINT('Ctrl Pts',(10.0830023568968,-61.130612691193,-233.199291525399));
#224420=CARTESIAN_POINT('Ctrl Pts',(18.0356123358478,-73.9925802279162,
-213.337833927419));
#224421=CARTESIAN_POINT('Ctrl Pts',(16.7281499098057,-71.8547048439406,
-216.642247555954));
#224422=CARTESIAN_POINT('Ctrl Pts',(15.4235797449726,-69.7165429992444,
-219.947634512312));
#224423=CARTESIAN_POINT('Ctrl Pts',(14.1251185099795,-67.5779955815387,
-223.255219367308));
#224424=CARTESIAN_POINT('Ctrl Pts',(12.8266572749865,-65.4394481638329,
-226.562804222303));
#224425=CARTESIAN_POINT('Ctrl Pts',(11.533736224421,-63.300450082589,-229.872316979927));
#224426=CARTESIAN_POINT('Ctrl Pts',(10.2559925260419,-61.1612854472096,
-233.187802584487));
#224427=CARTESIAN_POINT('Ctrl Pts',(19.4253300152602,-74.0979893885809,
-213.31813023739));
#224428=CARTESIAN_POINT('Ctrl Pts',(18.0070778075454,-71.9634650061557,
-216.620336307913));
#224429=CARTESIAN_POINT('Ctrl Pts',(16.5902654998976,-69.8286357051668,
-219.923012975971));
#224430=CARTESIAN_POINT('Ctrl Pts',(15.1764619582234,-67.6931640554191,
-223.22667147816));
#224431=CARTESIAN_POINT('Ctrl Pts',(13.7626584165491,-65.5576924056715,
-226.53032998035));
#224432=CARTESIAN_POINT('Ctrl Pts',(12.3515772232155,-63.4216427758444,
-229.83487943172));
#224433=CARTESIAN_POINT('Ctrl Pts',(10.9479532026221,-61.2839764712757,
-233.14184682084));
#224434=CARTESIAN_POINT('Ctrl Pts',(20.8193262495726,-74.1303947430786,
-213.294867150046));
#224435=CARTESIAN_POINT('Ctrl Pts',(19.2921867436174,-71.9987556912252,
-216.594831507688));
#224436=CARTESIAN_POINT('Ctrl Pts',(17.7650869650877,-69.8670241956512,
-219.894793488995));
#224437=CARTESIAN_POINT('Ctrl Pts',(16.2379643566434,-67.735090498351,-223.194688298922));
#224438=CARTESIAN_POINT('Ctrl Pts',(14.7108417481991,-65.6031568010509,
-226.494583108848));
#224439=CARTESIAN_POINT('Ctrl Pts',(13.1837369485187,-63.4710380794777,
-229.794436678806));
#224440=CARTESIAN_POINT('Ctrl Pts',(11.6562419786961,-61.3384163644667,
-233.0939430997));
#224441=CARTESIAN_POINT('Ctrl Pts',(22.1870742035852,-74.0934804397454,
-213.269235878432));
#224442=CARTESIAN_POINT('Ctrl Pts',(20.5563486581314,-71.9629449474402,
-216.566743885946));
#224443=CARTESIAN_POINT('Ctrl Pts',(18.9243205135732,-69.8327666793285,
-219.863841772445));
#224444=CARTESIAN_POINT('Ctrl Pts',(17.289717647084,-67.703338899474,-223.16015770219));
#224445=CARTESIAN_POINT('Ctrl Pts',(15.6551147805949,-65.5739111196196,
-226.456473631934));
#224446=CARTESIAN_POINT('Ctrl Pts',(14.0181153557698,-63.4451661048359,
-229.752051509661));
#224447=CARTESIAN_POINT('Ctrl Pts',(12.3752611396561,-61.3182690712579,
-233.045942634108));
#224448=CARTESIAN_POINT('Ctrl Pts',(22.8709481805915,-74.0750232880787,
-213.256420242625));
#224449=CARTESIAN_POINT('Ctrl Pts',(21.1884296153885,-71.9450395755477,
-216.552700075075));
#224450=CARTESIAN_POINT('Ctrl Pts',(19.5039372878161,-69.8156379211672,
-219.848365914171));
#224451=CARTESIAN_POINT('Ctrl Pts',(17.8155942923044,-67.6874631000356,
-223.142892403823));
#224452=CARTESIAN_POINT('Ctrl Pts',(16.1272512967927,-65.559288278904,-226.437418893476));
#224453=CARTESIAN_POINT('Ctrl Pts',(14.4353045593953,-63.432230117515,-229.730858925089));
#224454=CARTESIAN_POINT('Ctrl Pts',(12.7347707201362,-61.3081954246535,
-233.021942401313));
#224455=CARTESIAN_POINT('Ctrl Pts',(23.5480695180481,-74.0394366671371,
-213.24294581755));
#224456=CARTESIAN_POINT('Ctrl Pts',(21.8151227650933,-71.9095199232041,
-216.537959093058));
#224457=CARTESIAN_POINT('Ctrl Pts',(20.0795547520248,-69.7804677651607,
-219.832174698833));
#224458=CARTESIAN_POINT('Ctrl Pts',(18.3389963496171,-67.653239079547,-223.124983513773));
#224459=CARTESIAN_POINT('Ctrl Pts',(16.5984379472094,-65.5260103939333,
-226.417792328712));
#224460=CARTESIAN_POINT('Ctrl Pts',(14.8531613104273,-63.4004482694333,
-229.709234763845));
#224461=CARTESIAN_POINT('Ctrl Pts',(13.0971728800481,-61.2793476978764,
-232.998003019156));
#224462=CARTESIAN_POINT('Ctrl Pts',(24.2157714140089,-73.9880357308627,
-213.229014471039));
#224463=CARTESIAN_POINT('Ctrl Pts',(22.4339461787341,-71.8573077591636,
-216.522677077293));
#224464=CARTESIAN_POINT('Ctrl Pts',(20.6488795380189,-69.727793615988,-219.815393786219));
#224465=CARTESIAN_POINT('Ctrl Pts',(18.8578584941687,-67.6007885459759,
-223.106553748693));
#224466=CARTESIAN_POINT('Ctrl Pts',(17.0668374503185,-65.4737834759639,
-226.397713711167));
#224467=CARTESIAN_POINT('Ctrl Pts',(15.2701229993281,-63.3491012702381,
-229.687335801967));
#224468=CARTESIAN_POINT('Ctrl Pts',(13.4612647392516,-61.2303346129408,
-232.974299931676));
#224469=CARTESIAN_POINT('Ctrl Pts',(24.3826968879991,-73.9751854967941,
-213.225531634411));
#224470=CARTESIAN_POINT('Ctrl Pts',(22.5886520321442,-71.8442547181535,
-216.518856573352));
#224471=CARTESIAN_POINT('Ctrl Pts',(20.7912107345175,-69.7146250786948,
-219.811198558066));
#224472=CARTESIAN_POINT('Ctrl Pts',(18.9875740303066,-67.5876759125832,
-223.101946307423));
#224473=CARTESIAN_POINT('Ctrl Pts',(17.1839373260957,-65.4607267464716,
-226.39269405678));
#224474=CARTESIAN_POINT('Ctrl Pts',(15.3743634215533,-63.3362645204393,
-229.681861061497));
#224475=CARTESIAN_POINT('Ctrl Pts',(13.5522877040525,-61.2180813417068,
-232.968374159806));
#224476=CARTESIAN_POINT('Ctrl Pts',(24.5490260926448,-73.9613534513551,
-213.222016096025));
#224477=CARTESIAN_POINT('Ctrl Pts',(22.7428608767437,-71.8301631357306,
-216.514999213761));
#224478=CARTESIAN_POINT('Ctrl Pts',(20.9331465818466,-69.7003652432428,
-219.806964785417));
#224479=CARTESIAN_POINT('Ctrl Pts',(19.1170081030222,-67.573424236258,-223.09730631659));
#224480=CARTESIAN_POINT('Ctrl Pts',(17.3008696241978,-65.4464832292733,
-226.387647847762));
#224481=CARTESIAN_POINT('Ctrl Pts',(15.4785601554459,-63.3221993407807,
-229.676372916497));
#224482=CARTESIAN_POINT('Ctrl Pts',(13.6434360700701,-61.2045576567449,
-232.962469186235));
#224483=CARTESIAN_POINT('Ctrl Pts',(24.7147083990055,-73.9465669153719,
-213.218466861474));
#224484=CARTESIAN_POINT('Ctrl Pts',(22.896527662223,-71.8150523527131,-216.511104550879));
#224485=CARTESIAN_POINT('Ctrl Pts',(21.0746484989543,-69.6850253260801,
-219.802693125391));
#224486=CARTESIAN_POINT('Ctrl Pts',(19.2461305058791,-67.5580352841076,
-223.092636242469));
#224487=CARTESIAN_POINT('Ctrl Pts',(17.417612512804,-65.431045242135,-226.382579359546));
#224488=CARTESIAN_POINT('Ctrl Pts',(15.5827019558228,-63.3068875335093,
-229.670878428191));
#224489=CARTESIAN_POINT('Ctrl Pts',(13.7347113090105,-61.1897293326642,
-232.956594042948));
#224490=CARTESIAN_POINT('Ctrl Pts',(24.7975495521858,-73.9391736473804,
-213.216692244198));
#224491=CARTESIAN_POINT('Ctrl Pts',(22.9733610549627,-71.8074969612043,
-216.509157219438));
#224492=CARTESIAN_POINT('Ctrl Pts',(21.1453994575082,-69.6773553674987,
-219.800557295379));
#224493=CARTESIAN_POINT('Ctrl Pts',(19.3106917073076,-67.5503408080323,
-223.090301205408));
#224494=CARTESIAN_POINT('Ctrl Pts',(17.4759839571071,-65.4233262485659,
-226.380045115437));
#224495=CARTESIAN_POINT('Ctrl Pts',(15.6347728560114,-63.2992316298737,
-229.668131184037));
#224496=CARTESIAN_POINT('Ctrl Pts',(13.7803489284807,-61.1823151706239,
-232.953656471305));
#224497=CARTESIAN_POINT('Ctrl Pts',(24.8802289805,-73.9315417594893,-213.214909206118));
#224498=CARTESIAN_POINT('Ctrl Pts',(23.0500589324285,-71.7996867719131,
-216.507200566405));
#224499=CARTESIAN_POINT('Ctrl Pts',(21.2160419341602,-69.6694153895317,
-219.79841199949));
#224500=CARTESIAN_POINT('Ctrl Pts',(19.3751749925241,-67.5423620096871,
-223.087958654086));
#224501=CARTESIAN_POINT('Ctrl Pts',(17.5343080508878,-65.4153086298425,
-226.37750530868));
#224502=CARTESIAN_POINT('Ctrl Pts',(15.6868300264596,-63.2912640530134,
-229.665382361024));
#224503=CARTESIAN_POINT('Ctrl Pts',(13.8260182553397,-61.174574822688,-232.950726355029));
#224504=CARTESIAN_POINT('Ctrl Pts',(24.9627403530718,-73.9236746829435,
-213.213117642504));
#224505=CARTESIAN_POINT('Ctrl Pts',(23.126615659932,-71.7916242163204,-216.505234561518));
#224506=CARTESIAN_POINT('Ctrl Pts',(21.2865711101662,-69.6612067996815,
-219.796257356157));
#224507=CARTESIAN_POINT('Ctrl Pts',(19.4395765925294,-67.5340990890229,
-223.085608935934));
#224508=CARTESIAN_POINT('Ctrl Pts',(17.5925820748926,-65.4069913783643,
-226.374960515711));
#224509=CARTESIAN_POINT('Ctrl Pts',(15.7388720794492,-63.2829824280864,
-229.662632880377));
#224510=CARTESIAN_POINT('Ctrl Pts',(13.8717193997709,-61.1665038590085,
-232.947804805376));
#224511=CARTESIAN_POINT('Ctrl Pts',(25.0039960393577,-73.9197411446707,
-213.212221860697));
#224512=CARTESIAN_POINT('Ctrl Pts',(23.1648940236837,-71.787592938524,-216.504251559075));
#224513=CARTESIAN_POINT('Ctrl Pts',(21.3218356981692,-69.6571025047564,
-219.79518003449));
#224514=CARTESIAN_POINT('Ctrl Pts',(19.4717773925321,-67.5299676286908,
-223.084434076858));
#224515=CARTESIAN_POINT('Ctrl Pts',(17.621719086895,-65.4028327526252,-226.373688119227));
#224516=CARTESIAN_POINT('Ctrl Pts',(15.764893105944,-63.2788416156229,-229.661258140053));
#224517=CARTESIAN_POINT('Ctrl Pts',(13.8945699719865,-61.1624683771687,
-232.946344030549));
#224518=CARTESIAN_POINT('Ctrl Pts',(25.0452097116804,-73.9157488094,-213.211323947711));
#224519=CARTESIAN_POINT('Ctrl Pts',(23.2031370999057,-71.7834985692942,
-216.503266218939));
#224520=CARTESIAN_POINT('Ctrl Pts',(21.357071961051,-69.6529310569108,-219.794100376343));
#224521=CARTESIAN_POINT('Ctrl Pts',(19.5039577712971,-67.5257651375524,
-223.083257426481));
#224522=CARTESIAN_POINT('Ctrl Pts',(17.6508435815433,-65.3985992181939,
-226.372414476619));
#224523=CARTESIAN_POINT('Ctrl Pts',(15.7909103532289,-63.2746222900822,
-229.659883235697));
#224524=CARTESIAN_POINT('Ctrl Pts',(13.9174284977559,-61.1583502398543,
-232.944885397156));
#224525=CARTESIAN_POINT('Ctrl Pts',(25.0863805784989,-73.9116981070247,
-213.210423891692));
#224526=CARTESIAN_POINT('Ctrl Pts',(23.2413441840135,-71.7793414134085,
-216.502278538958));
#224527=CARTESIAN_POINT('Ctrl Pts',(21.3922792967075,-69.6486926323577,
-219.793018398826));
#224528=CARTESIAN_POINT('Ctrl Pts',(19.5361172580662,-67.5214916392097,
-223.082079030659));
#224529=CARTESIAN_POINT('Ctrl Pts',(17.679955219425,-65.3942906460616,-226.371139662493));
#224530=CARTESIAN_POINT('Ctrl Pts',(15.8169236486359,-63.2703241481897,
-229.658508284608));
#224531=CARTESIAN_POINT('Ctrl Pts',(13.9402949855555,-61.1541488842813,
-232.943429042643));
#224532=CARTESIAN_POINT('Ctrl Pts',(25.0966732952035,-73.9106854314309,
-213.210198877688));
#224533=CARTESIAN_POINT('Ctrl Pts',(23.2508959550404,-71.7783021244371,
-216.502031618964));
#224534=CARTESIAN_POINT('Ctrl Pts',(21.4010811306217,-69.6476330262194,
-219.792747904446));
#224535=CARTESIAN_POINT('Ctrl Pts',(19.5441571297585,-67.520423264624,-223.081784431704));
#224536=CARTESIAN_POINT('Ctrl Pts',(17.6872331288954,-65.3932135030285,
-226.370820958961));
#224537=CARTESIAN_POINT('Ctrl Pts',(15.8234269724877,-63.2692496127166,
-229.658164546835));
#224538=CARTESIAN_POINT('Ctrl Pts',(13.9460116075054,-61.1530985453881,
-232.943064954015));
#224539=CARTESIAN_POINT('Ctrl Pts',(25.1069633365636,-73.9096691078962,
-213.209973729747));
#224540=CARTESIAN_POINT('Ctrl Pts',(23.2604454765595,-71.7772589113024,
-216.501784552734));
#224541=CARTESIAN_POINT('Ctrl Pts',(21.409881156585,-69.6465692340378,-219.792477265113));
#224542=CARTESIAN_POINT('Ctrl Pts',(19.5521956957022,-67.5193504520834,
-223.081489723665));
#224543=CARTESIAN_POINT('Ctrl Pts',(17.6945102348195,-65.392131670129,-226.370502182217));
#224544=CARTESIAN_POINT('Ctrl Pts',(15.8299300493494,-63.2681701512003,
-229.657820806149));
#224545=CARTESIAN_POINT('Ctrl Pts',(13.9517287270644,-61.1520430053247,
-232.942701007811));
#224546=CARTESIAN_POINT('Ctrl Pts',(25.1172506902097,-73.9086491431441,
-213.209748447694));
#224547=CARTESIAN_POINT('Ctrl Pts',(23.2699927375595,-71.776211778772,-216.501537340246));
#224548=CARTESIAN_POINT('Ctrl Pts',(21.4186793651912,-69.6455012585676,
-219.792206481111));
#224549=CARTESIAN_POINT('Ctrl Pts',(19.5602329485438,-67.5182732019474,
-223.081194907278));
#224550=CARTESIAN_POINT('Ctrl Pts',(17.7017865318965,-65.3910451453272,
-226.370183333445));
#224551=CARTESIAN_POINT('Ctrl Pts',(15.836432876527,-63.2670857588602,-229.657477064395));
#224552=CARTESIAN_POINT('Ctrl Pts',(13.9574463443279,-61.1509822552403,
-232.942337206169));
#224553=CARTESIAN_POINT('Ctrl Pts',(25.1275380438559,-73.9076291783921,
-213.209523165641));
#224554=CARTESIAN_POINT('Ctrl Pts',(23.2795399985595,-71.7751646462416,
-216.501290127757));
#224555=CARTESIAN_POINT('Ctrl Pts',(21.4274775737974,-69.6444332830974,
-219.791935697108));
#224556=CARTESIAN_POINT('Ctrl Pts',(19.5682702013855,-67.5171959518114,
-223.080900090889));
#224557=CARTESIAN_POINT('Ctrl Pts',(17.7090628289735,-65.3899586205254,
-226.369864484671));
#224558=CARTESIAN_POINT('Ctrl Pts',(15.8429357037046,-63.2660013665201,
-229.65713332264));
#224559=CARTESIAN_POINT('Ctrl Pts',(13.9631639615914,-61.149921505156,-232.941973404527));
#224560=CARTESIAN_POINT('Ctrl Pts',(25.1372576920846,-73.906800444898,-213.209112994181));
#224561=CARTESIAN_POINT('Ctrl Pts',(23.2884525006053,-71.7743376152923,
-216.500839713002));
#224562=CARTESIAN_POINT('Ctrl Pts',(21.435563238532,-69.643620799134,-219.791441687824));
#224563=CARTESIAN_POINT('Ctrl Pts',(19.5754996444385,-67.5164229145748,
-223.080361001592));
#224564=CARTESIAN_POINT('Ctrl Pts',(17.7154360503449,-65.3892250300156,
-226.369280315361));
#224565=CARTESIAN_POINT('Ctrl Pts',(15.8484227674922,-63.2653312673536,
-229.656501770123));
#224566=CARTESIAN_POINT('Ctrl Pts',(13.9677245066283,-61.1493660025175,
-232.941302670312));
#224567=CARTESIAN_POINT('Ctrl Pts',(25.1485775908394,-73.9054141624897,
-213.20922679825));
#224568=CARTESIAN_POINT('Ctrl Pts',(23.2991570846935,-71.7728700013319,
-216.500965172341));
#224569=CARTESIAN_POINT('Ctrl Pts',(21.4456633269895,-69.642066256973,-219.791580356526));
#224570=CARTESIAN_POINT('Ctrl Pts',(19.5850156941798,-67.5147685546832,
-223.080514436398));
#224571=CARTESIAN_POINT('Ctrl Pts',(17.72436806137,-65.3874708523934,-226.369448516268));
#224572=CARTESIAN_POINT('Ctrl Pts',(15.8567904524694,-63.2634655201446,
-229.656686662214));
#224573=CARTESIAN_POINT('Ctrl Pts',(13.9755694621328,-61.1473556487549,
-232.941503186179));
#224574=CARTESIAN_POINT('Ctrl Pts',(25.171217388349,-73.9026415976731,-213.209454406389));
#224575=CARTESIAN_POINT('Ctrl Pts',(23.3205662528698,-71.7699347734113,
-216.501216091021));
#224576=CARTESIAN_POINT('Ctrl Pts',(21.4658635039045,-69.6389571726509,
-219.791857693933));
#224577=CARTESIAN_POINT('Ctrl Pts',(19.6040477936623,-67.5114598348999,
-223.080821306008));
#224578=CARTESIAN_POINT('Ctrl Pts',(17.7422320834202,-65.383962497149,-226.369784918083));
#224579=CARTESIAN_POINT('Ctrl Pts',(15.8735258224239,-63.2597340257264,
-229.657056446399));
#224580=CARTESIAN_POINT('Ctrl Pts',(13.9912593731417,-61.1433349412296,
-232.941904217913));
#224581=CARTESIAN_POINT('Ctrl Pts',(25.193849356443,-73.8998869012639,-213.209683688439));
#224582=CARTESIAN_POINT('Ctrl Pts',(23.3419708963093,-71.7670180254577,
-216.501468996797));
#224583=CARTESIAN_POINT('Ctrl Pts',(21.4860624620753,-69.6358671958947,
-219.792137371206));
#224584=CARTESIAN_POINT('Ctrl Pts',(19.62308191069,-67.5081709556807,-223.081130950866));
#224585=CARTESIAN_POINT('Ctrl Pts',(17.7601013593046,-65.3804747154667,
-226.370124530527));
#224586=CARTESIAN_POINT('Ctrl Pts',(15.8902696209903,-63.2560239166916,
-229.657429944766));
#224587=CARTESIAN_POINT('Ctrl Pts',(14.0069606167652,-61.1393368768376,
-232.942309711861));
#224588=CARTESIAN_POINT('Ctrl Pts',(25.2164735434192,-73.8971500307629,
-213.209914643404));
#224589=CARTESIAN_POINT('Ctrl Pts',(23.3633710413963,-71.7641197332832,
-216.501723891369));
#224590=CARTESIAN_POINT('Ctrl Pts',(21.5062602068588,-69.6327963210985,
-219.792419393227));
#224591=CARTESIAN_POINT('Ctrl Pts',(19.6421180325673,-67.5049019292739,
-223.081443379648));
#224592=CARTESIAN_POINT('Ctrl Pts',(17.7779758582759,-65.3770075374493,
-226.370467366069));
#224593=CARTESIAN_POINT('Ctrl Pts',(15.9070218020689,-63.2523352409534,
-229.65780717451));
#224594=CARTESIAN_POINT('Ctrl Pts',(14.0226731406812,-61.1353615142731,
-232.942719688923));
#224595=CARTESIAN_POINT('Ctrl Pts',(25.5784605350381,-73.8533601027457,
-213.213609922837));
#224596=CARTESIAN_POINT('Ctrl Pts',(23.7057733627864,-71.7177470584899,
-216.505802204519));
#224597=CARTESIAN_POINT('Ctrl Pts',(21.8294241233942,-69.5836623243583,
-219.796931745576));
#224598=CARTESIAN_POINT('Ctrl Pts',(19.9466959826056,-67.4525975067642,
-223.08644224016));
#224599=CARTESIAN_POINT('Ctrl Pts',(18.063967841817,-65.32153268917,-226.375952734744));
#224600=CARTESIAN_POINT('Ctrl Pts',(16.1750566993262,-63.1933164291426,
-229.663842850422));
#224601=CARTESIAN_POINT('Ctrl Pts',(14.274073523336,-61.0717557132421,-232.94927932191));
#224602=CARTESIAN_POINT('Ctrl Pts',(25.9384558510478,-73.8141338585575,
-213.217733341187));
#224603=CARTESIAN_POINT('Ctrl Pts',(24.0470243860156,-71.6760992561169,
-216.510389357129));
#224604=CARTESIAN_POINT('Ctrl Pts',(22.1522776113516,-69.5394185327721,
-219.802043797164));
#224605=CARTESIAN_POINT('Ctrl Pts',(20.2517872646464,-67.4053752329754,
-223.09215272069));
#224606=CARTESIAN_POINT('Ctrl Pts',(18.3512969179412,-65.2713319331787,
-226.382261644215));
#224607=CARTESIAN_POINT('Ctrl Pts',(16.4452373481732,-63.1397837380439,
-229.670831497313));
#224608=CARTESIAN_POINT('Ctrl Pts',(14.5283616228576,-61.0139593295415,
-232.956982844669));
#224609=CARTESIAN_POINT('Ctrl Pts',(26.2966554094189,-73.7792956476803,
-213.222281607897));
#224610=CARTESIAN_POINT('Ctrl Pts',(24.3872303655758,-71.6390760412376,
-216.515494177504));
#224611=CARTESIAN_POINT('Ctrl Pts',(22.4748413391966,-69.5000413221577,
-219.807779103235));
#224612=CARTESIAN_POINT('Ctrl Pts',(20.5573393020075,-67.3632863153329,
-223.098617135674));
#224613=CARTESIAN_POINT('Ctrl Pts',(18.6398372648184,-65.2265313085082,
-226.389455168112));
#224614=CARTESIAN_POINT('Ctrl Pts',(16.7173760151004,-63.0919383281592,
-229.678857882383));
#224615=CARTESIAN_POINT('Ctrl Pts',(14.7853232876775,-60.9622268937814,
-232.965939947976));
#224616=CARTESIAN_POINT('Ctrl Pts',(27.7294536429034,-73.6399428041712,
-213.240474674736));
#224617=CARTESIAN_POINT('Ctrl Pts',(25.7480542838167,-71.4909831817206,
-216.535913459003));
#224618=CARTESIAN_POINT('Ctrl Pts',(23.7650962505765,-69.3425324796999,
-219.830720327519));
#224619=CARTESIAN_POINT('Ctrl Pts',(21.779547451452,-67.194930644763,-223.124474795611));
#224620=CARTESIAN_POINT('Ctrl Pts',(19.7939986523274,-65.047328809826,-226.418229263702));
#224621=CARTESIAN_POINT('Ctrl Pts',(17.8059306828092,-62.9005566886207,
-229.710963422663));
#224622=CARTESIAN_POINT('Ctrl Pts',(15.8131699469571,-60.7552971507412,
-233.001768361203));
#224623=CARTESIAN_POINT('Ctrl Pts',(29.1336039587918,-73.5700373872199,
-213.265253638125));
#224624=CARTESIAN_POINT('Ctrl Pts',(27.0924699780351,-71.4163743252597,
-216.564463234942));
#224625=CARTESIAN_POINT('Ctrl Pts',(25.0512545912863,-69.2626269169371,
-219.863532185965));
#224626=CARTESIAN_POINT('Ctrl Pts',(23.009917484108,-67.1086533562946,-223.162319906733));
#224627=CARTESIAN_POINT('Ctrl Pts',(20.9685803769297,-64.9546797956521,
-226.461107627501));
#224628=CARTESIAN_POINT('Ctrl Pts',(18.9271177265018,-62.8005017163077,
-229.759627201665));
#224629=CARTESIAN_POINT('Ctrl Pts',(16.8854980114262,-60.6457046773919,
-233.057542008322));
#224630=CARTESIAN_POINT('Ctrl Pts',(30.5241947376933,-73.5610723424065,
-213.298768106723));
#224631=CARTESIAN_POINT('Ctrl Pts',(28.4276303246838,-71.4106207619993,
-216.603490576448));
#224632=CARTESIAN_POINT('Ctrl Pts',(26.3326980553491,-69.2597735546542,
-219.908997954484));
#224633=CARTESIAN_POINT('Ctrl Pts',(24.2404948075201,-67.1083375120314,
-223.215865028163));
#224634=CARTESIAN_POINT('Ctrl Pts',(22.1482915596912,-64.9569014694087,
-226.522732101842));
#224635=CARTESIAN_POINT('Ctrl Pts',(20.0587460706978,-62.804879241495,-229.830915083865));
#224636=CARTESIAN_POINT('Ctrl Pts',(17.9741423861781,-60.6519644373032,
-233.141673289922));
#224637=CARTESIAN_POINT('Ctrl Pts',(31.9147855165948,-73.552107297593,-213.332282575321));
#224638=CARTESIAN_POINT('Ctrl Pts',(29.7627906713323,-71.4048671987388,
-216.642517917954));
#224639=CARTESIAN_POINT('Ctrl Pts',(27.6141415194118,-69.2569201923712,
-219.954463723003));
#224640=CARTESIAN_POINT('Ctrl Pts',(25.4710721309322,-67.1080216677683,
-223.269410149593));
#224641=CARTESIAN_POINT('Ctrl Pts',(23.3280027424525,-64.9591231431653,
-226.584356576183));
#224642=CARTESIAN_POINT('Ctrl Pts',(21.1903744148938,-62.8092567666822,
-229.902202966066));
#224643=CARTESIAN_POINT('Ctrl Pts',(19.0627867609299,-60.6582241972144,
-233.225804571522));
#224644=CARTESIAN_POINT('Ctrl Pts',(33.2915597883743,-73.6042889215309,
-213.3745249105));
#224645=CARTESIAN_POINT('Ctrl Pts',(31.0883634812026,-71.4681526003391,
-216.692012555656));
#224646=CARTESIAN_POINT('Ctrl Pts',(28.8904868213177,-69.3312704464791,
-220.012578308793));
#224647=CARTESIAN_POINT('Ctrl Pts',(26.7014864455774,-67.1937325026255,
-223.338673968425));
#224648=CARTESIAN_POINT('Ctrl Pts',(24.5124860698371,-65.0561945587718,
-226.664769628056));
#224649=CARTESIAN_POINT('Ctrl Pts',(22.3321348006731,-62.917889592856,-229.996164050331));
#224650=CARTESIAN_POINT('Ctrl Pts',(20.1678151009338,-60.7799059276878,
-233.338582766125));
#224651=CARTESIAN_POINT('Ctrl Pts',(34.6658396818832,-73.7171632516111,
-213.428100838228));
#224652=CARTESIAN_POINT('Ctrl Pts',(32.4073514514279,-71.6005216742458,
-216.754800866965));
#224653=CARTESIAN_POINT('Ctrl Pts',(30.156682789701,-69.4835812050588,-220.0867754185));
#224654=CARTESIAN_POINT('Ctrl Pts',(27.9187794471608,-67.3680563271126,
-223.428575651002));
#224655=CARTESIAN_POINT('Ctrl Pts',(25.6808761046207,-65.2525314491663,
-226.770375883503));
#224656=CARTESIAN_POINT('Ctrl Pts',(23.4556914905238,-63.1380571190676,
-230.121736209584));
#224657=CARTESIAN_POINT('Ctrl Pts',(21.2513677279665,-61.0308575536311,
-233.492320591243));
#224658=CARTESIAN_POINT('',(1.75269631448936,-61.4233992294301,-232.850052402311));
#224659=CARTESIAN_POINT('',(3.75861995924126,-61.4153261928714,-232.250048639703));
#224660=CARTESIAN_POINT('Ctrl Pts',(1.75269750311554,-61.4233975212337,
-232.850057162107));
#224661=CARTESIAN_POINT('Ctrl Pts',(1.92316075991213,-61.4229613169472,
-232.80733217942));
#224662=CARTESIAN_POINT('Ctrl Pts',(2.09239735025022,-61.4224645393753,
-232.759040177349));
#224663=CARTESIAN_POINT('Ctrl Pts',(2.40516232917589,-61.4214325003053,
-232.659804474909));
#224664=CARTESIAN_POINT('Ctrl Pts',(2.54699173612178,-61.4209053575993,
-232.609626264845));
#224665=CARTESIAN_POINT('Ctrl Pts',(2.58749755058152,-61.4207526026485,
-232.595189827728));
#224666=CARTESIAN_POINT('Ctrl Pts',(2.59231693841156,-61.4207343791064,
-232.593474272114));
#224667=CARTESIAN_POINT('Ctrl Pts',(2.5994697764427,-61.420707260306,-232.590934719885));
#224668=CARTESIAN_POINT('Ctrl Pts',(2.60233972176209,-61.4206963617489,
-232.589917449231));
#224669=CARTESIAN_POINT('Ctrl Pts',(2.65446877101508,-61.4204981063414,
-232.571459343799));
#224670=CARTESIAN_POINT('Ctrl Pts',(2.70416777645081,-61.420303711325,-232.554260849743));
#224671=CARTESIAN_POINT('Ctrl Pts',(3.08402302180499,-61.4187763761994,
-232.425844903788));
#224672=CARTESIAN_POINT('Ctrl Pts',(3.41955797258862,-61.4171877854095,
-232.329833606325));
#224673=CARTESIAN_POINT('Ctrl Pts',(3.75861934084146,-61.4153271385636,
-232.25004598973));
#224674=CARTESIAN_POINT('',(-1.75269627833716,-61.4233992207715,-232.850052391314));
#224675=CARTESIAN_POINT('Ctrl Pts',(-1.75269547230688,-61.4234026156414,
-232.85005));
#224676=CARTESIAN_POINT('Ctrl Pts',(-1.17332845865336,-61.5217870874547,
-232.85005));
#224677=CARTESIAN_POINT('Ctrl Pts',(-0.588369382046338,-61.5708786969769,
-232.850050000284));
#224678=CARTESIAN_POINT('Ctrl Pts',(0.591121623461373,-61.5706529925896,
-232.850050000284));
#224679=CARTESIAN_POINT('Ctrl Pts',(1.17468362875101,-61.5215566961185,
-232.85005));
#224680=CARTESIAN_POINT('Ctrl Pts',(1.7526954934496,-61.4234026418405,-232.85005));
#224681=CARTESIAN_POINT('',(-3.75861995924035,-61.4153261928713,-232.250048639703));
#224682=CARTESIAN_POINT('Ctrl Pts',(-1.75269746119008,-61.4233975213411,
-232.850057127972));
#224683=CARTESIAN_POINT('Ctrl Pts',(-1.92316007055054,-61.4229613187217,
-232.80733218066));
#224684=CARTESIAN_POINT('Ctrl Pts',(-2.09239806687771,-61.422464537097,
-232.759039771134));
#224685=CARTESIAN_POINT('Ctrl Pts',(-2.40516295459882,-61.4214324981669,
-232.659804234222));
#224686=CARTESIAN_POINT('Ctrl Pts',(-2.54699180261749,-61.4209053573394,
-232.609626241571));
#224687=CARTESIAN_POINT('Ctrl Pts',(-2.58749737645083,-61.4207526033062,
-232.595189889748));
#224688=CARTESIAN_POINT('Ctrl Pts',(-2.59231675754469,-61.420734379791,
-232.593474336454));
#224689=CARTESIAN_POINT('Ctrl Pts',(-2.59946962941021,-61.4207072608641,
-232.590934772013));
#224690=CARTESIAN_POINT('Ctrl Pts',(-2.60233959172383,-61.4206963622429,
-232.589917495322));
#224691=CARTESIAN_POINT('Ctrl Pts',(-2.65446865657193,-61.420498106789,
-232.571459383405));
#224692=CARTESIAN_POINT('Ctrl Pts',(-2.70416771898085,-61.420303711556,
-232.554260869169));
#224693=CARTESIAN_POINT('Ctrl Pts',(-3.08402302193468,-61.4187763761988,
-232.42584490375));
#224694=CARTESIAN_POINT('Ctrl Pts',(-3.41955797265308,-61.4171877854092,
-232.329833606309));
#224695=CARTESIAN_POINT('Ctrl Pts',(-3.75861934084049,-61.4153271385636,
-232.250045989729));
#224696=CARTESIAN_POINT('Ctrl Pts',(-3.75861965563748,-61.4153243588594,
-232.25005));
#224697=CARTESIAN_POINT('Ctrl Pts',(-4.5339585652984,-61.2869745330173,
-232.25005));
#224698=CARTESIAN_POINT('Ctrl Pts',(-5.31753185133202,-61.2192652887292,
-232.250049999975));
#224699=CARTESIAN_POINT('Ctrl Pts',(-6.89308966243379,-61.2051366152526,
-232.250049999975));
#224700=CARTESIAN_POINT('Ctrl Pts',(-7.68211271552188,-61.2596464565366,
-232.25005));
#224701=CARTESIAN_POINT('Ctrl Pts',(-8.46313927246256,-61.3733404249057,
-232.25005));
#224702=CARTESIAN_POINT('',(33.4888861408047,-72.9429671618309,-214.578382767941));
#224703=CARTESIAN_POINT('Ctrl Pts',(-33.4888960070708,-72.9429805807943,
-214.578360966077));
#224704=CARTESIAN_POINT('Ctrl Pts',(-32.3582303407525,-72.9833613098026,
-214.304136356274));
#224705=CARTESIAN_POINT('Ctrl Pts',(-31.1954383806093,-73.0208514112019,
-214.148157206533));
#224706=CARTESIAN_POINT('Ctrl Pts',(-30.0308162541928,-73.0549738991022,
-214.07652205636));
#224707=CARTESIAN_POINT('Ctrl Pts',(-28.8424164729157,-73.08979305309,-214.003424358087));
#224708=CARTESIAN_POINT('Ctrl Pts',(-27.6841438207362,-73.1198927243157,
-214.026849366582));
#224709=CARTESIAN_POINT('Ctrl Pts',(-26.7546989061683,-73.1422369981543,
-214.085588387952));
#224710=CARTESIAN_POINT('Ctrl Pts',(-26.3846816526908,-73.1511323793728,
-214.108972723073));
#224711=CARTESIAN_POINT('Ctrl Pts',(-26.0470604925031,-73.1589301782192,
-214.137473495031));
#224712=CARTESIAN_POINT('Ctrl Pts',(-25.7490556660394,-73.1656334354033,
-214.1665654633));
#224713=CARTESIAN_POINT('Ctrl Pts',(-25.2381704858424,-73.1771251779869,
-214.216439338256));
#224714=CARTESIAN_POINT('Ctrl Pts',(-24.843656759113,-73.1854170412888,
-214.267796851654));
#224715=CARTESIAN_POINT('Ctrl Pts',(-24.6022876971483,-73.1904242292317,
-214.300631104614));
#224716=CARTESIAN_POINT('Ctrl Pts',(-24.5762615999557,-73.1909641391895,
-214.304171522975));
#224717=CARTESIAN_POINT('Ctrl Pts',(-24.5520172332706,-73.191465550504,
-214.307503072173));
#224718=CARTESIAN_POINT('Ctrl Pts',(-24.5296015630572,-73.1919280895696,
-214.310606246882));
#224719=CARTESIAN_POINT('Ctrl Pts',(-24.5181753315148,-73.192163865632,
-214.312188068545));
#224720=CARTESIAN_POINT('Ctrl Pts',(-24.5072235105972,-73.1923896531126,
-214.313705098403));
#224721=CARTESIAN_POINT('Ctrl Pts',(-24.4967513448984,-73.1926055432137,
-214.315147724587));
#224722=CARTESIAN_POINT('Ctrl Pts',(-24.4856096015616,-73.1928352370674,
-214.31668259055));
#224723=CARTESIAN_POINT('Ctrl Pts',(-24.475145401741,-73.1930508945055,
-214.318118499124));
#224724=CARTESIAN_POINT('Ctrl Pts',(-24.4645402940566,-73.193269393582,
-214.31956858846));
#224725=CARTESIAN_POINT('Ctrl Pts',(-24.4216369917593,-73.1941533385836,
-214.325434971244));
#224726=CARTESIAN_POINT('Ctrl Pts',(-24.3787176016695,-73.1950365526006,
-214.331215731291));
#224727=CARTESIAN_POINT('Ctrl Pts',(-24.3357827357383,-73.1959190376299,
-214.336909622653));
#224728=CARTESIAN_POINT('Ctrl Pts',(-24.2501463703594,-73.1976792110641,
-214.348266457021));
#224729=CARTESIAN_POINT('Ctrl Pts',(-24.1644484378959,-73.1994364840595,
-214.359277703943));
#224730=CARTESIAN_POINT('Ctrl Pts',(-24.0786937902358,-73.2011908763299,
-214.369933459421));
#224731=CARTESIAN_POINT('Ctrl Pts',(-23.9081084143817,-73.2046807590709,
-214.391130165404));
#224732=CARTESIAN_POINT('Ctrl Pts',(-23.73729861722,-73.2081592380516,-214.410920190191));
#224733=CARTESIAN_POINT('Ctrl Pts',(-23.5663025513546,-73.2116265266727,
-214.42922541616));
#224734=CARTESIAN_POINT('Ctrl Pts',(-22.8928093732761,-73.2252829533333,
-214.501323243384));
#224735=CARTESIAN_POINT('Ctrl Pts',(-22.2169419775558,-73.2387551891486,
-214.550192391158));
#224736=CARTESIAN_POINT('Ctrl Pts',(-21.5429340824075,-73.2520260634925,
-214.571593675925));
#224737=CARTESIAN_POINT('Ctrl Pts',(-20.2344232034334,-73.2777899804694,
-214.613141874609));
#224738=CARTESIAN_POINT('Ctrl Pts',(-18.9179325307332,-73.3030987781156,
-214.549221422764));
#224739=CARTESIAN_POINT('Ctrl Pts',(-17.6290654905074,-73.3276542359699,
-214.365597122485));
#224740=CARTESIAN_POINT('Ctrl Pts',(-17.3112709393207,-73.333708848637,
-214.320321077499));
#224741=CARTESIAN_POINT('Ctrl Pts',(-16.9943207454879,-73.3397323820754,
-214.267877114593));
#224742=CARTESIAN_POINT('Ctrl Pts',(-16.6776489964845,-73.3457377633419,
-214.208133599092));
#224743=CARTESIAN_POINT('Ctrl Pts',(-16.5202984040686,-73.348721769029,
-214.178447725354));
#224744=CARTESIAN_POINT('Ctrl Pts',(-16.3630167155269,-73.3517012823133,
-214.14695825813));
#224745=CARTESIAN_POINT('Ctrl Pts',(-16.2057362493982,-73.3546778160574,
-214.113641116658));
#224746=CARTESIAN_POINT('Ctrl Pts',(-16.1285703446302,-73.3561381812577,
-214.097294856825));
#224747=CARTESIAN_POINT('Ctrl Pts',(-16.0540481310187,-73.3575478723989,
-214.081112834302));
#224748=CARTESIAN_POINT('Ctrl Pts',(-15.9707337467274,-73.3591230654466,
-214.062497710563));
#224749=CARTESIAN_POINT('Ctrl Pts',(-15.9510424824022,-73.3594953606143,
-214.058098046266));
#224750=CARTESIAN_POINT('Ctrl Pts',(-15.9307720996078,-73.3598788385264,
-214.053523320411));
#224751=CARTESIAN_POINT('Ctrl Pts',(-15.9108326277847,-73.360255350698,
-214.049031142856));
#224752=CARTESIAN_POINT('Ctrl Pts',(-15.8886047025696,-73.3606750751755,
-214.044023398034));
#224753=CARTESIAN_POINT('Ctrl Pts',(-15.866490646101,-73.3610912795177,
-214.039079884622));
#224754=CARTESIAN_POINT('Ctrl Pts',(-15.8444879208456,-73.3615040573541,
-214.034198614662));
#224755=CARTESIAN_POINT('Ctrl Pts',(-15.7996818915998,-73.3623446321283,
-214.02425846761));
#224756=CARTESIAN_POINT('Ctrl Pts',(-15.7553375620968,-73.363170999314,
-214.014576371314));
#224757=CARTESIAN_POINT('Ctrl Pts',(-15.7114332100267,-73.363983929539,
-214.005136319819));
#224758=CARTESIAN_POINT('Ctrl Pts',(-14.8755074705471,-73.3794618780206,
-213.825400561189));
#224759=CARTESIAN_POINT('Ctrl Pts',(-14.200932295193,-73.3903009570716,
-213.725936317316));
#224760=CARTESIAN_POINT('Ctrl Pts',(-13.5220442722281,-73.4002664906795,
-213.649153708601));
#224761=CARTESIAN_POINT('Ctrl Pts',(-12.0023561450994,-73.4225742978466,
-213.477276145754));
#224762=CARTESIAN_POINT('Ctrl Pts',(-10.4375864502759,-73.4395813172516,
-213.449904713926));
#224763=CARTESIAN_POINT('Ctrl Pts',(-8.89412533715207,-73.4506496059436,
-213.554697369729));
#224764=CARTESIAN_POINT('Ctrl Pts',(-8.27388677673257,-73.455097388519,
-213.596808211022));
#224765=CARTESIAN_POINT('Ctrl Pts',(-7.65474848612153,-73.4586193936194,
-213.660275636283));
#224766=CARTESIAN_POINT('Ctrl Pts',(-7.03950648809697,-73.4612182559598,
-213.744499693054));
#224767=CARTESIAN_POINT('Ctrl Pts',(-6.8607698195727,-73.4619732629297,
-213.768967995552));
#224768=CARTESIAN_POINT('Ctrl Pts',(-6.68268475627248,-73.4626454086591,
-213.795231774059));
#224769=CARTESIAN_POINT('Ctrl Pts',(-6.51891006801078,-73.4632010570914,
-213.820863067777));
#224770=CARTESIAN_POINT('Ctrl Pts',(-6.06764672989509,-73.4647320859033,
-213.89148730945));
#224771=CARTESIAN_POINT('Ctrl Pts',(-5.69298242973501,-73.4655622034381,
-213.960560234722));
#224772=CARTESIAN_POINT('Ctrl Pts',(-5.3308760600164,-73.4660981256226,
-214.03375600607));
#224773=CARTESIAN_POINT('Ctrl Pts',(-5.31850955169774,-73.4661164282173,
-214.036255758051));
#224774=CARTESIAN_POINT('Ctrl Pts',(-5.30615791932013,-73.4661343368019,
-214.038761469138));
#224775=CARTESIAN_POINT('Ctrl Pts',(-5.29381864882765,-73.4661518572792,
-214.041273601485));
#224776=CARTESIAN_POINT('Ctrl Pts',(-5.2815968807776,-73.4661692109154,
-214.043761811699));
#224777=CARTESIAN_POINT('Ctrl Pts',(-5.26938778610787,-73.466186132111,
-214.046259128319));
#224778=CARTESIAN_POINT('Ctrl Pts',(-5.25718718520783,-73.4662027904425,
-214.04875708583));
#224779=CARTESIAN_POINT('Ctrl Pts',(-5.23494474483045,-73.4662331595979,
-214.053311014891));
#224780=CARTESIAN_POINT('Ctrl Pts',(-5.2127240106781,-73.466263272517,-214.05783355763));
#224781=CARTESIAN_POINT('Ctrl Pts',(-5.19051019778499,-73.4662931515064,
-214.062327747256));
#224782=CARTESIAN_POINT('Ctrl Pts',(-5.1460600974665,-73.4663529397149,
-214.071320673444));
#224783=CARTESIAN_POINT('Ctrl Pts',(-5.10163770420206,-73.4664117924303,
-214.080200219155));
#224784=CARTESIAN_POINT('Ctrl Pts',(-5.05712471353571,-73.4664698739798,
-214.088988919222));
#224785=CARTESIAN_POINT('Ctrl Pts',(-4.96883161704773,-73.4665850807942,
-214.106421617664));
#224786=CARTESIAN_POINT('Ctrl Pts',(-4.88018237053404,-73.4666972705213,
-214.123499182983));
#224787=CARTESIAN_POINT('Ctrl Pts',(-4.79025277101939,-73.4668075128244,
-214.140369998645));
#224788=CARTESIAN_POINT('Ctrl Pts',(-4.61905021585963,-73.4670173854812,
-214.172487641383));
#224789=CARTESIAN_POINT('Ctrl Pts',(-4.44321791793865,-73.4672204138825,
-214.203890324126));
#224790=CARTESIAN_POINT('Ctrl Pts',(-4.25629393769659,-73.4674212578825,
-214.235206565164));
#224791=CARTESIAN_POINT('Ctrl Pts',(-3.64983483109652,-73.4680728793205,
-214.336809470994));
#224792=CARTESIAN_POINT('Ctrl Pts',(-2.86106847301697,-73.4687282647771,
-214.442238213622));
#224793=CARTESIAN_POINT('Ctrl Pts',(-2.12288746980912,-73.4691288002137,
-214.503638101334));
#224794=CARTESIAN_POINT('Ctrl Pts',(-1.42250617613227,-73.4695088256087,
-214.561893912038));
#224795=CARTESIAN_POINT('Ctrl Pts',(-0.720121136870457,-73.4697481762702,
-214.589437542788));
#224796=CARTESIAN_POINT('Ctrl Pts',(-9.73630898126743E-13,-73.4697481762702,
-214.589437542788));
#224797=CARTESIAN_POINT('Ctrl Pts',(0.702421357999057,-73.4697481762702,
-214.589437542788));
#224798=CARTESIAN_POINT('Ctrl Pts',(1.40882352807894,-73.4695162472501,
-214.563032076116));
#224799=CARTESIAN_POINT('Ctrl Pts',(2.12288573821906,-73.4691288005736,
-214.503638278573));
#224800=CARTESIAN_POINT('Ctrl Pts',(2.75005748515334,-73.4687885002392,
-214.451471798912));
#224801=CARTESIAN_POINT('Ctrl Pts',(3.40090625139601,-73.4682792287222,
-214.369727571729));
#224802=CARTESIAN_POINT('Ctrl Pts',(3.92541310539679,-73.4677620863878,
-214.288535941429));
#224803=CARTESIAN_POINT('Ctrl Pts',(4.03901420267087,-73.467650080346,-214.270950931393));
#224804=CARTESIAN_POINT('Ctrl Pts',(4.14897936068259,-73.4675365646685,
-214.253185445256));
#224805=CARTESIAN_POINT('Ctrl Pts',(4.2562950728238,-73.4674212570593,-214.23520635228));
#224806=CARTESIAN_POINT('Ctrl Pts',(4.44044509701261,-73.467223393218,-214.204354854951));
#224807=CARTESIAN_POINT('Ctrl Pts',(4.61680175851431,-73.4670201417657,
-214.172909458352));
#224808=CARTESIAN_POINT('Ctrl Pts',(4.79025315005858,-73.4668075122857,
-214.140369931774));
#224809=CARTESIAN_POINT('Ctrl Pts',(4.87976449140688,-73.4666977826965,
-214.123577580643));
#224810=CARTESIAN_POINT('Ctrl Pts',(4.96850006460584,-73.4665855133531,
-214.106487083431));
#224811=CARTESIAN_POINT('Ctrl Pts',(5.05712477774532,-73.4664698738595,
-214.088988908638));
#224812=CARTESIAN_POINT('Ctrl Pts',(5.10158648516536,-73.4664118592364,
-214.080210333221));
#224813=CARTESIAN_POINT('Ctrl Pts',(5.14602026857021,-73.4663529932743,
-214.07132873217));
#224814=CARTESIAN_POINT('Ctrl Pts',(5.19051019684309,-73.4662931515016,
-214.06232774779));
#224815=CARTESIAN_POINT('Ctrl Pts',(5.2127183722053,-73.4662632800985,-214.057834698525));
#224816=CARTESIAN_POINT('Ctrl Pts',(5.23494054055089,-73.4662331653379,
-214.053311875695));
#224817=CARTESIAN_POINT('Ctrl Pts',(5.25718718445785,-73.4662027904434,
-214.048757085989));
#224818=CARTESIAN_POINT('Ctrl Pts',(5.26938721880819,-73.4661861328855,
-214.046259244468));
#224819=CARTESIAN_POINT('Ctrl Pts',(5.28159655675219,-73.4661692113754,
-214.043761877671));
#224820=CARTESIAN_POINT('Ctrl Pts',(5.2938186488238,-73.4661518572791,-214.04127360149));
#224821=CARTESIAN_POINT('Ctrl Pts',(5.30615807585072,-73.4661343365795,
-214.038761437274));
#224822=CARTESIAN_POINT('Ctrl Pts',(5.31850995238531,-73.4661164276243,
-214.036255677061));
#224823=CARTESIAN_POINT('Ctrl Pts',(5.33087606001262,-73.4660981256225,
-214.033756006075));
#224824=CARTESIAN_POINT('Ctrl Pts',(5.69862312937633,-73.4655538551284,
-213.959420030091));
#224825=CARTESIAN_POINT('Ctrl Pts',(6.07882234604323,-73.4646941697047,
-213.889738287654));
#224826=CARTESIAN_POINT('Ctrl Pts',(6.51891006800735,-73.4632010570914,
-213.820863067781));
#224827=CARTESIAN_POINT('Ctrl Pts',(7.07951671635194,-73.4612990525228,
-213.733126227511));
#224828=CARTESIAN_POINT('Ctrl Pts',(7.74704151965693,-73.4581513210782,
-213.649508682059));
#224829=CARTESIAN_POINT('Ctrl Pts',(8.38225235563468,-73.4541123126368,
-213.594313827671));
#224830=CARTESIAN_POINT('Ctrl Pts',(8.55274426588832,-73.4530282343659,
-213.579499413892));
#224831=CARTESIAN_POINT('Ctrl Pts',(8.72338814746169,-73.4518739766063,
-213.566289500818));
#224832=CARTESIAN_POINT('Ctrl Pts',(8.89412533714898,-73.4506496059436,
-213.55469736973));
#224833=CARTESIAN_POINT('Ctrl Pts',(10.4367821614907,-73.4395870848738,
-213.449959320781));
#224834=CARTESIAN_POINT('Ctrl Pts',(11.9885581120666,-73.4227768419441,
-213.47571558063));
#224835=CARTESIAN_POINT('Ctrl Pts',(13.5220442722263,-73.4002664906795,
-213.649153708599));
#224836=CARTESIAN_POINT('Ctrl Pts',(14.3005224069512,-73.3888390538237,
-213.737200013717));
#224837=CARTESIAN_POINT('Ctrl Pts',(15.1211380770204,-73.374913797141,-213.878214586776));
#224838=CARTESIAN_POINT('Ctrl Pts',(15.711433210026,-73.3639839295391,-214.005136319814));
#224839=CARTESIAN_POINT('Ctrl Pts',(15.7565784132858,-73.3631480237914,
-214.014843171719));
#224840=CARTESIAN_POINT('Ctrl Pts',(15.8008882476979,-73.3623220005201,
-214.024526095807));
#224841=CARTESIAN_POINT('Ctrl Pts',(15.8444879208452,-73.3615040573542,
-214.034198614657));
#224842=CARTESIAN_POINT('Ctrl Pts',(15.8667829643265,-73.3610857955387,
-214.039144734955));
#224843=CARTESIAN_POINT('Ctrl Pts',(15.8888923011116,-73.3606696445225,
-214.044088191306));
#224844=CARTESIAN_POINT('Ctrl Pts',(15.9108326277843,-73.360255350698,-214.049031142851));
#224845=CARTESIAN_POINT('Ctrl Pts',(15.9309288957193,-73.3598758777838,
-214.053558645112));
#224846=CARTESIAN_POINT('Ctrl Pts',(15.95088806449,-73.3594982801345,-214.058063544314));
#224847=CARTESIAN_POINT('Ctrl Pts',(15.9707337467294,-73.3591230654467,
-214.062497710559));
#224848=CARTESIAN_POINT('Ctrl Pts',(16.0506907171643,-73.3576113497325,
-214.080362679629));
#224849=CARTESIAN_POINT('Ctrl Pts',(16.1287529786783,-73.3561347249074,
-214.097333544679));
#224850=CARTESIAN_POINT('Ctrl Pts',(16.2057362493999,-73.3546778160574,
-214.113641116654));
#224851=CARTESIAN_POINT('Ctrl Pts',(16.3652674515949,-73.3516586871201,
-214.147435037562));
#224852=CARTESIAN_POINT('Ctrl Pts',(16.5201573269693,-73.3487244444233,
-214.178421109645));
#224853=CARTESIAN_POINT('Ctrl Pts',(16.6776489964862,-73.3457377633419,
-214.208133599088));
#224854=CARTESIAN_POINT('Ctrl Pts',(16.9698848482653,-73.3401957858362,
-214.263267020986));
#224855=CARTESIAN_POINT('Ctrl Pts',(17.2708194530509,-73.3344795291924,
-214.314557972668));
#224856=CARTESIAN_POINT('Ctrl Pts',(17.6290654905084,-73.3276542359699,
-214.365597122482));
#224857=CARTESIAN_POINT('Ctrl Pts',(18.0016463094319,-73.3205558369025,
-214.418678542084));
#224858=CARTESIAN_POINT('Ctrl Pts',(18.4365382335761,-73.3122584971473,
-214.472002564731));
#224859=CARTESIAN_POINT('Ctrl Pts',(18.9898749871452,-73.3016297273226,
-214.515254103018));
#224860=CARTESIAN_POINT('Ctrl Pts',(19.5172859611096,-73.2914989528728,
-214.556479154104));
#224861=CARTESIAN_POINT('Ctrl Pts',(20.0662563549184,-73.280892719631,-214.579525909555));
#224862=CARTESIAN_POINT('Ctrl Pts',(20.6050328168092,-73.2703945802866,
-214.583321183555));
#224863=CARTESIAN_POINT('Ctrl Pts',(20.9172357412455,-73.2643112599556,
-214.585520417792));
#224864=CARTESIAN_POINT('Ctrl Pts',(21.2297201296423,-73.2581930877065,
-214.581538931826));
#224865=CARTESIAN_POINT('Ctrl Pts',(21.5429340824073,-73.2520260634924,
-214.571593675926));
#224866=CARTESIAN_POINT('Ctrl Pts',(22.2161471553522,-73.2387708387955,
-214.550217628573));
#224867=CARTESIAN_POINT('Ctrl Pts',(22.8929026451804,-73.2252810620581,
-214.501313258575));
#224868=CARTESIAN_POINT('Ctrl Pts',(23.566302551354,-73.2116265266727,-214.429225416162));
#224869=CARTESIAN_POINT('Ctrl Pts',(23.7340873546836,-73.2082243528482,
-214.411263957672));
#224870=CARTESIAN_POINT('Ctrl Pts',(23.9005400109352,-73.2048355955593,
-214.392070604889));
#224871=CARTESIAN_POINT('Ctrl Pts',(24.0786937902351,-73.2011908763299,
-214.369933459424));
#224872=CARTESIAN_POINT('Ctrl Pts',(24.1624301494928,-73.1994777747612,
-214.359528493708));
#224873=CARTESIAN_POINT('Ctrl Pts',(24.2481278545952,-73.1977206997215,
-214.348534146447));
#224874=CARTESIAN_POINT('Ctrl Pts',(24.3357827357377,-73.1959190376298,
-214.336909622655));
#224875=CARTESIAN_POINT('Ctrl Pts',(24.3782426834008,-73.1950463140904,
-214.331278713511));
#224876=CARTESIAN_POINT('Ctrl Pts',(24.4211619094295,-73.1941631267963,
-214.325499931626));
#224877=CARTESIAN_POINT('Ctrl Pts',(24.4645402940559,-73.1932693935819,
-214.319568588463));
#224878=CARTESIAN_POINT('Ctrl Pts',(24.4752493247181,-73.1930487533603,
-214.318104289219));
#224879=CARTESIAN_POINT('Ctrl Pts',(24.4859863412596,-73.1928274703479,
-214.316630691588));
#224880=CARTESIAN_POINT('Ctrl Pts',(24.4967513448978,-73.1926055432136,
-214.315147724591));
#224881=CARTESIAN_POINT('Ctrl Pts',(24.5076725708397,-73.1923803954608,
-214.313643236697));
#224882=CARTESIAN_POINT('Ctrl Pts',(24.5186222445091,-73.1921546437477,
-214.312126198923));
#224883=CARTESIAN_POINT('Ctrl Pts',(24.5296015630537,-73.1919280895696,
-214.310606246885));
#224884=CARTESIAN_POINT('Ctrl Pts',(24.5536847868459,-73.1914311411526,
-214.307272219828));
#224885=CARTESIAN_POINT('Ctrl Pts',(24.5779134331013,-73.1909298720015,
-214.303946818507));
#224886=CARTESIAN_POINT('Ctrl Pts',(24.6022876971452,-73.1904242292317,
-214.300631104617));
#224887=CARTESIAN_POINT('Ctrl Pts',(24.954073049667,-73.1831264614014,-214.252776548783));
#224888=CARTESIAN_POINT('Ctrl Pts',(25.3362127923774,-73.1749198351962,
-214.206868205789));
#224889=CARTESIAN_POINT('Ctrl Pts',(25.7490556660367,-73.1656334354033,
-214.166565463302));
#224890=CARTESIAN_POINT('Ctrl Pts',(26.6546937674681,-73.1452622045691,
-214.07815483176));
#224891=CARTESIAN_POINT('Ctrl Pts',(27.7073087536273,-73.1198009845544,
-214.013625094252));
#224892=CARTESIAN_POINT('Ctrl Pts',(28.9155236124462,-73.0866210775832,
-214.033403996694));
#224893=CARTESIAN_POINT('Ctrl Pts',(29.2736562011569,-73.0767860669558,
-214.039266753208));
#224894=CARTESIAN_POINT('Ctrl Pts',(29.6479283148488,-73.0661922065524,
-214.052970868027));
#224895=CARTESIAN_POINT('Ctrl Pts',(30.0308162541926,-73.0549738991023,
-214.076522056359));
#224896=CARTESIAN_POINT('Ctrl Pts',(31.1936395115523,-73.0209041166128,
-214.148046559264));
#224897=CARTESIAN_POINT('Ctrl Pts',(32.3571796024045,-72.9833988359979,
-214.303881516735));
#224898=CARTESIAN_POINT('Ctrl Pts',(33.4888960070749,-72.9429805807943,
-214.578360966074));
#224899=CARTESIAN_POINT('',(21.0035817852092,-61.2574554370328,-232.850037376712));
#224900=CARTESIAN_POINT('Ctrl Pts',(21.0035817852092,-61.2574554370328,
-232.850037376712));
#224901=CARTESIAN_POINT('Ctrl Pts',(21.507201965559,-61.7327572754185,-232.106553581838));
#224902=CARTESIAN_POINT('Ctrl Pts',(22.0340605092179,-62.2294925524995,
-231.329524302083));
#224903=CARTESIAN_POINT('Ctrl Pts',(22.584297728091,-62.7476944804053,-230.518968394386));
#224904=CARTESIAN_POINT('Ctrl Pts',(23.0070557094251,-63.1458391232079,
-229.896202489894));
#224905=CARTESIAN_POINT('Ctrl Pts',(23.4436140473167,-63.556655839147,-229.253645314622));
#224906=CARTESIAN_POINT('Ctrl Pts',(23.8940180431183,-63.9801538708211,
-228.59129617684));
#224907=CARTESIAN_POINT('Ctrl Pts',(24.4123301828051,-64.4675033903552,
-227.829083580983));
#224908=CARTESIAN_POINT('Ctrl Pts',(24.9489959478791,-64.9716496124015,
-227.040665559205));
#224909=CARTESIAN_POINT('Ctrl Pts',(25.5041662984108,-65.4925976086513,
-226.226043613375));
#224910=CARTESIAN_POINT('Ctrl Pts',(25.7817514736766,-65.7530716067762,
-225.81873264046));
#224911=CARTESIAN_POINT('Ctrl Pts',(26.0639634999476,-66.0177457474341,
-225.404870543246));
#224912=CARTESIAN_POINT('Ctrl Pts',(26.3508255150318,-66.2866181925986,
-224.984456238475));
#224913=CARTESIAN_POINT('Ctrl Pts',(26.4942565225739,-66.4210544151808,
-224.774249086089));
#224914=CARTESIAN_POINT('Ctrl Pts',(26.6388500325804,-66.5565401775674,
-224.562403862182));
#224915=CARTESIAN_POINT('Ctrl Pts',(26.7846092496479,-66.693075046961,-224.348920320831));
#224916=CARTESIAN_POINT('Ctrl Pts',(26.8574888581816,-66.7613424816577,
-224.242178550156));
#224917=CARTESIAN_POINT('Ctrl Pts',(26.9306598938017,-66.8298721904186,
-224.135027198621));
#224918=CARTESIAN_POINT('Ctrl Pts',(27.0041227667667,-66.8986641033831,
-224.027466226649));
#224919=CARTESIAN_POINT('Ctrl Pts',(27.0408542032493,-66.9330600598653,
-223.973685740662));
#224920=CARTESIAN_POINT('Ctrl Pts',(27.0776585990868,-66.9675215672189,
-223.919802849465));
#224921=CARTESIAN_POINT('Ctrl Pts',(27.1145360066284,-67.0020486157321,
-223.865817547554));
#224922=CARTESIAN_POINT('Ctrl Pts',(27.1468037382272,-67.0322597831812,
-223.818580408381));
#224923=CARTESIAN_POINT('Ctrl Pts',(27.1791273694131,-67.0625211305701,
-223.771264861001));
#224924=CARTESIAN_POINT('Ctrl Pts',(27.2115069356365,-67.0928326509612,
-223.723870901481));
#224925=CARTESIAN_POINT('Ctrl Pts',(27.2161325879541,-67.09716286816,-223.717100335835));
#224926=CARTESIAN_POINT('Ctrl Pts',(27.221744269903,-67.1024160746729,-223.708886619672));
#224927=CARTESIAN_POINT('Ctrl Pts',(27.2253873172964,-67.1058263743519,
-223.703554403788));
#224928=CARTESIAN_POINT('Ctrl Pts',(27.2955613340804,-67.1715171000192,
-223.600842864093));
#224929=CARTESIAN_POINT('Ctrl Pts',(27.3660468581061,-67.2374900781918,
-223.497689857422));
#224930=CARTESIAN_POINT('Ctrl Pts',(27.4368442106614,-67.3037452399979,
-223.394095310731));
#224931=CARTESIAN_POINT('Ctrl Pts',(28.1054064990158,-67.9294141526563,
-222.415818515097));
#224932=CARTESIAN_POINT('Ctrl Pts',(28.8017874464413,-68.5802721850816,
-221.398191038935));
#224933=CARTESIAN_POINT('Ctrl Pts',(29.526328713446,-69.2563390389742,-220.341246127668));
#224934=CARTESIAN_POINT('Ctrl Pts',(30.1857768193341,-69.8716676980254,
-219.379257692358));
#224935=CARTESIAN_POINT('Ctrl Pts',(30.868552817987,-70.5078791976191,-218.384699241817));
#224936=CARTESIAN_POINT('Ctrl Pts',(31.5748931285518,-71.1649718599665,
-217.357564074703));
#224937=CARTESIAN_POINT('Ctrl Pts',(32.1946991469904,-71.7415635972682,
-216.456264023148));
#224938=CARTESIAN_POINT('Ctrl Pts',(32.8326493021217,-72.3342334965497,
-215.529880154047));
#224939=CARTESIAN_POINT('Ctrl Pts',(33.4888861408047,-72.9429671618309,
-214.578382767941));
#224940=CARTESIAN_POINT('',(20.3871357022548,-61.1221564407624,-232.850041788804));
#224941=CARTESIAN_POINT('Ctrl Pts',(20.3871899404023,-61.1221588841747,
-232.85005));
#224942=CARTESIAN_POINT('Ctrl Pts',(20.4903351182918,-61.1426979252128,
-232.85005));
#224943=CARTESIAN_POINT('Ctrl Pts',(20.5932743876311,-61.1642481051802,
-232.850050000001));
#224944=CARTESIAN_POINT('Ctrl Pts',(20.7987564077365,-61.2093548950276,
-232.850050000001));
#224945=CARTESIAN_POINT('Ctrl Pts',(20.9012901690195,-61.2329102063449,
-232.85005));
#224946=CARTESIAN_POINT('Ctrl Pts',(21.0035920114962,-61.2574518715881,
-232.85005));
#224947=CARTESIAN_POINT('',(13.6391777675809,-61.2898273935358,-232.85005));
#224948=CARTESIAN_POINT('Ctrl Pts',(13.6391777675808,-61.2898273935357,
-232.85005));
#224949=CARTESIAN_POINT('Ctrl Pts',(13.7679778534055,-61.2872620754521,
-232.820255967491));
#224950=CARTESIAN_POINT('Ctrl Pts',(13.8962943901741,-61.2846700045695,
-232.788034396798));
#224951=CARTESIAN_POINT('Ctrl Pts',(14.0579979554195,-61.2813584495603,
-232.744562636335));
#224952=CARTESIAN_POINT('Ctrl Pts',(14.0841407462284,-61.2808208278271,
-232.737348171446));
#224953=CARTESIAN_POINT('Ctrl Pts',(14.1136793541503,-61.2802122861796,
-232.729268530917));
#224954=CARTESIAN_POINT('Ctrl Pts',(14.1196218852399,-61.2800897833605,
-232.727647117922));
#224955=CARTESIAN_POINT('Ctrl Pts',(14.1382345388739,-61.2797058487444,
-232.72258133054));
#224956=CARTESIAN_POINT('Ctrl Pts',(14.1509054406719,-61.2794441266197,
-232.719151061028));
#224957=CARTESIAN_POINT('Ctrl Pts',(14.3680771090753,-61.2749523319826,
-232.660673210438));
#224958=CARTESIAN_POINT('Ctrl Pts',(14.5738916280709,-61.2706036847836,
-232.610036215021));
#224959=CARTESIAN_POINT('Ctrl Pts',(15.5130869595282,-61.2503314810904,
-232.401689231487));
#224960=CARTESIAN_POINT('Ctrl Pts',(16.2652400909217,-61.2328950900081,
-232.297341076677));
#224961=CARTESIAN_POINT('Ctrl Pts',(17.5574155716905,-61.2007887070003,
-232.254652621959));
#224962=CARTESIAN_POINT('Ctrl Pts',(18.1075672352859,-61.1864563064502,
-232.278708928573));
#224963=CARTESIAN_POINT('Ctrl Pts',(18.9473592855207,-61.1635855249077,
-232.402122405498));
#224964=CARTESIAN_POINT('Ctrl Pts',(19.2463100800112,-61.1552436964812,
-232.463744244733));
#224965=CARTESIAN_POINT('Ctrl Pts',(19.8287142286265,-61.1386226678887,
-232.626250777395));
#224966=CARTESIAN_POINT('Ctrl Pts',(20.1129420847393,-61.1303255101922,
-232.726867615163));
#224967=CARTESIAN_POINT('Ctrl Pts',(20.3871350980681,-61.1221605172865,
-232.850025366413));
#224968=CARTESIAN_POINT('',(10.1856061283693,-61.3499012171702,-232.85005));
#224969=CARTESIAN_POINT('Ctrl Pts',(10.1856061283695,-61.3499012171691,
-232.85005));
#224970=CARTESIAN_POINT('Ctrl Pts',(10.7540331802441,-61.4387873154263,
-232.85005));
#224971=CARTESIAN_POINT('Ctrl Pts',(11.3321672515837,-61.4795692676092,
-232.85005));
#224972=CARTESIAN_POINT('Ctrl Pts',(12.4893568167562,-61.4603506902607,
-232.85005));
#224973=CARTESIAN_POINT('Ctrl Pts',(13.0690230887892,-61.4003891841391,
-232.85005));
#224974=CARTESIAN_POINT('Ctrl Pts',(13.6391777675808,-61.2898273935355,
-232.85005));
#224975=CARTESIAN_POINT('',(8.46314246804488,-61.3733482641976,-232.250044026166));
#224976=CARTESIAN_POINT('Ctrl Pts',(10.1856061283698,-61.3499012171704,
-232.850049999998));
#224977=CARTESIAN_POINT('Ctrl Pts',(9.82032687378921,-61.3553338539534,
-232.743373739325));
#224978=CARTESIAN_POINT('Ctrl Pts',(9.60751931165371,-61.3583117635075,
-232.640308531512));
#224979=CARTESIAN_POINT('Ctrl Pts',(9.04581817610225,-61.3659623843548,
-232.420098274378));
#224980=CARTESIAN_POINT('Ctrl Pts',(8.75670787170129,-61.3697245641445,
-232.326864869009));
#224981=CARTESIAN_POINT('Ctrl Pts',(8.46321410432618,-61.3733513183578,
-232.25005));
#224982=CARTESIAN_POINT('Ctrl Pts',(3.75861965563843,-61.4153243588596,
-232.25005));
#224983=CARTESIAN_POINT('Ctrl Pts',(4.5340023135914,-61.2869672909125,-232.25005));
#224984=CARTESIAN_POINT('Ctrl Pts',(5.31762015306685,-61.2192576556064,
-232.250049999968));
#224985=CARTESIAN_POINT('Ctrl Pts',(6.89317806954359,-61.2051427085062,
-232.250049999968));
#224986=CARTESIAN_POINT('Ctrl Pts',(7.68215656537121,-61.2596528397479,
-232.25005));
#224987=CARTESIAN_POINT('Ctrl Pts',(8.463139272608,-61.3733404249266,-232.25005));
#224988=CARTESIAN_POINT('Ctrl Pts',(24.1738391241342,37.0431280107547,-233.208100039793));
#224989=CARTESIAN_POINT('Ctrl Pts',(27.6162083218107,41.0700375551415,-226.588760311268));
#224990=CARTESIAN_POINT('Ctrl Pts',(31.0681786417009,45.0961310980358,-219.973963300133));
#224991=CARTESIAN_POINT('Ctrl Pts',(34.5233304970369,49.1218089274639,-213.360583123942));
#224992=CARTESIAN_POINT('Ctrl Pts',(21.9374099124571,36.8211293809628,-233.1017016503));
#224993=CARTESIAN_POINT('Ctrl Pts',(25.111743736431,40.8399102882666,-226.485020448574));
#224994=CARTESIAN_POINT('Ctrl Pts',(28.2953870757527,44.857120760978,-219.871880044709));
#224995=CARTESIAN_POINT('Ctrl Pts',(31.4821075812935,48.8736850008129,-213.259832488631));
#224996=CARTESIAN_POINT('Ctrl Pts',(19.6791533800966,36.9243838380731,-233.031259797898));
#224997=CARTESIAN_POINT('Ctrl Pts',(22.5835629262214,40.9731440158751,-226.416479441913));
#224998=CARTESIAN_POINT('Ctrl Pts',(25.4972748241131,45.0198316409588,-219.804613185821));
#224999=CARTESIAN_POINT('Ctrl Pts',(28.4139919192639,49.0657183803849,-213.193598354232));
#225000=CARTESIAN_POINT('Ctrl Pts',(17.5054530978035,37.329644059109,-232.985683121183));
#225001=CARTESIAN_POINT('Ctrl Pts',(20.1305665853578,41.4552389705233,-226.372636955178));
#225002=CARTESIAN_POINT('Ctrl Pts',(22.7661343835796,45.5778704773325,-219.761939447884));
#225003=CARTESIAN_POINT('Ctrl Pts',(25.4048641344257,49.6994667549787,-213.151865731098));
#225004=CARTESIAN_POINT('Ctrl Pts',(17.2337405625169,37.3803015867384,-232.979986036594));
#225005=CARTESIAN_POINT('Ctrl Pts',(19.8239420427498,41.5155008398544,-226.367156644337));
#225006=CARTESIAN_POINT('Ctrl Pts',(22.4247418285129,45.6476253318793,-219.756605230642));
#225007=CARTESIAN_POINT('Ctrl Pts',(25.0287231613209,49.7786853018029,-213.146649153206));
#225008=CARTESIAN_POINT('Ctrl Pts',(16.9633432334929,37.4356224487032,-232.97468748568));
#225009=CARTESIAN_POINT('Ctrl Pts',(19.518484591489,41.5811860530679,-226.362072247411));
#225010=CARTESIAN_POINT('Ctrl Pts',(22.0843912488166,45.7235559153002,-219.751665537454));
#225011=CARTESIAN_POINT('Ctrl Pts',(24.6535036963345,49.8648302271687,-213.141825886988));
#225012=CARTESIAN_POINT('Ctrl Pts',(16.6944159673799,37.4955299722126,-232.969765709419));
#225013=CARTESIAN_POINT('Ctrl Pts',(19.2143590590312,41.6522508528778,-226.357368433448));
#225014=CARTESIAN_POINT('Ctrl Pts',(21.7452541089279,45.8056509057175,-219.747108569133));
#225015=CARTESIAN_POINT('Ctrl Pts',(24.2793821656715,49.9579228935011,-213.137386917182));
#225016=CARTESIAN_POINT('Ctrl Pts',(16.5599523343234,37.5254837339673,-232.967304821289));
#225017=CARTESIAN_POINT('Ctrl Pts',(19.0622962928022,41.6877832527827,-226.355016526466));
#225018=CARTESIAN_POINT('Ctrl Pts',(21.5756855389835,45.8466984009262,-219.744830084973));
#225019=CARTESIAN_POINT('Ctrl Pts',(24.09232140034,50.0044692266673,-213.135167432279));
#225020=CARTESIAN_POINT('Ctrl Pts',(16.4258562209343,37.5565842202126,-232.964938221388));
#225021=CARTESIAN_POINT('Ctrl Pts',(18.9105665123802,41.7246605912085,-226.352759839903));
#225022=CARTESIAN_POINT('Ctrl Pts',(21.4064203345213,45.8892870285343,-219.742647341783));
#225023=CARTESIAN_POINT('Ctrl Pts',(23.9055351228988,50.0527525170248,-213.133044069172));
#225024=CARTESIAN_POINT('Ctrl Pts',(16.2921470072812,37.5888221841555,-232.962663752566));
#225025=CARTESIAN_POINT('Ctrl Pts',(18.7591903623818,41.7628776356138,-226.35059690245));
#225026=CARTESIAN_POINT('Ctrl Pts',(21.2374799657885,45.9334155456487,-219.740559220295));
#225027=CARTESIAN_POINT('Ctrl Pts',(23.7190454157132,50.1027755574024,-213.131015984566));
#225028=CARTESIAN_POINT('Ctrl Pts',(16.2252924004546,37.6049411661268,-232.961526518156));
#225029=CARTESIAN_POINT('Ctrl Pts',(18.6835022873825,41.7819861578165,-226.349515433724));
#225030=CARTESIAN_POINT('Ctrl Pts',(21.1530097814222,45.9554798042059,-219.739515159551));
#225031=CARTESIAN_POINT('Ctrl Pts',(23.6258005621204,50.1277870775912,-213.130001942264));
#225032=CARTESIAN_POINT('Ctrl Pts',(16.1585345187945,37.6213445208979,-232.96041232234));
#225033=CARTESIAN_POINT('Ctrl Pts',(18.607902620454,41.8014296088707,-226.348457406886));
#225034=CARTESIAN_POINT('Ctrl Pts',(21.0686208064075,45.9779290368421,-219.738494757914));
#225035=CARTESIAN_POINT('Ctrl Pts',(23.53262985142,50.1532335364878,-213.12901172252));
#225036=CARTESIAN_POINT('Ctrl Pts',(16.0918757861226,37.6380311124284,-232.959320930339));
#225037=CARTESIAN_POINT('Ctrl Pts',(18.5323939450749,41.8212073484617,-226.347422665632));
#225038=CARTESIAN_POINT('Ctrl Pts',(20.9843157271392,46.0007630980888,-219.737497897487));
#225039=CARTESIAN_POINT('Ctrl Pts',(23.4395360459604,50.1791152901554,-213.128045237458));
#225040=CARTESIAN_POINT('Ctrl Pts',(16.0585464197866,37.6463744081936,-232.958775234339));
#225041=CARTESIAN_POINT('Ctrl Pts',(18.4946396073852,41.8310962182573,-226.346905295004));
#225042=CARTESIAN_POINT('Ctrl Pts',(20.942163187505,46.0121801287122,-219.736999467274));
#225043=CARTESIAN_POINT('Ctrl Pts',(23.3929891432306,50.1920561669893,-213.127561994927));
#225044=CARTESIAN_POINT('Ctrl Pts',(16.0340227552118,37.651660998028,-232.959574803646));
#225045=CARTESIAN_POINT('Ctrl Pts',(18.4657919650916,41.8377973386214,-226.347688324445));
#225046=CARTESIAN_POINT('Ctrl Pts',(20.9089874042012,46.0203250376801,-219.737774455135));
#225047=CARTESIAN_POINT('Ctrl Pts',(23.3554742352741,50.2016574692251,-213.128330340674));
#225048=CARTESIAN_POINT('Ctrl Pts',(16.0065882955589,37.6578607887702,-232.959932115556));
#225049=CARTESIAN_POINT('Ctrl Pts',(18.433980532035,41.8454422045226,-226.348044075791));
#225050=CARTESIAN_POINT('Ctrl Pts',(20.8728043396308,46.0294291007631,-219.738131122272));
#225051=CARTESIAN_POINT('Ctrl Pts',(23.3149134039151,50.2122277347419,-213.128687613044));
#225052=CARTESIAN_POINT('Ctrl Pts',(15.9791538359061,37.6640605795124,-232.960289427464));
#225053=CARTESIAN_POINT('Ctrl Pts',(18.4021690989782,41.8530870704238,-226.348399827135));
#225054=CARTESIAN_POINT('Ctrl Pts',(20.8366212750604,46.0385331638461,-219.738487789409));
#225055=CARTESIAN_POINT('Ctrl Pts',(23.2743525725561,50.2227980002586,-213.129044885415));
#225056=CARTESIAN_POINT('Ctrl Pts',(15.9517175466003,37.6701942678452,-232.960648289437));
#225057=CARTESIAN_POINT('Ctrl Pts',(18.3703417060476,41.8606571366407,-226.348757259569));
#225058=CARTESIAN_POINT('Ctrl Pts',(20.8004076106497,46.0475539212133,-219.738846178464));
#225059=CARTESIAN_POINT('Ctrl Pts',(23.2337464674417,50.2332764439494,-213.129403912862));
#225060=CARTESIAN_POINT('Ctrl Pts',(15.9242793293033,37.6762620249318,-232.961008682583));
#225061=CARTESIAN_POINT('Ctrl Pts',(18.3384986904741,41.8681523497137,-226.349116370535));
#225062=CARTESIAN_POINT('Ctrl Pts',(20.7641640754571,46.0564910996168,-219.739206294065));
#225063=CARTESIAN_POINT('Ctrl Pts',(23.1930961992297,50.2436625758447,-213.129764705805));
#225064=CARTESIAN_POINT('Ctrl Pts',(15.4852678525495,37.7733461383171,-232.966774972931));
#225065=CARTESIAN_POINT('Ctrl Pts',(17.8290104412988,41.9880757588812,-226.354862145998));
#225066=CARTESIAN_POINT('Ctrl Pts',(20.1842675123756,46.1994859540735,-219.744968143682));
#225067=CARTESIAN_POINT('Ctrl Pts',(22.542691907838,50.4098406861693,-213.135537392885));
#225068=CARTESIAN_POINT('Ctrl Pts',(15.0457657134741,37.8535630790418,-232.972927812655));
#225069=CARTESIAN_POINT('Ctrl Pts',(17.3155230681897,42.0888383893238,-226.361030538136));
#225070=CARTESIAN_POINT('Ctrl Pts',(19.5967238562187,46.3210799188354,-219.751163746593));
#225071=CARTESIAN_POINT('Ctrl Pts',(21.8809817406798,50.5523768769246,-213.141752862445));
#225072=CARTESIAN_POINT('Ctrl Pts',(14.6053482723449,37.9175430616014,-232.979423896539));
#225073=CARTESIAN_POINT('Ctrl Pts',(16.7994169624042,42.1702102018592,-226.367656683047));
#225074=CARTESIAN_POINT('Ctrl Pts',(19.0045202167024,46.4201832439773,-219.757864926228));
#225075=CARTESIAN_POINT('Ctrl Pts',(21.2125144100672,50.6693289807885,-213.14851265933));
#225076=CARTESIAN_POINT('Ctrl Pts',(13.7245133900865,38.0455030267203,-232.992416064308));
#225077=CARTESIAN_POINT('Ctrl Pts',(15.7672047508334,42.3329538269303,-226.380908972868));
#225078=CARTESIAN_POINT('Ctrl Pts',(17.8201129376698,46.6183898942611,-219.771267285497));
#225079=CARTESIAN_POINT('Ctrl Pts',(19.8755797488418,50.9032331885162,-213.162032253098));
#225080=CARTESIAN_POINT('Ctrl Pts',(12.8410916883673,38.1084776461205,-233.006963660748));
#225081=CARTESIAN_POINT('Ctrl Pts',(14.724086953151,42.4181211429224,-226.395942520899));
#225082=CARTESIAN_POINT('Ctrl Pts',(16.6157332633671,46.7264684524801,-219.786529994355));
#225083=CARTESIAN_POINT('Ctrl Pts',(18.5095511653412,51.0344230260212,-213.177478362809));
#225084=CARTESIAN_POINT('Ctrl Pts',(11.955172894378,38.1072504572934,-233.023244257721));
#225085=CARTESIAN_POINT('Ctrl Pts',(13.6810225510899,42.425138848756,-226.412704198706));
#225086=CARTESIAN_POINT('Ctrl Pts',(15.4140075684236,46.7422144596123,-219.803514561937));
#225087=CARTESIAN_POINT('Ctrl Pts',(17.1488260183707,51.0590344085956,-213.194641337275));
#225088=CARTESIAN_POINT('Ctrl Pts',(11.5122134973833,38.1066368628798,-233.031384556208));
#225089=CARTESIAN_POINT('Ctrl Pts',(13.1594903500593,42.4286477016728,-226.42108503761));
#225090=CARTESIAN_POINT('Ctrl Pts',(14.8131447209518,46.7500874631785,-219.812006845727));
#225091=CARTESIAN_POINT('Ctrl Pts',(16.4684634448856,51.0713400998828,-213.203222824509));
#225092=CARTESIAN_POINT('Ctrl Pts',(11.068442842925,38.0899454377874,-233.039926782418));
#225093=CARTESIAN_POINT('Ctrl Pts',(12.638087651299,42.4126385857459,-226.429918907221));
#225094=CARTESIAN_POINT('Ctrl Pts',(14.2132461865494,46.7349565804957,-219.820978804832));
#225095=CARTESIAN_POINT('Ctrl Pts',(15.7898789431435,51.0571445898823,-213.212305200586));
#225096=CARTESIAN_POINT('Ctrl Pts',(10.6242185846299,38.0568674493847,-233.048972600031));
#225097=CARTESIAN_POINT('Ctrl Pts',(12.1179517821572,42.3771929832929,-226.439171170324));
#225098=CARTESIAN_POINT('Ctrl Pts',(13.616560960907,46.6972819912565,-219.83032594524));
#225099=CARTESIAN_POINT('Ctrl Pts',(15.1165093571175,51.0172823841975,-213.221727885471));
#225100=CARTESIAN_POINT('Ctrl Pts',(10.4021064554823,38.0403284551833,-233.053495508837));
#225101=CARTESIAN_POINT('Ctrl Pts',(11.8578838475863,42.3594701820664,-226.443797301875));
#225102=CARTESIAN_POINT('Ctrl Pts',(13.3182183480858,46.6784446966368,-219.834999515444));
#225103=CARTESIAN_POINT('Ctrl Pts',(14.7798245641045,50.9973512813551,-213.226439227913));
#225104=CARTESIAN_POINT('Ctrl Pts',(10.1798442304524,38.0196877247783,-233.058136253378));
#225105=CARTESIAN_POINT('Ctrl Pts',(11.5981402637213,42.3368907999987,-226.448528404105));
#225106=CARTESIAN_POINT('Ctrl Pts',(13.0207092672998,46.6539843758851,-219.839771381179));
#225107=CARTESIAN_POINT('Ctrl Pts',(14.4444911339896,50.971027695944,-213.231243449257));
#225108=CARTESIAN_POINT('Ctrl Pts',(9.95736629516326,37.9948908576778,-233.062889218446));
#225109=CARTESIAN_POINT('Ctrl Pts',(11.3388927023683,42.3094675608905,-226.453369189966));
#225110=CARTESIAN_POINT('Ctrl Pts',(12.72441998614,46.6239835088188,-219.844651948282));
#225111=CARTESIAN_POINT('Ctrl Pts',(14.1111031532653,50.9384648126854,-213.236155478191));
#225112=CARTESIAN_POINT('Ctrl Pts',(9.90174681134099,37.9886916409027,-233.064077459713));
#225113=CARTESIAN_POINT('Ctrl Pts',(11.2740808120301,42.3026117511134,-226.454579386432));
#225114=CARTESIAN_POINT('Ctrl Pts',(12.65034766585,46.6164832920523,-219.845872090057));
#225115=CARTESIAN_POINT('Ctrl Pts',(14.0277561580842,50.9303240918707,-213.237383485424));
#225116=CARTESIAN_POINT('Ctrl Pts',(9.84611383502457,37.9822326217319,-233.065272735655));
#225117=CARTESIAN_POINT('Ctrl Pts',(11.2092999192987,42.2954531938643,-226.45579646572));
#225118=CARTESIAN_POINT('Ctrl Pts',(12.5763515947833,46.6086368083103,-219.847099060522));
#225119=CARTESIAN_POINT('Ctrl Pts',(13.9445307783566,50.9217934508064,-213.238618271349));
#225120=CARTESIAN_POINT('Ctrl Pts',(9.79046632326175,37.9755128618122,-233.066475001199));
#225121=CARTESIAN_POINT('Ctrl Pts',(11.1445526978925,42.2879920750123,-226.457020557358));
#225122=CARTESIAN_POINT('Ctrl Pts',(12.5024378319264,46.6004453814869,-219.84833309334));
#225123=CARTESIAN_POINT('Ctrl Pts',(13.8614363478657,50.9128753563308,-213.23986015266));
#225124=CARTESIAN_POINT('Ctrl Pts',(9.76264256738034,37.9721529818524,-233.067076133971));
#225125=CARTESIAN_POINT('Ctrl Pts',(11.1121790871894,42.2842615155863,-226.457632603177));
#225126=CARTESIAN_POINT('Ctrl Pts',(12.465480950498,46.5963496680752,-219.848950109749));
#225127=CARTESIAN_POINT('Ctrl Pts',(13.8198891326202,50.908416309093,-213.240481093316));
#225128=CARTESIAN_POINT('Ctrl Pts',(9.73481517756063,37.9687279161475,-233.067679014418));
#225129=CARTESIAN_POINT('Ctrl Pts',(11.0798138942533,42.2804553156771,-226.458246402439));
#225130=CARTESIAN_POINT('Ctrl Pts',(12.4285446462698,46.5921677191209,-219.849568892204));
#225131=CARTESIAN_POINT('Ctrl Pts',(13.7783746550183,50.9038603989768,-213.241103808359));
#225132=CARTESIAN_POINT('Ctrl Pts',(9.70698402304477,37.96523754405,-233.068283638575));
#225133=CARTESIAN_POINT('Ctrl Pts',(11.0474574528907,42.2765734980184,-226.458861973485));
#225134=CARTESIAN_POINT('Ctrl Pts',(12.3916296775021,46.5878997014944,-219.850189472689));
#225135=CARTESIAN_POINT('Ctrl Pts',(13.7368940838208,50.899207937222,-213.241728340674));
#225136=CARTESIAN_POINT('Ctrl Pts',(9.70002623441581,37.9643649510258,-233.068434794615));
#225137=CARTESIAN_POINT('Ctrl Pts',(11.0393683425501,42.2756030436037,-226.459015866247));
#225138=CARTESIAN_POINT('Ctrl Pts',(12.3824009353102,46.5868326970878,-219.850344617811));
#225139=CARTESIAN_POINT('Ctrl Pts',(13.7265239410214,50.8980448217833,-213.241884473752));
#225140=CARTESIAN_POINT('Ctrl Pts',(9.69306821049259,37.9634882763409,-233.068586059642));
#225141=CARTESIAN_POINT('Ctrl Pts',(11.0312797791815,42.274627863078,-226.459169869752));
#225142=CARTESIAN_POINT('Ctrl Pts',(12.3731735265874,46.5857603133937,-219.850499875318));
#225143=CARTESIAN_POINT('Ctrl Pts',(13.7161559173791,50.8968756718767,-213.242040720421));
#225144=CARTESIAN_POINT('Ctrl Pts',(9.68610994922948,37.9626075180887,-233.068737433605));
#225145=CARTESIAN_POINT('Ctrl Pts',(11.0231917679977,42.2736479567932,-226.4593239843));
#225146=CARTESIAN_POINT('Ctrl Pts',(12.3639474631874,46.5846825530287,-219.850655245729));
#225147=CARTESIAN_POINT('Ctrl Pts',(13.7057900311691,50.8957004923844,-213.242197081372));
#225148=CARTESIAN_POINT('Ctrl Pts',(9.67915168796636,37.9617267598364,-233.068888807568));
#225149=CARTESIAN_POINT('Ctrl Pts',(11.0151037568139,42.2726680505084,-226.45947809885));
#225150=CARTESIAN_POINT('Ctrl Pts',(12.3547213997873,46.5836047926636,-219.850810616141));
#225151=CARTESIAN_POINT('Ctrl Pts',(13.6954241449592,50.8945253128921,-213.242353442324));
#225152=CARTESIAN_POINT('Ctrl Pts',(9.67042752180553,37.9608610921302,-233.068693023327));
#225153=CARTESIAN_POINT('Ctrl Pts',(11.0052222966165,42.2717086326066,-226.459283167064));
#225154=CARTESIAN_POINT('Ctrl Pts',(12.3436850388287,46.5825507404394,-219.850615812936));
#225155=CARTESIAN_POINT('Ctrl Pts',(13.6832345689085,50.893376327398,-213.242158728148));
#225156=CARTESIAN_POINT('Ctrl Pts',(9.66184542602245,37.9600013369658,-233.068526032011));
#225157=CARTESIAN_POINT('Ctrl Pts',(10.9954862692264,42.2707559642258,-226.459117194178));
#225158=CARTESIAN_POINT('Ctrl Pts',(12.3327965955135,46.5815044535368,-219.850450070761));
#225159=CARTESIAN_POINT('Ctrl Pts',(13.6711951099458,50.8922361823624,-213.241993156658));
#225160=CARTESIAN_POINT('Ctrl Pts',(9.64468123445628,37.9582818266369,-233.068192049379));
#225161=CARTESIAN_POINT('Ctrl Pts',(10.9760142144462,42.2688506274643,-226.458785248407));
#225162=CARTESIAN_POINT('Ctrl Pts',(12.3110197088832,46.5794118797315,-219.850118586413));
#225163=CARTESIAN_POINT('Ctrl Pts',(13.6471161920205,50.8899558922912,-213.241662013679));
#225164=CARTESIAN_POINT('Ctrl Pts',(9.62751103593916,37.9565806023487,-233.067859586963));
#225165=CARTESIAN_POINT('Ctrl Pts',(10.9565400925601,42.2669669096503,-226.45845486089));
#225166=CARTESIAN_POINT('Ctrl Pts',(12.2892446808081,46.5773442546879,-219.84978869258));
#225167=CARTESIAN_POINT('Ctrl Pts',(13.6230430466713,50.8877038777316,-213.241332486873));
#225168=CARTESIAN_POINT('Ctrl Pts',(9.61033490623753,37.9548976948076,-233.067528635586));
#225169=CARTESIAN_POINT('Ctrl Pts',(10.9370639460897,42.2651048145231,-226.458126026541));
#225170=CARTESIAN_POINT('Ctrl Pts',(12.2674715123898,46.5753015551307,-219.849460386617));
#225171=CARTESIAN_POINT('Ctrl Pts',(13.5989756308849,50.8854800884845,-213.241004575592));
#225172=CARTESIAN_POINT('Ctrl Pts',(9.47292586862441,37.9414344344784,-233.064881024575));
#225173=CARTESIAN_POINT('Ctrl Pts',(10.781254774326,42.2502080535059,-226.455495351754));
#225174=CARTESIAN_POINT('Ctrl Pts',(12.0932861650433,46.5589599586724,-219.846833938909));
#225175=CARTESIAN_POINT('Ctrl Pts',(13.4064363045935,50.8676897745073,-213.238381285338));
#225176=CARTESIAN_POINT('Ctrl Pts',(9.33513720062877,37.9291434250167,-233.062330002944));
#225177=CARTESIAN_POINT('Ctrl Pts',(10.6253160438035,42.2366951589798,-226.452964024174));
#225178=CARTESIAN_POINT('Ctrl Pts',(11.9192198479895,46.5442136325115,-219.844309093483));
#225179=CARTESIAN_POINT('Ctrl Pts',(13.2142636771733,50.8517059403811,-213.235861394914));
#225180=CARTESIAN_POINT('Ctrl Pts',(9.19700793929405,37.9180405342928,-233.059871683743));
#225181=CARTESIAN_POINT('Ctrl Pts',(10.4692694200224,42.2245679458519,-226.450529821256));
#225182=CARTESIAN_POINT('Ctrl Pts',(11.7452730443862,46.5310503906422,-219.841884642173));
#225183=CARTESIAN_POINT('Ctrl Pts',(13.0224356883732,50.837502473063,-213.233444529244));
#225184=CARTESIAN_POINT('Ctrl Pts',(8.09197384861627,37.8292174085014,-233.040205130141));
#225185=CARTESIAN_POINT('Ctrl Pts',(9.22089642977294,42.127550240828,-226.431056197904));
#225186=CARTESIAN_POINT('Ctrl Pts',(10.3536986155595,46.4257444556877,-219.822489031695));
#225187=CARTESIAN_POINT('Ctrl Pts',(11.4878117779725,50.7238747345189,-213.214109603883));
#225188=CARTESIAN_POINT('Ctrl Pts',(6.96366628211354,37.817478743917,-233.026371514464));
#225189=CARTESIAN_POINT('Ctrl Pts',(7.96513083913426,42.1193492727609,-226.417759570225));
#225190=CARTESIAN_POINT('Ctrl Pts',(8.96999102861579,46.4210021903668,-219.809524838153));
#225191=CARTESIAN_POINT('Ctrl Pts',(9.97605097124068,50.7225615951693,-213.201412296365));
#225192=CARTESIAN_POINT('Ctrl Pts',(5.84306516179973,37.8861012056782,-233.018416954225));
#225193=CARTESIAN_POINT('Ctrl Pts',(6.71532812355339,42.200163598718,-226.410167180765));
#225194=CARTESIAN_POINT('Ctrl Pts',(7.59093984899072,46.5139246326119,-219.802167559906));
#225195=CARTESIAN_POINT('Ctrl Pts',(8.46772145573762,50.8275648303208,-213.194245174231));
#225196=CARTESIAN_POINT('Ctrl Pts',(5.28276460164283,37.9204124365589,-233.014439674105));
#225197=CARTESIAN_POINT('Ctrl Pts',(6.09042676576295,42.2405707616966,-226.406370986035));
#225198=CARTESIAN_POINT('Ctrl Pts',(6.90141425917819,46.5603858537345,-219.798488920782));
#225199=CARTESIAN_POINT('Ctrl Pts',(7.71355669798609,50.8800664478965,-213.190661613164));
#225200=CARTESIAN_POINT('Ctrl Pts',(4.72420359085666,37.9746163354193,-233.011901696954));
#225201=CARTESIAN_POINT('Ctrl Pts',(5.46710405454763,42.3031873848396,-226.404003962692));
#225202=CARTESIAN_POINT('Ctrl Pts',(6.21329977779021,46.631377304189,-219.796233811454));
#225203=CARTESIAN_POINT('Ctrl Pts',(6.96062066828757,50.9594220750768,-213.188496987808));
#225204=CARTESIAN_POINT('Ctrl Pts',(4.17154639348007,38.0479355872538,-233.010781243767));
#225205=CARTESIAN_POINT('Ctrl Pts',(4.84705870160623,42.3878146595778,-226.403055663777));
#225206=CARTESIAN_POINT('Ctrl Pts',(5.52606587862577,46.7272431542647,-219.795396517945));
#225207=CARTESIAN_POINT('Ctrl Pts',(6.20622728545421,51.0665072531629,-213.187749079048));
#225208=CARTESIAN_POINT('Ctrl Pts',(3.89521779479178,38.084595213171,-233.010221017175));
#225209=CARTESIAN_POINT('Ctrl Pts',(4.53703602513553,42.430128296947,-226.40258151432));
#225210=CARTESIAN_POINT('Ctrl Pts',(5.18244892904355,46.7751760793026,-219.79497787119));
#225211=CARTESIAN_POINT('Ctrl Pts',(5.82903059403753,51.120049842206,-213.187375124668));
#225212=CARTESIAN_POINT('Ctrl Pts',(3.62033230763568,38.1260099641606,-233.010008856396));
#225213=CARTESIAN_POINT('Ctrl Pts',(4.22782250111806,42.4779423112143,-226.402459711852));
#225214=CARTESIAN_POINT('Ctrl Pts',(4.83905947521474,46.8293464189,-219.794913824891));
#225215=CARTESIAN_POINT('Ctrl Pts',(5.45149186218708,51.1805647729974,-213.187357480979));
#225216=CARTESIAN_POINT('Ctrl Pts',(3.3472053680105,38.1720472809816,-233.010141828064));
#225217=CARTESIAN_POINT('Ctrl Pts',(3.91959777386105,42.5312252846951,-226.402693706711));
#225218=CARTESIAN_POINT('Ctrl Pts',(4.49591409333425,46.8898251581957,-219.79521026164));
#225219=CARTESIAN_POINT('Ctrl Pts',(5.07345273996658,51.2482268355656,-213.187703873502));
#225220=CARTESIAN_POINT('Ctrl Pts',(3.31306450055735,38.1778019455842,-233.010158449522));
#225221=CARTESIAN_POINT('Ctrl Pts',(3.88106968295392,42.5378856563802,-226.402722956068));
#225222=CARTESIAN_POINT('Ctrl Pts',(4.4530209205992,46.8973850006076,-219.795247316233));
#225223=CARTESIAN_POINT('Ctrl Pts',(5.02619784968901,51.2566845933866,-213.187747172567));
#225224=CARTESIAN_POINT('Ctrl Pts',(3.27895110668782,38.1836288427124,-233.010180490037));
#225225=CARTESIAN_POINT('Ctrl Pts',(3.84255704326453,42.5446314764555,-226.40275777909));
#225226=CARTESIAN_POINT('Ctrl Pts',(4.41013156071601,46.9050434021283,-219.795290009254));
#225227=CARTESIAN_POINT('Ctrl Pts',(4.97893513726685,51.2652540112937,-213.187796158858));
#225228=CARTESIAN_POINT('Ctrl Pts',(3.24486579879784,38.189527717747,-233.010207966644));
#225229=CARTESIAN_POINT('Ctrl Pts',(3.80406020697863,42.5514626799883,-226.402798194813));
#225230=CARTESIAN_POINT('Ctrl Pts',(4.36724604523574,46.9128004931692,-219.795338357216));
#225231=CARTESIAN_POINT('Ctrl Pts',(4.93166428986477,51.2739354189312,-213.187850846732));
#225232=CARTESIAN_POINT('Ctrl Pts',(3.22782314485287,38.1924771552642,-233.010221704948));
#225233=CARTESIAN_POINT('Ctrl Pts',(3.78481178883567,42.5548782817547,-226.402818402674));
#225234=CARTESIAN_POINT('Ctrl Pts',(4.34580328749561,46.9166790386897,-219.795362531197));
#225235=CARTESIAN_POINT('Ctrl Pts',(4.90802886616373,51.27827612275,-213.187878190669));
#225236=CARTESIAN_POINT('Ctrl Pts',(3.2091142548194,38.1957230397313,-233.010272450532));
#225237=CARTESIAN_POINT('Ctrl Pts',(3.76387619377607,42.5586038688915,-226.402879998958));
#225238=CARTESIAN_POINT('Ctrl Pts',(4.32265861601423,46.9208779346775,-219.795430892831));
#225239=CARTESIAN_POINT('Ctrl Pts',(4.8826791576102,51.2829464276728,-213.187951984205));
#225240=CARTESIAN_POINT('Ctrl Pts',(3.19521896463729,38.1981918611683,-233.010222308172));
#225241=CARTESIAN_POINT('Ctrl Pts',(3.74780277505935,42.5615272078309,-226.402828279549));
#225242=CARTESIAN_POINT('Ctrl Pts',(4.30440722078206,46.924258408687,-219.795377959448));
#225243=CARTESIAN_POINT('Ctrl Pts',(4.86224701055348,51.286785332518,-213.187898031142));
#225244=CARTESIAN_POINT('Ctrl Pts',(3.18132367445518,38.2006606826052,-233.010172165812));
#225245=CARTESIAN_POINT('Ctrl Pts',(3.73172935634261,42.5644505467704,-226.40277656014));
#225246=CARTESIAN_POINT('Ctrl Pts',(4.2861558255499,46.9276388826966,-219.795325026065));
#225247=CARTESIAN_POINT('Ctrl Pts',(4.84181486349676,51.2906242373631,-213.18784407808));
#225248=CARTESIAN_POINT('Ctrl Pts',(3.16743147142012,38.2031124001538,-233.010122353862));
#225249=CARTESIAN_POINT('Ctrl Pts',(3.71565332942976,42.5673549891757,-226.402725177996));
#225250=CARTESIAN_POINT('Ctrl Pts',(4.26789592397522,46.9309986996984,-219.795272437686));
#225251=CARTESIAN_POINT('Ctrl Pts',(4.82136828241006,51.2944407248906,-213.187790477329));
#225252=CARTESIAN_POINT('Ctrl Pts',(3.15354223077676,38.2055470668879,-233.010072871279));
#225253=CARTESIAN_POINT('Ctrl Pts',(3.69957471452757,42.5702405351138,-226.402674131436));
#225254=CARTESIAN_POINT('Ctrl Pts',(4.24962766557925,46.9343378075759,-219.795220191932));
#225255=CARTESIAN_POINT('Ctrl Pts',(4.80090754229887,51.2982346912123,-213.187737225894));
#225256=CARTESIAN_POINT('Ctrl Pts',(3.0979852682033,38.2152857338245,-233.009874940946));
#225257=CARTESIAN_POINT('Ctrl Pts',(3.63526025491884,42.5817827188659,-226.402469945196));
#225258=CARTESIAN_POINT('Ctrl Pts',(4.17655463199535,46.9476942390858,-219.795011208915));
#225259=CARTESIAN_POINT('Ctrl Pts',(4.71906458185412,51.3134105564988,-213.187524220153));
#225260=CARTESIAN_POINT('Ctrl Pts',(3.04247570622088,38.2247515964697,-233.009682277023));
#225261=CARTESIAN_POINT('Ctrl Pts',(3.57090438655314,42.5930225619112,-226.402271124004));
#225262=CARTESIAN_POINT('Ctrl Pts',(4.10334789020144,46.9607193231595,-219.794807702832));
#225263=CARTESIAN_POINT('Ctrl Pts',(4.63699508002042,51.3282260774085,-213.187316797717));
#225264=CARTESIAN_POINT('Ctrl Pts',(2.98700554062687,38.2339479819771,-233.00949483998));
#225265=CARTESIAN_POINT('Ctrl Pts',(3.50650841057442,42.603960046196,-226.402077594881));
#225266=CARTESIAN_POINT('Ctrl Pts',(4.03001700195513,46.9734097359153,-219.79460956207));
#225267=CARTESIAN_POINT('Ctrl Pts',(4.55471661214503,51.3426746460284,-213.187114813067));
#225268=CARTESIAN_POINT('Ctrl Pts',(2.87606520943884,38.2523407529919,-233.009119965892));
#225269=CARTESIAN_POINT('Ctrl Pts',(3.377716458617,42.6258350147655,-226.401690536636));
#225270=CARTESIAN_POINT('Ctrl Pts',(3.88335522546252,46.9987905614268,-219.794213280545));
#225271=CARTESIAN_POINT('Ctrl Pts',(4.39015967639427,51.371571783268,-213.186710843768));
#225272=CARTESIAN_POINT('Ctrl Pts',(2.76528247646328,38.2696557306506,-233.008765954417));
#225273=CARTESIAN_POINT('Ctrl Pts',(3.24876407214238,42.6465005820265,-226.401324592275));
#225274=CARTESIAN_POINT('Ctrl Pts',(3.73619687364432,47.022832683185,-219.793838397139));
#225275=CARTESIAN_POINT('Ctrl Pts',(4.22476690304323,51.399001049048,-213.186328554894));
#225276=CARTESIAN_POINT('Ctrl Pts',(2.65459305129999,38.2859181692768,-233.008433022771));
#225277=CARTESIAN_POINT('Ctrl Pts',(3.11966175705484,42.6659561887148,-226.400979835546));
#225278=CARTESIAN_POINT('Ctrl Pts',(3.58861830572296,47.0455097321839,-219.793484786749));
#225279=CARTESIAN_POINT('Ctrl Pts',(4.05867850381481,51.4249103438683,-213.185967647486));
#225280=CARTESIAN_POINT('Ctrl Pts',(1.76907764999372,38.4160176782863,-233.005769569593));
#225281=CARTESIAN_POINT('Ctrl Pts',(2.08684323635451,42.8216010422206,-226.398221781712));
#225282=CARTESIAN_POINT('Ctrl Pts',(2.40798976235202,47.2269261241753,-219.790655903623));
#225283=CARTESIAN_POINT('Ctrl Pts',(2.72997130998742,51.6321847024301,-213.183080388226));
#225284=CARTESIAN_POINT('Ctrl Pts',(0.890062972301118,38.479927604964,-233.004448903383));
#225285=CARTESIAN_POINT('Ctrl Pts',(1.04391929270151,42.8997957436814,-226.396837718844));
#225286=CARTESIAN_POINT('Ctrl Pts',(1.19912105624254,47.3196638824289,-219.789226534345));
#225287=CARTESIAN_POINT('Ctrl Pts',(1.35468411325127,51.7395320211862,-213.181615349858));
#225288=CARTESIAN_POINT('Ctrl Pts',(-3.8650254009658E-7,38.4799275828018,
-233.004448906301));
#225289=CARTESIAN_POINT('Ctrl Pts',(-2.20334945258451E-7,42.8997957173221,
-226.396837721859));
#225290=CARTESIAN_POINT('Ctrl Pts',(-5.48039408136561E-8,47.3196638518424,
-219.789226537417));
#225291=CARTESIAN_POINT('Ctrl Pts',(1.10556392490902E-7,51.7395319863627,
-213.181615352975));
#225292=CARTESIAN_POINT('Ctrl Pts',(-0.890063745306199,38.4799275606396,
-233.00444890922));
#225293=CARTESIAN_POINT('Ctrl Pts',(-1.0439197333714,42.8997956909628,-226.396837724873));
#225294=CARTESIAN_POINT('Ctrl Pts',(-1.19912116585042,47.3196638212559,
-219.789226540489));
#225295=CARTESIAN_POINT('Ctrl Pts',(-1.35468389213849,51.7395319515393,
-213.181615356092));
#225296=CARTESIAN_POINT('Ctrl Pts',(-1.76907793008316,38.4160177700962,
-233.00576958377));
#225297=CARTESIAN_POINT('Ctrl Pts',(-2.08684470470783,42.8216008459315,
-226.39822179569));
#225298=CARTESIAN_POINT('Ctrl Pts',(-2.40799248287211,47.2269256299894,
-219.790655917783));
#225299=CARTESIAN_POINT('Ctrl Pts',(-2.72997529686207,51.6321839080993,
-213.183080402463));
#225300=CARTESIAN_POINT('Ctrl Pts',(-2.65459339500538,38.2859181503802,
-233.008433046465));
#225301=CARTESIAN_POINT('Ctrl Pts',(-3.11966241780403,42.6659560328282,
-226.400979857926));
#225302=CARTESIAN_POINT('Ctrl Pts',(-3.58861921803428,47.0455094471256,
-219.793484808433));
#225303=CARTESIAN_POINT('Ctrl Pts',(-4.05867966122096,51.4249099306337,
-213.185967668711));
#225304=CARTESIAN_POINT('Ctrl Pts',(-2.76528282812066,38.2696556979156,
-233.008765979303));
#225305=CARTESIAN_POINT('Ctrl Pts',(-3.24876463194106,42.6465004311903,
-226.401324615705));
#225306=CARTESIAN_POINT('Ctrl Pts',(-3.73619755992955,47.0228324242676,
-219.793838419764));
#225307=CARTESIAN_POINT('Ctrl Pts',(-4.22476770676582,51.3990006834506,
-213.186328576992));
#225308=CARTESIAN_POINT('Ctrl Pts',(-2.87606561582561,38.252340690496,-233.00911999099));
#225309=CARTESIAN_POINT('Ctrl Pts',(-3.37771687383254,42.6258348673936,
-226.401690560757));
#225310=CARTESIAN_POINT('Ctrl Pts',(-3.88335557699796,46.9987903386579,
-219.794213304243));
#225311=CARTESIAN_POINT('Ctrl Pts',(-4.39015995698515,51.3715714863033,
-213.186710867252));
#225312=CARTESIAN_POINT('Ctrl Pts',(-2.98700605032629,38.2339478860131,
-233.009494864304));
#225313=CARTESIAN_POINT('Ctrl Pts',(-3.50650877598108,42.6039598904826,
-226.402077618808));
#225314=CARTESIAN_POINT('Ctrl Pts',(-4.0300171714589,46.9734095274016,-219.794609585932));
#225315=CARTESIAN_POINT('Ctrl Pts',(-4.55471658101984,51.342674385518,-213.18711483698));
#225316=CARTESIAN_POINT('Ctrl Pts',(-3.04247626757663,38.2247514837717,
-233.00968230096));
#225317=CARTESIAN_POINT('Ctrl Pts',(-3.57090472705535,42.5930224020271,
-226.402271147832));
#225318=CARTESIAN_POINT('Ctrl Pts',(-4.10334796868937,46.9607191217734,
-219.794807726776));
#225319=CARTESIAN_POINT('Ctrl Pts',(-4.63699489303719,51.3282258351254,
-213.187316821844));
#225320=CARTESIAN_POINT('Ctrl Pts',(-3.09798589335121,38.2152856034861,
-233.009874964222));
#225321=CARTESIAN_POINT('Ctrl Pts',(-3.63526059420306,42.5817825518452,
-226.402469968673));
#225322=CARTESIAN_POINT('Ctrl Pts',(-4.17655465764593,46.9476940393167,
-219.795011232678));
#225323=CARTESIAN_POINT('Ctrl Pts',(-4.71906429187351,51.3134103243417,
-213.187524244216));
#225324=CARTESIAN_POINT('Ctrl Pts',(-3.15354293202228,38.2055469196549,
-233.010072893454));
#225325=CARTESIAN_POINT('Ctrl Pts',(-3.69957509350717,42.5702403566339,
-226.402674154044));
#225326=CARTESIAN_POINT('Ctrl Pts',(-4.24962770925554,46.9343375997015,
-219.795220214898));
#225327=CARTESIAN_POINT('Ctrl Pts',(-4.8009072498816,51.2982344540852,-213.187737249183));
#225328=CARTESIAN_POINT('Ctrl Pts',(-3.16743219169004,38.2031122486971,
-233.010122375761));
#225329=CARTESIAN_POINT('Ctrl Pts',(-3.7156537183332,42.5673548078311,-226.402725200387));
#225330=CARTESIAN_POINT('Ctrl Pts',(-4.26789597215794,46.9309984897978,
-219.795272460453));
#225331=CARTESIAN_POINT('Ctrl Pts',(-4.82136798938362,51.2944404865211,
-213.187790500425));
#225332=CARTESIAN_POINT('Ctrl Pts',(-3.18132441451801,38.200660526972,-233.010172187407));
#225333=CARTESIAN_POINT('Ctrl Pts',(-3.73172975772618,42.5644503622906,
-226.402776582281));
#225334=CARTESIAN_POINT('Ctrl Pts',(-4.28615588266773,46.9276386701613,
-219.795325048593));
#225335=CARTESIAN_POINT('Ctrl Pts',(-4.84181457614597,51.2906239968065,
-213.187844100936));
#225336=CARTESIAN_POINT('Ctrl Pts',(-3.19521972526473,38.1981917014322,
-233.010222329432));
#225337=CARTESIAN_POINT('Ctrl Pts',(-3.74780319174879,42.5615270199239,
-226.402828301403));
#225338=CARTESIAN_POINT('Ctrl Pts',(-4.30440729177531,46.9242581928414,
-219.795377981691));
#225339=CARTESIAN_POINT('Ctrl Pts',(-4.86224673591111,51.2867850887177,
-213.187898053706));
#225340=CARTESIAN_POINT('Ctrl Pts',(-3.20911503601145,38.1957228758924,
-233.010272471457));
#225341=CARTESIAN_POINT('Ctrl Pts',(-3.76387662577141,42.5586036775571,
-226.402880020524));
#225342=CARTESIAN_POINT('Ctrl Pts',(-4.32265870088289,46.9208777155215,
-219.79543091479));
#225343=CARTESIAN_POINT('Ctrl Pts',(-4.88267889567624,51.282946180629,-213.187952006476));
#225344=CARTESIAN_POINT('Ctrl Pts',(-3.22782410538323,38.1924769641916,
-233.010221721999));
#225345=CARTESIAN_POINT('Ctrl Pts',(-3.78481240503387,42.5548780619928,
-226.40281841985));
#225346=CARTESIAN_POINT('Ctrl Pts',(-4.34580355870831,46.9166787905631,
-219.795362548448));
#225347=CARTESIAN_POINT('Ctrl Pts',(-4.90802879230411,51.2782758463453,
-213.187878207983));
#225348=CARTESIAN_POINT('Ctrl Pts',(-3.24486675962954,38.1895275274507,
-233.010207983672));
#225349=CARTESIAN_POINT('Ctrl Pts',(-3.8040608233549,42.5514624611386,-226.402798211965));
#225350=CARTESIAN_POINT('Ctrl Pts',(-4.36724631650623,46.912800246089,-219.795338374444));
#225351=CARTESIAN_POINT('Ctrl Pts',(-4.93166421594236,51.2739351437073,
-213.187850864022));
#225352=CARTESIAN_POINT('Ctrl Pts',(-3.27895206812217,38.1836286539689,
-233.010180507016));
#225353=CARTESIAN_POINT('Ctrl Pts',(-3.84255765999695,42.5446312594299,
-226.402757796196));
#225354=CARTESIAN_POINT('Ctrl Pts',(-4.41013183210206,46.905043157141,-219.795290026436));
#225355=CARTESIAN_POINT('Ctrl Pts',(-4.97893506321885,51.2652537384313,
-213.187796176101));
#225356=CARTESIAN_POINT('Ctrl Pts',(-3.31306546258716,38.1778017583963,
-233.010158466454));
#225357=CARTESIAN_POINT('Ctrl Pts',(-3.8810703000381,42.5378854411796,-226.402722973126));
#225358=CARTESIAN_POINT('Ctrl Pts',(-4.45302119209974,46.8973847577122,
-219.795247333368));
#225359=CARTESIAN_POINT('Ctrl Pts',(-5.0261977755178,51.2566843228826,-213.187747189765));
#225360=CARTESIAN_POINT('Ctrl Pts',(-3.34720633062972,38.1720470953519,
-233.010141844947));
#225361=CARTESIAN_POINT('Ctrl Pts',(-3.91959839129335,42.5312250713203,
-226.402693723722));
#225362=CARTESIAN_POINT('Ctrl Pts',(-4.4959143649488,46.8898249173908,-219.795210278728));
#225363=CARTESIAN_POINT('Ctrl Pts',(-5.07345266567515,51.2482265674168,
-213.187703890653));
#225364=CARTESIAN_POINT('Ctrl Pts',(-3.62033327497023,38.1260097909964,
-233.010008872892));
#225365=CARTESIAN_POINT('Ctrl Pts',(-4.22782312133536,42.4779421124458,
-226.402459728486));
#225366=CARTESIAN_POINT('Ctrl Pts',(-4.83905974774131,46.8293461948202,
-219.794913841607));
#225367=CARTESIAN_POINT('Ctrl Pts',(-5.45149178693396,51.1805645236904,
-213.187357497761));
#225368=CARTESIAN_POINT('Ctrl Pts',(-3.89521876641643,38.0845950526478,
-233.010221033278));
#225369=CARTESIAN_POINT('Ctrl Pts',(-4.53703664788045,42.4301281128367,
-226.402581530569));
#225370=CARTESIAN_POINT('Ctrl Pts',(-5.18244920243109,46.7751758718739,
-219.794977887527));
#225371=CARTESIAN_POINT('Ctrl Pts',(-5.82903051799349,51.1200496115382,
-213.187375141075));
#225372=CARTESIAN_POINT('Ctrl Pts',(-4.17154736896545,38.0479354395528,
-233.010781259488));
#225373=CARTESIAN_POINT('Ctrl Pts',(-4.84705932662186,42.3878144901718,
-226.403055679645));
#225374=CARTESIAN_POINT('Ctrl Pts',(-5.52606615282163,46.7272429633994,
-219.795396533901));
#225375=CARTESIAN_POINT('Ctrl Pts',(-6.20622720878553,51.0665070409123,
-213.187749095075));
#225376=CARTESIAN_POINT('Ctrl Pts',(-4.72420457406351,37.9746162133627,
-233.011901711911));
#225377=CARTESIAN_POINT('Ctrl Pts',(-5.46710468410469,42.3031872448421,
-226.404003977796));
#225378=CARTESIAN_POINT('Ctrl Pts',(-6.21330005360272,46.6313771464505,
-219.79623382665));
#225379=CARTESIAN_POINT('Ctrl Pts',(-6.96062059036963,50.9594218996606,
-213.188497003076));
#225380=CARTESIAN_POINT('Ctrl Pts',(-5.28276558977247,37.9204123410526,
-233.014439688315));
#225381=CARTESIAN_POINT('Ctrl Pts',(-6.0904273987647,42.2405706513073,-226.406371000396));
#225382=CARTESIAN_POINT('Ctrl Pts',(-6.90141453697469,46.5603857286617,
-219.798488935235));
#225383=CARTESIAN_POINT('Ctrl Pts',(-7.71355662058354,50.8800663082066,
-213.19066162769));
#225384=CARTESIAN_POINT('Ctrl Pts',(-5.84306615270387,37.8861011368416,
-233.018416967692));
#225385=CARTESIAN_POINT('Ctrl Pts',(-6.71532875876053,42.2001635180319,
-226.410167194365));
#225386=CARTESIAN_POINT('Ctrl Pts',(-7.59094012855401,46.513924540267,-219.80216757359));
#225387=CARTESIAN_POINT('Ctrl Pts',(-8.46772137968994,50.8275647263818,
-213.194245187983));
#225388=CARTESIAN_POINT('Ctrl Pts',(-6.96366727856668,37.8174787284193,
-233.026371526446));
#225389=CARTESIAN_POINT('Ctrl Pts',(-7.96513147875218,42.1193492514812,
-226.417759582303));
#225390=CARTESIAN_POINT('Ctrl Pts',(-8.96999131171265,46.4210021634777,
-219.8095248503));
#225391=CARTESIAN_POINT('Ctrl Pts',(-9.97605089790276,50.7225615627321,
-213.201412308567));
#225392=CARTESIAN_POINT('Ctrl Pts',(-8.09197483879552,37.8292174475599,
-233.040205140506));
#225393=CARTESIAN_POINT('Ctrl Pts',(-9.22089706830802,42.1275502793173,
-226.431056208459));
#225394=CARTESIAN_POINT('Ctrl Pts',(-10.3536989025166,46.4257444938288,
-219.822489042393));
#225395=CARTESIAN_POINT('Ctrl Pts',(-11.4878117132961,50.7238747723913,
-213.214109614699));
#225396=CARTESIAN_POINT('Ctrl Pts',(-9.19700891511567,37.9180406246053,
-233.059871692371));
#225397=CARTESIAN_POINT('Ctrl Pts',(-10.4692700536151,42.2245680436116,
-226.45052983021));
#225398=CARTESIAN_POINT('Ctrl Pts',(-11.7452733355946,46.5310504960556,
-219.841884651363));
#225399=CARTESIAN_POINT('Ctrl Pts',(-13.0224356370472,50.8375025861988,
-213.233444538625));
#225400=CARTESIAN_POINT('Ctrl Pts',(-9.33513817465568,37.929143521736,-233.062330011354));
#225401=CARTESIAN_POINT('Ctrl Pts',(-10.6253166767785,42.2366952641485,
-226.452964032928));
#225402=CARTESIAN_POINT('Ctrl Pts',(-11.9192201397294,46.544213746334,-219.844309102484));
#225403=CARTESIAN_POINT('Ctrl Pts',(-13.2142636275161,50.8517060629247,
-213.235861404116));
#225404=CARTESIAN_POINT('Ctrl Pts',(-9.47292684075068,37.9414345375616,
-233.064881032772));
#225405=CARTESIAN_POINT('Ctrl Pts',(-10.7812554066213,42.250208166077,-226.455495360308));
#225406=CARTESIAN_POINT('Ctrl Pts',(-12.0932864573056,46.5589600809337,
-219.84683394772));
#225407=CARTESIAN_POINT('Ctrl Pts',(-13.4064362566527,50.8676899065243,
-213.238381294356));
#225408=CARTESIAN_POINT('Ctrl Pts',(-9.61033587635758,37.9548978042124,
-233.067528643578));
#225409=CARTESIAN_POINT('Ctrl Pts',(-10.9370645776426,42.2651049344897,
-226.458126034897));
#225410=CARTESIAN_POINT('Ctrl Pts',(-12.2674718051654,46.5753016858586,
-219.849460395235));
#225411=CARTESIAN_POINT('Ctrl Pts',(-13.5989755847082,50.8854802300378,
-213.241004584421));
#225412=CARTESIAN_POINT('Ctrl Pts',(-9.62751200580844,37.9565807125437,
-233.067859594929));
#225413=CARTESIAN_POINT('Ctrl Pts',(-10.9565407240203,42.2669670305412,
-226.458454869221));
#225414=CARTESIAN_POINT('Ctrl Pts',(-12.2892449736479,46.5773443864743,
-219.849788701174));
#225415=CARTESIAN_POINT('Ctrl Pts',(-13.6230430007151,50.8877040204769,
-213.24133249568));
#225416=CARTESIAN_POINT('Ctrl Pts',(-9.64468220407303,37.9582819376215,
-233.068192057319));
#225417=CARTESIAN_POINT('Ctrl Pts',(-10.9760148458125,42.2688507492795,
-226.458785256713));
#225418=CARTESIAN_POINT('Ctrl Pts',(-12.3110200017871,46.5794120125766,
-219.850118594983));
#225419=CARTESIAN_POINT('Ctrl Pts',(-13.6471161462857,50.8899560362295,
-213.241662022461));
#225420=CARTESIAN_POINT('Ctrl Pts',(-9.66184639538513,37.9600014487392,
-233.068526039926));
#225421=CARTESIAN_POINT('Ctrl Pts',(-10.9954869004979,42.2707560869652,
-226.459117202459));
#225422=CARTESIAN_POINT('Ctrl Pts',(-12.3327968884813,46.5815045874411,
-219.850450079307));
#225423=CARTESIAN_POINT('Ctrl Pts',(-13.671195064433,50.8922363274947,-213.241993165417));
#225424=CARTESIAN_POINT('Ctrl Pts',(-9.67042849104117,37.9608612042982,
-233.068693031229));
#225425=CARTESIAN_POINT('Ctrl Pts',(-11.0052229278407,42.2717087558081,
-226.459283175332));
#225426=CARTESIAN_POINT('Ctrl Pts',(-12.3436853318284,46.5825508748733,
-219.850615821469));
#225427=CARTESIAN_POINT('Ctrl Pts',(-13.6832345235066,50.8933764731273,
-213.242158736895));
#225428=CARTESIAN_POINT('Ctrl Pts',(-9.67915246067952,37.9617268745383,
-233.068888776823));
#225429=CARTESIAN_POINT('Ctrl Pts',(-11.0151041884445,42.272668176984,-226.459478068261));
#225430=CARTESIAN_POINT('Ctrl Pts',(-12.3547214913109,46.5836049308703,
-219.850810585692));
#225431=CARTESIAN_POINT('Ctrl Pts',(-13.6954238965826,50.8945254628113,
-213.242353411989));
#225432=CARTESIAN_POINT('Ctrl Pts',(-9.68611072192926,37.9626076324355,
-233.068737402912));
#225433=CARTESIAN_POINT('Ctrl Pts',(-11.0231921996786,42.2736480828614,
-226.459323953766));
#225434=CARTESIAN_POINT('Ctrl Pts',(-12.3639475548251,46.584682690775,-219.850655215335));
#225435=CARTESIAN_POINT('Ctrl Pts',(-13.7057897829706,50.8957006417903,
-213.242197051092));
#225436=CARTESIAN_POINT('Ctrl Pts',(-9.69306898317901,37.9634883903329,
-233.068586029));
#225437=CARTESIAN_POINT('Ctrl Pts',(-11.0312802109126,42.2746279887388,
-226.459169839269));
#225438=CARTESIAN_POINT('Ctrl Pts',(-12.3731736183394,46.5857604506798,
-219.850499844976));
#225439=CARTESIAN_POINT('Ctrl Pts',(-13.7161556693587,50.8968758207694,
-213.242040690194));
#225440=CARTESIAN_POINT('Ctrl Pts',(-9.70002700708928,37.9643650646628,
-233.068434764026));
#225441=CARTESIAN_POINT('Ctrl Pts',(-11.039368774331,42.275603168857,-226.459015835818));
#225442=CARTESIAN_POINT('Ctrl Pts',(-12.3824010271756,46.5868328339135,
-219.850344587522));
#225443=CARTESIAN_POINT('Ctrl Pts',(-13.7265236931781,50.8980449701626,
-213.241884443579));
#225444=CARTESIAN_POINT('Ctrl Pts',(-9.70698479570498,37.9652376573323,
-233.068283608038));
#225445=CARTESIAN_POINT('Ctrl Pts',(-11.0474578847215,42.2765736228642,
-226.458861943109));
#225446=CARTESIAN_POINT('Ctrl Pts',(-12.3916297694808,46.5878998378596,
-219.850189442454));
#225447=CARTESIAN_POINT('Ctrl Pts',(-13.7368938361541,50.8992080850876,
-213.241728310554));
#225448=CARTESIAN_POINT('Ctrl Pts',(-9.73481595016779,37.9687280280104,
-233.067678984089));
#225449=CARTESIAN_POINT('Ctrl Pts',(-11.0798143262832,42.2804554388931,
-226.458246372274));
#225450=CARTESIAN_POINT('Ctrl Pts',(-12.4285447387014,46.5921678536441,
-219.849568862182));
#225451=CARTESIAN_POINT('Ctrl Pts',(-13.7783744080581,50.9038605447878,
-213.241103778454));
#225452=CARTESIAN_POINT('Ctrl Pts',(-9.76264333993521,37.9721530922971,
-233.067076103849));
#225453=CARTESIAN_POINT('Ctrl Pts',(-11.112179519415,42.2842616371721,-226.457632573223));
#225454=CARTESIAN_POINT('Ctrl Pts',(-12.4654810433745,46.5963498007545,
-219.848950079941));
#225455=CARTESIAN_POINT('Ctrl Pts',(-13.8198888863544,50.908416452846,-213.240481063626));
#225456=CARTESIAN_POINT('Ctrl Pts',(-9.79046709576529,37.9755129708399,
-233.066474971284));
#225457=CARTESIAN_POINT('Ctrl Pts',(-11.1445531303096,42.2879921949675,
-226.457020527615));
#225458=CARTESIAN_POINT('Ctrl Pts',(-12.5024379252396,46.6004455123205,
-219.848333063744));
#225459=CARTESIAN_POINT('Ctrl Pts',(-13.8614361022817,50.9128754980226,
-213.239860123184));
#225460=CARTESIAN_POINT('Ctrl Pts',(-9.84611460742545,37.9822327279253,
-233.065272706155));
#225461=CARTESIAN_POINT('Ctrl Pts',(-11.2093003520988,42.2954533105585,
-226.455796436398));
#225462=CARTESIAN_POINT('Ctrl Pts',(-12.5763516889697,46.6086369354524,
-219.847099031351));
#225463=CARTESIAN_POINT('Ctrl Pts',(-13.9445305341362,50.9217935883757,
-213.238618242301));
#225464=CARTESIAN_POINT('Ctrl Pts',(-9.90174758364278,37.9886917442662,
-233.064077430627));
#225465=CARTESIAN_POINT('Ctrl Pts',(-11.2740812451978,42.302611864545,-226.454579357529));
#225466=CARTESIAN_POINT('Ctrl Pts',(-12.6503477608772,46.6164834154958,
-219.845872061308));
#225467=CARTESIAN_POINT('Ctrl Pts',(-14.0277559151782,50.9303242253047,
-213.2373834568));
#225468=CARTESIAN_POINT('Ctrl Pts',(-9.95736706736925,37.9948909582156,
-233.062889189772));
#225469=CARTESIAN_POINT('Ctrl Pts',(-11.3388931358883,42.309467671058,-226.453369161482));
#225470=CARTESIAN_POINT('Ctrl Pts',(-12.7244200819753,46.6239836285565,
-219.844651919953));
#225471=CARTESIAN_POINT('Ctrl Pts',(-14.1111029116247,50.9384649419709,
-213.236155449989));
#225472=CARTESIAN_POINT('Ctrl Pts',(-10.1798450022751,38.0196878140133,
-233.058136226355));
#225473=CARTESIAN_POINT('Ctrl Pts',(-11.5981406986501,42.3368908971099,
-226.44852837729));
#225474=CARTESIAN_POINT('Ctrl Pts',(-13.0207093663679,46.6539844807995,
-219.839771354532));
#225475=CARTESIAN_POINT('Ctrl Pts',(-14.4444908974109,50.9710278086359,
-213.231243422746));
#225476=CARTESIAN_POINT('Ctrl Pts',(-10.4021072269767,38.0403285331826,
-233.053495483453));
#225477=CARTESIAN_POINT('Ctrl Pts',(-11.8578842836773,42.3594702660982,
-226.443797276706));
#225478=CARTESIAN_POINT('Ctrl Pts',(-13.3182184498665,46.6784447866133,
-219.834999490445));
#225479=CARTESIAN_POINT('Ctrl Pts',(-14.779824331803,50.9973513772468,-213.226439203051));
#225480=CARTESIAN_POINT('Ctrl Pts',(-10.624219355847,38.0568675162082,-233.048972576276));
#225481=CARTESIAN_POINT('Ctrl Pts',(-12.1179522191619,42.3771930542225,
-226.439171146782));
#225482=CARTESIAN_POINT('Ctrl Pts',(-13.6165610648823,46.6972820661859,
-219.830325921867));
#225483=CARTESIAN_POINT('Ctrl Pts',(-15.1165091283142,51.0172824630919,
-213.221727862234));
#225484=CARTESIAN_POINT('Ctrl Pts',(-11.0684436135876,38.0899454822592,
-233.039926761921));
#225485=CARTESIAN_POINT('Ctrl Pts',(-12.6380880901309,42.4126386304711,
-226.429918886935));
#225486=CARTESIAN_POINT('Ctrl Pts',(-14.213246294914,46.734956625331,-219.820978784711));
#225487=CARTESIAN_POINT('Ctrl Pts',(-15.7898787213367,51.0571446347821,
-213.212305180598));
#225488=CARTESIAN_POINT('Ctrl Pts',(-11.5122142673659,38.1066368853063,
-233.031384538877));
#225489=CARTESIAN_POINT('Ctrl Pts',(-13.1594907899084,42.4286477200682,
-226.421085020555));
#225490=CARTESIAN_POINT('Ctrl Pts',(-14.8131448321181,46.7500874773532,
-219.812006828876));
#225491=CARTESIAN_POINT('Ctrl Pts',(-16.4684632276865,51.0713401097786,
-213.203222807822));
#225492=CARTESIAN_POINT('Ctrl Pts',(-11.955173663454,38.1072504577147,-233.023244243446));
#225493=CARTESIAN_POINT('Ctrl Pts',(-13.6810229909314,42.4251388408351,
-226.412704184797));
#225494=CARTESIAN_POINT('Ctrl Pts',(-15.4140076804602,46.7422144431276,
-219.803514548276));
#225495=CARTESIAN_POINT('Ctrl Pts',(-17.1488258029255,51.0590343834786,
-213.194641323813));
#225496=CARTESIAN_POINT('Ctrl Pts',(-12.84109245563,38.1084776025314,-233.006963652583));
#225497=CARTESIAN_POINT('Ctrl Pts',(-14.7240873929774,42.4181210823689,
-226.39594251328));
#225498=CARTESIAN_POINT('Ctrl Pts',(-16.6157333771444,46.7264683746764,
-219.786529987073));
#225499=CARTESIAN_POINT('Ctrl Pts',(-18.5095509534035,51.0344229308787,
-213.177478355796));
#225500=CARTESIAN_POINT('Ctrl Pts',(-13.7245141560456,38.045502939269,-232.992416062106));
#225501=CARTESIAN_POINT('Ctrl Pts',(-15.7672051862484,42.332953713727,-226.380908971242));
#225502=CARTESIAN_POINT('Ctrl Pts',(-17.8201130442209,46.6183897548803,
-219.77126728422));
#225503=CARTESIAN_POINT('Ctrl Pts',(-19.8755795270071,50.9032330228086,
-213.162032252099));
#225504=CARTESIAN_POINT('Ctrl Pts',(-14.6053490349759,37.9175429299717,
-232.979423899816));
#225505=CARTESIAN_POINT('Ctrl Pts',(-16.7994173900859,42.1702100364746,
-226.367656687286));
#225506=CARTESIAN_POINT('Ctrl Pts',(-19.0045203102992,46.4201830445647,
-219.757864931005));
#225507=CARTESIAN_POINT('Ctrl Pts',(-21.2125141699292,50.6693287472216,
-213.14851266454));
#225508=CARTESIAN_POINT('Ctrl Pts',(-15.0457664744411,37.8535629253232,
-232.97292781867));
#225509=CARTESIAN_POINT('Ctrl Pts',(-17.3155234920046,42.0888381978483,
-226.361030545308));
#225510=CARTESIAN_POINT('Ctrl Pts',(-19.5967239433384,46.3210796894069,
-219.751163754398));
#225511=CARTESIAN_POINT('Ctrl Pts',(-21.8809814913902,50.552376609428,-213.14175287076));
#225512=CARTESIAN_POINT('Ctrl Pts',(-15.48526861201,37.7733459621789,-232.966774981656));
#225513=CARTESIAN_POINT('Ctrl Pts',(-17.8290108602587,41.988075541514,-226.354862155988));
#225514=CARTESIAN_POINT('Ctrl Pts',(-20.1842675910139,46.1994856953577,
-219.744968154358));
#225515=CARTESIAN_POINT('Ctrl Pts',(-22.5426916464067,50.4098403859979,
-213.135537404114));
#225516=CARTESIAN_POINT('Ctrl Pts',(-15.9242800874034,37.6762618259859,
-232.961008694015));
#225517=CARTESIAN_POINT('Ctrl Pts',(-18.3384991035959,41.8681521066547,
-226.349116383292));
#225518=CARTESIAN_POINT('Ctrl Pts',(-20.764164143618,46.056490812383,-219.739206307543));
#225519=CARTESIAN_POINT('Ctrl Pts',(-23.1930959226737,50.2436622443285,
-213.129764719864));
#225520=CARTESIAN_POINT('Ctrl Pts',(-15.9517183046155,37.6701940674739,
-232.960648301037));
#225521=CARTESIAN_POINT('Ctrl Pts',(-18.3703421188045,41.860656891976,-226.348757272499));
#225522=CARTESIAN_POINT('Ctrl Pts',(-20.8004076781558,46.0475536321971,
-219.738846192116));
#225523=CARTESIAN_POINT('Ctrl Pts',(-23.2337461899404,50.2332761104742,
-213.129403927098));
#225524=CARTESIAN_POINT('Ctrl Pts',(-15.9791545938371,37.6640603777139,
-232.960289439234));
#225525=CARTESIAN_POINT('Ctrl Pts',(-18.4021695113665,41.8530868241542,
-226.348399840238));
#225526=CARTESIAN_POINT('Ctrl Pts',(-20.8366213419039,46.0385328730506,
-219.738487803237));
#225527=CARTESIAN_POINT('Ctrl Pts',(-23.2743522940981,50.2227976648295,
-213.129044899828));
#225528=CARTESIAN_POINT('Ctrl Pts',(-16.0065890534061,37.6578605855432,
-232.959932127495));
#225529=CARTESIAN_POINT('Ctrl Pts',(-18.4339809440506,41.8454419566488,
-226.348044089065));
#225530=CARTESIAN_POINT('Ctrl Pts',(-20.8728044058038,46.0294288081912,
-219.738131136274));
#225531=CARTESIAN_POINT('Ctrl Pts',(-23.3149131244886,50.2122273973641,
-213.128687627634));
#225532=CARTESIAN_POINT('Ctrl Pts',(-16.0340235129751,37.6516607933725,
-232.959574815754));
#225533=CARTESIAN_POINT('Ctrl Pts',(-18.4657923767348,41.8377970891434,
-226.347688337893));
#225534=CARTESIAN_POINT('Ctrl Pts',(-20.9089874697038,46.0203247433318,
-219.737774469313));
#225535=CARTESIAN_POINT('Ctrl Pts',(-23.3554739548789,50.2016571298987,
-213.128330355439));
#225536=CARTESIAN_POINT('Ctrl Pts',(-16.0585473554683,37.6463741383586,
-232.958775273912));
#225537=CARTESIAN_POINT('Ctrl Pts',(-18.4946401987194,41.8310959004748,
-226.346905335007));
#225538=CARTESIAN_POINT('Ctrl Pts',(-20.9421634338297,46.0121797638875,
-219.736999507462));
#225539=CARTESIAN_POINT('Ctrl Pts',(-23.3929890444876,50.192055755358,-213.127562035262));
#225540=CARTESIAN_POINT('Ctrl Pts',(-16.0918767223523,37.6380308441171,
-232.959320969893));
#225541=CARTESIAN_POINT('Ctrl Pts',(-18.5323945369195,41.821207032461,-226.347422705618));
#225542=CARTESIAN_POINT('Ctrl Pts',(-20.9843159739407,46.0007627353008,
-219.737497937658));
#225543=CARTESIAN_POINT('Ctrl Pts',(-23.4395359476608,50.1791148808152,
-213.128045277776));
#225544=CARTESIAN_POINT('Ctrl Pts',(-16.1585354561205,37.6213442556341,
-232.960412361857));
#225545=CARTESIAN_POINT('Ctrl Pts',(-18.6079032133198,41.8014292964334,
-226.348457446837));
#225546=CARTESIAN_POINT('Ctrl Pts',(-21.0686210541628,45.9779286781272,
-219.73849479805));
#225547=CARTESIAN_POINT('Ctrl Pts',(-23.532629754007,50.1532331317297,-213.129011762805));
#225548=CARTESIAN_POINT('Ctrl Pts',(-16.2252933388625,37.6049409039171,
-232.961526557635));
#225549=CARTESIAN_POINT('Ctrl Pts',(-18.6835028812545,41.7819858489469,
-226.349515473638));
#225550=CARTESIAN_POINT('Ctrl Pts',(-21.1530100301158,45.955479449566,-219.739515199653));
#225551=CARTESIAN_POINT('Ctrl Pts',(-23.6258004655779,50.1277866774147,
-213.130001982515));
#225552=CARTESIAN_POINT('Ctrl Pts',(-16.2921479467574,37.5888219250063,
-232.962663792009));
#225553=CARTESIAN_POINT('Ctrl Pts',(-18.7591909572452,41.7628773303161,
-226.350596942329));
#225554=CARTESIAN_POINT('Ctrl Pts',(-21.2374802154051,45.9334151950853,
-219.740559260363));
#225555=CARTESIAN_POINT('Ctrl Pts',(-23.7190453200257,50.1027751618064,
-213.131016024784));
#225556=CARTESIAN_POINT('Ctrl Pts',(-16.425857162547,37.5565839671848,-232.964938260758));
#225557=CARTESIAN_POINT('Ctrl Pts',(-18.9105671092267,41.7246602930543,
-226.352759879711));
#225558=CARTESIAN_POINT('Ctrl Pts',(-21.4064205859838,45.889286686124,-219.742647381781));
#225559=CARTESIAN_POINT('Ctrl Pts',(-23.9055350289214,50.0527521305898,
-213.133044109322));
#225560=CARTESIAN_POINT('Ctrl Pts',(-16.5599532780166,37.5254834870874,
-232.967304860586));
#225561=CARTESIAN_POINT('Ctrl Pts',(-19.0622968915723,41.6877829617887,
-226.355016566202));
#225562=CARTESIAN_POINT('Ctrl Pts',(-21.5756857922305,45.8466980666759,
-219.744830124902));
#225563=CARTESIAN_POINT('Ctrl Pts',(-24.0923213080095,50.0044688493901,
-213.135167472361));
#225564=CARTESIAN_POINT('Ctrl Pts',(-16.6944169130979,37.4955297315077,
-232.969765748647));
#225565=CARTESIAN_POINT('Ctrl Pts',(-19.2143596596656,41.6522505690609,
-226.357368473114));
#225566=CARTESIAN_POINT('Ctrl Pts',(-21.7452543638979,45.8056505796339,
-219.747108608993));
#225567=CARTESIAN_POINT('Ctrl Pts',(-24.2793820749247,49.9579225253783,
-213.137386957196));
#225568=CARTESIAN_POINT('Ctrl Pts',(-16.9633441832605,37.4356222203481,
-232.974687524767));
#225569=CARTESIAN_POINT('Ctrl Pts',(-19.5184851958523,41.5811857836052,
-226.362072286937));
#225570=CARTESIAN_POINT('Ctrl Pts',(-22.0843915072326,45.72355560555,-219.751665577176));
#225571=CARTESIAN_POINT('Ctrl Pts',(-24.6535036087552,49.8648298773548,
-213.141825926864));
#225572=CARTESIAN_POINT('Ctrl Pts',(-17.2337415161106,37.3803013708413,
-232.97998607555));
#225573=CARTESIAN_POINT('Ctrl Pts',(-19.8239426506046,41.5155005848133,
-226.367156683727));
#225574=CARTESIAN_POINT('Ctrl Pts',(-22.424742090129,45.6476250384896,-219.756605270226));
#225575=CARTESIAN_POINT('Ctrl Pts',(-25.0287230766563,49.7786849702844,
-213.146649192944));
#225576=CARTESIAN_POINT('Ctrl Pts',(-17.5054540549992,37.3296438557812,
-232.985683160017));
#225577=CARTESIAN_POINT('Ctrl Pts',(-20.1305671964664,41.4552387299725,
-226.372636994436));
#225578=CARTESIAN_POINT('Ctrl Pts',(-22.7661346481492,45.5778702003308,
-219.761939487332));
#225579=CARTESIAN_POINT('Ctrl Pts',(-25.4048640524227,49.6994664417413,
-213.151865770696));
#225580=CARTESIAN_POINT('Ctrl Pts',(-19.6791543661082,36.9243837353004,
-233.031259835762));
#225581=CARTESIAN_POINT('Ctrl Pts',(-22.5835635633614,40.9731438912471,
-226.416479480112));
#225582=CARTESIAN_POINT('Ctrl Pts',(-25.4972751123102,45.0198314950608,
-219.804613224178));
#225583=CARTESIAN_POINT('Ctrl Pts',(-28.4139918585542,49.0657182133968,
-213.193598392712));
#225584=CARTESIAN_POINT('Ctrl Pts',(-21.9374109084496,36.8211293864807,
-233.101701686809));
#225585=CARTESIAN_POINT('Ctrl Pts',(-25.111744382231,40.8399102842966,-226.485020485526));
#225586=CARTESIAN_POINT('Ctrl Pts',(-28.2953873712226,44.8571207481071,
-219.871880081892));
#225587=CARTESIAN_POINT('Ctrl Pts',(-31.4821075264257,48.8736849792366,
-213.259832525996));
#225588=CARTESIAN_POINT('Ctrl Pts',(-24.1738401119771,37.0431281239647,
-233.208100074818));
#225589=CARTESIAN_POINT('Ctrl Pts',(-27.6162089587335,41.0700376714878,
-226.588760346578));
#225590=CARTESIAN_POINT('Ctrl Pts',(-31.0681789277548,45.0961312181189,
-219.973963335611));
#225591=CARTESIAN_POINT('Ctrl Pts',(-34.5233304322506,49.1218090514821,
-213.360583159555));
#225592=CARTESIAN_POINT('',(23.1986390639935,37.1456077148496,-232.850148134873));
#225593=CARTESIAN_POINT('',(23.9219400150789,37.2105701781699,-232.850048861683));
#225594=CARTESIAN_POINT('Ctrl Pts',(23.1986878229135,37.1456673944601,-232.85005));
#225595=CARTESIAN_POINT('Ctrl Pts',(23.3194048257383,37.1546203352643,-232.85005));
#225596=CARTESIAN_POINT('Ctrl Pts',(23.4400515103151,37.1645093048432,-232.85005));
#225597=CARTESIAN_POINT('Ctrl Pts',(23.6811421252914,37.1861530761466,-232.85005));
#225598=CARTESIAN_POINT('Ctrl Pts',(23.8015841730299,37.1979071335885,-232.85005));
#225599=CARTESIAN_POINT('Ctrl Pts',(23.9219289933242,37.2105934913504,-232.85005));
#225600=CARTESIAN_POINT('',(33.4675954689601,48.355842190426,-214.55199127893));
#225601=CARTESIAN_POINT('Ctrl Pts',(23.9219400150789,37.2105701781699,-232.850048861683));
#225602=CARTESIAN_POINT('Ctrl Pts',(24.4418606617069,37.878778891458,-231.743275247233));
#225603=CARTESIAN_POINT('Ctrl Pts',(24.9947791463521,38.5760331124526,-230.591022418697));
#225604=CARTESIAN_POINT('Ctrl Pts',(25.5827531876322,39.3022826557374,-229.39331304588));
#225605=CARTESIAN_POINT('Ctrl Pts',(25.7351746609535,39.4905495138209,-229.082828884338));
#225606=CARTESIAN_POINT('Ctrl Pts',(25.8899517028263,39.6807648773527,-228.769290034352));
#225607=CARTESIAN_POINT('Ctrl Pts',(26.0471192761083,39.8729278713654,-228.45269696414));
#225608=CARTESIAN_POINT('Ctrl Pts',(26.4288443515238,40.3396490394141,-227.683762819018));
#225609=CARTESIAN_POINT('Ctrl Pts',(26.8246878338526,40.8178589630018,-226.896809721117));
#225610=CARTESIAN_POINT('Ctrl Pts',(27.2352389947482,41.3075425018447,-226.091828317012));
#225611=CARTESIAN_POINT('Ctrl Pts',(27.440514575196,41.5523842712661,-225.689337614959));
#225612=CARTESIAN_POINT('Ctrl Pts',(27.6494678664072,41.8000944125765,-225.282339642736));
#225613=CARTESIAN_POINT('Ctrl Pts',(27.8621772375357,42.0506708295902,-224.870831918007));
#225614=CARTESIAN_POINT('Ctrl Pts',(27.9685319231,42.1759590380971,-224.665078055643));
#225615=CARTESIAN_POINT('Ctrl Pts',(28.0758256277802,42.3019638116919,-224.458196752125));
#225616=CARTESIAN_POINT('Ctrl Pts',(28.1840684939521,42.4286848767254,-224.250187589526));
#225617=CARTESIAN_POINT('Ctrl Pts',(28.238189927038,42.4920454092422,-224.146183008227));
#225618=CARTESIAN_POINT('Ctrl Pts',(28.292548650422,42.5555850143397,-224.041896461924));
#225619=CARTESIAN_POINT('Ctrl Pts',(28.3471459410457,42.6193036567116,-223.937327894143));
#225620=CARTESIAN_POINT('Ctrl Pts',(28.3744445863575,42.6511629778975,-223.885043610253));
#225621=CARTESIAN_POINT('Ctrl Pts',(28.4018028734742,42.6830670583836,-223.832688820977));
#225622=CARTESIAN_POINT('Ctrl Pts',(28.4292209631686,42.7150158936996,-223.78026351885));
#225623=CARTESIAN_POINT('Ctrl Pts',(28.4532117916512,42.742971124601,-223.734391379489));
#225624=CARTESIAN_POINT('Ctrl Pts',(28.477248406482,42.770960620918,-223.688465253726));
#225625=CARTESIAN_POINT('Ctrl Pts',(28.5013309157674,42.7989843796288,-223.642485136405));
#225626=CARTESIAN_POINT('Ctrl Pts',(28.5047712742368,42.8029877737304,-223.635916548216));
#225627=CARTESIAN_POINT('Ctrl Pts',(28.5087290203377,42.8075927211393,-223.628361017554));
#225628=CARTESIAN_POINT('Ctrl Pts',(28.5116548013666,42.8109966596226,-223.622776066215));
#225629=CARTESIAN_POINT('Ctrl Pts',(28.8371805675898,43.1897227748008,-223.001387949309));
#225630=CARTESIAN_POINT('Ctrl Pts',(29.1745459726135,43.5788145813041,-222.363412782327));
#225631=CARTESIAN_POINT('Ctrl Pts',(29.5240447341431,43.9782923394872,-221.70885488244));
#225632=CARTESIAN_POINT('Ctrl Pts',(29.5766255923689,44.0383923618034,-221.610378950841));
#225633=CARTESIAN_POINT('Ctrl Pts',(29.6294811733118,44.0987274444299,-221.511527682382));
#225634=CARTESIAN_POINT('Ctrl Pts',(29.6826125773133,44.1592976381529,-221.412301090776));
#225635=CARTESIAN_POINT('Ctrl Pts',(29.8857573664897,44.390884201043,-221.03291407078));
#225636=CARTESIAN_POINT('Ctrl Pts',(30.0929331856782,44.6259080707781,-220.648040158275));
#225637=CARTESIAN_POINT('Ctrl Pts',(30.3042007923876,44.864372719193,-220.257679030983));
#225638=CARTESIAN_POINT('Ctrl Pts',(30.4098345957423,44.9836050434004,-220.062498467337));
#225639=CARTESIAN_POINT('Ctrl Pts',(30.5164913454516,45.1036975586825,-219.865946097492));
#225640=CARTESIAN_POINT('Ctrl Pts',(30.6241789389476,45.2246506847414,-219.668021790972));
#225641=CARTESIAN_POINT('Ctrl Pts',(30.6780227356957,45.2851272477709,-219.569059637713));
#225642=CARTESIAN_POINT('Ctrl Pts',(30.7321242433433,45.3458189632478,-219.4697545001));
#225643=CARTESIAN_POINT('Ctrl Pts',(30.7864844571222,45.4067258825371,-219.370106358403));
#225644=CARTESIAN_POINT('Ctrl Pts',(30.8136645640117,45.4371793421818,-219.320282287555));
#225645=CARTESIAN_POINT('Ctrl Pts',(30.8409093474307,45.4676866027635,-219.270372465674));
#225646=CARTESIAN_POINT('Ctrl Pts',(30.8682189327952,45.4982476706417,-219.220376889958));
#225647=CARTESIAN_POINT('Ctrl Pts',(30.8887011218186,45.5211684715504,-219.182880208172));
#225648=CARTESIAN_POINT('Ctrl Pts',(30.9092197619361,45.5441195390619,-219.145335289853));
#225649=CARTESIAN_POINT('Ctrl Pts',(30.9297749062752,45.5671008758434,-219.107742133744));
#225650=CARTESIAN_POINT('Ctrl Pts',(30.9366266210549,45.5747613214372,-219.095211081708));
#225651=CARTESIAN_POINT('Ctrl Pts',(30.9443340309044,45.5833769999799,-219.081117624891));
#225652=CARTESIAN_POINT('Ctrl Pts',(30.9503422206756,45.5900923024801,-219.070132898319));
#225653=CARTESIAN_POINT('Ctrl Pts',(31.2808092427288,45.9594524764969,-218.465942615328));
#225654=CARTESIAN_POINT('Ctrl Pts',(31.6240078517053,46.3403008201657,-217.843285810584));
#225655=CARTESIAN_POINT('Ctrl Pts',(31.9801868039357,46.7326727266222,-217.202164072734));
#225656=CARTESIAN_POINT('Ctrl Pts',(32.3336946073896,47.1221020567942,-216.565850399861));
#225657=CARTESIAN_POINT('Ctrl Pts',(32.6999887764574,47.5228828432546,-215.911347715658));
#225658=CARTESIAN_POINT('Ctrl Pts',(33.0793631737681,47.935041240388,-215.23865685648));
#225659=CARTESIAN_POINT('Ctrl Pts',(33.2072821834606,48.0740144931206,-215.011836203464));
#225660=CARTESIAN_POINT('Ctrl Pts',(33.3366887540973,48.2142812245276,-214.782947673812));
#225661=CARTESIAN_POINT('Ctrl Pts',(33.4675954689601,48.355842190426,-214.55199127893));
#225662=CARTESIAN_POINT('Ctrl Pts',(33.4676028656973,48.3558414173478,-214.551973774401));
#225663=CARTESIAN_POINT('Ctrl Pts',(30.901862658951,48.7536658275797,-213.450221490923));
#225664=CARTESIAN_POINT('Ctrl Pts',(28.0171449119245,49.1337591199062,-213.211816166462));
#225665=CARTESIAN_POINT('Ctrl Pts',(25.2356859051905,49.4352084301762,-213.575672669215));
#225666=CARTESIAN_POINT('Ctrl Pts',(24.8032357476663,49.482076567149,-213.632243627676));
#225667=CARTESIAN_POINT('Ctrl Pts',(24.3877560644765,49.5255154092148,-213.701836863213));
#225668=CARTESIAN_POINT('Ctrl Pts',(24.03731337216,49.561263296092,-213.768798684283));
#225669=CARTESIAN_POINT('Ctrl Pts',(23.8252559380841,49.5828948076944,-213.80931815371));
#225670=CARTESIAN_POINT('Ctrl Pts',(23.6273316981886,49.6027398562885,-213.850344519519));
#225671=CARTESIAN_POINT('Ctrl Pts',(23.4328829972625,49.6219541201266,-213.893239486649));
#225672=CARTESIAN_POINT('Ctrl Pts',(23.3313424796551,49.6319877500057,-213.915639107446));
#225673=CARTESIAN_POINT('Ctrl Pts',(23.230757278012,49.6418462076065,-213.938569475617));
#225674=CARTESIAN_POINT('Ctrl Pts',(23.1296327664199,49.6516771209836,-213.96235621794));
#225675=CARTESIAN_POINT('Ctrl Pts',(23.085029569752,49.6560132622008,-213.972847885383));
#225676=CARTESIAN_POINT('Ctrl Pts',(23.0403017126433,49.6603474871157,-213.983418653291));
#225677=CARTESIAN_POINT('Ctrl Pts',(22.9952661957579,49.6647017043639,-213.993851883475));
#225678=CARTESIAN_POINT('Ctrl Pts',(22.9520128737166,49.6688836117539,-214.003872238435));
#225679=CARTESIAN_POINT('Ctrl Pts',(22.908490275569,49.6730813341779,-214.013831433549));
#225680=CARTESIAN_POINT('Ctrl Pts',(22.8645836069524,49.6773054855748,-214.02374962579));
#225681=CARTESIAN_POINT('Ctrl Pts',(22.7494415108754,49.6883830202935,-214.049759375103));
#225682=CARTESIAN_POINT('Ctrl Pts',(22.6316603245303,49.6996429322849,-214.075496523236));
#225683=CARTESIAN_POINT('Ctrl Pts',(22.5091539919612,49.7112704713707,-214.101231806193));
#225684=CARTESIAN_POINT('Ctrl Pts',(22.0167441198786,49.75800695359,-214.204673866071));
#225685=CARTESIAN_POINT('Ctrl Pts',(21.3972641828706,49.8152106337258,-214.315369623735));
#225686=CARTESIAN_POINT('Ctrl Pts',(20.796432808198,49.8685261402426,-214.394114559153));
#225687=CARTESIAN_POINT('Ctrl Pts',(19.4772558081119,49.9855849239708,-214.567005842891));
#225688=CARTESIAN_POINT('Ctrl Pts',(18.1397819123848,50.0948434821514,-214.617115230396));
#225689=CARTESIAN_POINT('Ctrl Pts',(16.8015661238258,50.1948649177512,-214.517648223079));
#225690=CARTESIAN_POINT('Ctrl Pts',(16.0733214987344,50.2492956556727,-214.463519199889));
#225691=CARTESIAN_POINT('Ctrl Pts',(15.4167055758679,50.2955918304614,-214.369161556618));
#225692=CARTESIAN_POINT('Ctrl Pts',(14.8786895652353,50.3323031651629,-214.269588134207));
#225693=CARTESIAN_POINT('Ctrl Pts',(14.5167312569262,50.3570012639959,-214.2025986268));
#225694=CARTESIAN_POINT('Ctrl Pts',(14.202155330086,50.3778195415913,-214.1327896286));
#225695=CARTESIAN_POINT('Ctrl Pts',(13.9364760833966,50.3951159243116,-214.068404584443));
#225696=CARTESIAN_POINT('Ctrl Pts',(13.8539190573513,50.4004905929638,-214.048397610493));
#225697=CARTESIAN_POINT('Ctrl Pts',(13.7760879080755,50.405523949103,-214.028903353814));
#225698=CARTESIAN_POINT('Ctrl Pts',(13.7030382763995,50.4102234769291,-214.010137001906));
#225699=CARTESIAN_POINT('Ctrl Pts',(13.6627871480097,50.4128129670273,-213.99979654128));
#225700=CARTESIAN_POINT('Ctrl Pts',(13.623987818724,50.4153010762635,-213.98967678931));
#225701=CARTESIAN_POINT('Ctrl Pts',(13.5866496246302,50.4176888915325,-213.979811340452));
#225702=CARTESIAN_POINT('Ctrl Pts',(13.5768617283821,50.4183148373951,-213.977225195294));
#225703=CARTESIAN_POINT('Ctrl Pts',(13.5671742371175,50.4189338907117,-213.974656515408));
#225704=CARTESIAN_POINT('Ctrl Pts',(13.5575873139323,50.4195460700437,-213.972105883982));
#225705=CARTESIAN_POINT('Ctrl Pts',(13.5466235875268,50.4202461660575,-213.969188949678));
#225706=CARTESIAN_POINT('Ctrl Pts',(13.5357905517574,50.4209372643919,-213.966298904327));
#225707=CARTESIAN_POINT('Ctrl Pts',(13.5250821831194,50.421619333823,-213.963461027108));
#225708=CARTESIAN_POINT('Ctrl Pts',(13.501794131956,50.4231026660043,-213.957289346613));
#225709=CARTESIAN_POINT('Ctrl Pts',(13.4791042282484,50.4245433767524,-213.951330941414));
#225710=CARTESIAN_POINT('Ctrl Pts',(13.4570189352174,50.4259417414909,-213.945579087136));
#225711=CARTESIAN_POINT('Ctrl Pts',(13.2532048418568,50.4388465483666,-213.892498108615));
#225712=CARTESIAN_POINT('Ctrl Pts',(13.0902503949803,50.4488803522574,-213.853486772554));
#225713=CARTESIAN_POINT('Ctrl Pts',(12.9104008459301,50.4597229754217,-213.813164200894));
#225714=CARTESIAN_POINT('Ctrl Pts',(11.4496555026504,50.5477872012135,-213.485662635884));
#225715=CARTESIAN_POINT('Ctrl Pts',(9.93840942401383,50.6207736864612,-213.359232839684));
#225716=CARTESIAN_POINT('Ctrl Pts',(8.43667805237259,50.6748332488454,-213.428209574319));
#225717=CARTESIAN_POINT('Ctrl Pts',(8.23238827711037,50.6821873043435,-213.437592904709));
#225718=CARTESIAN_POINT('Ctrl Pts',(8.02834204153374,50.6891969690078,-213.450528247198));
#225719=CARTESIAN_POINT('Ctrl Pts',(7.824503888911,50.6958660191919,-213.466980375523));
#225720=CARTESIAN_POINT('Ctrl Pts',(7.25602553293655,50.7144651412688,-213.512863242603));
#225721=CARTESIAN_POINT('Ctrl Pts',(6.6538362810014,50.7311625041638,-213.593251906418));
#225722=CARTESIAN_POINT('Ctrl Pts',(6.15552385199797,50.7430175186589,-213.680345086889));
#225723=CARTESIAN_POINT('Ctrl Pts',(5.72610318100236,50.7532335758609,-213.755397623852));
#225724=CARTESIAN_POINT('Ctrl Pts',(5.36706219916213,50.7604549681015,-213.832054599617));
#225725=CARTESIAN_POINT('Ctrl Pts',(5.00965909049245,50.7667680020115,-213.917612838338));
#225726=CARTESIAN_POINT('Ctrl Pts',(4.96190685115584,50.7676114795832,-213.929044181249));
#225727=CARTESIAN_POINT('Ctrl Pts',(4.91419131129741,50.7684360583204,-213.940659514235));
#225728=CARTESIAN_POINT('Ctrl Pts',(4.86635293877012,50.7692443949469,-213.952498814775));
#225729=CARTESIAN_POINT('Ctrl Pts',(4.8430126288082,50.7696387818463,-213.958275201591));
#225730=CARTESIAN_POINT('Ctrl Pts',(4.81964739249074,50.7700288847056,-213.964123321728));
#225731=CARTESIAN_POINT('Ctrl Pts',(4.7962245577203,50.7704163078938,-213.969988537243));
#225732=CARTESIAN_POINT('Ctrl Pts',(4.77566091609363,50.7707564388677,-213.975137793988));
#225733=CARTESIAN_POINT('Ctrl Pts',(4.75504506642069,50.7710952449316,-213.980267091875));
#225734=CARTESIAN_POINT('Ctrl Pts',(4.73436429387878,50.7714328972265,-213.985379046521));
#225735=CARTESIAN_POINT('Ctrl Pts',(4.65303700461145,50.7727607173458,-214.005481845554));
#225736=CARTESIAN_POINT('Ctrl Pts',(4.57070598326991,50.7740709043372,-214.025319649038));
#225737=CARTESIAN_POINT('Ctrl Pts',(4.48659701201007,50.7753721870468,-214.045025781685));
#225738=CARTESIAN_POINT('Ctrl Pts',(4.32894533783954,50.7778112776057,-214.081962445595));
#225739=CARTESIAN_POINT('Ctrl Pts',(4.16505838170397,50.7802213764123,-214.118471962292));
#225740=CARTESIAN_POINT('Ctrl Pts',(3.98974842067771,50.7826329069094,-214.155016004706));
#225741=CARTESIAN_POINT('Ctrl Pts',(3.57148470877949,50.7883864630175,-214.242204700306));
#225742=CARTESIAN_POINT('Ctrl Pts',(3.10286408217604,50.7938341521992,-214.324313596318));
#225743=CARTESIAN_POINT('Ctrl Pts',(2.65136385212586,50.7979637376852,-214.386713900287));
#225744=CARTESIAN_POINT('Ctrl Pts',(1.77493142783601,50.8059799077288,-214.507842630781));
#225745=CARTESIAN_POINT('Ctrl Pts',(0.886906888442037,50.8100674225229,
-214.57114562896));
#225746=CARTESIAN_POINT('Ctrl Pts',(7.57796986272652E-8,50.8100674233964,
-214.571145595706));
#225747=CARTESIAN_POINT('Ctrl Pts',(-0.689331197484988,50.8100674240753,
-214.57114556986));
#225748=CARTESIAN_POINT('Ctrl Pts',(-1.38062861972754,50.807607880196,-214.532824696008));
#225749=CARTESIAN_POINT('Ctrl Pts',(-2.06681665421521,50.8027193023931,
-214.458682419818));
#225750=CARTESIAN_POINT('Ctrl Pts',(-2.71339489002495,50.7981129148542,
-214.388819962695));
#225751=CARTESIAN_POINT('Ctrl Pts',(-3.37138077803095,50.7911390626746,
-214.283916861856));
#225752=CARTESIAN_POINT('Ctrl Pts',(-3.98974958328583,50.7826328964271,
-214.155015446714));
#225753=CARTESIAN_POINT('Ctrl Pts',(-4.1637062425794,50.7802399809838,-214.118753495326));
#225754=CARTESIAN_POINT('Ctrl Pts',(-4.3278016707857,50.777828977619,-214.08223006206));
#225755=CARTESIAN_POINT('Ctrl Pts',(-4.48659703808242,50.7753721929754,
-214.045025412884));
#225756=CARTESIAN_POINT('Ctrl Pts',(-4.5704464158805,50.7740749267689,-214.025380087345));
#225757=CARTESIAN_POINT('Ctrl Pts',(-4.65281520992318,50.77276434532,-214.005536277871));
#225758=CARTESIAN_POINT('Ctrl Pts',(-4.73436407287352,50.7714329078382,
-213.985378700013));
#225759=CARTESIAN_POINT('Ctrl Pts',(-4.75503326394108,50.7710954446939,
-213.980269605746));
#225760=CARTESIAN_POINT('Ctrl Pts',(-4.77564977279552,50.7707566302578,
-213.97514017803));
#225761=CARTESIAN_POINT('Ctrl Pts',(-4.79622435607242,50.7704163183534,
-213.96998817968));
#225762=CARTESIAN_POINT('Ctrl Pts',(-4.8196348408496,50.7700290994945,-213.964126054683));
#225763=CARTESIAN_POINT('Ctrl Pts',(-4.84300112848971,50.7696389832667,
-213.958277641287));
#225764=CARTESIAN_POINT('Ctrl Pts',(-4.86635294089622,50.7692444019801,
-213.952498409351));
#225765=CARTESIAN_POINT('Ctrl Pts',(-4.91415558624414,50.768436668988,-213.940667953976));
#225766=CARTESIAN_POINT('Ctrl Pts',(-4.96187958607181,50.7676119681406,
-213.929050309711));
#225767=CARTESIAN_POINT('Ctrl Pts',(-5.00965909045278,50.7667680089134,
-213.917612443077));
#225768=CARTESIAN_POINT('Ctrl Pts',(-5.36927133290557,50.7604159532737,
-213.831525387076));
#225769=CARTESIAN_POINT('Ctrl Pts',(-5.73167895489853,50.753100932397,-213.754422765144));
#225770=CARTESIAN_POINT('Ctrl Pts',(-6.15552383543092,50.7430175245826,
-213.680344773112));
#225771=CARTESIAN_POINT('Ctrl Pts',(-6.31572994732526,50.7392061689787,
-213.652344559767));
#225772=CARTESIAN_POINT('Ctrl Pts',(-6.48476935122518,50.7349828986066,
-213.624915677394));
#225773=CARTESIAN_POINT('Ctrl Pts',(-6.66599545505587,50.7301771498111,
-213.598432925724));
#225774=CARTESIAN_POINT('Ctrl Pts',(-7.23349350002257,50.715128252393,-213.515503869255));
#225775=CARTESIAN_POINT('Ctrl Pts',(-7.84439075174546,50.6961545036633,
-213.45541400729));
#225776=CARTESIAN_POINT('Ctrl Pts',(-8.436678010806,50.6748332530167,-213.428209423087));
#225777=CARTESIAN_POINT('Ctrl Pts',(-9.31368610829759,50.6432625764916,
-213.387927211592));
#225778=CARTESIAN_POINT('Ctrl Pts',(-10.1922509633074,50.6054259689156,
-213.412946620486));
#225779=CARTESIAN_POINT('Ctrl Pts',(-11.0647191696714,50.5616460640852,
-213.507390029984));
#225780=CARTESIAN_POINT('Ctrl Pts',(-11.6857669687375,50.5304822768665,
-213.574617547477));
#225781=CARTESIAN_POINT('Ctrl Pts',(-12.3036600542713,50.4963016674955,
-213.677132040931));
#225782=CARTESIAN_POINT('Ctrl Pts',(-12.9104007912719,50.4597229753191,
-213.81316438299));
#225783=CARTESIAN_POINT('Ctrl Pts',(-13.1010995860117,50.44822628145,-213.855919388702));
#225784=CARTESIAN_POINT('Ctrl Pts',(-13.2813016781285,50.4370675494195,
-213.899815823864));
#225785=CARTESIAN_POINT('Ctrl Pts',(-13.4570188815656,50.4259417407046,
-213.945579312412));
#225786=CARTESIAN_POINT('Ctrl Pts',(-13.4797777977165,50.4245007244427,
-213.951506605689));
#225787=CARTESIAN_POINT('Ctrl Pts',(-13.5024612388415,50.4230601703824,
-213.957466382958));
#225788=CARTESIAN_POINT('Ctrl Pts',(-13.5250821296103,50.4216193329497,
-213.963461257796));
#225789=CARTESIAN_POINT('Ctrl Pts',(-13.5359306197904,50.4209283384658,
-213.966336270167));
#225790=CARTESIAN_POINT('Ctrl Pts',(-13.54676299098,50.4202372600292,-213.969226285269));
#225791=CARTESIAN_POINT('Ctrl Pts',(-13.5575870608609,50.4195460819038,
-213.972106062562));
#225792=CARTESIAN_POINT('Ctrl Pts',(-13.5672802347205,50.4189271178902,
-213.974684961469));
#225793=CARTESIAN_POINT('Ctrl Pts',(-13.5769673322604,50.4183080796475,
-213.977253341563));
#225794=CARTESIAN_POINT('Ctrl Pts',(-13.5866493728619,50.417688903386,-213.979811516833));
#225795=CARTESIAN_POINT('Ctrl Pts',(-13.6255051838502,50.4152040350842,
-213.990077945045));
#225796=CARTESIAN_POINT('Ctrl Pts',(-13.6642796078801,50.412716947939,-214.000180186509));
#225797=CARTESIAN_POINT('Ctrl Pts',(-13.7030380297945,50.4102234887559,
-214.010137169485));
#225798=CARTESIAN_POINT('Ctrl Pts',(-13.7807410638259,50.40522459215,-214.030098967433));
#225799=CARTESIAN_POINT('Ctrl Pts',(-13.8583799763604,50.4002001721689,
-214.049478889196));
#225800=CARTESIAN_POINT('Ctrl Pts',(-13.9364758468782,50.3951159360852,
-214.068404734377));
#225801=CARTESIAN_POINT('Ctrl Pts',(-14.2341686709201,50.3757353902535,
-214.140547963741));
#225802=CARTESIAN_POINT('Ctrl Pts',(-14.5382696861838,50.3555315939824,
-214.206584999646));
#225803=CARTESIAN_POINT('Ctrl Pts',(-14.8786893660444,50.3323031767319,
-214.269588212978));
#225804=CARTESIAN_POINT('Ctrl Pts',(-15.3967781923265,50.2969515676985,
-214.365473565024));
#225805=CARTESIAN_POINT('Ctrl Pts',(-15.9993479121824,50.2548246171532,
-214.458020891098));
#225806=CARTESIAN_POINT('Ctrl Pts',(-16.8015659878209,50.1948649289014,
-214.517648156697));
#225807=CARTESIAN_POINT('Ctrl Pts',(-17.2395658580743,50.1621277761592,
-214.550203811312));
#225808=CARTESIAN_POINT('Ctrl Pts',(-17.7082120160163,50.1260503285933,
-214.567856665254));
#225809=CARTESIAN_POINT('Ctrl Pts',(-18.1637878991495,50.0898577036051,
-214.568151042825));
#225810=CARTESIAN_POINT('Ctrl Pts',(-19.0450457944776,50.0198473327658,
-214.568720481568));
#225811=CARTESIAN_POINT('Ctrl Pts',(-19.9260477691704,49.9457608258918,
-214.508186877708));
#225812=CARTESIAN_POINT('Ctrl Pts',(-20.7964327548152,49.8685261515117,
-214.394114193465));
#225813=CARTESIAN_POINT('Ctrl Pts',(-21.5053808339726,49.8056167781319,
-214.301199435384));
#225814=CARTESIAN_POINT('Ctrl Pts',(-22.2396557444683,49.7374282494541,
-214.16491573399));
#225815=CARTESIAN_POINT('Ctrl Pts',(-22.8645835730838,49.6773054980824,
-214.023749106193));
#225816=CARTESIAN_POINT('Ctrl Pts',(-22.9084582558125,49.6730844240313,
-214.013838136121));
#225817=CARTESIAN_POINT('Ctrl Pts',(-22.9519885580468,49.6688859720506,
-214.003877337734));
#225818=CARTESIAN_POINT('Ctrl Pts',(-22.9952661624728,49.6647017170029,
-213.993851354185));
#225819=CARTESIAN_POINT('Ctrl Pts',(-23.0402921169331,49.6603484243535,
-213.983420336001));
#225820=CARTESIAN_POINT('Ctrl Pts',(-23.0850289057069,49.6560133363786,
-213.972847495132));
#225821=CARTESIAN_POINT('Ctrl Pts',(-23.1296329441772,49.6516771132442,
-213.962355632284));
#225822=CARTESIAN_POINT('Ctrl Pts',(-23.2309014126094,49.6418322047861,
-213.938535034013));
#225823=CARTESIAN_POINT('Ctrl Pts',(-23.3315871269299,49.6319635848738,
-213.915584604225));
#225824=CARTESIAN_POINT('Ctrl Pts',(-23.4328831691411,49.6219541124168,
-213.893238920191));
#225825=CARTESIAN_POINT('Ctrl Pts',(-23.6291639753803,49.602558810478,-213.849939806204));
#225826=CARTESIAN_POINT('Ctrl Pts',(-23.8277143103713,49.5826440436499,
-213.808847903502));
#225827=CARTESIAN_POINT('Ctrl Pts',(-24.0373135320024,49.5612632885096,
-213.768798156763));
#225828=CARTESIAN_POINT('Ctrl Pts',(-24.3911283485615,49.525171418039,-213.701192019271));
#225829=CARTESIAN_POINT('Ctrl Pts',(-24.786966358124,49.4838398214064,-213.634371448189));
#225830=CARTESIAN_POINT('Ctrl Pts',(-25.2356860399355,49.4352084231262,
-213.57567222148));
#225831=CARTESIAN_POINT('Ctrl Pts',(-28.0133620326269,49.1341691039938,
-213.212310774616));
#225832=CARTESIAN_POINT('Ctrl Pts',(-30.9016860171707,48.7536932160381,
-213.450145604589));
#225833=CARTESIAN_POINT('Ctrl Pts',(-33.4676027871724,48.3558414255462,
-214.55197396609));
#225834=CARTESIAN_POINT('Ctrl Pts',(-23.1985904601668,37.1455480181648,
-232.850246331936));
#225835=CARTESIAN_POINT('Ctrl Pts',(-22.1564545595563,37.2602774694449,
-232.514130204924));
#225836=CARTESIAN_POINT('Ctrl Pts',(-21.0641804092463,37.3724708937409,
-232.345177904713));
#225837=CARTESIAN_POINT('Ctrl Pts',(-19.9681071327435,37.4761722827196,
-232.313659235738));
#225838=CARTESIAN_POINT('Ctrl Pts',(-19.2991366874209,37.5394647339204,
-232.294422330258));
#225839=CARTESIAN_POINT('Ctrl Pts',(-18.6376856229304,37.5985673286038,
-232.329772980603));
#225840=CARTESIAN_POINT('Ctrl Pts',(-18.0769455458819,37.64655661213,-232.388919611448));
#225841=CARTESIAN_POINT('Ctrl Pts',(-17.9570080780068,37.6568211061209,
-232.401570565833));
#225842=CARTESIAN_POINT('Ctrl Pts',(-17.8401560569646,37.6667188889414,
-232.41533436964));
#225843=CARTESIAN_POINT('Ctrl Pts',(-17.72605548882,37.6762929544425,-232.430022763024));
#225844=CARTESIAN_POINT('Ctrl Pts',(-17.4149087979919,37.7024009646557,
-232.470077296226));
#225845=CARTESIAN_POINT('Ctrl Pts',(-17.1241467866706,37.7261173291054,
-232.516791489072));
#225846=CARTESIAN_POINT('Ctrl Pts',(-16.8475890215201,37.7481654899999,
-232.567875869631));
#225847=CARTESIAN_POINT('Ctrl Pts',(-16.6967373793616,37.7601919152052,
-232.595740437786));
#225848=CARTESIAN_POINT('Ctrl Pts',(-16.5501315589411,37.7717180670409,
-232.624939985054));
#225849=CARTESIAN_POINT('Ctrl Pts',(-16.4068314221588,37.7828417554715,
-232.655316959781));
#225850=CARTESIAN_POINT('Ctrl Pts',(-16.3324722176574,37.7886138966669,
-232.67107973382));
#225851=CARTESIAN_POINT('Ctrl Pts',(-16.259003222542,37.7942775108324,-232.687161754288));
#225852=CARTESIAN_POINT('Ctrl Pts',(-16.1862882705909,37.7998456944697,
-232.70355571365));
#225853=CARTESIAN_POINT('Ctrl Pts',(-16.1550881440824,37.802234859686,-232.710589942407));
#225854=CARTESIAN_POINT('Ctrl Pts',(-16.1240153770202,37.8046073304442,
-232.717626099841));
#225855=CARTESIAN_POINT('Ctrl Pts',(-16.0930261937342,37.8069665902894,
-232.724502972898));
#225856=CARTESIAN_POINT('Ctrl Pts',(-16.063092214273,37.8092455156518,-232.731145683515));
#225857=CARTESIAN_POINT('Ctrl Pts',(-16.0332453620651,37.8115114139419,
-232.737684631239));
#225858=CARTESIAN_POINT('Ctrl Pts',(-16.003476624031,37.8137650756407,-232.744122743264));
#225859=CARTESIAN_POINT('Ctrl Pts',(-15.824134731135,37.827342270433,-232.782909177407));
#225860=CARTESIAN_POINT('Ctrl Pts',(-15.6476298224866,37.8404768185726,
-232.818057012347));
#225861=CARTESIAN_POINT('Ctrl Pts',(-15.4720288026693,37.853326932794,-232.850049999999));
#225862=CARTESIAN_POINT('',(-2.58126937689227,38.4029617620279,-232.850050996336));
#225863=CARTESIAN_POINT('Ctrl Pts',(-10.3603804086809,38.1653654608598,
-232.850050113495));
#225864=CARTESIAN_POINT('Ctrl Pts',(-9.71419790368592,38.196982639096,-232.721004312897));
#225865=CARTESIAN_POINT('Ctrl Pts',(-9.35549486807857,38.2135078924852,
-232.595584405869));
#225866=CARTESIAN_POINT('Ctrl Pts',(-7.88550439629379,38.2731624675052,
-232.364954948601));
#225867=CARTESIAN_POINT('Ctrl Pts',(-7.16548125236048,38.2987680162378,
-232.312392715194));
#225868=CARTESIAN_POINT('Ctrl Pts',(-5.68487376001899,38.3438073799782,
-232.321825074893));
#225869=CARTESIAN_POINT('Ctrl Pts',(-4.92650521021758,38.3627520068666,
-232.390644239872));
#225870=CARTESIAN_POINT('Ctrl Pts',(-3.50691587437607,38.3907272609826,
-232.631934382068));
#225871=CARTESIAN_POINT('Ctrl Pts',(-3.19597628779658,38.3954757183434,
-232.732911385662));
#225872=CARTESIAN_POINT('Ctrl Pts',(-2.58126982511239,38.4029609689687,
-232.850053829461));
#225873=CARTESIAN_POINT('',(2.58126928063572,38.4029617514691,-232.850050981496));
#225874=CARTESIAN_POINT('Ctrl Pts',(-2.58126959429465,38.4029635779833,
-232.85005));
#225875=CARTESIAN_POINT('Ctrl Pts',(-1.72249329171046,38.5235335172581,
-232.85005));
#225876=CARTESIAN_POINT('Ctrl Pts',(-0.867273575857391,38.583205095121,
-232.85005));
#225877=CARTESIAN_POINT('Ctrl Pts',(0.867251683657016,38.583206657092,-232.85005));
#225878=CARTESIAN_POINT('Ctrl Pts',(1.72248215657025,38.5235349591089,-232.85005));
#225879=CARTESIAN_POINT('Ctrl Pts',(2.58126949479989,38.4029635403769,-232.85005));
#225880=CARTESIAN_POINT('',(10.3603804821857,38.1653654824018,-232.850050038668));
#225881=CARTESIAN_POINT('Ctrl Pts',(10.3603804658313,38.1653654580635,-232.850050114597));
#225882=CARTESIAN_POINT('Ctrl Pts',(9.71419795896007,38.1969826365663,-232.721004310544));
#225883=CARTESIAN_POINT('Ctrl Pts',(9.35549489011901,38.2135078916454,-232.595584392477));
#225884=CARTESIAN_POINT('Ctrl Pts',(7.88550438721803,38.2731624678223,-232.364954942449));
#225885=CARTESIAN_POINT('Ctrl Pts',(7.16548124909485,38.2987680163253,-232.312392716592));
#225886=CARTESIAN_POINT('Ctrl Pts',(5.68487373797052,38.3438073806628,-232.321825087222));
#225887=CARTESIAN_POINT('Ctrl Pts',(4.9265051676737,38.3627520079171,-232.390644261604));
#225888=CARTESIAN_POINT('Ctrl Pts',(3.50691613666394,38.3907272556243,-232.631934364075));
#225889=CARTESIAN_POINT('Ctrl Pts',(3.19597714514061,38.3954757082021,-232.732911221419));
#225890=CARTESIAN_POINT('Ctrl Pts',(2.58126972217957,38.4029609702222,-232.850053772423));
#225891=CARTESIAN_POINT('',(15.4720289242324,37.8533269238987,-232.85005));
#225892=CARTESIAN_POINT('Ctrl Pts',(10.3603804783137,38.1653655319544,-232.85005));
#225893=CARTESIAN_POINT('Ctrl Pts',(11.193556676016,38.2304686654651,-232.85005));
#225894=CARTESIAN_POINT('Ctrl Pts',(12.0312562221273,38.2388535343039,-232.85005));
#225895=CARTESIAN_POINT('Ctrl Pts',(13.7409536714611,38.140257937513,-232.85005));
#225896=CARTESIAN_POINT('Ctrl Pts',(14.613269214461,38.0271219437723,-232.85005));
#225897=CARTESIAN_POINT('Ctrl Pts',(15.4720289242322,37.8533269238976,-232.85005));
#225898=CARTESIAN_POINT('Ctrl Pts',(23.1985903050735,37.1455480352391,-232.850246269746));
#225899=CARTESIAN_POINT('Ctrl Pts',(22.0455775581368,37.2724839932101,-232.478369482393));
#225900=CARTESIAN_POINT('Ctrl Pts',(20.8316287206699,37.3962101542244,-232.311280498896));
#225901=CARTESIAN_POINT('Ctrl Pts',(19.6181202835508,37.5089924027573,-232.30820532281));
#225902=CARTESIAN_POINT('Ctrl Pts',(18.9222079202927,37.5736697949445,-232.306441797323));
#225903=CARTESIAN_POINT('Ctrl Pts',(18.2806146166533,37.6297604507304,-232.358633251125));
#225904=CARTESIAN_POINT('Ctrl Pts',(17.7260544830199,37.6762930388382,-232.430022919809));
#225905=CARTESIAN_POINT('Ctrl Pts',(17.4149077894093,37.7024010477931,-232.470077474801));
#225906=CARTESIAN_POINT('Ctrl Pts',(17.1241457734926,37.7261174112266,-232.516791687499));
#225907=CARTESIAN_POINT('Ctrl Pts',(16.8475879986799,37.7481655715443,-232.567876087736));
#225908=CARTESIAN_POINT('Ctrl Pts',(16.6967363558847,37.7601919960656,-232.59574066577));
#225909=CARTESIAN_POINT('Ctrl Pts',(16.5501305330696,37.7717181473772,-232.624940222784));
#225910=CARTESIAN_POINT('Ctrl Pts',(16.4068303915331,37.7828418354739,-232.655317207503));
#225911=CARTESIAN_POINT('Ctrl Pts',(16.3324711865191,37.7886139763443,-232.671079986313));
#225912=CARTESIAN_POINT('Ctrl Pts',(16.2590021902051,37.794277590242,-232.687162011602));
#225913=CARTESIAN_POINT('Ctrl Pts',(16.1862872362639,37.7998457736738,-232.7035559759));
#225914=CARTESIAN_POINT('Ctrl Pts',(16.1550871799105,37.8022349333644,-232.710590190766));
#225915=CARTESIAN_POINT('Ctrl Pts',(16.1240144811553,37.80460739877,-232.71762632881));
#225916=CARTESIAN_POINT('Ctrl Pts',(16.0930253659941,37.8069666533067,-232.724503184806));
#225917=CARTESIAN_POINT('Ctrl Pts',(16.0630913871853,37.8092455785015,-232.7311458934));
#225918=CARTESIAN_POINT('Ctrl Pts',(16.0332445354967,37.8115114766347,-232.73768483914));
#225919=CARTESIAN_POINT('Ctrl Pts',(16.0034757978481,37.8137651381874,-232.744122949218));
#225920=CARTESIAN_POINT('Ctrl Pts',(15.8241342326628,37.8273423074652,-232.782909301255));
#225921=CARTESIAN_POINT('Ctrl Pts',(15.6476296366115,37.840476832073,-232.818057068527));
#225922=CARTESIAN_POINT('Ctrl Pts',(15.4720289242322,37.8533269238983,-232.850049999999));
#225923=CARTESIAN_POINT('Origin',(22.9178089794592,-52.5372975341153,-234.75005));
#225924=CARTESIAN_POINT('',(27.0625191140422,-59.958306757953,-232.85005));
#225925=CARTESIAN_POINT('',(23.2057914601203,-61.0324176680998,-232.85005));
#225926=CARTESIAN_POINT('Origin',(22.9178089794592,-52.5372975341153,-232.85005));
#225927=CARTESIAN_POINT('',(27.0625191140422,-59.958306757953,-232.25005));
#225928=CARTESIAN_POINT('',(27.0625191140422,-59.958306757953,-234.75005));
#225929=CARTESIAN_POINT('',(23.2057914601203,-61.0324176680998,-232.25005));
#225930=CARTESIAN_POINT('Origin',(22.9178089794592,-52.5372975341153,-232.25005));
#225931=CARTESIAN_POINT('',(23.2057914601203,-61.0324176680998,-234.75005));
#225932=CARTESIAN_POINT('Origin',(7.14692237356698E-14,623.509175991979,
-234.75005));
#225933=CARTESIAN_POINT('Origin',(7.14692237356698E-14,623.509175991979,
-232.25005));
#225934=CARTESIAN_POINT('Origin',(7.14692237356698E-14,623.509175991979,
-232.85005));
#225935=CARTESIAN_POINT('Origin',(-2.61456814389029E-14,-173.57701443073,
-234.75005));
#225936=CARTESIAN_POINT('',(25.8757946403502,36.8335750748777,-232.25005));
#225937=CARTESIAN_POINT('Origin',(-2.61456814389029E-14,-173.57701443073,
-232.25005));
#225938=CARTESIAN_POINT('',(25.8757946403502,36.8335750748777,-232.85005));
#225939=CARTESIAN_POINT('',(25.8757946403502,36.8335750748777,-234.75005));
#225940=CARTESIAN_POINT('Origin',(-2.61456814389029E-14,-173.57701443073,
-232.85005));
#225941=CARTESIAN_POINT('Origin',(-2.61456814389029E-14,-173.57701443073,
-232.85005));
#225942=CARTESIAN_POINT('Origin',(-2.61456814389029E-14,-173.57701443073,
-232.85005));
#225943=CARTESIAN_POINT('Origin',(24.838300653577,28.3971299569735,-234.75005));
#225944=CARTESIAN_POINT('',(29.3303337505005,35.613198045354,-232.85005));
#225945=CARTESIAN_POINT('Origin',(24.838300653577,28.3971299569735,-232.85005));
#225946=CARTESIAN_POINT('',(29.3303337505005,35.613198045354,-232.25005));
#225947=CARTESIAN_POINT('Origin',(24.838300653577,28.3971299569735,-232.25005));
#225948=CARTESIAN_POINT('',(29.3303337505005,35.613198045354,-234.75005));
#225949=CARTESIAN_POINT('Origin',(-6.29739814579425E-15,-11.5034818258363,
-234.75005));
#225950=CARTESIAN_POINT('',(46.0422390557602,19.4862297367486,-232.85005));
#225951=CARTESIAN_POINT('Origin',(-6.29739814579425E-15,-11.5034818258363,
-232.85005));
#225952=CARTESIAN_POINT('',(46.0422390557602,19.4862297367486,-232.25005));
#225953=CARTESIAN_POINT('Origin',(-6.29739814579425E-15,-11.5034818258363,
-232.25005));
#225954=CARTESIAN_POINT('',(46.0422390557602,19.4862297367486,-234.75005));
#225955=CARTESIAN_POINT('Origin',(38.9907249661392,14.740057695632,-234.75005));
#225956=CARTESIAN_POINT('',(47.4843254762175,15.0698309134599,-232.85005));
#225957=CARTESIAN_POINT('Origin',(38.9907249661392,14.740057695632,-232.85005));
#225958=CARTESIAN_POINT('',(47.4843254762175,15.0698309134599,-232.25005));
#225959=CARTESIAN_POINT('Origin',(38.9907249661392,14.740057695632,-232.25005));
#225960=CARTESIAN_POINT('',(47.4843254762175,15.0698309134599,-234.75005));
#225961=CARTESIAN_POINT('Origin',(-636.934816028482,-11.5034818258361,-234.75005));
#225962=CARTESIAN_POINT('',(47.7644117008771,6.45952891261178,-232.25005));
#225963=CARTESIAN_POINT('Origin',(-636.934816028482,-11.5034818258361,-232.25005));
#225964=CARTESIAN_POINT('',(47.7015217244055,8.71393886986192,-232.849988375574));
#225965=CARTESIAN_POINT('Ctrl Pts',(47.764411700877,6.45952891261171,-232.250050000001));
#225966=CARTESIAN_POINT('Ctrl Pts',(47.7539918567994,6.85670393504417,-232.299135434164));
#225967=CARTESIAN_POINT('Ctrl Pts',(47.7432936090854,7.25119812638128,-232.373336512398));
#225968=CARTESIAN_POINT('Ctrl Pts',(47.7222110876844,8.00529930166126,-232.573920981311));
#225969=CARTESIAN_POINT('Ctrl Pts',(47.7118378495729,8.36566358596881,-232.697530953773));
#225970=CARTESIAN_POINT('Ctrl Pts',(47.70155338045,8.71393369956125,-232.849926751148));
#225971=CARTESIAN_POINT('Origin',(-636.934816028482,-11.5034818258361,-232.85005));
#225972=CARTESIAN_POINT('Origin',(38.9907249661392,-37.7470213473046,-234.75005));
#225973=CARTESIAN_POINT('',(47.4843254762176,-38.0767945651323,-232.85005));
#225974=CARTESIAN_POINT('',(46.0422390557601,-42.4931933884212,-232.85005));
#225975=CARTESIAN_POINT('Origin',(38.9907249661392,-37.7470213473046,-232.85005));
#225976=CARTESIAN_POINT('',(47.4843254762176,-38.0767945651323,-232.25005));
#225977=CARTESIAN_POINT('',(47.4843254762176,-38.0767945651323,-234.75005));
#225978=CARTESIAN_POINT('',(46.0422390557601,-42.4931933884212,-232.25005));
#225979=CARTESIAN_POINT('Origin',(38.9907249661392,-37.7470213473046,-232.25005));
#225980=CARTESIAN_POINT('',(46.0422390557601,-42.4931933884212,-234.75005));
#225981=CARTESIAN_POINT('Origin',(-6.29739814579425E-15,-11.5034818258363,
-234.75005));
#225982=CARTESIAN_POINT('Origin',(-6.29739814579425E-15,-11.5034818258363,
-232.85005));
#225983=CARTESIAN_POINT('Origin',(-6.29739814579425E-15,-11.5034818258363,
-232.25005));
#225984=CARTESIAN_POINT('Ctrl Pts',(47.0185565395742,-41.6609971057424,
-232.962224970815));
#225985=CARTESIAN_POINT('Ctrl Pts',(47.4683098495203,-42.4379579278734,
-232.173885913265));
#225986=CARTESIAN_POINT('Ctrl Pts',(47.9182404464189,-43.214781541947,-231.385510833981));
#225987=CARTESIAN_POINT('Ctrl Pts',(48.3683681238743,-43.9914549619569,
-230.597098052473));
#225988=CARTESIAN_POINT('Ctrl Pts',(48.8184958013296,-44.7681283819668,
-229.808685270963));
#225989=CARTESIAN_POINT('Ctrl Pts',(49.2688205234849,-45.5446516231764,
-229.020234782073));
#225990=CARTESIAN_POINT('Ctrl Pts',(49.7193651569502,-46.321010055599,-228.231745013587));
#225991=CARTESIAN_POINT('Ctrl Pts',(50.6204544238808,-47.8737269204442,
-226.654765476616));
#225992=CARTESIAN_POINT('Ctrl Pts',(51.5224188067103,-49.4257867780962,
-225.077628467932));
#225993=CARTESIAN_POINT('Ctrl Pts',(52.4254879069396,-50.9770488729761,
-223.500324296104));
#225994=CARTESIAN_POINT('Ctrl Pts',(54.2316261073984,-54.079573062736,-220.345715952448));
#225995=CARTESIAN_POINT('Ctrl Pts',(56.0420505223762,-57.178961519516,-217.190418744692));
#225996=CARTESIAN_POINT('Ctrl Pts',(57.8597736100785,-60.2735586547801,
-214.03449525351));
#225997=CARTESIAN_POINT('Ctrl Pts',(47.0588574073719,-41.5858000428048,
-232.968566523408));
#225998=CARTESIAN_POINT('Ctrl Pts',(47.5093207248854,-42.363022265842,-232.17977481419));
#225999=CARTESIAN_POINT('Ctrl Pts',(47.9599297574655,-43.1401459593037,
-231.39096724535));
#226000=CARTESIAN_POINT('Ctrl Pts',(48.4106907142535,-43.9171701566874,
-230.602146349555));
#226001=CARTESIAN_POINT('Ctrl Pts',(48.8614516710415,-44.6941943540713,
-229.813325453759));
#226002=CARTESIAN_POINT('Ctrl Pts',(49.3123645814213,-45.4711190318301,
-229.024491224305));
#226003=CARTESIAN_POINT('Ctrl Pts',(49.7634348829592,-46.2479443404272,
-228.235646862402));
#226004=CARTESIAN_POINT('Ctrl Pts',(50.6655754860351,-47.8015949576215,
-226.657958138597));
#226005=CARTESIAN_POINT('Ctrl Pts',(51.5683478186111,-49.3548459662596,
-225.080227999184));
#226006=CARTESIAN_POINT('Ctrl Pts',(52.4717770943224,-50.9077187028313,
-223.502491635481));
#226007=CARTESIAN_POINT('Ctrl Pts',(54.2786356457449,-54.0134641759745,
-220.347018908076));
#226008=CARTESIAN_POINT('Ctrl Pts',(56.0882389522679,-57.1176157229696,
-217.191507400736));
#226009=CARTESIAN_POINT('Ctrl Pts',(57.8999640673718,-60.2209901065118,
-214.036411889894));
#226010=CARTESIAN_POINT('Ctrl Pts',(47.0788820514615,-41.5349619911827,
-232.977219483294));
#226011=CARTESIAN_POINT('Ctrl Pts',(47.5313585913162,-42.310877567243,-232.187698020531));
#226012=CARTESIAN_POINT('Ctrl Pts',(47.9838932303251,-43.0867923470826,
-231.398208761274));
#226013=CARTESIAN_POINT('Ctrl Pts',(48.4364687519895,-43.8627275668274,
-230.608763067264));
#226014=CARTESIAN_POINT('Ctrl Pts',(48.889044273654,-44.6386627865722,-229.819317373254));
#226015=CARTESIAN_POINT('Ctrl Pts',(49.3416606701069,-45.4146183959999,
-229.029915190037));
#226016=CARTESIAN_POINT('Ctrl Pts',(49.7943023545749,-46.1906112611962,
-228.240564453713));
#226017=CARTESIAN_POINT('Ctrl Pts',(50.6995857235109,-47.7425969915886,
-226.661862981063));
#226018=CARTESIAN_POINT('Ctrl Pts',(51.6049685652275,-49.2947346592046,
-225.083369244233));
#226019=CARTESIAN_POINT('Ctrl Pts',(52.5103464401617,-50.8471174431018,
-223.505116662391));
#226020=CARTESIAN_POINT('Ctrl Pts',(54.3211021900301,-53.951883010896,-220.348611498707));
#226021=CARTESIAN_POINT('Ctrl Pts',(56.1318167680608,-57.0576530539869,
-217.193082767306));
#226022=CARTESIAN_POINT('Ctrl Pts',(57.9419471071077,-60.1647335356702,
-214.038526270145));
#226023=CARTESIAN_POINT('Ctrl Pts',(47.0912031843055,-41.4946844018168,
-232.986503298756));
#226024=CARTESIAN_POINT('Ctrl Pts',(47.5465884139282,-42.2680813083878,
-232.195931935019));
#226025=CARTESIAN_POINT('Ctrl Pts',(48.0017768129395,-43.0417829154583,
-231.40555195953));
#226026=CARTESIAN_POINT('Ctrl Pts',(48.4567760318361,-43.8157641577748,
-230.615342754576));
#226027=CARTESIAN_POINT('Ctrl Pts',(48.9117752507326,-44.5897454000911,
-229.825133549621));
#226028=CARTESIAN_POINT('Ctrl Pts',(49.366585304478,-45.364006290321,-229.035095136287));
#226029=CARTESIAN_POINT('Ctrl Pts',(49.8212141883276,-46.1385240104118,
-228.245209329223));
#226030=CARTESIAN_POINT('Ctrl Pts',(50.7304719560267,-47.6875594505935,
-226.665437715093));
#226031=CARTESIAN_POINT('Ctrl Pts',(51.6390050797513,-49.2376203690394,
-225.086274713309));
#226032=CARTESIAN_POINT('Ctrl Pts',(52.5468787652607,-50.7885482821615,
-223.507599498114));
#226033=CARTESIAN_POINT('Ctrl Pts',(54.3626261362793,-53.8904041084056,
-220.350249067725));
#226034=CARTESIAN_POINT('Ctrl Pts',(56.1757402684043,-56.9957065400334,
-217.194831063113));
#226035=CARTESIAN_POINT('Ctrl Pts',(57.9867151256432,-60.1034983677464,
-214.040672462087));
#226036=CARTESIAN_POINT('Ctrl Pts',(47.1035243171495,-41.4544068124509,
-232.995787114217));
#226037=CARTESIAN_POINT('Ctrl Pts',(47.5618182365402,-42.2252850495327,
-232.204165849507));
#226038=CARTESIAN_POINT('Ctrl Pts',(48.0196603955539,-42.9967734838342,
-231.412895157786));
#226039=CARTESIAN_POINT('Ctrl Pts',(48.4770833116826,-43.7688007487221,
-230.621922441887));
#226040=CARTESIAN_POINT('Ctrl Pts',(48.9345062278113,-44.54082801361,-229.830949725988));
#226041=CARTESIAN_POINT('Ctrl Pts',(49.391509938849,-45.313394184642,-229.040275082537));
#226042=CARTESIAN_POINT('Ctrl Pts',(49.8481260220802,-46.0864367596275,
-228.249854204732));
#226043=CARTESIAN_POINT('Ctrl Pts',(50.7613581885425,-47.6325219095984,
-226.669012449123));
#226044=CARTESIAN_POINT('Ctrl Pts',(51.6730415942752,-49.1805060788742,
-225.089180182384));
#226045=CARTESIAN_POINT('Ctrl Pts',(52.5834110903597,-50.7299791212212,
-223.510082333838));
#226046=CARTESIAN_POINT('Ctrl Pts',(54.4041500825286,-53.8289252059152,
-220.351886636744));
#226047=CARTESIAN_POINT('Ctrl Pts',(56.2196637687479,-56.9337600260798,
-217.196579358919));
#226048=CARTESIAN_POINT('Ctrl Pts',(58.0314831441787,-60.0422631998226,
-214.04281865403));
#226049=CARTESIAN_POINT('Ctrl Pts',(47.1094181844823,-41.4235916164857,
-233.005271954373));
#226050=CARTESIAN_POINT('Ctrl Pts',(47.5714574466843,-42.1907462838401,
-232.21226382723));
#226051=CARTESIAN_POINT('Ctrl Pts',(48.0325802899557,-42.9590937957815,
-231.419919822014));
#226052=CARTESIAN_POINT('Ctrl Pts',(48.4929276099559,-43.7283935879396,
-230.628080779981));
#226053=CARTESIAN_POINT('Ctrl Pts',(48.9532749299561,-44.4976933800977,
-229.836241737948));
#226054=CARTESIAN_POINT('Ctrl Pts',(49.4128465653679,-45.2679465967797,
-229.044908707219));
#226055=CARTESIAN_POINT('Ctrl Pts',(49.8717607150419,-46.0389694518266,
-228.253966129662));
#226056=CARTESIAN_POINT('Ctrl Pts',(50.7895890143898,-47.5810151619205,
-226.672080974546));
#226057=CARTESIAN_POINT('Ctrl Pts',(51.7048034669659,-49.1261109180323,
-225.091738429241));
#226058=CARTESIAN_POINT('Ctrl Pts',(52.6181227187143,-50.6732510827466,
-223.512347273439));
#226059=CARTESIAN_POINT('Ctrl Pts',(54.4447612222111,-53.7675314121752,
-220.353564961834));
#226060=CARTESIAN_POINT('Ctrl Pts',(56.2639490448981,-56.8698182307502,
-217.198492064106));
#226061=CARTESIAN_POINT('Ctrl Pts',(58.0790346309092,-59.9760499787848,
-214.044995596012));
#226062=CARTESIAN_POINT('Ctrl Pts',(47.1301259245572,-41.3776365805516,
-233.007883276788));
#226063=CARTESIAN_POINT('Ctrl Pts',(47.5942000936469,-42.1428559602882,
-232.214484939109));
#226064=CARTESIAN_POINT('Ctrl Pts',(48.0571442886842,-42.9095264965149,
-231.42188110874));
#226065=CARTESIAN_POINT('Ctrl Pts',(48.5191679953314,-43.677310151957,-230.629855880101));
#226066=CARTESIAN_POINT('Ctrl Pts',(48.9811917019786,-44.445093807399,-229.837830651463));
#226067=CARTESIAN_POINT('Ctrl Pts',(49.4422942329435,-45.2139930242057,
-229.046386055781));
#226068=CARTESIAN_POINT('Ctrl Pts',(49.9026408989544,-45.9837637819335,
-228.255374275861));
#226069=CARTESIAN_POINT('Ctrl Pts',(50.8233342309762,-47.5233052973892,
-226.673350716021));
#226070=CARTESIAN_POINT('Ctrl Pts',(51.7410289944696,-49.0662933806299,
-225.093033330561));
#226071=CARTESIAN_POINT('Ctrl Pts',(52.6566611088264,-50.611475717687,-223.51371347964));
#226072=CARTESIAN_POINT('Ctrl Pts',(54.4879253375398,-53.7018403918012,
-220.355073777797));
#226073=CARTESIAN_POINT('Ctrl Pts',(56.3111024468989,-56.8007837303405,
-217.200320668143));
#226074=CARTESIAN_POINT('Ctrl Pts',(58.1301468566089,-59.9036654708269,
-214.047106057761));
#226075=CARTESIAN_POINT('Ctrl Pts',(47.171541404707,-41.2857265086834,-233.01310592162));
#226076=CARTESIAN_POINT('Ctrl Pts',(47.639685387572,-42.0470753131842,-232.218927162867));
#226077=CARTESIAN_POINT('Ctrl Pts',(48.1062722861412,-42.8103918979816,
-231.425803682192));
#226078=CARTESIAN_POINT('Ctrl Pts',(48.5716487660823,-43.5751432799917,
-230.633406080342));
#226079=CARTESIAN_POINT('Ctrl Pts',(49.0370252460235,-44.3398946620018,
-229.841008478492));
#226080=CARTESIAN_POINT('Ctrl Pts',(49.5011895680945,-45.1060858790577,
-229.049340752905));
#226081=CARTESIAN_POINT('Ctrl Pts',(49.9644012667793,-45.8733524421474,
-228.25819056826));
#226082=CARTESIAN_POINT('Ctrl Pts',(50.8908246641489,-47.4078855683268,
-226.675890198969));
#226083=CARTESIAN_POINT('Ctrl Pts',(51.8134800494771,-48.9466583058251,
-225.095623133202));
#226084=CARTESIAN_POINT('Ctrl Pts',(52.7337378890505,-50.4879249875678,
-223.516445892042));
#226085=CARTESIAN_POINT('Ctrl Pts',(54.5742535681973,-53.5704583510531,
-220.358091409721));
#226086=CARTESIAN_POINT('Ctrl Pts',(56.4054092509004,-56.6627147295212,
-217.203977876217));
#226087=CARTESIAN_POINT('Ctrl Pts',(58.2323713080084,-59.7588964549113,
-214.051326981263));
#226088=CARTESIAN_POINT('Ctrl Pts',(47.2037604911033,-41.2022757926265,
-233.020733994064));
#226089=CARTESIAN_POINT('Ctrl Pts',(47.6765307304169,-41.9587290407164,
-232.2257873802));
#226090=CARTESIAN_POINT('Ctrl Pts',(48.1471647665248,-42.7177804449826,
-231.432193257086));
#226091=CARTESIAN_POINT('Ctrl Pts',(48.6161649822748,-43.4787209967311,
-230.639525123807));
#226092=CARTESIAN_POINT('Ctrl Pts',(49.0851651980248,-44.2396615484797,
-229.846856990528));
#226093=CARTESIAN_POINT('Ctrl Pts',(49.5525384413198,-45.0024830404561,
-229.055111557421));
#226094=CARTESIAN_POINT('Ctrl Pts',(50.0187056640015,-45.76663525977,-228.263983251877));
#226095=CARTESIAN_POINT('Ctrl Pts',(50.9510401093651,-47.2949396983977,
-226.68172664079));
#226096=CARTESIAN_POINT('Ctrl Pts',(51.8786366079818,-48.8284550182444,
-225.101877330191));
#226097=CARTESIAN_POINT('Ctrl Pts',(52.8035983099936,-50.3646700206687,
-223.523161428396));
#226098=CARTESIAN_POINT('Ctrl Pts',(54.6535217140174,-53.4371000255173,
-220.365729624806));
#226099=CARTESIAN_POINT('Ctrl Pts',(56.4932286367666,-56.5200179818056,
-217.212714221123));
#226100=CARTESIAN_POINT('Ctrl Pts',(58.3292814169375,-59.6063766654718,
-214.060952327901));
#226101=CARTESIAN_POINT('Ctrl Pts',(47.2184619313714,-41.1386068777002,
-233.034226791445));
#226102=CARTESIAN_POINT('Ctrl Pts',(47.6994633038231,-41.8843414973674,
-232.236899734718));
#226103=CARTESIAN_POINT('Ctrl Pts',(48.1764662990288,-42.6351364657344,
-231.442184400327));
#226104=CARTESIAN_POINT('Ctrl Pts',(48.6511105129755,-43.3886793381388,
-230.648777192266));
#226105=CARTESIAN_POINT('Ctrl Pts',(49.1257547269221,-44.1422222105431,
-229.855369984204));
#226106=CARTESIAN_POINT('Ctrl Pts',(49.5980020098404,-44.8985826028918,
-229.063316695606));
#226107=CARTESIAN_POINT('Ctrl Pts',(50.0687290729088,-45.6566352866088,
-228.272029084797));
#226108=CARTESIAN_POINT('Ctrl Pts',(51.0101831990457,-47.1727406540429,
-226.689453863181));
#226109=CARTESIAN_POINT('Ctrl Pts',(51.9456932760972,-48.695455984225,-225.109865596097));
#226110=CARTESIAN_POINT('Ctrl Pts',(52.8784745199465,-50.2209883221406,
-223.531433290935));
#226111=CARTESIAN_POINT('Ctrl Pts',(54.7440370076451,-53.2720529979718,
-220.374568680612));
#226112=CARTESIAN_POINT('Ctrl Pts',(56.5988680832651,-56.3342829748578,
-217.222334895439));
#226113=CARTESIAN_POINT('Ctrl Pts',(58.4505854057776,-59.3994904876393,
-214.071174978969));
#226114=CARTESIAN_POINT('Ctrl Pts',(47.2331633716395,-41.074937962774,-233.047719588827));
#226115=CARTESIAN_POINT('Ctrl Pts',(47.7223958772293,-41.8099539540185,
-232.248012089236));
#226116=CARTESIAN_POINT('Ctrl Pts',(48.2057678315329,-42.5524924864862,
-231.452175543568));
#226117=CARTESIAN_POINT('Ctrl Pts',(48.6860560436761,-43.2986376795464,
-230.658029260724));
#226118=CARTESIAN_POINT('Ctrl Pts',(49.1663442558194,-44.0447828726065,
-229.86388297788));
#226119=CARTESIAN_POINT('Ctrl Pts',(49.6434655783611,-44.7946821653274,
-229.071521833792));
#226120=CARTESIAN_POINT('Ctrl Pts',(50.1187524818162,-45.5466353134476,
-228.280074917719));
#226121=CARTESIAN_POINT('Ctrl Pts',(51.0693262887264,-47.0505416096881,
-226.697181085572));
#226122=CARTESIAN_POINT('Ctrl Pts',(52.0127499442126,-48.5624569502057,
-225.117853862002));
#226123=CARTESIAN_POINT('Ctrl Pts',(52.9533507298994,-50.0773066236126,
-223.539705153474));
#226124=CARTESIAN_POINT('Ctrl Pts',(54.8345523012729,-53.1070059704263,
-220.383407736418));
#226125=CARTESIAN_POINT('Ctrl Pts',(56.7045075297636,-56.1485479679101,
-217.231955569755));
#226126=CARTESIAN_POINT('Ctrl Pts',(58.5718893946176,-59.1926043098068,
-214.081397630038));
#226127=CARTESIAN_POINT('Ctrl Pts',(47.2442225930031,-41.0165984906687,
-233.060484538427));
#226128=CARTESIAN_POINT('Ctrl Pts',(47.7410879851243,-41.7396655945174,
-232.258993064984));
#226129=CARTESIAN_POINT('Ctrl Pts',(48.2304947549091,-42.4727467259007,
-231.46264144105));
#226130=CARTESIAN_POINT('Ctrl Pts',(48.7165337536793,-43.2098774487494,
-230.66815609265));
#226131=CARTESIAN_POINT('Ctrl Pts',(49.2025727524494,-43.9470081715982,
-229.873670744249));
#226132=CARTESIAN_POINT('Ctrl Pts',(49.6850684896479,-44.6884971892255,
-229.081242904766));
#226133=CARTESIAN_POINT('Ctrl Pts',(50.1656830825472,-45.4321663014423,
-228.289778191998));
#226134=CARTESIAN_POINT('Ctrl Pts',(51.1269122683457,-46.9195045258758,
-226.706848766463));
#226135=CARTESIAN_POINT('Ctrl Pts',(52.0807938880043,-48.415379750843,-225.127702010668));
#226136=CARTESIAN_POINT('Ctrl Pts',(53.0320528840148,-49.9140824163154,
-223.549690567007));
#226137=CARTESIAN_POINT('Ctrl Pts',(54.9345708760356,-52.9114877472602,
-220.393667679684));
#226138=CARTESIAN_POINT('Ctrl Pts',(56.8264228500083,-55.9205802770675,
-217.24244325845));
#226139=CARTESIAN_POINT('Ctrl Pts',(58.7160309997225,-58.9319583435186,
-214.092043625716));
#226140=CARTESIAN_POINT('Ctrl Pts',(47.2640162261029,-40.9447914059068,
-233.067937997558));
#226141=CARTESIAN_POINT('Ctrl Pts',(47.7628369926546,-41.6622203630557,
-232.268067857029));
#226142=CARTESIAN_POINT('Ctrl Pts',(48.2549965369399,-42.3887167282325,
-231.472771264582));
#226143=CARTESIAN_POINT('Ctrl Pts',(48.7442220365055,-43.1188281595447,
-230.679129004258));
#226144=CARTESIAN_POINT('Ctrl Pts',(49.2334475360712,-43.8489395908569,
-229.885486743933));
#226145=CARTESIAN_POINT('Ctrl Pts',(49.7195709178301,-44.5829547593942,
-229.093671052645));
#226146=CARTESIAN_POINT('Ctrl Pts',(50.2040684510243,-45.3189094985237,
-228.302711021656));
#226147=CARTESIAN_POINT('Ctrl Pts',(51.1730635174128,-46.7908189767828,
-226.720790959677));
#226148=CARTESIAN_POINT('Ctrl Pts',(52.1357048103052,-48.2703270275798,
-225.142232468079));
#226149=CARTESIAN_POINT('Ctrl Pts',(53.0961142063379,-49.7523323833611,
-223.564687821978));
#226150=CARTESIAN_POINT('Ctrl Pts',(55.0169329984032,-52.7163430949238,
-220.409598529776));
#226151=CARTESIAN_POINT('Ctrl Pts',(56.9286455988057,-55.6906960308185,
-217.258791511269));
#226152=CARTESIAN_POINT('Ctrl Pts',(58.8384812385968,-58.6670561134909,
-214.108729566325));
#226153=CARTESIAN_POINT('Ctrl Pts',(47.2838098592026,-40.8729843211449,
-233.075391456688));
#226154=CARTESIAN_POINT('Ctrl Pts',(47.7845860001848,-41.584775131594,-232.277142649072));
#226155=CARTESIAN_POINT('Ctrl Pts',(48.2794983189707,-42.3046867305642,
-231.482901088115));
#226156=CARTESIAN_POINT('Ctrl Pts',(48.7719103193318,-43.02777887034,-230.690101915866));
#226157=CARTESIAN_POINT('Ctrl Pts',(49.2643223196929,-43.7508710101157,
-229.897302743617));
#226158=CARTESIAN_POINT('Ctrl Pts',(49.7540733460123,-44.4774123295628,
-229.106099200524));
#226159=CARTESIAN_POINT('Ctrl Pts',(50.2424538195015,-45.2056526956051,
-228.315643851313));
#226160=CARTESIAN_POINT('Ctrl Pts',(51.2192147664799,-46.6621334276898,
-226.734733152891));
#226161=CARTESIAN_POINT('Ctrl Pts',(52.1906157326061,-48.1252743043166,
-225.156762925491));
#226162=CARTESIAN_POINT('Ctrl Pts',(53.160175528661,-49.5905823504069,-223.57968507695));
#226163=CARTESIAN_POINT('Ctrl Pts',(55.0992951207707,-52.5211984425875,
-220.425529379868));
#226164=CARTESIAN_POINT('Ctrl Pts',(57.0308683476032,-55.4608117845694,
-217.275139764089));
#226165=CARTESIAN_POINT('Ctrl Pts',(58.960931477471,-58.4021538834631,-214.125415506933));
#226166=CARTESIAN_POINT('Ctrl Pts',(47.2969979727536,-40.8060289412791,
-233.085985533281));
#226167=CARTESIAN_POINT('Ctrl Pts',(47.8004278329226,-41.5103244226814,
-232.28875968809));
#226168=CARTESIAN_POINT('Ctrl Pts',(48.2986559156506,-42.2220372798219,
-231.495168009573));
#226169=CARTESIAN_POINT('Ctrl Pts',(48.7946878038133,-42.9366432257674,
-230.702889499098));
#226170=CARTESIAN_POINT('Ctrl Pts',(49.2907196919761,-43.6512491717128,
-229.910610988623));
#226171=CARTESIAN_POINT('Ctrl Pts',(49.7844091161609,-44.3689959246396,
-229.119784028342));
#226172=CARTESIAN_POINT('Ctrl Pts',(50.2768976831464,-45.088287213268,-228.329639845834));
#226173=CARTESIAN_POINT('Ctrl Pts',(51.2618748171174,-46.5268697905249,
-226.749351480816));
#226174=CARTESIAN_POINT('Ctrl Pts',(52.2421543662867,-47.9715077333147,
-225.171746235109));
#226175=CARTESIAN_POINT('Ctrl Pts',(53.2208294063969,-49.4181128068083,
-223.594959717073));
#226176=CARTESIAN_POINT('Ctrl Pts',(55.1781794866173,-52.3113229537955,
-220.441386681001));
#226177=CARTESIAN_POINT('Ctrl Pts',(57.1289452771368,-55.2127036344464,
-217.291264707778));
#226178=CARTESIAN_POINT('Ctrl Pts',(59.078404570546,-58.1156526803525,-214.141757511623));
#226179=CARTESIAN_POINT('Ctrl Pts',(47.3009006987844,-40.7491010613005,
-233.101301752625));
#226180=CARTESIAN_POINT('Ctrl Pts',(47.8070153253589,-41.445066041129,-232.304686649286));
#226181=CARTESIAN_POINT('Ctrl Pts',(48.3084583519731,-42.1479407187119,
-231.511460238167));
#226182=CARTESIAN_POINT('Ctrl Pts',(48.8079303323174,-42.8535202192507,
-230.719470612188));
#226183=CARTESIAN_POINT('Ctrl Pts',(49.3074023126618,-43.5590997197895,
-229.92748098621));
#226184=CARTESIAN_POINT('Ctrl Pts',(49.8047715089351,-44.2676134042324,
-229.136855227393));
#226185=CARTESIAN_POINT('Ctrl Pts',(50.3010627023117,-44.9775733943649,
-228.346875024182));
#226186=CARTESIAN_POINT('Ctrl Pts',(51.293645089065,-46.3974933746299,-226.766914617761));
#226187=CARTESIAN_POINT('Ctrl Pts',(52.2820103247895,-47.8230831255928,
-225.189490258971));
#226188=CARTESIAN_POINT('Ctrl Pts',(53.2689347752898,-49.2505213363517,
-223.612847133253));
#226189=CARTESIAN_POINT('Ctrl Pts',(55.2427836762905,-52.1053977578695,
-220.459560881818));
#226190=CARTESIAN_POINT('Ctrl Pts',(57.2107204090195,-54.9679461288674,
-217.309560330918));
#226191=CARTESIAN_POINT('Ctrl Pts',(59.1774846171821,-57.8319751776559,
-214.160152831317));
#226192=CARTESIAN_POINT('Ctrl Pts',(47.3048034248152,-40.692173181322,-233.11661797197));
#226193=CARTESIAN_POINT('Ctrl Pts',(47.8136028177951,-41.3798076595766,
-232.320613610482));
#226194=CARTESIAN_POINT('Ctrl Pts',(48.3182607882955,-42.0738441576018,
-231.527752466761));
#226195=CARTESIAN_POINT('Ctrl Pts',(48.8211728608215,-42.770397212734,-230.736051725279));
#226196=CARTESIAN_POINT('Ctrl Pts',(49.3240849333475,-43.4669502678662,
-229.944350983796));
#226197=CARTESIAN_POINT('Ctrl Pts',(49.8251339017092,-44.1662308838252,
-229.153926426443));
#226198=CARTESIAN_POINT('Ctrl Pts',(50.325227721477,-44.8668595754618,-228.364110202531));
#226199=CARTESIAN_POINT('Ctrl Pts',(51.3254153610126,-46.2681169587348,
-226.784477754705));
#226200=CARTESIAN_POINT('Ctrl Pts',(52.3218662832923,-47.674658517871,-225.207234282834));
#226201=CARTESIAN_POINT('Ctrl Pts',(53.3170401441828,-49.0829298658951,
-223.630734549434));
#226202=CARTESIAN_POINT('Ctrl Pts',(55.3073878659637,-51.8994725619434,
-220.477735082634));
#226203=CARTESIAN_POINT('Ctrl Pts',(57.2924955409022,-54.7231886232885,
-217.327855954057));
#226204=CARTESIAN_POINT('Ctrl Pts',(59.2765646638181,-57.5482976749593,
-214.178548151011));
#226205=CARTESIAN_POINT('Ctrl Pts',(47.3080516727752,-40.6337213157799,
-233.131438257577));
#226206=CARTESIAN_POINT('Ctrl Pts',(47.8183168860115,-41.3141454117954,
-232.336628860671));
#226207=CARTESIAN_POINT('Ctrl Pts',(48.3251567152684,-42.0000633572803,
-231.544500449812));
#226208=CARTESIAN_POINT('Ctrl Pts',(48.8305551087238,-42.688161659062,-230.753383167905));
#226209=CARTESIAN_POINT('Ctrl Pts',(49.3359535021791,-43.3762599608436,
-229.962265885999));
#226210=CARTESIAN_POINT('Ctrl Pts',(49.8398128115685,-44.0667165790755,
-229.172255055445));
#226211=CARTESIAN_POINT('Ctrl Pts',(50.3428831683021,-44.7583456287819,
-228.382778415603));
#226212=CARTESIAN_POINT('Ctrl Pts',(51.3490238817693,-46.1416037281948,
-226.803825135918));
#226213=CARTESIAN_POINT('Ctrl Pts',(52.3520777883286,-47.5294564292592,
-225.226968306426));
#226214=CARTESIAN_POINT('Ctrl Pts',(53.3540764188403,-48.9188259619783,
-223.65077630667));
#226215=CARTESIAN_POINT('Ctrl Pts',(55.3580736798637,-51.6975650274167,
-220.498392307158));
#226216=CARTESIAN_POINT('Ctrl Pts',(57.35774124088,-54.4825830356932,-217.348785724916));
#226217=CARTESIAN_POINT('Ctrl Pts',(59.3565528325338,-57.2688342364512,
-214.199700145503));
#226218=CARTESIAN_POINT('Ctrl Pts',(47.3143897740156,-40.5659557077008,
-233.143618951735));
#226219=CARTESIAN_POINT('Ctrl Pts',(47.8252832097387,-41.239862847313,-232.350527479362));
#226220=CARTESIAN_POINT('Ctrl Pts',(48.3335556171132,-41.9180591247534,
-231.559510554001));
#226221=CARTESIAN_POINT('Ctrl Pts',(48.84072766068,-42.5979714018469,-230.769289654088));
#226222=CARTESIAN_POINT('Ctrl Pts',(49.3478997042467,-43.2778836789405,
-229.979068754174));
#226223=CARTESIAN_POINT('Ctrl Pts',(49.853896141919,-43.9596488205701,-229.189715484531));
#226224=CARTESIAN_POINT('Ctrl Pts',(50.3592905012865,-44.6423395873253,
-228.400785431186));
#226225=CARTESIAN_POINT('Ctrl Pts',(51.3700792200214,-46.0077211208357,
-226.822925324494));
#226226=CARTESIAN_POINT('Ctrl Pts',(52.3785121216331,-47.3767293468831,
-225.246725326938));
#226227=CARTESIAN_POINT('Ctrl Pts',(53.3861409718259,-48.7469431347296,
-223.67105962423));
#226228=CARTESIAN_POINT('Ctrl Pts',(55.4013986722116,-51.4873707104227,
-220.519728218813));
#226229=CARTESIAN_POINT('Ctrl Pts',(57.4133569116451,-54.2327814391975,
-217.37062149599));
#226230=CARTESIAN_POINT('Ctrl Pts',(59.4246687676614,-56.9791795051587,
-214.221940194738));
#226231=CARTESIAN_POINT('Ctrl Pts',(47.320727875256,-40.4981900996217,-233.155799645893));
#226232=CARTESIAN_POINT('Ctrl Pts',(47.8322495334659,-41.1655802828307,
-232.364426098052));
#226233=CARTESIAN_POINT('Ctrl Pts',(48.3419545189581,-41.8360548922265,
-231.574520658189));
#226234=CARTESIAN_POINT('Ctrl Pts',(48.8509002126362,-42.507781144632,-230.785196140269));
#226235=CARTESIAN_POINT('Ctrl Pts',(49.3598459063144,-43.1795073970375,
-229.995871622349));
#226236=CARTESIAN_POINT('Ctrl Pts',(49.8679794722695,-43.8525810620647,
-229.207175913618));
#226237=CARTESIAN_POINT('Ctrl Pts',(50.3756978342709,-44.5263335458687,
-228.418792446769));
#226238=CARTESIAN_POINT('Ctrl Pts',(51.3911345582736,-45.8738385134766,
-226.842025513071));
#226239=CARTESIAN_POINT('Ctrl Pts',(52.4049464549377,-47.224002264507,-225.266482347449));
#226240=CARTESIAN_POINT('Ctrl Pts',(53.4182055248116,-48.5750603074809,
-223.691342941789));
#226241=CARTESIAN_POINT('Ctrl Pts',(55.4447236645594,-51.2771763934287,
-220.541064130469));
#226242=CARTESIAN_POINT('Ctrl Pts',(57.4689725824102,-53.9829798427017,
-217.392457267063));
#226243=CARTESIAN_POINT('Ctrl Pts',(59.492784702789,-56.6895247738662,-214.244180243974));
#226244=CARTESIAN_POINT('Ctrl Pts',(47.3211789031199,-40.4350426000942,
-233.171747992562));
#226245=CARTESIAN_POINT('Ctrl Pts',(47.8337422070404,-41.0944281592508,
-232.381526838764));
#226246=CARTESIAN_POINT('Ctrl Pts',(48.3450895420457,-41.7559741023036,
-231.59233795934));
#226247=CARTESIAN_POINT('Ctrl Pts',(48.8559011403763,-42.4184505962563,
-230.803585490448));
#226248=CARTESIAN_POINT('Ctrl Pts',(49.3667127387069,-43.080927090209,-230.014833021558));
#226249=CARTESIAN_POINT('Ctrl Pts',(49.87695729968,-43.7443929697667,-229.226546244883));
#226250=CARTESIAN_POINT('Ctrl Pts',(50.3869032026916,-44.4083742082442,
-228.43849935464));
#226251=CARTESIAN_POINT('Ctrl Pts',(51.4067950087149,-45.7363366851993,
-226.862405574156));
#226252=CARTESIAN_POINT('Ctrl Pts',(52.4255193465988,-47.0663149534946,
-225.287250420734));
#226253=CARTESIAN_POINT('Ctrl Pts',(53.4438309990515,-48.3970017219875,
-223.712420269846));
#226254=CARTESIAN_POINT('Ctrl Pts',(55.4804543039569,-51.0583752589733,
-220.562759968072));
#226255=CARTESIAN_POINT('Ctrl Pts',(57.5153972302706,-53.7226435757235,
-217.414431597513));
#226256=CARTESIAN_POINT('Ctrl Pts',(59.5500043535892,-56.3875253353041,
-214.266381372884));
#226257=CARTESIAN_POINT('Ctrl Pts',(47.3174213500927,-40.3725566206431,
-233.190758458866));
#226258=CARTESIAN_POINT('Ctrl Pts',(47.8304331865629,-41.0247379875799,
-232.40178755381));
#226259=CARTESIAN_POINT('Ctrl Pts',(48.3427237376172,-41.6782347797706,
-231.613445913152));
#226260=CARTESIAN_POINT('Ctrl Pts',(48.8546863035239,-42.3323210585191,
-230.825382497106));
#226261=CARTESIAN_POINT('Ctrl Pts',(49.3666488694307,-42.9864073372676,
-230.037319081059));
#226262=CARTESIAN_POINT('Ctrl Pts',(49.8782662454544,-43.6411158354054,
-229.249550061497));
#226263=CARTESIAN_POINT('Ctrl Pts',(50.3896983451462,-44.2961564367811,
-228.461936921534));
#226264=CARTESIAN_POINT('Ctrl Pts',(51.4125625445298,-45.6062376395327,
-226.886710641608));
#226265=CARTESIAN_POINT('Ctrl Pts',(52.4347028263001,-46.9176171020422,
-225.312093851176));
#226266=CARTESIAN_POINT('Ctrl Pts',(53.4565811414505,-48.229468784563,-223.737696459652));
#226267=CARTESIAN_POINT('Ctrl Pts',(55.5003377717513,-50.8531721496045,
-220.588901676603));
#226268=CARTESIAN_POINT('Ctrl Pts',(57.5430330553295,-53.4787928890259,
-217.440999537853));
#226269=CARTESIAN_POINT('Ctrl Pts',(59.5855147104668,-56.1048379574655,
-214.293293254791));
#226270=CARTESIAN_POINT('Ctrl Pts',(47.3136637970655,-40.310070641192,-233.20976892517));
#226271=CARTESIAN_POINT('Ctrl Pts',(47.8271241660854,-40.955047815909,-232.422048268856));
#226272=CARTESIAN_POINT('Ctrl Pts',(48.3403579331886,-41.6004954572377,
-231.634553866964));
#226273=CARTESIAN_POINT('Ctrl Pts',(48.8534714666716,-42.246191520782,-230.847179503763));
#226274=CARTESIAN_POINT('Ctrl Pts',(49.3665850001545,-42.8918875843263,
-230.059805140562));
#226275=CARTESIAN_POINT('Ctrl Pts',(49.8795751912289,-43.537838701044,-229.272553878112));
#226276=CARTESIAN_POINT('Ctrl Pts',(50.3924934876008,-44.183938665318,-228.485374488428));
#226277=CARTESIAN_POINT('Ctrl Pts',(51.4183300803446,-45.476138593866,-226.911015709061));
#226278=CARTESIAN_POINT('Ctrl Pts',(52.4438863060015,-46.7689192505898,
-225.336937281619));
#226279=CARTESIAN_POINT('Ctrl Pts',(53.4693312838495,-48.0619358471384,
-223.762972649457));
#226280=CARTESIAN_POINT('Ctrl Pts',(55.5202212395457,-50.6479690402357,
-220.615043385133));
#226281=CARTESIAN_POINT('Ctrl Pts',(57.5706688803884,-53.2349422023283,
-217.467567478191));
#226282=CARTESIAN_POINT('Ctrl Pts',(59.6210250673444,-55.8221505796269,
-214.320205136697));
#226283=CARTESIAN_POINT('Ctrl Pts',(47.3091454883712,-40.242131557965,-233.229003132042));
#226284=CARTESIAN_POINT('Ctrl Pts',(47.8231540168911,-40.8795018283497,
-232.442071186825));
#226285=CARTESIAN_POINT('Ctrl Pts',(48.337145706421,-41.5169166318385,-231.655160989632));
#226286=CARTESIAN_POINT('Ctrl Pts',(48.8511232816408,-42.1543682290027,
-230.868268963674));
#226287=CARTESIAN_POINT('Ctrl Pts',(49.3651008568606,-42.7918198261669,
-230.081376937717));
#226288=CARTESIAN_POINT('Ctrl Pts',(49.8790645191143,-43.4293078274282,
-229.294502880311));
#226289=CARTESIAN_POINT('Ctrl Pts',(50.3930177372337,-44.066823718135,-228.507642672989));
#226290=CARTESIAN_POINT('Ctrl Pts',(51.4209241734724,-45.3418554995486,
-226.933922258343));
#226291=CARTESIAN_POINT('Ctrl Pts',(52.4487896446279,-46.616996929731,-225.36025631034));
#226292=CARTESIAN_POINT('Ctrl Pts',(53.4766337325378,-47.8922016232008,
-223.786622036391));
#226293=CARTESIAN_POINT('Ctrl Pts',(55.5323219083575,-50.4426110101405,
-220.639353488495));
#226294=CARTESIAN_POINT('Ctrl Pts',(57.5879280964248,-52.9932654200165,
-217.492207602051));
#226295=CARTESIAN_POINT('Ctrl Pts',(59.6435178458378,-55.5440119530488,
-214.345108432027));
#226296=CARTESIAN_POINT('Ctrl Pts',(47.3051413523369,-40.1629192793609,
-233.246904846954));
#226297=CARTESIAN_POINT('Ctrl Pts',(47.819327369804,-40.7940757964512,-232.460673323282));
#226298=CARTESIAN_POINT('Ctrl Pts',(48.3336083951406,-41.4250391409392,
-231.674348554294));
#226299=CARTESIAN_POINT('Ctrl Pts',(48.8479443642697,-42.0558912348621,
-230.88796994392));
#226300=CARTESIAN_POINT('Ctrl Pts',(49.3622803333988,-42.6867433287849,
-230.101591333545));
#226301=CARTESIAN_POINT('Ctrl Pts',(49.8766723259409,-43.3174819888763,
-229.315157839431));
#226302=CARTESIAN_POINT('Ctrl Pts',(50.3910998220442,-43.9481493585103,
-228.52868979147));
#226303=CARTESIAN_POINT('Ctrl Pts',(51.4199548142509,-45.2094840977783,
-226.955753695549));
#226304=CARTESIAN_POINT('Ctrl Pts',(52.4489487693187,-46.4705399682764,
-225.382682428314));
#226305=CARTESIAN_POINT('Ctrl Pts',(53.4780084556675,-47.7314680211233,
-223.809549063998));
#226306=CARTESIAN_POINT('Ctrl Pts',(55.536127828365,-50.253324126817,-220.663282335366));
#226307=CARTESIAN_POINT('Ctrl Pts',(57.5945065616385,-52.7746765489683,
-217.516770963173));
#226308=CARTESIAN_POINT('Ctrl Pts',(59.6529740461698,-55.2958790062696,
-214.370186647608));
#226309=CARTESIAN_POINT('Ctrl Pts',(47.3011370887008,-40.083704476459,-233.264807132349));
#226310=CARTESIAN_POINT('Ctrl Pts',(47.8155006007713,-40.7086470422379,
-232.479276052542));
#226311=CARTESIAN_POINT('Ctrl Pts',(48.330070971135,-41.3331587221332,-231.693536730416));
#226312=CARTESIAN_POINT('Ctrl Pts',(48.8447653455944,-41.957411102505,-230.907671551986));
#226313=CARTESIAN_POINT('Ctrl Pts',(49.3594597200539,-42.5816634828768,
-230.121806373556));
#226314=CARTESIAN_POINT('Ctrl Pts',(49.8742800565343,-43.2056525867135,
-229.335813456774));
#226315=CARTESIAN_POINT('Ctrl Pts',(50.3891818457356,-43.8294712170295,
-228.549737580672));
#226316=CARTESIAN_POINT('Ctrl Pts',(51.4189854241382,-45.0771084776612,
-226.977585828468));
#226317=CARTESIAN_POINT('Ctrl Pts',(52.4491078990803,-46.3240783396034,
-225.405109260954));
#226318=CARTESIAN_POINT('Ctrl Pts',(53.4793832226061,-47.5707292968664,
-223.832476822232));
#226319=CARTESIAN_POINT('Ctrl Pts',(55.5399338696578,-50.0640312113922,
-220.68721194479));
#226320=CARTESIAN_POINT('Ctrl Pts',(57.6010852364915,-52.5560807120374,
-217.541335107067));
#226321=CARTESIAN_POINT('Ctrl Pts',(59.6624305478473,-55.0477381521116,
-214.39526566237));
#226322=CARTESIAN_POINT('Ctrl Pts',(47.2844095710387,-40.0223529985484,
-233.29571384424));
#226323=CARTESIAN_POINT('Ctrl Pts',(47.799865767177,-40.6397128949599,-232.509454608122));
#226324=CARTESIAN_POINT('Ctrl Pts',(48.3153486991529,-41.2570069665437,
-231.72316146998));
#226325=CARTESIAN_POINT('Ctrl Pts',(48.8308531059458,-41.8742482184852,
-230.936841114977));
#226326=CARTESIAN_POINT('Ctrl Pts',(49.3463575127388,-42.4914894704268,
-230.150520759975));
#226327=CARTESIAN_POINT('Ctrl Pts',(49.8618834246415,-43.1086778283034,
-229.364173149988));
#226328=CARTESIAN_POINT('Ctrl Pts',(50.3774268752988,-43.7258231065776,
-228.577803332719));
#226329=CARTESIAN_POINT('Ctrl Pts',(51.4085137766134,-44.9601136631259,
-227.005063698182));
#226330=CARTESIAN_POINT('Ctrl Pts',(52.4396702308542,-46.1942333889078,
-225.432235999036));
#226331=CARTESIAN_POINT('Ctrl Pts',(53.4708746321289,-47.4282358136099,
-223.859347784982));
#226332=CARTESIAN_POINT('Ctrl Pts',(55.5332834346784,-49.8962406630142,
-220.713571356874));
#226333=CARTESIAN_POINT('Ctrl Pts',(57.5958804822797,-52.3637850919073,
-217.567557391373));
#226334=CARTESIAN_POINT('Ctrl Pts',(59.658577156368,-54.831089092749,-214.42141923076));
#226335=CARTESIAN_POINT('Ctrl Pts',(47.269359813636,-39.9199414144257,-233.323677937652));
#226336=CARTESIAN_POINT('Ctrl Pts',(47.7852688958474,-40.5328114906027,
-232.537018038148));
#226337=CARTESIAN_POINT('Ctrl Pts',(48.3011810934468,-41.1456737613432,
-231.750354102807));
#226338=CARTESIAN_POINT('Ctrl Pts',(48.8170958227919,-41.7585296857987,
-230.963686885275));
#226339=CARTESIAN_POINT('Ctrl Pts',(49.3330105521369,-42.3713856102541,
-230.177019667743));
#226340=CARTESIAN_POINT('Ctrl Pts',(49.8489278162636,-42.9842351808713,
-229.390349164127));
#226341=CARTESIAN_POINT('Ctrl Pts',(50.3648471682373,-43.5970795157942,
-228.603675952145));
#226342=CARTESIAN_POINT('Ctrl Pts',(51.3966858721847,-44.8227681856401,
-227.03032952818));
#226343=CARTESIAN_POINT('Ctrl Pts',(52.4285328613266,-46.0484360781329,
-225.456972356173));
#226344=CARTESIAN_POINT('Ctrl Pts',(53.4603856521184,-47.2740894119757,
-223.883607650579));
#226345=CARTESIAN_POINT('Ctrl Pts',(55.5240912337022,-49.7253960796616,
-220.736878239389));
#226346=CARTESIAN_POINT('Ctrl Pts',(57.5878196113417,-52.1766455410871,
-217.590119225487));
#226347=CARTESIAN_POINT('Ctrl Pts',(59.6515602724445,-54.6278641542596,
-214.443344242486));
#226348=CARTESIAN_POINT('',(47.5799752941295,-40.2889415902933,-232.85005));
#226349=CARTESIAN_POINT('',(47.0825542278859,-41.7715518798765,-232.850050000968));
#226350=CARTESIAN_POINT('Ctrl Pts',(47.5799752940314,-40.2889415926919,
-232.85005));
#226351=CARTESIAN_POINT('Ctrl Pts',(47.5775945735868,-40.3473480101173,
-232.85005));
#226352=CARTESIAN_POINT('Ctrl Pts',(47.5746791399166,-40.3934055204136,
-232.85005));
#226353=CARTESIAN_POINT('Ctrl Pts',(47.5660677926235,-40.4699741879599,
-232.85005));
#226354=CARTESIAN_POINT('Ctrl Pts',(47.5635310903242,-40.4915421250293,
-232.850049999998));
#226355=CARTESIAN_POINT('Ctrl Pts',(47.5531956971805,-40.5727355789934,
-232.850049999998));
#226356=CARTESIAN_POINT('Ctrl Pts',(47.5435314537204,-40.6342224874872,
-232.85005));
#226357=CARTESIAN_POINT('Ctrl Pts',(47.498863464585,-40.8512217208458,-232.85005));
#226358=CARTESIAN_POINT('Ctrl Pts',(47.4667238050309,-40.9561283613665,
-232.850050000008));
#226359=CARTESIAN_POINT('Ctrl Pts',(47.4103530292664,-41.1136517562587,
-232.850050000008));
#226360=CARTESIAN_POINT('Ctrl Pts',(47.3884688969554,-41.1712462220726,
-232.850050000436));
#226361=CARTESIAN_POINT('Ctrl Pts',(47.3415687154481,-41.2863061130767,
-232.850050000436));
#226362=CARTESIAN_POINT('Ctrl Pts',(47.3098061178227,-41.3563636655023,
-232.850049999917));
#226363=CARTESIAN_POINT('Ctrl Pts',(47.238535493308,-41.4987551852984,-232.850049999917));
#226364=CARTESIAN_POINT('Ctrl Pts',(47.2078203687848,-41.5594829940685,
-232.850050000009));
#226365=CARTESIAN_POINT('Ctrl Pts',(47.1722887237613,-41.6240970447738,
-232.850050000009));
#226366=CARTESIAN_POINT('Ctrl Pts',(47.1600291820282,-41.6454764695154,
-232.85005));
#226367=CARTESIAN_POINT('Ctrl Pts',(47.1263867106497,-41.7020987847656,
-232.85005));
#226368=CARTESIAN_POINT('Ctrl Pts',(47.1037445726029,-41.7383217640954,
-232.85005));
#226369=CARTESIAN_POINT('Ctrl Pts',(47.0825542565969,-41.7715518684049,
-232.85005));
#226370=CARTESIAN_POINT('',(57.733985310444,-60.0593815363208,-214.252907888001));
#226371=CARTESIAN_POINT('Ctrl Pts',(47.0825542096955,-41.7715519112001,
-232.850049982949));
#226372=CARTESIAN_POINT('Ctrl Pts',(47.9607606644449,-43.2885970115993,
-231.310756440341));
#226373=CARTESIAN_POINT('Ctrl Pts',(48.8396331722643,-44.8051274616754,
-229.771321514311));
#226374=CARTESIAN_POINT('Ctrl Pts',(49.7193526002943,-46.3210209808882,
-228.231740696015));
#226375=CARTESIAN_POINT('Ctrl Pts',(50.6068212501588,-47.8502676156323,
-226.67859810687));
#226376=CARTESIAN_POINT('Ctrl Pts',(51.4951510340416,-49.3788667920708,
-225.125307245091));
#226377=CARTESIAN_POINT('Ctrl Pts',(52.3845369850665,-50.9067042966212,
-223.571849770436));
#226378=CARTESIAN_POINT('Ctrl Pts',(52.3981868919341,-50.9301528788952,
-223.548007984058));
#226379=CARTESIAN_POINT('Ctrl Pts',(52.4118370435254,-50.9536012831489,
-223.524166157505));
#226380=CARTESIAN_POINT('Ctrl Pts',(52.4254874411528,-50.9770495086906,
-223.500324290775));
#226381=CARTESIAN_POINT('Ctrl Pts',(54.1899580063524,-54.008001785955,-220.418489371959));
#226382=CARTESIAN_POINT('Ctrl Pts',(55.9585237261342,-57.035959927734,-217.335999861453));
#226383=CARTESIAN_POINT('Ctrl Pts',(57.7339853077823,-60.0593815358969,
-214.252907939395));
#226384=CARTESIAN_POINT('',(59.5601545409129,-55.0066093843694,-214.536876504828));
#226385=CARTESIAN_POINT('Ctrl Pts',(59.5601545409136,-55.0066093843693,
-214.536876504827));
#226386=CARTESIAN_POINT('Ctrl Pts',(59.5534103769403,-55.183285281497,-214.523179687364));
#226387=CARTESIAN_POINT('Ctrl Pts',(59.5413857023832,-55.3595267001454,
-214.509940774492));
#226388=CARTESIAN_POINT('Ctrl Pts',(59.5048392787739,-55.7306111662553,
-214.483592249558));
#226389=CARTESIAN_POINT('Ctrl Pts',(59.4790426192872,-55.9255750687639,
-214.470456744663));
#226390=CARTESIAN_POINT('Ctrl Pts',(59.4374186268297,-56.1761840233205,
-214.453298735629));
#226391=CARTESIAN_POINT('Ctrl Pts',(59.4271923857434,-56.2341662641521,
-214.449364106042));
#226392=CARTESIAN_POINT('Ctrl Pts',(59.3290041047216,-56.7600810968204,
-214.414327664314));
#226393=CARTESIAN_POINT('Ctrl Pts',(59.2036000752591,-57.2212958998854,
-214.387817887177));
#226394=CARTESIAN_POINT('Ctrl Pts',(58.9920439420324,-57.8080590467771,
-214.35489987404));
#226395=CARTESIAN_POINT('Ctrl Pts',(58.9383051097013,-57.9461281140662,
-214.347431324614));
#226396=CARTESIAN_POINT('Ctrl Pts',(58.7834285639215,-58.3162123489988,
-214.328364513275));
#226397=CARTESIAN_POINT('Ctrl Pts',(58.6754718372346,-58.5458967426914,
-214.316667298022));
#226398=CARTESIAN_POINT('Ctrl Pts',(58.4793456692785,-58.920803329709,-214.298260215069));
#226399=CARTESIAN_POINT('Ctrl Pts',(58.3955443144802,-59.0701807393243,
-214.291807992095));
#226400=CARTESIAN_POINT('Ctrl Pts',(58.2554398199234,-59.3038767790683,
-214.282137443959));
#226401=CARTESIAN_POINT('Ctrl Pts',(58.2014468386641,-59.3905132232272,
-214.278624601648));
#226402=CARTESIAN_POINT('Ctrl Pts',(58.0758641218467,-59.5844450019102,
-214.270199768697));
#226403=CARTESIAN_POINT('Ctrl Pts',(58.0026577731459,-59.6923453371106,
-214.265296898901));
#226404=CARTESIAN_POINT('Ctrl Pts',(57.8636814802851,-59.8874642716893,
-214.258285826271));
#226405=CARTESIAN_POINT('Ctrl Pts',(57.799587863237,-59.9740538268332,-214.255565510063));
#226406=CARTESIAN_POINT('Ctrl Pts',(57.7339853360531,-60.0593815526408,
-214.252907779836));
#226407=CARTESIAN_POINT('',(59.5781472511572,-54.5406860123134,-214.555282751782));
#226408=CARTESIAN_POINT('Ctrl Pts',(59.5601545409116,-55.0066093843694,
-214.53687650483));
#226409=CARTESIAN_POINT('Ctrl Pts',(59.5631405773446,-54.9283846158517,
-214.542940888217));
#226410=CARTESIAN_POINT('Ctrl Pts',(59.5661299872555,-54.8504833727614,
-214.547589274133));
#226411=CARTESIAN_POINT('Ctrl Pts',(59.572151316647,-54.6945566512149,-214.553743244933));
#226412=CARTESIAN_POINT('Ctrl Pts',(59.5751126784951,-54.6183446757107,
-214.555228232806));
#226413=CARTESIAN_POINT('Ctrl Pts',(59.5781472511111,-54.540686012984,-214.55528275182));
#226414=CARTESIAN_POINT('Ctrl Pts',(47.5799752942349,-40.2889415880665,
-232.85005));
#226415=CARTESIAN_POINT('Ctrl Pts',(51.5792492625364,-45.0398156733569,
-226.7519456074));
#226416=CARTESIAN_POINT('Ctrl Pts',(55.5786810873963,-49.7902940354523,
-220.653636556059));
#226417=CARTESIAN_POINT('Ctrl Pts',(59.5781472511525,-54.540686011977,-214.555282751822));
#226418=CARTESIAN_POINT('Ctrl Pts',(24.9017054131522,-60.8052918727755,
-233.340945144186));
#226419=CARTESIAN_POINT('Ctrl Pts',(25.5906443745351,-61.3025059726095,
-232.554279700873));
#226420=CARTESIAN_POINT('Ctrl Pts',(26.2795988326832,-61.7997136258234,
-231.767623645885));
#226421=CARTESIAN_POINT('Ctrl Pts',(26.9685652314336,-62.2969163567666,
-230.980974825615));
#226422=CARTESIAN_POINT('Ctrl Pts',(27.6575316301841,-62.7941190877098,
-230.194326005343));
#226423=CARTESIAN_POINT('Ctrl Pts',(28.346509997394,-63.2913168845119,-229.407684436704));
#226424=CARTESIAN_POINT('Ctrl Pts',(29.0354977836505,-63.7885108411498,
-228.621048576497));
#226425=CARTESIAN_POINT('Ctrl Pts',(30.4134733561636,-64.7828987544258,
-227.047776856082));
#226426=CARTESIAN_POINT('Ctrl Pts',(31.7914861973683,-65.7772714817533,
-225.474527722644));
#226427=CARTESIAN_POINT('Ctrl Pts',(33.1695232342839,-66.7716346400439,
-223.90129326724));
#226428=CARTESIAN_POINT('Ctrl Pts',(35.925597308115,-68.7603609566252,-220.754824356431));
#226429=CARTESIAN_POINT('Ctrl Pts',(38.6817661332381,-70.749049871159,-217.608412929565));
#226430=CARTESIAN_POINT('Ctrl Pts',(41.437980641355,-72.7377225056729,-214.462029323759));
#226431=CARTESIAN_POINT('Ctrl Pts',(24.9106027465158,-60.8049715273879,
-233.340948124015));
#226432=CARTESIAN_POINT('Ctrl Pts',(25.5998098315156,-61.3021744082037,
-232.554282687331));
#226433=CARTESIAN_POINT('Ctrl Pts',(26.2890324103538,-61.7993707608737,
-231.767626642701));
#226434=CARTESIAN_POINT('Ctrl Pts',(26.9782669268481,-62.2965621103122,
-230.980977835653));
#226435=CARTESIAN_POINT('Ctrl Pts',(27.6675014433422,-62.7937534597507,
-230.194329028605));
#226436=CARTESIAN_POINT('Ctrl Pts',(28.3567479253494,-63.2909397940828,
-229.407687476061));
#226437=CARTESIAN_POINT('Ctrl Pts',(29.0460038234333,-63.7881222076912,
-228.621051634203));
#226438=CARTESIAN_POINT('Ctrl Pts',(30.424515619601,-64.7824870349079,-227.047779950486));
#226439=CARTESIAN_POINT('Ctrl Pts',(31.8030646725822,-65.776836354002,-225.474530862664));
#226440=CARTESIAN_POINT('Ctrl Pts',(33.1816379091815,-66.771175783969,-223.901296458627));
#226441=CARTESIAN_POINT('Ctrl Pts',(35.9387843823801,-68.759854643903,-220.754827650554));
#226442=CARTESIAN_POINT('Ctrl Pts',(38.6960255585086,-70.7484948217514,
-217.608416348934));
#226443=CARTESIAN_POINT('Ctrl Pts',(41.4533123673286,-72.737117447414,-214.462032879015));
#226444=CARTESIAN_POINT('Ctrl Pts',(24.9204263182847,-60.8042678820624,
-233.341483208271));
#226445=CARTESIAN_POINT('Ctrl Pts',(25.6098926659838,-61.3014622348707,
-232.554814099759));
#226446=CARTESIAN_POINT('Ctrl Pts',(26.2993748034754,-61.7986498568027,
-231.768154572902));
#226447=CARTESIAN_POINT('Ctrl Pts',(26.9888691299455,-62.2958322905427,
-230.981502444082));
#226448=CARTESIAN_POINT('Ctrl Pts',(27.6783634564157,-62.7930147242826,
-230.194850315263));
#226449=CARTESIAN_POINT('Ctrl Pts',(28.3678699996353,-63.2901919580089,
-229.408205601368));
#226450=CARTESIAN_POINT('Ctrl Pts',(29.0573861713395,-63.7873651018695,
-228.621566733601));
#226451=CARTESIAN_POINT('Ctrl Pts',(30.4364185147476,-64.7817113895908,
-227.048288998068));
#226452=CARTESIAN_POINT('Ctrl Pts',(31.8154889591027,-65.776041494825,-225.475034396628));
#226453=CARTESIAN_POINT('Ctrl Pts',(33.1945841923364,-66.7703611350645,
-223.901794865388));
#226454=CARTESIAN_POINT('Ctrl Pts',(35.9527746588037,-68.7590004155436,
-220.755315802909));
#226455=CARTESIAN_POINT('Ctrl Pts',(38.7110622045295,-70.7475987291489,
-217.608895764391));
#226456=CARTESIAN_POINT('Ctrl Pts',(41.4693966584753,-72.7361776662597,
-214.462504384327));
#226457=CARTESIAN_POINT('Ctrl Pts',(24.9262307371789,-60.8052629613404,
-233.339663481057));
#226458=CARTESIAN_POINT('Ctrl Pts',(25.6159901042832,-61.3024373924278,
-232.553007006783));
#226459=CARTESIAN_POINT('Ctrl Pts',(26.3057643351287,-61.7996053791141,
-231.766359540212));
#226460=CARTESIAN_POINT('Ctrl Pts',(26.9955499476215,-62.2967684208872,
-230.979718973407));
#226461=CARTESIAN_POINT('Ctrl Pts',(27.6853355601145,-62.7939314626603,
-230.193078406603));
#226462=CARTESIAN_POINT('Ctrl Pts',(28.3751325826488,-63.2910895473583,
-229.406444756795));
#226463=CARTESIAN_POINT('Ctrl Pts',(29.0649385371855,-63.7882437431482,
-228.619816524538));
#226464=CARTESIAN_POINT('Ctrl Pts',(30.4445504462589,-64.7825521347279,
-227.046560060024));
#226465=CARTESIAN_POINT('Ctrl Pts',(31.8241976850135,-65.7768451422546,
-225.473325024605));
#226466=CARTESIAN_POINT('Ctrl Pts',(33.2038676569546,-66.7711282018108,
-223.90010380027));
#226467=CARTESIAN_POINT('Ctrl Pts',(35.9632076008367,-68.7596943209232,
-220.753661351601));
#226468=CARTESIAN_POINT('Ctrl Pts',(38.7226365397166,-70.7482214856064,
-217.607272976111));
#226469=CARTESIAN_POINT('Ctrl Pts',(41.4821077889028,-72.7367298763208,
-214.460910461991));
#226470=CARTESIAN_POINT('Ctrl Pts',(24.9320351560731,-60.8062580406183,
-233.337843753845));
#226471=CARTESIAN_POINT('Ctrl Pts',(25.6220875425827,-61.3034125499849,
-232.551199913808));
#226472=CARTESIAN_POINT('Ctrl Pts',(26.312153866782,-61.8005609014255,-231.764564507522));
#226473=CARTESIAN_POINT('Ctrl Pts',(27.0022307652976,-62.2977045512317,
-230.977935502733));
#226474=CARTESIAN_POINT('Ctrl Pts',(27.6923076638132,-62.794848201038,-230.191306497943));
#226475=CARTESIAN_POINT('Ctrl Pts',(28.3823951656622,-63.2919871367077,
-229.404683912223));
#226476=CARTESIAN_POINT('Ctrl Pts',(29.0724909030316,-63.7891223844269,
-228.618066315475));
#226477=CARTESIAN_POINT('Ctrl Pts',(30.4526823777702,-64.7833928798651,
-227.044831121978));
#226478=CARTESIAN_POINT('Ctrl Pts',(31.8329064109243,-65.7776487896842,
-225.471615652582));
#226479=CARTESIAN_POINT('Ctrl Pts',(33.2131511215727,-66.7718952685571,
-223.898412735151));
#226480=CARTESIAN_POINT('Ctrl Pts',(35.9736405428697,-68.7603882263028,
-220.752006900292));
#226481=CARTESIAN_POINT('Ctrl Pts',(38.7342108749039,-70.7488442420639,
-217.605650187832));
#226482=CARTESIAN_POINT('Ctrl Pts',(41.4948189193303,-72.737282086382,-214.459316539654));
#226483=CARTESIAN_POINT('Ctrl Pts',(24.9376768366503,-60.8072592698702,
-233.336009748324));
#226484=CARTESIAN_POINT('Ctrl Pts',(25.6280319185531,-61.3043928842789,
-232.549378593582));
#226485=CARTESIAN_POINT('Ctrl Pts',(26.318399828189,-61.8015207131228,-231.762755190619));
#226486=CARTESIAN_POINT('Ctrl Pts',(27.0087773823957,-62.2986441421295,
-230.976137619604));
#226487=CARTESIAN_POINT('Ctrl Pts',(27.6991549366024,-62.7957675711362,
-230.189520048589));
#226488=CARTESIAN_POINT('Ctrl Pts',(28.3895421644288,-63.2928865877122,
-229.402908327074));
#226489=CARTESIAN_POINT('Ctrl Pts',(29.0799368492491,-63.7900021575995,
-228.616301118674));
#226490=CARTESIAN_POINT('Ctrl Pts',(30.4607262188897,-64.7842332973742,
-227.043086701871));
#226491=CARTESIAN_POINT('Ctrl Pts',(31.8415450550293,-65.778450807822,-225.469890119541));
#226492=CARTESIAN_POINT('Ctrl Pts',(33.2223823764397,-66.772659477679,-223.89670475417));
#226493=CARTESIAN_POINT('Ctrl Pts',(35.9840570192604,-68.7610768173931,
-220.750334023428));
#226494=CARTESIAN_POINT('Ctrl Pts',(38.7458039689211,-70.7494595084382,
-217.604007176241));
#226495=CARTESIAN_POINT('Ctrl Pts',(41.5075840172059,-72.7378246702262,
-214.457700600944));
#226496=CARTESIAN_POINT('Ctrl Pts',(24.9431675857188,-60.8082654676189,
-233.334164524199));
#226497=CARTESIAN_POINT('Ctrl Pts',(25.6338346604351,-61.3053771897629,
-232.547545996672));
#226498=CARTESIAN_POINT('Ctrl Pts',(26.3245132764945,-61.8024835845448,
-231.760934436748));
#226499=CARTESIAN_POINT('Ctrl Pts',(27.0152005013104,-62.2995859346266,
-230.97432807854));
#226500=CARTESIAN_POINT('Ctrl Pts',(27.7058877261263,-62.7966882847084,
-230.187721720333));
#226501=CARTESIAN_POINT('Ctrl Pts',(28.3965835877948,-63.2937865778419,
-229.401120580787));
#226502=CARTESIAN_POINT('Ctrl Pts',(29.0872860637793,-63.7908816992324,
-228.614523442413));
#226503=CARTESIAN_POINT('Ctrl Pts',(30.4686910157482,-64.7850719420134,
-227.041329165664));
#226504=CARTESIAN_POINT('Ctrl Pts',(31.8501220936262,-65.7792496428099,
-225.468150694098));
#226505=CARTESIAN_POINT('Ctrl Pts',(33.231569388313,-66.7734191417836,-223.894982065188));
#226506=CARTESIAN_POINT('Ctrl Pts',(35.9944639776866,-68.7617581397308,
-220.748644807367));
#226507=CARTESIAN_POINT('Ctrl Pts',(38.7574219835962,-70.7500649666192,
-217.602346047653));
#226508=CARTESIAN_POINT('Ctrl Pts',(41.5204085705364,-72.7383548951067,
-214.45606483788));
#226509=CARTESIAN_POINT('Ctrl Pts',(24.9541490838557,-60.8102778631162,
-233.330474075949));
#226510=CARTESIAN_POINT('Ctrl Pts',(25.6454401441992,-61.307345800731,-232.543880802852));
#226511=CARTESIAN_POINT('Ctrl Pts',(26.3367401731056,-61.8044093273887,
-231.757292929005));
#226512=CARTESIAN_POINT('Ctrl Pts',(27.0280467391398,-62.3014695196208,
-230.970708996412));
#226513=CARTESIAN_POINT('Ctrl Pts',(27.719353305174,-62.7985297118529,-230.18412506382));
#226514=CARTESIAN_POINT('Ctrl Pts',(28.4106664345268,-63.2955865581015,
-229.397545088212));
#226515=CARTESIAN_POINT('Ctrl Pts',(29.1019844928396,-63.7926407824983,
-228.610968089891));
#226516=CARTESIAN_POINT('Ctrl Pts',(30.4846206094652,-64.7867492312918,
-227.037814093248));
#226517=CARTESIAN_POINT('Ctrl Pts',(31.8672761708201,-65.7808473127859,
-225.464671843211));
#226518=CARTESIAN_POINT('Ctrl Pts',(33.2499434120597,-66.7749384699927,
-223.891536687223));
#226519=CARTESIAN_POINT('Ctrl Pts',(36.0152778945389,-68.7631207844063,
-220.745266375246));
#226520=CARTESIAN_POINT('Ctrl Pts',(38.7806580129467,-70.7512758829813,
-217.599023790475));
#226521=CARTESIAN_POINT('Ctrl Pts',(41.5460576771974,-72.7394153448676,
-214.45279331175));
#226522=CARTESIAN_POINT('Ctrl Pts',(24.96452603429,-60.8123106330865,-233.326738316813));
#226523=CARTESIAN_POINT('Ctrl Pts',(25.6564783942742,-61.3093307323952,
-232.540170136386));
#226524=CARTESIAN_POINT('Ctrl Pts',(26.3484364151579,-61.8063476946002,
-231.753605361133));
#226525=CARTESIAN_POINT('Ctrl Pts',(27.0403984599708,-62.3033622546844,
-230.967043014045));
#226526=CARTESIAN_POINT('Ctrl Pts',(27.7323605047837,-62.8003768147686,
-230.180480666957));
#226527=CARTESIAN_POINT('Ctrl Pts',(28.4243265937515,-63.2973889636564,
-229.393920760111));
#226528=CARTESIAN_POINT('Ctrl Pts',(29.1162956595838,-63.794399180595,-228.607362656609));
#226529=CARTESIAN_POINT('Ctrl Pts',(30.5002337912484,-64.7884196144722,
-227.034246449605));
#226530=CARTESIAN_POINT('Ctrl Pts',(31.8841836526759,-65.7824324003622,
-225.461137349913));
#226531=CARTESIAN_POINT('Ctrl Pts',(33.2681403403832,-66.7764397401221,
-223.888032432174));
#226532=CARTESIAN_POINT('Ctrl Pts',(36.0360537157978,-68.7644544196418,
-220.741822596696));
#226533=CARTESIAN_POINT('Ctrl Pts',(38.8039937558954,-70.7524476024647,
-217.595629106873));
#226534=CARTESIAN_POINT('Ctrl Pts',(41.5719446953938,-72.740426365189,-214.449442564061));
#226535=CARTESIAN_POINT('Ctrl Pts',(24.9744025307133,-60.8143487212353,
-233.322986925177));
#226536=CARTESIAN_POINT('Ctrl Pts',(25.6670491804662,-61.3113173869818,
-232.536442059561));
#226537=CARTESIAN_POINT('Ctrl Pts',(26.3596977749792,-61.8082844221729,
-231.749898382092));
#226538=CARTESIAN_POINT('Ctrl Pts',(27.0523477402915,-62.3052500852752,
-230.96335555072));
#226539=CARTESIAN_POINT('Ctrl Pts',(27.7449977056038,-62.8022157483775,
-230.176812719347));
#226540=CARTESIAN_POINT('Ctrl Pts',(28.4376490490292,-63.2991800360968,
-229.390270738434));
#226541=CARTESIAN_POINT('Ctrl Pts',(29.1303013990492,-63.7961431156999,
-228.603729386647));
#226542=CARTESIAN_POINT('Ctrl Pts',(30.5156060990893,-64.7900692749063,
-227.030646683075));
#226543=CARTESIAN_POINT('Ctrl Pts',(31.9009147636639,-65.7839906295158,
-225.45756645914));
#226544=CARTESIAN_POINT('Ctrl Pts',(33.2862256991509,-66.777907941617,-223.884487706564));
#226545=CARTESIAN_POINT('Ctrl Pts',(36.0568475701252,-68.7657425658195,
-220.738330201412));
#226546=CARTESIAN_POINT('Ctrl Pts',(38.827478307619,-70.7535611178629,-217.592178452254));
#226547=CARTESIAN_POINT('Ctrl Pts',(41.5981125175426,-72.7413660196969,
-214.446029255158));
#226548=CARTESIAN_POINT('Ctrl Pts',(24.9941555235601,-60.8184248975328,
-233.315484141906));
#226549=CARTESIAN_POINT('Ctrl Pts',(25.6881907528502,-61.3152906961552,
-232.528985905911));
#226550=CARTESIAN_POINT('Ctrl Pts',(26.3822204946216,-61.8121578773183,
-231.74248442401));
#226551=CARTESIAN_POINT('Ctrl Pts',(27.0762463009327,-62.3090257464567,
-230.955980624069));
#226552=CARTESIAN_POINT('Ctrl Pts',(27.7702721072438,-62.8058936155951,
-230.169476824128));
#226553=CARTESIAN_POINT('Ctrl Pts',(28.4642939595846,-63.3027621809775,
-229.382970695078));
#226554=CARTESIAN_POINT('Ctrl Pts',(29.1583128779801,-63.7996309859099,
-228.596462846723));
#226555=CARTESIAN_POINT('Ctrl Pts',(30.5463507147712,-64.7933685957745,
-227.023447150014));
#226556=CARTESIAN_POINT('Ctrl Pts',(31.9343769856396,-65.7871070878229,
-225.450424677593));
#226557=CARTESIAN_POINT('Ctrl Pts',(33.3223964166864,-66.7808443446069,
-223.877398255344));
#226558=CARTESIAN_POINT('Ctrl Pts',(36.0984352787801,-68.768318858175,-220.731345410844));
#226559=CARTESIAN_POINT('Ctrl Pts',(38.8744474110663,-70.7557881486592,
-217.585277143015));
#226560=CARTESIAN_POINT('Ctrl Pts',(41.6504481618404,-72.7432453287128,
-214.439202637353));
#226561=CARTESIAN_POINT('Ctrl Pts',(25.0118948272389,-60.8225311816015,
-233.307912950748));
#226562=CARTESIAN_POINT('Ctrl Pts',(25.7074533125622,-61.319278145358,-232.521455721897));
#226563=CARTESIAN_POINT('Ctrl Pts',(26.4029963020791,-61.8160309424671,
-231.734989391403));
#226564=CARTESIAN_POINT('Ctrl Pts',(27.0985290755007,-62.3127871125508,
-230.948517073201));
#226565=CARTESIAN_POINT('Ctrl Pts',(27.7940618489222,-62.8095432826346,
-230.162044755));
#226566=CARTESIAN_POINT('Ctrl Pts',(28.489584316755,-63.3063028673177,-229.375566396309));
#226567=CARTESIAN_POINT('Ctrl Pts',(29.1850996372909,-63.8030643940992,
-228.589083860001));
#226568=CARTESIAN_POINT('Ctrl Pts',(30.5761302783625,-64.7965874476622,
-227.016118787385));
#226569=CARTESIAN_POINT('Ctrl Pts',(31.9671328527444,-65.7901180259831,
-225.443137312419));
#226570=CARTESIAN_POINT('Ctrl Pts',(33.3581205213136,-66.7836499900577,
-223.870147199431));
#226571=CARTESIAN_POINT('Ctrl Pts',(36.140095858452,-68.7707139182068,-220.724166973453));
#226572=CARTESIAN_POINT('Ctrl Pts',(38.9220129137361,-70.7577827632511,
-217.578152986549));
#226573=CARTESIAN_POINT('Ctrl Pts',(41.7039086779697,-72.7448392550568,
-214.432127077688));
#226574=CARTESIAN_POINT('Ctrl Pts',(25.028605078732,-60.8264461849104,-233.300589177504));
#226575=CARTESIAN_POINT('Ctrl Pts',(25.7257590504183,-61.3230773961178,
-232.514138876127));
#226576=CARTESIAN_POINT('Ctrl Pts',(26.4228956738429,-61.8197151427821,
-231.727678440368));
#226577=CARTESIAN_POINT('Ctrl Pts',(27.1200213189657,-62.3163563966737,
-230.941211605428));
#226578=CARTESIAN_POINT('Ctrl Pts',(27.8171469640885,-62.8129976505652,
-230.154744770487));
#226579=CARTESIAN_POINT('Ctrl Pts',(28.514261502952,-63.3096424726104,-229.368271461406));
#226580=CARTESIAN_POINT('Ctrl Pts',(29.2113685617452,-63.8062891397564,
-228.581793805278));
#226581=CARTESIAN_POINT('Ctrl Pts',(30.6055826793317,-64.7995824740485,
-227.008838493021));
#226582=CARTESIAN_POINT('Ctrl Pts',(31.9997674609787,-65.7928829112188,
-225.435866135329));
#226583=CARTESIAN_POINT('Ctrl Pts',(33.393937296167,-66.786183616434,-223.862885177104));
#226584=CARTESIAN_POINT('Ctrl Pts',(36.1822769665438,-68.7727850268643,
-220.716923260653));
#226585=CARTESIAN_POINT('Ctrl Pts',(38.9705580867346,-70.7593869240872,
-217.570927667784));
#226586=CARTESIAN_POINT('Ctrl Pts',(41.7588188049893,-72.745971187409,-214.424920813073));
#226587=CARTESIAN_POINT('Ctrl Pts',(25.0620255817184,-60.8342761915281,
-233.285941631018));
#226588=CARTESIAN_POINT('Ctrl Pts',(25.7623705261304,-61.3306758976375,
-232.499505184585));
#226589=CARTESIAN_POINT('Ctrl Pts',(26.4626944173704,-61.8270835434123,
-231.713056538299));
#226590=CARTESIAN_POINT('Ctrl Pts',(27.1630058058958,-62.3234949649194,
-230.926600669881));
#226591=CARTESIAN_POINT('Ctrl Pts',(27.8633171944211,-62.8199063864266,
-230.140144801462));
#226592=CARTESIAN_POINT('Ctrl Pts',(28.5636158753459,-63.3163216831959,
-229.353681591601));
#226593=CARTESIAN_POINT('Ctrl Pts',(29.2639064106539,-63.8127386310709,
-228.567213695831));
#226594=CARTESIAN_POINT('Ctrl Pts',(30.6644874812699,-64.8055725268209,
-226.994277904292));
#226595=CARTESIAN_POINT('Ctrl Pts',(32.0650366774472,-65.7984126816902,
-225.421323781149));
#226596=CARTESIAN_POINT('Ctrl Pts',(33.4655708458739,-66.7912508691866,
-223.848361132451));
#226597=CARTESIAN_POINT('Ctrl Pts',(36.2666391827274,-68.7769272441794,
-220.702435835054));
#226598=CARTESIAN_POINT('Ctrl Pts',(39.0676484327315,-70.7625952457594,
-217.556477030254));
#226599=CARTESIAN_POINT('Ctrl Pts',(41.8686390590285,-72.7482350521135,
-214.410508283843));
#226600=CARTESIAN_POINT('Ctrl Pts',(25.0913820158672,-60.8413726539041,
-233.272320165694));
#226601=CARTESIAN_POINT('Ctrl Pts',(25.7952223871138,-61.337539263733,-232.485770621816));
#226602=CARTESIAN_POINT('Ctrl Pts',(26.4990562522867,-61.8337088794851,
-231.699217348229));
#226603=CARTESIAN_POINT('Ctrl Pts',(27.2028964362607,-62.3298740344814,
-230.912668010765));
#226604=CARTESIAN_POINT('Ctrl Pts',(27.9067366202345,-62.8260391894777,
-230.126118673301));
#226605=CARTESIAN_POINT('Ctrl Pts',(28.6105819801057,-63.3222004675808,
-229.339572581631));
#226606=CARTESIAN_POINT('Ctrl Pts',(29.314434077262,-63.8183564731875,-228.553030636562));
#226607=CARTESIAN_POINT('Ctrl Pts',(30.7221382715748,-64.8106684844009,
-226.97994674642));
#226608=CARTESIAN_POINT('Ctrl Pts',(32.1298688397377,-65.8029595883788,
-225.406879087961));
#226609=CARTESIAN_POINT('Ctrl Pts',(33.5376184032793,-66.7952312053955,
-223.833823110276));
#226610=CARTESIAN_POINT('Ctrl Pts',(36.3531175303626,-68.7797744394288,
-220.687711154908));
#226611=CARTESIAN_POINT('Ctrl Pts',(39.1686880217984,-70.7642419152226,
-217.541643153526));
#226612=CARTESIAN_POINT('Ctrl Pts',(41.9842864659859,-72.7486501639975,
-214.39559293419));
#226613=CARTESIAN_POINT('Ctrl Pts',(25.1256029177818,-60.8447964462213,
-233.262708527412));
#226614=CARTESIAN_POINT('Ctrl Pts',(25.8323432559684,-61.3411439778804,
-232.475469715128));
#226615=CARTESIAN_POINT('Ctrl Pts',(26.5393879179131,-61.8373317659467,
-231.688406549544));
#226616=CARTESIAN_POINT('Ctrl Pts',(27.2465878469089,-62.3334358738351,
-230.90143275512));
#226617=CARTESIAN_POINT('Ctrl Pts',(27.9537877759048,-62.8295399817235,
-230.114458960696));
#226618=CARTESIAN_POINT('Ctrl Pts',(28.6611482655484,-63.3255577393973,
-229.327577621181));
#226619=CARTESIAN_POINT('Ctrl Pts',(29.3686016850915,-63.8215238522036,
-228.540749713863));
#226620=CARTESIAN_POINT('Ctrl Pts',(30.7835085241778,-64.8134560778162,
-226.967093899227));
#226621=CARTESIAN_POINT('Ctrl Pts',(32.198778370749,-65.8051862301184,-225.3936468087));
#226622=CARTESIAN_POINT('Ctrl Pts',(33.6141958867398,-66.7968253706499,
-223.820284551445));
#226623=CARTESIAN_POINT('Ctrl Pts',(36.4450309187215,-68.7801036517128,
-220.673560036935));
#226624=CARTESIAN_POINT('Ctrl Pts',(39.2764551401188,-70.7630188613062,
-217.527174130311));
#226625=CARTESIAN_POINT('Ctrl Pts',(42.1080287367154,-72.7457990899024,
-214.3808746454));
#226626=CARTESIAN_POINT('Ctrl Pts',(25.1598238196964,-60.8482202385386,
-233.25309688913));
#226627=CARTESIAN_POINT('Ctrl Pts',(25.8694641248229,-61.3447486920278,
-232.465168808441));
#226628=CARTESIAN_POINT('Ctrl Pts',(26.5797195835393,-61.8409546524082,
-231.677595750858));
#226629=CARTESIAN_POINT('Ctrl Pts',(27.2902792575572,-62.3369977131888,
-230.890197499475));
#226630=CARTESIAN_POINT('Ctrl Pts',(28.000838931575,-62.8330407739693,-230.102799248092));
#226631=CARTESIAN_POINT('Ctrl Pts',(28.711714550991,-63.3289150112138,-229.315582660731));
#226632=CARTESIAN_POINT('Ctrl Pts',(29.4227692929209,-63.8246912312197,
-228.528468791165));
#226633=CARTESIAN_POINT('Ctrl Pts',(30.8448787767808,-64.8162436712314,
-226.954241052034));
#226634=CARTESIAN_POINT('Ctrl Pts',(32.2676879017602,-65.8074128718581,
-225.380414529439));
#226635=CARTESIAN_POINT('Ctrl Pts',(33.6907733702002,-66.7984195359043,
-223.806745992614));
#226636=CARTESIAN_POINT('Ctrl Pts',(36.5369443070804,-68.7804328639968,
-220.659408918962));
#226637=CARTESIAN_POINT('Ctrl Pts',(39.3842222584393,-70.7617958073898,
-217.512705107097));
#226638=CARTESIAN_POINT('Ctrl Pts',(42.2317710074449,-72.7429480158072,
-214.366156356611));
#226639=CARTESIAN_POINT('Ctrl Pts',(25.1936739556362,-60.8507158919519,
-233.244352036751));
#226640=CARTESIAN_POINT('Ctrl Pts',(25.9062554175954,-61.3475191565963,
-232.455522106742));
#226641=CARTESIAN_POINT('Ctrl Pts',(26.6199310089813,-61.8437435167674,
-231.667324698448));
#226642=CARTESIAN_POINT('Ctrl Pts',(27.3341145564557,-62.3396921598031,
-230.879418569252));
#226643=CARTESIAN_POINT('Ctrl Pts',(28.0482981039303,-62.8356408028389,
-230.091512440055));
#226644=CARTESIAN_POINT('Ctrl Pts',(28.7630142200764,-63.3313013469077,
-229.303912100956));
#226645=CARTESIAN_POINT('Ctrl Pts',(29.4780199079502,-63.8268014559396,
-228.516477155575));
#226646=CARTESIAN_POINT('Ctrl Pts',(30.9080312836978,-64.8178016740036,
-226.941607264814));
#226647=CARTESIAN_POINT('Ctrl Pts',(32.3391739164292,-65.8081747617964,
-225.367383553375));
#226648=CARTESIAN_POINT('Ctrl Pts',(33.7707373952718,-66.7982992813128,
-223.793398542109));
#226649=CARTESIAN_POINT('Ctrl Pts',(36.6338643529568,-68.7785483203456,
-220.645428519576));
#226650=CARTESIAN_POINT('Ctrl Pts',(39.498692720429,-70.7577954999793,-217.498424772054));
#226651=CARTESIAN_POINT('Ctrl Pts',(42.363907023339,-72.7367527914189,-214.351639090142));
#226652=CARTESIAN_POINT('Ctrl Pts',(25.2239774050683,-60.8541676049626,
-233.234470884236));
#226653=CARTESIAN_POINT('Ctrl Pts',(25.9398083842247,-61.3511430455559,
-232.444758300872));
#226654=CARTESIAN_POINT('Ctrl Pts',(26.6572825734193,-61.8472255929447,
-231.655996189968));
#226655=CARTESIAN_POINT('Ctrl Pts',(27.3754647705453,-62.3429113806012,
-230.867638000096));
#226656=CARTESIAN_POINT('Ctrl Pts',(28.0936469676712,-62.8385971682577,
-230.079279810225));
#226657=CARTESIAN_POINT('Ctrl Pts',(28.8125820204444,-63.3338632665416,
-229.291352292986));
#226658=CARTESIAN_POINT('Ctrl Pts',(29.5319096752348,-63.8289050323554,
-228.503647571677));
#226659=CARTESIAN_POINT('Ctrl Pts',(30.9705649848157,-64.8189885639829,
-226.928238129057));
#226660=CARTESIAN_POINT('Ctrl Pts',(32.4107560406701,-65.8081944618785,
-225.353700434162));
#226661=CARTESIAN_POINT('Ctrl Pts',(33.8514884032197,-66.7970717553631,
-223.779466811102));
#226662=CARTESIAN_POINT('Ctrl Pts',(36.732953128319,-68.7748263423323,-220.630999564983));
#226663=CARTESIAN_POINT('Ctrl Pts',(39.6166287632978,-70.7512448922044,
-217.483776946995));
#226664=CARTESIAN_POINT('Ctrl Pts',(42.5007756355285,-72.7273057434785,
-214.336817183699));
#226665=CARTESIAN_POINT('Ctrl Pts',(25.2542808545004,-60.8576193179734,
-233.224589731722));
#226666=CARTESIAN_POINT('Ctrl Pts',(25.9733613508541,-61.3547669345154,
-232.433994495002));
#226667=CARTESIAN_POINT('Ctrl Pts',(26.6946341378572,-61.850707669122,-231.644667681488));
#226668=CARTESIAN_POINT('Ctrl Pts',(27.4168149846347,-62.3461306013993,
-230.855857430941));
#226669=CARTESIAN_POINT('Ctrl Pts',(28.1389958314122,-62.8415535336766,
-230.067047180394));
#226670=CARTESIAN_POINT('Ctrl Pts',(28.8621498208122,-63.3364251861756,
-229.278792485017));
#226671=CARTESIAN_POINT('Ctrl Pts',(29.5857994425194,-63.8310086087711,
-228.490817987778));
#226672=CARTESIAN_POINT('Ctrl Pts',(31.0330986859336,-64.8201754539622,
-226.914868993301));
#226673=CARTESIAN_POINT('Ctrl Pts',(32.482338164911,-65.8082141619607,-225.340017314949));
#226674=CARTESIAN_POINT('Ctrl Pts',(33.9322394111677,-66.7958442294134,
-223.765535080096));
#226675=CARTESIAN_POINT('Ctrl Pts',(36.8320419036812,-68.771104364319,-220.61657061039));
#226676=CARTESIAN_POINT('Ctrl Pts',(39.7345648061665,-70.7446942844296,
-217.469129121935));
#226677=CARTESIAN_POINT('Ctrl Pts',(42.637644247718,-72.7178586955381,-214.321995277256));
#226678=CARTESIAN_POINT('Ctrl Pts',(25.2821906319223,-60.8614218083708,
-233.214245961014));
#226679=CARTESIAN_POINT('Ctrl Pts',(26.0046873376329,-61.35871072973,-232.422705498826));
#226680=CARTESIAN_POINT('Ctrl Pts',(26.7300272921764,-61.854405153137,-231.632810266957));
#226681=CARTESIAN_POINT('Ctrl Pts',(27.4564885610292,-62.3494441225829,
-230.843550233226));
#226682=CARTESIAN_POINT('Ctrl Pts',(28.182949829882,-62.8444830920289,-230.054290199494));
#226683=CARTESIAN_POINT('Ctrl Pts',(28.9106256129361,-63.3388181928255,
-229.265721482054));
#226684=CARTESIAN_POINT('Ctrl Pts',(29.6389030120051,-63.8327945119493,
-228.477491114052));
#226685=CARTESIAN_POINT('Ctrl Pts',(31.0954578101431,-64.8207471501967,
-226.901030378049));
#226686=CARTESIAN_POINT('Ctrl Pts',(32.5543706785782,-65.8072943179338,
-225.32589662341));
#226687=CARTESIAN_POINT('Ctrl Pts',(34.0140584320924,-66.7933503332008,
-223.751191978427));
#226688=CARTESIAN_POINT('Ctrl Pts',(36.933433939121,-68.7654623637348,-220.60178268846));
#226689=CARTESIAN_POINT('Ctrl Pts',(39.8560206222034,-70.7355537328838,
-217.454158252827));
#226690=CARTESIAN_POINT('Ctrl Pts',(42.7792356116896,-72.705154549818,-214.306877306875));
#226691=CARTESIAN_POINT('Ctrl Pts',(25.3082796911041,-60.8654535469475,
-233.203637421846));
#226692=CARTESIAN_POINT('Ctrl Pts',(26.0341343285133,-61.3629238744168,
-232.411039848471));
#226693=CARTESIAN_POINT('Ctrl Pts',(26.7636013838676,-61.8583152760603,
-231.620533187723));
#226694=CARTESIAN_POINT('Ctrl Pts',(27.4944243031966,-62.3528874641244,
-230.830789824077));
#226695=CARTESIAN_POINT('Ctrl Pts',(28.2252472225255,-62.8474596521885,
-230.041046460431));
#226696=CARTESIAN_POINT('Ctrl Pts',(28.9575562895767,-63.3411438699236,
-229.252145525666));
#226697=CARTESIAN_POINT('Ctrl Pts',(29.6905827327532,-63.8343860369735,
-228.463645185323));
#226698=CARTESIAN_POINT('Ctrl Pts',(31.1566356191065,-64.8208703710732,
-226.886644504638));
#226699=CARTESIAN_POINT('Ctrl Pts',(32.6255046561051,-65.8056211821729,
-225.311217867621));
#226700=CARTESIAN_POINT('Ctrl Pts',(34.0952688014063,-66.7897856212239,
-223.736281731367));
#226701=CARTESIAN_POINT('Ctrl Pts',(37.034797092009,-68.7581144993257,-220.58640945886));
#226702=CARTESIAN_POINT('Ctrl Pts',(39.9780639773415,-70.7240153450236,
-217.438595831035));
#226703=CARTESIAN_POINT('Ctrl Pts',(42.922034708619,-72.6893523415957,-214.291161723059));
#226704=CARTESIAN_POINT('Ctrl Pts',(25.3604578094675,-60.8735170241007,
-233.18242034351));
#226705=CARTESIAN_POINT('Ctrl Pts',(26.0930283102741,-61.3713501637903,
-232.387708547763));
#226706=CARTESIAN_POINT('Ctrl Pts',(26.8307495672501,-61.866135521907,-231.595979029253));
#226707=CARTESIAN_POINT('Ctrl Pts',(27.5702957875313,-62.3597741472074,
-230.805269005779));
#226708=CARTESIAN_POINT('Ctrl Pts',(28.3098420078126,-62.8534127725078,
-230.014558982304));
#226709=CARTESIAN_POINT('Ctrl Pts',(29.0514176428578,-63.3457952241198,
-229.224993612889));
#226710=CARTESIAN_POINT('Ctrl Pts',(29.7939421742496,-63.8375690870219,
-228.435953327864));
#226711=CARTESIAN_POINT('Ctrl Pts',(31.2789912370331,-64.8211168128261,
-226.857872757815));
#226712=CARTESIAN_POINT('Ctrl Pts',(32.767772611159,-65.8022749106513,-225.281860356042));
#226713=CARTESIAN_POINT('Ctrl Pts',(34.2576895400343,-66.7826561972701,
-223.706461237247));
#226714=CARTESIAN_POINT('Ctrl Pts',(37.237523397785,-68.7434187705077,-220.555662999657));
#226715=CARTESIAN_POINT('Ctrl Pts',(40.2221506876178,-70.7009385693032,
-217.407470987453));
#226716=CARTESIAN_POINT('Ctrl Pts',(43.2076329024777,-72.657747925151,-214.259730555427));
#226717=CARTESIAN_POINT('Ctrl Pts',(25.4136698948603,-60.8775733111457,
-233.1647909109));
#226718=CARTESIAN_POINT('Ctrl Pts',(26.1536009721352,-61.3753309304317,
-232.367988911507));
#226719=CARTESIAN_POINT('Ctrl Pts',(26.9003944903513,-61.8688530492783,
-231.575160164634));
#226720=CARTESIAN_POINT('Ctrl Pts',(27.6494543016586,-62.3608735835334,
-230.783584826932));
#226721=CARTESIAN_POINT('Ctrl Pts',(28.3985141129659,-62.8528941177885,
-229.992009489228));
#226722=CARTESIAN_POINT('Ctrl Pts',(29.1501449587015,-63.3432443646947,
-229.201875553329));
#226723=CARTESIAN_POINT('Ctrl Pts',(29.902937659956,-63.8328099372364,-228.412377972218));
#226724=CARTESIAN_POINT('Ctrl Pts',(31.4085230624649,-64.8119410823196,
-226.833382809995));
#226725=CARTESIAN_POINT('Ctrl Pts',(32.9186915675153,-65.7879847694566,
-225.256902902535));
#226726=CARTESIAN_POINT('Ctrl Pts',(34.4301958247084,-66.7630648301267,
-223.681133553689));
#226727=CARTESIAN_POINT('Ctrl Pts',(37.4532043390948,-68.7132249514667,
-220.529594855996));
#226728=CARTESIAN_POINT('Ctrl Pts',(40.4819176467888,-70.6593236327973,
-217.381117488375));
#226729=CARTESIAN_POINT('Ctrl Pts',(43.5116000921785,-72.6045769412523,
-214.233142011455));
#226730=CARTESIAN_POINT('Ctrl Pts',(25.4734681104549,-60.8745649395491,
-233.152705479171));
#226731=CARTESIAN_POINT('Ctrl Pts',(26.2191301593905,-61.3728030581697,
-232.352982827705));
#226732=CARTESIAN_POINT('Ctrl Pts',(26.9737314089713,-61.8653651155087,
-231.558531400184));
#226733=CARTESIAN_POINT('Ctrl Pts',(27.7312103498245,-62.3559170177131,
-230.765669056017));
#226734=CARTESIAN_POINT('Ctrl Pts',(28.4886892906776,-62.8464689199175,
-229.972806711851));
#226735=CARTESIAN_POINT('Ctrl Pts',(29.2494572009032,-63.3347856810085,
-229.181797847991));
#226736=CARTESIAN_POINT('Ctrl Pts',(30.0116917876015,-63.8220563583486,
-228.391588810695));
#226737=CARTESIAN_POINT('Ctrl Pts',(31.5361609609982,-64.7965977130286,
-226.811170736103));
#226738=CARTESIAN_POINT('Ctrl Pts',(33.0664220838837,-65.7670232712464,
-225.233920858118));
#226739=CARTESIAN_POINT('Ctrl Pts',(34.5983413220466,-66.7361768147042,
-223.657538786233));
#226740=CARTESIAN_POINT('Ctrl Pts',(37.6621797983723,-68.6744839016197,
-220.504774642461));
#226741=CARTESIAN_POINT('Ctrl Pts',(40.7331349268486,-70.6074216926982,
-217.355782960055));
#226742=CARTESIAN_POINT('Ctrl Pts',(43.8052734509942,-72.5392749729601,
-214.207386766717));
#226743=CARTESIAN_POINT('Ctrl Pts',(25.5332663260497,-60.8715565679525,
-233.140620047442));
#226744=CARTESIAN_POINT('Ctrl Pts',(26.2846593466459,-61.3702751859077,
-232.337976743902));
#226745=CARTESIAN_POINT('Ctrl Pts',(27.0470683275914,-61.861877181739,-231.541902635733));
#226746=CARTESIAN_POINT('Ctrl Pts',(27.8129663979903,-62.3509604518928,
-230.747753285103));
#226747=CARTESIAN_POINT('Ctrl Pts',(28.5788644683892,-62.8400437220466,
-229.953603934473));
#226748=CARTESIAN_POINT('Ctrl Pts',(29.3487694431048,-63.3263269973223,
-229.161720142653));
#226749=CARTESIAN_POINT('Ctrl Pts',(30.120445915247,-63.8113027794608,-228.370799649172));
#226750=CARTESIAN_POINT('Ctrl Pts',(31.6637988595316,-64.7812543437376,
-226.788958662211));
#226751=CARTESIAN_POINT('Ctrl Pts',(33.2141526002521,-65.7460617730361,
-225.210938813702));
#226752=CARTESIAN_POINT('Ctrl Pts',(34.7664868193848,-66.7092887992816,
-223.633944018777));
#226753=CARTESIAN_POINT('Ctrl Pts',(37.8711552576499,-68.6357428517727,
-220.479954428925));
#226754=CARTESIAN_POINT('Ctrl Pts',(40.9843522069086,-70.555519752599,-217.330448431736));
#226755=CARTESIAN_POINT('Ctrl Pts',(44.0989468098099,-72.4739730046678,
-214.18163152198));
#226756=CARTESIAN_POINT('Ctrl Pts',(25.5832151954094,-60.8726283032168,
-233.124939038994));
#226757=CARTESIAN_POINT('Ctrl Pts',(26.3412812962705,-61.3709102534954,
-232.320159632019));
#226758=CARTESIAN_POINT('Ctrl Pts',(27.1119488435164,-61.8607811001136,
-231.522967655684));
#226759=CARTESIAN_POINT('Ctrl Pts',(27.8865579092606,-62.347663656611,-230.727938128436));
#226760=CARTESIAN_POINT('Ctrl Pts',(28.6611669750047,-62.8345462131084,
-229.932908601188));
#226761=CARTESIAN_POINT('Ctrl Pts',(29.4403191496334,-63.3181119795184,
-229.140447526113));
#226762=CARTESIAN_POINT('Ctrl Pts',(30.2214658612003,-63.8001296619401,
-228.349062770292));
#226763=CARTESIAN_POINT('Ctrl Pts',(31.783759284334,-64.7641650267834,-226.766293258651));
#226764=CARTESIAN_POINT('Ctrl Pts',(33.353939516948,-65.7221108760403,-225.187799366854));
#226765=CARTESIAN_POINT('Ctrl Pts',(34.9263287803327,-66.6781922113775,
-223.610428795026));
#226766=CARTESIAN_POINT('Ctrl Pts',(38.071107307102,-68.590354882052,-220.455687651369));
#226767=CARTESIAN_POINT('Ctrl Pts',(41.2254251684497,-70.494636879644,-217.305890990877));
#226768=CARTESIAN_POINT('Ctrl Pts',(44.381286951629,-72.3973753477236,-214.156833956015));
#226769=CARTESIAN_POINT('Ctrl Pts',(25.6298304748707,-60.8753734341798,
-233.107177069033));
#226770=CARTESIAN_POINT('Ctrl Pts',(26.3965314717851,-61.3714239166506,
-232.301492490062));
#226771=CARTESIAN_POINT('Ctrl Pts',(27.1765365083298,-61.8582017525339,
-231.503828898795));
#226772=CARTESIAN_POINT('Ctrl Pts',(27.960699151696,-62.3416685933693,-230.708430592375));
#226773=CARTESIAN_POINT('Ctrl Pts',(28.7448617950622,-62.8251354342047,
-229.913032285956));
#226774=CARTESIAN_POINT('Ctrl Pts',(29.5338172036037,-63.3049330183218,
-229.120332249855));
#226775=CARTESIAN_POINT('Ctrl Pts',(30.3248744392529,-63.7830152939694,
-228.328756578445));
#226776=CARTESIAN_POINT('Ctrl Pts',(31.9069889105511,-64.7391798452646,
-226.745605235623));
#226777=CARTESIAN_POINT('Ctrl Pts',(33.4974147722857,-65.6885985452027,
-225.166922566632));
#226778=CARTESIAN_POINT('Ctrl Pts',(35.0901638016772,-66.6359498673557,
-223.589403428947));
#226779=CARTESIAN_POINT('Ctrl Pts',(38.2756618604604,-68.5306525116616,
-220.434365153576));
#226780=CARTESIAN_POINT('Ctrl Pts',(41.4711974327502,-70.4166207416591,
-217.284462017333));
#226781=CARTESIAN_POINT('Ctrl Pts',(44.6683526580257,-72.3008817462311,
-214.135317230106));
#226782=CARTESIAN_POINT('Ctrl Pts',(25.6764457543321,-60.8781185651427,
-233.089415099072));
#226783=CARTESIAN_POINT('Ctrl Pts',(26.4517816472997,-61.3719375798059,
-232.282825348105));
#226784=CARTESIAN_POINT('Ctrl Pts',(27.2411241731431,-61.8556224049542,
-231.484690141905));
#226785=CARTESIAN_POINT('Ctrl Pts',(28.0348403941315,-62.3356735301276,
-230.688923056315));
#226786=CARTESIAN_POINT('Ctrl Pts',(28.8285566151198,-62.8157246553009,
-229.893155970723));
#226787=CARTESIAN_POINT('Ctrl Pts',(29.6273152575741,-63.2917540571251,
-229.100216973599));
#226788=CARTESIAN_POINT('Ctrl Pts',(30.4282830173054,-63.7659009259987,
-228.308450386598));
#226789=CARTESIAN_POINT('Ctrl Pts',(32.0302185367682,-64.7141946637459,
-226.724917212596));
#226790=CARTESIAN_POINT('Ctrl Pts',(33.6408900276233,-65.6550862143651,
-225.14604576641));
#226791=CARTESIAN_POINT('Ctrl Pts',(35.2539988230218,-66.5937075233338,
-223.568378062868));
#226792=CARTESIAN_POINT('Ctrl Pts',(38.4802164138187,-68.4709501412712,
-220.413042655783));
#226793=CARTESIAN_POINT('Ctrl Pts',(41.7169696970508,-70.3386046036742,
-217.263033043788));
#226794=CARTESIAN_POINT('Ctrl Pts',(44.9554183644225,-72.2043881447385,
-214.113800504198));
#226795=CARTESIAN_POINT('Ctrl Pts',(25.7357162038904,-60.870117557065,-233.078364689706));
#226796=CARTESIAN_POINT('Ctrl Pts',(26.5183910989635,-61.3620069392732,
-232.270042402379));
#226797=CARTESIAN_POINT('Ctrl Pts',(27.3162411879881,-61.842621457398,-231.470961385261));
#226798=CARTESIAN_POINT('Ctrl Pts',(28.1188352251337,-62.3191557444292,
-230.674449007438));
#226799=CARTESIAN_POINT('Ctrl Pts',(28.9214292622792,-62.7956900314603,
-229.877936629616));
#226800=CARTESIAN_POINT('Ctrl Pts',(29.7294897040872,-63.2677206749556,
-229.084499084141));
#226801=CARTESIAN_POINT('Ctrl Pts',(30.5399444913362,-63.7376360518426,
-228.292329686201));
#226802=CARTESIAN_POINT('Ctrl Pts',(32.1608540658341,-64.6774668056166,
-226.707990890321));
#226803=CARTESIAN_POINT('Ctrl Pts',(33.7912315861003,-65.6089833988707,
-225.128696643096));
#226804=CARTESIAN_POINT('Ctrl Pts',(35.4242480247001,-66.5379429467924,
-223.550693656299));
#226805=CARTESIAN_POINT('Ctrl Pts',(38.6902809018998,-68.3958620426357,
-220.394687682705));
#226806=CARTESIAN_POINT('Ctrl Pts',(41.9677233302676,-70.2429924486788,
-217.244409494466));
#226807=CARTESIAN_POINT('Ctrl Pts',(45.2469984405841,-72.088022285615,-214.09495601129));
#226808=CARTESIAN_POINT('Ctrl Pts',(25.8011224073928,-60.8541224995348,
-233.072388186401));
#226809=CARTESIAN_POINT('Ctrl Pts',(26.5882772139689,-61.345584476566,-232.260902563554));
#226810=CARTESIAN_POINT('Ctrl Pts',(27.3926111430279,-61.824140301072,-231.460141397784));
#226811=CARTESIAN_POINT('Ctrl Pts',(28.2023317845711,-62.2979002023416,
-230.662317129508));
#226812=CARTESIAN_POINT('Ctrl Pts',(29.0120524261143,-62.7716601036112,
-229.864492861231));
#226813=CARTESIAN_POINT('Ctrl Pts',(29.8279705672755,-63.2401673093096,
-229.070199114559));
#226814=CARTESIAN_POINT('Ctrl Pts',(30.6466000725898,-63.7061844369386,
-228.277344321055));
#226815=CARTESIAN_POINT('Ctrl Pts',(32.2838590832184,-64.6382186921966,
-226.691634734048));
#226816=CARTESIAN_POINT('Ctrl Pts',(33.9318380253269,-65.5604762032412,
-225.111654172302));
#226817=CARTESIAN_POINT('Ctrl Pts',(35.582792800409,-66.4797047104531,-223.533108945327));
#226818=CARTESIAN_POINT('Ctrl Pts',(38.884702350573,-68.3181617248767,-220.376018491376));
#226819=CARTESIAN_POINT('Ctrl Pts',(42.1994895547755,-70.143871943617,-217.225335489343));
#226820=CARTESIAN_POINT('Ctrl Pts',(45.5163300351324,-71.9671084389128,
-214.075544244624));
#226821=CARTESIAN_POINT('Ctrl Pts',(25.8665286108953,-60.8381274420046,
-233.066411683095));
#226822=CARTESIAN_POINT('Ctrl Pts',(26.6581633289744,-61.3291620138588,
-232.251762724729));
#226823=CARTESIAN_POINT('Ctrl Pts',(27.4689810980677,-61.805659144746,-231.449321410308));
#226824=CARTESIAN_POINT('Ctrl Pts',(28.2858283440085,-62.276644660254,-230.650185251577));
#226825=CARTESIAN_POINT('Ctrl Pts',(29.1026755899493,-62.747630175762,-229.851049092846));
#226826=CARTESIAN_POINT('Ctrl Pts',(29.9264514304638,-63.2126139436637,
-229.055899144978));
#226827=CARTESIAN_POINT('Ctrl Pts',(30.7532556538434,-63.6747328220346,
-228.26235895591));
#226828=CARTESIAN_POINT('Ctrl Pts',(32.4068641006027,-64.5989705787766,
-226.675278577774));
#226829=CARTESIAN_POINT('Ctrl Pts',(34.0724444645535,-65.5119690076117,
-225.094611701508));
#226830=CARTESIAN_POINT('Ctrl Pts',(35.7413375761177,-66.4214664741137,
-223.515524234354));
#226831=CARTESIAN_POINT('Ctrl Pts',(39.0791237992462,-68.2404614071178,
-220.357349300048));
#226832=CARTESIAN_POINT('Ctrl Pts',(42.4312557792835,-70.0447514385552,
-217.206261484219));
#226833=CARTESIAN_POINT('Ctrl Pts',(45.7856616296808,-71.8461945922107,
-214.056132477959));
#226834=CARTESIAN_POINT('Ctrl Pts',(25.9160424850282,-60.8332597800929,
-233.053095414693));
#226835=CARTESIAN_POINT('Ctrl Pts',(26.7216988487821,-61.3154617178527,
-232.241381282086));
#226836=CARTESIAN_POINT('Ctrl Pts',(27.5420567082342,-61.7860906307777,
-231.439128672818));
#226837=CARTESIAN_POINT('Ctrl Pts',(28.3681860245984,-62.2513966239306,
-230.64015111493));
#226838=CARTESIAN_POINT('Ctrl Pts',(29.1943153409628,-62.7167026170834,
-229.841173557043));
#226839=CARTESIAN_POINT('Ctrl Pts',(30.0266724628494,-63.1764484440297,
-229.045833737559));
#226840=CARTESIAN_POINT('Ctrl Pts',(30.8620259206422,-63.633275037949,-228.252108649693));
#226841=CARTESIAN_POINT('Ctrl Pts',(32.5327328362278,-64.5469282257876,
-226.664658473961));
#226842=CARTESIAN_POINT('Ctrl Pts',(34.215164199298,-65.4492058327905,-225.083554042117));
#226843=CARTESIAN_POINT('Ctrl Pts',(35.9011649485234,-66.3475812818863,
-223.504153956677));
#226844=CARTESIAN_POINT('Ctrl Pts',(39.273166446974,-68.1443321800779,-220.345353785796));
#226845=CARTESIAN_POINT('Ctrl Pts',(42.6601436512792,-69.9251393601785,
-217.193943963384));
#226846=CARTESIAN_POINT('Ctrl Pts',(46.0496409219808,-71.7026940143502,
-214.043578157589));
#226847=CARTESIAN_POINT('Ctrl Pts',(25.9715990783732,-60.8263824397187,
-233.038076562284));
#226848=CARTESIAN_POINT('Ctrl Pts',(26.7915895883623,-61.2972176688764,
-232.2311442104));
#226849=CARTESIAN_POINT('Ctrl Pts',(27.6213469993979,-61.7602848222496,
-231.430540367037));
#226850=CARTESIAN_POINT('Ctrl Pts',(28.4556335624375,-62.2192160084591,
-230.63258019833));
#226851=CARTESIAN_POINT('Ctrl Pts',(29.289920125477,-62.6781471946685,-229.834620029623));
#226852=CARTESIAN_POINT('Ctrl Pts',(30.1289511322075,-63.1328363273331,
-229.039478997096));
#226853=CARTESIAN_POINT('Ctrl Pts',(30.9705439434446,-63.5850360083551,
-228.245754373682));
#226854=CARTESIAN_POINT('Ctrl Pts',(32.6537295659188,-64.4894353703992,
-226.658305126855));
#226855=CARTESIAN_POINT('Ctrl Pts',(34.3469173915073,-65.3841225672083,
-225.076391213479));
#226856=CARTESIAN_POINT('Ctrl Pts',(36.0437616605612,-66.2748188763012,
-223.496282027351));
#226857=CARTESIAN_POINT('Ctrl Pts',(39.4374501986691,-68.0562114944868,
-220.336063655097));
#226858=CARTESIAN_POINT('Ctrl Pts',(42.8459482063409,-69.8217123813687,
-217.183304075329));
#226859=CARTESIAN_POINT('Ctrl Pts',(46.2577049582974,-71.5830236206181,
-214.031928620936));
#226860=CARTESIAN_POINT('Ctrl Pts',(26.0271556717183,-60.8195050993445,
-233.023057709875));
#226861=CARTESIAN_POINT('Ctrl Pts',(26.8614803279425,-61.2789736199002,
-232.220907138713));
#226862=CARTESIAN_POINT('Ctrl Pts',(27.7006372905616,-61.7344790137215,
-231.421952061255));
#226863=CARTESIAN_POINT('Ctrl Pts',(28.5430811002764,-62.1870353929875,
-230.62500928173));
#226864=CARTESIAN_POINT('Ctrl Pts',(29.3855249099912,-62.6395917722535,
-229.828066502204));
#226865=CARTESIAN_POINT('Ctrl Pts',(30.2312298015655,-63.0892242106365,
-229.033124256632));
#226866=CARTESIAN_POINT('Ctrl Pts',(31.0790619662469,-63.5367969787612,
-228.239400097671));
#226867=CARTESIAN_POINT('Ctrl Pts',(32.7747262956096,-64.4319425150107,
-226.651951779748));
#226868=CARTESIAN_POINT('Ctrl Pts',(34.4786705837165,-65.3190393016261,
-225.069228384841));
#226869=CARTESIAN_POINT('Ctrl Pts',(36.1863583725991,-66.202056470716,-223.488410098027));
#226870=CARTESIAN_POINT('Ctrl Pts',(39.6017339503642,-67.9680908088958,
-220.326773524398));
#226871=CARTESIAN_POINT('Ctrl Pts',(43.0317527614028,-69.7182854025588,
-217.172664187274));
#226872=CARTESIAN_POINT('Ctrl Pts',(46.4657689946141,-71.4633532268859,
-214.020279084284));
#226873=CARTESIAN_POINT('Ctrl Pts',(26.1079086334631,-60.7917651170397,
-233.017180488577));
#226874=CARTESIAN_POINT('Ctrl Pts',(26.9477933569846,-61.2457491809832,
-232.216198008803));
#226875=CARTESIAN_POINT('Ctrl Pts',(27.791602857653,-61.6966607926582,-231.417878001952));
#226876=CARTESIAN_POINT('Ctrl Pts',(28.6380092466183,-62.1453058875298,
-230.62119554679));
#226877=CARTESIAN_POINT('Ctrl Pts',(29.4844156355837,-62.5939509824013,
-229.824513091628));
#226878=CARTESIAN_POINT('Ctrl Pts',(30.3334386001484,-63.0403250798734,
-229.029487457053));
#226879=CARTESIAN_POINT('Ctrl Pts',(31.1842647171309,-63.485002448237,-228.23553480923));
#226880=CARTESIAN_POINT('Ctrl Pts',(32.8859169510958,-64.3743571849642,
-226.647629513582));
#226881=CARTESIAN_POINT('Ctrl Pts',(34.5946426558381,-65.2570271773188,
-225.063918430622));
#226882=CARTESIAN_POINT('Ctrl Pts',(36.3070242103916,-66.1357954693092,
-223.482151043919));
#226883=CARTESIAN_POINT('Ctrl Pts',(39.7317873194987,-67.8933320532899,
-220.318616270514));
#226884=CARTESIAN_POINT('Ctrl Pts',(43.1708142706306,-69.6356764040323,
-217.162686067389));
#226885=CARTESIAN_POINT('Ctrl Pts',(46.6146568592818,-71.3718952390485,
-214.008891200286));
#226886=CARTESIAN_POINT('Ctrl Pts',(26.1949495995768,-60.7559954632254,
-233.015310708939));
#226887=CARTESIAN_POINT('Ctrl Pts',(27.0387644538443,-61.2057327308231,
-232.215070168042));
#226888=CARTESIAN_POINT('Ctrl Pts',(27.8858336675415,-61.6529664487026,
-231.417079914153));
#226889=CARTESIAN_POINT('Ctrl Pts',(28.7351647823697,-62.0982646553384,
-230.620551354198));
#226890=CARTESIAN_POINT('Ctrl Pts',(29.5844958971979,-62.5435628619743,
-229.824022794242));
#226891=CARTESIAN_POINT('Ctrl Pts',(30.4361008904608,-62.9869237960558,
-229.028968199982));
#226892=CARTESIAN_POINT('Ctrl Pts',(31.2893382107612,-63.4287766497893,
-228.234911333144));
#226893=CARTESIAN_POINT('Ctrl Pts',(32.9958128513619,-64.3124823572563,
-226.646797599469));
#226894=CARTESIAN_POINT('Ctrl Pts',(34.7087066827471,-65.190229522585,-225.062593091688));
#226895=CARTESIAN_POINT('Ctrl Pts',(36.425148099657,-66.0642498543572,-223.480334162157));
#226896=CARTESIAN_POINT('Ctrl Pts',(39.8580309334768,-67.8122905179015,
-220.315816303095));
#226897=CARTESIAN_POINT('Ctrl Pts',(43.304744476869,-69.545794357118,-217.158884043615));
#226898=CARTESIAN_POINT('Ctrl Pts',(46.7566079538913,-71.2728084364657,
-214.004305067604));
#226899=CARTESIAN_POINT('Ctrl Pts',(26.2384700826335,-60.7381106363183,
-233.014375819121));
#226900=CARTESIAN_POINT('Ctrl Pts',(27.0842500022742,-61.1857245057431,
-232.21450624766));
#226901=CARTESIAN_POINT('Ctrl Pts',(27.9329490724857,-61.6311192767247,
-231.416680870253));
#226902=CARTESIAN_POINT('Ctrl Pts',(28.7837425502454,-62.0747440392428,
-230.620229257902));
#226903=CARTESIAN_POINT('Ctrl Pts',(29.634536028005,-62.5183688017608,-229.82377764555));
#226904=CARTESIAN_POINT('Ctrl Pts',(30.487432035617,-62.960223154147,-229.028708571446));
#226905=CARTESIAN_POINT('Ctrl Pts',(31.3418749575762,-63.4006637505655,
-228.234599595102));
#226906=CARTESIAN_POINT('Ctrl Pts',(33.0507608014949,-64.2815449434024,
-226.646381642412));
#226907=CARTESIAN_POINT('Ctrl Pts',(34.7657386962016,-65.1568306952181,
-225.061930422221));
#226908=CARTESIAN_POINT('Ctrl Pts',(36.4842100442897,-66.0284770468812,
-223.479425721276));
#226909=CARTESIAN_POINT('Ctrl Pts',(39.9211527404658,-67.7717697502073,
-220.314416319386));
#226910=CARTESIAN_POINT('Ctrl Pts',(43.3717095799881,-69.5008533336608,
-217.156983031728));
#226911=CARTESIAN_POINT('Ctrl Pts',(46.827583501196,-71.2232650351743,-214.002012001263));
#226912=CARTESIAN_POINT('Ctrl Pts',(26.2629114467516,-60.7391039700744,
-233.002893197821));
#226913=CARTESIAN_POINT('Ctrl Pts',(27.114397963117,-61.1810939660079,-232.20584360482));
#226914=CARTESIAN_POINT('Ctrl Pts',(27.9674707129322,-61.6219011639104,
-231.409926775993));
#226915=CARTESIAN_POINT('Ctrl Pts',(28.8218440521233,-62.0616481295084,
-230.614892210633));
#226916=CARTESIAN_POINT('Ctrl Pts',(29.6762173913143,-62.5013950951064,
-229.819857645272));
#226917=CARTESIAN_POINT('Ctrl Pts',(30.5318920874236,-62.9400822869671,
-229.025706439153));
#226918=CARTESIAN_POINT('Ctrl Pts',(31.3886377598337,-63.3778284552318,
-228.232247232636));
#226919=CARTESIAN_POINT('Ctrl Pts',(33.102129104654,-64.2533207917612,-226.645328819602));
#226920=CARTESIAN_POINT('Ctrl Pts',(34.8198706879942,-65.1250606034272,
-225.061147334889));
#226921=CARTESIAN_POINT('Ctrl Pts',(36.5405225399701,-65.9938853198046,
-223.478668525429));
#226922=CARTESIAN_POINT('Ctrl Pts',(39.981826243922,-67.7315347525594,-220.313710906511));
#226923=CARTESIAN_POINT('Ctrl Pts',(43.4345244003096,-69.457683375828,-217.155376526334));
#226924=CARTESIAN_POINT('Ctrl Pts',(46.8928095579913,-71.1769737453648,
-213.999726959588));
#226925=CARTESIAN_POINT('Ctrl Pts',(26.2982843226441,-60.7344827742712,
-232.991392546795));
#226926=CARTESIAN_POINT('Ctrl Pts',(27.1539710903761,-61.1717772412952,
-232.196575481186));
#226927=CARTESIAN_POINT('Ctrl Pts',(28.0105205110111,-61.6084763232924,
-231.402405653547));
#226928=CARTESIAN_POINT('Ctrl Pts',(28.8678178196021,-62.0446142255719,
-230.608774353877));
#226929=CARTESIAN_POINT('Ctrl Pts',(29.725115128193,-62.4807521278514,-229.815143054206));
#226930=CARTESIAN_POINT('Ctrl Pts',(30.5831604852668,-62.9163290490967,
-229.022050566726));
#226931=CARTESIAN_POINT('Ctrl Pts',(31.441855894783,-63.3513820288522,-228.22940826535));
#226932=CARTESIAN_POINT('Ctrl Pts',(33.1592467138153,-64.2214879883631,
-226.644123662598));
#226933=CARTESIAN_POINT('Ctrl Pts',(34.879225924468,-65.0894996057218,-225.060627483752));
#226934=CARTESIAN_POINT('Ctrl Pts',(36.6011749254936,-65.955713208232,-223.478393801851));
#226935=CARTESIAN_POINT('Ctrl Pts',(40.045072927545,-67.6881404132524,-220.313926438049));
#226936=CARTESIAN_POINT('Ctrl Pts',(43.4967433028155,-69.4134193510673,
-217.154414312055));
#226937=CARTESIAN_POINT('Ctrl Pts',(46.9530675926807,-71.1335421841428,
-213.997473502442));
#226938=CARTESIAN_POINT('Ctrl Pts',(26.3336571985367,-60.7298615784681,
-232.97989189577));
#226939=CARTESIAN_POINT('Ctrl Pts',(27.1935442176352,-61.1624605165825,
-232.187307357553));
#226940=CARTESIAN_POINT('Ctrl Pts',(28.0535703090899,-61.5950514826745,
-231.3948845311));
#226941=CARTESIAN_POINT('Ctrl Pts',(28.9137915870808,-62.0275803216354,
-230.60265649712));
#226942=CARTESIAN_POINT('Ctrl Pts',(29.7740128650717,-62.4601091605963,
-229.810428463141));
#226943=CARTESIAN_POINT('Ctrl Pts',(30.6344288831099,-62.8925758112263,
-229.018394694299));
#226944=CARTESIAN_POINT('Ctrl Pts',(31.4950740297321,-63.3249356024725,
-228.226569298064));
#226945=CARTESIAN_POINT('Ctrl Pts',(33.2163643229766,-64.189655184965,-226.642918505594));
#226946=CARTESIAN_POINT('Ctrl Pts',(34.9385811609418,-65.0539386080163,
-225.060107632614));
#226947=CARTESIAN_POINT('Ctrl Pts',(36.6618273110172,-65.9175410966594,
-223.478119078272));
#226948=CARTESIAN_POINT('Ctrl Pts',(40.108319611168,-67.6447460739454,-220.314141969587));
#226949=CARTESIAN_POINT('Ctrl Pts',(43.5589622053215,-69.3691553263065,
-217.153452097777));
#226950=CARTESIAN_POINT('Ctrl Pts',(47.01332562737,-71.0901106229208,-213.995220045295));
#226951=CARTESIAN_POINT('Ctrl Pts',(26.3821787340349,-60.7171127522114,
-232.969564324364));
#226952=CARTESIAN_POINT('Ctrl Pts',(27.2445605117317,-61.1462290233331,
-232.178536730278));
#226953=CARTESIAN_POINT('Ctrl Pts',(28.1068458309989,-61.5755390840377,
-231.387516472179));
#226954=CARTESIAN_POINT('Ctrl Pts',(28.9690444318655,-62.0050437616364,
-230.596514709636));
#226955=CARTESIAN_POINT('Ctrl Pts',(29.8312430327322,-62.4345484392352,
-229.805512947091));
#226956=CARTESIAN_POINT('Ctrl Pts',(30.6933548791156,-62.8642478097168,
-229.014529680654));
#226957=CARTESIAN_POINT('Ctrl Pts',(31.5553928365677,-63.294139004949,-228.223577554036));
#226958=CARTESIAN_POINT('Ctrl Pts',(33.279468751472,-64.1539213954133,-226.641673300801));
#226959=CARTESIAN_POINT('Ctrl Pts',(35.0032446885496,-65.0144779934189,
-225.059892398919));
#226960=CARTESIAN_POINT('Ctrl Pts',(36.7268700953622,-65.8757200976626,
-223.47835238333));
#226961=CARTESIAN_POINT('Ctrl Pts',(40.1741209089872,-67.59820430615,-220.315272352152));
#226962=CARTESIAN_POINT('Ctrl Pts',(43.6206707171006,-69.3236781200416,
-217.153178316448));
#226963=CARTESIAN_POINT('Ctrl Pts',(47.0687185474759,-71.0494058698413,
-213.993041121244));
#226964=CARTESIAN_POINT('Ctrl Pts',(26.4599578544128,-60.6835996873818,
-232.962469394759));
#226965=CARTESIAN_POINT('Ctrl Pts',(27.3226882880111,-61.1109358874724,
-232.172413742166));
#226966=CARTESIAN_POINT('Ctrl Pts',(28.1852243300615,-61.5385403473352,
-231.38229745923));
#226967=CARTESIAN_POINT('Ctrl Pts',(29.0475520792886,-61.9664437404056,
-230.59212149004));
#226968=CARTESIAN_POINT('Ctrl Pts',(29.9098798285159,-62.3943471334761,
-229.801945520851));
#226969=CARTESIAN_POINT('Ctrl Pts',(30.7719992834121,-62.8225494254431,
-229.011709845514));
#226970=CARTESIAN_POINT('Ctrl Pts',(31.6338956495273,-63.2510852212965,
-228.221416509758));
#226971=CARTESIAN_POINT('Ctrl Pts',(33.3576883817577,-64.1081568130033,
-226.640829838246));
#226972=CARTESIAN_POINT('Ctrl Pts',(35.0805895076854,-64.966557214572,-225.060010587067));
#226973=CARTESIAN_POINT('Ctrl Pts',(36.8024707859496,-65.826619215018,-223.47899392047));
#226974=CARTESIAN_POINT('Ctrl Pts',(40.2462333424779,-67.54674321591,-220.316960587274));
#226975=CARTESIAN_POINT('Ctrl Pts',(43.6859139831841,-69.2733920499482,
-217.154070226751));
#226976=CARTESIAN_POINT('Ctrl Pts',(47.1204141132129,-71.0104275193633,
-213.991161055977));
#226977=CARTESIAN_POINT('',(26.5827141673278,-60.7444095340058,-232.85005));
#226978=CARTESIAN_POINT('',(25.3523897646956,-61.114818041723,-232.850050017304));
#226979=CARTESIAN_POINT('Ctrl Pts',(26.5827141673278,-60.7444095340058,
-232.85005));
#226980=CARTESIAN_POINT('Ctrl Pts',(26.5498602974857,-60.7619654664071,
-232.85005));
#226981=CARTESIAN_POINT('Ctrl Pts',(26.5113303465769,-60.7822271546458,
-232.85005));
#226982=CARTESIAN_POINT('Ctrl Pts',(26.4606301262639,-60.8074293646313,
-232.85005));
#226983=CARTESIAN_POINT('Ctrl Pts',(26.4425447461125,-60.8161729408406,
-232.850050000068));
#226984=CARTESIAN_POINT('Ctrl Pts',(26.387379862291,-60.8413638763713,-232.850050000068));
#226985=CARTESIAN_POINT('Ctrl Pts',(26.3144842454907,-60.8727542686262,
-232.85005));
#226986=CARTESIAN_POINT('Ctrl Pts',(26.1773907479988,-60.9311707559402,
-232.85005));
#226987=CARTESIAN_POINT('Ctrl Pts',(26.1245297076587,-60.9517310532191,
-232.850050000385));
#226988=CARTESIAN_POINT('Ctrl Pts',(26.0341733047922,-60.9830151315338,
-232.850050000385));
#226989=CARTESIAN_POINT('Ctrl Pts',(26.0105117414057,-60.991031970563,-232.850050000013));
#226990=CARTESIAN_POINT('Ctrl Pts',(25.9127285916415,-61.0232844425691,
-232.850050000013));
#226991=CARTESIAN_POINT('Ctrl Pts',(25.8684101044803,-61.0357482370295,
-232.85005));
#226992=CARTESIAN_POINT('Ctrl Pts',(25.7993139457216,-61.0535328833358,
-232.85005));
#226993=CARTESIAN_POINT('Ctrl Pts',(25.7541116741092,-61.0637255831382,
-232.850049999959));
#226994=CARTESIAN_POINT('Ctrl Pts',(25.6627893930028,-61.0828302915598,
-232.850049999959));
#226995=CARTESIAN_POINT('Ctrl Pts',(25.615699312088,-61.0907535096604,-232.850050000018));
#226996=CARTESIAN_POINT('Ctrl Pts',(25.526867967465,-61.1018068046011,-232.850050000018));
#226997=CARTESIAN_POINT('Ctrl Pts',(25.4884409885479,-61.1060188193343,
-232.85005));
#226998=CARTESIAN_POINT('Ctrl Pts',(25.4120097345976,-61.1125648908878,
-232.85005));
#226999=CARTESIAN_POINT('Ctrl Pts',(25.3780718523939,-61.1138880467002,
-232.85005));
#227000=CARTESIAN_POINT('Ctrl Pts',(25.3523897698351,-61.1148181836303,
-232.85005));
#227001=CARTESIAN_POINT('',(41.3748964727292,-72.6655519634609,-214.574036901741));
#227002=CARTESIAN_POINT('Ctrl Pts',(25.3523897720293,-61.114817956777,-232.850049970045));
#227003=CARTESIAN_POINT('Ctrl Pts',(30.6926995480076,-64.965287483333,-226.757725855014));
#227004=CARTESIAN_POINT('Ctrl Pts',(36.0337490039693,-68.8154400690564,
-220.665850944208));
#227005=CARTESIAN_POINT('Ctrl Pts',(41.3748962564069,-72.665551761209,-214.574036584249));
#227006=CARTESIAN_POINT('',(41.8937014876592,-72.6456596144325,-214.55018589167));
#227007=CARTESIAN_POINT('Ctrl Pts',(41.8937014876741,-72.6456596144277,
-214.55018589184));
#227008=CARTESIAN_POINT('Ctrl Pts',(41.8056994101465,-72.6489893684936,
-214.558007661286));
#227009=CARTESIAN_POINT('Ctrl Pts',(41.718477292423,-72.6523092351335,-214.564017375719));
#227010=CARTESIAN_POINT('Ctrl Pts',(41.5868861587709,-72.6573541922645,
-214.570073878361));
#227011=CARTESIAN_POINT('Ctrl Pts',(41.5433370473638,-72.659029772319,-214.571581799465));
#227012=CARTESIAN_POINT('Ctrl Pts',(41.4786634332878,-72.6615274743735,
-214.573057636199));
#227013=CARTESIAN_POINT('Ctrl Pts',(41.457775058709,-72.6623356153501,-214.573417187359));
#227014=CARTESIAN_POINT('Ctrl Pts',(41.4163541860228,-72.6639409738462,
-214.573897183768));
#227015=CARTESIAN_POINT('Ctrl Pts',(41.4039880684433,-72.6644207369686,
-214.574006351066));
#227016=CARTESIAN_POINT('Ctrl Pts',(41.3748964708024,-72.6655518905448,
-214.574037743505));
#227017=CARTESIAN_POINT('',(46.8664918907845,-70.8820281261857,-214.224994454969));
#227018=CARTESIAN_POINT('Ctrl Pts',(46.8664918907845,-70.8820281261857,
-214.224994454969));
#227019=CARTESIAN_POINT('Ctrl Pts',(46.7744407826316,-70.9511131613396,
-214.228242207602));
#227020=CARTESIAN_POINT('Ctrl Pts',(46.6807272794255,-71.0186224422586,
-214.231828155423));
#227021=CARTESIAN_POINT('Ctrl Pts',(46.5495229903282,-71.1092838966295,
-214.237663532242));
#227022=CARTESIAN_POINT('Ctrl Pts',(46.5126373770964,-71.1343646693495,
-214.239393263803));
#227023=CARTESIAN_POINT('Ctrl Pts',(46.3057923038342,-71.2726997130295,
-214.249757794807));
#227024=CARTESIAN_POINT('Ctrl Pts',(46.1254151596486,-71.3847351188338,
-214.258939730929));
#227025=CARTESIAN_POINT('Ctrl Pts',(45.7687595219198,-71.5880113823786,
-214.276898214196));
#227026=CARTESIAN_POINT('Ctrl Pts',(45.5977961988715,-71.6781131952535,
-214.286477772542));
#227027=CARTESIAN_POINT('Ctrl Pts',(45.3185014974946,-71.8138089269496,
-214.303180438964));
#227028=CARTESIAN_POINT('Ctrl Pts',(45.2120152038829,-71.8629654498041,
-214.309490070268));
#227029=CARTESIAN_POINT('Ctrl Pts',(45.046199456443,-71.9355486918505,-214.319240105013));
#227030=CARTESIAN_POINT('Ctrl Pts',(44.9874097484588,-71.9605279865678,
-214.322717043278));
#227031=CARTESIAN_POINT('Ctrl Pts',(44.7920434632078,-72.0410490486407,
-214.334469550239));
#227032=CARTESIAN_POINT('Ctrl Pts',(44.654581930388,-72.0937224739647,-214.343103618599));
#227033=CARTESIAN_POINT('Ctrl Pts',(44.0770061030001,-72.2986437300476,
-214.380774049815));
#227034=CARTESIAN_POINT('Ctrl Pts',(43.6246516203705,-72.4199541120767,
-214.411162580918));
#227035=CARTESIAN_POINT('Ctrl Pts',(43.0535644970527,-72.5255358981687,
-214.454758498744));
#227036=CARTESIAN_POINT('Ctrl Pts',(42.9403769886009,-72.5441841201559,
-214.463730404259));
#227037=CARTESIAN_POINT('Ctrl Pts',(42.745348495263,-72.5724398999531,-214.479262989101));
#227038=CARTESIAN_POINT('Ctrl Pts',(42.6635003407055,-72.5831344326108,
-214.485726488452));
#227039=CARTESIAN_POINT('Ctrl Pts',(42.3528138940059,-72.6193128180452,
-214.510537926902));
#227040=CARTESIAN_POINT('Ctrl Pts',(42.1239061674215,-72.6369493090089,
-214.529724921202));
#227041=CARTESIAN_POINT('Ctrl Pts',(41.8937014876739,-72.6456596144296,
-214.550185891837));
#227042=CARTESIAN_POINT('Ctrl Pts',(26.5827166017585,-60.7444082341964,
-232.850049999054));
#227043=CARTESIAN_POINT('Ctrl Pts',(27.4045078646348,-61.1514990596195,
-232.097463289075));
#227044=CARTESIAN_POINT('Ctrl Pts',(28.2261236616022,-61.5588353729273,
-231.344820212495));
#227045=CARTESIAN_POINT('Ctrl Pts',(29.0475520765728,-61.9664437417409,
-230.592121490192));
#227046=CARTESIAN_POINT('Ctrl Pts',(29.9098779960546,-62.3943462284576,
-229.801947196275));
#227047=CARTESIAN_POINT('Ctrl Pts',(30.7719974086774,-62.8225485010969,
-229.011711557785));
#227048=CARTESIAN_POINT('Ctrl Pts',(31.6338956347565,-63.2510852293973,
-228.221416510165));
#227049=CARTESIAN_POINT('Ctrl Pts',(33.3576804074389,-64.1081528789503,
-226.640837124115));
#227050=CARTESIAN_POINT('Ctrl Pts',(35.0805811947291,-64.9665531261144,
-225.060018166533));
#227051=CARTESIAN_POINT('Ctrl Pts',(36.8024706731575,-65.8266192882738,
-223.478993919512));
#227052=CARTESIAN_POINT('Ctrl Pts',(40.1613324575101,-67.5043363544868,
-220.394915649693));
#227053=CARTESIAN_POINT('Ctrl Pts',(43.5163436116641,-69.1882768775022,
-217.309992116266));
#227054=CARTESIAN_POINT('Ctrl Pts',(46.8664917825725,-70.8820279699867,
-214.22499462617));
#227055=CARTESIAN_POINT('Ctrl Pts',(28.811481324712,36.2672238003158,-232.961663720964));
#227056=CARTESIAN_POINT('Ctrl Pts',(29.5645263655861,36.6399226415611,-232.177270818232));
#227057=CARTESIAN_POINT('Ctrl Pts',(30.3173414199567,37.0126142771829,-231.392803581211));
#227058=CARTESIAN_POINT('Ctrl Pts',(31.069911071871,37.385324556228,-230.608260371606));
#227059=CARTESIAN_POINT('Ctrl Pts',(31.8224807237854,37.7580348352731,-229.823717162));
#227060=CARTESIAN_POINT('Ctrl Pts',(32.5748049718356,38.1307637318441,-229.039097966911));
#227061=CARTESIAN_POINT('Ctrl Pts',(33.326867581659,38.5035402264522,-228.254401763819));
#227062=CARTESIAN_POINT('Ctrl Pts',(34.8309928013059,39.2490932156681,-226.685009357635));
#227063=CARTESIAN_POINT('Ctrl Pts',(36.3340721635766,39.9948325139069,-225.115307761803));
#227064=CARTESIAN_POINT('Ctrl Pts',(37.8359666905481,40.7410341111373,-223.545299801334));
#227065=CARTESIAN_POINT('Ctrl Pts',(40.8397557444911,42.233437305598,-220.405283880397));
#227066=CARTESIAN_POINT('Ctrl Pts',(43.8388051696003,43.7275965705222,-217.264000696622));
#227067=CARTESIAN_POINT('Ctrl Pts',(46.8319258491792,45.2266492383781,-214.121813627025));
#227068=CARTESIAN_POINT('Ctrl Pts',(28.7546828535794,36.2946048538794,-232.967923270373));
#227069=CARTESIAN_POINT('Ctrl Pts',(29.5075354964661,36.6682851435785,-232.18296040294));
#227070=CARTESIAN_POINT('Ctrl Pts',(30.260203356218,37.041928546648,-231.397949783602));
#227071=CARTESIAN_POINT('Ctrl Pts',(31.012687072449,37.4155430678739,-230.612897000714));
#227072=CARTESIAN_POINT('Ctrl Pts',(31.7651707886799,37.7891575890997,-229.827844217825));
#227073=CARTESIAN_POINT('Ctrl Pts',(32.5174703341753,38.1627432696007,-229.042749264024));
#227074=CARTESIAN_POINT('Ctrl Pts',(33.2695884278607,38.5363065970483,-228.257619016064));
#227075=CARTESIAN_POINT('Ctrl Pts',(34.7738246152316,39.2834332519434,-226.687358520144));
#227076=CARTESIAN_POINT('Ctrl Pts',(36.2773319082997,40.0304737792722,-225.116955396868));
#227077=CARTESIAN_POINT('Ctrl Pts',(37.7801639596043,40.7774501421753,-223.546481445834));
#227078=CARTESIAN_POINT('Ctrl Pts',(40.7858280622135,42.2714028679817,-220.405533543764));
#227079=CARTESIAN_POINT('Ctrl Pts',(43.788714991937,43.7652295475826,-217.264288793245));
#227080=CARTESIAN_POINT('Ctrl Pts',(46.7899896154941,45.2580776239732,-214.123556902107));
#227081=CARTESIAN_POINT('Ctrl Pts',(28.7154411546286,36.3084021057357,-232.976115945722));
#227082=CARTESIAN_POINT('Ctrl Pts',(29.4668698155753,36.6840531650027,-232.190299004213));
#227083=CARTESIAN_POINT('Ctrl Pts',(30.2182278401491,37.0595754047064,-231.404498974189));
#227084=CARTESIAN_POINT('Ctrl Pts',(30.9695388460574,37.4349506564828,-230.618731646667));
#227085=CARTESIAN_POINT('Ctrl Pts',(31.7208498519656,37.8103259082591,-229.832964319146));
#227086=CARTESIAN_POINT('Ctrl Pts',(32.4721138113312,38.1855541511188,-229.047229657302));
#227087=CARTESIAN_POINT('Ctrl Pts',(33.2233504871597,38.560617867947,-228.261540054661));
#227088=CARTESIAN_POINT('Ctrl Pts',(34.7258238388169,39.3107453016035,-226.690160849379));
#227089=CARTESIAN_POINT('Ctrl Pts',(36.2281910213353,40.0602134993234,-225.11896419415));
#227090=CARTESIAN_POINT('Ctrl Pts',(37.7305702572955,40.808893913642,-223.548016395278));
#227091=CARTESIAN_POINT('Ctrl Pts',(40.7353287292159,42.3062547422792,-220.406120797533));
#227092=CARTESIAN_POINT('Ctrl Pts',(43.7401655452353,43.8004441673505,-217.265239990539));
#227093=CARTESIAN_POINT('Ctrl Pts',(46.7455490797692,45.2906625887397,-214.1255539434));
#227094=CARTESIAN_POINT('Ctrl Pts',(28.6836693563314,36.3172916302978,-232.984586371767));
#227095=CARTESIAN_POINT('Ctrl Pts',(29.4328038186657,36.6955273714839,-232.197666951892));
#227096=CARTESIAN_POINT('Ctrl Pts',(30.1821597301324,37.0733995616469,-231.410933917807));
#227097=CARTESIAN_POINT('Ctrl Pts',(30.9317206554361,37.4509071831741,-230.624372601034));
#227098=CARTESIAN_POINT('Ctrl Pts',(31.6812815807397,37.8284148047014,-229.83781128426));
#227099=CARTESIAN_POINT('Ctrl Pts',(32.4310475185464,38.2055578694789,-229.051421689267));
#227100=CARTESIAN_POINT('Ctrl Pts',(33.1810027512314,38.5823363130566,-228.265190292231));
#227101=CARTESIAN_POINT('Ctrl Pts',(34.6809132166015,39.3358932002121,-226.69272749816));
#227102=CARTESIAN_POINT('Ctrl Pts',(36.1815801312299,40.0879909915779,-225.120896504533));
#227103=CARTESIAN_POINT('Ctrl Pts',(37.6828865095192,40.8386380933409,-223.549601777981));
#227104=CARTESIAN_POINT('Ctrl Pts',(40.6854992660978,42.3399322968669,-220.407012324875));
#227105=CARTESIAN_POINT('Ctrl Pts',(43.6906591856765,43.835419294533,-217.266555597716));
#227106=CARTESIAN_POINT('Ctrl Pts',(46.6975653758367,45.3252553963054,-214.127639057046));
#227107=CARTESIAN_POINT('Ctrl Pts',(28.6518975580342,36.3261811548597,-232.993056797812));
#227108=CARTESIAN_POINT('Ctrl Pts',(29.398737821756,36.7070015779651,-232.205034899571));
#227109=CARTESIAN_POINT('Ctrl Pts',(30.1460916201158,37.0872237185874,-231.417368861425));
#227110=CARTESIAN_POINT('Ctrl Pts',(30.8939024648147,37.4668637098655,-230.6300135554));
#227111=CARTESIAN_POINT('Ctrl Pts',(31.6417133095137,37.8465037011437,-229.842658249374));
#227112=CARTESIAN_POINT('Ctrl Pts',(32.3899812257617,38.225561587839,-229.055613721231));
#227113=CARTESIAN_POINT('Ctrl Pts',(33.1386550153031,38.6040547581662,-228.268840529801));
#227114=CARTESIAN_POINT('Ctrl Pts',(34.6360025943859,39.3610410988206,-226.69529414694));
#227115=CARTESIAN_POINT('Ctrl Pts',(36.1349692411245,40.1157684838324,-225.122828814917));
#227116=CARTESIAN_POINT('Ctrl Pts',(37.6352027617429,40.8683822730397,-223.551187160683));
#227117=CARTESIAN_POINT('Ctrl Pts',(40.6356698029797,42.3736098514546,-220.407903852216));
#227118=CARTESIAN_POINT('Ctrl Pts',(43.6411528261178,43.8703944217154,-217.267871204892));
#227119=CARTESIAN_POINT('Ctrl Pts',(46.6495816719042,45.3598482038711,-214.129724170691));
#227120=CARTESIAN_POINT('Ctrl Pts',(28.6268841990247,36.3309725707821,-233.001464510274));
#227121=CARTESIAN_POINT('Ctrl Pts',(29.3705829350163,36.7149391799052,-232.212094488675));
#227122=CARTESIAN_POINT('Ctrl Pts',(30.1153093882969,37.097903168935,-231.423383830337));
#227123=CARTESIAN_POINT('Ctrl Pts',(30.8608649961116,37.4799665704452,-230.635190635126));
#227124=CARTESIAN_POINT('Ctrl Pts',(31.6064206039263,37.8620299719552,-229.846997439915));
#227125=CARTESIAN_POINT('Ctrl Pts',(32.3528061165871,38.2431927923484,-229.059322438005));
#227126=CARTESIAN_POINT('Ctrl Pts',(33.0998655521803,38.6235441089799,-228.272058763276));
#227127=CARTESIAN_POINT('Ctrl Pts',(34.5939844233666,39.3842467422428,-226.697531413816));
#227128=CARTESIAN_POINT('Ctrl Pts',(36.0907758686695,40.1417143786457,-225.124632267967));
#227129=CARTESIAN_POINT('Ctrl Pts',(37.5893556701601,40.8965147834728,-223.552789136373));
#227130=CARTESIAN_POINT('Ctrl Pts',(40.5865152731412,42.4061155931272,-220.409102873187));
#227131=CARTESIAN_POINT('Ctrl Pts',(43.5906769196312,43.9051501453593,-217.269543315155));
#227132=CARTESIAN_POINT('Ctrl Pts',(46.598054657578,45.3964490821564,-214.13189626583));
#227133=CARTESIAN_POINT('Ctrl Pts',(28.5917373044541,36.3459190971896,-233.004412799005));
#227134=CARTESIAN_POINT('Ctrl Pts',(29.3336456870839,36.7317236596899,-232.214541575288));
#227135=CARTESIAN_POINT('Ctrl Pts',(30.0768533355596,37.1163079376712,-231.425484075423));
#227136=CARTESIAN_POINT('Ctrl Pts',(30.8210649438641,37.4998384795814,-230.63703601277));
#227137=CARTESIAN_POINT('Ctrl Pts',(31.5652765521686,37.8833690214916,-229.848587950118));
#227138=CARTESIAN_POINT('Ctrl Pts',(32.3104940183536,38.2658454573702,-229.060750983011));
#227139=CARTESIAN_POINT('Ctrl Pts',(33.056499757863,38.6474031071304,-228.273381017246));
#227140=CARTESIAN_POINT('Ctrl Pts',(34.5485112368819,39.4105184066505,-226.698641085717));
#227141=CARTESIAN_POINT('Ctrl Pts',(36.0436413480666,40.1699780267802,-225.125745165631));
#227142=CARTESIAN_POINT('Ctrl Pts',(37.5407436150405,40.9265749496157,-223.553976309726));
#227143=CARTESIAN_POINT('Ctrl Pts',(40.5349481489884,42.439768795287,-220.410438597917));
#227144=CARTESIAN_POINT('Ctrl Pts',(43.536857304037,43.9416524034681,-217.271298591679));
#227145=CARTESIAN_POINT('Ctrl Pts',(46.5420263558244,45.4357480033572,-214.134039310084));
#227146=CARTESIAN_POINT('Ctrl Pts',(28.5214435153128,36.3758121500046,-233.010309376466));
#227147=CARTESIAN_POINT('Ctrl Pts',(29.2597711912192,36.7652926192596,-232.219435748514));
#227148=CARTESIAN_POINT('Ctrl Pts',(29.9999412300851,37.1531174751436,-231.429684565593));
#227149=CARTESIAN_POINT('Ctrl Pts',(30.741464839369,37.539582297854,-230.640726768058));
#227150=CARTESIAN_POINT('Ctrl Pts',(31.482988448653,37.9260471205643,-229.851768970523));
#227151=CARTESIAN_POINT('Ctrl Pts',(32.2258698218865,38.3111507874138,-229.063608073021));
#227152=CARTESIAN_POINT('Ctrl Pts',(32.9697681692284,38.6951211034311,-228.276025525187));
#227153=CARTESIAN_POINT('Ctrl Pts',(34.4575648639124,39.4630617354659,-226.700860429518));
#227154=CARTESIAN_POINT('Ctrl Pts',(35.9493723068607,40.2265053230493,-225.12797096096));
#227155=CARTESIAN_POINT('Ctrl Pts',(37.4435195048015,40.9866952819017,-223.556350656432));
#227156=CARTESIAN_POINT('Ctrl Pts',(40.4318139006829,42.5070751996064,-220.413110047378));
#227157=CARTESIAN_POINT('Ctrl Pts',(43.4292180728484,44.0146569196856,-217.274809144726));
#227158=CARTESIAN_POINT('Ctrl Pts',(46.4299697523172,45.5143458457586,-214.138325398592));
#227159=CARTESIAN_POINT('Ctrl Pts',(28.4570930103932,36.3999229344231,-233.01764278364));
#227160=CARTESIAN_POINT('Ctrl Pts',(29.1907924187055,36.7937286595564,-232.225654625907));
#227161=CARTESIAN_POINT('Ctrl Pts',(29.9270887829037,37.1852362696201,-231.435207732835));
#227162=CARTESIAN_POINT('Ctrl Pts',(30.6652441216594,37.5749249395508,-230.645813317621));
#227163=CARTESIAN_POINT('Ctrl Pts',(31.403399460415,37.9646136094813,-229.856418902407));
#227164=CARTESIAN_POINT('Ctrl Pts',(32.1434103450723,38.3524880305972,-229.06807638164));
#227165=CARTESIAN_POINT('Ctrl Pts',(32.884729259185,38.7389448417248,-228.280447107729));
#227166=CARTESIAN_POINT('Ctrl Pts',(34.3673670874105,39.5118584639798,-226.705188559907));
#227167=CARTESIAN_POINT('Ctrl Pts',(35.8551295881073,40.2791804937992,-225.132717154794));
#227168=CARTESIAN_POINT('Ctrl Pts',(37.3455152808298,41.0429334678829,-223.561600885392));
#227169=CARTESIAN_POINT('Ctrl Pts',(40.3262866662749,42.5704394160502,-220.419368346588));
#227170=CARTESIAN_POINT('Ctrl Pts',(43.3172378956761,44.0839938761798,-217.282413069526));
#227171=CARTESIAN_POINT('Ctrl Pts',(46.3111674951612,45.590157065165,-214.147042344173));
#227172=CARTESIAN_POINT('Ctrl Pts',(28.404523824249,36.4142111160726,-233.028222391732));
#227173=CARTESIAN_POINT('Ctrl Pts',(29.1296788023777,36.8148442685854,-232.23397055258));
#227174=CARTESIAN_POINT('Ctrl Pts',(29.8595774687733,37.2115210846296,-231.442464211111));
#227175=CARTESIAN_POINT('Ctrl Pts',(30.5921210784794,37.6056911614944,-230.652400010517));
#227176=CARTESIAN_POINT('Ctrl Pts',(31.3246646881855,37.9998612383593,-229.862335809922));
#227177=CARTESIAN_POINT('Ctrl Pts',(32.0599114204536,38.3914951944436,-229.073755169551));
#227178=CARTESIAN_POINT('Ctrl Pts',(32.7968044445028,38.7814033859296,-228.286041512615));
#227179=CARTESIAN_POINT('Ctrl Pts',(34.2705904926014,39.5612197689016,-226.710614198745));
#227180=CARTESIAN_POINT('Ctrl Pts',(35.7508066075144,40.334264217189,-225.138570075993));
#227181=CARTESIAN_POINT('Ctrl Pts',(37.2337704007868,41.1036371719424,-223.567901121106));
#227182=CARTESIAN_POINT('Ctrl Pts',(40.1996979873318,42.6423830814493,-220.426563211331));
#227183=CARTESIAN_POINT('Ctrl Pts',(43.1764747241572,44.166666266985,-217.290698996916));
#227184=CARTESIAN_POINT('Ctrl Pts',(46.1558000266483,45.6842043061087,-214.156194672008));
#227185=CARTESIAN_POINT('Ctrl Pts',(28.3519546381049,36.428499297722,-233.038801999823));
#227186=CARTESIAN_POINT('Ctrl Pts',(29.0685651860499,36.8359598776144,-232.242286479252));
#227187=CARTESIAN_POINT('Ctrl Pts',(29.7920661546429,37.237805899639,-231.449720689388));
#227188=CARTESIAN_POINT('Ctrl Pts',(30.5189980352994,37.6364573834381,-230.658986703413));
#227189=CARTESIAN_POINT('Ctrl Pts',(31.2459299159559,38.0351088672372,-229.868252717438));
#227190=CARTESIAN_POINT('Ctrl Pts',(31.9764124958348,38.4305023582899,-229.079433957463));
#227191=CARTESIAN_POINT('Ctrl Pts',(32.7088796298207,38.8238619301343,-228.291635917502));
#227192=CARTESIAN_POINT('Ctrl Pts',(34.1738138977924,39.6105810738233,-226.716039837583));
#227193=CARTESIAN_POINT('Ctrl Pts',(35.6464836269217,40.3893479405787,-225.144422997191));
#227194=CARTESIAN_POINT('Ctrl Pts',(37.122025520744,41.1643408760019,-223.574201356819));
#227195=CARTESIAN_POINT('Ctrl Pts',(40.0731093083885,42.7143267468484,-220.433758076075));
#227196=CARTESIAN_POINT('Ctrl Pts',(43.0357115526382,44.2493386577901,-217.298984924306));
#227197=CARTESIAN_POINT('Ctrl Pts',(46.0004325581354,45.7782515470524,-214.165346999843));
#227198=CARTESIAN_POINT('Ctrl Pts',(28.3059764599357,36.4381392896391,-233.049914691876));
#227199=CARTESIAN_POINT('Ctrl Pts',(29.0134341565471,36.8517973543695,-232.2517252646));
#227200=CARTESIAN_POINT('Ctrl Pts',(29.7298662406445,37.2584322913983,-231.458644991706));
#227201=CARTESIAN_POINT('Ctrl Pts',(30.4501559342506,37.6615657444315,-230.667588797462));
#227202=CARTESIAN_POINT('Ctrl Pts',(31.1704456278568,38.0646991974648,-229.876532603218));
#227203=CARTESIAN_POINT('Ctrl Pts',(31.8948332263391,38.464199380249,-229.087662159456));
#227204=CARTESIAN_POINT('Ctrl Pts',(32.6213338477217,38.8616012616129,-228.299865510382));
#227205=CARTESIAN_POINT('Ctrl Pts',(34.0743350904866,39.6564050243409,-226.724272212234));
#227206=CARTESIAN_POINT('Ctrl Pts',(35.5355956082815,40.4430010719712,-225.152884082953));
#227207=CARTESIAN_POINT('Ctrl Pts',(36.9996482985433,41.2260174336112,-223.582843540199));
#227208=CARTESIAN_POINT('Ctrl Pts',(39.9277536790671,42.792050156891,-220.442762454692));
#227209=CARTESIAN_POINT('Ctrl Pts',(42.8672926273489,44.3436915722972,-217.308286098109));
#227210=CARTESIAN_POINT('Ctrl Pts',(45.8087507912112,45.889714665516,-214.174855839415));
#227211=CARTESIAN_POINT('Ctrl Pts',(28.2536248719719,36.45164456484,-233.058476234802));
#227212=CARTESIAN_POINT('Ctrl Pts',(28.956246064681,36.8674691193729,-232.261151946464));
#227213=CARTESIAN_POINT('Ctrl Pts',(29.6674872789167,37.2766580792002,-231.468687139439));
#227214=CARTESIAN_POINT('Ctrl Pts',(30.3823793991597,37.6826022896234,-230.678128469586));
#227215=CARTESIAN_POINT('Ctrl Pts',(31.0972715194027,38.0885465000466,-229.887569799732));
#227216=CARTESIAN_POINT('Ctrl Pts',(31.8160539135098,38.4911129154006,-229.099074756418));
#227217=CARTESIAN_POINT('Ctrl Pts',(32.5368266733684,38.8917474183737,-228.311589632248));
#227218=CARTESIAN_POINT('Ctrl Pts',(33.9783721930855,39.6930164243198,-226.736619383908));
#227219=CARTESIAN_POINT('Ctrl Pts',(35.4277003933768,40.4867262619234,-225.16560579597));
#227220=CARTESIAN_POINT('Ctrl Pts',(36.8796336124663,41.2771645198602,-223.595856775541));
#227221=CARTESIAN_POINT('Ctrl Pts',(39.7835000506455,42.8580410357338,-220.456358734683));
#227222=CARTESIAN_POINT('Ctrl Pts',(42.6980566108585,44.4257389283559,-217.322125580858));
#227223=CARTESIAN_POINT('Ctrl Pts',(45.6143789670139,45.9882588716253,-214.18887606046));
#227224=CARTESIAN_POINT('Ctrl Pts',(28.2012732840083,36.4651498400409,-233.067037777728));
#227225=CARTESIAN_POINT('Ctrl Pts',(28.8990579728149,36.8831408843765,-232.270578628329));
#227226=CARTESIAN_POINT('Ctrl Pts',(29.6051083171889,37.2948838670021,-231.478729287174));
#227227=CARTESIAN_POINT('Ctrl Pts',(30.3146028640688,37.7036388348153,-230.688668141709));
#227228=CARTESIAN_POINT('Ctrl Pts',(31.0240974109487,38.1123938026283,-229.898606996244));
#227229=CARTESIAN_POINT('Ctrl Pts',(31.7372746006804,38.5180264505524,-229.110487353379));
#227230=CARTESIAN_POINT('Ctrl Pts',(32.4523194990151,38.9218935751344,-228.323313754114));
#227231=CARTESIAN_POINT('Ctrl Pts',(33.8824092956843,39.7296278242987,-226.748966555583));
#227232=CARTESIAN_POINT('Ctrl Pts',(35.3198051784721,40.5304514518755,-225.178327508987));
#227233=CARTESIAN_POINT('Ctrl Pts',(36.7596189263893,41.3283116061093,-223.608870010882));
#227234=CARTESIAN_POINT('Ctrl Pts',(39.6392464222237,42.9240319145765,-220.469955014674));
#227235=CARTESIAN_POINT('Ctrl Pts',(42.5288205943682,44.5077862844145,-217.335965063606));
#227236=CARTESIAN_POINT('Ctrl Pts',(45.4200071428167,46.0868030777345,-214.202896281505));
#227237=CARTESIAN_POINT('Ctrl Pts',(28.1478839352704,36.477738188472,-233.075828397652));
#227238=CARTESIAN_POINT('Ctrl Pts',(28.8401821644882,36.8980247568529,-232.280146620628));
#227239=CARTESIAN_POINT('Ctrl Pts',(29.5403735836712,37.3124695266811,-231.488827353208));
#227240=CARTESIAN_POINT('Ctrl Pts',(30.2438219273577,37.724159990219,-230.69919181366));
#227241=CARTESIAN_POINT('Ctrl Pts',(30.9472702710442,38.1358504537568,-229.909556274112));
#227242=CARTESIAN_POINT('Ctrl Pts',(31.6542085880957,38.5446552966966,-229.121751411976));
#227243=CARTESIAN_POINT('Ctrl Pts',(32.3629082299762,38.9518393215846,-228.334837279587));
#227244=CARTESIAN_POINT('Ctrl Pts',(33.7803075137374,39.7662073713606,-226.761009014808));
#227245=CARTESIAN_POINT('Ctrl Pts',(35.204598643849,40.5742293326632,-225.190672920757));
#227246=CARTESIAN_POINT('Ctrl Pts',(36.6311571182707,41.3795423287398,-223.621449299399));
#227247=CARTESIAN_POINT('Ctrl Pts',(39.4842740671139,42.9901683208929,-220.483002056683));
#227248=CARTESIAN_POINT('Ctrl Pts',(42.3467314369201,44.5898405345135,-217.349193442931));
#227249=CARTESIAN_POINT('Ctrl Pts',(45.2106913777692,46.1851488860278,-214.216254607896));
#227250=CARTESIAN_POINT('Ctrl Pts',(28.0986638608654,36.4864396316355,-233.086219707902));
#227251=CARTESIAN_POINT('Ctrl Pts',(28.7855090882708,36.908671912885,-232.291339757935));
#227252=CARTESIAN_POINT('Ctrl Pts',(29.4797969634702,37.3255148395588,-231.50054713919));
#227253=CARTESIAN_POINT('Ctrl Pts',(30.1771392417705,37.7398414336408,-230.711331015122));
#227254=CARTESIAN_POINT('Ctrl Pts',(30.8744815200707,38.1541680277229,-229.922114891055));
#227255=CARTESIAN_POINT('Ctrl Pts',(31.5751008302705,38.565853402466,-229.134613456395));
#227256=CARTESIAN_POINT('Ctrl Pts',(32.2773697651967,38.9760615626091,-228.347946926293));
#227257=CARTESIAN_POINT('Ctrl Pts',(33.6819076350491,39.7964778828953,-226.77461386609));
#227258=CARTESIAN_POINT('Ctrl Pts',(35.092901360331,40.6111090059392,-225.204554400508));
#227259=CARTESIAN_POINT('Ctrl Pts',(36.506013012055,41.4232755079927,-223.635540355772));
#227260=CARTESIAN_POINT('Ctrl Pts',(39.3322363155031,43.0476085120996,-220.4975122663));
#227261=CARTESIAN_POINT('Ctrl Pts',(42.1671908002668,44.6619661512638,-217.363841724096));
#227262=CARTESIAN_POINT('Ctrl Pts',(45.0035463653253,46.2723209746968,-214.23099286058));
#227263=CARTESIAN_POINT('Ctrl Pts',(28.0494437864605,36.495141074799,-233.096611018152));
#227264=CARTESIAN_POINT('Ctrl Pts',(28.7308360120535,36.9193190689171,-232.302532895241));
#227265=CARTESIAN_POINT('Ctrl Pts',(29.4192203432693,37.3385601524366,-231.512266925172));
#227266=CARTESIAN_POINT('Ctrl Pts',(30.1104565561833,37.7555228770627,-230.723470216585));
#227267=CARTESIAN_POINT('Ctrl Pts',(30.8016927690973,38.1724856016888,-229.934673507997));
#227268=CARTESIAN_POINT('Ctrl Pts',(31.4959930724453,38.5870515082353,-229.147475500813));
#227269=CARTESIAN_POINT('Ctrl Pts',(32.1918313004172,39.0002838036336,-228.361056572999));
#227270=CARTESIAN_POINT('Ctrl Pts',(33.5835077563608,39.82674839443,-226.788218717371));
#227271=CARTESIAN_POINT('Ctrl Pts',(34.981204076813,40.6479886792153,-225.218435880259));
#227272=CARTESIAN_POINT('Ctrl Pts',(36.3808689058395,41.4670086872456,-223.649631412145));
#227273=CARTESIAN_POINT('Ctrl Pts',(39.1801985638925,43.1050487033063,-220.512022475916));
#227274=CARTESIAN_POINT('Ctrl Pts',(41.9876501636135,44.7340917680141,-217.378490005261));
#227275=CARTESIAN_POINT('Ctrl Pts',(44.7964013528814,46.3594930633657,-214.245731113265));
#227276=CARTESIAN_POINT('Ctrl Pts',(28.0080391125216,36.4973005693799,-233.110468735653));
#227277=CARTESIAN_POINT('Ctrl Pts',(28.6837630172434,36.9232178045066,-232.317064221622));
#227278=CARTESIAN_POINT('Ctrl Pts',(29.3659479014001,37.344725328937,-231.527181895889));
#227279=CARTESIAN_POINT('Ctrl Pts',(30.0508000045693,37.7641807455897,-230.73868064955));
#227280=CARTESIAN_POINT('Ctrl Pts',(30.7356521077386,38.1836361622425,-229.950179403211));
#227281=CARTESIAN_POINT('Ctrl Pts',(31.423362687773,38.6009356192233,-229.163175043223));
#227282=CARTESIAN_POINT('Ctrl Pts',(32.1125182041085,39.0170287271978,-228.376907373423));
#227283=CARTESIAN_POINT('Ctrl Pts',(33.4908292367796,39.849214943147,-226.804372033824));
#227284=CARTESIAN_POINT('Ctrl Pts',(34.8747945827483,40.6766756124477,-225.234724065505));
#227285=CARTESIAN_POINT('Ctrl Pts',(36.2606283272941,41.5021120342519,-223.666013493501));
#227286=CARTESIAN_POINT('Ctrl Pts',(39.0322958163857,43.1529848778602,-220.528592349493));
#227287=CARTESIAN_POINT('Ctrl Pts',(41.8116561460013,44.7956635400236,-217.395064921228));
#227288=CARTESIAN_POINT('Ctrl Pts',(44.5922760617361,46.4350000670329,-214.262289445508));
#227289=CARTESIAN_POINT('Ctrl Pts',(27.9635611001738,36.4990952898012,-233.124907406577));
#227290=CARTESIAN_POINT('Ctrl Pts',(28.6335193341731,36.9265762879192,-232.332215621801));
#227291=CARTESIAN_POINT('Ctrl Pts',(29.3093382993415,37.3501779403658,-231.542719800075));
#227292=CARTESIAN_POINT('Ctrl Pts',(29.9876295989316,37.7719445682467,-230.754510440041));
#227293=CARTESIAN_POINT('Ctrl Pts',(30.6659208985218,38.1937111961276,-229.966301080007));
#227294=CARTESIAN_POINT('Ctrl Pts',(31.346850346985,38.6135550182896,-229.179478141202));
#227295=CARTESIAN_POINT('Ctrl Pts',(32.0291309789057,39.032311940978,-228.393348201459));
#227296=CARTESIAN_POINT('Ctrl Pts',(33.3936922427472,39.869825786355,-226.821088321973));
#227297=CARTESIAN_POINT('Ctrl Pts',(34.7635386549114,40.7030825753783,-225.251542754464));
#227298=CARTESIAN_POINT('Ctrl Pts',(36.1351659076718,41.5344930728638,-223.682897927105));
#227299=CARTESIAN_POINT('Ctrl Pts',(38.8784204131928,43.1973140678347,-220.545608272386));
#227300=CARTESIAN_POINT('Ctrl Pts',(41.6289795635766,44.8526757118206,-217.412042386738));
#227301=CARTESIAN_POINT('Ctrl Pts',(44.3807833059246,46.5049749771785,-214.279216302521));
#227302=CARTESIAN_POINT('Ctrl Pts',(27.9190830878262,36.5008900102226,-233.139346077501));
#227303=CARTESIAN_POINT('Ctrl Pts',(28.5832756511028,36.9299347713319,-232.34736702198));
#227304=CARTESIAN_POINT('Ctrl Pts',(29.2527286972829,37.3556305517945,-231.558257704261));
#227305=CARTESIAN_POINT('Ctrl Pts',(29.9244591932939,37.7797083909036,-230.770340230532));
#227306=CARTESIAN_POINT('Ctrl Pts',(30.5961896893049,38.2037862300127,-229.982422756802));
#227307=CARTESIAN_POINT('Ctrl Pts',(31.270338006197,38.626174417356,-229.195781239181));
#227308=CARTESIAN_POINT('Ctrl Pts',(31.945743753703,39.0475951547582,-228.409789029494));
#227309=CARTESIAN_POINT('Ctrl Pts',(33.2965552487149,39.8904366295628,-226.837804610121));
#227310=CARTESIAN_POINT('Ctrl Pts',(34.6522827270746,40.7294895383089,-225.268361443424));
#227311=CARTESIAN_POINT('Ctrl Pts',(36.0097034880497,41.5668741114757,-223.699782360708));
#227312=CARTESIAN_POINT('Ctrl Pts',(38.7245450099999,43.2416432578092,-220.56262419528));
#227313=CARTESIAN_POINT('Ctrl Pts',(41.4463029811519,44.9096878836177,-217.429019852247));
#227314=CARTESIAN_POINT('Ctrl Pts',(44.169290550113,46.5749498873242,-214.296143159535));
#227315=CARTESIAN_POINT('Ctrl Pts',(27.864102341306,36.5072827075644,-233.150523220819));
#227316=CARTESIAN_POINT('Ctrl Pts',(28.523209294369,36.9372652461925,-232.359742014691));
#227317=CARTESIAN_POINT('Ctrl Pts',(29.1867208754184,37.3645078673026,-231.571344200798));
#227318=CARTESIAN_POINT('Ctrl Pts',(29.8522042860804,37.7903963835451,-230.783978402477));
#227319=CARTESIAN_POINT('Ctrl Pts',(30.5176876967423,38.2162848997876,-229.996612604157));
#227320=CARTESIAN_POINT('Ctrl Pts',(31.1852516294648,38.6407638308456,-229.210342644892));
#227321=CARTESIAN_POINT('Ctrl Pts',(31.8539198779964,39.0644229189197,-228.424644456938));
#227322=CARTESIAN_POINT('Ctrl Pts',(33.1912563750597,39.9117410950679,-226.853248081031));
#227323=CARTESIAN_POINT('Ctrl Pts',(34.532908053201,40.7558486265409,-225.284087692051));
#227324=CARTESIAN_POINT('Ctrl Pts',(35.8760898321597,41.5985105380543,-223.715714506644));
#227325=CARTESIAN_POINT('Ctrl Pts',(38.5624533900771,43.2838343610812,-220.578968135829));
#227326=CARTESIAN_POINT('Ctrl Pts',(41.2550333439266,44.9633461404957,-217.4454372649));
#227327=CARTESIAN_POINT('Ctrl Pts',(43.9487716799902,46.6404014421116,-214.312594508648));
#227328=CARTESIAN_POINT('Ctrl Pts',(27.8054264163448,36.5146074937637,-233.160277704479));
#227329=CARTESIAN_POINT('Ctrl Pts',(28.4608655062395,36.9445884335815,-232.371247983632));
#227330=CARTESIAN_POINT('Ctrl Pts',(29.1196314139931,37.372514313029,-231.584005383938));
#227331=CARTESIAN_POINT('Ctrl Pts',(29.7799261927146,37.7994041715398,-230.797562749801));
#227332=CARTESIAN_POINT('Ctrl Pts',(30.4402209714361,38.2262940300507,-230.011120115663));
#227333=CARTESIAN_POINT('Ctrl Pts',(31.1021216515676,38.6521081108545,-229.225521863909));
#227334=CARTESIAN_POINT('Ctrl Pts',(31.7648888134181,39.0772864601489,-228.440373573626));
#227335=CARTESIAN_POINT('Ctrl Pts',(33.090423137119,39.9276431587379,-226.87007699306));
#227336=CARTESIAN_POINT('Ctrl Pts',(34.4193423302246,40.7755094860917,-225.301539303434));
#227337=CARTESIAN_POINT('Ctrl Pts',(35.7494892631586,41.6222215800908,-223.73364023664));
#227338=CARTESIAN_POINT('Ctrl Pts',(38.4097831290267,43.3156457680889,-220.597842103052));
#227339=CARTESIAN_POINT('Ctrl Pts',(41.0750442414306,45.0044380406571,-217.464638507897));
#227340=CARTESIAN_POINT('Ctrl Pts',(43.7412542098013,46.69118281627,-214.332014574282));
#227341=CARTESIAN_POINT('Ctrl Pts',(27.7467504913837,36.5219322799631,-233.170032188139));
#227342=CARTESIAN_POINT('Ctrl Pts',(28.3985217181101,36.9519116209705,-232.382753952573));
#227343=CARTESIAN_POINT('Ctrl Pts',(29.0525419525678,37.3805207587552,-231.59666656708));
#227344=CARTESIAN_POINT('Ctrl Pts',(29.707648099349,37.8084119595345,-230.811147097123));
#227345=CARTESIAN_POINT('Ctrl Pts',(30.3627542461301,38.2363031603138,-230.025627627167));
#227346=CARTESIAN_POINT('Ctrl Pts',(31.0189916736704,38.6634523908632,-229.240701082927));
#227347=CARTESIAN_POINT('Ctrl Pts',(31.6758577488396,39.0901500013781,-228.456102690314));
#227348=CARTESIAN_POINT('Ctrl Pts',(32.9895898991783,39.9435452224079,-226.886905905089));
#227349=CARTESIAN_POINT('Ctrl Pts',(34.305776607248,40.7951703456425,-225.318990914817));
#227350=CARTESIAN_POINT('Ctrl Pts',(35.6228886941575,41.6459326221272,-223.751565966636));
#227351=CARTESIAN_POINT('Ctrl Pts',(38.2571128679763,43.3474571750966,-220.616716070273));
#227352=CARTESIAN_POINT('Ctrl Pts',(40.8950551389346,45.0455299408185,-217.483839750893));
#227353=CARTESIAN_POINT('Ctrl Pts',(43.5337367396124,46.7419641904284,-214.351434639915));
#227354=CARTESIAN_POINT('Ctrl Pts',(27.7033987843753,36.5184180776487,-233.188057587778));
#227355=CARTESIAN_POINT('Ctrl Pts',(28.3494461390117,36.9495031672888,-232.401244113014));
#227356=CARTESIAN_POINT('Ctrl Pts',(28.9972196129455,37.3795877937595,-231.615362013826));
#227357=CARTESIAN_POINT('Ctrl Pts',(29.6459149724228,37.8090935762025,-230.829970164246));
#227358=CARTESIAN_POINT('Ctrl Pts',(30.2946103319002,38.2385993586454,-230.044578314665));
#227359=CARTESIAN_POINT('Ctrl Pts',(30.944252415395,38.6675143670179,-229.259690921114));
#227360=CARTESIAN_POINT('Ctrl Pts',(31.5944542499059,39.0960490201859,-228.475099818776));
#227361=CARTESIAN_POINT('Ctrl Pts',(32.8948579189276,39.9531183265218,-226.905917614101));
#227362=CARTESIAN_POINT('Ctrl Pts',(34.1974465074261,40.8086969168544,-225.337892124046));
#227363=CARTESIAN_POINT('Ctrl Pts',(35.5009303646614,41.6635101961778,-223.770343407667));
#227364=CARTESIAN_POINT('Ctrl Pts',(38.1078980791321,43.3731367548243,-220.635245974907));
#227365=CARTESIAN_POINT('Ctrl Pts',(40.7184182146441,45.0797275518329,-217.502045328114));
#227366=CARTESIAN_POINT('Ctrl Pts',(43.329743245898,46.7848839191427,-214.369334331916));
#227367=CARTESIAN_POINT('Ctrl Pts',(27.6544884050101,36.5134544997187,-233.208489782041));
#227368=CARTESIAN_POINT('Ctrl Pts',(28.2958883125488,36.9453045586868,-232.422071262426));
#227369=CARTESIAN_POINT('Ctrl Pts',(28.9385402233851,37.3764580517972,-231.636337934604));
#227370=CARTESIAN_POINT('Ctrl Pts',(29.5819207190053,37.8071775310161,-230.850998973988));
#227371=CARTESIAN_POINT('Ctrl Pts',(30.2253012146256,38.2378970102351,-230.065660013372));
#227372=CARTESIAN_POINT('Ctrl Pts',(30.8694237090864,38.6681763110842,-229.280723186985));
#227373=CARTESIAN_POINT('Ctrl Pts',(31.5140148312165,39.0981569518477,-228.496039104459));
#227374=CARTESIAN_POINT('Ctrl Pts',(32.8031970754766,39.9581182333748,-226.926670939409));
#227375=CARTESIAN_POINT('Ctrl Pts',(34.094212486763,40.8169068877022,-225.358291458816));
#227376=CARTESIAN_POINT('Ctrl Pts',(35.3860663228485,41.675053386644,-223.79036645522));
#227377=CARTESIAN_POINT('Ctrl Pts',(37.9697739950195,43.3913463845276,-220.654516448028));
#227378=CARTESIAN_POINT('Ctrl Pts',(40.5567806505099,45.1051056979372,-217.520458021817));
#227379=CARTESIAN_POINT('Ctrl Pts',(43.1447063347815,46.8176414904025,-214.386944837765));
#227380=CARTESIAN_POINT('Ctrl Pts',(27.6055780256448,36.5084909217888,-233.228921976304));
#227381=CARTESIAN_POINT('Ctrl Pts',(28.2423304860859,36.9411059500847,-232.442898411838));
#227382=CARTESIAN_POINT('Ctrl Pts',(28.8798608338247,37.3733283098348,-231.657313855381));
#227383=CARTESIAN_POINT('Ctrl Pts',(29.5179264655878,37.8052614858298,-230.87202778373));
#227384=CARTESIAN_POINT('Ctrl Pts',(30.1559920973509,38.2371946618249,-230.08674171208));
#227385=CARTESIAN_POINT('Ctrl Pts',(30.7945950027779,38.6688382551504,-229.301755452856));
#227386=CARTESIAN_POINT('Ctrl Pts',(31.433575412527,39.1002648835096,-228.516978390142));
#227387=CARTESIAN_POINT('Ctrl Pts',(32.7115362320255,39.9631181402278,-226.947424264716));
#227388=CARTESIAN_POINT('Ctrl Pts',(33.9909784660999,40.82511685855,-225.378690793586));
#227389=CARTESIAN_POINT('Ctrl Pts',(35.2712022810355,41.6865965771103,-223.810389502773));
#227390=CARTESIAN_POINT('Ctrl Pts',(37.8316499109069,43.4095560142309,-220.673786921149));
#227391=CARTESIAN_POINT('Ctrl Pts',(40.3951430863757,45.1304838440415,-217.53887071552));
#227392=CARTESIAN_POINT('Ctrl Pts',(42.9596694236649,46.8503990616624,-214.404555343614));
#227393=CARTESIAN_POINT('Ctrl Pts',(27.5495579756445,36.5028921654741,-233.251051919951));
#227394=CARTESIAN_POINT('Ctrl Pts',(28.1827688115622,36.9359521258547,-232.465366213753));
#227395=CARTESIAN_POINT('Ctrl Pts',(28.8164085091962,37.3688162618127,-231.679931708896));
#227396=CARTESIAN_POINT('Ctrl Pts',(29.45037829501,37.8015234896747,-230.894689344989));
#227397=CARTESIAN_POINT('Ctrl Pts',(30.0843480808238,38.2342307175367,-230.109446981082));
#227398=CARTESIAN_POINT('Ctrl Pts',(30.7186486771531,38.6667807943463,-229.324397213218));
#227399=CARTESIAN_POINT('Ctrl Pts',(31.3532086585038,39.0992026045944,-228.539497756859));
#227400=CARTESIAN_POINT('Ctrl Pts',(32.6223286212052,39.9640462250905,-226.96969884414));
#227401=CARTESIAN_POINT('Ctrl Pts',(33.8924746608402,40.828381296436,-225.400494315711));
#227402=CARTESIAN_POINT('Ctrl Pts',(35.1632781294504,41.6923616886714,-223.831668727949));
#227403=CARTESIAN_POINT('Ctrl Pts',(37.7048850666709,43.4203224731419,-220.694017552425));
#227404=CARTESIAN_POINT('Ctrl Pts',(40.2490633538194,45.1468896454712,-217.55784834607));
#227405=CARTESIAN_POINT('Ctrl Pts',(42.7944274621604,46.8726693939935,-214.42236887553));
#227406=CARTESIAN_POINT('Ctrl Pts',(27.4675166955088,36.501209334595,-233.2699618027));
#227407=CARTESIAN_POINT('Ctrl Pts',(28.0986597880893,36.9344896240505,-232.484645254214));
#227408=CARTESIAN_POINT('Ctrl Pts',(28.7300030462673,37.3676977230337,-231.69945191414));
#227409=CARTESIAN_POINT('Ctrl Pts',(29.3615087464634,37.8008474937043,-230.914358703846));
#227410=CARTESIAN_POINT('Ctrl Pts',(29.9930144466596,38.2339972643749,-230.129265493552));
#227411=CARTESIAN_POINT('Ctrl Pts',(30.624682800611,38.6670886387032,-229.344272547955));
#227412=CARTESIAN_POINT('Ctrl Pts',(31.2564852375126,39.1001323034766,-228.559362491382));
#227413=CARTESIAN_POINT('Ctrl Pts',(32.5200901113159,39.9662196330235,-226.989542378236));
#227414=CARTESIAN_POINT('Ctrl Pts',(33.7842270188127,40.8321176985828,-225.420051188828));
#227415=CARTESIAN_POINT('Ctrl Pts',(35.0487393284727,41.6978863030865,-223.850794334856));
#227416=CARTESIAN_POINT('Ctrl Pts',(37.5777639477929,43.429423512094,-220.712280626913));
#227417=CARTESIAN_POINT('Ctrl Pts',(40.1082645173074,45.1604528702306,-217.574688874121));
#227418=CARTESIAN_POINT('Ctrl Pts',(42.6395909737856,46.8912293280373,-214.437630225606));
#227419=CARTESIAN_POINT('',(27.8050196335447,36.7328855798153,-232.850049995496));
#227420=CARTESIAN_POINT('',(28.9186324328831,36.3202559616763,-232.850049990517));
#227421=CARTESIAN_POINT('Ctrl Pts',(27.8050196334018,36.7328855787358,-232.85005));
#227422=CARTESIAN_POINT('Ctrl Pts',(27.8957217939294,36.7208730140292,-232.85005));
#227423=CARTESIAN_POINT('Ctrl Pts',(27.9536434306237,36.7103454425016,-232.850049999997));
#227424=CARTESIAN_POINT('Ctrl Pts',(28.0509870287882,36.6868458484317,-232.850049999997));
#227425=CARTESIAN_POINT('Ctrl Pts',(28.0803209311281,36.6793979170128,-232.850049999947));
#227426=CARTESIAN_POINT('Ctrl Pts',(28.1944269137096,36.649053901996,-232.850049999947));
#227427=CARTESIAN_POINT('Ctrl Pts',(28.2694640302114,36.6259313942996,-232.850050000001));
#227428=CARTESIAN_POINT('Ctrl Pts',(28.4201368589766,36.5675330811538,-232.850050000001));
#227429=CARTESIAN_POINT('Ctrl Pts',(28.4595308694401,36.5515483381828,-232.850050000008));
#227430=CARTESIAN_POINT('Ctrl Pts',(28.5248449659433,36.5234632061754,-232.850050000008));
#227431=CARTESIAN_POINT('Ctrl Pts',(28.5526105252556,36.5109406727164,-232.85005));
#227432=CARTESIAN_POINT('Ctrl Pts',(28.6047252501233,36.4866036083131,-232.85005));
#227433=CARTESIAN_POINT('Ctrl Pts',(28.6308279330002,36.4740323136216,-232.85005));
#227434=CARTESIAN_POINT('Ctrl Pts',(28.6952211500754,36.442440071217,-232.85005));
#227435=CARTESIAN_POINT('Ctrl Pts',(28.7462884613452,36.4168028902437,-232.850050000002));
#227436=CARTESIAN_POINT('Ctrl Pts',(28.7999670577683,36.3884950980527,-232.850050000002));
#227437=CARTESIAN_POINT('Ctrl Pts',(28.8178719483369,36.3786725027028,-232.85005));
#227438=CARTESIAN_POINT('Ctrl Pts',(28.8625139388136,36.353549720413,-232.85005));
#227439=CARTESIAN_POINT('Ctrl Pts',(28.8919158089781,36.3362438515589,-232.85005));
#227440=CARTESIAN_POINT('Ctrl Pts',(28.9186324246664,36.3202560005055,-232.85005));
#227441=CARTESIAN_POINT('',(46.6391379812522,45.1301057287331,-214.324193081127));
#227442=CARTESIAN_POINT('Ctrl Pts',(28.9186324530669,36.3202559475719,-232.850049971551));
#227443=CARTESIAN_POINT('Ctrl Pts',(30.3889628274848,37.0479740123936,-231.318454284006));
#227444=CARTESIAN_POINT('Ctrl Pts',(31.8584196044282,37.7756558134426,-229.786568839607));
#227445=CARTESIAN_POINT('Ctrl Pts',(33.3268737332982,38.5035276796851,-228.254395210835));
#227446=CARTESIAN_POINT('Ctrl Pts',(34.8098341713358,39.2385899198853,-226.707085811785));
#227447=CARTESIAN_POINT('Ctrl Pts',(36.2917724634469,39.9738456977312,-225.159482536368));
#227448=CARTESIAN_POINT('Ctrl Pts',(37.7725665108881,40.7095346352291,-223.61157467501));
#227449=CARTESIAN_POINT('Ctrl Pts',(37.793700233912,40.7200343034737,-223.589483111322));
#227450=CARTESIAN_POINT('Ctrl Pts',(37.8148337232645,40.7305340582079,-223.567391484236));
#227451=CARTESIAN_POINT('Ctrl Pts',(37.8359669785468,40.7410339005308,-223.54529979386));
#227452=CARTESIAN_POINT('Ctrl Pts',(40.7752670935121,42.2013951811095,-220.472696581748));
#227453=CARTESIAN_POINT('Ctrl Pts',(43.710029434473,43.6634416063072,-217.398883050629));
#227454=CARTESIAN_POINT('Ctrl Pts',(46.6391379662423,45.1301057056288,-214.324193130075));
#227455=CARTESIAN_POINT('',(42.9717852817483,46.7498147039571,-214.534096350323));
#227456=CARTESIAN_POINT('Ctrl Pts',(42.9717852817571,46.749814703953,-214.534096350459));
#227457=CARTESIAN_POINT('Ctrl Pts',(43.0986721931634,46.725774799666,-214.525192835447));
#227458=CARTESIAN_POINT('Ctrl Pts',(43.2250603487411,46.6989506892725,-214.516517597904));
#227459=CARTESIAN_POINT('Ctrl Pts',(43.4873979542363,46.637223499967,-214.499052367716));
#227460=CARTESIAN_POINT('Ctrl Pts',(43.623673328713,46.6017076161697,-214.490110644586));
#227461=CARTESIAN_POINT('Ctrl Pts',(43.8528808070891,46.5361367088664,-214.475014174639));
#227462=CARTESIAN_POINT('Ctrl Pts',(43.9471502952977,46.5074540597886,-214.468951067943));
#227463=CARTESIAN_POINT('Ctrl Pts',(44.1657362377398,46.4369225436547,-214.455376470192));
#227464=CARTESIAN_POINT('Ctrl Pts',(44.289571969337,46.3939046796098,-214.447959352174));
#227465=CARTESIAN_POINT('Ctrl Pts',(44.5758870687418,46.2872516657367,-214.430838622362));
#227466=CARTESIAN_POINT('Ctrl Pts',(44.7376694321899,46.2214844640658,-214.421105848154));
#227467=CARTESIAN_POINT('Ctrl Pts',(44.9968192003615,46.1070741799036,-214.406088225855));
#227468=CARTESIAN_POINT('Ctrl Pts',(45.0953309344668,46.0613945558291,-214.400545485095));
#227469=CARTESIAN_POINT('Ctrl Pts',(45.358658729469,45.9333375459576,-214.386175771069));
#227470=CARTESIAN_POINT('Ctrl Pts',(45.5225973319306,45.8471698157457,-214.377106636997));
#227471=CARTESIAN_POINT('Ctrl Pts',(45.7910067954592,45.6952312414373,-214.362880563453));
#227472=CARTESIAN_POINT('Ctrl Pts',(45.8980961664271,45.6315653232451,-214.357676228462));
#227473=CARTESIAN_POINT('Ctrl Pts',(46.0677903918145,45.5257929939876,-214.349632079145));
#227474=CARTESIAN_POINT('Ctrl Pts',(46.1316130052832,45.4848666362459,-214.346627166679));
#227475=CARTESIAN_POINT('Ctrl Pts',(46.2762133611491,45.3894937682619,-214.339569954194));
#227476=CARTESIAN_POINT('Ctrl Pts',(46.3575523973275,45.3339263995932,-214.335548815045));
#227477=CARTESIAN_POINT('Ctrl Pts',(46.5062346419673,45.2285595755895,-214.329247262279));
#227478=CARTESIAN_POINT('Ctrl Pts',(46.5731746847777,45.1796922524229,-214.326639483788));
#227479=CARTESIAN_POINT('Ctrl Pts',(46.6391379874981,45.1301057436029,-214.324192948146));
#227480=CARTESIAN_POINT('',(42.5495440915934,46.8296601108864,-214.549225395662));
#227481=CARTESIAN_POINT('Ctrl Pts',(42.9717852817571,46.7498147039531,-214.534096350459));
#227482=CARTESIAN_POINT('Ctrl Pts',(42.9007618486797,46.7632707532202,-214.539079986663));
#227483=CARTESIAN_POINT('Ctrl Pts',(42.8299856383427,46.7766655446186,-214.542913387513));
#227484=CARTESIAN_POINT('Ctrl Pts',(42.6887342414797,46.8033747711886,-214.547975651047));
#227485=CARTESIAN_POINT('Ctrl Pts',(42.6197623734487,46.8164057424326,-214.549201731095));
#227486=CARTESIAN_POINT('Ctrl Pts',(42.5495441334904,46.8296600955011,-214.549225427215));
#227487=CARTESIAN_POINT('Ctrl Pts',(27.805019639331,36.7328855899921,-232.85005));
#227488=CARTESIAN_POINT('Ctrl Pts',(32.7122624052548,40.1011588208396,-226.745065671994));
#227489=CARTESIAN_POINT('Ctrl Pts',(37.6297308332976,43.4657453232396,-220.646376054327));
#227490=CARTESIAN_POINT('Ctrl Pts',(42.5495441536942,46.8296600915864,-214.549225432877));
#227491=CARTESIAN_POINT('Ctrl Pts',(47.3114554705886,16.8460380888807,-233.260539515782));
#227492=CARTESIAN_POINT('Ctrl Pts',(48.3395590816568,17.8367146054412,-231.692947455239));
#227493=CARTESIAN_POINT('Ctrl Pts',(49.3676726219367,18.8273604593628,-230.125342611939));
#227494=CARTESIAN_POINT('Ctrl Pts',(50.3957927612346,19.8179857984423,-228.557729212486));
#227495=CARTESIAN_POINT('Ctrl Pts',(51.4239129005325,20.8086111375217,-226.990115813032));
#227496=CARTESIAN_POINT('Ctrl Pts',(52.4520396931497,21.7992157970736,-225.422493789));
#227497=CARTESIAN_POINT('Ctrl Pts',(53.480171119088,22.7898059407486,-223.854865709355));
#227498=CARTESIAN_POINT('Ctrl Pts',(55.5364339709647,24.7709862280985,-220.719609550066));
#227499=CARTESIAN_POINT('Ctrl Pts',(57.5927150219887,26.7521094718628,-217.584329593504));
#227500=CARTESIAN_POINT('Ctrl Pts',(59.6490056999632,28.7332018665566,-214.449036765473));
#227501=CARTESIAN_POINT('Ctrl Pts',(47.3110520982437,16.8559465263517,-233.26053824229));
#227502=CARTESIAN_POINT('Ctrl Pts',(48.3391380137511,17.8470909658639,-231.692946212383));
#227503=CARTESIAN_POINT('Ctrl Pts',(49.3672339116285,18.8382047449221,-230.125341393407));
#227504=CARTESIAN_POINT('Ctrl Pts',(50.3953364602535,19.82929801124,-228.55772801405));
#227505=CARTESIAN_POINT('Ctrl Pts',(51.4234390088786,20.8203912775578,-226.990114634692));
#227506=CARTESIAN_POINT('Ctrl Pts',(52.4515482625761,21.8114638664511,-225.422492626496));
#227507=CARTESIAN_POINT('Ctrl Pts',(53.4796622004807,22.8025219415151,-223.854864559695));
#227508=CARTESIAN_POINT('Ctrl Pts',(55.5358900762899,24.7846380916432,-220.719608426093));
#227509=CARTESIAN_POINT('Ctrl Pts',(57.5921363546469,26.7666972063695,-217.58432848346));
#227510=CARTESIAN_POINT('Ctrl Pts',(59.6483924596735,28.7487254799229,-214.449035662994));
#227511=CARTESIAN_POINT('Ctrl Pts',(47.3103397682614,16.8668521773429,-233.260936805424));
#227512=CARTESIAN_POINT('Ctrl Pts',(48.3384173520821,17.8584323054149,-231.693333771247));
#227513=CARTESIAN_POINT('Ctrl Pts',(49.3665034987094,18.8499861389194,-230.125719739421));
#227514=CARTESIAN_POINT('Ctrl Pts',(50.3945954284579,19.8415221922535,-228.558098269208));
#227515=CARTESIAN_POINT('Ctrl Pts',(51.4226873582065,20.8330582455877,-226.990476798996));
#227516=CARTESIAN_POINT('Ctrl Pts',(52.4507851140727,21.8245763873091,-225.422847835511));
#227517=CARTESIAN_POINT('Ctrl Pts',(53.4788869862349,22.8160818579234,-223.855213570177));
#227518=CARTESIAN_POINT('Ctrl Pts',(55.5350907305594,24.7990927991518,-220.719945039509));
#227519=CARTESIAN_POINT('Ctrl Pts',(57.5913106558967,26.7820539269176,-217.584655665656));
#227520=CARTESIAN_POINT('Ctrl Pts',(59.6475394024948,28.7649878151953,-214.449354892196));
#227521=CARTESIAN_POINT('Ctrl Pts',(47.3110535174895,16.873256830116,-233.259496526039));
#227522=CARTESIAN_POINT('Ctrl Pts',(48.3390812029547,17.8654084135782,-231.691932847844));
#227523=CARTESIAN_POINT('Ctrl Pts',(49.3671224159146,18.8575190179354,-230.124352092621));
#227524=CARTESIAN_POINT('Ctrl Pts',(50.3951725945636,19.8496024611769,-228.556760010403));
#227525=CARTESIAN_POINT('Ctrl Pts',(51.4232227732125,20.8416859044184,-226.989167928185));
#227526=CARTESIAN_POINT('Ctrl Pts',(52.4512819949066,21.8337419536198,-225.421564422348));
#227527=CARTESIAN_POINT('Ctrl Pts',(53.4793475235956,22.8257789108232,-223.853952950714));
#227528=CARTESIAN_POINT('Ctrl Pts',(55.5354785809735,24.8098528252302,-220.718730007446));
#227529=CARTESIAN_POINT('Ctrl Pts',(57.5916344152767,26.7938517410564,-217.583475771517));
#227530=CARTESIAN_POINT('Ctrl Pts',(59.6478035550371,28.7778105309341,-214.448204781494));
#227531=CARTESIAN_POINT('Ctrl Pts',(47.3117672667176,16.8796614828891,-233.258056246654));
#227532=CARTESIAN_POINT('Ctrl Pts',(48.3397450538273,17.8723845217414,-231.690531924442));
#227533=CARTESIAN_POINT('Ctrl Pts',(49.3677413331199,18.8650518969515,-230.122984445821));
#227534=CARTESIAN_POINT('Ctrl Pts',(50.3957497606693,19.8576827301003,-228.555421751598));
#227535=CARTESIAN_POINT('Ctrl Pts',(51.4237581882186,20.8503135632492,-226.987859057374));
#227536=CARTESIAN_POINT('Ctrl Pts',(52.4517788757404,21.8429075199303,-225.420281009185));
#227537=CARTESIAN_POINT('Ctrl Pts',(53.4798080609562,22.835475963723,-223.852692331251));
#227538=CARTESIAN_POINT('Ctrl Pts',(55.5358664313876,24.8206128513086,-220.717514975384));
#227539=CARTESIAN_POINT('Ctrl Pts',(57.5919581746568,26.8056495551953,-217.582295877378));
#227540=CARTESIAN_POINT('Ctrl Pts',(59.6480677075794,28.790633246673,-214.447054670791));
#227541=CARTESIAN_POINT('Ctrl Pts',(47.3124780096108,16.8859145617117,-233.256609308214));
#227542=CARTESIAN_POINT('Ctrl Pts',(48.3404033416989,17.879229404878,-231.689125142628));
#227543=CARTESIAN_POINT('Ctrl Pts',(49.3683527798054,18.8724721952687,-230.121611075758));
#227544=CARTESIAN_POINT('Ctrl Pts',(50.3963178475467,19.8656683126149,-228.554077618338));
#227545=CARTESIAN_POINT('Ctrl Pts',(51.424282915288,20.8588644299609,-226.986544160919));
#227546=CARTESIAN_POINT('Ctrl Pts',(52.4522637695665,21.8520134082152,-225.418991120778));
#227547=CARTESIAN_POINT('Ctrl Pts',(53.480255460339,22.8451301056268,-223.851424659566));
#227548=CARTESIAN_POINT('Ctrl Pts',(55.5362388418842,24.83136350045,-220.716291737142));
#227549=CARTESIAN_POINT('Ctrl Pts',(57.5922647611927,26.8174702004918,-217.581106138124));
#227550=CARTESIAN_POINT('Ctrl Pts',(59.6483130536229,28.8035108935828,-214.4458930656));
#227551=CARTESIAN_POINT('Ctrl Pts',(47.3131850756779,16.8920273532507,-233.255157881008));
#227552=CARTESIAN_POINT('Ctrl Pts',(48.3410552958596,17.8859535740668,-231.68771449894));
#227553=CARTESIAN_POINT('Ctrl Pts',(49.3689559345468,18.8797895866585,-230.120233792132));
#227554=CARTESIAN_POINT('Ctrl Pts',(50.3968759670817,19.8735681235901,-228.552729269786));
#227555=CARTESIAN_POINT('Ctrl Pts',(51.4247959996165,20.8673466605217,-226.98522474744));
#227556=CARTESIAN_POINT('Ctrl Pts',(52.4527356437508,21.8610670819393,-225.417696146955));
#227557=CARTESIAN_POINT('Ctrl Pts',(53.4806885888443,22.8547481865589,-223.850151240679));
#227558=CARTESIAN_POINT('Ctrl Pts',(55.5365944790313,24.8421103957982,-220.715061428126));
#227559=CARTESIAN_POINT('Ctrl Pts',(57.5925525533974,26.8293183807281,-217.579907651647));
#227560=CARTESIAN_POINT('Ctrl Pts',(59.6485376230928,28.8164474339779,-214.444721098757));
#227561=CARTESIAN_POINT('Ctrl Pts',(47.3145992078122,16.9042529363287,-233.252255026597));
#227562=CARTESIAN_POINT('Ctrl Pts',(48.342359204181,17.8994019124442,-231.684893211564));
#227563=CARTESIAN_POINT('Ctrl Pts',(49.3701622440295,18.8944243694381,-230.117479224879));
#227564=CARTESIAN_POINT('Ctrl Pts',(50.3979922061516,19.8893677455407,-228.55003257268));
#227565=CARTESIAN_POINT('Ctrl Pts',(51.4258221682736,20.8843111216433,-226.982585920481));
#227566=CARTESIAN_POINT('Ctrl Pts',(52.4536793921196,21.8791744293876,-225.41510619931));
#227567=CARTESIAN_POINT('Ctrl Pts',(53.4815548458549,22.8739843484231,-223.847604402904));
#227568=CARTESIAN_POINT('Ctrl Pts',(55.5373057533255,24.8636041864943,-220.712600810094));
#227569=CARTESIAN_POINT('Ctrl Pts',(57.5931281378066,26.8530147412008,-217.577510678694));
#227570=CARTESIAN_POINT('Ctrl Pts',(59.6489867620326,28.8423205147682,-214.442377165073));
#227571=CARTESIAN_POINT('Ctrl Pts',(47.3159989701972,16.9159167325326,-233.249334003942));
#227572=CARTESIAN_POINT('Ctrl Pts',(48.3436380292726,17.9123669615539,-231.682056339452));
#227573=CARTESIAN_POINT('Ctrl Pts',(49.3713355823747,18.9086472103352,-230.114708908922));
#227574=CARTESIAN_POINT('Ctrl Pts',(50.3990687332636,19.9048240492912,-228.547318949062));
#227575=CARTESIAN_POINT('Ctrl Pts',(51.4268018841524,20.9010008882471,-226.979928989203));
#227576=CARTESIAN_POINT('Ctrl Pts',(52.45457115623,21.8970728138782,-225.412495889199));
#227577=CARTESIAN_POINT('Ctrl Pts',(53.4823640955953,22.8930761954416,-223.84503456711));
#227578=CARTESIAN_POINT('Ctrl Pts',(55.537949974326,24.8850829585685,-220.710111922933));
#227579=CARTESIAN_POINT('Ctrl Pts',(57.5936285702719,26.8768212639349,-217.575078740198));
#227580=CARTESIAN_POINT('Ctrl Pts',(59.6493528038196,28.8684292299185,-214.439991823286));
#227581=CARTESIAN_POINT('Ctrl Pts',(47.317375174873,16.9271166732568,-233.246414795271));
#227582=CARTESIAN_POINT('Ctrl Pts',(48.3448826696721,17.9249382396269,-231.679221637881));
#227583=CARTESIAN_POINT('Ctrl Pts',(49.3724670545446,18.9225395323645,-230.111938592781));
#227584=CARTESIAN_POINT('Ctrl Pts',(50.4000965635423,19.9200114073275,-228.544602587596));
#227585=CARTESIAN_POINT('Ctrl Pts',(51.42772607254,20.9174832822903,-226.977266582412));
#227586=CARTESIAN_POINT('Ctrl Pts',(52.4554015221151,21.9148234426101,-225.409876692422));
#227587=CARTESIAN_POINT('Ctrl Pts',(53.4831063385788,22.9120795922463,-223.842452376097));
#227588=CARTESIAN_POINT('Ctrl Pts',(55.5385159715063,24.9065918915186,-220.707603743446));
#227589=CARTESIAN_POINT('Ctrl Pts',(57.5940405653775,26.9007754041514,-217.572620374409));
#227590=CARTESIAN_POINT('Ctrl Pts',(59.6496198849772,28.8948045789125,-214.437573677779));
#227591=CARTESIAN_POINT('Ctrl Pts',(47.3201275842246,16.9495165547055,-233.240576377928));
#227592=CARTESIAN_POINT('Ctrl Pts',(48.3473719504709,17.9500807957729,-231.67355223474));
#227593=CARTESIAN_POINT('Ctrl Pts',(49.3747299988842,18.9503241764231,-230.106397960498));
#227594=CARTESIAN_POINT('Ctrl Pts',(50.4021522240997,19.9503861234,-228.539169864665));
#227595=CARTESIAN_POINT('Ctrl Pts',(51.4295744493152,20.9504480703769,-226.97194176883));
#227596=CARTESIAN_POINT('Ctrl Pts',(52.4570622538851,21.9503247000739,-225.40463829887));
#227597=CARTESIAN_POINT('Ctrl Pts',(53.4845908245458,22.9500863858554,-223.837287994071));
#227598=CARTESIAN_POINT('Ctrl Pts',(55.539647965867,24.9496097574185,-220.702587384473));
#227599=CARTESIAN_POINT('Ctrl Pts',(57.5948645555888,26.9486836845843,-217.56770364283));
#227600=CARTESIAN_POINT('Ctrl Pts',(59.6501540472924,28.9475552769007,-214.432737386764));
#227601=CARTESIAN_POINT('Ctrl Pts',(47.3227915814476,16.9700523845408,-233.234742668299));
#227602=CARTESIAN_POINT('Ctrl Pts',(48.3497283291618,17.9736436661242,-231.667890368169));
#227603=CARTESIAN_POINT('Ctrl Pts',(49.3768283745781,18.9767837847294,-230.100856716523));
#227604=CARTESIAN_POINT('Ctrl Pts',(50.4040153385433,19.9796831826563,-228.533725925203));
#227605=CARTESIAN_POINT('Ctrl Pts',(51.4312023025085,20.9825825805833,-226.966595133883));
#227606=CARTESIAN_POINT('Ctrl Pts',(52.4584786467041,21.9852345805636,-225.399364559241));
#227607=CARTESIAN_POINT('Ctrl Pts',(53.4858082893199,22.9877393389703,-223.832074478405));
#227608=CARTESIAN_POINT('Ctrl Pts',(55.5404675745514,24.9927488557837,-220.697494316732));
#227609=CARTESIAN_POINT('Ctrl Pts',(57.5953351427,26.9971831704407,-217.562681699479));
#227610=CARTESIAN_POINT('Ctrl Pts',(59.6502925248986,29.0013735664462,-214.427770494967));
#227611=CARTESIAN_POINT('Ctrl Pts',(47.3252263828413,16.9896223025012,-233.229110072315));
#227612=CARTESIAN_POINT('Ctrl Pts',(48.3518314896857,17.9964142568803,-231.662398987523));
#227613=CARTESIAN_POINT('Ctrl Pts',(49.3786544580299,19.0026193721543,-230.095454289591));
#227614=CARTESIAN_POINT('Ctrl Pts',(50.4055851760868,20.0085325545711,-228.528392739382));
#227615=CARTESIAN_POINT('Ctrl Pts',(51.4325158941438,21.0144457369877,-226.961331189173));
#227616=CARTESIAN_POINT('Ctrl Pts',(52.459558588544,22.0200559113108,-225.394148461867));
#227617=CARTESIAN_POINT('Ctrl Pts',(53.4866652007083,23.0254932317529,-223.826896445521));
#227618=CARTESIAN_POINT('Ctrl Pts',(55.5408784250369,25.0363678726369,-220.692392412828));
#227619=CARTESIAN_POINT('Ctrl Pts',(57.5953414810798,27.046567195329,-217.557617709049));
#227620=CARTESIAN_POINT('Ctrl Pts',(59.6499065909155,29.0564953668167,-214.422734451764));
#227621=CARTESIAN_POINT('Ctrl Pts',(47.3300959856285,17.0287621384219,-233.217844880347));
#227622=CARTESIAN_POINT('Ctrl Pts',(48.3560378107335,18.0419554383925,-231.651416226232));
#227623=CARTESIAN_POINT('Ctrl Pts',(49.3823066249335,19.0542905470043,-230.08464943573));
#227624=CARTESIAN_POINT('Ctrl Pts',(50.4087248511739,20.0662312984004,-228.517726367742));
#227625=CARTESIAN_POINT('Ctrl Pts',(51.4351430774143,21.0781720497965,-226.950803299753));
#227626=CARTESIAN_POINT('Ctrl Pts',(52.4617184722238,22.0896985728052,-225.383716267118));
#227627=CARTESIAN_POINT('Ctrl Pts',(53.4883790234851,23.1010010173179,-223.816540379752));
#227628=CARTESIAN_POINT('Ctrl Pts',(55.5417001260078,25.1236059063434,-220.68218860502));
#227629=CARTESIAN_POINT('Ctrl Pts',(57.5953541578395,27.1453352451054,-217.54748972819));
#227630=CARTESIAN_POINT('Ctrl Pts',(59.6491347229493,29.1667389675576,-214.412662365356));
#227631=CARTESIAN_POINT('Ctrl Pts',(47.3340807471002,17.0640763095221,-233.207405072206));
#227632=CARTESIAN_POINT('Ctrl Pts',(48.3592415226016,18.084391760883,-231.641145159187));
#227633=CARTESIAN_POINT('Ctrl Pts',(49.3848779968831,19.1035202524442,-230.074425303614));
#227634=CARTESIAN_POINT('Ctrl Pts',(50.4106976289339,20.1221883131755,-228.507525821657));
#227635=CARTESIAN_POINT('Ctrl Pts',(51.4365172609848,21.1408563739068,-226.9406263397));
#227636=CARTESIAN_POINT('Ctrl Pts',(52.4625365580142,22.1590237254166,-225.373531896091));
#227637=CARTESIAN_POINT('Ctrl Pts',(53.4886544050993,23.1769445199182,-223.806341423117));
#227638=CARTESIAN_POINT('Ctrl Pts',(55.5408900992694,25.2127861089213,-220.671960477169));
#227639=CARTESIAN_POINT('Ctrl Pts',(57.593512687643,27.2476605248632,-217.537203022514));
#227640=CARTESIAN_POINT('Ctrl Pts',(59.6462671267447,29.2822144774089,-214.402322487616));
#227641=CARTESIAN_POINT('Ctrl Pts',(47.3352334252266,17.1035049830549,-233.199529035477));
#227642=CARTESIAN_POINT('Ctrl Pts',(48.3600042849483,18.1301783396072,-231.632852310436));
#227643=CARTESIAN_POINT('Ctrl Pts',(49.3851454200133,19.1559450105208,-230.065825712809));
#227644=CARTESIAN_POINT('Ctrl Pts',(50.4104205557466,20.1813828669923,-228.498672133956));
#227645=CARTESIAN_POINT('Ctrl Pts',(51.4356956914798,21.2068207234638,-226.931518555102));
#227646=CARTESIAN_POINT('Ctrl Pts',(52.4611193627566,22.2318946684557,-225.364224580397));
#227647=CARTESIAN_POINT('Ctrl Pts',(53.4866146769212,23.2567945291104,-223.79686392097));
#227648=CARTESIAN_POINT('Ctrl Pts',(55.5376053052503,25.3065942504197,-220.662142602115));
#227649=CARTESIAN_POINT('Ctrl Pts',(57.5888779614229,27.3557092766758,-217.527159175984));
#227650=CARTESIAN_POINT('Ctrl Pts',(59.6402468289299,29.4046011172088,-214.392093753442));
#227651=CARTESIAN_POINT('Ctrl Pts',(47.3375387814793,17.1823623301207,-233.18377696202));
#227652=CARTESIAN_POINT('Ctrl Pts',(48.3615298096416,18.2217514970558,-231.616266612933));
#227653=CARTESIAN_POINT('Ctrl Pts',(49.3856802662736,19.2607945266738,-230.048626531198));
#227654=CARTESIAN_POINT('Ctrl Pts',(50.4098664093718,20.299771974626,-228.480964758552));
#227655=CARTESIAN_POINT('Ctrl Pts',(51.43405255247,21.3387494225781,-226.913302985906));
#227656=CARTESIAN_POINT('Ctrl Pts',(52.4582849722416,22.377636554534,-225.34560994901));
#227657=CARTESIAN_POINT('Ctrl Pts',(53.4825352205651,23.4164945474948,-223.777908916675));
#227658=CARTESIAN_POINT('Ctrl Pts',(55.5310357172121,25.4942105334166,-220.642506852006));
#227659=CARTESIAN_POINT('Ctrl Pts',(57.5796085089827,27.5718067803009,-217.507071482923));
#227660=CARTESIAN_POINT('Ctrl Pts',(59.6282062333003,29.6493743968087,-214.371636285096));
#227661=CARTESIAN_POINT('Ctrl Pts',(47.3383263868385,17.2535337845356,-233.16852831652));
#227662=CARTESIAN_POINT('Ctrl Pts',(48.3611580995056,18.3073838091979,-231.599694154632));
#227663=CARTESIAN_POINT('Ctrl Pts',(49.3835577975687,19.3623427162029,-230.031292497904));
#227664=CARTESIAN_POINT('Ctrl Pts',(50.4058155742669,20.4176535575179,-228.463032821567));
#227665=CARTESIAN_POINT('Ctrl Pts',(51.4280733509651,21.4729643988329,-226.894773145231));
#227666=CARTESIAN_POINT('Ctrl Pts',(52.4501722979439,22.5286737057843,-225.326672671531));
#227667=CARTESIAN_POINT('Ctrl Pts',(53.472204800048,23.5845483661524,-223.75864059823));
#227668=CARTESIAN_POINT('Ctrl Pts',(55.5162698042562,25.6962976868884,-220.622576451631));
#227669=CARTESIAN_POINT('Ctrl Pts',(57.5600729846415,27.8087001526143,-217.486782588132));
#227670=CARTESIAN_POINT('Ctrl Pts',(59.6038198261226,29.9212462142014,-214.351060388696));
#227671=CARTESIAN_POINT('Ctrl Pts',(47.3388947489722,17.3172597414177,-233.15277350217));
#227672=CARTESIAN_POINT('Ctrl Pts',(48.3602977670814,18.3855423142397,-231.582083581833));
#227673=CARTESIAN_POINT('Ctrl Pts',(49.3799313248768,19.4576103826212,-230.012850342708));
#227674=CARTESIAN_POINT('Ctrl Pts',(50.3991818891466,20.5304657339301,-228.443915670914));
#227675=CARTESIAN_POINT('Ctrl Pts',(51.4184324534164,21.6033210852391,-226.874980999121));
#227676=CARTESIAN_POINT('Ctrl Pts',(52.4371748506907,22.6772399564986,-225.306453273624));
#227677=CARTESIAN_POINT('Ctrl Pts',(53.4557277384216,23.7515480681017,-223.738076580824));
#227678=CARTESIAN_POINT('Ctrl Pts',(55.4928335138835,25.9001642913079,-220.601323195224));
#227679=CARTESIAN_POINT('Ctrl Pts',(57.529175347697,28.050353188994,-217.465180895102));
#227680=CARTESIAN_POINT('Ctrl Pts',(59.5653551090103,30.2008561303528,-214.329177297802));
#227681=CARTESIAN_POINT('Ctrl Pts',(47.3394631111059,17.3809856982998,-233.13701868782));
#227682=CARTESIAN_POINT('Ctrl Pts',(48.3594374346572,18.4637008192816,-231.564473009033));
#227683=CARTESIAN_POINT('Ctrl Pts',(49.3763048521849,19.5528780490395,-229.994408187512));
#227684=CARTESIAN_POINT('Ctrl Pts',(50.3925482040264,20.6432779103424,-228.424798520261));
#227685=CARTESIAN_POINT('Ctrl Pts',(51.4087915558678,21.7336777716453,-226.85518885301));
#227686=CARTESIAN_POINT('Ctrl Pts',(52.4241774034375,22.8258062072129,-225.286233875719));
#227687=CARTESIAN_POINT('Ctrl Pts',(53.4392506767952,23.9185477700511,-223.717512563418));
#227688=CARTESIAN_POINT('Ctrl Pts',(55.4693972235108,26.1040308957274,-220.580069938817));
#227689=CARTESIAN_POINT('Ctrl Pts',(57.4982777107523,28.2920062253737,-217.443579202073));
#227690=CARTESIAN_POINT('Ctrl Pts',(59.526890391898,30.4804660465043,-214.307294206909));
#227691=CARTESIAN_POINT('Ctrl Pts',(47.3366602074855,17.444170151716,-233.123362358707));
#227692=CARTESIAN_POINT('Ctrl Pts',(48.3540763070954,18.5429695999985,-231.549048499502));
#227693=CARTESIAN_POINT('Ctrl Pts',(49.3667036858826,19.6512330207133,-229.97834790794));
#227694=CARTESIAN_POINT('Ctrl Pts',(50.378495909681,20.7610182295588,-228.40819979349));
#227695=CARTESIAN_POINT('Ctrl Pts',(51.3902881334795,21.8708034384043,-226.83805167904));
#227696=CARTESIAN_POINT('Ctrl Pts',(52.4008473220208,22.9829339492799,-225.268781019355));
#227697=CARTESIAN_POINT('Ctrl Pts',(53.4109754339125,24.0958567445521,-223.699807621397));
#227698=CARTESIAN_POINT('Ctrl Pts',(55.4312316576958,26.3217023350964,-220.561860825481));
#227699=CARTESIAN_POINT('Ctrl Pts',(57.4497270949821,28.5507997267972,-217.425137866697));
#227700=CARTESIAN_POINT('Ctrl Pts',(59.4678639415957,30.7804881980906,-214.288663699106));
#227701=CARTESIAN_POINT('Ctrl Pts',(47.3285982419782,17.5118110061916,-233.112766042078));
#227702=CARTESIAN_POINT('Ctrl Pts',(48.3441007183216,18.6236888893903,-231.535741196264));
#227703=CARTESIAN_POINT('Ctrl Pts',(49.3524346981868,19.7490902161012,-229.963964803722));
#227704=CARTESIAN_POINT('Ctrl Pts',(50.3595015772335,20.8765891331594,-228.392921090687));
#227705=CARTESIAN_POINT('Ctrl Pts',(51.3665684562802,22.0040880502176,-226.821877377652));
#227706=CARTESIAN_POINT('Ctrl Pts',(52.3717783622527,23.1348854144855,-225.252060380076));
#227707=CARTESIAN_POINT('Ctrl Pts',(53.3763360684624,24.2667864286898,-223.682648344784));
#227708=CARTESIAN_POINT('Ctrl Pts',(55.3854514808819,26.5305884570984,-220.5438242742));
#227709=CARTESIAN_POINT('Ctrl Pts',(57.3919042457265,28.7989304812669,-217.40667659104));
#227710=CARTESIAN_POINT('Ctrl Pts',(59.397804330835,31.0680944254412,-214.269858953779));
#227711=CARTESIAN_POINT('Ctrl Pts',(47.3205362764709,17.5794518606674,-233.102169725448));
#227712=CARTESIAN_POINT('Ctrl Pts',(48.3341251295478,18.7044081787822,-231.522433893026));
#227713=CARTESIAN_POINT('Ctrl Pts',(49.338165710491,19.8469474114891,-229.949581699504));
#227714=CARTESIAN_POINT('Ctrl Pts',(50.3405072447859,20.99216003676,-228.377642387885));
#227715=CARTESIAN_POINT('Ctrl Pts',(51.3428487790808,22.1373726620309,-226.805703076266));
#227716=CARTESIAN_POINT('Ctrl Pts',(52.3427094024845,23.2868368796911,-225.235339740797));
#227717=CARTESIAN_POINT('Ctrl Pts',(53.3416967030123,24.4377161128276,-223.665489068171));
#227718=CARTESIAN_POINT('Ctrl Pts',(55.3396713040681,26.7394745791004,-220.525787722919));
#227719=CARTESIAN_POINT('Ctrl Pts',(57.334081396471,29.0470612357366,-217.388215315384));
#227720=CARTESIAN_POINT('Ctrl Pts',(59.3277447200742,31.3557006527919,-214.251054208451));
#227721=CARTESIAN_POINT('Ctrl Pts',(47.3141359442706,17.638980093523,-233.090010378228));
#227722=CARTESIAN_POINT('Ctrl Pts',(48.32443367589,18.7780728965381,-231.50825504547));
#227723=CARTESIAN_POINT('Ctrl Pts',(49.3229723535216,19.9379411976756,-229.93469251917));
#227724=CARTESIAN_POINT('Ctrl Pts',(50.3194004745391,21.1008963306773,-228.36214789025));
#227725=CARTESIAN_POINT('Ctrl Pts',(51.3158285955566,22.2638514636789,-226.78960326133));
#227726=CARTESIAN_POINT('Ctrl Pts',(52.3091900605982,23.4317796609776,-225.218887494463));
#227727=CARTESIAN_POINT('Ctrl Pts',(53.3014701549735,24.6013499668753,-223.648755791418));
#227728=CARTESIAN_POINT('Ctrl Pts',(55.2860303437241,26.9404905786706,-220.508492385326));
#227729=CARTESIAN_POINT('Ctrl Pts',(57.2661781231904,29.2864048695037,-217.370664238171));
#227730=CARTESIAN_POINT('Ctrl Pts',(59.2453960697349,31.6335238048983,-214.233295308244));
#227731=CARTESIAN_POINT('Ctrl Pts',(47.3068095033878,17.6967086574683,-233.077497779098));
#227732=CARTESIAN_POINT('Ctrl Pts',(48.3116549954781,18.8520796703188,-231.494638672248));
#227733=CARTESIAN_POINT('Ctrl Pts',(49.3030451918381,20.0301039514678,-229.920713549775));
#227734=CARTESIAN_POINT('Ctrl Pts',(50.2920112564435,21.2114530404761,-228.347855989514));
#227735=CARTESIAN_POINT('Ctrl Pts',(51.280977321049,22.3928021294844,-226.774998429254));
#227736=CARTESIAN_POINT('Ctrl Pts',(52.2664287923936,23.5795439345552,-225.204106117501));
#227737=CARTESIAN_POINT('Ctrl Pts',(53.2506399867227,24.7680561731562,-223.633834433041));
#227738=CARTESIAN_POINT('Ctrl Pts',(55.2190623753812,27.1450806503585,-220.493291064124));
#227739=CARTESIAN_POINT('Ctrl Pts',(57.1824244494106,29.5294142243635,-217.355341819955));
#227740=CARTESIAN_POINT('Ctrl Pts',(59.1447159484551,31.9150218118753,-214.217874373197));
#227741=CARTESIAN_POINT('Ctrl Pts',(47.2994830625051,17.7544372214138,-233.064985179967));
#227742=CARTESIAN_POINT('Ctrl Pts',(48.2988763150662,18.9260864440995,-231.481022299027));
#227743=CARTESIAN_POINT('Ctrl Pts',(49.2831180301545,20.12226670526,-229.90673458038));
#227744=CARTESIAN_POINT('Ctrl Pts',(50.264622038348,21.3220097502749,-228.333564088779));
#227745=CARTESIAN_POINT('Ctrl Pts',(51.2461260465415,22.5217527952899,-226.760393597177));
#227746=CARTESIAN_POINT('Ctrl Pts',(52.2236675241889,23.7273082081328,-225.189324740538));
#227747=CARTESIAN_POINT('Ctrl Pts',(53.199809818472,24.9347623794372,-223.618913074665));
#227748=CARTESIAN_POINT('Ctrl Pts',(55.1520944070382,27.3496707220463,-220.478089742921));
#227749=CARTESIAN_POINT('Ctrl Pts',(57.0986707756308,29.7724235792233,-217.34001940174));
#227750=CARTESIAN_POINT('Ctrl Pts',(59.0440358271753,32.1965198188522,-214.20245343815));
#227751=CARTESIAN_POINT('Ctrl Pts',(47.2842338109509,17.8211612809678,-233.056043673691));
#227752=CARTESIAN_POINT('Ctrl Pts',(48.2782304069827,19.0073087386684,-231.47028620506));
#227753=CARTESIAN_POINT('Ctrl Pts',(49.2548742655618,20.2206444917306,-229.89534347711));
#227754=CARTESIAN_POINT('Ctrl Pts',(50.2283116608323,21.437958506772,-228.321621606276));
#227755=CARTESIAN_POINT('Ctrl Pts',(51.2017490561027,22.6552725218134,-226.747899735443));
#227756=CARTESIAN_POINT('Ctrl Pts',(52.1706012443748,23.8790456722595,-225.176507139922));
#227757=CARTESIAN_POINT('Ctrl Pts',(53.1378257718042,25.1049289791612,-223.60583742058));
#227758=CARTESIAN_POINT('Ctrl Pts',(55.072274826663,27.5566955929646,-220.464497981896));
#227759=CARTESIAN_POINT('Ctrl Pts',(57.0000906545182,30.0171778123751,-217.326191699464));
#227760=CARTESIAN_POINT('Ctrl Pts',(58.9264876034895,32.47914368792,-214.188435032943));
#227761=CARTESIAN_POINT('Ctrl Pts',(47.2636279462708,17.8918194961353,-233.049292072559));
#227762=CARTESIAN_POINT('Ctrl Pts',(48.2527927601426,19.0896993463335,-231.461117845357));
#227763=CARTESIAN_POINT('Ctrl Pts',(49.2222701184903,20.3177090530585,-229.885189443365));
#227764=CARTESIAN_POINT('Ctrl Pts',(50.1877928495361,21.5503879875109,-228.310673435979));
#227765=CARTESIAN_POINT('Ctrl Pts',(51.1533155805818,22.7830669219633,-226.736157428594));
#227766=CARTESIAN_POINT('Ctrl Pts',(52.1134152350247,24.0230769225979,-225.164293315049));
#227767=CARTESIAN_POINT('Ctrl Pts',(53.0715402305708,25.265515738592,-223.593249605752));
#227768=CARTESIAN_POINT('Ctrl Pts',(54.9877902216631,27.75039337058,-220.451162187155));
#227769=CARTESIAN_POINT('Ctrl Pts',(56.8960314270369,30.2452705785478,-217.312517061756));
#227770=CARTESIAN_POINT('Ctrl Pts',(58.8025041724956,32.7418818204746,-214.174488273677));
#227771=CARTESIAN_POINT('Ctrl Pts',(47.2430220815907,17.9624777113029,-233.042540471425));
#227772=CARTESIAN_POINT('Ctrl Pts',(48.2273551133025,19.1720899539984,-231.451949485653));
#227773=CARTESIAN_POINT('Ctrl Pts',(49.1896659714189,20.4147736143863,-229.87503540962));
#227774=CARTESIAN_POINT('Ctrl Pts',(50.1472740382399,21.6628174682499,-228.299725265682));
#227775=CARTESIAN_POINT('Ctrl Pts',(51.1048821050609,22.9108613221134,-226.724415121745));
#227776=CARTESIAN_POINT('Ctrl Pts',(52.0562292256746,24.1671081729364,-225.152079490178));
#227777=CARTESIAN_POINT('Ctrl Pts',(53.0052546893374,25.4261024980228,-223.580661790924));
#227778=CARTESIAN_POINT('Ctrl Pts',(54.9033056166631,27.9440911481955,-220.437826392414));
#227779=CARTESIAN_POINT('Ctrl Pts',(56.7919721995556,30.4733633447205,-217.298842424047));
#227780=CARTESIAN_POINT('Ctrl Pts',(58.6785207415017,33.0046199530293,-214.16054151441));
#227781=CARTESIAN_POINT('Ctrl Pts',(47.2289637142144,18.0209926675766,-233.031939311332));
#227782=CARTESIAN_POINT('Ctrl Pts',(48.1993754505405,19.2535954323428,-231.443888976038));
#227783=CARTESIAN_POINT('Ctrl Pts',(49.1516972038829,20.512132417265,-229.866635744028));
#227784=CARTESIAN_POINT('Ctrl Pts',(50.0988311928047,21.7766727071225,-228.291351005029));
#227785=CARTESIAN_POINT('Ctrl Pts',(51.0459651817265,23.0412129969801,-226.716066266029));
#227786=CARTESIAN_POINT('Ctrl Pts',(51.9869923629565,24.3134260425889,-225.14358686793));
#227787=CARTESIAN_POINT('Ctrl Pts',(52.9255304548883,25.5884625672894,-223.572054708453));
#227788=CARTESIAN_POINT('Ctrl Pts',(54.802606638752,28.1385356166903,-220.4289903895));
#227789=CARTESIAN_POINT('Ctrl Pts',(56.6697948095651,30.6999604033981,-217.289804946001));
#227790=CARTESIAN_POINT('Ctrl Pts',(58.5345519359632,33.2635581737269,-214.151359869686));
#227791=CARTESIAN_POINT('Ctrl Pts',(47.2098674957262,18.0858618424364,-233.021306146667));
#227792=CARTESIAN_POINT('Ctrl Pts',(48.1660577345037,19.3384804806313,-231.436445859109));
#227793=CARTESIAN_POINT('Ctrl Pts',(49.1090703108757,20.6096704873925,-229.859386110464));
#227794=CARTESIAN_POINT('Ctrl Pts',(50.0473336065433,21.8864233995054,-228.284270940977));
#227795=CARTESIAN_POINT('Ctrl Pts',(50.9855969022109,23.1631763116183,-226.709155771488));
#227796=CARTESIAN_POINT('Ctrl Pts',(51.9186177626333,24.4464108695765,-225.136458640789));
#227797=CARTESIAN_POINT('Ctrl Pts',(52.8491949026841,25.7323667348012,-223.564699625624));
#227798=CARTESIAN_POINT('Ctrl Pts',(54.7103491827856,28.3042784652506,-220.421181595292));
#227799=CARTESIAN_POINT('Ctrl Pts',(56.5618994916621,30.8869590362523,-217.281419567094));
#227800=CARTESIAN_POINT('Ctrl Pts',(58.4105543383496,33.4721882778783,-214.142529225918));
#227801=CARTESIAN_POINT('Ctrl Pts',(47.2003193864821,18.1182964298664,-233.015989564334));
#227802=CARTESIAN_POINT('Ctrl Pts',(48.1493988764852,19.3809230047756,-231.432724300644));
#227803=CARTESIAN_POINT('Ctrl Pts',(49.0877568643722,20.6584395224563,-229.855761293683));
#227804=CARTESIAN_POINT('Ctrl Pts',(50.0215848134126,21.9412987456968,-228.28073090895));
#227805=CARTESIAN_POINT('Ctrl Pts',(50.9554127624531,23.2241579689375,-226.705700524218));
#227806=CARTESIAN_POINT('Ctrl Pts',(51.8844304624717,24.5129032830703,-225.132894527219));
#227807=CARTESIAN_POINT('Ctrl Pts',(52.811027126582,25.8043188185571,-223.561022084209));
#227808=CARTESIAN_POINT('Ctrl Pts',(54.6642204548024,28.3871498895308,-220.417277198188));
#227809=CARTESIAN_POINT('Ctrl Pts',(56.5079518327106,30.9804583526794,-217.27722687764));
#227810=CARTESIAN_POINT('Ctrl Pts',(58.3485555395427,33.5765033299539,-214.138113904034));
#227811=CARTESIAN_POINT('Ctrl Pts',(47.1871564758985,18.1551125368272,-233.011717209266));
#227812=CARTESIAN_POINT('Ctrl Pts',(48.1304013675538,19.4253209084676,-231.429532035792));
#227813=CARTESIAN_POINT('Ctrl Pts',(49.0646491667038,20.7079796621986,-229.852677272917));
#227814=CARTESIAN_POINT('Ctrl Pts',(49.9946730832209,21.9956338703083,-228.277678228496));
#227815=CARTESIAN_POINT('Ctrl Pts',(50.924696999738,23.283288078418,-226.702679184075));
#227816=CARTESIAN_POINT('Ctrl Pts',(51.8503135061499,24.5763104484158,-225.129741714031));
#227817=CARTESIAN_POINT('Ctrl Pts',(52.7735535901599,25.8719374112347,-223.557730749151));
#227818=CARTESIAN_POINT('Ctrl Pts',(54.62003375818,28.4631913368726,-220.413708819391));
#227819=CARTESIAN_POINT('Ctrl Pts',(56.4572435867786,31.0646235309543,-217.273328544292));
#227820=CARTESIAN_POINT('Ctrl Pts',(58.2910871452732,33.6689870195509,-214.133955876969));
#227821=CARTESIAN_POINT('Ctrl Pts',(47.1711020320382,18.1951169691784,-233.008152197064));
#227822=CARTESIAN_POINT('Ctrl Pts',(48.1091754301695,19.471620881615,-231.426873602798));
#227823=CARTESIAN_POINT('Ctrl Pts',(49.0396359981975,20.7586423084589,-229.850155627119));
#227824=CARTESIAN_POINT('Ctrl Pts',(49.9662083070876,22.0502814645383,-228.275198729438));
#227825=CARTESIAN_POINT('Ctrl Pts',(50.8927806159777,23.3419206206176,-226.700241831756));
#227826=CARTESIAN_POINT('Ctrl Pts',(51.8153427493086,24.6384368291909,-225.12719326289));
#227827=CARTESIAN_POINT('Ctrl Pts',(52.7356127602431,25.9374582798656,-223.555055698046));
#227828=CARTESIAN_POINT('Ctrl Pts',(54.5761527821122,28.535501181215,-220.410780568357));
#227829=CARTESIAN_POINT('Ctrl Pts',(56.4077512436301,31.1433164616566,-217.270071905955));
#227830=CARTESIAN_POINT('Ctrl Pts',(58.2358086912436,33.7542064961608,-214.130435725157));
#227831=CARTESIAN_POINT('Ctrl Pts',(47.1550475881779,18.2351214015296,-233.004587184861));
#227832=CARTESIAN_POINT('Ctrl Pts',(48.0879494927851,19.5179208547626,-231.424215169804));
#227833=CARTESIAN_POINT('Ctrl Pts',(49.0146228296911,20.8093049547191,-229.847633981322));
#227834=CARTESIAN_POINT('Ctrl Pts',(49.9377435309543,22.1049290587682,-228.272719230379));
#227835=CARTESIAN_POINT('Ctrl Pts',(50.8608642322175,23.4005531628173,-226.697804479436));
#227836=CARTESIAN_POINT('Ctrl Pts',(51.7803719924673,24.7005632099661,-225.124644811749));
#227837=CARTESIAN_POINT('Ctrl Pts',(52.6976719303263,26.0029791484965,-223.55238064694));
#227838=CARTESIAN_POINT('Ctrl Pts',(54.5322718060444,28.6078110255573,-220.407852317323));
#227839=CARTESIAN_POINT('Ctrl Pts',(56.3582589004816,31.2220093923588,-217.266815267618));
#227840=CARTESIAN_POINT('Ctrl Pts',(58.1805302372139,33.8394259727705,-214.126915573344));
#227841=CARTESIAN_POINT('Ctrl Pts',(47.1344245348341,18.280247344257,-233.002416451326));
#227842=CARTESIAN_POINT('Ctrl Pts',(48.0632007737606,19.5675523920502,-231.422572450694));
#227843=CARTESIAN_POINT('Ctrl Pts',(48.9866364942849,20.8622514679632,-229.846057608697));
#227844=CARTESIAN_POINT('Ctrl Pts',(49.906818406825,22.1608591102461,-228.271124311316));
#227845=CARTESIAN_POINT('Ctrl Pts',(50.8270003193651,23.459466752529,-226.696191013934));
#227846=CARTESIAN_POINT('Ctrl Pts',(51.7438894778481,24.7620852261766,-225.12290336813));
#227847=CARTESIAN_POINT('Ctrl Pts',(52.6586605054972,26.0670146466549,-223.550499793187));
#227848=CARTESIAN_POINT('Ctrl Pts',(54.4882025607956,28.6768734876113,-220.405692643303));
#227849=CARTESIAN_POINT('Ctrl Pts',(56.3094666870994,31.2957331374271,-217.264328106627));
#227850=CARTESIAN_POINT('Ctrl Pts',(58.1268789337879,33.9179256653815,-214.124164876537));
#227851=CARTESIAN_POINT('Ctrl Pts',(47.1150642483994,18.3236858273299,-232.999295710587));
#227852=CARTESIAN_POINT('Ctrl Pts',(48.0392206238659,19.6158965079908,-231.420362484156));
#227853=CARTESIAN_POINT('Ctrl Pts',(48.9590100671071,20.9141580894346,-229.844205156969));
#227854=CARTESIAN_POINT('Ctrl Pts',(49.8759725739142,22.2158319633755,-228.269472472139));
#227855=CARTESIAN_POINT('Ctrl Pts',(50.7929350807213,23.5175058373164,-226.694739787308));
#227856=CARTESIAN_POINT('Ctrl Pts',(51.7070476323962,24.8226580511233,-225.12147447558));
#227857=CARTESIAN_POINT('Ctrl Pts',(52.6192352667853,26.1299128826243,-223.549042364026));
#227858=CARTESIAN_POINT('Ctrl Pts',(54.4436105355637,28.7444225456263,-220.404178140919));
#227859=CARTESIAN_POINT('Ctrl Pts',(56.2604448907417,31.367132192526,-217.262559371757));
#227860=CARTESIAN_POINT('Ctrl Pts',(58.0734857403641,33.9931206393803,-214.122173015364));
#227861=CARTESIAN_POINT('Ctrl Pts',(47.0957039619647,18.3671243104028,-232.996174969848));
#227862=CARTESIAN_POINT('Ctrl Pts',(48.0152404739711,19.6642406239314,-231.41815251762));
#227863=CARTESIAN_POINT('Ctrl Pts',(48.9313836399292,20.966064710906,-229.842352705242));
#227864=CARTESIAN_POINT('Ctrl Pts',(49.8451267410034,22.2708048165049,-228.267820632962));
#227865=CARTESIAN_POINT('Ctrl Pts',(50.7588698420775,23.575544922104,-226.693288560683));
#227866=CARTESIAN_POINT('Ctrl Pts',(51.6702057869443,24.8832308760699,-225.12004558303));
#227867=CARTESIAN_POINT('Ctrl Pts',(52.5798100280734,26.1928111185938,-223.547584934865));
#227868=CARTESIAN_POINT('Ctrl Pts',(54.3990185103318,28.8119716036413,-220.402663638535));
#227869=CARTESIAN_POINT('Ctrl Pts',(56.2114230943841,31.438531247625,-217.260790636888));
#227870=CARTESIAN_POINT('Ctrl Pts',(58.0200925469402,34.0683156133792,-214.120181154191));
#227871=CARTESIAN_POINT('Ctrl Pts',(47.0872924863604,18.3980576618883,-232.988186791018));
#227872=CARTESIAN_POINT('Ctrl Pts',(47.999710015843,19.7029483255535,-231.41245041461));
#227873=CARTESIAN_POINT('Ctrl Pts',(48.9104078061524,21.0102083195229,-229.837920310538));
#227874=CARTESIAN_POINT('Ctrl Pts',(49.819663384006,22.3192314144748,-228.264239293901));
#227875=CARTESIAN_POINT('Ctrl Pts',(50.7289189618596,23.6282545094267,-226.690558277265));
#227876=CARTESIAN_POINT('Ctrl Pts',(51.636732524911,24.9390441962169,-225.117729434238));
#227877=CARTESIAN_POINT('Ctrl Pts',(52.5433419461414,26.2511531262214,-223.545508348952));
#227878=CARTESIAN_POINT('Ctrl Pts',(54.3565607886023,28.8753709862302,-220.401066178378));
#227879=CARTESIAN_POINT('Ctrl Pts',(56.1649975877485,31.5047913007538,-217.259011215537));
#227880=CARTESIAN_POINT('Ctrl Pts',(57.9700993556152,34.1370914402818,-214.118198613889));
#227881=CARTESIAN_POINT('Ctrl Pts',(47.07151283755,18.4392609475024,-232.980675631547));
#227882=CARTESIAN_POINT('Ctrl Pts',(47.9784669049768,19.7494077885448,-231.40663525448));
#227883=CARTESIAN_POINT('Ctrl Pts',(48.8846403863511,21.0606622046162,-229.833271513153));
#227884=CARTESIAN_POINT('Ctrl Pts',(49.7901160730939,22.3727913382652,-228.260434083043));
#227885=CARTESIAN_POINT('Ctrl Pts',(50.6955917598367,23.6849204719142,-226.687596652933));
#227886=CARTESIAN_POINT('Ctrl Pts',(51.6003698589295,24.9979251551198,-225.115286361312));
#227887=CARTESIAN_POINT('Ctrl Pts',(52.5045272731894,26.3116209606581,-223.543390841591));
#227888=CARTESIAN_POINT('Ctrl Pts',(54.3128421017092,28.939012571735,-220.399599802148));
#227889=CARTESIAN_POINT('Ctrl Pts',(56.1186826713171,31.569141738417,-217.257449700108));
#227890=CARTESIAN_POINT('Ctrl Pts',(57.9225686339535,34.2009514305169,-214.116344107367));
#227891=CARTESIAN_POINT('Ctrl Pts',(47.0636230131447,18.4598625903094,-232.976920051811));
#227892=CARTESIAN_POINT('Ctrl Pts',(47.9678453495437,19.7726375200406,-231.403727674415));
#227893=CARTESIAN_POINT('Ctrl Pts',(48.8717566764505,21.0858891471629,-229.830947114461));
#227894=CARTESIAN_POINT('Ctrl Pts',(49.7753424176378,22.3995713001604,-228.258531477614));
#227895=CARTESIAN_POINT('Ctrl Pts',(50.6789281588252,23.713253453158,-226.686115840768));
#227896=CARTESIAN_POINT('Ctrl Pts',(51.5821885259387,25.0273656345712,-225.114064824849));
#227897=CARTESIAN_POINT('Ctrl Pts',(52.4851199367133,26.3418548778766,-223.54233208791));
#227898=CARTESIAN_POINT('Ctrl Pts',(54.2909827582626,28.9708333644873,-220.398866614033));
#227899=CARTESIAN_POINT('Ctrl Pts',(56.0955252131014,31.6013169572485,-217.256668942392));
#227900=CARTESIAN_POINT('Ctrl Pts',(57.8988032731226,34.2328814256343,-214.115416854107));
#227901=CARTESIAN_POINT('Ctrl Pts',(47.0538541139573,18.4830182871128,-232.973265811648));
#227902=CARTESIAN_POINT('Ctrl Pts',(47.955722927223,19.7978606128634,-231.400808363276));
#227903=CARTESIAN_POINT('Ctrl Pts',(48.8576105358869,21.1127453662178,-229.828584127488));
#227904=CARTESIAN_POINT('Ctrl Pts',(49.7594936036301,22.4276796074738,-228.256586850871));
#227905=CARTESIAN_POINT('Ctrl Pts',(50.6613766713732,23.7426138487298,-226.684589574255));
#227906=CARTESIAN_POINT('Ctrl Pts',(51.5632551884987,25.0575975968797,-225.112819267293));
#227907=CARTESIAN_POINT('Ctrl Pts',(52.4651047016009,26.3726371360198,-223.541268381319));
#227908=CARTESIAN_POINT('Ctrl Pts',(54.2688037278052,29.0027162143,-220.398166609371));
#227909=CARTESIAN_POINT('Ctrl Pts',(56.0723874025208,31.6330198944631,-217.255944116137));
#227910=CARTESIAN_POINT('Ctrl Pts',(57.875649653532,34.2635844996751,-214.114522751136));
#227911=CARTESIAN_POINT('Ctrl Pts',(47.0405353763693,18.5106352292473,-232.969983979348));
#227912=CARTESIAN_POINT('Ctrl Pts',(47.9405971515569,19.8268187140002,-231.398125716493));
#227913=CARTESIAN_POINT('Ctrl Pts',(48.8408986391317,21.1427526567519,-229.826381496195));
#227914=CARTESIAN_POINT('Ctrl Pts',(49.7414431123329,22.4584427038901,-228.254759191353));
#227915=CARTESIAN_POINT('Ctrl Pts',(50.6419875855342,23.7741327510283,-226.683136886512));
#227916=CARTESIAN_POINT('Ctrl Pts',(51.5427750540585,25.0895788993504,-225.111636500013));
#227917=CARTESIAN_POINT('Ctrl Pts',(52.443808131774,26.4047878990792,-223.540266455142));
#227918=CARTESIAN_POINT('Ctrl Pts',(54.2458742872048,29.0352058985368,-220.397526365399));
#227919=CARTESIAN_POINT('Ctrl Pts',(56.0489238784563,31.6646741163143,-217.255307216989));
#227920=CARTESIAN_POINT('Ctrl Pts',(57.852967529916,34.2932604357928,-214.113682169595));
#227921=CARTESIAN_POINT('Ctrl Pts',(47.0338760075754,18.5244437003147,-232.968343063198));
#227922=CARTESIAN_POINT('Ctrl Pts',(47.9330342637239,19.8412977645685,-231.396784393101));
#227923=CARTESIAN_POINT('Ctrl Pts',(48.8325426907541,21.1577563020188,-229.825280180548));
#227924=CARTESIAN_POINT('Ctrl Pts',(49.7324178666844,22.4738242520981,-228.253845361594));
#227925=CARTESIAN_POINT('Ctrl Pts',(50.6322930426146,23.7898922021775,-226.682410542641));
#227926=CARTESIAN_POINT('Ctrl Pts',(51.5325349868385,25.1055695505858,-225.111045116373));
#227927=CARTESIAN_POINT('Ctrl Pts',(52.4331598468605,26.4208632806089,-223.539765492053));
#227928=CARTESIAN_POINT('Ctrl Pts',(54.2344095669047,29.0514507406552,-220.397206243413));
#227929=CARTESIAN_POINT('Ctrl Pts',(56.0371921164241,31.6805012272399,-217.254988767415));
#227930=CARTESIAN_POINT('Ctrl Pts',(57.8416264681079,34.3080984038517,-214.113261878824));
#227931=CARTESIAN_POINT('Ctrl Pts',(47.0263410003839,18.5393529178172,-232.966789761807));
#227932=CARTESIAN_POINT('Ctrl Pts',(47.9247284510372,19.856700801254,-231.395498625619));
#227933=CARTESIAN_POINT('Ctrl Pts',(48.8235505406218,21.1735412519938,-229.824216617793));
#227934=CARTESIAN_POINT('Ctrl Pts',(49.7228457883083,22.4898650532266,-228.252959195293));
#227935=CARTESIAN_POINT('Ctrl Pts',(50.6221410359948,23.8061888544594,-226.681701772792));
#227936=CARTESIAN_POINT('Ctrl Pts',(51.5219094725163,25.1219959484843,-225.110468904466));
#227937=CARTESIAN_POINT('Ctrl Pts',(52.4221921058014,26.4372796694717,-223.539279612374));
#227938=CARTESIAN_POINT('Ctrl Pts',(54.2227573723716,29.0678471114466,-220.396901028191));
#227939=CARTESIAN_POINT('Ctrl Pts',(56.0253786795592,31.6963162745203,-217.254692290257));
#227940=CARTESIAN_POINT('Ctrl Pts',(57.8304030425693,34.3226797077107,-214.112855014843));
#227941=CARTESIAN_POINT('Ctrl Pts',(47.0177828560111,18.5555300817996,-232.96533252157));
#227942=CARTESIAN_POINT('Ctrl Pts',(47.9155370349421,19.8731929180949,-231.394280823516));
#227943=CARTESIAN_POINT('Ctrl Pts',(48.8137913023007,21.1902606020353,-229.823202807664));
#227944=CARTESIAN_POINT('Ctrl Pts',(49.7126093236726,22.5067040125525,-228.252111396185));
#227945=CARTESIAN_POINT('Ctrl Pts',(50.6114273450444,23.8231474230696,-226.681019984706));
#227946=CARTESIAN_POINT('Ctrl Pts',(51.5108090328418,25.1389665178458,-225.109915092335));
#227947=CARTESIAN_POINT('Ctrl Pts',(52.4108279627846,26.4541313607334,-223.538814574431));
#227948=CARTESIAN_POINT('Ctrl Pts',(54.2108658226704,29.0844610465087,-220.396613538622));
#227949=CARTESIAN_POINT('Ctrl Pts',(56.0134397408495,31.7121723231175,-217.254421501589));
#227950=CARTESIAN_POINT('Ctrl Pts',(57.8192783928772,34.3370299914758,-214.112464332901));
#227951=CARTESIAN_POINT('Ctrl Pts',(47.0135037838248,18.5636186637907,-232.964603901451));
#227952=CARTESIAN_POINT('Ctrl Pts',(47.9109413268945,19.8814389765153,-231.393671922464));
#227953=CARTESIAN_POINT('Ctrl Pts',(48.8089116831402,21.1986202770561,-229.822695902599));
#227954=CARTESIAN_POINT('Ctrl Pts',(49.7074910913547,22.5151234922153,-228.251687496631));
#227955=CARTESIAN_POINT('Ctrl Pts',(50.6060704995693,23.8316267073747,-226.680679090663));
#227956=CARTESIAN_POINT('Ctrl Pts',(51.5052588130045,25.1474518025266,-225.109638186271));
#227957=CARTESIAN_POINT('Ctrl Pts',(52.4051458912763,26.4625572063643,-223.538582055459));
#227958=CARTESIAN_POINT('Ctrl Pts',(54.2049200478198,29.0927680140397,-220.396469793837));
#227959=CARTESIAN_POINT('Ctrl Pts',(56.0074702714946,31.7201003474161,-217.254286107255));
#227960=CARTESIAN_POINT('Ctrl Pts',(57.8137160680311,34.3442051333583,-214.11226899193));
#227961=CARTESIAN_POINT('Ctrl Pts',(47.0089694792463,18.5720236309689,-232.963899094952));
#227962=CARTESIAN_POINT('Ctrl Pts',(47.9061246605823,19.8899568147843,-231.393079846389));
#227963=CARTESIAN_POINT('Ctrl Pts',(48.8038406245385,21.2072131852528,-229.822201313241));
#227964=CARTESIAN_POINT('Ctrl Pts',(49.7022070147003,22.523742233991,-228.251273097427));
#227965=CARTESIAN_POINT('Ctrl Pts',(50.6005734048621,23.8402712827293,-226.680344881612));
#227966=CARTESIAN_POINT('Ctrl Pts',(51.4995899823701,25.1560729994673,-225.109366839153));
#227967=CARTESIAN_POINT('Ctrl Pts',(52.3993648097282,26.4710917806424,-223.538354716999));
#227968=CARTESIAN_POINT('Ctrl Pts',(54.1989144644443,29.1011293429925,-220.39633047269));
#227969=CARTESIAN_POINT('Ctrl Pts',(56.0014694266273,31.7280386185765,-217.25415713023));
#227970=CARTESIAN_POINT('Ctrl Pts',(57.8081784241041,34.3513225267891,-214.112077698071));
#227971=CARTESIAN_POINT('Ctrl Pts',(47.0041643855294,18.580762838696,-232.963218170749));
#227972=CARTESIAN_POINT('Ctrl Pts',(47.9010716022698,19.8987644772325,-231.392505287657));
#227973=CARTESIAN_POINT('Ctrl Pts',(48.7985636253896,21.2160564611115,-229.821719884836));
#227974=CARTESIAN_POINT('Ctrl Pts',(49.6967438426135,22.5325760511435,-228.250869035074));
#227975=CARTESIAN_POINT('Ctrl Pts',(50.5949240598375,23.8490956411754,-226.680018185312));
#227976=CARTESIAN_POINT('Ctrl Pts',(51.4937920916948,25.1648428846195,-225.10910171349));
#227977=CARTESIAN_POINT('Ctrl Pts',(52.3934756614324,26.4797462844595,-223.53813309987));
#227978=CARTESIAN_POINT('Ctrl Pts',(54.1928428009075,29.1095530841393,-220.396195872632));
#227979=CARTESIAN_POINT('Ctrl Pts',(55.9954317595172,31.7359937276413,-217.254034998605));
#227980=CARTESIAN_POINT('Ctrl Pts',(57.8026630300816,34.3583854144121,-214.111890802731));
#227981=CARTESIAN_POINT('Ctrl Pts',(46.9993592918125,18.5895020464233,-232.962537246545));
#227982=CARTESIAN_POINT('Ctrl Pts',(47.8960185439573,19.9075721396807,-231.391930728925));
#227983=CARTESIAN_POINT('Ctrl Pts',(48.7932866262407,21.2248997369702,-229.821238456431));
#227984=CARTESIAN_POINT('Ctrl Pts',(49.6912806705268,22.5414098682959,-228.250464972721));
#227985=CARTESIAN_POINT('Ctrl Pts',(50.5892747148128,23.8579199996217,-226.679691489012));
#227986=CARTESIAN_POINT('Ctrl Pts',(51.4879942010195,25.1736127697718,-225.108836587826));
#227987=CARTESIAN_POINT('Ctrl Pts',(52.3875865131366,26.4884007882765,-223.537911482743));
#227988=CARTESIAN_POINT('Ctrl Pts',(54.1867711373708,29.117976825286,-220.396061272575));
#227989=CARTESIAN_POINT('Ctrl Pts',(55.9893940924071,31.7439488367061,-217.25391286698));
#227990=CARTESIAN_POINT('Ctrl Pts',(57.7971476360592,34.365448302035,-214.11170390739));
#227991=CARTESIAN_POINT('Ctrl Pts',(46.9913120403997,18.6016320696042,-232.962809737275));
#227992=CARTESIAN_POINT('Ctrl Pts',(47.8881017068652,19.919347208754,-231.392174086571));
#227993=CARTESIAN_POINT('Ctrl Pts',(48.7854927208081,21.2363283107576,-229.821456748291));
#227994=CARTESIAN_POINT('Ctrl Pts',(49.6835984491062,22.5525036430274,-228.250662893886));
#227995=CARTESIAN_POINT('Ctrl Pts',(50.5817041774044,23.8686789752972,-226.679869039482));
#227996=CARTESIAN_POINT('Ctrl Pts',(51.480524130202,25.1840486327538,-225.108998471456));
#227997=CARTESIAN_POINT('Ctrl Pts',(52.3802004849816,26.4985292873713,-223.538062914284));
#227998=CARTESIAN_POINT('Ctrl Pts',(54.1795531945409,29.1274905966065,-220.396191799938));
#227999=CARTESIAN_POINT('Ctrl Pts',(55.9822813208348,31.7529097593695,-217.254043978496));
#228000=CARTESIAN_POINT('Ctrl Pts',(57.7900093367969,34.3739628192697,-214.111856605281));
#228001=CARTESIAN_POINT('Ctrl Pts',(46.9840049393815,18.6129810161854,-232.962872244472));
#228002=CARTESIAN_POINT('Ctrl Pts',(47.8808382771992,19.9304390734321,-231.392237704844));
#228003=CARTESIAN_POINT('Ctrl Pts',(48.7782728428765,21.247161929372,-229.821521522905));
#228004=CARTESIAN_POINT('Ctrl Pts',(49.6764219919997,22.5630778387597,-228.250728876356));
#228005=CARTESIAN_POINT('Ctrl Pts',(50.5745711411229,23.8789937481474,-226.679936229808));
#228006=CARTESIAN_POINT('Ctrl Pts',(51.4734343837544,25.1941028059552,-225.109066921118));
#228007=CARTESIAN_POINT('Ctrl Pts',(52.3731538889575,26.508321667889,-223.538132682591));
#228008=CARTESIAN_POINT('Ctrl Pts',(54.1725928993637,29.1367593917566,-220.396264205537));
#228009=CARTESIAN_POINT('Ctrl Pts',(55.9754067618462,31.7616502024816,-217.254119255235));
#228010=CARTESIAN_POINT('Ctrl Pts',(57.7832199428974,34.3821699572177,-214.111935079921));
#228011=CARTESIAN_POINT('',(47.0649767742812,18.6816981840219,-232.850050031414));
#228012=CARTESIAN_POINT('',(47.5797438888055,17.1282946860168,-232.850050025775));
#228013=CARTESIAN_POINT('Ctrl Pts',(47.0649772746806,18.681698503234,-232.85005));
#228014=CARTESIAN_POINT('Ctrl Pts',(47.0894454875514,18.6433419440303,-232.85005));
#228015=CARTESIAN_POINT('Ctrl Pts',(47.1308648548305,18.5779811902918,-232.850050000004));
#228016=CARTESIAN_POINT('Ctrl Pts',(47.1945089631974,18.4622232724225,-232.850050000004));
#228017=CARTESIAN_POINT('Ctrl Pts',(47.228457737075,18.3956815601865,-232.850049999972));
#228018=CARTESIAN_POINT('Ctrl Pts',(47.2942811083109,18.2644664453497,-232.850049999972));
#228019=CARTESIAN_POINT('Ctrl Pts',(47.3292660641502,18.1888432668772,-232.850050000077));
#228020=CARTESIAN_POINT('Ctrl Pts',(47.3838144288267,18.0534939114453,-232.850050000077));
#228021=CARTESIAN_POINT('Ctrl Pts',(47.4061285795857,17.9946070609481,-232.850050000004));
#228022=CARTESIAN_POINT('Ctrl Pts',(47.4807135149771,17.7819049672691,-232.850050000004));
#228023=CARTESIAN_POINT('Ctrl Pts',(47.5062786117714,17.6714141232655,-232.850050000232));
#228024=CARTESIAN_POINT('Ctrl Pts',(47.5414163429777,17.4969266356066,-232.850050000232));
#228025=CARTESIAN_POINT('Ctrl Pts',(47.5518232649238,17.4292236058328,-232.85005));
#228026=CARTESIAN_POINT('Ctrl Pts',(47.5744421319946,17.2492890927419,-232.85005));
#228027=CARTESIAN_POINT('Ctrl Pts',(47.5778246725068,17.1749507868806,-232.85005));
#228028=CARTESIAN_POINT('Ctrl Pts',(47.5797441362696,17.1282946961977,-232.85005));
#228029=CARTESIAN_POINT('',(59.5744430571196,28.6979747816085,-214.56059856522));
#228030=CARTESIAN_POINT('Ctrl Pts',(59.574442786197,28.6979745676233,-214.560598252186));
#228031=CARTESIAN_POINT('Ctrl Pts',(55.5761465166848,24.8416079159137,-220.657162906121));
#228032=CARTESIAN_POINT('Ctrl Pts',(51.5778799971752,20.9851500975526,-226.753689417593));
#228033=CARTESIAN_POINT('Ctrl Pts',(47.5797437329671,17.1282947147807,-232.85004994177));
#228034=CARTESIAN_POINT('',(59.5599473199192,29.0716011550534,-214.548757454512));
#228035=CARTESIAN_POINT('Ctrl Pts',(59.5599473199158,29.0716011550592,-214.548757454608));
#228036=CARTESIAN_POINT('Ctrl Pts',(59.562335847696,29.0094631058834,-214.552626620787));
#228037=CARTESIAN_POINT('Ctrl Pts',(59.5647394386419,28.9472090864927,-214.555583575921));
#228038=CARTESIAN_POINT('Ctrl Pts',(59.5683821822733,28.8533107884066,-214.558574296067));
#228039=CARTESIAN_POINT('Ctrl Pts',(59.5696089211159,28.8217653832972,-214.559329741406));
#228040=CARTESIAN_POINT('Ctrl Pts',(59.5720174159227,28.7599810676142,-214.560318279807));
#228041=CARTESIAN_POINT('Ctrl Pts',(59.5727190081475,28.7420025676916,-214.5605526967));
#228042=CARTESIAN_POINT('Ctrl Pts',(59.5744429767042,28.6979747794677,-214.560599513176));
#228043=CARTESIAN_POINT('',(57.6802384108496,34.1916869461204,-214.317651786459));
#228044=CARTESIAN_POINT('Ctrl Pts',(57.6802384405887,34.1916869762635,-214.317652096406));
#228045=CARTESIAN_POINT('Ctrl Pts',(57.7110766561566,34.1523839012924,-214.318515520258));
#228046=CARTESIAN_POINT('Ctrl Pts',(57.7444787489014,34.1091244865649,-214.319516304846));
#228047=CARTESIAN_POINT('Ctrl Pts',(57.8155385849077,34.0150346366398,-214.321768181642));
#228048=CARTESIAN_POINT('Ctrl Pts',(57.8508234071893,33.9673227106139,-214.32296093355));
#228049=CARTESIAN_POINT('Ctrl Pts',(57.9661234018469,33.8080831440916,-214.32727701056));
#228050=CARTESIAN_POINT('Ctrl Pts',(58.0434074298077,33.6958767305193,-214.331195699283));
#228051=CARTESIAN_POINT('Ctrl Pts',(58.1756532244486,33.4942246550505,-214.338033936497));
#228052=CARTESIAN_POINT('Ctrl Pts',(58.2321817369315,33.4045586829631,-214.340952245207));
#228053=CARTESIAN_POINT('Ctrl Pts',(58.3756461183976,33.1676840614643,-214.348689659444));
#228054=CARTESIAN_POINT('Ctrl Pts',(58.4602479257748,33.018425566341,-214.353756590895));
#228055=CARTESIAN_POINT('Ctrl Pts',(58.6568844792401,32.6464976653534,-214.368544945655));
#228056=CARTESIAN_POINT('Ctrl Pts',(58.7646217839372,32.420153660951,-214.377793138464));
#228057=CARTESIAN_POINT('Ctrl Pts',(58.9195386090982,32.0554702584067,-214.392846705455));
#228058=CARTESIAN_POINT('Ctrl Pts',(58.9732785720272,31.919705788645,-214.398754579606));
#228059=CARTESIAN_POINT('Ctrl Pts',(59.1078149579066,31.553570829642,-214.415391307452));
#228060=CARTESIAN_POINT('Ctrl Pts',(59.1824588553372,31.3211191066135,-214.426591762045));
#228061=CARTESIAN_POINT('Ctrl Pts',(59.2717173594831,30.9979484732622,-214.442018247785));
#228062=CARTESIAN_POINT('Ctrl Pts',(59.2947355260367,30.9092561462818,-214.446284061645));
#228063=CARTESIAN_POINT('Ctrl Pts',(59.3544699104682,30.6634680434043,-214.458293748763));
#228064=CARTESIAN_POINT('Ctrl Pts',(59.388219665549,30.5059342511955,-214.466398394895));
#228065=CARTESIAN_POINT('Ctrl Pts',(59.459087253972,30.1244208307842,-214.487274531045));
#228066=CARTESIAN_POINT('Ctrl Pts',(59.4920723938872,29.8990070152647,-214.499666866016));
#228067=CARTESIAN_POINT('Ctrl Pts',(59.5376880887883,29.4727426573021,-214.524039704182));
#228068=CARTESIAN_POINT('Ctrl Pts',(59.552234017423,29.272264329899,-214.536262708201));
#228069=CARTESIAN_POINT('Ctrl Pts',(59.559947319918,29.0716011550591,-214.548757454604));
#228070=CARTESIAN_POINT('Ctrl Pts',(47.064976549062,18.6816980304454,-232.850049773951));
#228071=CARTESIAN_POINT('Ctrl Pts',(48.8271464669406,21.2716316239801,-229.763684175805));
#228072=CARTESIAN_POINT('Ctrl Pts',(50.5916241034348,23.8587402441049,-226.676997721226));
#228073=CARTESIAN_POINT('Ctrl Pts',(54.1292220261611,29.0291984552365,-220.499446390719));
#228074=CARTESIAN_POINT('Ctrl Pts',(55.9023301608819,31.6125420406575,-217.408571384037));
#228075=CARTESIAN_POINT('Ctrl Pts',(57.680238354192,34.1916868896098,-214.317651706715));
#228076=CARTESIAN_POINT('Origin',(41.5452362233251,-63.7990866568863,-205.306318983907));
#228077=CARTESIAN_POINT('',(47.2772325636527,-70.8123207858077,-202.84995));
#228078=CARTESIAN_POINT('',(41.9017397792002,-72.8497297394107,-202.84995));
#228079=CARTESIAN_POINT('Origin',(41.5452362233251,-63.7990866568863,-202.84995));
#228080=CARTESIAN_POINT('',(47.1516276096017,-70.6586401308144,-214.220867040027));
#228081=CARTESIAN_POINT('',(47.250099122033,-70.7791223733342,-205.306318983907));
#228082=CARTESIAN_POINT('Ctrl Pts',(47.1516276096073,-70.658640130818,-214.220867039664));
#228083=CARTESIAN_POINT('Ctrl Pts',(47.1049465298329,-70.6968004924595,
-214.220539579083));
#228084=CARTESIAN_POINT('Ctrl Pts',(47.0581254645249,-70.7342797725841,
-214.220714572147));
#228085=CARTESIAN_POINT('Ctrl Pts',(46.9626662222936,-70.8090665014228,
-214.222095580797));
#228086=CARTESIAN_POINT('Ctrl Pts',(46.9147757072848,-70.845791160474,-214.22327290135));
#228087=CARTESIAN_POINT('Ctrl Pts',(46.8664918175106,-70.8820283127247,
-214.224988432219));
#228088=CARTESIAN_POINT('',(41.9000522051254,-72.8068868830794,-205.306318983907));
#228089=CARTESIAN_POINT('Origin',(0.,-12.9675000200281,-205.306318983907));
#228090=CARTESIAN_POINT('Ctrl Pts',(50.9302694868398,-67.3511117059353,
-214.24934096937));
#228091=CARTESIAN_POINT('Ctrl Pts',(50.6301450874053,-67.6322327827628,
-214.247062743179));
#228092=CARTESIAN_POINT('Ctrl Pts',(50.3277270489376,-67.9108411525983,
-214.244646208668));
#228093=CARTESIAN_POINT('Ctrl Pts',(49.7080810417752,-68.4722815055611,
-214.240153263142));
#228094=CARTESIAN_POINT('Ctrl Pts',(49.3907687171516,-68.7548784336109,
-214.238095007482));
#228095=CARTESIAN_POINT('Ctrl Pts',(48.439158745486,-69.5878975442323,-214.231198509906));
#228096=CARTESIAN_POINT('Ctrl Pts',(47.7996962354047,-70.1288637578719,
-214.225413141189));
#228097=CARTESIAN_POINT('Ctrl Pts',(47.1516276096073,-70.658640130818,-214.220867039664));
#228098=CARTESIAN_POINT('',(57.7103246972002,-60.4088156810276,-202.84995));
#228099=CARTESIAN_POINT('Origin',(0.,-12.9675000200281,-202.84995));
#228100=CARTESIAN_POINT('',(57.55661147574,-60.2824542804282,-214.249782619794));
#228101=CARTESIAN_POINT('',(57.677203474973,-60.3815880685163,-205.306318983907));
#228102=CARTESIAN_POINT('Ctrl Pts',(57.5566114760922,-60.2824542808246,
-214.249782589791));
#228103=CARTESIAN_POINT('Ctrl Pts',(57.0250153199809,-60.9290548756098,
-214.252086125667));
#228104=CARTESIAN_POINT('Ctrl Pts',(56.4825490095513,-61.5666907428382,
-214.255305282268));
#228105=CARTESIAN_POINT('Ctrl Pts',(55.3753515253954,-62.8244435216547,
-214.258374348072));
#228106=CARTESIAN_POINT('Ctrl Pts',(54.8117226674573,-63.4434099518073,
-214.259195881146));
#228107=CARTESIAN_POINT('Ctrl Pts',(54.2386983288856,-64.0517945375328,
-214.260116172733));
#228108=CARTESIAN_POINT('Origin',(50.7133971693864,-54.6569255427236,-205.306318983907));
#228109=CARTESIAN_POINT('',(59.7639914300581,-55.014666400457,-202.84995));
#228110=CARTESIAN_POINT('Origin',(50.7133971693864,-54.6569255427236,-202.84995));
#228111=CARTESIAN_POINT('',(59.7211488048338,-55.0129729693901,-205.306318983907));
#228112=CARTESIAN_POINT('Origin',(53.6115278221397,-57.0237333927552,-218.549922256745));
#228113=CARTESIAN_POINT('Origin',(50.7133971693864,28.7219255026674,-205.306318983907));
#228114=CARTESIAN_POINT('',(57.7103246972002,34.4738156409714,-202.84995));
#228115=CARTESIAN_POINT('',(59.7639914300583,29.0796663604006,-202.84995));
#228116=CARTESIAN_POINT('Origin',(50.7133971693864,28.7219255026674,-202.84995));
#228117=CARTESIAN_POINT('',(57.555715349607,34.3467175710979,-214.316254908503));
#228118=CARTESIAN_POINT('',(57.677203474973,34.44658802846,-205.306318983907));
#228119=CARTESIAN_POINT('Origin',(53.9184245358859,31.3368194791132,-218.66087791612));
#228120=CARTESIAN_POINT('',(59.7211488048339,29.0779729293336,-205.306318983907));
#228121=CARTESIAN_POINT('Origin',(0.,-12.9675000200281,-205.306318983907));
#228122=CARTESIAN_POINT('Ctrl Pts',(54.1218033362461,38.2387592926022,-214.333529894748));
#228123=CARTESIAN_POINT('Ctrl Pts',(54.7165719869227,37.6101910901286,-214.330972785209));
#228124=CARTESIAN_POINT('Ctrl Pts',(55.3004791816396,36.9711411157046,-214.328783039069));
#228125=CARTESIAN_POINT('Ctrl Pts',(56.4462564532789,35.6724908998646,-214.323424691429));
#228126=CARTESIAN_POINT('Ctrl Pts',(57.006890673464,35.0142562800167,-214.319260128838));
#228127=CARTESIAN_POINT('Ctrl Pts',(57.5557151719484,34.346717423436,-214.316255263493));
#228128=CARTESIAN_POINT('',(47.0132029332902,45.0921138114136,-202.84995));
#228129=CARTESIAN_POINT('Origin',(0.,-12.9675000200281,-202.84995));
#228130=CARTESIAN_POINT('',(46.8872094279775,44.936516366183,-214.320099730218));
#228131=CARTESIAN_POINT('',(46.9862210240714,45.0587921244845,-205.306318983907));
#228132=CARTESIAN_POINT('Ctrl Pts',(46.8872094285464,44.9365163666477,-214.32009968902));
#228133=CARTESIAN_POINT('Ctrl Pts',(47.5590386445095,44.3924387483626,-214.323238559856));
#228134=CARTESIAN_POINT('Ctrl Pts',(48.2215138694951,43.8365850803835,-214.326981002858));
#228135=CARTESIAN_POINT('Ctrl Pts',(49.2064774018634,42.9804492021061,-214.330624876612));
#228136=CARTESIAN_POINT('Ctrl Pts',(49.534775993172,42.6899700282977,-214.331589339685));
#228137=CARTESIAN_POINT('Ctrl Pts',(50.1777464098916,42.1108600896211,-214.333796679539));
#228138=CARTESIAN_POINT('Ctrl Pts',(50.4923590575389,41.8225600986686,-214.334966128449));
#228139=CARTESIAN_POINT('Ctrl Pts',(50.804536443953,41.5315226006458,-214.335913275952));
#228140=CARTESIAN_POINT('Origin',(41.3132181298675,38.0528376956935,-205.306318983907));
#228141=CARTESIAN_POINT('',(43.0099907914441,46.9501517582364,-202.84995));
#228142=CARTESIAN_POINT('Origin',(41.3132181298675,38.0528376956935,-202.84995));
#228143=CARTESIAN_POINT('',(43.001958811097,46.9080347125589,-205.306318983907));
#228144=CARTESIAN_POINT('Origin',(43.9075665164217,41.2822320849722,-218.664372653694));
#228145=CARTESIAN_POINT('Origin',(0.,990.91999998,-205.306318983907));
#228146=CARTESIAN_POINT('Origin',(0.,990.91999998,-202.84995));
#228147=CARTESIAN_POINT('Ctrl Pts',(41.3748964705092,-72.6655519150593,
-214.574036340781));
#228148=CARTESIAN_POINT('Ctrl Pts',(40.060737297785,-72.7166606458032,-214.574827132799));
#228149=CARTESIAN_POINT('Ctrl Pts',(38.7464886157294,-72.7653339442147,
-214.575594614694));
#228150=CARTESIAN_POINT('Ctrl Pts',(36.1178116825572,-72.8578102048044,
-214.577053530196));
#228151=CARTESIAN_POINT('Ctrl Pts',(34.8033909849928,-72.9016129087915,
-214.577744931393));
#228152=CARTESIAN_POINT('Ctrl Pts',(33.4888918292045,-72.9429801998252,
-214.57839031164));
#228153=CARTESIAN_POINT('Origin',(-476.643301415307,-33.8122127813758,-202.84995));
#228154=CARTESIAN_POINT('',(43.478316039927,49.4058943061501,-202.84995));
#228155=CARTESIAN_POINT('Origin',(0.,-178.58000002,-202.84995));
#228156=CARTESIAN_POINT('',(42.0001381210477,-75.3477925421285,-202.84995));
#228157=CARTESIAN_POINT('Origin',(0.,990.91999998,-202.84995));
#228158=CARTESIAN_POINT('',(48.8593175837476,-72.7480395125837,-202.84995));
#228159=CARTESIAN_POINT('Origin',(41.5452362233251,-63.7990866568863,-202.84995));
#228160=CARTESIAN_POINT('',(59.6415426483635,-61.9963915768841,-202.84995));
#228161=CARTESIAN_POINT('Origin',(0.,-12.9675000200281,-202.84995));
#228162=CARTESIAN_POINT('',(62.2620407574844,-55.1134062492798,-202.84995));
#228163=CARTESIAN_POINT('Origin',(50.7133971693864,-54.6569255427236,-202.84995));
#228164=CARTESIAN_POINT('',(62.2620407574844,29.1784062092233,-202.84995));
#228165=CARTESIAN_POINT('Origin',(-1004.,-12.967500020028,-202.84995));
#228166=CARTESIAN_POINT('',(59.6415426483635,36.0613915368278,-202.84995));
#228167=CARTESIAN_POINT('Origin',(50.7133971693864,28.7219255026674,-202.84995));
#228168=CARTESIAN_POINT('',(48.5864524674565,47.0350203720195,-202.84995));
#228169=CARTESIAN_POINT('Origin',(0.,-12.9675000200281,-202.84995));
#228170=CARTESIAN_POINT('Origin',(41.3132181298675,38.0528376956935,-202.84995));
#228171=CARTESIAN_POINT('Origin',(0.,-178.58000002,-202.84995));
#228172=CARTESIAN_POINT('Origin',(-1004.,-12.967500020028,-202.84995));
#228173=CARTESIAN_POINT('Origin',(-1004.,-12.967500020028,-179.606318983907));
#228174=CARTESIAN_POINT('',(62.6666822880186,29.1944003864053,-179.64995));
#228175=CARTESIAN_POINT('',(62.6666822880186,-55.1294004264619,-179.64995));
#228176=CARTESIAN_POINT('Origin',(-1004.,-12.967500020028,-179.64995));
#228177=CARTESIAN_POINT('',(62.6674432759984,29.1944304658105,-179.606318983907));
#228178=CARTESIAN_POINT('',(62.6674432759983,-55.1294305058671,-179.606318983907));
#228179=CARTESIAN_POINT('Origin',(50.7133971693864,28.7219255026673,-179.606318983907));
#228180=CARTESIAN_POINT('',(59.9543671306402,36.3185518471891,-179.64995));
#228181=CARTESIAN_POINT('Origin',(50.7133971693864,28.7219255026673,-179.64995));
#228182=CARTESIAN_POINT('',(59.9549554431411,36.3190354750184,-179.606318983907));
#228183=CARTESIAN_POINT('Origin',(0.,-12.9675000200281,-179.606318983907));
#228184=CARTESIAN_POINT('',(48.8412921507357,47.3497382103492,-179.64995));
#228185=CARTESIAN_POINT('Origin',(0.,-12.9675000200281,-179.64995));
#228186=CARTESIAN_POINT('',(48.8417714142841,47.3503300835849,-179.606318983907));
#228187=CARTESIAN_POINT('Origin',(41.3132181298675,38.0528376956935,-179.606318983907));
#228188=CARTESIAN_POINT('',(43.5541767698386,49.8036828575113,-179.64995));
#228189=CARTESIAN_POINT('Origin',(41.3132181298675,38.0528376956935,-179.64995));
#228190=CARTESIAN_POINT('',(43.5543194371113,49.8044309574546,-179.606318983907));
#228191=CARTESIAN_POINT('Origin',(0.,-178.58000002,-179.606318983907));
#228192=CARTESIAN_POINT('Origin',(0.,-178.58000002,-179.64995));
#228193=CARTESIAN_POINT('Origin',(0.,990.91999998,-179.606318983907));
#228194=CARTESIAN_POINT('',(42.0160769799045,-75.7524362554308,-179.64995));
#228195=CARTESIAN_POINT('Origin',(0.,990.91999998,-179.64995));
#228196=CARTESIAN_POINT('',(42.0161069552755,-75.7531972475156,-179.606318983907));
#228197=CARTESIAN_POINT('Origin',(41.5452362233251,-63.7990866568863,-179.606318983907));
#228198=CARTESIAN_POINT('',(49.1155884655664,-73.0615930440079,-179.64995));
#228199=CARTESIAN_POINT('Origin',(41.5452362233251,-63.7990866568863,-179.64995));
#228200=CARTESIAN_POINT('',(49.1160704206943,-73.0621827275931,-179.606318983907));
#228201=CARTESIAN_POINT('Origin',(0.,-12.9675000200281,-179.606318983907));
#228202=CARTESIAN_POINT('',(59.9543671306402,-62.2535518872453,-179.64995));
#228203=CARTESIAN_POINT('Origin',(0.,-12.9675000200281,-179.64995));
#228204=CARTESIAN_POINT('',(59.9549554431411,-62.2540355150746,-179.606318983907));
#228205=CARTESIAN_POINT('Origin',(50.7133971693864,-54.6569255427236,-179.606318983907));
#228206=CARTESIAN_POINT('Origin',(50.7133971693864,-54.6569255427236,-179.64995));
#228207=CARTESIAN_POINT('Ctrl Pts',(47.5079779560868,-40.2034134198457,
-232.959831751742));
#228208=CARTESIAN_POINT('Ctrl Pts',(51.5558271984379,-45.0119998619165,
-226.787659137649));
#228209=CARTESIAN_POINT('Ctrl Pts',(55.603839292235,-49.8201780781628,-220.615275392699));
#228210=CARTESIAN_POINT('Ctrl Pts',(59.6518858770376,-54.6282695245469,
-214.442846690034));
#228211=CARTESIAN_POINT('Ctrl Pts',(47.6083941910801,-37.6707809958978,
-232.96396511673));
#228212=CARTESIAN_POINT('Ctrl Pts',(51.6738491177805,-42.0114382175837,
-226.791891649754));
#228213=CARTESIAN_POINT('Ctrl Pts',(55.7393519427245,-46.3514436774691,
-220.61950573142));
#228214=CARTESIAN_POINT('Ctrl Pts',(59.8047170999058,-50.6912943906935,
-214.447047813144));
#228215=CARTESIAN_POINT('Ctrl Pts',(47.6970999179399,-35.0937046824551,
-232.967721023846));
#228216=CARTESIAN_POINT('Ctrl Pts',(51.7757137841176,-39.0045377390498,
-226.795568831742));
#228217=CARTESIAN_POINT('Ctrl Pts',(55.8544675412487,-42.9147019697459,
-220.623140932772));
#228218=CARTESIAN_POINT('Ctrl Pts',(59.9332050840609,-46.8246892042479,
-214.450640245293));
#228219=CARTESIAN_POINT('Ctrl Pts',(47.7724784290048,-32.4865586987341,
-232.970973990925));
#228220=CARTESIAN_POINT('Ctrl Pts',(51.8616631458841,-35.9897429718971,
-226.798709657862));
#228221=CARTESIAN_POINT('Ctrl Pts',(55.9509791745034,-39.4923578424338,
-220.626231304292));
#228222=CARTESIAN_POINT('Ctrl Pts',(60.0403077603802,-42.9948148700989,
-214.453693714461));
#228223=CARTESIAN_POINT('',(47.8511644984997,-32.6020541825672,-232.850071652983));
#228224=CARTESIAN_POINT('Ctrl Pts',(47.8511937435036,-32.6021335774055,
-232.85005));
#228225=CARTESIAN_POINT('Ctrl Pts',(47.8129987256184,-33.8832172184,-232.85005));
#228226=CARTESIAN_POINT('Ctrl Pts',(47.7712743196191,-35.1649732916759,
-232.850050000001));
#228227=CARTESIAN_POINT('Ctrl Pts',(47.6808913011582,-37.7267114902632,
-232.850050000001));
#228228=CARTESIAN_POINT('Ctrl Pts',(47.632174582744,-39.0083318774292,-232.85005));
#228229=CARTESIAN_POINT('Ctrl Pts',(47.5799752941153,-40.2889415902927,
-232.85005));
#228230=CARTESIAN_POINT('',(59.8539589593084,-46.7516609733785,-214.560268061993));
#228231=CARTESIAN_POINT('Ctrl Pts',(59.8539609358748,-46.7516610380391,
-214.560271423235));
#228232=CARTESIAN_POINT('Ctrl Pts',(59.8127437126661,-48.0499861503362,
-214.559533037022));
#228233=CARTESIAN_POINT('Ctrl Pts',(59.7691506214273,-49.3482347291554,
-214.558748583908));
#228234=CARTESIAN_POINT('Ctrl Pts',(59.6772124392584,-51.9445894630818,
-214.557078958964));
#228235=CARTESIAN_POINT('Ctrl Pts',(59.6288676637839,-53.2426846405684,
-214.556193992093));
#228236=CARTESIAN_POINT('Ctrl Pts',(59.5781472511379,-54.5406860123126,
-214.555282751789));
#228237=CARTESIAN_POINT('Ctrl Pts',(47.8511937435036,-32.6021335774055,
-232.85005));
#228238=CARTESIAN_POINT('Ctrl Pts',(49.7758731984242,-34.86623842913,-229.917938358392));
#228239=CARTESIAN_POINT('Ctrl Pts',(52.0064725897652,-37.4944438140806,
-226.519199308918));
#228240=CARTESIAN_POINT('Ctrl Pts',(55.7540093783891,-41.9130969187513,
-220.808621196108));
#228241=CARTESIAN_POINT('Ctrl Pts',(57.9042257787852,-44.4502782671364,
-217.531776078052));
#228242=CARTESIAN_POINT('Ctrl Pts',(59.8539550780058,-46.7516786353963,
-214.56027919439));
#228243=CARTESIAN_POINT('Ctrl Pts',(47.7752156818158,9.29411691894321,-232.968782926844));
#228244=CARTESIAN_POINT('Ctrl Pts',(51.8633248967382,11.8855265874929,-226.79842796189));
#228245=CARTESIAN_POINT('Ctrl Pts',(55.9515262957967,14.4763668580276,-220.627916411389));
#228246=CARTESIAN_POINT('Ctrl Pts',(60.0397300597283,17.0670490879089,-214.457361414306));
#228247=CARTESIAN_POINT('Ctrl Pts',(47.6990097155228,11.9175493678758,-232.966275794525));
#228248=CARTESIAN_POINT('Ctrl Pts',(51.7765308861555,14.9186157818217,-226.796020622489));
#228249=CARTESIAN_POINT('Ctrl Pts',(55.8541462985605,17.9190127102163,-220.625556640966));
#228250=CARTESIAN_POINT('Ctrl Pts',(59.9317344440901,20.9192322601435,-214.455037317351));
#228251=CARTESIAN_POINT('Ctrl Pts',(47.6093150514154,14.5106669763354,-232.963237198889));
#228252=CARTESIAN_POINT('Ctrl Pts',(51.673625611954,17.943733161272,-226.793068881834));
#228253=CARTESIAN_POINT('Ctrl Pts',(55.7379386239558,21.3761434795959,-220.622650915033));
#228254=CARTESIAN_POINT('Ctrl Pts',(59.8021028749556,24.8083979649139,-214.45217527183));
#228255=CARTESIAN_POINT('Ctrl Pts',(47.5077687575999,17.0588630313157,-232.959797430566));
#228256=CARTESIAN_POINT('Ctrl Pts',(51.5543587613359,20.962467251341,-226.789554159174));
#228257=CARTESIAN_POINT('Ctrl Pts',(55.6010831372117,24.8656613676635,-220.619139657106));
#228258=CARTESIAN_POINT('Ctrl Pts',(59.6478359854379,28.7687682426261,-214.448688656128));
#228259=CARTESIAN_POINT('',(59.8522817881067,20.867066521038,-214.564623195848));
#228260=CARTESIAN_POINT('Ctrl Pts',(59.5744430045609,28.6979747791773,-214.56059791914));
#228261=CARTESIAN_POINT('Ctrl Pts',(59.6255523742396,27.3929948773228,-214.561350802779));
#228262=CARTESIAN_POINT('Ctrl Pts',(59.6742602842766,26.0879255239846,-214.562076913704));
#228263=CARTESIAN_POINT('Ctrl Pts',(59.7668739927674,23.4776073684025,-214.563426526322));
#228264=CARTESIAN_POINT('Ctrl Pts',(59.8107792367937,22.1723757799868,-214.564049821487));
#228265=CARTESIAN_POINT('Ctrl Pts',(59.8522829924889,20.8670665606092,-214.564626087295));
#228266=CARTESIAN_POINT('',(47.852464780151,9.39110652846466,-232.850060330938));
#228267=CARTESIAN_POINT('Ctrl Pts',(47.5797436947461,17.1282946781069,-232.85005));
#228268=CARTESIAN_POINT('Ctrl Pts',(47.6322830986107,15.8393171716267,-232.85005));
#228269=CARTESIAN_POINT('Ctrl Pts',(47.6812964150144,14.5493107491212,-232.850050000002));
#228270=CARTESIAN_POINT('Ctrl Pts',(47.7721850391674,11.9708027192356,-232.850050000002));
#228271=CARTESIAN_POINT('Ctrl Pts',(47.814119381983,10.6806307165504,-232.85005));
#228272=CARTESIAN_POINT('Ctrl Pts',(47.8524795676142,9.39114590592673,-232.85005));
#228273=CARTESIAN_POINT('Ctrl Pts',(59.8522793526707,20.8670811307954,-214.564630777766));
#228274=CARTESIAN_POINT('Ctrl Pts',(57.9231697045554,19.0197027185266,-217.504721750272));
#228275=CARTESIAN_POINT('Ctrl Pts',(55.7588763923175,16.9478031006038,-220.803046854349));
#228276=CARTESIAN_POINT('Ctrl Pts',(52.0105370813373,13.3623506098877,-226.514897692767));
#228277=CARTESIAN_POINT('Ctrl Pts',(49.77648563263,11.2269580610392,-229.918931538715));
#228278=CARTESIAN_POINT('Ctrl Pts',(47.8524795676142,9.39114590592673,-232.85005));
#228279=CARTESIAN_POINT('Origin',(-1004.,-12.967500020028,-205.306318983907));
#228280=CARTESIAN_POINT('Ctrl Pts',(59.8522836403995,20.8670540894923,-214.564611698659));
#228281=CARTESIAN_POINT('Ctrl Pts',(59.8645512089436,20.5617173212634,-214.418212675891));
#228282=CARTESIAN_POINT('Ctrl Pts',(59.8766484531353,20.2499789990107,-214.285665596515));
#228283=CARTESIAN_POINT('Ctrl Pts',(59.8885301586884,19.9332173750779,-214.16622369325));
#228284=CARTESIAN_POINT('Ctrl Pts',(59.9748434130117,17.6321397659663,-213.298552017052));
#228285=CARTESIAN_POINT('Ctrl Pts',(60.0479352384608,15.1082501424152,-213.117891206253));
#228286=CARTESIAN_POINT('Ctrl Pts',(60.1030981576493,12.6512459219475,-213.346442200715));
#228287=CARTESIAN_POINT('Ctrl Pts',(60.111409107162,12.2810690290415,-213.38087612488));
#228288=CARTESIAN_POINT('Ctrl Pts',(60.119458031761,11.9059152175497,-213.425731330273));
#228289=CARTESIAN_POINT('Ctrl Pts',(60.1268679612506,11.5449119912611,-213.477614509765));
#228290=CARTESIAN_POINT('Ctrl Pts',(60.1377410433281,11.0151879614781,-213.553746147705));
#228291=CARTESIAN_POINT('Ctrl Pts',(60.1459757707366,10.5818923445005,-213.633116799817));
#228292=CARTESIAN_POINT('Ctrl Pts',(60.1532641850396,10.1814317298332,-213.714618736487));
#228293=CARTESIAN_POINT('Ctrl Pts',(60.1571763074449,9.96648086700407,-213.758365639347));
#228294=CARTESIAN_POINT('Ctrl Pts',(60.1608006466485,9.76108925215223,-213.803062347839));
#228295=CARTESIAN_POINT('Ctrl Pts',(60.1643187438617,9.5558923299876,-213.850313921784));
#228296=CARTESIAN_POINT('Ctrl Pts',(60.1647663228057,9.52978679163128,-213.856325355888));
#228297=CARTESIAN_POINT('Ctrl Pts',(60.1652121278246,9.50368446580734,-213.862379491625));
#228298=CARTESIAN_POINT('Ctrl Pts',(60.1656564875316,9.47756602057091,-213.868480820893));
#228299=CARTESIAN_POINT('Ctrl Pts',(60.1660491443594,9.45448655208617,-213.873872238157));
#228300=CARTESIAN_POINT('Ctrl Pts',(60.1664410470053,9.43139075002552,-213.879283604594));
#228301=CARTESIAN_POINT('Ctrl Pts',(60.1668339732078,9.40824978917476,-213.884647521255));
#228302=CARTESIAN_POINT('Ctrl Pts',(60.1675888932483,9.36378959540017,-213.894953090485));
#228303=CARTESIAN_POINT('Ctrl Pts',(60.1683459618837,9.3191789651953,-213.905157368098));
#228304=CARTESIAN_POINT('Ctrl Pts',(60.1691067978077,9.27432300489259,-213.91527730166));
#228305=CARTESIAN_POINT('Ctrl Pts',(60.1705954940518,9.18655519908565,-213.935078557895));
#228306=CARTESIAN_POINT('Ctrl Pts',(60.1720986097153,9.09784859398319,-213.95455921771));
#228307=CARTESIAN_POINT('Ctrl Pts',(60.1736282672258,9.00748926176066,-213.973818634937));
#228308=CARTESIAN_POINT('Ctrl Pts',(60.179215127641,8.67746442098616,-214.044160966466));
#228309=CARTESIAN_POINT('Ctrl Pts',(60.1853553620167,8.313505199782,-214.113465883361));
#228310=CARTESIAN_POINT('Ctrl Pts',(60.1914134093591,7.95361934628413,-214.171719071268));
#228311=CARTESIAN_POINT('Ctrl Pts',(60.2137472534459,6.62684950002414,-214.386477646556));
#228312=CARTESIAN_POINT('Ctrl Pts',(60.236418104203,5.27038456544939,-214.469588956065));
#228313=CARTESIAN_POINT('Ctrl Pts',(60.2591685013589,3.93463693001196,-214.381568911362));
#228314=CARTESIAN_POINT('Ctrl Pts',(60.2705679513422,3.26533923572927,-214.337465061647));
#228315=CARTESIAN_POINT('Ctrl Pts',(60.2826202444479,2.56566381509912,-214.241040503754));
#228316=CARTESIAN_POINT('Ctrl Pts',(60.292057365503,2.02427812018547,-214.137294054647));
#228317=CARTESIAN_POINT('Ctrl Pts',(60.2979421316388,1.68668276825177,-214.07260021562));
#228318=CARTESIAN_POINT('Ctrl Pts',(60.303185101195,1.38822157872398,-214.004609259439));
#228319=CARTESIAN_POINT('Ctrl Pts',(60.3084747241415,1.08920916466885,-213.927821213477));
#228320=CARTESIAN_POINT('Ctrl Pts',(60.3091581982912,1.05057365935606,-213.917899401477));
#228321=CARTESIAN_POINT('Ctrl Pts',(60.3098424352801,1.01193290476613,-213.907817486517));
#228322=CARTESIAN_POINT('Ctrl Pts',(60.3105289330055,0.97320334128505,-213.897551739282));
#228323=CARTESIAN_POINT('Ctrl Pts',(60.3112345718811,0.933393907674637,
-213.886999759185));
#228324=CARTESIAN_POINT('Ctrl Pts',(60.3119438877353,0.893513565114629,
-213.87616273221));
#228325=CARTESIAN_POINT('Ctrl Pts',(60.3126540303502,0.853391001986721,
-213.865328893283));
#228326=CARTESIAN_POINT('Ctrl Pts',(60.3142387111129,0.763857642626977,
-213.841153219592));
#228327=CARTESIAN_POINT('Ctrl Pts',(60.3158218668931,0.67301495760972,-213.817396808284));
#228328=CARTESIAN_POINT('Ctrl Pts',(60.3174186631855,0.579830242826636,
-213.793870865919));
#228329=CARTESIAN_POINT('Ctrl Pts',(60.3203923825933,0.406292017442597,
-213.750058419876));
#228330=CARTESIAN_POINT('Ctrl Pts',(60.3234151563689,0.224650876038405,
-213.706988287316));
#228331=CARTESIAN_POINT('Ctrl Pts',(60.3265631280972,0.028098083539605,
-213.664136837394));
#228332=CARTESIAN_POINT('Ctrl Pts',(60.3270570609419,-0.00274205363575723,
-213.657413226007));
#228333=CARTESIAN_POINT('Ctrl Pts',(60.3275540187065,-0.0339498222745532,
-213.650696726108));
#228334=CARTESIAN_POINT('Ctrl Pts',(60.3280542241711,-0.0655521844311571,
-213.643987602863));
#228335=CARTESIAN_POINT('Ctrl Pts',(60.3362065460935,-0.58060579349666,
-213.534642670864));
#228336=CARTESIAN_POINT('Ctrl Pts',(60.3443922093042,-1.15323528491378,
-213.43974077698));
#228337=CARTESIAN_POINT('Ctrl Pts',(60.3513604009398,-1.70571517675348,
-213.375438538189));
#228338=CARTESIAN_POINT('Ctrl Pts',(60.3631824450793,-2.64303751361287,
-213.266345111226));
#228339=CARTESIAN_POINT('Ctrl Pts',(60.3725736741095,-3.58991685287568,
-213.230688335639));
#228340=CARTESIAN_POINT('Ctrl Pts',(60.3794425164094,-4.53314772643593,
-213.26537659776));
#228341=CARTESIAN_POINT('Ctrl Pts',(60.3850857563185,-5.30807862114289,
-213.293875459232));
#228342=CARTESIAN_POINT('Ctrl Pts',(60.389031621255,-6.08056089768238,-213.369825212478));
#228343=CARTESIAN_POINT('Ctrl Pts',(60.3913108160445,-6.84593414020724,
-213.491429597462));
#228344=CARTESIAN_POINT('Ctrl Pts',(60.3924832204613,-7.23963764207369,
-213.553982179065));
#228345=CARTESIAN_POINT('Ctrl Pts',(60.393210861424,-7.65045599546225,-213.633390155684));
#228346=CARTESIAN_POINT('Ctrl Pts',(60.3934920217241,-7.992850845975,-213.708959851915));
#228347=CARTESIAN_POINT('Ctrl Pts',(60.3936603081493,-8.19778875984038,
-213.754191536544));
#228348=CARTESIAN_POINT('Ctrl Pts',(60.3936984229566,-8.38332920162743,
-213.798440546674));
#228349=CARTESIAN_POINT('Ctrl Pts',(60.393651903161,-8.56176805395002,-213.843419246263));
#228350=CARTESIAN_POINT('Ctrl Pts',(60.393645715246,-8.58550342183546,-213.849402169644));
#228351=CARTESIAN_POINT('Ctrl Pts',(60.3936379471922,-8.60911262131737,
-213.855400254366));
#228352=CARTESIAN_POINT('Ctrl Pts',(60.3936286330974,-8.63262423355807,
-213.86141955001));
#228353=CARTESIAN_POINT('Ctrl Pts',(60.3936240106306,-8.6442927477634,-213.864406849902));
#228354=CARTESIAN_POINT('Ctrl Pts',(60.3936189488047,-8.6559364513167,-213.867402543179));
#228355=CARTESIAN_POINT('Ctrl Pts',(60.3936136334464,-8.66756126923334,
-213.870397484014));
#228356=CARTESIAN_POINT('Ctrl Pts',(60.3936089954616,-8.67770465498889,
-213.873010758511));
#228357=CARTESIAN_POINT('Ctrl Pts',(60.3936043793879,-8.68783651798294,
-213.875611805623));
#228358=CARTESIAN_POINT('Ctrl Pts',(60.3935997841399,-8.69795915571535,
-213.878201268307));
#228359=CARTESIAN_POINT('Ctrl Pts',(60.3935813536366,-8.73855877228198,
-213.888587019024));
#228360=CARTESIAN_POINT('Ctrl Pts',(60.3935632575531,-8.77901001068321,
-213.898786760882));
#228361=CARTESIAN_POINT('Ctrl Pts',(60.3935454305537,-8.81946085570324,
-213.9088392194));
#228362=CARTESIAN_POINT('Ctrl Pts',(60.3935099629075,-8.89993969675756,
-213.928839054034));
#228363=CARTESIAN_POINT('Ctrl Pts',(60.3934755529649,-8.98041627708718,
-213.948259982409));
#228364=CARTESIAN_POINT('Ctrl Pts',(60.3934417749187,-9.06205842258955,
-213.967356720238));
#228365=CARTESIAN_POINT('Ctrl Pts',(60.3932951820256,-9.41637608343349,
-214.05023439862));
#228366=CARTESIAN_POINT('Ctrl Pts',(60.3931504054315,-9.80790367131028,
-214.132035127045));
#228367=CARTESIAN_POINT('Ctrl Pts',(60.3930198925774,-10.2869497542045,
-214.208627827912));
#228368=CARTESIAN_POINT('Ctrl Pts',(60.3927828642322,-11.1569598468437,
-214.34773015054));
#228369=CARTESIAN_POINT('Ctrl Pts',(60.3926877370732,-12.0336216853539,
-214.418420118334));
#228370=CARTESIAN_POINT('Ctrl Pts',(60.3927142613205,-12.9140676164264,
-214.419432663803));
#228371=CARTESIAN_POINT('Ctrl Pts',(60.3927287431374,-13.3947770850747,
-214.419985497517));
#228372=CARTESIAN_POINT('Ctrl Pts',(60.3927779546511,-13.8744234185498,
-214.399911341721));
#228373=CARTESIAN_POINT('Ctrl Pts',(60.3928549418663,-14.3538708453102,
-214.359724352712));
#228374=CARTESIAN_POINT('Ctrl Pts',(60.3929949672705,-15.2258964087699,
-214.286631705262));
#228375=CARTESIAN_POINT('Ctrl Pts',(60.393246335082,-16.1546220845523,-214.127978078364));
#228376=CARTESIAN_POINT('Ctrl Pts',(60.393432985145,-16.8311197866803,-213.976604381314));
#228377=CARTESIAN_POINT('Ctrl Pts',(60.3934565432232,-16.9165040912767,
-213.95749871722));
#228378=CARTESIAN_POINT('Ctrl Pts',(60.3934796365261,-16.9997898733473,
-213.938272995079));
#228379=CARTESIAN_POINT('Ctrl Pts',(60.3935024947112,-17.0821483260314,
-213.918723916564));
#228380=CARTESIAN_POINT('Ctrl Pts',(60.3935141968303,-17.1243112718209,
-213.908715875971));
#228381=CARTESIAN_POINT('Ctrl Pts',(60.3935258376588,-17.1662309100972,
-213.898622064381));
#228382=CARTESIAN_POINT('Ctrl Pts',(60.3935374491214,-17.2080633558844,
-213.888408909728));
#228383=CARTESIAN_POINT('Ctrl Pts',(60.393543288067,-17.2290992392794,-213.883273117969));
#228384=CARTESIAN_POINT('Ctrl Pts',(60.393549119591,-17.2501130687725,-213.878107082029));
#228385=CARTESIAN_POINT('Ctrl Pts',(60.393554947749,-17.2711246845471,-213.872906131118));
#228386=CARTESIAN_POINT('Ctrl Pts',(60.3935615224738,-17.2948278156789,
-213.867038956371));
#228387=CARTESIAN_POINT('Ctrl Pts',(60.3935675567513,-17.3185350501925,
-213.861156493035));
#228388=CARTESIAN_POINT('Ctrl Pts',(60.3935716543076,-17.3422928483403,
-213.855327567938));
#228389=CARTESIAN_POINT('Ctrl Pts',(60.3936041243251,-17.5305553343437,
-213.80913776858));
#228390=CARTESIAN_POINT('Ctrl Pts',(60.3935458845432,-17.7216373314267,
-213.76477468205));
#228391=CARTESIAN_POINT('Ctrl Pts',(60.3933602461435,-17.9298338823286,
-213.719802565618));
#228392=CARTESIAN_POINT('Ctrl Pts',(60.39306103192,-18.26540760757,-213.64731596304));
#228393=CARTESIAN_POINT('Ctrl Pts',(60.3923553391731,-18.6775129550453,
-213.567607646044));
#228394=CARTESIAN_POINT('Ctrl Pts',(60.3910564967462,-19.1075296034981,
-213.499906653704));
#228395=CARTESIAN_POINT('Ctrl Pts',(60.3887092138914,-19.8846605974914,
-213.377556647813));
#228396=CARTESIAN_POINT('Ctrl Pts',(60.3846983903845,-20.6691345815781,
-213.299096394904));
#228397=CARTESIAN_POINT('Ctrl Pts',(60.3789612071656,-21.4554845530463,
-213.268525469849));
#228398=CARTESIAN_POINT('Ctrl Pts',(60.3679012957514,-22.9713784495681,
-213.209592068205));
#228399=CARTESIAN_POINT('Ctrl Pts',(60.3502984944823,-24.5000103406799,
-213.329130293887));
#228400=CARTESIAN_POINT('Ctrl Pts',(60.3264857554362,-25.9796130521886,
-213.6570101885));
#228401=CARTESIAN_POINT('Ctrl Pts',(60.3234504544022,-26.1682112487886,
-213.698803540421));
#228402=CARTESIAN_POINT('Ctrl Pts',(60.3204565330099,-26.3472746066277,
-213.742037759624));
#228403=CARTESIAN_POINT('Ctrl Pts',(60.3175367315417,-26.516649532719,-213.78578065973));
#228404=CARTESIAN_POINT('Ctrl Pts',(60.3159762978469,-26.6071688178879,
-213.8091582407));
#228405=CARTESIAN_POINT('Ctrl Pts',(60.3144291687252,-26.6953838659096,
-213.832796220738));
#228406=CARTESIAN_POINT('Ctrl Pts',(60.3128853379364,-26.7820351410228,
-213.856805411057));
#228407=CARTESIAN_POINT('Ctrl Pts',(60.3124915944157,-26.8041349581722,
-213.862928791414));
#228408=CARTESIAN_POINT('Ctrl Pts',(60.3120980566698,-26.8261330430226,
-213.86907659917));
#228409=CARTESIAN_POINT('Ctrl Pts',(60.311704540284,-26.8480416873385,-213.875251256029));
#228410=CARTESIAN_POINT('Ctrl Pts',(60.3115355397114,-26.8574506308241,
-213.877903040255));
#228411=CARTESIAN_POINT('Ctrl Pts',(60.3113666893836,-26.8668457943141,
-213.880549365385));
#228412=CARTESIAN_POINT('Ctrl Pts',(60.311198146228,-26.8762313719384,-213.883178158384));
#228413=CARTESIAN_POINT('Ctrl Pts',(60.3110325273771,-26.8854541052786,
-213.88576134056));
#228414=CARTESIAN_POINT('Ctrl Pts',(60.3108671528631,-26.8946666125183,
-213.888331312463));
#228415=CARTESIAN_POINT('Ctrl Pts',(60.3107020058,-26.9038697912027,-213.890888412478));
#228416=CARTESIAN_POINT('Ctrl Pts',(60.3100371478399,-26.9409204446891,
-213.901182923738));
#228417=CARTESIAN_POINT('Ctrl Pts',(60.3093759742381,-26.9778199604901,
-213.911268999765));
#228418=CARTESIAN_POINT('Ctrl Pts',(60.308717400326,-27.0146264313552,-213.921167211129));
#228419=CARTESIAN_POINT('Ctrl Pts',(60.3034328975206,-27.3099674628848,
-214.000592048285));
#228420=CARTESIAN_POINT('Ctrl Pts',(60.2983146403093,-27.5991766863688,
-214.068573069905));
#228421=CARTESIAN_POINT('Ctrl Pts',(60.2928256973098,-27.9124538529063,
-214.131004935625));
#228422=CARTESIAN_POINT('Ctrl Pts',(60.2839179962428,-28.420853985854,-214.23232214678));
#228423=CARTESIAN_POINT('Ctrl Pts',(60.2740350908593,-28.9922802878306,
-214.323849549145));
#228424=CARTESIAN_POINT('Ctrl Pts',(60.2607587673069,-29.7735994708971,
-214.377595134823));
#228425=CARTESIAN_POINT('Ctrl Pts',(60.2541200133809,-30.1642939107765,
-214.404470324819));
#228426=CARTESIAN_POINT('Ctrl Pts',(60.2465848770941,-30.6109031181337,
-214.418187345506));
#228427=CARTESIAN_POINT('Ctrl Pts',(60.2393799757732,-31.0395548240251,
-214.41394184185));
#228428=CARTESIAN_POINT('Ctrl Pts',(60.2238711390327,-31.9622446748815,
-214.404803226323));
#228429=CARTESIAN_POINT('Ctrl Pts',(60.2084782565981,-32.8840406813232,
-214.32066535048));
#228430=CARTESIAN_POINT('Ctrl Pts',(60.1931159963307,-33.7953694742733,
-214.178967256063));
#228431=CARTESIAN_POINT('Ctrl Pts',(60.1870407676876,-34.1557676637223,
-214.122930689379));
#228432=CARTESIAN_POINT('Ctrl Pts',(60.1809699443647,-34.5145264949527,
-214.05797839233));
#228433=CARTESIAN_POINT('Ctrl Pts',(60.1749016871999,-34.8710225250701,
-213.985271624848));
#228434=CARTESIAN_POINT('Ctrl Pts',(60.1733510559208,-34.962118515264,-213.96669275042));
#228435=CARTESIAN_POINT('Ctrl Pts',(60.1718496862809,-35.0501934642886,
-213.948229706883));
#228436=CARTESIAN_POINT('Ctrl Pts',(60.1702373704645,-35.144617230878,-213.927869919498));
#228437=CARTESIAN_POINT('Ctrl Pts',(60.1694999096097,-35.1878059355439,
-213.918557509327));
#228438=CARTESIAN_POINT('Ctrl Pts',(60.1687161169395,-35.2336749127147,
-213.908549231463));
#228439=CARTESIAN_POINT('Ctrl Pts',(60.1678875012017,-35.2821213266032,
-213.897823414987));
#228440=CARTESIAN_POINT('Ctrl Pts',(60.1675039091746,-35.3045486801578,
-213.892858100551));
#228441=CARTESIAN_POINT('Ctrl Pts',(60.1671107108273,-35.3275283964064,
-213.887738985336));
#228442=CARTESIAN_POINT('Ctrl Pts',(60.1667080521215,-35.3510503623432,
-213.882463780837));
#228443=CARTESIAN_POINT('Ctrl Pts',(60.1665110501776,-35.36255855265,-213.879882871679));
#228444=CARTESIAN_POINT('Ctrl Pts',(60.1663118308306,-35.3741960784182,
-213.877262456815));
#228445=CARTESIAN_POINT('Ctrl Pts',(60.1661102633079,-35.385963215018,-213.874608964427));
#228446=CARTESIAN_POINT('Ctrl Pts',(60.1658814425207,-35.3993213464457,
-213.871596702288));
#228447=CARTESIAN_POINT('Ctrl Pts',(60.1656492765433,-35.4128496429707,
-213.868556305922));
#228448=CARTESIAN_POINT('Ctrl Pts',(60.1654137561779,-35.4265466933703,
-213.865488895693));
#228449=CARTESIAN_POINT('Ctrl Pts',(60.1622181589696,-35.6123915817958,
-213.823869532767));
#228450=CARTESIAN_POINT('Ctrl Pts',(60.1584061287036,-35.8293021918035,
-213.77724655845));
#228451=CARTESIAN_POINT('Ctrl Pts',(60.1539472537289,-36.0737459393782,
-213.728630617293));
#228452=CARTESIAN_POINT('Ctrl Pts',(60.1418239904513,-36.7383655856395,
-213.596448428404));
#228453=CARTESIAN_POINT('Ctrl Pts',(60.1249235460784,-37.60627443831,-213.44889762005));
#228454=CARTESIAN_POINT('Ctrl Pts',(60.1024025775608,-38.6088068260868,
-213.355157950907));
#228455=CARTESIAN_POINT('Ctrl Pts',(60.0855450330225,-39.3592290099679,
-213.284991312808));
#228456=CARTESIAN_POINT('Ctrl Pts',(60.0650589990151,-40.201475398557,-213.246373506945));
#228457=CARTESIAN_POINT('Ctrl Pts',(60.0426804011851,-41.0361098556587,
-213.267082162192));
#228458=CARTESIAN_POINT('Ctrl Pts',(59.9898111721685,-43.0079259896632,
-213.316006167403));
#228459=CARTESIAN_POINT('Ctrl Pts',(59.9251807248048,-44.9966985869325,
-213.673380572917));
#228460=CARTESIAN_POINT('Ctrl Pts',(59.8539617334964,-46.7516465273356,
-214.56025213689));
#228461=CARTESIAN_POINT('Ctrl Pts',(27.7161624394018,36.671894066742,-232.960596901862));
#228462=CARTESIAN_POINT('Ctrl Pts',(32.6826602701726,40.0809702013776,-226.781662197074));
#228463=CARTESIAN_POINT('Ctrl Pts',(37.6596812128995,43.4862512150987,-220.609204852275));
#228464=CARTESIAN_POINT('Ctrl Pts',(42.6390550299281,46.8908628802244,-214.438294417841));
#228465=CARTESIAN_POINT('Ctrl Pts',(25.7658626658342,36.9296719371149,-232.9601933409));
#228466=CARTESIAN_POINT('Ctrl Pts',(30.3639150200345,40.4303260414807,-226.78272680046));
#228467=CARTESIAN_POINT('Ctrl Pts',(34.9732667504195,43.9421267939794,-220.610591760459));
#228468=CARTESIAN_POINT('Ctrl Pts',(39.587510189865,47.4674439422847,-214.439830103812));
#228469=CARTESIAN_POINT('Ctrl Pts',(23.8044899907809,37.1610589494743,-232.959868581815));
#228470=CARTESIAN_POINT('Ctrl Pts',(28.0381839166385,40.7424490125755,-226.783608200302));
#228471=CARTESIAN_POINT('Ctrl Pts',(32.283433258083,44.3482400615009,-220.611766381486));
#228472=CARTESIAN_POINT('Ctrl Pts',(36.5352279127207,47.9802021638173,-214.441141334719));
#228473=CARTESIAN_POINT('Ctrl Pts',(21.8343359993853,37.3653585113446,-232.959639066595));
#228474=CARTESIAN_POINT('Ctrl Pts',(25.7068670980457,41.0171742382378,-226.784363424386));
#228475=CARTESIAN_POINT('Ctrl Pts',(29.5908265861273,44.7050007481411,-220.612769983421));
#228476=CARTESIAN_POINT('Ctrl Pts',(33.4823003440903,48.4301227180298,-214.442258946369));
#228477=CARTESIAN_POINT('Origin',(0.081845539031451,-172.6064917085,-232.850229531936));
#228478=CARTESIAN_POINT('Ctrl Pts',(33.4676030960081,48.3558410747994,-214.551991263944));
#228479=CARTESIAN_POINT('Ctrl Pts',(34.9861734114818,48.1318948267819,-214.55162202599));
#228480=CARTESIAN_POINT('Ctrl Pts',(36.5024600851346,47.8927123421817,-214.551192124635));
#228481=CARTESIAN_POINT('Ctrl Pts',(39.5300010313928,47.3839475975032,-214.550248247582));
#228482=CARTESIAN_POINT('Ctrl Pts',(41.0411838620008,47.1143772812309,-214.549734342172));
#228483=CARTESIAN_POINT('Ctrl Pts',(42.5495440258949,46.8296601163999,-214.549225394084));
#228484=CARTESIAN_POINT('Origin',(0.,-178.58000002,-205.306318983907));
#228485=CARTESIAN_POINT('Origin',(-296.501483394397,-25.4138432731711,-232.85005));
#228486=CARTESIAN_POINT('',(47.6963129678558,-31.8956500568736,-232.849931336942));
#228487=CARTESIAN_POINT('Origin',(-636.934816028482,-11.5034818258361,-232.85005));
#228488=CARTESIAN_POINT('Origin',(7.14692237356698E-14,623.509175991979,
-232.85005));
#228489=CARTESIAN_POINT('Origin',(0.0517782016034563,643.799970559412,-232.855108208931));
#228490=CARTESIAN_POINT('Ctrl Pts',(47.0825541999675,-41.7715518943956,
-232.85005));
#228491=CARTESIAN_POINT('Ctrl Pts',(46.9318448322354,-42.007890420054,-232.85005));
#228492=CARTESIAN_POINT('Ctrl Pts',(46.7904073409416,-42.2260229336685,
-232.85005));
#228493=CARTESIAN_POINT('Ctrl Pts',(46.4935676457423,-42.6770301148581,
-232.85005));
#228494=CARTESIAN_POINT('Ctrl Pts',(46.3418104287774,-42.9039683373476,
-232.85005));
#228495=CARTESIAN_POINT('Ctrl Pts',(45.8752836487346,-43.5906554858084,
-232.85005));
#228496=CARTESIAN_POINT('Ctrl Pts',(45.5551891811445,-44.0469551838861,
-232.85005));
#228497=CARTESIAN_POINT('Ctrl Pts',(44.5502158895002,-45.4345413296961,
-232.85005));
#228498=CARTESIAN_POINT('Ctrl Pts',(43.8423500925479,-46.3501756007396,
-232.85005));
#228499=CARTESIAN_POINT('Ctrl Pts',(41.5657247068443,-49.1071648985416,
-232.85005));
#228500=CARTESIAN_POINT('Ctrl Pts',(39.8686235209266,-50.9065939957913,
-232.85005));
#228501=CARTESIAN_POINT('Ctrl Pts',(36.3067467195521,-54.2094198597324,
-232.85005));
#228502=CARTESIAN_POINT('Ctrl Pts',(34.3620921324372,-55.7799933590787,
-232.85005));
#228503=CARTESIAN_POINT('Ctrl Pts',(29.6879676367398,-59.0721262304426,
-232.85005));
#228504=CARTESIAN_POINT('Ctrl Pts',(27.4993652273042,-60.2539775291619,
-232.85005));
#228505=CARTESIAN_POINT('Ctrl Pts',(26.5827048610814,-60.7443921296953,
-232.85005));
#228506=CARTESIAN_POINT('Ctrl Pts',(47.6963552853062,-31.896163686755,-232.85005));
#228507=CARTESIAN_POINT('Ctrl Pts',(47.7198209970693,-32.0141643773227,
-232.85005));
#228508=CARTESIAN_POINT('Ctrl Pts',(47.7444480612295,-32.1319277281135,
-232.850050000009));
#228509=CARTESIAN_POINT('Ctrl Pts',(47.7960571707317,-32.3672278207787,
-232.850050000009));
#228510=CARTESIAN_POINT('Ctrl Pts',(47.8230417127431,-32.4847512555908,
-232.85005));
#228511=CARTESIAN_POINT('Ctrl Pts',(47.8511636801433,-32.6020082275363,
-232.85005));
#228512=CARTESIAN_POINT('Ctrl Pts',(20.5341645416114,-61.1949426407512,
-232.965861592748));
#228513=CARTESIAN_POINT('Ctrl Pts',(24.8619705593691,-65.1326290782542,
-226.800008788317));
#228514=CARTESIAN_POINT('Ctrl Pts',(29.1902811104598,-69.0724625871147,
-220.634368994467));
#228515=CARTESIAN_POINT('Ctrl Pts',(33.5187281767876,-73.0145710177392,
-214.468761046583));
#228516=CARTESIAN_POINT('Ctrl Pts',(22.115564575717,-61.1500631726904,-232.964012351071));
#228517=CARTESIAN_POINT('Ctrl Pts',(26.7965523266534,-65.0759017171342,
-226.798067164761));
#228518=CARTESIAN_POINT('Ctrl Pts',(31.4781225651976,-69.0031581792391,
-220.632397171727));
#228519=CARTESIAN_POINT('Ctrl Pts',(36.1598241774431,-72.9319991467586,
-214.466766784373));
#228520=CARTESIAN_POINT('Ctrl Pts',(23.6900699183709,-61.1001919234539,
-232.961968408598));
#228521=CARTESIAN_POINT('Ctrl Pts',(28.7297131786069,-65.012574288375,-226.795902612053));
#228522=CARTESIAN_POINT('Ctrl Pts',(33.7700272351411,-68.9255509631158,
-220.630194103463));
#228523=CARTESIAN_POINT('Ctrl Pts',(38.8104606792061,-72.8393402290212,
-214.464534772546));
#228524=CARTESIAN_POINT('Ctrl Pts',(25.2562521239792,-61.0455007230049,
-232.959725695103));
#228525=CARTESIAN_POINT('Ctrl Pts',(30.6613188291079,-64.9426708583199,
-226.793511106062));
#228526=CARTESIAN_POINT('Ctrl Pts',(36.0671479350067,-68.8395145916166,
-220.627759071707));
#228527=CARTESIAN_POINT('Ctrl Pts',(41.4730739204624,-72.736318130574,-214.462066626483));
#228528=CARTESIAN_POINT('Origin',(0.,-12.9675000200281,-215.85005));
#228529=CARTESIAN_POINT('',(48.0827620446561,42.0414223951255,-215.85005));
#228530=CARTESIAN_POINT('Ctrl Pts',(49.1680521502591,41.0865353784011,-215.85005));
#228531=CARTESIAN_POINT('Ctrl Pts',(48.9895221708308,41.2470622045083,-215.85005));
#228532=CARTESIAN_POINT('Ctrl Pts',(48.810181579503,41.4065414287308,-215.850050000001));
#228533=CARTESIAN_POINT('Ctrl Pts',(48.4494381147294,41.7239310827547,-215.850050000001));
#228534=CARTESIAN_POINT('Ctrl Pts',(48.2659997961092,41.883627806787,-215.85005));
#228535=CARTESIAN_POINT('Ctrl Pts',(48.0827620446562,42.0414223951256,-215.85005));
#228536=CARTESIAN_POINT('',(54.6458252041307,35.5078877047659,-215.85005));
#228537=CARTESIAN_POINT('Origin',(48.892180948596,36.2913696007177,-215.85005));
#228538=CARTESIAN_POINT('Ctrl Pts',(54.6458252041307,35.5078877047659,-215.85005));
#228539=CARTESIAN_POINT('Ctrl Pts',(54.4879844434674,35.6891073117587,-215.85005));
#228540=CARTESIAN_POINT('Ctrl Pts',(54.3295470137666,35.869077059399,-215.85005));
#228541=CARTESIAN_POINT('Ctrl Pts',(54.0105884027086,36.2276517825792,-215.85005));
#228542=CARTESIAN_POINT('Ctrl Pts',(53.8480676261596,36.4085164872071,-215.85005));
#228543=CARTESIAN_POINT('Ctrl Pts',(53.6858060762413,36.5871897873468,-215.85005));
#228544=CARTESIAN_POINT('Ctrl Pts',(46.9910749481346,18.573078208412,-232.979487417878));
#228545=CARTESIAN_POINT('Ctrl Pts',(48.777813963045,21.1992978212187,-229.849984990042));
#228546=CARTESIAN_POINT('Ctrl Pts',(50.5669117785144,23.8226213730258,-226.720151765023));
#228547=CARTESIAN_POINT('Ctrl Pts',(52.3593746083135,26.4424369538029,-223.59005292932));
#228548=CARTESIAN_POINT('Ctrl Pts',(54.1518374381127,29.06225253458,-220.459954093617));
#228549=CARTESIAN_POINT('Ctrl Pts',(55.9476448491922,31.678562291835,-217.329579884935));
#228550=CARTESIAN_POINT('Ctrl Pts',(57.7483973817176,34.2905533170906,-214.199162765268));
#228551=CARTESIAN_POINT('Ctrl Pts',(45.9478671932277,20.2170814818308,-232.97487795833));
#228552=CARTESIAN_POINT('Ctrl Pts',(47.742137018698,22.773387445697,-229.848036259254));
#228553=CARTESIAN_POINT('Ctrl Pts',(49.5390933433176,25.3254669009981,-226.72056760043));
#228554=CARTESIAN_POINT('Ctrl Pts',(51.3405748716693,27.8719256903179,-223.592376908212));
#228555=CARTESIAN_POINT('Ctrl Pts',(53.1420564000211,30.4183844796377,-220.464186215995));
#228556=CARTESIAN_POINT('Ctrl Pts',(54.9479893176734,32.9592452374763,-217.335250628456));
#228557=CARTESIAN_POINT('Ctrl Pts',(56.7618317615675,35.4923074576668,-214.205720218898));
#228558=CARTESIAN_POINT('Ctrl Pts',(44.7615745302087,21.8990643607635,-232.969037860444));
#228559=CARTESIAN_POINT('Ctrl Pts',(46.6097944788647,24.3412907086997,-229.843779326009));
#228560=CARTESIAN_POINT('Ctrl Pts',(48.4600741151173,26.7788374139345,-226.718163107495));
#228561=CARTESIAN_POINT('Ctrl Pts',(50.314645520879,29.2097033728254,-223.592001377317));
#228562=CARTESIAN_POINT('Ctrl Pts',(52.1692169266407,31.6405693317163,-220.465839647138));
#228563=CARTESIAN_POINT('Ctrl Pts',(54.0277552893424,34.0649668687443,-217.339108786108));
#228564=CARTESIAN_POINT('Ctrl Pts',(55.8965060194204,36.4779337667532,-214.211679223185));
#228565=CARTESIAN_POINT('Ctrl Pts',(43.422273991912,23.5661942096002,-232.965337149737));
#228566=CARTESIAN_POINT('Ctrl Pts',(45.3530981989507,25.8862379834418,-229.841157038659));
#228567=CARTESIAN_POINT('Ctrl Pts',(47.2852714213136,28.2012404581192,-226.716776130434));
#228568=CARTESIAN_POINT('Ctrl Pts',(49.2205702668173,30.5094898312471,-223.59207508571));
#228569=CARTESIAN_POINT('Ctrl Pts',(51.155869112321,32.817739204375,-220.467374040986));
#228570=CARTESIAN_POINT('Ctrl Pts',(53.0939569308302,35.1194950308581,-217.342336617277));
#228571=CARTESIAN_POINT('Ctrl Pts',(55.0403804700997,37.4099350168284,-214.216875626567));
#228572=CARTESIAN_POINT('Ctrl Pts',(42.0829734536151,25.2333240584369,-232.96163643903));
#228573=CARTESIAN_POINT('Ctrl Pts',(44.0964019190368,27.4311852581839,-229.838534751308));
#228574=CARTESIAN_POINT('Ctrl Pts',(46.1104687275099,29.6236435023039,-226.715389153373));
#228575=CARTESIAN_POINT('Ctrl Pts',(48.1264950127556,31.8092762896688,-223.592148794104));
#228576=CARTESIAN_POINT('Ctrl Pts',(50.1425212980013,33.9949090770337,-220.468908434835));
#228577=CARTESIAN_POINT('Ctrl Pts',(52.1601585723181,36.1740231929721,-217.345564448446));
#228578=CARTESIAN_POINT('Ctrl Pts',(54.1842549207791,38.3419362669036,-214.22207202995));
#228579=CARTESIAN_POINT('Ctrl Pts',(40.5861557408476,26.890319992193,-232.960340269022));
#228580=CARTESIAN_POINT('Ctrl Pts',(42.7119476104226,28.9566971003925,-229.837640649106));
#228581=CARTESIAN_POINT('Ctrl Pts',(44.8377162696882,31.0173031877438,-226.714988934497));
#228582=CARTESIAN_POINT('Ctrl Pts',(46.9640447743127,33.0713690029734,-223.592432090741));
#228583=CARTESIAN_POINT('Ctrl Pts',(49.0903732789372,35.1254348182031,-220.469875246985));
#228584=CARTESIAN_POINT('Ctrl Pts',(51.2170775857911,37.1731632837144,-217.347402715892));
#228585=CARTESIAN_POINT('Ctrl Pts',(53.3465595646389,39.2117870653358,-214.225170223039));
#228586=CARTESIAN_POINT('Ctrl Pts',(38.9866932910313,28.4456556381462,-232.962790912271));
#228587=CARTESIAN_POINT('Ctrl Pts',(41.2391357104746,30.3925039299732,-229.839958591048));
#228588=CARTESIAN_POINT('Ctrl Pts',(43.490849558744,32.3336071411576,-226.717133201801));
#228589=CARTESIAN_POINT('Ctrl Pts',(45.7416073381742,34.2690638917383,-223.59431099442));
#228590=CARTESIAN_POINT('Ctrl Pts',(47.9923651176044,36.2045206423189,-220.471488787039));
#228591=CARTESIAN_POINT('Ctrl Pts',(50.2421837638693,38.1343124474224,-217.348670714219));
#228592=CARTESIAN_POINT('Ctrl Pts',(52.490668536736,40.0587201499459,-214.225843430884));
#228593=CARTESIAN_POINT('Ctrl Pts',(37.3872308412151,30.0009912840992,-232.96524155552));
#228594=CARTESIAN_POINT('Ctrl Pts',(39.7663238105267,31.8283107595538,-229.842276532991));
#228595=CARTESIAN_POINT('Ctrl Pts',(42.1439828477997,33.6499110945716,-226.719277469106));
#228596=CARTESIAN_POINT('Ctrl Pts',(44.5191699020356,35.4667587805032,-223.596189898099));
#228597=CARTESIAN_POINT('Ctrl Pts',(46.8943569562715,37.2836064664347,-220.473102327093));
#228598=CARTESIAN_POINT('Ctrl Pts',(49.2672899419476,39.0954616111304,-217.349938712546));
#228599=CARTESIAN_POINT('Ctrl Pts',(51.6347775088331,40.905653234556,-214.226516638731));
#228600=CARTESIAN_POINT('Ctrl Pts',(35.6766644639054,31.4635880480613,-232.97088766827));
#228601=CARTESIAN_POINT('Ctrl Pts',(38.1975797295179,33.1824169992017,-229.847322479379));
#228602=CARTESIAN_POINT('Ctrl Pts',(40.7164614543727,34.8957848961753,-226.723562794745));
#228603=CARTESIAN_POINT('Ctrl Pts',(43.231587976361,36.605521367383,-223.599359264791));
#228604=CARTESIAN_POINT('Ctrl Pts',(45.7467144983492,38.3152578385909,-220.475155734837));
#228605=CARTESIAN_POINT('Ctrl Pts',(48.2584201480868,40.0209091135152,-217.350539684011));
#228606=CARTESIAN_POINT('Ctrl Pts',(50.7614553754203,41.7288322173994,-214.224825362635));
#228607=CARTESIAN_POINT('Ctrl Pts',(33.949434877602,32.770352829909,-232.980025784665));
#228608=CARTESIAN_POINT('Ctrl Pts',(36.6048862944054,34.4080943544835,-229.854970428563));
#228609=CARTESIAN_POINT('Ctrl Pts',(39.2576627597897,36.0413528393508,-226.72942775857));
#228610=CARTESIAN_POINT('Ctrl Pts',(41.9056884039802,37.6725825561817,-223.603007266837));
#228611=CARTESIAN_POINT('Ctrl Pts',(44.5537140481708,39.3038122730124,-220.476586775106));
#228612=CARTESIAN_POINT('Ctrl Pts',(47.1972705274053,40.9325619164058,-217.349301164816));
#228613=CARTESIAN_POINT('Ctrl Pts',(49.8308862116777,42.5662844245855,-214.220385090245));
#228614=CARTESIAN_POINT('Ctrl Pts',(33.0858200844503,33.4237352208328,-232.984594842862));
#228615=CARTESIAN_POINT('Ctrl Pts',(35.8085395768491,35.0209330321244,-229.858794403155));
#228616=CARTESIAN_POINT('Ctrl Pts',(38.5282634124981,36.6141368109387,-226.732360240482));
#228617=CARTESIAN_POINT('Ctrl Pts',(41.2427386177898,38.2061131505809,-223.604831267861));
#228618=CARTESIAN_POINT('Ctrl Pts',(43.9572138230815,39.7980894902232,-220.47730229524));
#228619=CARTESIAN_POINT('Ctrl Pts',(46.6666957170646,41.3883883178512,-217.348681905218));
#228620=CARTESIAN_POINT('Ctrl Pts',(49.3656016298064,42.9850105281785,-214.21816495405));
#228621=CARTESIAN_POINT('Ctrl Pts',(32.216695486199,34.0396911750287,-232.98970214378));
#228622=CARTESIAN_POINT('Ctrl Pts',(35.0051317985077,35.6029084387718,-229.862997039215));
#228623=CARTESIAN_POINT('Ctrl Pts',(37.7903020546954,37.1627315739784,-226.7354929936));
#228624=CARTESIAN_POINT('Ctrl Pts',(40.5699478215597,38.7220617966288,-223.60669458574));
#228625=CARTESIAN_POINT('Ctrl Pts',(43.3495935884239,40.2813920192791,-220.477896177879));
#228626=CARTESIAN_POINT('Ctrl Pts',(46.1238945065879,41.8398602062025,-217.347790101788));
#228627=CARTESIAN_POINT('Ctrl Pts',(48.8878519146755,43.4051188865968,-214.215677456544));
#228628=CARTESIAN_POINT('Ctrl Pts',(31.3497500510356,34.6184286458191,-232.99511552399));
#228629=CARTESIAN_POINT('Ctrl Pts',(34.1981927402684,36.1561028618858,-229.86725871849));
#228630=CARTESIAN_POINT('Ctrl Pts',(37.0431800113206,37.6911082882257,-226.738459395528));
#228631=CARTESIAN_POINT('Ctrl Pts',(39.8826292444588,39.2262665988641,-223.608273410873));
#228632=CARTESIAN_POINT('Ctrl Pts',(42.722078477597,40.7614249095024,-220.47808742622));
#228633=CARTESIAN_POINT('Ctrl Pts',(45.5561045113048,42.2964603802716,-217.34649079771));
#228634=CARTESIAN_POINT('Ctrl Pts',(48.3805813576904,43.8381246360801,-214.213011833879));
#228635=CARTESIAN_POINT('Ctrl Pts',(30.916277333454,34.9077973812142,-232.997822214095));
#228636=CARTESIAN_POINT('Ctrl Pts',(33.7947232111487,36.4327000734428,-229.869389558127));
#228637=CARTESIAN_POINT('Ctrl Pts',(36.6696189896331,37.9552966453494,-226.739942596491));
#228638=CARTESIAN_POINT('Ctrl Pts',(39.5389699559083,39.4783689999817,-223.60906282344));
#228639=CARTESIAN_POINT('Ctrl Pts',(42.4083209221835,41.001441354614,-220.47818305039));
#228640=CARTESIAN_POINT('Ctrl Pts',(45.2722095136632,42.5247604673061,-217.345841145671));
#228641=CARTESIAN_POINT('Ctrl Pts',(48.1269460791978,44.0546275108218,-214.211679022545));
#228642=CARTESIAN_POINT('Ctrl Pts',(30.4833514870981,35.1878641409515,-233.000603030011));
#228643=CARTESIAN_POINT('Ctrl Pts',(33.3903722647552,36.7021050405422,-229.871531357437));
#228644=CARTESIAN_POINT('Ctrl Pts',(36.2937694734405,38.2144329802205,-226.741379545545));
#228645=CARTESIAN_POINT('Ctrl Pts',(39.1916813033838,39.727537057445,-223.60977593002));
#228646=CARTESIAN_POINT('Ctrl Pts',(42.089593133327,41.2406411346694,-220.478172314495));
#228647=CARTESIAN_POINT('Ctrl Pts',(44.9820725042275,42.7543411128055,-217.345083947855));
#228648=CARTESIAN_POINT('Ctrl Pts',(47.8659336123358,44.2743593115718,-214.210293173543));
#228649=CARTESIAN_POINT('Ctrl Pts',(30.0519450660363,35.4586704870703,-233.00341455534));
#228650=CARTESIAN_POINT('Ctrl Pts',(32.9855855312196,36.9645966036217,-229.87362179639));
#228651=CARTESIAN_POINT('Ctrl Pts',(35.9155640960709,38.4690265434296,-226.742700788357));
#228652=CARTESIAN_POINT('Ctrl Pts',(38.8401926838925,39.9745043257835,-223.610348870589));
#228653=CARTESIAN_POINT('Ctrl Pts',(41.7648212717142,41.4799821081373,-220.477996952821));
#228654=CARTESIAN_POINT('Ctrl Pts',(44.6841307999907,42.986369790773,-217.344180493823));
#228655=CARTESIAN_POINT('Ctrl Pts',(47.5954455649975,44.4987574479709,-214.208828131933));
#228656=CARTESIAN_POINT('Ctrl Pts',(29.8362418555055,35.5940736601297,-233.004820318005));
#228657=CARTESIAN_POINT('Ctrl Pts',(32.7831921644516,37.0958423851614,-229.874667015866));
#228658=CARTESIAN_POINT('Ctrl Pts',(35.7264614073862,38.5963233250342,-226.743361409764));
#228659=CARTESIAN_POINT('Ctrl Pts',(38.664448374147,40.0979879599528,-223.610635340874));
#228660=CARTESIAN_POINT('Ctrl Pts',(41.6024353409078,41.5996525948713,-220.477909271983));
#228661=CARTESIAN_POINT('Ctrl Pts',(44.5351599478724,43.1023841297568,-217.343728766806));
#228662=CARTESIAN_POINT('Ctrl Pts',(47.4602015413284,44.6109565161706,-214.208095611128));
#228663=CARTESIAN_POINT('Ctrl Pts',(29.6209186123181,35.727161889339,-233.006233607583));
#228664=CARTESIAN_POINT('Ctrl Pts',(32.5806898644201,37.2253600131119,-229.875699165609));
#228665=CARTESIAN_POINT('Ctrl Pts',(35.5367698105028,38.7224845297496,-226.743992894479));
#228666=CARTESIAN_POINT('Ctrl Pts',(38.4876542293243,40.2209213875052,-223.610886590344));
#228667=CARTESIAN_POINT('Ctrl Pts',(41.4385386481458,41.7193582452608,-220.477780286209));
#228668=CARTESIAN_POINT('Ctrl Pts',(44.3842382725856,43.2190102201042,-217.343240349689));
#228669=CARTESIAN_POINT('Ctrl Pts',(47.3225890909698,44.7243219112958,-214.207343022243));
#228670=CARTESIAN_POINT('Ctrl Pts',(29.4060975644904,35.8579413159883,-233.007648088092));
#228671=CARTESIAN_POINT('Ctrl Pts',(32.3781342806196,37.3531855340767,-229.87670909491));
#228672=CARTESIAN_POINT('Ctrl Pts',(35.3464811752108,38.8475743913038,-226.744585492565));
#228673=CARTESIAN_POINT('Ctrl Pts',(38.3097398506307,40.3433960477796,-223.611093856846));
#228674=CARTESIAN_POINT('Ctrl Pts',(41.2729985260507,41.8392177042554,-220.477602221127));
#228675=CARTESIAN_POINT('Ctrl Pts',(44.231172512421,43.3363922589179,-217.342710032053));
#228676=CARTESIAN_POINT('Ctrl Pts',(47.182348866173,44.8390312087872,-214.206565980874));
#228677=CARTESIAN_POINT('Ctrl Pts',(29.2986870405764,35.9233310293129,-233.008355328346));
#228678=CARTESIAN_POINT('Ctrl Pts',(32.2768564887194,37.4170982945592,-229.877214059559));
#228679=CARTESIAN_POINT('Ctrl Pts',(35.2513368575648,38.9101193220809,-226.744881791608));
#228680=CARTESIAN_POINT('Ctrl Pts',(38.220782661284,40.4046333779168,-223.611197490097));
#228681=CARTESIAN_POINT('Ctrl Pts',(41.1902284650032,41.8991474337527,-220.477513188586));
#228682=CARTESIAN_POINT('Ctrl Pts',(44.1546396323386,43.3950832783248,-217.342444873235));
#228683=CARTESIAN_POINT('Ctrl Pts',(47.1122287537746,44.8963858575329,-214.206177460189));
#228684=CARTESIAN_POINT('Ctrl Pts',(29.1914020723121,35.98814355176,-233.009062856813));
#228685=CARTESIAN_POINT('Ctrl Pts',(32.1755653742122,37.4805880407614,-229.877713455064));
#228686=CARTESIAN_POINT('Ctrl Pts',(35.1560432829324,38.9723964221036,-226.745168359446));
#228687=CARTESIAN_POINT('Ctrl Pts',(38.1315454230114,40.4657560119625,-223.611290121901));
#228688=CARTESIAN_POINT('Ctrl Pts',(41.1070475630904,41.9591156018214,-220.477411884356));
#228689=CARTESIAN_POINT('Ctrl Pts',(44.0775707523758,43.4539632651818,-217.342169238531));
#228690=CARTESIAN_POINT('Ctrl Pts',(47.0414517295384,44.9540764555871,-214.205782818867));
#228691=CARTESIAN_POINT('Ctrl Pts',(29.0842579792521,36.0523797092374,-233.009769824147));
#228692=CARTESIAN_POINT('Ctrl Pts',(32.0742678787604,37.5436593534111,-229.878206054095));
#228693=CARTESIAN_POINT('Ctrl Pts',(35.0605994496261,39.0344137463011,-226.745443927067));
#228694=CARTESIAN_POINT('Ctrl Pts',(38.0420193927072,40.5267753480634,-223.611370632498));
#228695=CARTESIAN_POINT('Ctrl Pts',(41.0234393357883,42.0191369498257,-220.477297337928));
#228696=CARTESIAN_POINT('Ctrl Pts',(43.9999418407127,43.5130501216253,-217.341882483075));
#228697=CARTESIAN_POINT('Ctrl Pts',(46.9699855652835,45.0121250312964,-214.205381478311));
#228698=CARTESIAN_POINT('Ctrl Pts',(29.030685932722,36.0844977879761,-233.010123307814));
#228699=CARTESIAN_POINT('Ctrl Pts',(32.0236191310345,37.5751950097359,-229.878452353611));
#228700=CARTESIAN_POINT('Ctrl Pts',(35.012877532973,39.0654224083999,-226.745581710878));
#228701=CARTESIAN_POINT('Ctrl Pts',(37.997256377555,40.5572850161139,-223.611410887796));
#228702=CARTESIAN_POINT('Ctrl Pts',(40.9816352221372,42.0491476238279,-220.477240064714));
#228703=CARTESIAN_POINT('Ctrl Pts',(43.9611273848811,43.5425935498471,-217.341739105347));
#228704=CARTESIAN_POINT('Ctrl Pts',(46.934252483156,45.041149319151,-214.205180808032));
#228705=CARTESIAN_POINT('Ctrl Pts',(28.9771491054224,36.1164717760765,-233.010476650599));
#228706=CARTESIAN_POINT('Ctrl Pts',(31.9729687878842,37.6066260584536,-229.878696953144));
#228707=CARTESIAN_POINT('Ctrl Pts',(34.9651180517945,39.0963661267734,-226.745716744168));
#228708=CARTESIAN_POINT('Ctrl Pts',(37.952421164982,40.5877688592974,-223.611448112616));
#228709=CARTESIAN_POINT('Ctrl Pts',(40.9397242781695,42.0791715918215,-220.477179481064));
#228710=CARTESIAN_POINT('Ctrl Pts',(43.9221729224182,43.5721886941534,-217.341592947587));
#228711=CARTESIAN_POINT('Ctrl Pts',(46.8983471180018,45.0702630995771,-214.204978462744));
#228712=CARTESIAN_POINT('Ctrl Pts',(28.9236494148868,36.1483017803918,-233.01082974273));
#228713=CARTESIAN_POINT('Ctrl Pts',(31.9223177157407,37.6379530768432,-229.878939694123));
#228714=CARTESIAN_POINT('Ctrl Pts',(34.9173208817124,39.1272459095225,-226.745848865747));
#228715=CARTESIAN_POINT('Ctrl Pts',(37.9075126656038,40.6182282999103,-223.611482166239));
#228716=CARTESIAN_POINT('Ctrl Pts',(40.8977044494953,42.109210690298,-220.477115466732));
#228717=CARTESIAN_POINT('Ctrl Pts',(43.8830754570229,43.6018377843273,-217.341443930439));
#228718=CARTESIAN_POINT('Ctrl Pts',(46.8622654530928,45.0994691148216,-214.204774369339));
#228719=CARTESIAN_POINT('Ctrl Pts',(28.8701497243513,36.1801317847072,-233.011182834863));
#228720=CARTESIAN_POINT('Ctrl Pts',(31.871666643597,37.6692800952327,-229.879182435101));
#228721=CARTESIAN_POINT('Ctrl Pts',(34.8695237116303,39.1581256922717,-226.745980987327));
#228722=CARTESIAN_POINT('Ctrl Pts',(37.8626041662257,40.6486877405231,-223.611516219864));
#228723=CARTESIAN_POINT('Ctrl Pts',(40.8556846208211,42.1392497887745,-220.4770514524));
#228724=CARTESIAN_POINT('Ctrl Pts',(43.8439779916275,43.6314868745012,-217.341294913291));
#228725=CARTESIAN_POINT('Ctrl Pts',(46.8261837881837,45.128675130066,-214.204570275934));
#228726=CARTESIAN_POINT('Ctrl Pts',(28.818156654463,36.2102288606094,-233.012213872822));
#228727=CARTESIAN_POINT('Ctrl Pts',(31.8223098653572,37.6990724529492,-229.880007982271));
#228728=CARTESIAN_POINT('Ctrl Pts',(34.8228081429799,39.18767633626,-226.746603037528));
#228729=CARTESIAN_POINT('Ctrl Pts',(37.8185924512592,40.6780007601943,-223.611963071785));
#228730=CARTESIAN_POINT('Ctrl Pts',(40.8143767595385,42.1683251841286,-220.477323106043));
#228731=CARTESIAN_POINT('Ctrl Pts',(43.8054348260158,43.6603350812977,-217.341420791685));
#228732=CARTESIAN_POINT('Ctrl Pts',(46.7905804536569,45.1571425161278,-214.2046126078));
#228733=CARTESIAN_POINT('Ctrl Pts',(28.7632636728437,36.243359951239,-233.011888154992));
#228734=CARTESIAN_POINT('Ctrl Pts',(31.7703631777874,37.7316226214323,-229.879662179404));
#228735=CARTESIAN_POINT('Ctrl Pts',(34.7738161809111,39.2196944596949,-226.746236332649));
#228736=CARTESIAN_POINT('Ctrl Pts',(37.7725662199917,40.7095348345317,-223.611574672556));
#228737=CARTESIAN_POINT('Ctrl Pts',(40.7713162590722,42.1993752093685,-220.476913012461));
#228738=CARTESIAN_POINT('Ctrl Pts',(43.7653510607838,43.6909491168262,-217.340988222568));
#228739=CARTESIAN_POINT('Ctrl Pts',(46.7534875501661,45.1873665995436,-214.204156771482));
#228740=CARTESIAN_POINT('',(46.7405472321667,30.7185439590785,-225.418940742796));
#228741=CARTESIAN_POINT('Ctrl Pts',(54.6458252041307,35.5078877047659,-215.85005));
#228742=CARTESIAN_POINT('Ctrl Pts',(54.5943354599542,35.0871229746991,-216.179655766508));
#228743=CARTESIAN_POINT('Ctrl Pts',(54.4989704544248,34.6852639063571,-216.528294351258));
#228744=CARTESIAN_POINT('Ctrl Pts',(54.2127819562334,33.8548754267304,-217.317195844125));
#228745=CARTESIAN_POINT('Ctrl Pts',(54.0059798594749,33.4340164710517,-217.764515858296));
#228746=CARTESIAN_POINT('Ctrl Pts',(53.2992114884488,32.3315417080536,-219.068798253937));
#228747=CARTESIAN_POINT('Ctrl Pts',(52.6935858718955,31.7306722066013,-219.95737939011));
#228748=CARTESIAN_POINT('Ctrl Pts',(51.1420742506923,30.731323527294,-221.883755596029));
#228749=CARTESIAN_POINT('Ctrl Pts',(50.1720764170543,30.4163412364309,-222.887463984116));
#228750=CARTESIAN_POINT('Ctrl Pts',(48.7953703105921,30.3299008816871,-224.056790691687));
#228751=CARTESIAN_POINT('Ctrl Pts',(48.3973293063562,30.3422930432357,-224.368248809743));
#228752=CARTESIAN_POINT('Ctrl Pts',(47.582248831158,30.4570387035492,-224.938952843229));
#228753=CARTESIAN_POINT('Ctrl Pts',(47.1618710045203,30.5599614053015,-225.200460249291));
#228754=CARTESIAN_POINT('Ctrl Pts',(46.7405472321717,30.7185439590994,-225.41894074279));
#228755=CARTESIAN_POINT('',(46.4511396589728,30.4281656954994,-225.850049999692));
#228756=CARTESIAN_POINT('Ctrl Pts',(46.4511396588546,30.4281656952997,-225.850049999478));
#228757=CARTESIAN_POINT('Ctrl Pts',(46.4993753881247,30.4765632101155,-225.778199403668));
#228758=CARTESIAN_POINT('Ctrl Pts',(46.547609928457,30.5249595320058,-225.706349252241));
#228759=CARTESIAN_POINT('Ctrl Pts',(46.6440796088716,30.6217527775478,-225.56264542894));
#228760=CARTESIAN_POINT('Ctrl Pts',(46.6923132704823,30.6701482177691,-225.490793959434));
#228761=CARTESIAN_POINT('Ctrl Pts',(46.7405472321751,30.7185439590791,-225.418940742802));
#228762=CARTESIAN_POINT('',(45.7333210481289,31.2122413341206,-225.850044625428));
#228763=CARTESIAN_POINT('Ctrl Pts',(46.4511396584396,30.4281656950207,-225.85005));
#228764=CARTESIAN_POINT('Ctrl Pts',(46.3327936010765,30.5600059656552,-225.85005));
#228765=CARTESIAN_POINT('Ctrl Pts',(46.2137942830087,30.6912801197937,-225.85005));
#228766=CARTESIAN_POINT('Ctrl Pts',(45.9745262547338,30.9526355221877,-225.85005));
#228767=CARTESIAN_POINT('Ctrl Pts',(45.8542372584541,31.0827388231335,-225.85005));
#228768=CARTESIAN_POINT('Ctrl Pts',(45.7333160885807,31.2122314446859,-225.85005));
#228769=CARTESIAN_POINT('Ctrl Pts',(45.7333215220983,31.2122476865619,-225.850034141972));
#228770=CARTESIAN_POINT('Ctrl Pts',(45.3379480310533,31.4554802421263,-225.979545398304));
#228771=CARTESIAN_POINT('Ctrl Pts',(44.9654369203883,31.7493278392119,-226.049149720515));
#228772=CARTESIAN_POINT('Ctrl Pts',(44.2902370695759,32.435117692196,-226.049169157732));
#228773=CARTESIAN_POINT('Ctrl Pts',(44.0028843799733,32.8110880152495,-225.979845479737));
#228774=CARTESIAN_POINT('Ctrl Pts',(43.7661192039793,33.2092653548652,-225.85004993015));
#228775=CARTESIAN_POINT('Ctrl Pts',(48.0827620446562,42.0414223951255,-215.85005));
#228776=CARTESIAN_POINT('Ctrl Pts',(47.691890257726,41.9918377457907,-216.158510565839));
#228777=CARTESIAN_POINT('Ctrl Pts',(47.3178589833685,41.9044704486236,-216.483755325416));
#228778=CARTESIAN_POINT('Ctrl Pts',(46.5278541131957,41.6412341609588,-217.232695618651));
#228779=CARTESIAN_POINT('Ctrl Pts',(46.1204261816246,41.4485202650666,-217.663837570769));
#228780=CARTESIAN_POINT('Ctrl Pts',(44.9817998525948,40.7494982164769,-219.000277705729));
#228781=CARTESIAN_POINT('Ctrl Pts',(44.3453100117888,40.117856186638,-219.946031814402));
#228782=CARTESIAN_POINT('Ctrl Pts',(43.3187329856903,38.5182399992516,-221.954309494373));
#228783=CARTESIAN_POINT('Ctrl Pts',(43.0024705252185,37.5284133108539,-222.985431128923));
#228784=CARTESIAN_POINT('Ctrl Pts',(42.9307447595918,36.1378442918464,-224.156404719666));
#228785=CARTESIAN_POINT('Ctrl Pts',(42.9463038154196,35.7490409902397,-224.457196959694));
#228786=CARTESIAN_POINT('Ctrl Pts',(43.0642975219611,34.9494394059176,-225.008393072079));
#228787=CARTESIAN_POINT('Ctrl Pts',(43.1679394115603,34.5354819113177,-225.26038854254));
#228788=CARTESIAN_POINT('Ctrl Pts',(43.3259173910694,34.1204116753624,-225.468974352254));
#228789=CARTESIAN_POINT('Ctrl Pts',(28.918632420916,36.3202559369514,-232.85005));
#228790=CARTESIAN_POINT('Ctrl Pts',(29.1405722429424,36.1874419307081,-232.85005));
#228791=CARTESIAN_POINT('Ctrl Pts',(29.3442027713421,36.0636271479844,-232.85005));
#228792=CARTESIAN_POINT('Ctrl Pts',(29.7663007847196,35.8033260589225,-232.85005));
#228793=CARTESIAN_POINT('Ctrl Pts',(29.9787466996505,35.6703265943621,-232.85005));
#228794=CARTESIAN_POINT('Ctrl Pts',(30.6209255013567,35.2622379995143,-232.85005));
#228795=CARTESIAN_POINT('Ctrl Pts',(31.0479818197507,34.9825440512594,-232.85005));
#228796=CARTESIAN_POINT('Ctrl Pts',(32.3437566649085,34.1080837663653,-232.85005));
#228797=CARTESIAN_POINT('Ctrl Pts',(33.2007785122792,33.4934899779854,-232.85005));
#228798=CARTESIAN_POINT('Ctrl Pts',(35.7754719960827,31.5304296840008,-232.85005));
#228799=CARTESIAN_POINT('Ctrl Pts',(37.4639373139647,30.0758667472212,-232.85005));
#228800=CARTESIAN_POINT('Ctrl Pts',(40.5990894760027,27.0270783922585,-232.85005));
#228801=CARTESIAN_POINT('Ctrl Pts',(42.1044452521521,25.3726646453478,-232.85005));
#228802=CARTESIAN_POINT('Ctrl Pts',(44.7627079511811,22.0795000960729,-232.85005));
#228803=CARTESIAN_POINT('Ctrl Pts',(45.9624973465495,20.4083241018545,-232.85005));
#228804=CARTESIAN_POINT('Ctrl Pts',(47.0649763530314,18.681697915047,-232.85005));
#228805=CARTESIAN_POINT('Origin',(0.,-12.9675000200281,-215.85005));
#228806=CARTESIAN_POINT('',(53.9390346875574,-61.9113848028035,-215.85005));
#228807=CARTESIAN_POINT('Ctrl Pts',(53.7300151844417,-62.1425230012532,
-215.85005));
#228808=CARTESIAN_POINT('Ctrl Pts',(53.7649393991663,-62.1040873964302,
-215.85005));
#228809=CARTESIAN_POINT('Ctrl Pts',(53.7998169861779,-62.0656105112122,
-215.85005));
#228810=CARTESIAN_POINT('Ctrl Pts',(53.8694902457069,-61.9885636960997,
-215.85005));
#228811=CARTESIAN_POINT('Ctrl Pts',(53.9042848508501,-61.9499949024173,
-215.85005));
#228812=CARTESIAN_POINT('Ctrl Pts',(53.9390346875573,-61.9113848028035,
-215.85005));
#228813=CARTESIAN_POINT('',(48.06997860106,-67.6025450092472,-215.850048906121));
#228814=CARTESIAN_POINT('Origin',(48.1334350484927,-61.7961505568785,-215.85005));
#228815=CARTESIAN_POINT('Ctrl Pts',(48.0699790998778,-67.6025411378175,
-215.85005));
#228816=CARTESIAN_POINT('Ctrl Pts',(48.2218940855867,-67.4735199039321,
-215.85005));
#228817=CARTESIAN_POINT('Ctrl Pts',(48.3737209284913,-67.3434180280897,
-215.850049999999));
#228818=CARTESIAN_POINT('Ctrl Pts',(48.673346523466,-67.0844676986175,-215.850049999999));
#228819=CARTESIAN_POINT('Ctrl Pts',(48.8227466277686,-66.9542303125478,
-215.85005));
#228820=CARTESIAN_POINT('Ctrl Pts',(48.9715866554311,-66.8233021636441,
-215.85005));
#228821=CARTESIAN_POINT('Ctrl Pts',(26.2545891898305,-60.7273783411365,
-233.020937743651));
#228822=CARTESIAN_POINT('Ctrl Pts',(29.704767491125,-62.4315344808983,-229.869275405273));
#228823=CARTESIAN_POINT('Ctrl Pts',(33.1518809533354,-64.139871089189,-226.716620552092));
#228824=CARTESIAN_POINT('Ctrl Pts',(36.5949698446713,-65.8547248151706,
-223.563151715778));
#228825=CARTESIAN_POINT('Ctrl Pts',(40.038058736007,-67.5695785411523,-220.409682879464));
#228826=CARTESIAN_POINT('Ctrl Pts',(43.4771077064633,-69.2909019608329,
-217.255357871467));
#228827=CARTESIAN_POINT('Ctrl Pts',(46.911032093483,-71.0224993808136,-214.10099631368));
#228828=CARTESIAN_POINT('Ctrl Pts',(26.3772071408559,-60.6610527709189,
-233.021822686564));
#228829=CARTESIAN_POINT('Ctrl Pts',(29.8198922647338,-62.3656430824214,
-229.870183157334));
#228830=CARTESIAN_POINT('Ctrl Pts',(33.2595071470079,-64.0744068681985,
-226.717552132221));
#228831=CARTESIAN_POINT('Ctrl Pts',(36.6950887844903,-65.7896831337175,
-223.564108323038));
#228832=CARTESIAN_POINT('Ctrl Pts',(40.1306704219727,-67.5049593992365,
-220.410664513854));
#228833=CARTESIAN_POINT('Ctrl Pts',(43.5622034605361,-69.2267005231895,
-217.256365654455));
#228834=CARTESIAN_POINT('Ctrl Pts',(46.9885985225256,-70.9587167786769,
-214.102032318221));
#228835=CARTESIAN_POINT('Ctrl Pts',(26.4972071576729,-60.5976714014882,
-233.021374771214));
#228836=CARTESIAN_POINT('Ctrl Pts',(29.9328875356291,-62.3022271706743,
-229.870039558606));
#228837=CARTESIAN_POINT('Ctrl Pts',(33.3654481367504,-64.010966733861,-226.717674406878));
#228838=CARTESIAN_POINT('Ctrl Pts',(36.793844127674,-65.7263329827881,-223.564425346624));
#228839=CARTESIAN_POINT('Ctrl Pts',(40.2222401185977,-67.4416992317152,
-220.411176286369));
#228840=CARTESIAN_POINT('Ctrl Pts',(43.6464575126834,-69.1636354921494,
-217.256997787241));
#228841=CARTESIAN_POINT('Ctrl Pts',(47.0652610833278,-70.8962157902618,
-214.102692345356));
#228842=CARTESIAN_POINT('Ctrl Pts',(26.6170765305167,-60.5338892284733,
-233.020688145171));
#228843=CARTESIAN_POINT('Ctrl Pts',(30.045545113986,-62.238632000908,-229.869690768214));
#228844=CARTESIAN_POINT('Ctrl Pts',(33.4708476093749,-63.9475635251553,
-226.717626646141));
#228845=CARTESIAN_POINT('Ctrl Pts',(36.8918444428126,-65.6632431316632,
-223.564602851986));
#228846=CARTESIAN_POINT('Ctrl Pts',(40.3128412762504,-67.378922738171,-220.411579057831));
#228847=CARTESIAN_POINT('Ctrl Pts',(43.7295213469238,-69.1012807810974,
-217.257546349595));
#228848=CARTESIAN_POINT('Ctrl Pts',(47.140464436521,-70.8347129400802,-214.103279186265));
#228849=CARTESIAN_POINT('Ctrl Pts',(26.7369459033605,-60.4701070554585,
-233.020001519128));
#228850=CARTESIAN_POINT('Ctrl Pts',(30.1582026923428,-62.1750368311418,
-229.869341977822));
#228851=CARTESIAN_POINT('Ctrl Pts',(33.5762470819994,-63.8841603164497,
-226.717578885404));
#228852=CARTESIAN_POINT('Ctrl Pts',(36.9898447579513,-65.6001532805383,
-223.564780357348));
#228853=CARTESIAN_POINT('Ctrl Pts',(40.4034424339031,-67.3161462446269,
-220.411981829292));
#228854=CARTESIAN_POINT('Ctrl Pts',(43.8125851811644,-69.0389260700454,
-217.258094911949));
#228855=CARTESIAN_POINT('Ctrl Pts',(47.2156677897142,-70.7732100898985,
-214.103866027175));
#228856=CARTESIAN_POINT('Ctrl Pts',(26.8570455332274,-60.4056521569874,
-233.019306732319));
#228857=CARTESIAN_POINT('Ctrl Pts',(30.2708768025335,-62.1109922428301,
-229.868974562847));
#228858=CARTESIAN_POINT('Ctrl Pts',(33.6814570870323,-63.8205250164116,
-226.717508054876));
#228859=CARTESIAN_POINT('Ctrl Pts',(37.0874578686263,-65.5370390313854,
-223.564936035396));
#228860=CARTESIAN_POINT('Ctrl Pts',(40.4934586502203,-67.2535530463592,
-220.412364015916));
#228861=CARTESIAN_POINT('Ctrl Pts',(43.8948755984016,-68.9769508862391,
-217.258629913538));
#228862=CARTESIAN_POINT('Ctrl Pts',(47.289907411692,-70.7122816555241,-214.104447241908));
#228863=CARTESIAN_POINT('Ctrl Pts',(26.9773582084069,-60.3405190002037,
-233.018605415792));
#228864=CARTESIAN_POINT('Ctrl Pts',(30.383562017878,-62.046487235826,-229.868590727832));
#228865=CARTESIAN_POINT('Ctrl Pts',(33.786482884195,-63.7566420726074,-226.717416049128));
#228866=CARTESIAN_POINT('Ctrl Pts',(37.1846995203357,-65.4738805679581,
-223.56507131637));
#228867=CARTESIAN_POINT('Ctrl Pts',(40.5829161564765,-67.1911190633088,
-220.412726583613));
#228868=CARTESIAN_POINT('Ctrl Pts',(43.9764292691396,-68.9153271247727,
-217.259151804163));
#228869=CARTESIAN_POINT('Ctrl Pts',(47.3632316759027,-70.6518934365393,
-214.105023471352));
#228870=CARTESIAN_POINT('Ctrl Pts',(27.2179835587658,-60.2102526866361,
-233.017202782736));
#228871=CARTESIAN_POINT('Ctrl Pts',(30.608932448567,-61.9174772218177,-229.867823057804));
#228872=CARTESIAN_POINT('Ctrl Pts',(33.9965344785202,-63.628876184999,-226.717232037632));
#228873=CARTESIAN_POINT('Ctrl Pts',(37.3791828237546,-65.3475636411034,
-223.565341878319));
#228874=CARTESIAN_POINT('Ctrl Pts',(40.761831168989,-67.0662510972078,-220.413451719006));
#228875=CARTESIAN_POINT('Ctrl Pts',(44.1395366106154,-68.7920796018397,
-217.260195585412));
#228876=CARTESIAN_POINT('Ctrl Pts',(47.509880204324,-70.5311169985697,-214.10617593024));
#228877=CARTESIAN_POINT('Ctrl Pts',(27.4594610774215,-60.0772732757658,
-233.015774094218));
#228878=CARTESIAN_POINT('Ctrl Pts',(30.8343473371973,-61.7866254642456,
-229.866989782546));
#228879=CARTESIAN_POINT('Ctrl Pts',(34.2058492100272,-63.5001197459416,
-226.716963322528));
#228880=CARTESIAN_POINT('Ctrl Pts',(37.5721802072639,-65.2210699553996,
-223.565530811621));
#228881=CARTESIAN_POINT('Ctrl Pts',(40.9385112045005,-66.9420201648576,
-220.414098300713));
#228882=CARTESIAN_POINT('Ctrl Pts',(44.2996968466345,-68.6702379154868,
-217.261186869816));
#228883=CARTESIAN_POINT('Ctrl Pts',(47.6528670748933,-70.412501654795,-214.107308443709));
#228884=CARTESIAN_POINT('Ctrl Pts',(27.7016532108346,-59.9415372606891,
-233.014331652954));
#228885=CARTESIAN_POINT('Ctrl Pts',(31.05976276075,-61.6538447557032,-229.866107695338));
#228886=CARTESIAN_POINT('Ctrl Pts',(34.4144695478916,-63.3702479288391,
-226.716625256232));
#228887=CARTESIAN_POINT('Ctrl Pts',(37.7638186351444,-65.0942396965474,
-223.565650201608));
#228888=CARTESIAN_POINT('Ctrl Pts',(41.1131677223973,-66.8182314642556,
-220.414675146985));
#228889=CARTESIAN_POINT('Ctrl Pts',(44.4572046958943,-68.5495754713907,
-217.262129974306));
#228890=CARTESIAN_POINT('Ctrl Pts',(47.7925819070095,-70.295770952258,-214.1084263508));
#228891=CARTESIAN_POINT('Ctrl Pts',(28.1860374776607,-59.6700652305358,
-233.011446770425));
#228892=CARTESIAN_POINT('Ctrl Pts',(31.5105936078552,-61.3882833386183,
-229.864343520922));
#228893=CARTESIAN_POINT('Ctrl Pts',(34.8317102236203,-63.1105042946341,
-226.715949123638));
#228894=CARTESIAN_POINT('Ctrl Pts',(38.1470954909054,-64.8405791788429,
-223.565888981583));
#228895=CARTESIAN_POINT('Ctrl Pts',(41.4624807581906,-66.5706540630517,
-220.415828839529));
#228896=CARTESIAN_POINT('Ctrl Pts',(44.772220394414,-68.3082505831985,-217.264016183284));
#228897=CARTESIAN_POINT('Ctrl Pts',(48.0720115712419,-70.062309547184,-214.110662164981));
#228898=CARTESIAN_POINT('Ctrl Pts',(28.673279908832,-59.3875657071804,-233.008507940657));
#228899=CARTESIAN_POINT('Ctrl Pts',(31.9614269102671,-61.115004898578,-229.862385501452));
#228900=CARTESIAN_POINT('Ctrl Pts',(35.2461728642701,-62.846298987024,-226.714996249958));
#228901=CARTESIAN_POINT('Ctrl Pts',(38.5249351802734,-64.5855733702612,
-223.565849736452));
#228902=CARTESIAN_POINT('Ctrl Pts',(41.8036974962768,-66.3248477534984,
-220.416703222945));
#228903=CARTESIAN_POINT('Ctrl Pts',(45.0766243118393,-68.0716449683638,
-217.26570937755));
#228904=CARTESIAN_POINT('Ctrl Pts',(48.338349401543,-69.8363895329911,-214.112840467621));
#228905=CARTESIAN_POINT('Ctrl Pts',(29.1622830188973,-59.093703206177,-233.005601149464));
#228906=CARTESIAN_POINT('Ctrl Pts',(32.4119055964007,-60.8333256128672,
-229.860352517102));
#228907=CARTESIAN_POINT('Ctrl Pts',(35.6582030143032,-62.5766317072687,
-226.713886241748));
#228908=CARTESIAN_POINT('Ctrl Pts',(38.8983695571512,-64.3279278794606,
-223.565632722533));
#228909=CARTESIAN_POINT('Ctrl Pts',(42.1385360999994,-66.0792240516524,
-220.417379203317));
#228910=CARTESIAN_POINT('Ctrl Pts',(45.3727988408086,-67.8379178590787,
-217.267251393612));
#228911=CARTESIAN_POINT('Ctrl Pts',(48.5947562955792,-69.6157591498535,
-214.114999659484));
#228912=CARTESIAN_POINT('Ctrl Pts',(30.1402892390281,-58.5059782041702,
-232.999787567079));
#228913=CARTESIAN_POINT('Ctrl Pts',(33.312862968668,-60.2699670414456,-229.856286548401));
#228914=CARTESIAN_POINT('Ctrl Pts',(36.4822633143695,-62.0372971477581,
-226.711666225327));
#228915=CARTESIAN_POINT('Ctrl Pts',(39.645238310907,-63.8126368978593,-223.565198694695));
#228916=CARTESIAN_POINT('Ctrl Pts',(42.8082133074446,-65.5879766479605,
-220.418731164063));
#228917=CARTESIAN_POINT('Ctrl Pts',(45.9651478987472,-67.3704636405086,
-217.270335425737));
#228918=CARTESIAN_POINT('Ctrl Pts',(49.1075700836515,-69.1744983835783,
-214.119318043209));
#228919=CARTESIAN_POINT('Ctrl Pts',(31.1253296771952,-57.8727830755883,
-232.994119837029));
#228920=CARTESIAN_POINT('Ctrl Pts',(34.2123982630523,-59.6729838063912,
-229.851946789728));
#228921=CARTESIAN_POINT('Ctrl Pts',(37.2965847816597,-61.4760996503049,
-226.708845019593));
#228922=CARTESIAN_POINT('Ctrl Pts',(40.374466421429,-63.2867830742773,-223.564079694009));
#228923=CARTESIAN_POINT('Ctrl Pts',(43.4523480611983,-65.0974664982497,
-220.419314368426));
#228924=CARTESIAN_POINT('Ctrl Pts',(46.5245369999706,-66.9145532819642,
-217.272835132396));
#228925=CARTESIAN_POINT('Ctrl Pts',(49.5806341150271,-68.7543693866452,
-214.123609471056));
#228926=CARTESIAN_POINT('Ctrl Pts',(32.1087006613968,-57.191646012686,-232.989078118058));
#228927=CARTESIAN_POINT('Ctrl Pts',(35.1076397475695,-59.0371491145894,
-229.847995786691));
#228928=CARTESIAN_POINT('Ctrl Pts',(38.1040273439412,-60.8851347665649,
-226.706162642268));
#228929=CARTESIAN_POINT('Ctrl Pts',(41.0945558666574,-62.7399255565489,
-223.562922655666));
#228930=CARTESIAN_POINT('Ctrl Pts',(44.0850843893735,-64.5947163465329,
-220.419682669063));
#228931=CARTESIAN_POINT('Ctrl Pts',(47.0704902905866,-66.4550539448948,
-217.275009748779));
#228932=CARTESIAN_POINT('Ctrl Pts',(50.0397793224693,-68.3371871397263,
-214.127816818154));
#228933=CARTESIAN_POINT('Ctrl Pts',(34.0754426298001,-55.8293718868815,
-232.978994680116));
#228934=CARTESIAN_POINT('Ctrl Pts',(36.898122716604,-57.765479730986,-229.840093780616));
#228935=CARTESIAN_POINT('Ctrl Pts',(39.7189124685042,-59.7032049990848,
-226.700797887619));
#228936=CARTESIAN_POINT('Ctrl Pts',(42.5347347571142,-61.6462105210921,
-223.560608578979));
#228937=CARTESIAN_POINT('Ctrl Pts',(45.3505570457242,-63.5892160430994,
-220.420419270338));
#228938=CARTESIAN_POINT('Ctrl Pts',(48.1623968718184,-65.5360552707562,
-217.279358981544));
#228939=CARTESIAN_POINT('Ctrl Pts',(50.9580697373535,-67.5028226458884,
-214.13623151235));
#228940=CARTESIAN_POINT('Ctrl Pts',(36.0418015499852,-54.2678518298554,
-232.972801817804));
#228941=CARTESIAN_POINT('Ctrl Pts',(38.677172296014,-56.3317754242655,-229.834906922101));
#228942=CARTESIAN_POINT('Ctrl Pts',(41.3112311995406,-58.3966848422808,
-226.696862079201));
#228943=CARTESIAN_POINT('Ctrl Pts',(43.9416573065822,-60.4651362830048,
-223.558498608177));
#228944=CARTESIAN_POINT('Ctrl Pts',(46.5720834136237,-62.5335877237288,
-220.420135137153));
#228945=CARTESIAN_POINT('Ctrl Pts',(49.1998046996963,-64.6044563549465,
-217.281452032185));
#228946=CARTESIAN_POINT('Ctrl Pts',(51.8146256937275,-66.6895540609604,
-214.142095885467));
#228947=CARTESIAN_POINT('Ctrl Pts',(37.882123536986,-52.5752193780183,-232.970806720566));
#228948=CARTESIAN_POINT('Ctrl Pts',(40.3469003584876,-54.7858287675482,
-229.833381329414));
#228949=CARTESIAN_POINT('Ctrl Pts',(42.8110087314114,-56.9968033268292,
-226.695906966754));
#228950=CARTESIAN_POINT('Ctrl Pts',(45.2731441984033,-59.2095312210711,
-223.558332736904));
#228951=CARTESIAN_POINT('Ctrl Pts',(47.7352796653952,-61.4222591153131,
-220.420758507053));
#228952=CARTESIAN_POINT('Ctrl Pts',(50.1959790879104,-63.636130388643,-217.283078469976));
#228953=CARTESIAN_POINT('Ctrl Pts',(52.6494272678771,-65.857552778289,-214.145217662806));
#228954=CARTESIAN_POINT('Ctrl Pts',(39.7224455239868,-50.8825869261812,
-232.968811623327));
#228955=CARTESIAN_POINT('Ctrl Pts',(42.0166284209611,-53.2398821108309,
-229.831855736726));
#228956=CARTESIAN_POINT('Ctrl Pts',(44.3107862632822,-55.5969218113776,
-226.694951854308));
#228957=CARTESIAN_POINT('Ctrl Pts',(46.6046310902244,-57.9539261591375,
-223.55816686563));
#228958=CARTESIAN_POINT('Ctrl Pts',(48.8984759171666,-60.3109305068973,
-220.421381876952));
#228959=CARTESIAN_POINT('Ctrl Pts',(51.1921534761245,-62.6678044223395,
-217.284704907766));
#228960=CARTESIAN_POINT('Ctrl Pts',(53.4842288420267,-65.0255514956176,
-214.148339440146));
#228961=CARTESIAN_POINT('Ctrl Pts',(41.4461104147051,-49.0481855160699,
-232.97166665431));
#228962=CARTESIAN_POINT('Ctrl Pts',(43.5856625816949,-51.5719501776712,
-229.834567875703));
#228963=CARTESIAN_POINT('Ctrl Pts',(45.725755460948,-54.09499526448,-226.697476434552));
#228964=CARTESIAN_POINT('Ctrl Pts',(47.8671575840062,-56.616542818236,-223.560361067685));
#228965=CARTESIAN_POINT('Ctrl Pts',(50.0085597070645,-59.138090371992,-220.423245700818));
#228966=CARTESIAN_POINT('Ctrl Pts',(52.1509051960796,-61.6584905278127,
-217.286128821816));
#228967=CARTESIAN_POINT('Ctrl Pts',(54.2979333072227,-64.1740643125789,
-214.148798365297));
#228968=CARTESIAN_POINT('Ctrl Pts',(42.9734424791526,-47.1926155685251,
-232.978313839575));
#228969=CARTESIAN_POINT('Ctrl Pts',(44.9946071331279,-49.8757842370209,
-229.840273609375));
#228970=CARTESIAN_POINT('Ctrl Pts',(47.0170439436796,-52.5576635978524,
-226.702063718992));
#228971=CARTESIAN_POINT('Ctrl Pts',(49.0424058070309,-55.2367916852255,
-223.563495724472));
#228972=CARTESIAN_POINT('Ctrl Pts',(51.0677676703821,-57.9159197725986,
-220.424927729951));
#228973=CARTESIAN_POINT('Ctrl Pts',(53.0955326872786,-60.5927163347612,
-217.286025395512));
#228974=CARTESIAN_POINT('Ctrl Pts',(55.1321416284158,-63.2617424152049,
-214.146274180285));
#228975=CARTESIAN_POINT('Ctrl Pts',(43.7371085113763,-46.2648305947527,
-232.981637432207));
#228976=CARTESIAN_POINT('Ctrl Pts',(45.6990794088443,-49.0277012666958,
-229.84312647621));
#228977=CARTESIAN_POINT('Ctrl Pts',(47.6626881850455,-51.7889977645385,
-226.704357361211));
#228978=CARTESIAN_POINT('Ctrl Pts',(49.6300299185432,-54.5469161187202,
-223.565063052865));
#228979=CARTESIAN_POINT('Ctrl Pts',(51.5973716520409,-57.3048344729019,
-220.425768744518));
#228980=CARTESIAN_POINT('Ctrl Pts',(53.5678464328781,-60.0598292382354,
-217.285973682359));
#228981=CARTESIAN_POINT('Ctrl Pts',(55.5492457890124,-62.8055814665179,
-214.145012087778));
#228982=CARTESIAN_POINT('Ctrl Pts',(44.4530216283881,-45.330501487166,-232.985755113274));
#228983=CARTESIAN_POINT('Ctrl Pts',(46.364564734047,-48.1716118824616,-229.846604427224));
#228984=CARTESIAN_POINT('Ctrl Pts',(48.2780837959556,-51.0109018738896,
-226.707080446303));
#228985=CARTESIAN_POINT('Ctrl Pts',(50.19592152344,-53.846435222383,-223.566845772292));
#228986=CARTESIAN_POINT('Ctrl Pts',(52.1137592509244,-56.6819685708763,
-220.42661109828));
#228987=CARTESIAN_POINT('Ctrl Pts',(54.0353913811122,-59.5141054680716,
-217.285678387203));
#228988=CARTESIAN_POINT('Ctrl Pts',(55.9686189515471,-62.3368927213004,
-214.143346745665));
#228989=CARTESIAN_POINT('Ctrl Pts',(45.122678945944,-44.3985758751927,-232.990284156912));
#228990=CARTESIAN_POINT('Ctrl Pts',(46.9953289795326,-47.3107844763396,
-229.850249364904));
#228991=CARTESIAN_POINT('Ctrl Pts',(48.8702338796761,-50.2209949619586,
-226.709744329754));
#228992=CARTESIAN_POINT('Ctrl Pts',(50.7497258393681,-53.1273622037278,
-223.56843670589));
#228993=CARTESIAN_POINT('Ctrl Pts',(52.62921779906,-56.033729445497,-220.427129082025));
#228994=CARTESIAN_POINT('Ctrl Pts',(54.5128930537055,-58.9365113017985,
-217.285019110898));
#228995=CARTESIAN_POINT('Ctrl Pts',(56.4076769323115,-61.8306798185293,
-214.141539423862));
#228996=CARTESIAN_POINT('Ctrl Pts',(45.457507604722,-43.9326130692061,-232.99254867873));
#228997=CARTESIAN_POINT('Ctrl Pts',(47.3107111022754,-46.8803707732786,
-229.852071833745));
#228998=CARTESIAN_POINT('Ctrl Pts',(49.1663089215364,-49.8260415059931,
-226.711076271479));
#228999=CARTESIAN_POINT('Ctrl Pts',(51.0266279973321,-52.7678256944002,
-223.569232172689));
#229000=CARTESIAN_POINT('Ctrl Pts',(52.8869470731278,-55.7096098828074,
-220.427388073898));
#229001=CARTESIAN_POINT('Ctrl Pts',(54.7516438900022,-58.6477142186619,
-217.284689472746));
#229002=CARTESIAN_POINT('Ctrl Pts',(56.6272059226936,-61.5775733671438,
-214.14063576296));
#229003=CARTESIAN_POINT('Ctrl Pts',(45.7807674564663,-43.4672624822902,
-232.994913812328));
#229004=CARTESIAN_POINT('Ctrl Pts',(47.617410659328,-46.4487812870827,-229.853931471351));
#229005=CARTESIAN_POINT('Ctrl Pts',(49.4565719492878,-49.4281424234071,
-226.71238699417));
#229006=CARTESIAN_POINT('Ctrl Pts',(51.3005099358702,-52.4036466369632,
-223.569971790265));
#229007=CARTESIAN_POINT('Ctrl Pts',(53.1444479224527,-55.3791508505193,
-220.427556586359));
#229008=CARTESIAN_POINT('Ctrl Pts',(54.992887213388,-58.3509530949211,-217.284258923378));
#229009=CARTESIAN_POINT('Ctrl Pts',(56.8516818382195,-61.3150753857701,
-214.139681306367));
#229010=CARTESIAN_POINT('Ctrl Pts',(46.0926567139982,-43.0036690826345,
-232.997311586148));
#229011=CARTESIAN_POINT('Ctrl Pts',(47.9159791152656,-46.0164399058077,
-229.855739900183));
#229012=CARTESIAN_POINT('Ctrl Pts',(49.7419098599322,-49.0270196364001,
-226.713581949947));
#229013=CARTESIAN_POINT('Ctrl Pts',(51.5725780231494,-52.0338565143131,
-223.570570609253));
#229014=CARTESIAN_POINT('Ctrl Pts',(53.4032461863666,-55.0406933922261,
-220.427559268559));
#229015=CARTESIAN_POINT('Ctrl Pts',(55.2384359222485,-58.0439012335412,
-217.283679691665));
#229016=CARTESIAN_POINT('Ctrl Pts',(57.083299585097,-61.0401022731089,-214.13864916931));
#229017=CARTESIAN_POINT('Ctrl Pts',(46.2486013427642,-42.7718723828066,
-232.998510473058));
#229018=CARTESIAN_POINT('Ctrl Pts',(48.0652633432344,-45.8002692151702,
-229.856644114599));
#229019=CARTESIAN_POINT('Ctrl Pts',(49.8845788152544,-48.8264582428966,
-226.714179427834));
#229020=CARTESIAN_POINT('Ctrl Pts',(51.708612066789,-51.848961452988,-223.570870018747));
#229021=CARTESIAN_POINT('Ctrl Pts',(53.5326453183235,-54.8714646630795,
-220.427560609659));
#229022=CARTESIAN_POINT('Ctrl Pts',(55.3612102766787,-57.8903753028513,
-217.283390075808));
#229023=CARTESIAN_POINT('Ctrl Pts',(57.1991084585358,-60.9026157167782,
-214.13813310078));
#229024=CARTESIAN_POINT('Ctrl Pts',(46.4017035779887,-42.5405150976846,
-232.999717286874));
#229025=CARTESIAN_POINT('Ctrl Pts',(48.2125150982371,-45.5839105491989,
-229.857535197574));
#229026=CARTESIAN_POINT('Ctrl Pts',(50.0260166354934,-48.6250910294446,
-226.714747674137));
#229027=CARTESIAN_POINT('Ctrl Pts',(51.844192559889,-51.6626639281839,-223.571133990991));
#229028=CARTESIAN_POINT('Ctrl Pts',(53.6623684842846,-54.7002368269232,
-220.427520307844));
#229029=CARTESIAN_POINT('Ctrl Pts',(55.4850604557961,-57.7342773380644,
-217.283063148945));
#229030=CARTESIAN_POINT('Ctrl Pts',(57.3167022282962,-60.7620113048676,
-214.137597228726));
#229031=CARTESIAN_POINT('Ctrl Pts',(46.5519897086414,-42.3097409936012,
-233.000922137489));
#229032=CARTESIAN_POINT('Ctrl Pts',(48.3578050935127,-45.3674166545976,
-229.858400212826));
#229033=CARTESIAN_POINT('Ctrl Pts',(50.166334738395,-48.4228838232303,-226.715273522923));
#229034=CARTESIAN_POINT('Ctrl Pts',(51.9794693444289,-51.4748446769843,
-223.571351034937));
#229035=CARTESIAN_POINT('Ctrl Pts',(53.7926039504629,-54.5268055307383,
-220.427428546952));
#229036=CARTESIAN_POINT('Ctrl Pts',(55.6102096831407,-57.5753202178,-217.28269273506));
#229037=CARTESIAN_POINT('Ctrl Pts',(57.4363509894997,-60.6179092484165,
-214.137036747929));
#229038=CARTESIAN_POINT('Ctrl Pts',(46.6271327739678,-42.1943539415595,
-233.001524562797));
#229039=CARTESIAN_POINT('Ctrl Pts',(48.4304500911505,-45.2591697072969,
-229.858832720452));
#229040=CARTESIAN_POINT('Ctrl Pts',(50.2364937898458,-48.3217802201232,
-226.715536447315));
#229041=CARTESIAN_POINT('Ctrl Pts',(52.0471077366989,-51.3809350513845,
-223.571459556911));
#229042=CARTESIAN_POINT('Ctrl Pts',(53.857721683552,-54.4400898826458,-220.427382666507));
#229043=CARTESIAN_POINT('Ctrl Pts',(55.672784296813,-57.4958416576678,-217.282507528118));
#229044=CARTESIAN_POINT('Ctrl Pts',(57.4961753701015,-60.5458582201909,
-214.136756507531));
#229045=CARTESIAN_POINT('Ctrl Pts',(46.7015718287581,-42.0791126910049,
-233.00212648283));
#229046=CARTESIAN_POINT('Ctrl Pts',(48.5026046671152,-45.1508889484801,
-229.859258692179));
#229047=CARTESIAN_POINT('Ctrl Pts',(50.3063729152009,-48.2204666245557,
-226.715788761507));
#229048=CARTESIAN_POINT('Ctrl Pts',(52.1146701884246,-51.2866450128194,
-223.571556342237));
#229049=CARTESIAN_POINT('Ctrl Pts',(53.9229674616482,-54.3528234010831,
-220.427323922968));
#229050=CARTESIAN_POINT('Ctrl Pts',(55.7356836352042,-57.4156483458129,
-217.282311452432));
#229051=CARTESIAN_POINT('Ctrl Pts',(57.5565134471849,-60.4729328402728,
-214.136470106837));
#229052=CARTESIAN_POINT('Ctrl Pts',(46.7753102520778,-41.9640352485997,
-233.002726574857));
#229053=CARTESIAN_POINT('Ctrl Pts',(48.5742777683907,-45.0425809377688,
-229.859676400769));
#229054=CARTESIAN_POINT('Ctrl Pts',(50.3759860497308,-48.1189387987811,
-226.716028769071));
#229055=CARTESIAN_POINT('Ctrl Pts',(52.1821753368859,-51.191959764097,-223.571639944857));
#229056=CARTESIAN_POINT('Ctrl Pts',(53.9883646240409,-54.264980729413,-220.427251120643));
#229057=CARTESIAN_POINT('Ctrl Pts',(55.7989353732621,-57.3347046065519,
-217.282103770803));
#229058=CARTESIAN_POINT('Ctrl Pts',(57.6173986625019,-60.3990859831037,
-214.136176919604));
#229059=CARTESIAN_POINT('Ctrl Pts',(46.8121794637376,-41.9064965273971,
-233.003026620871));
#229060=CARTESIAN_POINT('Ctrl Pts',(48.6101143190285,-44.9884269324132,
-229.859885255064));
#229061=CARTESIAN_POINT('Ctrl Pts',(50.4107926169958,-48.0681748858937,
-226.716148772852));
#229062=CARTESIAN_POINT('Ctrl Pts',(52.2159279111165,-51.1446171397359,
-223.571681746167));
#229063=CARTESIAN_POINT('Ctrl Pts',(54.0210632052373,-54.221059393578,-220.427214719482));
#229064=CARTESIAN_POINT('Ctrl Pts',(55.8305612422911,-57.2942327369214,
-217.281999929988));
#229065=CARTESIAN_POINT('Ctrl Pts',(57.6478412701604,-60.3621625545191,
-214.136030325987));
#229066=CARTESIAN_POINT('Ctrl Pts',(46.8488735184923,-41.8489987585935,
-233.003326208986));
#229067=CARTESIAN_POINT('Ctrl Pts',(48.645830502103,-44.9342661136713,-229.860092042457));
#229068=CARTESIAN_POINT('Ctrl Pts',(50.4455326865456,-48.0173574158033,
-226.716265699565));
#229069=CARTESIAN_POINT('Ctrl Pts',(52.2496661584613,-51.0971757139789,
-223.571720251843));
#229070=CARTESIAN_POINT('Ctrl Pts',(54.053799630377,-54.1769940121544,-220.427174804122));
#229071=CARTESIAN_POINT('Ctrl Pts',(55.8622752088309,-57.2535732626049,
-217.281893188185));
#229072=CARTESIAN_POINT('Ctrl Pts',(57.6784206589513,-60.3250087601744,
-214.135882035655));
#229073=CARTESIAN_POINT('Ctrl Pts',(46.8853928444761,-41.791544195152,-233.003625168491));
#229074=CARTESIAN_POINT('Ctrl Pts',(48.681427442577,-44.8800992987762,-229.860296540463));
#229075=CARTESIAN_POINT('Ctrl Pts',(50.4802079998591,-47.9664858608819,
-226.716379335157));
#229076=CARTESIAN_POINT('Ctrl Pts',(52.2833924017896,-51.0496336439922,
-223.57175528194));
#229077=CARTESIAN_POINT('Ctrl Pts',(54.0865768037201,-54.1327814271025,
-220.427131228723));
#229078=CARTESIAN_POINT('Ctrl Pts',(55.8940807177617,-57.2127217368356,
-217.281783456688));
#229079=CARTESIAN_POINT('Ctrl Pts',(57.7091409883845,-60.287618730288,-214.135731970477));
#229080=CARTESIAN_POINT('Ctrl Pts',(46.9219121704599,-41.7340896317106,
-233.003924127997));
#229081=CARTESIAN_POINT('Ctrl Pts',(48.7170243830511,-44.8259324838809,
-229.860501038468));
#229082=CARTESIAN_POINT('Ctrl Pts',(50.5148833131725,-47.9156143059604,
-226.716492970748));
#229083=CARTESIAN_POINT('Ctrl Pts',(52.3171186451179,-51.0020915740055,
-223.571790312035));
#229084=CARTESIAN_POINT('Ctrl Pts',(54.1193539770633,-54.0885688420506,
-220.427087653323));
#229085=CARTESIAN_POINT('Ctrl Pts',(55.9258862266926,-57.1718702110663,
-217.28167372519));
#229086=CARTESIAN_POINT('Ctrl Pts',(57.7398613178177,-60.2502287004015,
-214.1355819053));
#229087=CARTESIAN_POINT('Ctrl Pts',(46.9566286849537,-41.6781739629451,
-233.004786483119));
#229088=CARTESIAN_POINT('Ctrl Pts',(48.7510652266437,-44.7730579825931,
-229.861179418927));
#229089=CARTESIAN_POINT('Ctrl Pts',(50.5482471004081,-47.8657963569279,
-226.716997721658));
#229090=CARTESIAN_POINT('Ctrl Pts',(52.3497454436632,-50.9553990731154,
-223.572150029539));
#229091=CARTESIAN_POINT('Ctrl Pts',(54.1512437869183,-54.045001789303,-220.427302337419));
#229092=CARTESIAN_POINT('Ctrl Pts',(55.9569880950718,-57.1314927928873,
-217.28177244287));
#229093=CARTESIAN_POINT('Ctrl Pts',(57.7699448315789,-60.2132374154909,
-214.135620383829));
#229094=CARTESIAN_POINT('Ctrl Pts',(46.9944270680642,-41.6193123752663,
-233.004519986905));
#229095=CARTESIAN_POINT('Ctrl Pts',(48.7878616654988,-44.7175816808496,
-229.860902939557));
#229096=CARTESIAN_POINT('Ctrl Pts',(50.5840414119712,-47.8137084153908,
-226.716710153573));
#229097=CARTESIAN_POINT('Ctrl Pts',(52.3845374377678,-50.9067036630134,
-223.571849766529));
#229098=CARTESIAN_POINT('Ctrl Pts',(54.1850334635645,-53.999698910636,-220.426989379484));
#229099=CARTESIAN_POINT('Ctrl Pts',(55.9897753069174,-57.0895865666151,
-217.281445207064));
#229100=CARTESIAN_POINT('Ctrl Pts',(57.8017289442242,-60.1747340778167,
-214.135276372889));
#229101=CARTESIAN_POINT('',(42.5905577899916,-59.5881438265759,-225.000659040692));
#229102=CARTESIAN_POINT('Ctrl Pts',(48.0699773995699,-67.6025469094394,
-215.850046920284));
#229103=CARTESIAN_POINT('Ctrl Pts',(47.7935023710083,-67.6024435901635,
-216.017223628435));
#229104=CARTESIAN_POINT('Ctrl Pts',(47.5226056108187,-67.582824338481,-216.193667415816));
#229105=CARTESIAN_POINT('Ctrl Pts',(46.977436852346,-67.5066353741775,-216.573412312879));
#229106=CARTESIAN_POINT('Ctrl Pts',(46.7040353171343,-67.4475753904985,
-216.777867265333));
#229107=CARTESIAN_POINT('Ctrl Pts',(45.9194030179712,-67.2207720759173,
-217.404700028598));
#229108=CARTESIAN_POINT('Ctrl Pts',(45.4358292265538,-67.0029495672137,
-217.845716150032));
#229109=CARTESIAN_POINT('Ctrl Pts',(44.3014622491286,-66.3069334262244,
-219.018073172323));
#229110=CARTESIAN_POINT('Ctrl Pts',(43.7134054388236,-65.7467619649099,
-219.774958898585));
#229111=CARTESIAN_POINT('Ctrl Pts',(42.671590937337,-64.2628736065213,-221.493288736666));
#229112=CARTESIAN_POINT('Ctrl Pts',(42.3167080561812,-63.2947927751779,
-222.43402647705));
#229113=CARTESIAN_POINT('Ctrl Pts',(42.1771404629389,-61.8708033766555,
-223.580484791701));
#229114=CARTESIAN_POINT('Ctrl Pts',(42.1800068789037,-61.4303388698659,
-223.906345139465));
#229115=CARTESIAN_POINT('Ctrl Pts',(42.2949054530161,-60.5240489278744,
-224.504112440003));
#229116=CARTESIAN_POINT('Ctrl Pts',(42.408777306269,-60.0550288946459,-224.777157735681));
#229117=CARTESIAN_POINT('Ctrl Pts',(42.5905622784972,-59.5881432109375,
-225.000654103808));
#229118=CARTESIAN_POINT('Ctrl Pts',(41.9650124840222,-58.9506172433346,
-225.850033985948));
#229119=CARTESIAN_POINT('Ctrl Pts',(42.1735122754178,-59.1631093475985,
-225.566889535856));
#229120=CARTESIAN_POINT('Ctrl Pts',(42.3820244017841,-59.3756157357695,
-225.283764882133));
#229121=CARTESIAN_POINT('Ctrl Pts',(42.590551250619,-59.5881391761779,-225.000663880113));
#229122=CARTESIAN_POINT('Ctrl Pts',(46.0300272746615,-56.2113956834816,
-225.073027562072));
#229123=CARTESIAN_POINT('Ctrl Pts',(46.4556946111428,-56.0546198433881,
-224.882973868584));
#229124=CARTESIAN_POINT('Ctrl Pts',(46.8821025220939,-55.9535510454092,
-224.650935135084));
#229125=CARTESIAN_POINT('Ctrl Pts',(47.8275283497954,-55.8299386675253,
-224.064731751774));
#229126=CARTESIAN_POINT('Ctrl Pts',(48.3429266049596,-55.835913891429,-223.692840875377));
#229127=CARTESIAN_POINT('Ctrl Pts',(49.8207751121238,-56.031385302888,-222.507098599534));
#229128=CARTESIAN_POINT('Ctrl Pts',(50.7673640957262,-56.4134990790704,
-221.576308252714));
#229129=CARTESIAN_POINT('Ctrl Pts',(52.1947859669311,-57.4789725689598,
-219.875568079017));
#229130=CARTESIAN_POINT('Ctrl Pts',(52.7242457809075,-58.0629688538461,
-219.129990774748));
#229131=CARTESIAN_POINT('Ctrl Pts',(53.3981925598294,-59.2055512880101,
-217.935308076124));
#229132=CARTESIAN_POINT('Ctrl Pts',(53.6140169907078,-59.7152280480568,
-217.464070022383));
#229133=CARTESIAN_POINT('Ctrl Pts',(53.823623756443,-60.5278747738901,-216.806115800707));
#229134=CARTESIAN_POINT('Ctrl Pts',(53.8746160000559,-60.8015922181664,
-216.59808676812));
#229135=CARTESIAN_POINT('Ctrl Pts',(53.9357818734408,-61.3524150136747,
-216.207348054255));
#229136=CARTESIAN_POINT('Ctrl Pts',(53.9476675105347,-61.6291888829114,
-216.023694309118));
#229137=CARTESIAN_POINT('Ctrl Pts',(53.9390346875573,-61.9113848028035,
-215.85005));
#229138=CARTESIAN_POINT('Origin',(-296.501483394397,-25.4138432731711,-232.85005));
#229139=CARTESIAN_POINT('Origin',(-296.501483394397,-25.4138432731711,-232.85005));
#229140=CARTESIAN_POINT('Origin',(-296.501483394397,-25.4138432731711,-232.85005));
#229141=CARTESIAN_POINT('Ctrl Pts',(47.8524635552839,9.39108009190695,-232.85005));
#229142=CARTESIAN_POINT('Ctrl Pts',(47.8251207475469,9.27869452829692,-232.85005));
#229143=CARTESIAN_POINT('Ctrl Pts',(47.7988578503937,9.16605178669897,-232.850050000002));
#229144=CARTESIAN_POINT('Ctrl Pts',(47.748545239995,8.94041318528332,-232.850050000002));
#229145=CARTESIAN_POINT('Ctrl Pts',(47.724495099355,8.82742853781197,-232.85005));
#229146=CARTESIAN_POINT('Ctrl Pts',(47.7015450634132,8.71421534318054,-232.85005));
#229147=CARTESIAN_POINT('Origin',(-296.501483394397,-25.4138432731711,-232.85005));
#229148=CARTESIAN_POINT('',(47.8903177140771,0.753846963912772,-232.850053817009));
#229149=CARTESIAN_POINT('',(47.9312868154534,-1.80167576439666,-232.850051862368));
#229150=CARTESIAN_POINT('Origin',(-636.934816028482,-11.5034818258361,-232.85005));
#229151=CARTESIAN_POINT('Ctrl Pts',(47.8903230579921,0.75384761155793,-232.85005));
#229152=CARTESIAN_POINT('Ctrl Pts',(47.9416806402025,0.330080749513371,
-232.85005));
#229153=CARTESIAN_POINT('Ctrl Pts',(47.9708351916769,-0.0957528761675352,
-232.850050000016));
#229154=CARTESIAN_POINT('Ctrl Pts',(47.9845049252711,-0.949121595702693,
-232.850050000016));
#229155=CARTESIAN_POINT('Ctrl Pts',(47.9690400279578,-1.37636719046752,
-232.85005));
#229156=CARTESIAN_POINT('Ctrl Pts',(47.931289209931,-1.8016759769328,-232.85005));
#229157=CARTESIAN_POINT('Origin',(-296.501483394397,-25.4138432731711,-232.85005));
#229158=CARTESIAN_POINT('',(47.9981322791795,-9.91532742768912,-232.850009339772));
#229159=CARTESIAN_POINT('',(47.997728950092,-13.2576713000527,-232.850013208975));
#229160=CARTESIAN_POINT('Origin',(-636.934816028482,-11.5034818258361,-232.85005));
#229161=CARTESIAN_POINT('Ctrl Pts',(47.9981596989455,-9.91572581758462,
-232.85005));
#229162=CARTESIAN_POINT('Ctrl Pts',(48.0735876072948,-10.4686220040327,
-232.85005));
#229163=CARTESIAN_POINT('Ctrl Pts',(48.111732737437,-11.0279091079018,-232.850050000004));
#229164=CARTESIAN_POINT('Ctrl Pts',(48.1116193885485,-12.1445472383142,
-232.850050000004));
#229165=CARTESIAN_POINT('Ctrl Pts',(48.0733656267235,-12.7040603360745,
-232.85005));
#229166=CARTESIAN_POINT('Ctrl Pts',(47.9977546165575,-13.2572998177683,
-232.85005));
#229167=CARTESIAN_POINT('Origin',(-296.501483394397,-25.4138432731711,-232.85005));
#229168=CARTESIAN_POINT('',(47.9291893708826,-21.3522304066337,-232.850051757442));
#229169=CARTESIAN_POINT('',(47.8870567810509,-23.9416215055321,-232.850052596546));
#229170=CARTESIAN_POINT('Origin',(-636.934816028482,-11.5034818258361,-232.85005));
#229171=CARTESIAN_POINT('Ctrl Pts',(47.9291915823105,-21.3522302047528,
-232.85005));
#229172=CARTESIAN_POINT('Ctrl Pts',(47.9685182384575,-21.7830192761799,
-232.85005));
#229173=CARTESIAN_POINT('Ctrl Pts',(47.9846715385175,-22.2158717781124,
-232.850050000025));
#229174=CARTESIAN_POINT('Ctrl Pts',(47.9706154668222,-23.0806717086304,
-232.850050000025));
#229175=CARTESIAN_POINT('Ctrl Pts',(47.9403670434393,-23.5122314437053,
-232.85005));
#229176=CARTESIAN_POINT('Ctrl Pts',(47.8870605128751,-23.9416219688181,
-232.85005));
#229177=CARTESIAN_POINT('Origin',(-296.501483394397,-25.4138432731711,-232.85005));
#229178=CARTESIAN_POINT('Origin',(-296.501483394397,-25.4138432731711,-232.85005));
#229179=CARTESIAN_POINT('Origin',(7.14692237356698E-14,623.509175991979,
-232.85005));
#229180=CARTESIAN_POINT('Origin',(0.128459562639233,-12.6359082483571,-225.85005));
#229181=CARTESIAN_POINT('',(46.7347424436738,30.7127197009669,-225.85005));
#229182=CARTESIAN_POINT('',(53.8170476734233,37.8187794096849,-225.85005));
#229183=CARTESIAN_POINT('Origin',(48.892180948596,36.2913696007177,-225.85005));
#229184=CARTESIAN_POINT('Origin',(-636.934816028482,-11.5034818258361,-234.75005));
#229185=CARTESIAN_POINT('',(47.9849429580539,-16.0452820755244,-232.250052142049));
#229186=CARTESIAN_POINT('Ctrl Pts',(47.9849415007718,-16.0452825742631,
-232.250056396759));
#229187=CARTESIAN_POINT('Ctrl Pts',(47.9880651131551,-15.5742306821435,
-232.306343147701));
#229188=CARTESIAN_POINT('Ctrl Pts',(47.9906783186251,-15.1065446149,-232.390988202577));
#229189=CARTESIAN_POINT('Ctrl Pts',(47.9942849350889,-14.320313988702,-232.579502137916));
#229190=CARTESIAN_POINT('Ctrl Pts',(47.9949617724352,-14.1407707776584,
-232.63620114363));
#229191=CARTESIAN_POINT('Ctrl Pts',(47.9965339240141,-13.6931733666124,
-232.756352689264));
#229192=CARTESIAN_POINT('Ctrl Pts',(47.9971930434381,-13.4765686882966,
-232.806954412833));
#229193=CARTESIAN_POINT('Ctrl Pts',(47.9977536577186,-13.2576742406487,
-232.849976417951));
#229194=CARTESIAN_POINT('',(47.9866836135147,-7.23226647128749,-232.25005191098));
#229195=CARTESIAN_POINT('Ctrl Pts',(47.9866823371376,-7.23226600773658,
-232.250055704934));
#229196=CARTESIAN_POINT('Ctrl Pts',(47.9895098141047,-7.68567315065749,
-232.306404893475));
#229197=CARTESIAN_POINT('Ctrl Pts',(47.9918619737062,-8.13535273752232,
-232.390421945344));
#229198=CARTESIAN_POINT('Ctrl Pts',(47.995107332478,-8.89528528307897,-232.579944924862));
#229199=CARTESIAN_POINT('Ctrl Pts',(47.9956980243111,-9.06520173917856,
-232.636698278921));
#229200=CARTESIAN_POINT('Ctrl Pts',(47.9971000735034,-9.49971705152388,
-232.757828882289));
#229201=CARTESIAN_POINT('Ctrl Pts',(47.9976741114909,-9.70630395457126,
-232.807646456627));
#229202=CARTESIAN_POINT('Ctrl Pts',(47.9981587677023,-9.91532414481652,
-232.849968679543));
#229203=CARTESIAN_POINT('Origin',(-636.934816028482,-11.5034818258361,-232.25005));
#229204=CARTESIAN_POINT('Origin',(-636.934816028482,-11.5034818258361,-234.75005));
#229205=CARTESIAN_POINT('',(47.8275275119674,3.86645886896208,-232.25005));
#229206=CARTESIAN_POINT('',(47.964414121789,-4.51936150138566,-232.250085462548));
#229207=CARTESIAN_POINT('Origin',(-636.934816028482,-11.5034818258361,-232.25005));
#229208=CARTESIAN_POINT('Ctrl Pts',(47.9312856139398,-1.80167637106908,
-232.850055542859));
#229209=CARTESIAN_POINT('Ctrl Pts',(47.9394982187954,-2.38141739947619,
-232.757175193342));
#229210=CARTESIAN_POINT('Ctrl Pts',(47.9438448367591,-2.72209125825006,
-232.634139478141));
#229211=CARTESIAN_POINT('Ctrl Pts',(47.9546121728049,-3.60581024688955,
-232.397143115093));
#229212=CARTESIAN_POINT('Ctrl Pts',(47.9597127880174,-4.06055719278633,
-232.308472253132));
#229213=CARTESIAN_POINT('Ctrl Pts',(47.9643913372341,-4.51935999242227,
-232.250120925096));
#229214=CARTESIAN_POINT('Ctrl Pts',(47.8275275119675,3.86645886896215,-232.250050000001));
#229215=CARTESIAN_POINT('Ctrl Pts',(47.8393033810286,3.34181977921867,-232.308606692494));
#229216=CARTESIAN_POINT('Ctrl Pts',(47.8504216708135,2.81940125771994,-232.399682736104));
#229217=CARTESIAN_POINT('Ctrl Pts',(47.8640428170577,2.14390431818647,-232.555058644712));
#229218=CARTESIAN_POINT('Ctrl Pts',(47.8678682595302,1.94983002712611,-232.604470061216));
#229219=CARTESIAN_POINT('Ctrl Pts',(47.8765736965627,1.50418121395801,-232.718114713146));
#229220=CARTESIAN_POINT('Ctrl Pts',(47.8835694576844,1.13072531539176,-232.79486347822));
#229221=CARTESIAN_POINT('Ctrl Pts',(47.8903149889077,0.753848021453941,
-232.850061370667));
#229222=CARTESIAN_POINT('Origin',(-636.934816028482,-11.5034818258361,-234.75005));
#229223=CARTESIAN_POINT('',(47.7599172087245,-29.6370001055535,-232.25005));
#229224=CARTESIAN_POINT('Ctrl Pts',(47.7599172087245,-29.6370001055535,
-232.25005));
#229225=CARTESIAN_POINT('Ctrl Pts',(47.7493722429097,-30.0351623619991,
-232.296082730074));
#229226=CARTESIAN_POINT('Ctrl Pts',(47.7385258657941,-30.4314329746859,
-232.367779772163));
#229227=CARTESIAN_POINT('Ctrl Pts',(47.7172003916566,-31.187345806892,-232.567309385582));
#229228=CARTESIAN_POINT('Ctrl Pts',(47.7067067250054,-31.5486321455587,
-232.692442513232));
#229229=CARTESIAN_POINT('Ctrl Pts',(47.6963708708293,-31.895640436697,-232.849812673883));
#229230=CARTESIAN_POINT('Origin',(-636.934816028482,-11.5034818258361,-232.25005));
#229231=CARTESIAN_POINT('Origin',(-636.934816028482,-11.5034818258361,-234.75005));
#229232=CARTESIAN_POINT('',(47.9620917742134,-18.7116135554145,-232.250083778217));
#229233=CARTESIAN_POINT('',(47.8203127443142,-27.1915604710334,-232.250049983782));
#229234=CARTESIAN_POINT('Origin',(-636.934816028482,-11.5034818258361,-232.25005));
#229235=CARTESIAN_POINT('Ctrl Pts',(47.8870548777005,-23.9416222224618,
-232.850057734118));
#229236=CARTESIAN_POINT('Ctrl Pts',(47.8808419217875,-24.2836965162462,
-232.800020744849));
#229237=CARTESIAN_POINT('Ctrl Pts',(47.8744102330396,-24.6236650946738,
-232.733213391966));
#229238=CARTESIAN_POINT('Ctrl Pts',(47.8666304747006,-25.0195680911603,
-232.639069109827));
#229239=CARTESIAN_POINT('Ctrl Pts',(47.8654339475289,-25.0799470332769,
-232.624108273732));
#229240=CARTESIAN_POINT('Ctrl Pts',(47.8619240948933,-25.2566749049009,
-232.580479584125));
#229241=CARTESIAN_POINT('Ctrl Pts',(47.8588236469908,-25.4102068712725,
-232.544854491086));
#229242=CARTESIAN_POINT('Ctrl Pts',(47.8446425337259,-26.1008593428925,
-232.395217345887));
#229243=CARTESIAN_POINT('Ctrl Pts',(47.8328230396433,-26.6455101093032,
-232.305849122883));
#229244=CARTESIAN_POINT('Ctrl Pts',(47.8203127558795,-27.1915604680009,
-232.250049951514));
#229245=CARTESIAN_POINT('Ctrl Pts',(47.9620703905618,-18.7116148344343,
-232.250117556434));
#229246=CARTESIAN_POINT('Ctrl Pts',(47.9573554139265,-19.1596188894641,
-232.306669891439));
#229247=CARTESIAN_POINT('Ctrl Pts',(47.9522383472777,-19.6037872884333,
-232.393382749302));
#229248=CARTESIAN_POINT('Ctrl Pts',(47.9411866433024,-20.4904993022866,
-232.635960657363));
#229249=CARTESIAN_POINT('Ctrl Pts',(47.937212253039,-20.7942559961686,-232.756243969882));
#229250=CARTESIAN_POINT('Ctrl Pts',(47.9291882608127,-21.3522298073388,
-232.850055227));
#229251=CARTESIAN_POINT('Origin',(7.14692237356698E-14,623.509175991979,
-234.75005));
#229252=CARTESIAN_POINT('Origin',(7.14692237356698E-14,623.509175991979,
-232.25005));
#229253=CARTESIAN_POINT('Origin',(49.9798730220992,-67.1190133783941,-228.35005));
#229254=CARTESIAN_POINT('',(42.5792116384512,-59.576583500476,-225.85005));
#229255=CARTESIAN_POINT('Origin',(48.892180948596,36.2913696007177,-218.306418983907));
#229256=CARTESIAN_POINT('',(46.7347424436738,30.7127197009669,-225.85005));
#229257=CARTESIAN_POINT('Origin',(53.8170476734233,37.8187794096849,-228.35005));
#229258=CARTESIAN_POINT('Ctrl Pts',(47.6009947863409,-32.6895605159758,
-233.446187702606));
#229259=CARTESIAN_POINT('Ctrl Pts',(49.8025157165519,-35.2628848633458,
-230.069700789871));
#229260=CARTESIAN_POINT('Ctrl Pts',(52.004194845104,-37.8467163541935,-226.701486649479));
#229261=CARTESIAN_POINT('Ctrl Pts',(54.2056301169259,-40.4346768564372,
-223.336322656971));
#229262=CARTESIAN_POINT('Ctrl Pts',(56.4070653887478,-43.0226373586808,
-219.971158664462));
#229263=CARTESIAN_POINT('Ctrl Pts',(58.6083138625641,-45.6150709680905,
-216.609349785985));
#229264=CARTESIAN_POINT('Ctrl Pts',(60.8093841578956,-48.2097095522884,
-213.249138279223));
#229265=CARTESIAN_POINT('Ctrl Pts',(47.1654872359782,-30.7268333335968,
-233.215238694904));
#229266=CARTESIAN_POINT('Ctrl Pts',(49.3424661286879,-33.1216582244425,
-229.854296748355));
#229267=CARTESIAN_POINT('Ctrl Pts',(51.5175746565146,-35.5225299367126,
-226.496223095384));
#229268=CARTESIAN_POINT('Ctrl Pts',(53.691970049721,-37.9257105515243,-223.139241204672));
#229269=CARTESIAN_POINT('Ctrl Pts',(55.8663654429275,-40.3288911663362,
-219.782259313959));
#229270=CARTESIAN_POINT('Ctrl Pts',(58.0399820141948,-42.7345941518082,
-216.426471773175));
#229271=CARTESIAN_POINT('Ctrl Pts',(60.2132186858487,-45.1415311212291,
-213.071269036894));
#229272=CARTESIAN_POINT('Ctrl Pts',(47.0914518599014,-28.7082056053768,
-233.076532045377));
#229273=CARTESIAN_POINT('Ctrl Pts',(49.2577871721353,-30.9207984180132,
-229.722627951761));
#229274=CARTESIAN_POINT('Ctrl Pts',(51.4233225017517,-33.1352914201321,
-226.36927473658));
#229275=CARTESIAN_POINT('Ctrl Pts',(53.588559980291,-35.3505224606949,-223.016143793358));
#229276=CARTESIAN_POINT('Ctrl Pts',(55.7537974588302,-37.5657535012578,
-219.663012850137));
#229277=CARTESIAN_POINT('Ctrl Pts',(57.9187078478837,-39.7817869473385,
-216.310121456173));
#229278=CARTESIAN_POINT('Ctrl Pts',(60.0834610972678,-41.9982150734171,
-212.9573503068));
#229279=CARTESIAN_POINT('Ctrl Pts',(47.338918326904,-26.7547399443242,-232.989202284253));
#229280=CARTESIAN_POINT('Ctrl Pts',(49.5169190710851,-28.779613867576,-229.63849750905));
#229281=CARTESIAN_POINT('Ctrl Pts',(51.6953679974136,-30.8032553785755,
-226.287341083189));
#229282=CARTESIAN_POINT('Ctrl Pts',(53.8739882225852,-32.826417079771,-222.936006744139));
#229283=CARTESIAN_POINT('Ctrl Pts',(56.0526084477568,-34.8495787809666,
-219.584672405089));
#229284=CARTESIAN_POINT('Ctrl Pts',(58.2314156201025,-36.8722190976995,
-216.233145260744));
#229285=CARTESIAN_POINT('Ctrl Pts',(60.4103139494413,-38.8946025877681,
-212.88152253822));
#229286=CARTESIAN_POINT('Ctrl Pts',(47.4007849436546,-26.2663735290611,
-232.967369843972));
#229287=CARTESIAN_POINT('Ctrl Pts',(49.5817020458226,-28.2443177299668,
-229.617464898372));
#229288=CARTESIAN_POINT('Ctrl Pts',(51.7633793713291,-30.2202463681864,
-226.266857669841));
#229289=CARTESIAN_POINT('Ctrl Pts',(53.9453452831587,-32.19539073454,-222.915972481834));
#229290=CARTESIAN_POINT('Ctrl Pts',(56.1273111949884,-34.1705351008938,
-219.565087293826));
#229291=CARTESIAN_POINT('Ctrl Pts',(58.3095925631572,-36.1448271352898,
-216.213901211887));
#229292=CARTESIAN_POINT('Ctrl Pts',(60.4920271624846,-38.1186994663558,
-212.862565596074));
#229293=CARTESIAN_POINT('Ctrl Pts',(47.4827081594745,-25.7820909390022,
-232.948908323096));
#229294=CARTESIAN_POINT('Ctrl Pts',(49.667931620883,-27.7127600601,-229.599541574634));
#229295=CARTESIAN_POINT('Ctrl Pts',(51.854254699843,-29.6406887254791,-226.249310199414));
#229296=CARTESIAN_POINT('Ctrl Pts',(54.0409905357308,-31.5675524127984,
-222.898733386289));
#229297=CARTESIAN_POINT('Ctrl Pts',(56.2277263716187,-33.4944161001178,
-219.548156573164));
#229298=CARTESIAN_POINT('Ctrl Pts',(58.4149145994856,-35.4201220699693,
-216.197206631876));
#229299=CARTESIAN_POINT('Ctrl Pts',(60.6023211750695,-37.3452584113098,
-212.84607035725));
#229300=CARTESIAN_POINT('Ctrl Pts',(47.5841424907316,-25.3031332383162,
-232.93329091056));
#229301=CARTESIAN_POINT('Ctrl Pts',(49.7751430286533,-27.1862918963392,
-229.584271284343));
#229302=CARTESIAN_POINT('Ctrl Pts',(51.9676091114587,-29.0660086976874,
-226.234288856273));
#229303=CARTESIAN_POINT('Ctrl Pts',(54.1606184685044,-30.9443917197372,
-222.883917182185));
#229304=CARTESIAN_POINT('Ctrl Pts',(56.3536278255502,-32.822774741787,-219.533545508098));
#229305=CARTESIAN_POINT('Ctrl Pts',(58.5472344262499,-34.6997069346566,
-216.182754549711));
#229306=CARTESIAN_POINT('Ctrl Pts',(60.7411272633344,-36.5759265044021,
-212.831752983035));
#229307=CARTESIAN_POINT('Ctrl Pts',(47.6095010735459,-25.1833938131447,
-232.929386557426));
#229308=CARTESIAN_POINT('Ctrl Pts',(49.8019458805959,-27.054674855399,-229.58045371177));
#229309=CARTESIAN_POINT('Ctrl Pts',(51.9959477143626,-28.9223386907395,
-226.230533520487));
#229310=CARTESIAN_POINT('Ctrl Pts',(54.1905254516978,-30.7886015464719,
-222.88021313116));
#229311=CARTESIAN_POINT('Ctrl Pts',(56.3851031890331,-32.6548644022043,
-219.529892741831));
#229312=CARTESIAN_POINT('Ctrl Pts',(58.5803143829409,-34.5196031508285,
-216.179141529169));
#229313=CARTESIAN_POINT('Ctrl Pts',(60.7758287854006,-36.3835935276752,
-212.828173639481));
#229314=CARTESIAN_POINT('Ctrl Pts',(47.6360799530631,-25.0639872883753,
-232.925661119858));
#229315=CARTESIAN_POINT('Ctrl Pts',(49.8300607835295,-26.9233759839715,
-229.576802907687));
#229316=CARTESIAN_POINT('Ctrl Pts',(52.0256918558292,-28.7789735949605,
-226.226936900208));
#229317=CARTESIAN_POINT('Ctrl Pts',(54.2219318772968,-30.6331037731025,
-222.876661247257));
#229318=CARTESIAN_POINT('Ctrl Pts',(56.4181718987644,-32.4872339512444,
-219.526385594307));
#229319=CARTESIAN_POINT('Ctrl Pts',(58.6150821083144,-34.339767514325,-216.175669238136));
#229320=CARTESIAN_POINT('Ctrl Pts',(60.8123126810755,-36.1915173917436,
-212.824730931321));
#229321=CARTESIAN_POINT('Ctrl Pts',(47.6638721879803,-24.9449332806664,
-232.922108625287));
#229322=CARTESIAN_POINT('Ctrl Pts',(49.8594817505659,-26.7924165735007,
-229.57331360468));
#229323=CARTESIAN_POINT('Ctrl Pts',(52.0568366301129,-28.6359358440905,
-226.223494218563));
#229324=CARTESIAN_POINT('Ctrl Pts',(54.2548339484627,-30.4779217969194,
-222.873257153795));
#229325=CARTESIAN_POINT('Ctrl Pts',(56.4528312668125,-32.3199077497483,
-219.523020089027));
#229326=CARTESIAN_POINT('Ctrl Pts',(58.6515360594894,-34.1602251482123,
-216.172334004182));
#229327=CARTESIAN_POINT('Ctrl Pts',(60.85057856534,-35.9997238912687,-212.821421441686));
#229328=CARTESIAN_POINT('Ctrl Pts',(47.6656092026626,-24.9374924051846,
-232.921886594377));
#229329=CARTESIAN_POINT('Ctrl Pts',(49.8613205610057,-26.7842316103463,
-229.573095523243));
#229330=CARTESIAN_POINT('Ctrl Pts',(52.0587831785056,-28.6269959846611,
-226.223279050959));
#229331=CARTESIAN_POINT('Ctrl Pts',(54.2568903279106,-30.468222923408,-222.873044397953));
#229332=CARTESIAN_POINT('Ctrl Pts',(56.4549974773155,-32.3094498621548,
-219.522809744947));
#229333=CARTESIAN_POINT('Ctrl Pts',(58.6538144314378,-34.1490037503303,
-216.17212555206));
#229334=CARTESIAN_POINT('Ctrl Pts',(60.8529701831065,-35.987736797489,-212.821214598585));
#229335=CARTESIAN_POINT('Ctrl Pts',(47.6673509571934,-24.9300529067585,
-232.921665239305));
#229336=CARTESIAN_POINT('Ctrl Pts',(49.8631644734026,-26.7760479732408,
-229.5728780729));
#229337=CARTESIAN_POINT('Ctrl Pts',(52.0607351982457,-28.6180574039478,
-226.223064484881));
#229338=CARTESIAN_POINT('Ctrl Pts',(54.2589525498347,-30.4585252835005,
-222.872832219598));
#229339=CARTESIAN_POINT('Ctrl Pts',(56.4571699014236,-32.2989931630532,
-219.522599954314));
#229340=CARTESIAN_POINT('Ctrl Pts',(58.6560993902921,-34.1377834980502,
-216.171917635457));
#229341=CARTESIAN_POINT('Ctrl Pts',(60.8553687618446,-35.9757508077661,
-212.821008275995));
#229342=CARTESIAN_POINT('Ctrl Pts',(47.6690974499491,-24.9226147901915,
-232.921444558725));
#229343=CARTESIAN_POINT('Ctrl Pts',(49.8650134863522,-26.7678656673941,
-229.572661252457));
#229344=CARTESIAN_POINT('Ctrl Pts',(52.0626926881854,-28.6091201074371,
-226.222850519243));
#229345=CARTESIAN_POINT('Ctrl Pts',(54.261020613352,-30.4488288829175,-222.87262061773));
#229346=CARTESIAN_POINT('Ctrl Pts',(56.4593485385187,-32.2885376583978,
-219.522390716218));
#229347=CARTESIAN_POINT('Ctrl Pts',(58.65839093571,-34.1265643975113,-216.171710253535));
#229348=CARTESIAN_POINT('Ctrl Pts',(60.8577743014912,-35.9637659284024,
-212.820802473134));
#229349=CARTESIAN_POINT('Ctrl Pts',(47.6708439427048,-24.9151766736244,
-232.921223878144));
#229350=CARTESIAN_POINT('Ctrl Pts',(49.8668624993017,-26.7596833615473,
-229.572444432014));
#229351=CARTESIAN_POINT('Ctrl Pts',(52.064650178125,-28.6001828109265,-226.222636553605));
#229352=CARTESIAN_POINT('Ctrl Pts',(54.2630886768694,-30.4391324823344,
-222.872409015864));
#229353=CARTESIAN_POINT('Ctrl Pts',(56.4615271756139,-32.2780821537422,
-219.522181478123));
#229354=CARTESIAN_POINT('Ctrl Pts',(58.6606824811278,-34.1153452969724,
-216.171502871612));
#229355=CARTESIAN_POINT('Ctrl Pts',(60.8601798411379,-35.9517810490386,
-212.820596670274));
#229356=CARTESIAN_POINT('Ctrl Pts',(47.6712594337893,-24.9108968675569,
-232.921857349187));
#229357=CARTESIAN_POINT('Ctrl Pts',(49.8674442055454,-26.7545468321646,
-229.573062291402));
#229358=CARTESIAN_POINT('Ctrl Pts',(52.0653826207377,-28.5942132778735,
-226.223242591862));
#229359=CARTESIAN_POINT('Ctrl Pts',(54.2639659675545,-30.4323399214299,
-222.873005200592));
#229360=CARTESIAN_POINT('Ctrl Pts',(56.4625493143714,-32.2704665649863,
-219.522767809321));
#229361=CARTESIAN_POINT('Ctrl Pts',(58.6618430388141,-34.1069173291204,
-216.172081363551));
#229362=CARTESIAN_POINT('Ctrl Pts',(60.8614757011049,-35.9425461532316,
-212.821168459392));
#229363=CARTESIAN_POINT('Ctrl Pts',(47.6722605345507,-24.9052129322023,
-232.922111326828));
#229364=CARTESIAN_POINT('Ctrl Pts',(49.8685827056453,-26.7480556997355,
-229.573309285042));
#229365=CARTESIAN_POINT('Ctrl Pts',(52.0666525755381,-28.5869233597964,
-226.223484274919));
#229366=CARTESIAN_POINT('Ctrl Pts',(54.2653650437259,-30.4242549380612,
-222.873242451443));
#229367=CARTESIAN_POINT('Ctrl Pts',(56.4640775119137,-32.2615865163259,
-219.523000627968));
#229368=CARTESIAN_POINT('Ctrl Pts',(58.6634978294311,-34.0972461434794,
-216.172310647723));
#229369=CARTESIAN_POINT('Ctrl Pts',(60.8632558396737,-35.9320858909674,
-212.821394718674));
#229370=CARTESIAN_POINT('Ctrl Pts',(47.6742627360736,-24.8938450614933,
-232.922619282109));
#229371=CARTESIAN_POINT('Ctrl Pts',(49.8708597058451,-26.7350734348772,
-229.573803272322));
#229372=CARTESIAN_POINT('Ctrl Pts',(52.069192485139,-28.5723435236424,-226.223967641033));
#229373=CARTESIAN_POINT('Ctrl Pts',(54.2681631960686,-30.4080849713239,
-222.873716953146));
#229374=CARTESIAN_POINT('Ctrl Pts',(56.4671339069982,-32.2438264190054,
-219.523466265261));
#229375=CARTESIAN_POINT('Ctrl Pts',(58.666807410665,-34.0779037721973,-216.172769216067));
#229376=CARTESIAN_POINT('Ctrl Pts',(60.8668161168113,-35.9111653664389,
-212.821847237238));
#229377=CARTESIAN_POINT('Ctrl Pts',(47.6762483602964,-24.8824767178353,
-232.923127796013));
#229378=CARTESIAN_POINT('Ctrl Pts',(49.8731187515493,-26.722089328055,-229.574297740375));
#229379=CARTESIAN_POINT('Ctrl Pts',(52.0717130787027,-28.557760578718,-226.224451450989));
#229380=CARTESIAN_POINT('Ctrl Pts',(54.2709406860775,-30.3919106496837,
-222.874191872023));
#229381=CARTESIAN_POINT('Ctrl Pts',(56.4701682934522,-32.2260607206496,
-219.523932293058));
#229382=CARTESIAN_POINT('Ctrl Pts',(58.6700936511245,-34.0585545809213,
-216.173228160698));
#229383=CARTESIAN_POINT('Ctrl Pts',(60.8703517304133,-35.8902368104956,
-212.822300122054));
#229384=CARTESIAN_POINT('Ctrl Pts',(47.6782174267913,-24.8711079134889,
-232.92363686464));
#229385=CARTESIAN_POINT('Ctrl Pts',(49.8753598495424,-26.7091034156505,
-229.574792687293));
#229386=CARTESIAN_POINT('Ctrl Pts',(52.0742143523489,-28.5431745827215,
-226.224935704284));
#229387=CARTESIAN_POINT('Ctrl Pts',(54.2736974997456,-30.3757320511356,
-222.874667208678));
#229388=CARTESIAN_POINT('Ctrl Pts',(56.4731806471424,-32.2082895195496,
-219.524398713072));
#229389=CARTESIAN_POINT('Ctrl Pts',(58.6733565172052,-34.0391986871267,
-216.173687484148));
#229390=CARTESIAN_POINT('Ctrl Pts',(60.8738626376389,-35.8693003593042,
-212.822753376317));
#229391=CARTESIAN_POINT('Ctrl Pts',(47.6821555597811,-24.8483703047961,
-232.924655001894));
#229392=CARTESIAN_POINT('Ctrl Pts',(49.8798420455288,-26.6831315908415,
-229.575782581129));
#229393=CARTESIAN_POINT('Ctrl Pts',(52.0792168996413,-28.5140025907287,
-226.225904210874));
#229394=CARTESIAN_POINT('Ctrl Pts',(54.2792111270821,-30.3433748540391,
-222.875617881988));
#229395=CARTESIAN_POINT('Ctrl Pts',(56.4792053545228,-32.1727471173495,
-219.525331553101));
#229396=CARTESIAN_POINT('Ctrl Pts',(58.6798822493665,-34.0004868995374,
-216.174606131045));
#229397=CARTESIAN_POINT('Ctrl Pts',(60.88088445209,-35.8274274569215,-212.823659884843));
#229398=CARTESIAN_POINT('Ctrl Pts',(47.6860274619745,-24.8256308534282,
-232.925675358015));
#229399=CARTESIAN_POINT('Ctrl Pts',(49.8842524507179,-26.657152543721,-229.576774390365));
#229400=CARTESIAN_POINT('Ctrl Pts',(52.0841421672651,-28.4848183944506,
-226.22687449075));
#229401=CARTESIAN_POINT('Ctrl Pts',(54.2846420490225,-30.3110005493018,
-222.876570226337));
#229402=CARTESIAN_POINT('Ctrl Pts',(56.4851419307799,-32.1371827041529,
-219.526265961925));
#229403=CARTESIAN_POINT('Ctrl Pts',(58.6863144839206,-33.9617483018504,
-216.17552629313));
#229404=CARTESIAN_POINT('Ctrl Pts',(60.887807440924,-35.7855229735214,-212.824567871073));
#229405=CARTESIAN_POINT('Ctrl Pts',(47.6898332885707,-24.8028896565292,
-232.926697902178));
#229406=CARTESIAN_POINT('Ctrl Pts',(49.8885911188174,-26.6311665651389,
-229.577768100455));
#229407=CARTESIAN_POINT('Ctrl Pts',(52.0889901241519,-28.455622455455,-226.227846540711));
#229408=CARTESIAN_POINT('Ctrl Pts',(54.2899901539046,-30.2786097609959,
-222.877524247479));
#229409=CARTESIAN_POINT('Ctrl Pts',(56.4909901836572,-32.1015970665369,
-219.527201954246));
#229410=CARTESIAN_POINT('Ctrl Pts',(58.6926529531334,-33.9229838341469,
-216.176447991634));
#229411=CARTESIAN_POINT('Ctrl Pts',(60.8946312627443,-35.7435879987355,
-212.825477361568));
#229412=CARTESIAN_POINT('Ctrl Pts',(47.6974449417632,-24.7574072627311,
-232.928742990504));
#229413=CARTESIAN_POINT('Ctrl Pts',(49.8972684550162,-26.5791946079747,
-229.579755520635));
#229414=CARTESIAN_POINT('Ctrl Pts',(52.0986860379256,-28.3972305774635,
-226.229790640633));
#229415=CARTESIAN_POINT('Ctrl Pts',(54.3006863636687,-30.2138281843841,
-222.879432289762));
#229416=CARTESIAN_POINT('Ctrl Pts',(56.5026866894118,-32.0304257913048,
-219.529073938891));
#229417=CARTESIAN_POINT('Ctrl Pts',(58.705329891559,-33.8454548987401,-216.178291388644));
#229418=CARTESIAN_POINT('Ctrl Pts',(60.9082789063849,-35.6597180491639,
-212.827296342558));
#229419=CARTESIAN_POINT('Ctrl Pts',(47.7047922944592,-24.7119178879782,
-232.930796830484));
#229420=CARTESIAN_POINT('Ctrl Pts',(49.9056588436001,-26.5271949252194,
-229.581750543243));
#229421=CARTESIAN_POINT('Ctrl Pts',(52.1080727087613,-28.3387917286268,
-226.231741819771));
#229422=CARTESIAN_POINT('Ctrl Pts',(54.3110513046474,-30.1489806733496,
-222.881347038));
#229423=CARTESIAN_POINT('Ctrl Pts',(56.5140299005335,-31.9591696180724,
-219.530952256228));
#229424=CARTESIAN_POINT('Ctrl Pts',(58.7176317671225,-33.7678224828936,
-216.180140930006));
#229425=CARTESIAN_POINT('Ctrl Pts',(60.9215298801705,-35.5757261336416,
-212.829121339267));
#229426=CARTESIAN_POINT('Ctrl Pts',(47.7118765658424,-24.6664222949089,
-232.932859181476));
#229427=CARTESIAN_POINT('Ctrl Pts',(49.9137627052303,-26.4751698404963,
-229.583753063685));
#229428=CARTESIAN_POINT('Ctrl Pts',(52.1171498878757,-28.280309601158,-226.233700065929));
#229429=CARTESIAN_POINT('Ctrl Pts',(54.321084090016,-30.084072222256,-222.883268552734));
#229430=CARTESIAN_POINT('Ctrl Pts',(56.5250182921564,-31.887834843354,-219.53283703954));
#229431=CARTESIAN_POINT('Ctrl Pts',(58.7295564557497,-33.6900941117383,
-216.181996801466));
#229432=CARTESIAN_POINT('Ctrl Pts',(60.9343814743951,-35.4916209740569,
-212.830952580145));
#229433=CARTESIAN_POINT('Ctrl Pts',(47.740213651375,-24.4844399226315,-232.941108585445));
#229434=CARTESIAN_POINT('Ctrl Pts',(49.9461781517511,-26.2670695016037,
-229.591763145452));
#229435=CARTESIAN_POINT('Ctrl Pts',(52.1534586043331,-28.0463810912831,
-226.241533050557));
#229436=CARTESIAN_POINT('Ctrl Pts',(54.3612152314905,-29.8244384178816,
-222.890954611672));
#229437=CARTESIAN_POINT('Ctrl Pts',(56.5689718586478,-31.6024957444801,
-219.540376172787));
#229438=CARTESIAN_POINT('Ctrl Pts',(58.7772552102583,-33.379180627117,-216.189420287308));
#229439=CARTESIAN_POINT('Ctrl Pts',(60.9857878512938,-35.1552003357181,
-212.838277543654));
#229440=CARTESIAN_POINT('Ctrl Pts',(47.764342072931,-24.3023583702358,-232.949493972115));
#229441=CARTESIAN_POINT('Ctrl Pts',(49.974009394549,-26.0585628024136,-229.599892861619));
#229442=CARTESIAN_POINT('Ctrl Pts',(52.1848154405255,-27.8117601296424,
-226.249478738948));
#229443=CARTESIAN_POINT('Ctrl Pts',(54.3960316866775,-29.5638295270311,
-222.898748539061));
#229444=CARTESIAN_POINT('Ctrl Pts',(56.6072479328295,-31.3158989244199,
-219.548018339173));
#229445=CARTESIAN_POINT('Ctrl Pts',(58.8189184722057,-33.0667317389572,
-216.196944624725));
#229446=CARTESIAN_POINT('Ctrl Pts',(61.0308035579046,-34.8169676574521,
-212.845701979688));
#229447=CARTESIAN_POINT('Ctrl Pts',(47.7843348584855,-24.1202237497555,
-232.95800139794));
#229448=CARTESIAN_POINT('Ctrl Pts',(49.99728150262,-25.8497978524297,-229.608138122646));
#229449=CARTESIAN_POINT('Ctrl Pts',(52.2112045262045,-27.5766829623168,
-226.257539270556));
#229450=CARTESIAN_POINT('Ctrl Pts',(54.4254782083431,-29.3025655601605,
-222.906657351959));
#229451=CARTESIAN_POINT('Ctrl Pts',(56.6397518904817,-31.0284481580042,
-219.555775433364));
#229452=CARTESIAN_POINT('Ctrl Pts',(58.8544142415175,-32.7532300084283,
-216.204585123186));
#229453=CARTESIAN_POINT('Ctrl Pts',(61.0692598838066,-34.4774822060492,
-212.853243959114));
#229454=CARTESIAN_POINT('Ctrl Pts',(47.8643060007033,-23.3916852678342,
-232.992031101241));
#229455=CARTESIAN_POINT('Ctrl Pts',(50.090369934904,-25.0147380524944,-229.641119166754));
#229456=CARTESIAN_POINT('Ctrl Pts',(52.3167608689203,-26.6363742930146,
-226.289781396988));
#229457=CARTESIAN_POINT('Ctrl Pts',(54.5432642950053,-28.2575096926779,
-222.938292603557));
#229458=CARTESIAN_POINT('Ctrl Pts',(56.7697677210903,-29.8786450923411,
-219.586803810126));
#229459=CARTESIAN_POINT('Ctrl Pts',(58.9963973187644,-31.499223086313,-216.235147117033));
#229460=CARTESIAN_POINT('Ctrl Pts',(61.2230851874141,-33.1195404004377,
-212.883411876817));
#229461=CARTESIAN_POINT('Ctrl Pts',(47.878298880158,-22.6624540792437,-233.028057892109));
#229462=CARTESIAN_POINT('Ctrl Pts',(50.1105261899139,-24.1755656136661,
-229.675981641008));
#229463=CARTESIAN_POINT('Ctrl Pts',(52.3426487730065,-25.6886770024113,
-226.323884260853));
#229464=CARTESIAN_POINT('Ctrl Pts',(54.5747380925437,-27.201784204638,-222.971780574238));
#229465=CARTESIAN_POINT('Ctrl Pts',(56.8068274120809,-28.7148914068648,
-219.619676887624));
#229466=CARTESIAN_POINT('Ctrl Pts',(59.0388786006661,-30.2279951799507,
-216.267565846653));
#229467=CARTESIAN_POINT('Ctrl Pts',(61.2709129905723,-31.7410962361218,
-212.915451703421));
#229468=CARTESIAN_POINT('Ctrl Pts',(47.8281547001989,-21.9381226823642,
-233.066054879848));
#229469=CARTESIAN_POINT('Ctrl Pts',(50.0590295861697,-23.3420565686501,
-229.712518150776));
#229470=CARTESIAN_POINT('Ctrl Pts',(52.2896542767201,-24.7475525298228,
-226.359471317301));
#229471=CARTESIAN_POINT('Ctrl Pts',(54.5201844975327,-26.1536136226082,
-223.006599089445));
#229472=CARTESIAN_POINT('Ctrl Pts',(56.7507147183453,-27.5596747153937,
-219.653726861588));
#229473=CARTESIAN_POINT('Ctrl Pts',(58.9811415508881,-28.9663610919618,
-216.301048580499));
#229474=CARTESIAN_POINT('Ctrl Pts',(61.2115183316506,-30.3733436736124,
-212.948461459071));
#229475=CARTESIAN_POINT('Ctrl Pts',(47.8030826102193,-21.5759569839245,
-233.085053373718));
#229476=CARTESIAN_POINT('Ctrl Pts',(50.0332812842976,-22.9253020461421,
-229.730786405659));
#229477=CARTESIAN_POINT('Ctrl Pts',(52.2631570285769,-24.2769902935286,
-226.377264845526));
#229478=CARTESIAN_POINT('Ctrl Pts',(54.4929077000272,-25.6295283315933,
-223.024008347048));
#229479=CARTESIAN_POINT('Ctrl Pts',(56.7226583714774,-26.9820663696581,
-219.67075184857));
#229480=CARTESIAN_POINT('Ctrl Pts',(58.9522730259992,-28.3355440479673,
-216.317789947423));
#229481=CARTESIAN_POINT('Ctrl Pts',(61.1818210021897,-29.6894673923576,
-212.964966336897));
#229482=CARTESIAN_POINT('Ctrl Pts',(47.761964930595,-21.2148494647643,-233.104496710832));
#229483=CARTESIAN_POINT('Ctrl Pts',(49.9896217363213,-22.5099538605863,
-229.749470483377));
#229484=CARTESIAN_POINT('Ctrl Pts',(52.2169611837896,-23.8081676354522,
-226.395455605453));
#229485=CARTESIAN_POINT('Ctrl Pts',(54.4441695190511,-25.1075159192911,
-223.041799887511));
#229486=CARTESIAN_POINT('Ctrl Pts',(56.6713778543125,-26.4068642031302,
-219.688144169568));
#229487=CARTESIAN_POINT('Ctrl Pts',(58.8984458054575,-27.7074649475142,
-216.33488775531));
#229488=CARTESIAN_POINT('Ctrl Pts',(61.1254428175118,-29.0086615021396,
-212.981818623129));
#229489=CARTESIAN_POINT('Ctrl Pts',(47.7047603197491,-20.8556613435138,
-233.124453388251));
#229490=CARTESIAN_POINT('Ctrl Pts',(49.9281792692869,-22.0972013968281,
-229.768548954079));
#229491=CARTESIAN_POINT('Ctrl Pts',(52.1513679132233,-23.3426563590316,
-226.413955402434));
#229492=CARTESIAN_POINT('Ctrl Pts',(54.374445390284,-24.58956219214,-223.059830549548));
#229493=CARTESIAN_POINT('Ctrl Pts',(56.5975228673448,-25.8364680252484,
-219.705705696663));
#229494=CARTESIAN_POINT('Ctrl Pts',(58.8204852380101,-27.0849692159872,
-216.352100946617));
#229495=CARTESIAN_POINT('Ctrl Pts',(61.0433852523227,-28.3342355002131,
-212.998740881412));
#229496=CARTESIAN_POINT('Ctrl Pts',(47.6761580143262,-20.6760672828885,
-233.134431726961));
#229497=CARTESIAN_POINT('Ctrl Pts',(49.8974580357697,-21.890825164949,-229.77808818943));
#229498=CARTESIAN_POINT('Ctrl Pts',(52.11857127794,-23.1099007208212,-226.423205300924));
#229499=CARTESIAN_POINT('Ctrl Pts',(54.3395833259005,-24.3305853285644,
-223.068845880567));
#229500=CARTESIAN_POINT('Ctrl Pts',(56.5605953738609,-25.5512699363075,
-219.714486460211));
#229501=CARTESIAN_POINT('Ctrl Pts',(58.7815049542864,-26.7737213502237,
-216.36070754227));
#229502=CARTESIAN_POINT('Ctrl Pts',(61.0023564697282,-27.9970224992499,
-213.007202010553));
#229503=CARTESIAN_POINT('Ctrl Pts',(47.6435322539531,-20.4969288626005,
-233.144529615889));
#229504=CARTESIAN_POINT('Ctrl Pts',(49.8622910488621,-21.6850934492459,
-229.78772367565));
#229505=CARTESIAN_POINT('Ctrl Pts',(52.0809282278205,-22.8779807020543,
-226.432534208105));
#229506=CARTESIAN_POINT('Ctrl Pts',(54.2994812233516,-24.0726404406297,
-223.077926048768));
#229507=CARTESIAN_POINT('Ctrl Pts',(56.5180342188827,-25.2673001792052,
-219.723317889431));
#229508=CARTESIAN_POINT('Ctrl Pts',(58.7365053698609,-26.4639027275198,
-216.369353764958));
#229509=CARTESIAN_POINT('Ctrl Pts',(60.9549262461142,-27.6614430666891,
-213.015693423744));
#229510=CARTESIAN_POINT('Ctrl Pts',(47.6068679344032,-20.3182727557442,
-233.154731928786));
#229511=CARTESIAN_POINT('Ctrl Pts',(49.8226916006283,-21.4801411515154,
-229.797451628545));
#229512=CARTESIAN_POINT('Ctrl Pts',(52.0384807122269,-22.6471217996642,
-226.441944079533));
#229513=CARTESIAN_POINT('Ctrl Pts',(54.254210599501,-23.8160385972306,-223.087077428057));
#229514=CARTESIAN_POINT('Ctrl Pts',(56.4699404867752,-24.984955394797,-219.732210776581));
#229515=CARTESIAN_POINT('Ctrl Pts',(58.6856178886063,-26.1559896665116,
-216.378053163374));
#229516=CARTESIAN_POINT('Ctrl Pts',(60.9012568321316,-27.3280508969457,
-213.024230834597));
#229517=CARTESIAN_POINT('Ctrl Pts',(47.6022848944595,-20.2959407423872,
-233.156007217897));
#229518=CARTESIAN_POINT('Ctrl Pts',(49.8177416695991,-21.4545221142991,
-229.798667622657));
#229519=CARTESIAN_POINT('Ctrl Pts',(52.0331747727777,-22.6182644368655,
-226.443120313462));
#229520=CARTESIAN_POINT('Ctrl Pts',(54.2485517715197,-23.7839633668058,
-223.088221350469));
#229521=CARTESIAN_POINT('Ctrl Pts',(56.4639287702618,-24.949662296746,-219.733322387475));
#229522=CARTESIAN_POINT('Ctrl Pts',(58.6792569534495,-26.1175005338857,
-216.379140588177));
#229523=CARTESIAN_POINT('Ctrl Pts',(60.8945481553838,-27.2863768757278,
-213.025298010954));
#229524=CARTESIAN_POINT('Ctrl Pts',(47.5976387390489,-20.2736162584332,
-233.157284142165));
#229525=CARTESIAN_POINT('Ctrl Pts',(49.8127224773379,-21.4289152517019,
-229.799885067328));
#229526=CARTESIAN_POINT('Ctrl Pts',(52.0277937637733,-22.5894236531258,
-226.444297819366));
#229527=CARTESIAN_POINT('Ctrl Pts',(54.2428121888309,-23.7519091227437,
-223.089366393269));
#229528=CARTESIAN_POINT('Ctrl Pts',(56.4578306138885,-24.9143945923615,
-219.734434967173));
#229529=CARTESIAN_POINT('Ctrl Pts',(58.6728040284611,-26.079041180752,-216.380228852809));
#229530=CARTESIAN_POINT('Ctrl Pts',(60.8877420013067,-27.2447370368634,
-213.02636591529));
#229531=CARTESIAN_POINT('Ctrl Pts',(47.592929427391,-20.2512993504693,-233.15856267521));
#229532=CARTESIAN_POINT('Ctrl Pts',(49.8076340463092,-21.4033208239495,
-229.801103960199));
#229533=CARTESIAN_POINT('Ctrl Pts',(52.0223377673611,-22.5605998880764,
-226.445476607082));
#229534=CARTESIAN_POINT('Ctrl Pts',(54.2369919941413,-23.7198764736633,
-223.090512575624));
#229535=CARTESIAN_POINT('Ctrl Pts',(56.4516462209215,-24.8791530592503,
-219.735548544168));
#229536=CARTESIAN_POINT('Ctrl Pts',(58.6662593777807,-26.0406125417595,
-216.381317991529));
#229537=CARTESIAN_POINT('Ctrl Pts',(60.880838695562,-27.2031324672545,-213.027434586363));
#229538=CARTESIAN_POINT('Ctrl Pts',(47.5917520994765,-20.2457201234783,
-233.158882308471));
#229539=CARTESIAN_POINT('Ctrl Pts',(49.8063619385521,-21.3969222170114,
-229.801408683416));
#229540=CARTESIAN_POINT('Ctrl Pts',(52.0209737682581,-22.553393946814,-226.445771304011));
#229541=CARTESIAN_POINT('Ctrl Pts',(54.235536945469,-23.7118683113933,-223.090799121214));
#229542=CARTESIAN_POINT('Ctrl Pts',(56.4501001226798,-24.8703426759725,
-219.735826938416));
#229543=CARTESIAN_POINT('Ctrl Pts',(58.6646232151106,-26.0310053820113,
-216.38159027621));
#229544=CARTESIAN_POINT('Ctrl Pts',(60.8791128691258,-27.1927313248522,
-213.027701754131));
#229545=CARTESIAN_POINT('Ctrl Pts',(47.590570824284,-20.2401413699817,-233.159202042285));
#229546=CARTESIAN_POINT('Ctrl Pts',(49.805085503368,-21.3905243872477,-229.801713497152));
#229547=CARTESIAN_POINT('Ctrl Pts',(52.0196050824424,-22.5461890692189,
-226.44606608106));
#229548=CARTESIAN_POINT('Ctrl Pts',(54.23407685855,-23.7038614988106,-223.091085738033));
#229549=CARTESIAN_POINT('Ctrl Pts',(56.4485486346576,-24.8615339284022,
-219.736105395004));
#229550=CARTESIAN_POINT('Ctrl Pts',(58.6629813195933,-26.0214001419017,
-216.381862615529));
#229551=CARTESIAN_POINT('Ctrl Pts',(60.8773809707203,-27.1823323867845,
-213.027968969829));
#229552=CARTESIAN_POINT('Ctrl Pts',(47.5893856011509,-20.2345630906963,
-233.159521876246));
#229553=CARTESIAN_POINT('Ctrl Pts',(49.8038047411002,-21.384127338717,-229.802018401381));
#229554=CARTESIAN_POINT('Ctrl Pts',(52.0182317111982,-22.5389852621582,
-226.446360938398));
#229555=CARTESIAN_POINT('Ctrl Pts',(54.2326117356213,-23.695856045427,-223.091372426396));
#229556=CARTESIAN_POINT('Ctrl Pts',(56.4469917600444,-24.8527268286958,
-219.736383914393));
#229557=CARTESIAN_POINT('Ctrl Pts',(58.661333695373,-26.0117968360436,-216.38213501004));
#229558=CARTESIAN_POINT('Ctrl Pts',(60.8756430054541,-27.1719356700459,
-213.028236234081));
#229559=CARTESIAN_POINT('Ctrl Pts',(47.5882003780178,-20.2289848114109,
-233.159841710208));
#229560=CARTESIAN_POINT('Ctrl Pts',(49.8025239788324,-21.3777302901863,
-229.80232330561));
#229561=CARTESIAN_POINT('Ctrl Pts',(52.016858339954,-22.5317814550976,-226.446655795734));
#229562=CARTESIAN_POINT('Ctrl Pts',(54.2311466126926,-23.6878505920434,
-223.091659114758));
#229563=CARTESIAN_POINT('Ctrl Pts',(56.4454348854312,-24.8439197289892,
-219.736662433782));
#229564=CARTESIAN_POINT('Ctrl Pts',(58.6596860711528,-26.0021935301855,
-216.382407404553));
#229565=CARTESIAN_POINT('Ctrl Pts',(60.8739050401878,-27.1615389533073,
-213.028503498334));
#229566=CARTESIAN_POINT('Ctrl Pts',(47.5869813026369,-20.2248085548944,
-233.160629240458));
#229567=CARTESIAN_POINT('Ctrl Pts',(49.8012014928958,-21.3726770899824,
-229.803070732654));
#229568=CARTESIAN_POINT('Ctrl Pts',(52.0154387418326,-22.5258822594507,
-226.447376788852));
#229569=CARTESIAN_POINT('Ctrl Pts',(54.2296316602861,-23.6811178430054,
-223.092358686209));
#229570=CARTESIAN_POINT('Ctrl Pts',(56.4438245787395,-24.8363534265602,
-219.737340583566));
#229571=CARTESIAN_POINT('Ctrl Pts',(58.6579824964894,-25.9938070865368,
-216.383069654941));
#229572=CARTESIAN_POINT('Ctrl Pts',(60.8721090250117,-27.1523390690596,
-213.029152473631));
#229573=CARTESIAN_POINT('Ctrl Pts',(47.5858317128383,-20.2171701221733,
-233.160261571908));
#229574=CARTESIAN_POINT('Ctrl Pts',(49.7999665889626,-21.3643065199923,
-229.802725125393));
#229575=CARTESIAN_POINT('Ctrl Pts',(52.0141165726974,-22.5167636487862,
-226.447045200389));
#229576=CARTESIAN_POINT('Ctrl Pts',(54.22822178586,-23.6712455217665,-223.092038389655));
#229577=CARTESIAN_POINT('Ctrl Pts',(56.4423269990226,-24.8257273947467,
-219.737031578921));
#229578=CARTESIAN_POINT('Ctrl Pts',(58.6563966485487,-25.9824210519681,
-216.382768874591));
#229579=CARTESIAN_POINT('Ctrl Pts',(60.8704347151645,-27.140190085957,-213.028858518708));
#229580=CARTESIAN_POINT('Ctrl Pts',(47.5835325332411,-20.2018932567312,
-233.159526234808));
#229581=CARTESIAN_POINT('Ctrl Pts',(49.7974967810963,-21.3475653800119,
-229.802033910872));
#229582=CARTESIAN_POINT('Ctrl Pts',(52.011472234427,-22.4985264274573,-226.446382023462));
#229583=CARTESIAN_POINT('Ctrl Pts',(54.2254020370079,-23.6515008792884,
-223.091397796547));
#229584=CARTESIAN_POINT('Ctrl Pts',(56.4393318395888,-24.8044753311196,
-219.73641356963));
#229585=CARTESIAN_POINT('Ctrl Pts',(58.6532249526671,-25.9596489828307,
-216.382167313891));
#229586=CARTESIAN_POINT('Ctrl Pts',(60.8670860954703,-27.1158921197517,
-213.028270608861));
#229587=CARTESIAN_POINT('Ctrl Pts',(47.5812532984532,-20.1866126886901,
-233.158794242262));
#229588=CARTESIAN_POINT('Ctrl Pts',(49.7950482868299,-21.3308210270913,
-229.801345761373));
#229589=CARTESIAN_POINT('Ctrl Pts',(52.0088506546361,-22.4802865538093,
-226.445721752729));
#229590=CARTESIAN_POINT('Ctrl Pts',(54.2226065119627,-23.6317541556473,
-223.090759984216));
#229591=CARTESIAN_POINT('Ctrl Pts',(56.4363623692893,-24.7832217574852,
-219.735798215704));
#229592=CARTESIAN_POINT('Ctrl Pts',(58.6500804360107,-25.9368759906632,
-216.38156832305));
#229593=CARTESIAN_POINT('Ctrl Pts',(60.8637661551428,-27.0915938204597,
-213.027685199469));
#229594=CARTESIAN_POINT('Ctrl Pts',(47.5789940164766,-20.1713284656181,
-233.15806557645));
#229595=CARTESIAN_POINT('Ctrl Pts',(49.7926211103158,-21.3140735095608,
-229.800660662664));
#229596=CARTESIAN_POINT('Ctrl Pts',(52.0062518326129,-22.4620440746829,
-226.445064375697));
#229597=CARTESIAN_POINT('Ctrl Pts',(54.2198352050027,-23.6120053955637,
-223.090124941524));
#229598=CARTESIAN_POINT('Ctrl Pts',(56.4334185773924,-24.7619667164447,
-219.735185507351));
#229599=CARTESIAN_POINT('Ctrl Pts',(58.6469630826069,-25.9141021151943,
-216.380971893111));
#229600=CARTESIAN_POINT('Ctrl Pts',(60.8604748729077,-27.0672952246279,
-213.027102282233));
#229601=CARTESIAN_POINT('Ctrl Pts',(47.5699568885701,-20.1101915733302,
-233.155150913204));
#229602=CARTESIAN_POINT('Ctrl Pts',(49.7829124042595,-21.2470834394385,
-229.797920267832));
#229603=CARTESIAN_POINT('Ctrl Pts',(51.9958565445205,-22.3890741581773,
-226.44243486757));
#229604=CARTESIAN_POINT('Ctrl Pts',(54.2087499771628,-23.5330103552298,
-223.087584770755));
#229605=CARTESIAN_POINT('Ctrl Pts',(56.421643409805,-24.6769465522823,-219.732734673941));
#229606=CARTESIAN_POINT('Ctrl Pts',(58.6344936689916,-25.8230066133188,
-216.378586173355));
#229607=CARTESIAN_POINT('Ctrl Pts',(60.847309743967,-26.9701008413005,-213.024770613288));
#229608=CARTESIAN_POINT('Ctrl Pts',(47.5612390015556,-20.0489962009945,
-233.152289471859));
#229609=CARTESIAN_POINT('Ctrl Pts',(49.7735447794099,-21.1800427364387,
-229.795228681509));
#229610=CARTESIAN_POINT('Ctrl Pts',(51.9858253784452,-22.3160625550462,
-226.43985165536));
#229611=CARTESIAN_POINT('Ctrl Pts',(54.1980522368575,-23.453982732959,-223.08508891153));
#229612=CARTESIAN_POINT('Ctrl Pts',(56.4102790952697,-24.5919029108718,
-219.730326167701));
#229613=CARTESIAN_POINT('Ctrl Pts',(58.6224588662923,-25.7318969799296,
-216.376241426438));
#229614=CARTESIAN_POINT('Ctrl Pts',(60.8346031435815,-26.87290171468,-213.022478817573));
#229615=CARTESIAN_POINT('Ctrl Pts',(47.552840900575,-19.9877453892004,-233.149480158731));
#229616=CARTESIAN_POINT('Ctrl Pts',(49.764518524335,-21.1129544864435,-229.792585026173));
#229617=CARTESIAN_POINT('Ctrl Pts',(51.976158307113,-22.2430122546447,-226.437313966284));
#229618=CARTESIAN_POINT('Ctrl Pts',(54.1877416326195,-23.3749253815565,
-223.082636672215));
#229619=CARTESIAN_POINT('Ctrl Pts',(56.399324958126,-24.5068385084684,-219.727959378147));
#229620=CARTESIAN_POINT('Ctrl Pts',(58.6108576613275,-25.6407757471239,
-216.373937091928));
#229621=CARTESIAN_POINT('Ctrl Pts',(60.8223537175678,-26.7757001729515,
-213.02022637406));
#229622=CARTESIAN_POINT('Ctrl Pts',(47.5360446986138,-19.8652437656123,
-233.143861532478));
#229623=CARTESIAN_POINT('Ctrl Pts',(49.7464660141853,-20.9787779864532,
-229.787297715501));
#229624=CARTESIAN_POINT('Ctrl Pts',(51.9568241644486,-22.0969116538416,
-226.432238588131));
#229625=CARTESIAN_POINT('Ctrl Pts',(54.1671204241435,-23.2168106787515,
-223.077732193586));
#229626=CARTESIAN_POINT('Ctrl Pts',(56.3774166838384,-24.3367097036616,
-219.723225799041));
#229627=CARTESIAN_POINT('Ctrl Pts',(58.5876552513978,-25.4585332815125,
-216.369328422911));
#229628=CARTESIAN_POINT('Ctrl Pts',(60.7978548655404,-26.5812970894946,
-213.015721487035));
#229629=CARTESIAN_POINT('Ctrl Pts',(47.5205275923637,-19.7425203876807,
-233.138451347457));
#229630=CARTESIAN_POINT('Ctrl Pts',(49.7297789491929,-20.8444113076799,
-229.782202077174));
#229631=CARTESIAN_POINT('Ctrl Pts',(51.9389463734439,-21.9506562752646,
-226.42734526098));
#229632=CARTESIAN_POINT('Ctrl Pts',(54.1480477377855,-23.0585770723389,
-223.073002160992));
#229633=CARTESIAN_POINT('Ctrl Pts',(56.3571491021271,-24.1664978694133,
-219.718659061004));
#229634=CARTESIAN_POINT('Ctrl Pts',(58.5661872185244,-25.276244433579,-216.364881382949));
#229635=CARTESIAN_POINT('Ctrl Pts',(60.7751846995537,-26.3868843615641,
-213.011373992336));
#229636=CARTESIAN_POINT('Ctrl Pts',(47.5062945476757,-19.6195995248629,
-233.133241732319));
#229637=CARTESIAN_POINT('Ctrl Pts',(49.7144600590333,-20.7098790140667,
-229.777291719128));
#229638=CARTESIAN_POINT('Ctrl Pts',(51.9225250540634,-21.8042698865183,
-226.422628306549));
#229639=CARTESIAN_POINT('Ctrl Pts',(54.1305210352282,-22.9002472192685,
-223.06844144768));
#229640=CARTESIAN_POINT('Ctrl Pts',(56.3385170163929,-23.9962245520186,
-219.714254588812));
#229641=CARTESIAN_POINT('Ctrl Pts',(58.5464456271153,-25.0939292676188,
-216.360591734734));
#229642=CARTESIAN_POINT('Ctrl Pts',(60.7543325255676,-26.1924804157199,
-213.007179917814));
#229643=CARTESIAN_POINT('Ctrl Pts',(47.3924301901722,-18.6362326223204,
-233.091564811217));
#229644=CARTESIAN_POINT('Ctrl Pts',(49.5919089377565,-19.6336206651606,
-229.73800885476));
#229645=CARTESIAN_POINT('Ctrl Pts',(51.7911544990196,-20.633178776548,-226.384892671102));
#229646=CARTESIAN_POINT('Ctrl Pts',(53.9903074147697,-21.6336083947046,
-223.031955741188));
#229647=CARTESIAN_POINT('Ctrl Pts',(56.1894603305198,-22.6340380128611,
-219.679018811274));
#229648=CARTESIAN_POINT('Ctrl Pts',(58.3885128958421,-23.6354079399365,
-216.326274549018));
#229649=CARTESIAN_POINT('Ctrl Pts',(60.5875151336786,-24.637248848966,-212.973627321642));
#229650=CARTESIAN_POINT('Ctrl Pts',(47.3611092111201,-17.6397302500457,
-233.062531430769));
#229651=CARTESIAN_POINT('Ctrl Pts',(49.5571768913406,-18.5464340199547,
-229.71043415307));
#229652=CARTESIAN_POINT('Ctrl Pts',(51.753139481442,-19.4535001698865,-226.358317180801));
#229653=CARTESIAN_POINT('Ctrl Pts',(53.9490641998496,-20.3607169575665,
-223.006196302843));
#229654=CARTESIAN_POINT('Ctrl Pts',(56.1449889182572,-21.2679337452465,
-219.654075424885));
#229655=CARTESIAN_POINT('Ctrl Pts',(58.3408717515618,-22.175311849639,-216.301949384044));
#229656=CARTESIAN_POINT('Ctrl Pts',(60.5367349311551,-23.0827722988975,
-212.949821974785));
#229657=CARTESIAN_POINT('Ctrl Pts',(47.4134504259477,-16.6473487128058,
-233.044455194982));
#229658=CARTESIAN_POINT('Ctrl Pts',(49.6106642054098,-17.4639704569693,
-229.692980964189));
#229659=CARTESIAN_POINT('Ctrl Pts',(51.808075938482,-18.2792435060293,-226.341309714209));
#229660=CARTESIAN_POINT('Ctrl Pts',(54.0055642141686,-19.0939722550291,
-222.989556757961));
#229661=CARTESIAN_POINT('Ctrl Pts',(56.2030524898552,-19.9087010040289,
-219.637803801712));
#229662=CARTESIAN_POINT('Ctrl Pts',(58.4006240585482,-20.7228430676927,
-216.285963294552));
#229663=CARTESIAN_POINT('Ctrl Pts',(60.5982364662104,-21.5366903458251,
-212.934078132851));
#229664=CARTESIAN_POINT('Ctrl Pts',(47.4396210333615,-16.1511579441859,
-233.035417077088));
#229665=CARTESIAN_POINT('Ctrl Pts',(49.6374078624443,-16.9227386754765,
-229.684254369749));
#229666=CARTESIAN_POINT('Ctrl Pts',(51.835544167002,-17.6921151741007,-226.332805980913));
#229667=CARTESIAN_POINT('Ctrl Pts',(54.0338142213281,-18.4605999037604,
-222.98123698552));
#229668=CARTESIAN_POINT('Ctrl Pts',(56.2320842756543,-19.2290846334201,
-219.629667990126));
#229669=CARTESIAN_POINT('Ctrl Pts',(58.4305002120414,-19.9966086767195,
-216.277970249807));
#229670=CARTESIAN_POINT('Ctrl Pts',(60.6289872337381,-20.7636493692889,
-212.926206211883));
#229671=CARTESIAN_POINT('Ctrl Pts',(47.4866458063998,-15.6558748576279,
-233.029111826755));
#229672=CARTESIAN_POINT('Ctrl Pts',(49.68616076798,-16.3826093301408,-229.678058258297));
#229673=CARTESIAN_POINT('Ctrl Pts',(51.8862243890013,-17.1062920942477,
-226.326700188893));
#229674=CARTESIAN_POINT('Ctrl Pts',(54.0864948338312,-17.8287356549779,
-222.97520798459));
#229675=CARTESIAN_POINT('Ctrl Pts',(56.2867652786612,-18.551179215708,-219.623715780286));
#229676=CARTESIAN_POINT('Ctrl Pts',(58.4872620760191,-19.2722889032489,
-216.272081643134));
#229677=CARTESIAN_POINT('Ctrl Pts',(60.6878681298499,-19.9927261544104,
-212.920372770536));
#229678=CARTESIAN_POINT('Ctrl Pts',(47.554307632397,-15.1637468311187,-233.025453073475));
#229679=CARTESIAN_POINT('Ctrl Pts',(49.7567152646595,-15.8456016742832,
-229.674306559616));
#229680=CARTESIAN_POINT('Ctrl Pts',(51.9599159483462,-16.5235645049904,
-226.322904658655));
#229681=CARTESIAN_POINT('Ctrl Pts',(54.1634104836589,-17.1999459798668,
-222.971380331423));
#229682=CARTESIAN_POINT('Ctrl Pts',(56.3669050189717,-17.8763274547433,
-219.619856004191));
#229683=CARTESIAN_POINT('Ctrl Pts',(58.5707224241369,-18.5510070650469,
-216.268204278443));
#229684=CARTESIAN_POINT('Ctrl Pts',(60.7746940090617,-19.2248286528632,
-212.916482666117));
#229685=CARTESIAN_POINT('Ctrl Pts',(47.5881385453956,-14.9176828178641,
-233.023623696835));
#229686=CARTESIAN_POINT('Ctrl Pts',(49.7919925129992,-15.5770978463543,
-229.672430710276));
#229687=CARTESIAN_POINT('Ctrl Pts',(51.9967617280187,-16.2322007103616,
-226.321006893536));
#229688=CARTESIAN_POINT('Ctrl Pts',(54.2018683085728,-16.8855511423113,
-222.96946650484));
#229689=CARTESIAN_POINT('Ctrl Pts',(56.4069748891269,-17.538901574261,-219.617926116144));
#229690=CARTESIAN_POINT('Ctrl Pts',(58.6124525981959,-18.1903661459459,
-216.266265596097));
#229691=CARTESIAN_POINT('Ctrl Pts',(60.8181069486676,-18.8408799020897,
-212.914537613908));
#229692=CARTESIAN_POINT('Ctrl Pts',(47.6271129859842,-14.672424944912,-233.022456269286));
#229693=CARTESIAN_POINT('Ctrl Pts',(49.8327089180398,-15.3093857877439,
-229.671166307109));
#229694=CARTESIAN_POINT('Ctrl Pts',(52.0393530559316,-15.9416180264796,
-226.319687040658));
#229695=CARTESIAN_POINT('Ctrl Pts',(54.2463813625237,-16.5719288708872,
-222.968103360071));
#229696=CARTESIAN_POINT('Ctrl Pts',(56.4534096691157,-17.2022397152948,
-219.616519679485));
#229697=CARTESIAN_POINT('Ctrl Pts',(58.6608611565012,-17.830482853318,-216.264830059583));
#229698=CARTESIAN_POINT('Ctrl Pts',(60.8685133335648,-18.4576836904079,
-212.913078722092));
#229699=CARTESIAN_POINT('Ctrl Pts',(47.6711899624377,-14.4281659124299,
-233.021940707592));
#229700=CARTESIAN_POINT('Ctrl Pts',(49.8788265984679,-15.0426590253955,
-229.670504307963));
#229701=CARTESIAN_POINT('Ctrl Pts',(52.0876575029478,-15.6520019918285,
-226.318937245156));
#229702=CARTESIAN_POINT('Ctrl Pts',(54.296923205648,-16.259253814469,-222.967284070276));
#229703=CARTESIAN_POINT('Ctrl Pts',(56.5061889083483,-16.8665056371095,
-219.615630895396));
#229704=CARTESIAN_POINT('Ctrl Pts',(58.7159343195776,-17.4715067819979,
-216.263892782403));
#229705=CARTESIAN_POINT('Ctrl Pts',(60.9259062922535,-18.0753740181923,
-212.912101903999));
#229706=CARTESIAN_POINT('Ctrl Pts',(47.6932284506644,-14.3060363961889,
-233.021682926744));
#229707=CARTESIAN_POINT('Ctrl Pts',(49.901885438682,-14.9092956442213,-229.670173308391));
#229708=CARTESIAN_POINT('Ctrl Pts',(52.1118097264559,-15.507193974503,-226.318562347407));
#229709=CARTESIAN_POINT('Ctrl Pts',(54.3221941272102,-16.1029162862599,
-222.966874425379));
#229710=CARTESIAN_POINT('Ctrl Pts',(56.5325785279645,-16.6986385980169,
-219.615186503351));
#229711=CARTESIAN_POINT('Ctrl Pts',(58.7434709011157,-17.2920187463379,
-216.263424143813));
#229712=CARTESIAN_POINT('Ctrl Pts',(60.9546027715979,-17.8842191820846,
-212.911613494952));
#229713=CARTESIAN_POINT('Ctrl Pts',(47.7165427070916,-14.1841566123428,
-233.021588374054));
#229714=CARTESIAN_POINT('Ctrl Pts',(49.9262946886754,-14.7761786009886,
-229.669993107177));
#229715=CARTESIAN_POINT('Ctrl Pts',(52.1373902989064,-15.3626276289524,
-226.318330125135));
#229716=CARTESIAN_POINT('Ctrl Pts',(54.3489722985157,-15.9468155679217,
-222.966600877007));
#229717=CARTESIAN_POINT('Ctrl Pts',(56.560554298125,-16.531003506891,-219.614871628879));
#229718=CARTESIAN_POINT('Ctrl Pts',(58.7726736592232,-17.1127575167165,
-216.263080155467));
#229719=CARTESIAN_POINT('Ctrl Pts',(60.9850459116547,-17.6932859799952,
-212.911245674445));
#229720=CARTESIAN_POINT('Ctrl Pts',(47.7411284099535,-14.0625507697344,
-233.021657357818));
#229721=CARTESIAN_POINT('Ctrl Pts',(49.9520501521893,-14.6433321699676,
-229.669963755451));
#229722=CARTESIAN_POINT('Ctrl Pts',(52.164395575698,-15.2183262074345,-226.318240561216));
#229723=CARTESIAN_POINT('Ctrl Pts',(54.3772547239517,-15.7909735318649,
-222.966463366842));
#229724=CARTESIAN_POINT('Ctrl Pts',(56.5901138722054,-16.3636208562953,
-219.614686172468));
#229725=CARTESIAN_POINT('Ctrl Pts',(58.8035410200603,-16.9337418020372,
-216.262860718253));
#229726=CARTESIAN_POINT('Ctrl Pts',(61.0172349543283,-17.5025911610169,
-212.910998351897));
#229727=CARTESIAN_POINT('Ctrl Pts',(47.7442016228112,-14.0473500394083,
-233.021665980788));
#229728=CARTESIAN_POINT('Ctrl Pts',(49.9552695851286,-14.62672636609,-229.669960086485));
#229729=CARTESIAN_POINT('Ctrl Pts',(52.167771235297,-15.2002885297448,-226.318229365726));
#229730=CARTESIAN_POINT('Ctrl Pts',(54.3807900271312,-15.7714932773578,
-222.966446178071));
#229731=CARTESIAN_POINT('Ctrl Pts',(56.5938088189654,-16.3426980249709,
-219.614662990416));
#229732=CARTESIAN_POINT('Ctrl Pts',(58.8073994401649,-16.9113648377023,
-216.262833288602));
#229733=CARTESIAN_POINT('Ctrl Pts',(61.0212585846625,-17.4787543086446,
-212.910967436579));
#229734=CARTESIAN_POINT('Ctrl Pts',(47.7476113419008,-14.0307623608562,
-233.021648099596));
#229735=CARTESIAN_POINT('Ctrl Pts',(49.9588045578851,-14.6087951143449,
-229.669924789137));
#229736=CARTESIAN_POINT('Ctrl Pts',(52.1714498515783,-15.180967081333,-226.318183716026));
#229737=CARTESIAN_POINT('Ctrl Pts',(54.3846185831211,-15.7507631661298,
-222.966392342634));
#229738=CARTESIAN_POINT('Ctrl Pts',(56.5977873146637,-16.3205592509265,
-219.614600969242));
#229739=CARTESIAN_POINT('Ctrl Pts',(58.8115349286387,-16.887797426467,-216.262765580964));
#229740=CARTESIAN_POINT('Ctrl Pts',(61.0255542724185,-17.4537483605921,
-212.910895097936));
#229741=CARTESIAN_POINT('Ctrl Pts',(47.7498680445413,-14.0193937377161,
-233.021742568709));
#229742=CARTESIAN_POINT('Ctrl Pts',(49.9612716248183,-14.5958520941202,
-229.670020033279));
#229743=CARTESIAN_POINT('Ctrl Pts',(52.1741145339256,-15.1664771156592,
-226.318278543544));
#229744=CARTESIAN_POINT('Ctrl Pts',(54.3874764662403,-15.7347368225257,
-222.966486672088));
#229745=CARTESIAN_POINT('Ctrl Pts',(56.600838398555,-16.3029965293923,-219.614694800631));
#229746=CARTESIAN_POINT('Ctrl Pts',(58.8147742803545,-16.8687098306404,
-216.262858729364));
#229747=CARTESIAN_POINT('Ctrl Pts',(61.0289796285328,-17.4331414974815,
-212.910987583833));
#229748=CARTESIAN_POINT('Ctrl Pts',(47.7521247471819,-14.008025114576,-233.021837037822));
#229749=CARTESIAN_POINT('Ctrl Pts',(49.9637386917516,-14.5829090738954,
-229.670115277422));
#229750=CARTESIAN_POINT('Ctrl Pts',(52.1767792162729,-15.1519871499853,
-226.318373371061));
#229751=CARTESIAN_POINT('Ctrl Pts',(54.3903343493595,-15.7187104789216,
-222.966581001541));
#229752=CARTESIAN_POINT('Ctrl Pts',(56.6038894824462,-16.2854338078579,
-219.61478863202));
#229753=CARTESIAN_POINT('Ctrl Pts',(58.8180136320704,-16.8496222348139,
-216.262951877763));
#229754=CARTESIAN_POINT('Ctrl Pts',(61.0324049846472,-17.4125346343709,
-212.91108006973));
#229755=CARTESIAN_POINT('Ctrl Pts',(47.7543654978573,-13.9966521764404,
-233.021931550365));
#229756=CARTESIAN_POINT('Ctrl Pts',(49.9661881993766,-14.5699622186276,
-229.67021053026));
#229757=CARTESIAN_POINT('Ctrl Pts',(52.1794248253455,-15.137493805192,-226.318468190145));
#229758=CARTESIAN_POINT('Ctrl Pts',(54.3931716728027,-15.7026812170992,
-222.966675309108));
#229759=CARTESIAN_POINT('Ctrl Pts',(56.60691852026,-16.2678686290064,-219.614882428071));
#229760=CARTESIAN_POINT('Ctrl Pts',(58.821229483535,-16.8305326445432,-216.263044982252));
#229761=CARTESIAN_POINT('Ctrl Pts',(61.0358053997983,-17.391926245276,-212.911172504828));
#229762=CARTESIAN_POINT('Ctrl Pts',(47.7565902716679,-13.9852750117499,
-233.022026107165));
#229763=CARTESIAN_POINT('Ctrl Pts',(49.9686201309427,-14.5570115979937,
-229.670305792423));
#229764=CARTESIAN_POINT('Ctrl Pts',(52.1820513513198,-15.1229971351898,
-226.318563001159));
#229765=CARTESIAN_POINT('Ctrl Pts',(54.3959884334715,-15.6866490761195,
-222.966769594939));
#229766=CARTESIAN_POINT('Ctrl Pts',(56.6099255156231,-16.2503010170492,
-219.614976188718));
#229767=CARTESIAN_POINT('Ctrl Pts',(58.8244218448074,-16.8114410702517,
-216.26313804258));
#229768=CARTESIAN_POINT('Ctrl Pts',(61.0391808904015,-17.371316327283,-212.911264888718));
#229769=CARTESIAN_POINT('Ctrl Pts',(47.7610398192893,-13.962520682369,-233.022215220766));
#229770=CARTESIAN_POINT('Ctrl Pts',(49.973483994075,-14.5311103567258,-229.670496316751));
#229771=CARTESIAN_POINT('Ctrl Pts',(52.1873044032685,-15.0940037951854,
-226.318752623187));
#229772=CARTESIAN_POINT('Ctrl Pts',(54.4016219548089,-15.6545847941602,
-222.9669581666));
#229773=CARTESIAN_POINT('Ctrl Pts',(56.6159395063494,-16.2151657931349,
-219.615163710013));
#229774=CARTESIAN_POINT('Ctrl Pts',(58.8308065673522,-16.7732579216688,
-216.263324163236));
#229775=CARTESIAN_POINT('Ctrl Pts',(61.0459318716081,-17.3300964912969,
-212.911449656498));
#229776=CARTESIAN_POINT('Ctrl Pts',(47.7654254592341,-13.9397494467436,
-233.022404511428));
#229777=CARTESIAN_POINT('Ctrl Pts',(49.9782775528494,-14.5051940539731,
-229.670686878432));
#229778=CARTESIAN_POINT('Ctrl Pts',(52.1924811227502,-15.064997154331,-226.318942212994));
#229779=CARTESIAN_POINT('Ctrl Pts',(54.4071732250129,-15.6225089955621,
-222.967146651374));
#229780=CARTESIAN_POINT('Ctrl Pts',(56.6218653272756,-16.1800208367931,
-219.615351089753));
#229781=CARTESIAN_POINT('Ctrl Pts',(58.8370973291551,-16.7350668370003,
-216.263510107308));
#229782=CARTESIAN_POINT('Ctrl Pts',(61.0525831546696,-17.2888705397188,
-212.911634219511));
#229783=CARTESIAN_POINT('Ctrl Pts',(47.7697469949171,-13.9169620127152,
-233.022593985349));
#229784=CARTESIAN_POINT('Ctrl Pts',(49.983000674726,-14.4792632474105,-229.670877481921));
#229785=CARTESIAN_POINT('Ctrl Pts',(52.1975814320602,-15.0359776440825,
-226.319131772858));
#229786=CARTESIAN_POINT('Ctrl Pts',(54.4126422197256,-15.5904219929251,
-222.967335049774));
#229787=CARTESIAN_POINT('Ctrl Pts',(56.627703007391,-16.1448663417677,-219.615538326691));
#229788=CARTESIAN_POINT('Ctrl Pts',(58.8432942103714,-16.6968678996294,
-216.263695872058));
#229789=CARTESIAN_POINT('Ctrl Pts',(61.0591348703587,-17.2476384491985,
-212.91181857376));
#229790=CARTESIAN_POINT('Ctrl Pts',(47.7783900662832,-13.8713871446584,
-233.022972933189));
#229791=CARTESIAN_POINT('Ctrl Pts',(49.9924469184794,-14.4274016342853,
-229.671258688898));
#229792=CARTESIAN_POINT('Ctrl Pts',(52.2077820506802,-14.9779386235856,
-226.319510892586));
#229793=CARTESIAN_POINT('Ctrl Pts',(54.423580209151,-15.5262479876512,-222.967711846576));
#229794=CARTESIAN_POINT('Ctrl Pts',(56.6393783676217,-16.0745573517168,
-219.615912800565));
#229795=CARTESIAN_POINT('Ctrl Pts',(58.8556879728042,-16.6204700248875,
-216.264067401558));
#229796=CARTESIAN_POINT('Ctrl Pts',(61.0722383017368,-17.1651742681581,
-212.91218728226));
#229797=CARTESIAN_POINT('Ctrl Pts',(47.7867767171158,-13.8257474826836,
-233.023352614608));
#229798=CARTESIAN_POINT('Ctrl Pts',(50.0016114126724,-14.3754820056756,
-229.6716400639));
#229799=CARTESIAN_POINT('Ctrl Pts',(52.2176770274244,-14.9198481253495,
-226.319889893413));
#229800=CARTESIAN_POINT('Ctrl Pts',(54.4341890960325,-15.4620291661139,
-222.968088298805));
#229801=CARTESIAN_POINT('Ctrl Pts',(56.6507011646406,-16.0042102068785,
-219.616286704198));
#229802=CARTESIAN_POINT('Ctrl Pts',(58.8677062133155,-16.5440407393228,
-216.264438214748));
#229803=CARTESIAN_POINT('Ctrl Pts',(61.0849434643637,-17.0826855313617,
-212.912555156691));
#229804=CARTESIAN_POINT('Ctrl Pts',(47.794905416537,-13.7800486938334,-233.0237330726));
#229805=CARTESIAN_POINT('Ctrl Pts',(50.0104931205382,-14.3235088264801,
-229.67202163298));
#229806=CARTESIAN_POINT('Ctrl Pts',(52.2272657548643,-14.8617096033744,
-226.320268783124));
#229807=CARTESIAN_POINT('Ctrl Pts',(54.4444686924125,-15.3977680306514,
-222.968464399553));
#229808=CARTESIAN_POINT('Ctrl Pts',(56.6616716299607,-15.9338264579286,
-219.616660015982));
#229809=CARTESIAN_POINT('Ctrl Pts',(58.8793495680496,-16.4675807101401,
-216.264808277961));
#229810=CARTESIAN_POINT('Ctrl Pts',(61.0972513955672,-17.0001720517288,
-212.912922153302));
#229811=CARTESIAN_POINT('Ctrl Pts',(47.9249646072757,-13.0488680722298,
-233.029820400472));
#229812=CARTESIAN_POINT('Ctrl Pts',(50.1526004463906,-13.4919379593521,
-229.678126738255));
#229813=CARTESIAN_POINT('Ctrl Pts',(52.3806853939039,-13.9314932517732,
-226.326331018504));
#229814=CARTESIAN_POINT('Ctrl Pts',(54.6089422344929,-14.3695898632513,
-222.974482011522));
#229815=CARTESIAN_POINT('Ctrl Pts',(56.8371990750819,-14.8076864747294,
-219.622633004539));
#229816=CARTESIAN_POINT('Ctrl Pts',(59.0656432437958,-15.2442202432178,
-216.270729289381));
#229817=CARTESIAN_POINT('Ctrl Pts',(61.2941782948235,-15.6799563776017,
-212.918794099076));
#229818=CARTESIAN_POINT('Ctrl Pts',(47.9883865798889,-12.3026122775794,
-233.036124708431));
#229819=CARTESIAN_POINT('Ctrl Pts',(50.2219072486975,-12.6466684930416,
-229.684291138819));
#229820=CARTESIAN_POINT('Ctrl Pts',(52.4554840800718,-12.9889576988494,
-226.332367209873));
#229821=CARTESIAN_POINT('Ctrl Pts',(54.6890840421723,-13.3305248173704,
-222.980406475497));
#229822=CARTESIAN_POINT('Ctrl Pts',(56.9226840042728,-13.6720919358914,
-219.628445741121));
#229823=CARTESIAN_POINT('Ctrl Pts',(59.1563087897256,-14.0128828330946,
-216.276445414441));
#229824=CARTESIAN_POINT('Ctrl Pts',(61.3899461914607,-14.353280946091,-212.924425089962));
#229825=CARTESIAN_POINT('Ctrl Pts',(47.9834035327445,-11.5593373188707,
-233.042545221464));
#229826=CARTESIAN_POINT('Ctrl Pts',(50.2170610824398,-11.8031522322565,
-229.690412491071));
#229827=CARTESIAN_POINT('Ctrl Pts',(52.4507177144441,-12.0469951332675,
-226.33828118561));
#229828=CARTESIAN_POINT('Ctrl Pts',(54.684373970075,-12.2908494697823,-222.986150461423));
#229829=CARTESIAN_POINT('Ctrl Pts',(56.9180302257058,-12.5347038062971,
-219.634019737236));
#229830=CARTESIAN_POINT('Ctrl Pts',(59.1516860770602,-12.7785704359954,
-216.281889638136));
#229831=CARTESIAN_POINT('Ctrl Pts',(61.3853417234255,-13.0224432858052,
-212.92975985503));
#229832=CARTESIAN_POINT('Ctrl Pts',(47.9784204856001,-10.8160623601621,
-233.048965734498));
#229833=CARTESIAN_POINT('Ctrl Pts',(50.2122149161821,-10.9596359714715,
-229.696533843322));
#229834=CARTESIAN_POINT('Ctrl Pts',(52.4459513488164,-11.1050325676855,
-226.344195161346));
#229835=CARTESIAN_POINT('Ctrl Pts',(54.6796638979776,-11.2511741221942,
-222.991894447348));
#229836=CARTESIAN_POINT('Ctrl Pts',(56.9133764471387,-11.3973156767028,
-219.639593733351));
#229837=CARTESIAN_POINT('Ctrl Pts',(59.1470633643947,-11.5442580388962,
-216.287333861831));
#229838=CARTESIAN_POINT('Ctrl Pts',(61.3807372553903,-11.6916056255194,
-212.935094620098));
#229839=CARTESIAN_POINT('Ctrl Pts',(47.9050040452069,-10.0714896149287,
-233.055533041971));
#229840=CARTESIAN_POINT('Ctrl Pts',(50.1331992952188,-10.115921730292,-229.702631915958));
#229841=CARTESIAN_POINT('Ctrl Pts',(52.3616168326291,-10.1639774224541,
-226.349993898252));
#229842=CARTESIAN_POINT('Ctrl Pts',(54.5901116210639,-10.2135334694198,
-222.997453498015));
#229843=CARTESIAN_POINT('Ctrl Pts',(56.8186064094987,-10.2630895163856,
-219.644913097779));
#229844=CARTESIAN_POINT('Ctrl Pts',(59.0471872279132,-10.3142538392508,
-216.292479809858));
#229845=CARTESIAN_POINT('Ctrl Pts',(61.2758070478567,-10.3662378430004,
-212.940097419686));
#229846=CARTESIAN_POINT('Ctrl Pts',(47.7656170077038,-9.34368646884676,
-233.062037879842));
#229847=CARTESIAN_POINT('Ctrl Pts',(49.9819449608238,-9.2874213104565,-229.708539095772));
#229848=CARTESIAN_POINT('Ctrl Pts',(52.1991449367821,-9.23662705053824,
-226.355554581771));
#229849=CARTESIAN_POINT('Ctrl Pts',(54.4166431400134,-9.18805051768256,
-223.002741959001));
#229850=CARTESIAN_POINT('Ctrl Pts',(56.6341413432447,-9.13947398482688,
-219.649929336231));
#229851=CARTESIAN_POINT('Ctrl Pts',(58.8519736255103,-9.09328518499885,
-216.297310379527));
#229852=CARTESIAN_POINT('Ctrl Pts',(61.069957421301,-9.04829813924799,-212.94477788882));
#229853=CARTESIAN_POINT('Ctrl Pts',(47.7569053178599,-9.29819877221664,
-233.062444432209));
#229854=CARTESIAN_POINT('Ctrl Pts',(49.9724915649241,-9.23564003421678,
-229.708908294511));
#229855=CARTESIAN_POINT('Ctrl Pts',(52.1889904432917,-9.1786676522935,-226.355902124491));
#229856=CARTESIAN_POINT('Ctrl Pts',(54.4058013599478,-9.12395783319898,
-223.003072487813));
#229857=CARTESIAN_POINT('Ctrl Pts',(56.6226122766038,-9.06924801410446,
-219.650242851134));
#229858=CARTESIAN_POINT('Ctrl Pts',(58.8397727753602,-9.01697464410811,
-216.297612290131));
#229859=CARTESIAN_POINT('Ctrl Pts',(61.0570918196413,-8.96592690776347,
-212.945070418141));
#229860=CARTESIAN_POINT('Ctrl Pts',(47.7479382353889,-9.25277671838467,
-233.062850739409));
#229861=CARTESIAN_POINT('Ctrl Pts',(49.9627575429261,-9.18391816356222,
-229.70927675202));
#229862=CARTESIAN_POINT('Ctrl Pts',(52.1785315662453,-9.12076168624719,
-226.356248750518));
#229863=CARTESIAN_POINT('Ctrl Pts',(54.394631899532,-9.05991249164631,-223.003401978127));
#229864=CARTESIAN_POINT('Ctrl Pts',(56.6107322328186,-8.99906329704543,
-219.650555205738));
#229865=CARTESIAN_POINT('Ctrl Pts',(58.827198181488,-8.9406991939707,-216.297912995698));
#229866=CARTESIAN_POINT('Ctrl Pts',(61.0438299379249,-8.88358449709214,
-212.945361716967));
#229867=CARTESIAN_POINT('Ctrl Pts',(47.7387173442106,-9.207425908897,-233.06325682779));
#229868=CARTESIAN_POINT('Ctrl Pts',(49.9527439997195,-9.13226010185821,
-229.709644459743));
#229869=CARTESIAN_POINT('Ctrl Pts',(52.1677689925887,-9.06291255266274,
-226.356594439508));
#229870=CARTESIAN_POINT('Ctrl Pts',(54.383135035575,-8.99591694925441,-223.003730400442));
#229871=CARTESIAN_POINT('Ctrl Pts',(56.5985010785614,-8.92892134584607,
-219.650866361376));
#229872=CARTESIAN_POINT('Ctrl Pts',(58.8142493132399,-8.86445947120716,
-216.2982124531));
#229873=CARTESIAN_POINT('Ctrl Pts',(61.030170850553,-8.80127069719074,-212.945651738761));
#229874=CARTESIAN_POINT('Ctrl Pts',(47.7341068986215,-9.18475050415316,
-233.063459871981));
#229875=CARTESIAN_POINT('Ctrl Pts',(49.9477372281162,-9.10643107100621,
-229.709828313605));
#229876=CARTESIAN_POINT('Ctrl Pts',(52.1623877057604,-9.03398798587052,
-226.356767284002));
#229877=CARTESIAN_POINT('Ctrl Pts',(54.3773866035966,-8.96391917805846,
-223.003894611599));
#229878=CARTESIAN_POINT('Ctrl Pts',(56.5923855014328,-8.89385037024639,
-219.651021939195));
#229879=CARTESIAN_POINT('Ctrl Pts',(58.8077748791159,-8.8263396098254,-216.298362181801));
#229880=CARTESIAN_POINT('Ctrl Pts',(61.0233413068671,-8.76011379724005,
-212.945796749657));
#229881=CARTESIAN_POINT('Ctrl Pts',(47.7294330017316,-9.16209291048223,
-233.063662861321));
#229882=CARTESIAN_POINT('Ctrl Pts',(49.9426605766967,-9.08061799234707,
-229.710011979809));
#229883=CARTESIAN_POINT('Ctrl Pts',(52.1569304950676,-9.0050776271462,-226.356939894011));
#229884=CARTESIAN_POINT('Ctrl Pts',(54.3715563208665,-8.93193385660108,
-223.004058555517));
#229885=CARTESIAN_POINT('Ctrl Pts',(56.5861821466654,-8.85879008605595,
-219.651177217023));
#229886=CARTESIAN_POINT('Ctrl Pts',(58.8012068762785,-8.78822868023012,
-216.29851159821));
#229887=CARTESIAN_POINT('Ctrl Pts',(61.0164124615696,-8.71896404992253,
-212.945941441045));
#229888=CARTESIAN_POINT('Ctrl Pts',(47.724695856798,-9.13945382791814,-233.06386579822));
#229889=CARTESIAN_POINT('Ctrl Pts',(49.9375141864838,-9.05482141596443,
-229.710195456012));
#229890=CARTESIAN_POINT('Ctrl Pts',(52.1513974481024,-8.97618190118969,
-226.357112265619));
#229891=CARTESIAN_POINT('Ctrl Pts',(54.3656442227822,-8.89996129157268,
-223.00422222707));
#229892=CARTESIAN_POINT('Ctrl Pts',(56.579890997462,-8.82374068195567,-219.651332188522));
#229893=CARTESIAN_POINT('Ctrl Pts',(58.7945452376739,-8.75012676166283,
-216.298660695422));
#229894=CARTESIAN_POINT('Ctrl Pts',(61.0093841977678,-8.67782142864838,
-212.946085805591));
#229895=CARTESIAN_POINT('Ctrl Pts',(47.7235115705647,-9.13379405727712,
-233.063916532445));
#229896=CARTESIAN_POINT('Ctrl Pts',(49.9362275889306,-9.04837227186877,
-229.710241325062));
#229897=CARTESIAN_POINT('Ctrl Pts',(52.1500141863611,-8.96895796970056,
-226.357155358521));
#229898=CARTESIAN_POINT('Ctrl Pts',(54.3641661982611,-8.89196815031558,
-223.004263144959));
#229899=CARTESIAN_POINT('Ctrl Pts',(56.5783182101612,-8.8149783309306,-219.651370931397));
#229900=CARTESIAN_POINT('Ctrl Pts',(58.7928798280227,-8.740601282021,-216.298697969725));
#229901=CARTESIAN_POINT('Ctrl Pts',(61.0076271318174,-8.66753577332984,
-212.946121896728));
#229902=CARTESIAN_POINT('Ctrl Pts',(47.7223233313458,-9.1281354435798,-233.063967263389));
#229903=CARTESIAN_POINT('Ctrl Pts',(49.9349366327123,-9.04192415916445,
-229.710287182234));
#229904=CARTESIAN_POINT('Ctrl Pts',(52.1486261848584,-8.96173495275868,
-226.357198436518));
#229905=CARTESIAN_POINT('Ctrl Pts',(54.362683060283,-8.88397580633452,-223.004304045819));
#229906=CARTESIAN_POINT('Ctrl Pts',(56.5767399357077,-8.80621665991036,
-219.651409655121));
#229907=CARTESIAN_POINT('Ctrl Pts',(58.7912085661337,-8.73107636556752,
-216.298735224073));
#229908=CARTESIAN_POINT('Ctrl Pts',(61.0058638522065,-8.6572505633881,-212.946157967432));
#229909=CARTESIAN_POINT('Ctrl Pts',(47.7211311423516,-9.12247799776195,
-233.064017991084));
#229910=CARTESIAN_POINT('Ctrl Pts',(49.9336413200512,-9.03547708644307,
-229.710333027481));
#229911=CARTESIAN_POINT('Ctrl Pts',(52.1472334449741,-8.95451285699648,
-226.357241499541));
#229912=CARTESIAN_POINT('Ctrl Pts',(54.3611948094061,-8.87598426441826,
-223.004344929563));
#229913=CARTESIAN_POINT('Ctrl Pts',(56.5751561738381,-8.79745567184005,
-219.651448359586));
#229914=CARTESIAN_POINT('Ctrl Pts',(58.7895314509544,-8.72155201353807,
-216.298772458348));
#229915=CARTESIAN_POINT('Ctrl Pts',(61.004094357101,-8.64696579840547,-212.94619401758));
#229916=CARTESIAN_POINT('Ctrl Pts',(47.7199389533574,-9.11682055194411,
-233.06406871878));
#229917=CARTESIAN_POINT('Ctrl Pts',(49.9323460073902,-9.02903001372169,
-229.710378872728));
#229918=CARTESIAN_POINT('Ctrl Pts',(52.1458407050898,-8.94729076123427,
-226.357284562563));
#229919=CARTESIAN_POINT('Ctrl Pts',(54.3597065585291,-8.86799272250201,
-223.004385813307));
#229920=CARTESIAN_POINT('Ctrl Pts',(56.5735724119685,-8.78869468376974,
-219.651487064051));
#229921=CARTESIAN_POINT('Ctrl Pts',(58.7878543357751,-8.71202766150863,
-216.298809692624));
#229922=CARTESIAN_POINT('Ctrl Pts',(61.0023248619954,-8.63668103342285,
-212.946230067727));
#229923=CARTESIAN_POINT('Ctrl Pts',(47.7182360912236,-9.10778365437469,
-233.063849433542));
#229924=CARTESIAN_POINT('Ctrl Pts',(49.9305863062102,-9.01935713306031,
-229.710182118577));
#229925=CARTESIAN_POINT('Ctrl Pts',(52.1440124956181,-8.93694685535236,
-226.357101968979));
#229926=CARTESIAN_POINT('Ctrl Pts',(54.3578060024431,-8.85696406828125,
-223.004214571289));
#229927=CARTESIAN_POINT('Ctrl Pts',(56.5715995092681,-8.77698128121015,
-219.6513271736));
#229928=CARTESIAN_POINT('Ctrl Pts',(58.7858047409113,-8.69961462920092,
-216.298657989792));
#229929=CARTESIAN_POINT('Ctrl Pts',(61.0001966476166,-8.62356104366905,
-212.946085129856));
#229930=CARTESIAN_POINT('Ctrl Pts',(47.716754038316,-9.10015869973864,-233.063744037883));
#229931=CARTESIAN_POINT('Ctrl Pts',(49.9290284754874,-9.01103194700285,
-229.71008770866));
#229932=CARTESIAN_POINT('Ctrl Pts',(52.1423745037473,-8.92790717652798,
-226.357014582869));
#229933=CARTESIAN_POINT('Ctrl Pts',(54.3560864243857,-8.84720424996069,
-223.004132836908));
#229934=CARTESIAN_POINT('Ctrl Pts',(56.5697983450241,-8.7665013233934,-219.651251090947));
#229935=CARTESIAN_POINT('Ctrl Pts',(58.78392037252,-8.68840842352587,-216.298586025925));
#229936=CARTESIAN_POINT('Ctrl Pts',(60.9982283640248,-8.61162556319128,
-212.946016581829));
#229937=CARTESIAN_POINT('Ctrl Pts',(47.7137899325008,-9.08490879046653,
-233.063533246565));
#229938=CARTESIAN_POINT('Ctrl Pts',(49.9259128140418,-8.99438157488791,
-229.709898888829));
#229939=CARTESIAN_POINT('Ctrl Pts',(52.1390985200058,-8.90982781887923,
-226.356839810649));
#229940=CARTESIAN_POINT('Ctrl Pts',(54.3526472682709,-8.82768461331957,
-223.003969368145));
#229941=CARTESIAN_POINT('Ctrl Pts',(56.5661960165361,-8.74554140775991,
-219.65109892564));
#229942=CARTESIAN_POINT('Ctrl Pts',(58.7801516357373,-8.66599601217575,
-216.29844209819));
#229943=CARTESIAN_POINT('Ctrl Pts',(60.994291796841,-8.58775460223573,-212.945879485775));
#229944=CARTESIAN_POINT('Ctrl Pts',(47.7108458380545,-9.0696549360132,-233.063325140892));
#229945=CARTESIAN_POINT('Ctrl Pts',(49.9228183148681,-8.97772727901907,
-229.709712530571));
#229946=CARTESIAN_POINT('Ctrl Pts',(52.1358449148446,-8.89174460779308,
-226.356667358174));
#229947=CARTESIAN_POINT('Ctrl Pts',(54.3492317256771,-8.80816120630022,
-223.003808105078));
#229948=CARTESIAN_POINT('Ctrl Pts',(56.5626185365097,-8.72457780480736,
-219.650948851983));
#229949=CARTESIAN_POINT('Ctrl Pts',(58.7764090043429,-8.64358001183346,
-216.29830017932));
#229950=CARTESIAN_POINT('Ctrl Pts',(60.9903826008572,-8.56388015589151,
-212.945744329977));
#229951=CARTESIAN_POINT('Ctrl Pts',(47.7079217613744,-9.05439718416747,
-233.063119714194));
#229952=CARTESIAN_POINT('Ctrl Pts',(49.9197449843438,-8.96106910734242,
-229.709528628916));
#229953=CARTESIAN_POINT('Ctrl Pts',(52.1326136936507,-8.87365758922025,
-226.356497221309));
#229954=CARTESIAN_POINT('Ctrl Pts',(54.3458398007892,-8.78863407215474,
-223.003649044211));
#229955=CARTESIAN_POINT('Ctrl Pts',(56.5590659079277,-8.70361055508924,
-219.650800867113));
#229956=CARTESIAN_POINT('Ctrl Pts',(58.7726924798428,-8.62116045955843,
-216.298160266832));
#229957=CARTESIAN_POINT('Ctrl Pts',(60.9865007760101,-8.54000225738003,
-212.945611112248));
#229958=CARTESIAN_POINT('Ctrl Pts',(47.6845291479335,-8.93233516940169,
-233.061476300607));
#229959=CARTESIAN_POINT('Ctrl Pts',(49.8951583401493,-8.82780373392919,
-229.708057415679));
#229960=CARTESIAN_POINT('Ctrl Pts',(52.1067639241,-8.72896144063768,-226.355136126385));
#229961=CARTESIAN_POINT('Ctrl Pts',(54.3187044016857,-8.63241699899096,
-223.002376557269));
#229962=CARTESIAN_POINT('Ctrl Pts',(56.5306448792714,-8.53587255734424,
-219.649616988152));
#229963=CARTESIAN_POINT('Ctrl Pts',(58.7429602838421,-8.44180404135816,
-216.297040966938));
#229964=CARTESIAN_POINT('Ctrl Pts',(60.9554461772338,-8.34897906928816,
-212.944545370418));
#229965=CARTESIAN_POINT('Ctrl Pts',(47.6624176231886,-8.81002372665067,
-233.060004253171));
#229966=CARTESIAN_POINT('Ctrl Pts',(49.8719264576024,-8.69429031390039,
-229.706743359295));
#229967=CARTESIAN_POINT('Ctrl Pts',(52.0823467043952,-8.58402161768034,
-226.353923176935));
#229968=CARTESIAN_POINT('Ctrl Pts',(54.2930805177033,-8.47596139420291,
-223.001244967003));
#229969=CARTESIAN_POINT('Ctrl Pts',(56.5038143310114,-8.36790117072548,
-219.648566757072));
#229970=CARTESIAN_POINT('Ctrl Pts',(58.7148989206583,-8.26222030325806,
-216.296050047426));
#229971=CARTESIAN_POINT('Ctrl Pts',(60.9261433256064,-8.15773494598065,
-212.943603641929));
#229972=CARTESIAN_POINT('Ctrl Pts',(47.6415907958571,-8.68748728842518,
-233.058700763469));
#229973=CARTESIAN_POINT('Ctrl Pts',(49.8500528218283,-8.56055336019126,
-229.705584368071));
#229974=CARTESIAN_POINT('Ctrl Pts',(52.0593649584596,-8.43886161373385,
-226.352856624949));
#229975=CARTESIAN_POINT('Ctrl Pts',(54.2689704157657,-8.31928937162988,
-223.000252784861));
#229976=CARTESIAN_POINT('Ctrl Pts',(56.4785758730718,-8.19971712952592,
-219.647648944772));
#229977=CARTESIAN_POINT('Ctrl Pts',(58.6885092193172,-8.08242819326595,
-216.295186431349));
#229978=CARTESIAN_POINT('Ctrl Pts',(60.8985922273728,-7.96628687259449,
-212.942784965869));
#229979=CARTESIAN_POINT('Ctrl Pts',(47.5999371411941,-8.4424144119742,-233.056093784063));
#229980=CARTESIAN_POINT('Ctrl Pts',(49.8063055502802,-8.29307945277301,
-229.703266385626));
#229981=CARTESIAN_POINT('Ctrl Pts',(52.0134014665884,-8.14854160584086,
-226.350723520978));
#229982=CARTESIAN_POINT('Ctrl Pts',(54.2207502118905,-8.00594532648383,
-222.998268420575));
#229983=CARTESIAN_POINT('Ctrl Pts',(56.4280989571927,-7.8633490471268,-219.645813320171));
#229984=CARTESIAN_POINT('Ctrl Pts',(58.6357298166351,-7.72284397328174,
-216.293459199193));
#229985=CARTESIAN_POINT('Ctrl Pts',(60.8434900309058,-7.58339072582217,
-212.941147613748));
#229986=CARTESIAN_POINT('Ctrl Pts',(47.563421718127,-8.1964416177969,-233.054159991154));
#229987=CARTESIAN_POINT('Ctrl Pts',(49.7679908920149,-8.02471146303938,
-229.70156787831));
#229988=CARTESIAN_POINT('Ctrl Pts',(51.9731795871583,-7.85734092078273,
-226.34917536569));
#229989=CARTESIAN_POINT('Ctrl Pts',(54.1785849234471,-7.6917356528382,-222.996841160495));
#229990=CARTESIAN_POINT('Ctrl Pts',(56.3839902597359,-7.52613038489368,
-219.644506955299));
#229991=CARTESIAN_POINT('Ctrl Pts',(58.5896369612844,-7.36242630195994,
-216.292240840726));
#229992=CARTESIAN_POINT('Ctrl Pts',(60.7953947813852,-7.19967881344745,
-212.94000219184));
#229993=CARTESIAN_POINT('Ctrl Pts',(47.5320802669249,-7.94976361170966,
-233.052889623343));
#229994=CARTESIAN_POINT('Ctrl Pts',(49.7351412982067,-7.7556448112324,-229.700481632561));
#229995=CARTESIAN_POINT('Ctrl Pts',(51.9387261626187,-7.5654468780096,-226.348205936691));
#229996=CARTESIAN_POINT('Ctrl Pts',(54.1424952790584,-7.37683668146129,
-222.995965483144));
#229997=CARTESIAN_POINT('Ctrl Pts',(56.3462643954981,-7.18822648491298,
-219.643725029598));
#229998=CARTESIAN_POINT('Ctrl Pts',(58.5502384998489,-7.00132626939384,
-216.291526839263));
#229999=CARTESIAN_POINT('Ctrl Pts',(60.7543073371829,-6.81528655387943,
-212.939344378339));
#230000=CARTESIAN_POINT('Ctrl Pts',(47.4693973645209,-7.45640759953517,
-233.050348887721));
#230001=CARTESIAN_POINT('Ctrl Pts',(49.6694421105903,-7.21751150761842,
-229.698309141063));
#230002=CARTESIAN_POINT('Ctrl Pts',(51.8698193135396,-6.98165879246334,
-226.346267078691));
#230003=CARTESIAN_POINT('Ctrl Pts',(54.0703159902812,-6.74703873870746,
-222.994214128443));
#230004=CARTESIAN_POINT('Ctrl Pts',(56.2708126670227,-6.51241868495157,
-219.642161178194));
#230005=CARTESIAN_POINT('Ctrl Pts',(58.4714415769781,-6.27912620426164,
-216.290098836338));
#230006=CARTESIAN_POINT('Ctrl Pts',(60.6721324487782,-6.0465020347434,-212.938028751337));
#230007=CARTESIAN_POINT('Ctrl Pts',(47.4274705119234,-6.96033315507766,
-233.050468098652));
#230008=CARTESIAN_POINT('Ctrl Pts',(49.6256461602249,-6.6766507592267,-229.698589268665));
#230009=CARTESIAN_POINT('Ctrl Pts',(51.8240141959171,-6.39514045095797,
-226.346644939574));
#230010=CARTESIAN_POINT('Ctrl Pts',(54.0224528528355,-6.11450731222085,
-222.994669506924));
#230011=CARTESIAN_POINT('Ctrl Pts',(56.220891509754,-5.83387417348373,-219.642694074275));
#230012=CARTESIAN_POINT('Ctrl Pts',(58.419407944269,-5.55418636991015,-216.29068621863));
#230013=CARTESIAN_POINT('Ctrl Pts',(60.6179613338852,-5.27497371477569,
-212.938660660107));
#230014=CARTESIAN_POINT('Ctrl Pts',(47.4064137512828,-6.46376836204135,
-233.053237209745));
#230015=CARTESIAN_POINT('Ctrl Pts',(49.6038760388037,-6.13507130643716,
-229.701318673814));
#230016=CARTESIAN_POINT('Ctrl Pts',(51.8014392198341,-5.80767781765755,
-226.34934009846));
#230017=CARTESIAN_POINT('Ctrl Pts',(53.999040049297,-5.48080969928608,-222.997335349492));
#230018=CARTESIAN_POINT('Ctrl Pts',(56.19664087876,-5.15394158091461,-219.645330600522));
#230019=CARTESIAN_POINT('Ctrl Pts',(58.3942830138637,-4.82763991403419,
-216.293298098971));
#230020=CARTESIAN_POINT('Ctrl Pts',(60.5919449770341,-4.50162265073271,
-212.941251066378));
#230021=CARTESIAN_POINT('Ctrl Pts',(47.3643002300016,-5.47063877596875,
-233.058775431931));
#230022=CARTESIAN_POINT('Ctrl Pts',(49.5603357959614,-5.05191240085809,
-229.706777484113));
#230023=CARTESIAN_POINT('Ctrl Pts',(51.7562892676681,-4.63275255105671,
-226.354730416234));
#230024=CARTESIAN_POINT('Ctrl Pts',(53.9522144422201,-4.21341447341654,
-223.002667034626));
#230025=CARTESIAN_POINT('Ctrl Pts',(56.148139616772,-3.79407639577637,-219.650603653018));
#230026=CARTESIAN_POINT('Ctrl Pts',(58.3440331530531,-3.37454700228228,
-216.298521859654));
#230027=CARTESIAN_POINT('Ctrl Pts',(60.5399122633319,-2.95492052264675,
-212.94643187892));
#230028=CARTESIAN_POINT('Ctrl Pts',(47.4059785054068,-4.47517271098946,
-233.07487888378));
#230029=CARTESIAN_POINT('Ctrl Pts',(49.6051283878,-3.96564508196357,-229.721994650771));
#230030=CARTESIAN_POINT('Ctrl Pts',(51.8041981735258,-3.45390472955758,
-226.369343135129));
#230031=CARTESIAN_POINT('Ctrl Pts',(54.0032355320804,-2.94127591256867,
-223.016786754993));
#230032=CARTESIAN_POINT('Ctrl Pts',(56.202272890635,-2.42864709557977,-219.664230374857));
#230033=CARTESIAN_POINT('Ctrl Pts',(58.4012751950854,-1.91505962733557,
-216.311776149656));
#230034=CARTESIAN_POINT('Ctrl Pts',(60.6002595528876,-1.40099202884052,
-212.959373373456));
#230035=CARTESIAN_POINT('Ctrl Pts',(47.5294508970783,-3.49440615205346,
-233.102402864825));
#230036=CARTESIAN_POINT('Ctrl Pts',(49.7371099711637,-2.89175495532409,
-229.747791831751));
#230037=CARTESIAN_POINT('Ctrl Pts',(51.9449186325461,-2.28501732803231,
-226.3940294043));
#230038=CARTESIAN_POINT('Ctrl Pts',(54.1527566412239,-1.67669958626741,
-223.040576342272));
#230039=CARTESIAN_POINT('Ctrl Pts',(56.3605946499017,-1.0683818445025,-219.687123280246));
#230040=CARTESIAN_POINT('Ctrl Pts',(58.5684718967623,-0.458344461962341,
-216.334011708901));
#230041=CARTESIAN_POINT('Ctrl Pts',(60.7763601725369,0.15253653159383,-212.981062249621));
#230042=CARTESIAN_POINT('Ctrl Pts',(47.5448849460372,-3.37181033218646,
-233.105843362456));
#230043=CARTESIAN_POINT('Ctrl Pts',(49.7536076690841,-2.75751868949416,
-229.751016479375));
#230044=CARTESIAN_POINT('Ctrl Pts',(51.9625086899236,-2.13890640284165,
-226.397115187946));
#230045=CARTESIAN_POINT('Ctrl Pts',(54.1714467798668,-1.51862754547975,
-223.043550040683));
#230046=CARTESIAN_POINT('Ctrl Pts',(56.38038486981,-0.898348688117847,-219.68998489342));
#230047=CARTESIAN_POINT('Ctrl Pts',(58.5893714844719,-0.276255066290686,
-216.336791153806));
#230048=CARTESIAN_POINT('Ctrl Pts',(60.798372749993,0.346727601648124,-212.983773359142));
#230049=CARTESIAN_POINT('Ctrl Pts',(47.5615915692654,-3.24943555854357,
-233.109464818529));
#230050=CARTESIAN_POINT('Ctrl Pts',(49.7714637647986,-2.62347002868952,
-229.7544084453));
#230051=CARTESIAN_POINT('Ctrl Pts',(51.9815466632923,-1.99294743735296,
-226.40036014233));
#230052=CARTESIAN_POINT('Ctrl Pts',(54.1916753900507,-1.36067182993002,
-223.046676420892));
#230053=CARTESIAN_POINT('Ctrl Pts',(56.401804116809,-0.728396222507082,
-219.692992699454));
#230054=CARTESIAN_POINT('Ctrl Pts',(58.6119918904791,-0.0942105190696879,
-216.339712230689));
#230055=CARTESIAN_POINT('Ctrl Pts',(60.8221984456974,0.540909515678286,
-212.986622360574));
#230056=CARTESIAN_POINT('Ctrl Pts',(47.5795644264693,-3.1273054400959,-233.113272591666));
#230057=CARTESIAN_POINT('Ctrl Pts',(49.7906742268616,-2.48963297721053,
-229.757972064269));
#230058=CARTESIAN_POINT('Ctrl Pts',(52.0020311559296,-1.84716370589099,
-226.403768144263));
#230059=CARTESIAN_POINT('Ctrl Pts',(54.2134437517945,-1.20285465735803,
-223.049959011375));
#230060=CARTESIAN_POINT('Ctrl Pts',(56.4248563476593,-0.558545608825073,
-219.696149878487));
#230061=CARTESIAN_POINT('Ctrl Pts',(58.6363398184349,0.0877694602078754,
-216.342777920879));
#230062=CARTESIAN_POINT('Ctrl Pts',(60.8478467270347,0.735064158177848,
-212.989612083611));
#230063=CARTESIAN_POINT('Ctrl Pts',(47.5885508550713,-3.06624038087206,
-233.115176478235));
#230064=CARTESIAN_POINT('Ctrl Pts',(49.8002794578931,-2.42271445147103,
-229.759753873753));
#230065=CARTESIAN_POINT('Ctrl Pts',(52.0122734022483,-1.77427184016,-226.405472145231));
#230066=CARTESIAN_POINT('Ctrl Pts',(54.2243279326664,-1.12394607107203,
-223.051600306617));
#230067=CARTESIAN_POINT('Ctrl Pts',(56.4363824630845,-0.473620301984068,
-219.697728468003));
#230068=CARTESIAN_POINT('Ctrl Pts',(58.6485137824127,0.178759449846657,
-216.344310765974));
#230069=CARTESIAN_POINT('Ctrl Pts',(60.8606708677034,0.832141479427629,
-212.99110694513));
#230070=CARTESIAN_POINT('Ctrl Pts',(47.5978538522586,-3.00523648529404,
-233.117126961161));
#230071=CARTESIAN_POINT('Ctrl Pts',(49.8102232873676,-2.35584882925707,
-229.761578609019));
#230072=CARTESIAN_POINT('Ctrl Pts',(52.0228772837467,-1.70142378458667,
-226.407216918259));
#230073=CARTESIAN_POINT('Ctrl Pts',(54.2355970556278,-1.04507212252995,
-223.053280662751));
#230074=CARTESIAN_POINT('Ctrl Pts',(56.448316827509,-0.388720460473239,
-219.699344407242));
#230075=CARTESIAN_POINT('Ctrl Pts',(58.6611196292105,0.269733294988998,
-216.345879769661));
#230076=CARTESIAN_POINT('Ctrl Pts',(60.873950656561,0.929211980164266,-212.992636991345));
#230077=CARTESIAN_POINT('Ctrl Pts',(47.6074726880044,-2.94429670427164,
-233.119124814901));
#230078=CARTESIAN_POINT('Ctrl Pts',(49.8205052535735,-2.2890391191441,-229.763446888111));
#230079=CARTESIAN_POINT('Ctrl Pts',(52.0338426588191,-1.6286224591917,-226.409003009738));
#230080=CARTESIAN_POINT('Ctrl Pts',(54.2472513064603,-0.966235601713411,
-223.055000571257));
#230081=CARTESIAN_POINT('Ctrl Pts',(56.4606599541014,-0.303848744235122,
-219.700998132776));
#230082=CARTESIAN_POINT('Ctrl Pts',(58.6741582110175,0.36068851501233,-216.347485336292));
#230083=CARTESIAN_POINT('Ctrl Pts',(60.8876872878579,1.02627337962685,-212.994202601728));
#230084=CARTESIAN_POINT('Ctrl Pts',(47.6122821058773,-2.91382681376045,
-233.120123741771));
#230085=CARTESIAN_POINT('Ctrl Pts',(49.8256462366764,-2.25563426408762,
-229.764381027656));
#230086=CARTESIAN_POINT('Ctrl Pts',(52.0393253463554,-1.59222179649422,
-226.409896055477));
#230087=CARTESIAN_POINT('Ctrl Pts',(54.2530784318765,-0.926817341305142,
-223.05586052551));
#230088=CARTESIAN_POINT('Ctrl Pts',(56.4668315173976,-0.261412886116064,
-219.701824995542));
#230089=CARTESIAN_POINT('Ctrl Pts',(58.680677501921,0.406166125023995,-216.348288119608));
#230090=CARTESIAN_POINT('Ctrl Pts',(60.8945556035063,1.07480407935814,-212.99498540692));
#230091=CARTESIAN_POINT('Ctrl Pts',(47.6166843338988,-2.89479809257736,
-233.118546667211));
#230092=CARTESIAN_POINT('Ctrl Pts',(49.8304641874375,-2.23319920218914,
-229.762886946434));
#230093=CARTESIAN_POINT('Ctrl Pts',(52.0445356905235,-1.56647045026326,
-226.408456344895));
#230094=CARTESIAN_POINT('Ctrl Pts',(54.2586738605045,-0.897786580916013,
-223.054464805284));
#230095=CARTESIAN_POINT('Ctrl Pts',(56.4728120304856,-0.229102711568775,
-219.700473265674));
#230096=CARTESIAN_POINT('Ctrl Pts',(58.6870347127076,0.44171613101905,-216.346968914843));
#230097=CARTESIAN_POINT('Ctrl Pts',(60.9012859052481,1.11357395216271,-212.993693318827));
#230098=CARTESIAN_POINT('Ctrl Pts',(47.6211124898449,-2.8723889492326,-233.117728387381));
#230099=CARTESIAN_POINT('Ctrl Pts',(49.8352745925261,-2.20751597714286,
-229.762108046517));
#230100=CARTESIAN_POINT('Ctrl Pts',(52.0497152441705,-1.53755916668926,
-226.407703586764));
#230101=CARTESIAN_POINT('Ctrl Pts',(54.2642183610334,-0.865666855062723,
-223.053733238581));
#230102=CARTESIAN_POINT('Ctrl Pts',(56.4787214778963,-0.193774543436184,
-219.699762890398));
#230103=CARTESIAN_POINT('Ctrl Pts',(58.6933043194368,0.480231871349857,
-216.346274307009));
#230104=CARTESIAN_POINT('Ctrl Pts',(60.9079135866709,1.15526652998651,-212.993011881675));
#230105=CARTESIAN_POINT('Ctrl Pts',(47.6255406457911,-2.84997980588785,
-233.116910107551));
#230106=CARTESIAN_POINT('Ctrl Pts',(49.8400849976146,-2.18183275209659,
-229.761329146599));
#230107=CARTESIAN_POINT('Ctrl Pts',(52.0548947978176,-1.50864788311527,
-226.406950828634));
#230108=CARTESIAN_POINT('Ctrl Pts',(54.2697628615623,-0.83354712920943,
-223.053001671879));
#230109=CARTESIAN_POINT('Ctrl Pts',(56.4846309253071,-0.158446375303592,
-219.699052515123));
#230110=CARTESIAN_POINT('Ctrl Pts',(58.699573926166,0.518747611680667,-216.345579699174));
#230111=CARTESIAN_POINT('Ctrl Pts',(60.9145412680937,1.1969591078103,-212.992330444524));
#230112=CARTESIAN_POINT('Ctrl Pts',(47.6299049832871,-2.82756442152549,
-233.116092453226));
#230113=CARTESIAN_POINT('Ctrl Pts',(49.8448255724277,-2.15613841592184,
-229.760550756022));
#230114=CARTESIAN_POINT('Ctrl Pts',(52.0599987949363,-1.47972090207117,
-226.406198468922));
#230115=CARTESIAN_POINT('Ctrl Pts',(54.2752261916461,-0.801407134891986,
-223.052270410334));
#230116=CARTESIAN_POINT('Ctrl Pts',(56.4904535883559,-0.123093367712802,
-219.698342351745));
#230117=CARTESIAN_POINT('Ctrl Pts',(58.7057512556755,0.557292721778429,
-216.344885224803));
#230118=CARTESIAN_POINT('Ctrl Pts',(60.9210712376979,1.23868559335551,-212.991649073236));
#230119=CARTESIAN_POINT('Ctrl Pts',(47.6342055660403,-2.80514285302076,
-233.11527543729));
#230120=CARTESIAN_POINT('Ctrl Pts',(49.8494963118054,-2.13043323572804,
-229.759772872591));
#230121=CARTESIAN_POINT('Ctrl Pts',(52.0650271669924,-1.4507786685942,-226.405446498001));
#230122=CARTESIAN_POINT('Ctrl Pts',(54.2806082192958,-0.769247485060314,
-223.051539438634));
#230123=CARTESIAN_POINT('Ctrl Pts',(56.4961892715991,-0.0877163015264225,
-219.697632379269));
#230124=CARTESIAN_POINT('Ctrl Pts',(58.7118360495897,0.595866264290071,
-216.344190859432));
#230125=CARTESIAN_POINT('Ctrl Pts',(60.9275031739158,1.28044489740776,-212.990967740646));
#230126=CARTESIAN_POINT('Ctrl Pts',(47.6686102280658,-2.62577030498296,
-233.108739309799));
#230127=CARTESIAN_POINT('Ctrl Pts',(49.8868622268275,-1.92479179417762,
-229.753549805137));
#230128=CARTESIAN_POINT('Ctrl Pts',(52.1052541434417,-1.21924080077849,
-226.399430730627));
#230129=CARTESIAN_POINT('Ctrl Pts',(54.3236644404932,-0.511970286406943,
-223.045691665041));
#230130=CARTESIAN_POINT('Ctrl Pts',(56.5420747375447,0.195300227964602,
-219.691952599455));
#230131=CARTESIAN_POINT('Ctrl Pts',(58.7605144009039,0.904454604383199,
-216.338635936458));
#230132=CARTESIAN_POINT('Ctrl Pts',(60.9789586636595,1.61451932982577,-212.985517079921));
#230133=CARTESIAN_POINT('Ctrl Pts',(47.6989353797486,-2.4460016880478,-233.102243720839));
#230134=CARTESIAN_POINT('Ctrl Pts',(49.9197589274877,-1.71845616621595,
-229.747358791629));
#230135=CARTESIAN_POINT('Ctrl Pts',(52.1406411035373,-0.986726750840026,
-226.393439406672));
#230136=CARTESIAN_POINT('Ctrl Pts',(54.3615170914844,-0.253435215006592,
-223.039861978631));
#230137=CARTESIAN_POINT('Ctrl Pts',(56.5823930794315,0.479856320826842,
-219.686284550589));
#230138=CARTESIAN_POINT('Ctrl Pts',(58.8032699357002,1.21486234957556,-216.333087493431));
#230139=CARTESIAN_POINT('Ctrl Pts',(61.0241393837606,1.95069381201327,-212.980068394613));
#230140=CARTESIAN_POINT('Ctrl Pts',(47.725208148176,-2.26586793370592,-233.095797498554));
#230141=CARTESIAN_POINT('Ctrl Pts',(49.9481820104395,-1.51156427070571,
-229.741201508812));
#230142=CARTESIAN_POINT('Ctrl Pts',(52.171153048358,-0.753464571140378,
-226.387470648604));
#230143=CARTESIAN_POINT('Ctrl Pts',(54.3941000891112,0.00604443117689846,
-223.034045756));
#230144=CARTESIAN_POINT('Ctrl Pts',(56.6170471298644,0.765553433494175,
-219.680620863394));
#230145=CARTESIAN_POINT('Ctrl Pts',(58.8399741136204,1.52661141375358,-216.32753645248));
#230146=CARTESIAN_POINT('Ctrl Pts',(61.0628850955307,2.28841296751785,-212.974611260487));
#230147=CARTESIAN_POINT('Ctrl Pts',(47.777753685031,-1.90560042502214,-233.082905053984));
#230148=CARTESIAN_POINT('Ctrl Pts',(50.0050281763432,-1.0977804796852,-229.72888694318));
#230149=CARTESIAN_POINT('Ctrl Pts',(52.2321769379993,-0.286940211741083,
-226.375533132468));
#230150=CARTESIAN_POINT('Ctrl Pts',(54.4592660843647,0.525003723543879,
-223.022413310737));
#230151=CARTESIAN_POINT('Ctrl Pts',(56.6863552307302,1.33694765882884,-219.669293489006));
#230152=CARTESIAN_POINT('Ctrl Pts',(58.9133824694609,2.15010954210964,-216.316434370579));
#230153=CARTESIAN_POINT('Ctrl Pts',(61.140376519071,2.96385127852703,-212.963696992235));
#230154=CARTESIAN_POINT('Ctrl Pts',(47.8141039634246,-1.54378581355141,
-233.070233320969));
#230155=CARTESIAN_POINT('Ctrl Pts',(50.043980577362,-0.681755118427429,
-229.716715414099));
#230156=CARTESIAN_POINT('Ctrl Pts',(52.2736848111942,0.182550353550442,
-226.363684359704));
#230157=CARTESIAN_POINT('Ctrl Pts',(54.5033194303334,1.04768172667892,-223.010825413529));
#230158=CARTESIAN_POINT('Ctrl Pts',(56.7329540494726,1.91281309980739,-219.657966467354));
#230159=CARTESIAN_POINT('Ctrl Pts',(58.9625137255313,2.77885743664385,-216.305299102755));
#230160=CARTESIAN_POINT('Ctrl Pts',(61.192035920041,3.64533504273501,-212.952721389729));
#230161=CARTESIAN_POINT('Ctrl Pts',(47.8343566648447,-1.18129562201859,
-233.057735449668));
#230162=CARTESIAN_POINT('Ctrl Pts',(50.0649792011103,-0.264693413707682,
-229.704700485746));
#230163=CARTESIAN_POINT('Ctrl Pts',(52.2954559925465,0.653414022650932,
-226.351982116141));
#230164=CARTESIAN_POINT('Ctrl Pts',(54.525876562459,1.57206651464896,-222.999376095285));
#230165=CARTESIAN_POINT('Ctrl Pts',(56.7562971323714,2.49071900664698,-219.646770074429));
#230166=CARTESIAN_POINT('Ctrl Pts',(58.9866565003629,3.40997442959623,-216.294288989989));
#230167=CARTESIAN_POINT('Ctrl Pts',(61.2169859241647,4.32951560431301,-212.941866493395));
#230168=CARTESIAN_POINT('Ctrl Pts',(47.8748620676848,-0.456315238952961,
-233.032739707064));
#230169=CARTESIAN_POINT('Ctrl Pts',(50.106976448607,0.569429995731811,-229.68067062904));
#230170=CARTESIAN_POINT('Ctrl Pts',(52.3389983552511,1.59514136085191,-226.328577629014));
#230171=CARTESIAN_POINT('Ctrl Pts',(54.5709908267102,2.62083609058904,-222.976477458797));
#230172=CARTESIAN_POINT('Ctrl Pts',(56.8029832981692,3.64653082032617,-219.624377288579));
#230173=CARTESIAN_POINT('Ctrl Pts',(59.0349420500259,4.672208415501,-216.272268764454));
#230174=CARTESIAN_POINT('Ctrl Pts',(61.2668859324121,5.69787672746903,-212.920156700729));
#230175=CARTESIAN_POINT('Ctrl Pts',(47.8510697790929,0.272029506621824,
-233.008563181426));
#230176=CARTESIAN_POINT('Ctrl Pts',(50.0771558477705,1.40772928337885,-229.657271695028));
#230177=CARTESIAN_POINT('Ctrl Pts',(52.3034810716587,2.54196481575621,-226.305687299172));
#230178=CARTESIAN_POINT('Ctrl Pts',(54.5298878738176,3.67568259184972,-222.953998949698));
#230179=CARTESIAN_POINT('Ctrl Pts',(56.7562946759763,4.80940036794322,-219.602310600225));
#230180=CARTESIAN_POINT('Ctrl Pts',(58.9827932020866,5.94254191761289,-216.250506712501));
#230181=CARTESIAN_POINT('Ctrl Pts',(61.2093339293867,7.07541394960212,-212.898648776991));
#230182=CARTESIAN_POINT('Ctrl Pts',(47.7616858294571,0.998150138415235,
-232.985293804272));
#230183=CARTESIAN_POINT('Ctrl Pts',(49.9747881970607,2.24045815861694,-229.634704119062));
#230184=CARTESIAN_POINT('Ctrl Pts',(52.1886983731474,3.47997469249725,-226.283620725365));
#230185=CARTESIAN_POINT('Ctrl Pts',(54.4028959591866,4.71845222593428,-222.932344808848));
#230186=CARTESIAN_POINT('Ctrl Pts',(56.6170935452258,5.95692975937132,-219.581068892331));
#230187=CARTESIAN_POINT('Ctrl Pts',(58.8316104681301,7.19426601066472,-216.229583902017));
#230188=CARTESIAN_POINT('Ctrl Pts',(61.046277219474,8.43105358570855,-212.877995957148));
#230189=CARTESIAN_POINT('Ctrl Pts',(47.7393398420482,1.17968029636359,-232.979476459983));
#230190=CARTESIAN_POINT('Ctrl Pts',(49.9491962843832,2.44864037742646,-229.629062225071));
#230191=CARTESIAN_POINT('Ctrl Pts',(52.1600026985195,3.71447716168251,-226.278104081914));
#230192=CARTESIAN_POINT('Ctrl Pts',(54.3711479805289,4.97914463445542,-222.926931273635));
#230193=CARTESIAN_POINT('Ctrl Pts',(56.5822932625382,6.24381210722835,-219.575758465357));
#230194=CARTESIAN_POINT('Ctrl Pts',(58.7938147846409,7.50719703392768,-216.224353199397));
#230195=CARTESIAN_POINT('Ctrl Pts',(61.0055130419957,8.76996349473516,-212.872832752187));
#230196=CARTESIAN_POINT('Ctrl Pts',(47.7128809309633,1.36106465955398,-232.973714427979));
#230197=CARTESIAN_POINT('Ctrl Pts',(49.9190688863809,2.65647440303478,-229.623470833417));
#230198=CARTESIAN_POINT('Ctrl Pts',(52.1263647289421,3.94843444171322,-226.272637535688));
#230199=CARTESIAN_POINT('Ctrl Pts',(54.3340573658958,5.23909322841377,-222.921567986388));
#230200=CARTESIAN_POINT('Ctrl Pts',(56.5417500028495,6.52975201511432,-219.570498437088));
#230201=CARTESIAN_POINT('Ctrl Pts',(58.7498827079224,7.81898619339649,-216.219173942379));
#230202=CARTESIAN_POINT('Ctrl Pts',(60.9582225191604,9.10753070501037,-212.867722142776));
#230203=CARTESIAN_POINT('Ctrl Pts',(47.6822473288034,1.54226015711989,-232.968019332623));
#230204=CARTESIAN_POINT('Ctrl Pts',(49.8843891563535,2.86381435135825,-229.6179346096));
#230205=CARTESIAN_POINT('Ctrl Pts',(52.0878067306158,4.18161224455118,-226.267221321995));
#230206=CARTESIAN_POINT('Ctrl Pts',(54.2916843246343,5.49797977211644,-222.916251722872));
#230207=CARTESIAN_POINT('Ctrl Pts',(56.4955619186529,6.81434729968171,-219.565282123748));
#230208=CARTESIAN_POINT('Ctrl Pts',(58.6999487759841,8.12915246217079,-216.214037028638));
#230209=CARTESIAN_POINT('Ctrl Pts',(60.9045760974657,9.44319745618915,-212.862653075561));
#230210=CARTESIAN_POINT('Ctrl Pts',(47.6745889282634,1.58755903151136,-232.966595558784));
#230211=CARTESIAN_POINT('Ctrl Pts',(49.8757192238467,2.91564933843912,-229.616550553645));
#230212=CARTESIAN_POINT('Ctrl Pts',(52.0781672310342,4.23990669526066,-226.265867268572));
#230213=CARTESIAN_POINT('Ctrl Pts',(54.281091064319,5.56270140804211,-222.914922656992));
#230214=CARTESIAN_POINT('Ctrl Pts',(56.4840148976038,6.88549612082355,-219.563978045413));
#230215=CARTESIAN_POINT('Ctrl Pts',(58.6874652929996,8.20669402936436,-216.212752800202));
#230216=CARTESIAN_POINT('Ctrl Pts',(60.891164492042,9.52711414398385,-212.861385808758));
#230217=CARTESIAN_POINT('Ctrl Pts',(47.6666695671617,1.63284608999026,-232.96517598567));
#230218=CARTESIAN_POINT('Ctrl Pts',(49.8667647552568,2.96745344462007,-229.615169968288));
#230219=CARTESIAN_POINT('Ctrl Pts',(52.0682202296165,4.29815242923168,-226.264516384494));
#230220=CARTESIAN_POINT('Ctrl Pts',(54.2701676639963,5.62735666781534,-222.913596554258));
#230221=CARTESIAN_POINT('Ctrl Pts',(56.4721150983761,6.956560906399,-219.562676724022));
#230222=CARTESIAN_POINT('Ctrl Pts',(58.6746067250159,8.28413416941793,-216.211471242811));
#230223=CARTESIAN_POINT('Ctrl Pts',(60.8773556798765,9.61091205669726,-212.860121162684));
#230224=CARTESIAN_POINT('Ctrl Pts',(47.6584881964675,1.67812063274807,-232.963760828248));
#230225=CARTESIAN_POINT('Ctrl Pts',(49.8575254560703,3.01922438781437,-229.613792971254));
#230226=CARTESIAN_POINT('Ctrl Pts',(52.0579660735326,4.35634578681776,-226.263168720394));
#230227=CARTESIAN_POINT('Ctrl Pts',(54.2589150870478,5.6919405831028,-222.912273412552));
#230228=CARTESIAN_POINT('Ctrl Pts',(56.459864100563,7.02753537938784,-219.56137810471));
#230229=CARTESIAN_POINT('Ctrl Pts',(58.6613752354701,8.36146537341484,-216.210192263444));
#230230=CARTESIAN_POINT('Ctrl Pts',(60.8631523975563,9.69458248633691,-212.858859013292));
#230231=CARTESIAN_POINT('Ctrl Pts',(47.6543975111204,1.70075790412697,-232.963053249537));
#230232=CARTESIAN_POINT('Ctrl Pts',(49.8529058064771,3.04510985941153,-229.613104472738));
#230233=CARTESIAN_POINT('Ctrl Pts',(52.0528389954907,4.38544246561079,-226.262494888344));
#230234=CARTESIAN_POINT('Ctrl Pts',(54.2532887985736,5.72423254074652,-222.911611841699));
#230235=CARTESIAN_POINT('Ctrl Pts',(56.4537386016565,7.06302261588225,-219.560728795054));
#230236=CARTESIAN_POINT('Ctrl Pts',(58.6547594906971,8.4001309754133,-216.209552773761));
#230237=CARTESIAN_POINT('Ctrl Pts',(60.8560507563961,9.73641770115673,-212.858227938596));
#230238=CARTESIAN_POINT('Ctrl Pts',(47.6502413228594,1.72339204637661,-232.962346774948));
#230239=CARTESIAN_POINT('Ctrl Pts',(49.8482149490333,3.07098704024018,-229.612416871579));
#230240=CARTESIAN_POINT('Ctrl Pts',(52.0476351287711,4.41452605031363,-226.261821861581));
#230241=CARTESIAN_POINT('Ctrl Pts',(54.2475802160774,5.75650666229548,-222.910951011405));
#230242=CARTESIAN_POINT('Ctrl Pts',(56.4475253033837,7.09848727427732,-219.560080161228));
#230243=CARTESIAN_POINT('Ctrl Pts',(58.6480505159108,8.43876934344246,-216.208913928891));
#230244=CARTESIAN_POINT('Ctrl Pts',(60.8488504981511,9.77822104524949,-212.857597488374));
#230245=CARTESIAN_POINT('Ctrl Pts',(47.6460194974834,1.74602297076459,-232.961641432517));
#230246=CARTESIAN_POINT('Ctrl Pts',(49.8434528457034,3.09685564489722,-229.611730184141));
#230247=CARTESIAN_POINT('Ctrl Pts',(52.042354516691,4.44359608350473,-226.26114964818));
#230248=CARTESIAN_POINT('Ctrl Pts',(54.2417894607756,5.78876232686925,-222.91029092321));
#230249=CARTESIAN_POINT('Ctrl Pts',(56.4412244048602,7.13392857023377,-219.559432198239));
#230250=CARTESIAN_POINT('Ctrl Pts',(58.6412485837932,8.47737953915866,-216.208275719059));
#230251=CARTESIAN_POINT('Ctrl Pts',(60.8415519676109,9.81999143035988,-212.856967648949));
#230252=CARTESIAN_POINT('Ctrl Pts',(47.6439085847953,1.75733843295859,-232.961288761302));
#230253=CARTESIAN_POINT('Ctrl Pts',(49.8410717940384,3.10978994722575,-229.611386840422));
#230254=CARTESIAN_POINT('Ctrl Pts',(52.0397142106509,4.45813110010028,-226.26081354148));
#230255=CARTESIAN_POINT('Ctrl Pts',(54.2388940831247,5.80489015915614,-222.909960879112));
#230256=CARTESIAN_POINT('Ctrl Pts',(56.4380739555984,7.151649218212,-219.559108216744));
#230257=CARTESIAN_POINT('Ctrl Pts',(58.6378476177344,8.49668463701677,-216.207956614142));
#230258=CARTESIAN_POINT('Ctrl Pts',(60.8379027023408,9.84087662291507,-212.856652729236));
#230259=CARTESIAN_POINT('Ctrl Pts',(47.6422722132824,1.76718782952786,-232.960678696067));
#230260=CARTESIAN_POINT('Ctrl Pts',(49.8391375264504,3.12130996362475,-229.610790689353));
#230261=CARTESIAN_POINT('Ctrl Pts',(52.0375016868396,4.47128714932663,-226.260228329323));
#230262=CARTESIAN_POINT('Ctrl Pts',(54.2364107003475,5.81966765975101,-222.909384848415));
#230263=CARTESIAN_POINT('Ctrl Pts',(56.4353197138554,7.16804817017539,-219.558541367508));
#230264=CARTESIAN_POINT('Ctrl Pts',(58.6348306124533,8.51468948441525,-216.207397187139));
#230265=CARTESIAN_POINT('Ctrl Pts',(60.8346268351599,9.86047939512299,-212.856099681471));
#230266=CARTESIAN_POINT('Ctrl Pts',(47.6389054467951,1.78211913870348,-232.960962398579));
#230267=CARTESIAN_POINT('Ctrl Pts',(49.8355621025854,3.13772585835723,-229.611072178893));
#230268=CARTESIAN_POINT('Ctrl Pts',(52.033706981916,4.48921062136337,-226.260507824327));
#230269=CARTESIAN_POINT('Ctrl Pts',(54.2323930398121,5.83910740022999,-222.909662643248));
#230270=CARTESIAN_POINT('Ctrl Pts',(56.4310790977081,7.18900417909662,-219.558817462169));
#230271=CARTESIAN_POINT('Ctrl Pts',(58.6303629299522,8.5371712694402,-216.207671846982));
#230272=CARTESIAN_POINT('Ctrl Pts',(60.8299301929379,9.88449155844584,-212.856373094261));
#230273=CARTESIAN_POINT('Ctrl Pts',(47.6355386803079,1.79705044787909,-232.961246101092));
#230274=CARTESIAN_POINT('Ctrl Pts',(49.8319866787204,3.15414175308971,-229.611353668433));
#230275=CARTESIAN_POINT('Ctrl Pts',(52.0299122769924,4.5071340934001,-226.260787319329));
#230276=CARTESIAN_POINT('Ctrl Pts',(54.2283753792766,5.85854714070898,-222.90994043808));
#230277=CARTESIAN_POINT('Ctrl Pts',(56.4268384815609,7.20996018801785,-219.55909355683));
#230278=CARTESIAN_POINT('Ctrl Pts',(58.6258952474512,8.55965305446516,-216.207946506826));
#230279=CARTESIAN_POINT('Ctrl Pts',(60.825233550716,9.90850372176869,-212.856646507051));
#230280=CARTESIAN_POINT('Ctrl Pts',(47.6321910253286,1.81198694050772,-232.961532361149));
#230281=CARTESIAN_POINT('Ctrl Pts',(49.8284317983937,3.17056265356817,-229.61163754231));
#230282=CARTESIAN_POINT('Ctrl Pts',(52.026139583098,4.52506239807395,-226.261069085663));
#230283=CARTESIAN_POINT('Ctrl Pts',(54.22438120628,5.87799154637645,-222.910220412602));
#230284=CARTESIAN_POINT('Ctrl Pts',(56.422622829462,7.23092069467897,-219.559371739542));
#230285=CARTESIAN_POINT('Ctrl Pts',(58.6214540165528,8.58213917498653,-216.208223186853));
#230286=CARTESIAN_POINT('Ctrl Pts',(60.8205648517821,9.93252006210882,-212.856921883345));
#230287=CARTESIAN_POINT('Ctrl Pts',(47.628862493758,1.82692857762527,-232.96182118511));
#230288=CARTESIAN_POINT('Ctrl Pts',(49.8248974717912,3.18698851762863,-229.611923806209));
#230289=CARTESIAN_POINT('Ctrl Pts',(52.0223889083793,4.54299549104381,-226.26135312848));
#230290=CARTESIAN_POINT('Ctrl Pts',(54.2204105268588,5.89744057105422,-222.91050257153));
#230291=CARTESIAN_POINT('Ctrl Pts',(56.4184321453384,7.25188565106463,-219.559652014579));
#230292=CARTESIAN_POINT('Ctrl Pts',(58.6170392389817,8.60462958153552,-216.208501890991));
#230293=CARTESIAN_POINT('Ctrl Pts',(60.8159240956269,9.95654052871553,-212.857199226772));
#230294=CARTESIAN_POINT('Ctrl Pts',(47.602234241193,1.94646167456563,-232.964131776795));
#230295=CARTESIAN_POINT('Ctrl Pts',(49.7966228589716,3.3183954301123,-229.614213917398));
#230296=CARTESIAN_POINT('Ctrl Pts',(51.9923835106293,4.68646023480269,-226.263625471024));
#230297=CARTESIAN_POINT('Ctrl Pts',(54.1886450914894,6.05303276847634,-222.912759842952));
#230298=CARTESIAN_POINT('Ctrl Pts',(56.3849066723495,7.41960530214998,-219.561894214879));
#230299=CARTESIAN_POINT('Ctrl Pts',(58.5817210184137,8.78455283392743,-216.210731524094));
#230300=CARTESIAN_POINT('Ctrl Pts',(60.7787980463854,10.1487042615692,-212.859417974186));
#230301=CARTESIAN_POINT('Ctrl Pts',(47.5768298455065,2.06632401207208,-232.96660639255));
#230302=CARTESIAN_POINT('Ctrl Pts',(49.7696636517176,3.45012000579785,-229.616656935729));
#230303=CARTESIAN_POINT('Ctrl Pts',(51.9637873118318,4.83023142413465,-226.266043461076));
#230304=CARTESIAN_POINT('Ctrl Pts',(54.158383220178,6.2089205777349,-222.915156874141));
#230305=CARTESIAN_POINT('Ctrl Pts',(56.3529791285242,7.58760973133515,-219.564270287207));
#230306=CARTESIAN_POINT('Ctrl Pts',(58.5480957918528,8.96475038827362,-216.213090667097));
#230307=CARTESIAN_POINT('Ctrl Pts',(60.7434603178749,10.3411320720609,-212.861762587924));
#230308=CARTESIAN_POINT('Ctrl Pts',(47.5526556810106,2.18649568630384,-232.969248737689));
#230309=CARTESIAN_POINT('Ctrl Pts',(49.7440252884103,3.58214069800097,-229.619256142275));
#230310=CARTESIAN_POINT('Ctrl Pts',(51.9366046755093,4.97428639343047,-226.268610062602));
#230311=CARTESIAN_POINT('Ctrl Pts',(54.129628172195,6.36508038888444,-222.917696367826));
#230312=CARTESIAN_POINT('Ctrl Pts',(56.3226516688807,7.7558743843384,-219.56678267305));
#230313=CARTESIAN_POINT('Ctrl Pts',(58.5161645712576,9.14519694298261,-216.215581556974));
#230314=CARTESIAN_POINT('Ctrl Pts',(60.7099107655409,10.5337979996055,-212.864235131559));
#230315=CARTESIAN_POINT('Ctrl Pts',(47.4559590230269,2.66718238323085,-232.979818118251));
#230316=CARTESIAN_POINT('Ctrl Pts',(49.6414718351808,4.11022346681344,-229.629652968461));
#230317=CARTESIAN_POINT('Ctrl Pts',(51.8278741302197,5.55050627061373,-226.278876468708));
#230318=CARTESIAN_POINT('Ctrl Pts',(54.0146079802632,6.98971963348256,-222.927854342566));
#230319=CARTESIAN_POINT('Ctrl Pts',(56.2013418303068,8.4289329963514,-219.576832216423));
#230320=CARTESIAN_POINT('Ctrl Pts',(58.3884396888769,9.86698316181859,-216.225545116483));
#230321=CARTESIAN_POINT('Ctrl Pts',(60.5757125562048,11.3044617097837,-212.874125306097));
#230322=CARTESIAN_POINT('Ctrl Pts',(47.3789343509497,3.15281732296621,-232.993054381077));
#230323=CARTESIAN_POINT('Ctrl Pts',(49.5600425408639,4.64304306902027,-229.642534956489));
#230324=CARTESIAN_POINT('Ctrl Pts',(51.7417525219173,6.13126572956288,-226.291508540064));
#230325=CARTESIAN_POINT('Ctrl Pts',(53.9236899017093,7.61871011984863,-222.94028097047));
#230326=CARTESIAN_POINT('Ctrl Pts',(56.1056272815015,9.10615451013438,-219.589053400875));
#230327=CARTESIAN_POINT('Ctrl Pts',(58.2878135060677,10.5927527992689,-216.237608203082));
#230328=CARTESIAN_POINT('Ctrl Pts',(60.4701203002903,12.0789347832393,-212.886054712549));
#230329=CARTESIAN_POINT('Ctrl Pts',(47.3220782931503,3.64213739520988,-233.009326653747));
#230330=CARTESIAN_POINT('Ctrl Pts',(49.5001561272747,5.17923014873171,-229.65822098902));
#230331=CARTESIAN_POINT('Ctrl Pts',(51.6785800990322,6.71512263630363,-226.306791304678));
#230332=CARTESIAN_POINT('Ctrl Pts',(53.8571359353927,8.25054831515734,-222.955233810924));
#230333=CARTESIAN_POINT('Ctrl Pts',(56.0356917717532,9.78597399401105,-219.603676317171));
#230334=CARTESIAN_POINT('Ctrl Pts',(58.2143916305598,11.3208922926972,-216.251980359006));
#230335=CARTESIAN_POINT('Ctrl Pts',(60.3931615898891,12.8555608031383,-212.900215711346));
#230336=CARTESIAN_POINT('Ctrl Pts',(47.0946540619524,5.59941768418452,-233.074415744431));
#230337=CARTESIAN_POINT('Ctrl Pts',(49.2606104729176,7.3239784675775,-229.720965119143));
#230338=CARTESIAN_POINT('Ctrl Pts',(51.4258904074922,9.05055026326663,-226.367922363131));
#230339=CARTESIAN_POINT('Ctrl Pts',(53.5909200701262,10.7779010963922,-223.015045172743));
#230340=CARTESIAN_POINT('Ctrl Pts',(55.7559497327601,12.5052519295177,-219.662167982355));
#230341=CARTESIAN_POINT('Ctrl Pts',(57.9207041285279,14.2334502664104,-216.309468982699));
#230342=CARTESIAN_POINT('Ctrl Pts',(60.0853267482839,15.9620648827344,-212.956859706535));
#230343=CARTESIAN_POINT('Ctrl Pts',(47.1914720210979,7.6140088721643,-233.185323795226));
#230344=CARTESIAN_POINT('Ctrl Pts',(49.3672203068766,9.52128975296003,-229.826228944008));
#230345=CARTESIAN_POINT('Ctrl Pts',(51.5415920964213,11.4345056878504,-226.469384191172));
#230346=CARTESIAN_POINT('Ctrl Pts',(53.7154316537813,13.3500108047595,-223.113404278841));
#230347=CARTESIAN_POINT('Ctrl Pts',(55.8892712111413,15.2655159216685,-219.757424366509));
#230348=CARTESIAN_POINT('Ctrl Pts',(58.0625313135173,17.1835155618891,-216.402388112408));
#230349=CARTESIAN_POINT('Ctrl Pts',(60.2355063327765,19.10274141504,-213.047815750158));
#230350=CARTESIAN_POINT('Ctrl Pts',(47.6396641907623,9.56951109638858,-233.375524009166));
#230351=CARTESIAN_POINT('Ctrl Pts',(49.8405355389308,11.6556158167396,-230.003433166063));
#230352=CARTESIAN_POINT('Ctrl Pts',(52.0418116007037,13.7520462993107,-226.638133451275));
#230353=CARTESIAN_POINT('Ctrl Pts',(54.2429855256817,15.8525357612388,-223.275331821509));
#230354=CARTESIAN_POINT('Ctrl Pts',(56.4441594506596,17.9530252231669,-219.912530191744));
#230355=CARTESIAN_POINT('Ctrl Pts',(58.6452885751193,20.0579121947712,-216.552478218177));
#230356=CARTESIAN_POINT('Ctrl Pts',(60.846321628963,22.164968605821,-213.193734192871));
#230357=CARTESIAN_POINT('',(47.764389394009,6.457751620915,-232.249941470341));
#230358=CARTESIAN_POINT('Ctrl Pts',(47.7643209768376,6.45773200978314,-232.25005));
#230359=CARTESIAN_POINT('Ctrl Pts',(47.7428191347604,6.03142608206569,-232.25005));
#230360=CARTESIAN_POINT('Ctrl Pts',(47.736924890541,5.60456323298173,-232.25005));
#230361=CARTESIAN_POINT('Ctrl Pts',(47.7570432133228,4.73973393711202,-232.25005));
#230362=CARTESIAN_POINT('Ctrl Pts',(47.7839000023451,4.3022757671813,-232.25005));
#230363=CARTESIAN_POINT('Ctrl Pts',(47.8275275119679,3.86645886896212,-232.25005));
#230364=CARTESIAN_POINT('Ctrl Pts',(47.9644369063438,-4.51936301034905,
-232.25005));
#230365=CARTESIAN_POINT('Ctrl Pts',(47.9319477127382,-4.97119958827373,
-232.25005));
#230366=CARTESIAN_POINT('Ctrl Pts',(47.9174772002993,-5.4242563204813,-232.25005));
#230367=CARTESIAN_POINT('Ctrl Pts',(47.9248943476532,-6.33010682966948,
-232.25005));
#230368=CARTESIAN_POINT('Ctrl Pts',(47.9467635068849,-6.78180672474201,
-232.25005));
#230369=CARTESIAN_POINT('Ctrl Pts',(47.9866861404266,-7.23226624733622,
-232.25005));
#230370=CARTESIAN_POINT('Ctrl Pts',(47.9849458443841,-16.0452823276962,
-232.25005));
#230371=CARTESIAN_POINT('Ctrl Pts',(47.9462873350434,-16.4877633300649,
-232.25005));
#230372=CARTESIAN_POINT('Ctrl Pts',(47.925045029397,-16.9313785096498,-232.25005));
#230373=CARTESIAN_POINT('Ctrl Pts',(47.9174315480329,-17.8216218039863,
-232.25005));
#230374=CARTESIAN_POINT('Ctrl Pts',(47.9311272354818,-18.2671770665058,
-232.25005));
#230375=CARTESIAN_POINT('Ctrl Pts',(47.962113157865,-18.7116122763947,-232.25005));
#230376=CARTESIAN_POINT('',(47.7598796739981,-29.633055067729,-232.249824579212));
#230377=CARTESIAN_POINT('Ctrl Pts',(47.8203127214913,-27.1915604688603,
-232.25005));
#230378=CARTESIAN_POINT('Ctrl Pts',(47.7812806514964,-27.6015079559573,
-232.25005));
#230379=CARTESIAN_POINT('Ctrl Pts',(47.7568712560738,-28.0131227629508,
-232.250050000005));
#230380=CARTESIAN_POINT('Ctrl Pts',(47.7374545095719,-28.8282292839852,
-232.250050000005));
#230381=CARTESIAN_POINT('Ctrl Pts',(47.7417582300801,-29.2308218767449,
-232.25005));
#230382=CARTESIAN_POINT('Ctrl Pts',(47.7597386834877,-29.6330167878826,
-232.25005));
#230383=CARTESIAN_POINT('Ctrl Pts',(47.7600215786063,-29.6330588251263,
-232.249824579212));
#230384=CARTESIAN_POINT('Ctrl Pts',(47.7599867924269,-29.6343725853688,
-232.249899719474));
#230385=CARTESIAN_POINT('Ctrl Pts',(47.7599520024663,-29.6356863455112,
-232.249974859737));
#230386=CARTESIAN_POINT('Ctrl Pts',(47.7599172087245,-29.6370001055535,
-232.25005));
#230387=CARTESIAN_POINT('Ctrl Pts',(47.7644117008771,6.45952891261178,-232.25005));
#230388=CARTESIAN_POINT('Ctrl Pts',(47.7644272274268,6.45893708439671,-232.250013823447));
#230389=CARTESIAN_POINT('Ctrl Pts',(47.7644427532091,6.45834525616151,-232.249977646894));
#230390=CARTESIAN_POINT('Ctrl Pts',(47.7644582782241,6.45775342790618,-232.249941470341));
#230391=CARTESIAN_POINT('Origin',(48.1334350484927,-61.7961505568785,-218.306418983907));
#230392=CARTESIAN_POINT('Origin',(24.838300653577,28.3971299569735,-229.35005));
#230393=CARTESIAN_POINT('',(24.960358769668,29.3896529120211,-229.35005));
#230394=CARTESIAN_POINT('',(25.366775135568,29.2460791438418,-229.35005));
#230395=CARTESIAN_POINT('Origin',(-6.29739814579425E-15,-11.5034818258363,
-229.35005));
#230396=CARTESIAN_POINT('',(39.8203148590359,15.2984308769399,-229.35005));
#230397=CARTESIAN_POINT('Origin',(38.9907249661392,14.740057695632,-229.35005));
#230398=CARTESIAN_POINT('',(39.989972084972,14.7788545447883,-229.35005));
#230399=CARTESIAN_POINT('Origin',(-636.934816028482,-11.5034818258361,-229.35005));
#230400=CARTESIAN_POINT('Origin',(38.9907249661392,-37.7470213473046,-229.35005));
#230401=CARTESIAN_POINT('',(39.989972084972,-37.7858181964606,-229.35005));
#230402=CARTESIAN_POINT('',(39.8203148590358,-38.3053945286125,-229.35005));
#230403=CARTESIAN_POINT('Origin',(-6.29739814579425E-15,-11.5034818258363,
-229.35005));
#230404=CARTESIAN_POINT('Origin',(22.9178089794592,-52.5372975341153,-229.35005));
#230405=CARTESIAN_POINT('',(23.4054219364689,-53.410357442802,-229.35005));
#230406=CARTESIAN_POINT('',(22.9516892713016,-53.5367234322311,-229.35005));
#230407=CARTESIAN_POINT('Origin',(48.892180948596,36.2913696007177,-218.35005));
#230408=CARTESIAN_POINT('',(48.892180948596,32.9413696007177,-218.35005));
#230409=CARTESIAN_POINT('Origin',(48.892180948596,36.2913696007177,-218.35005));
#230410=CARTESIAN_POINT('Origin',(48.892180948596,36.2913696007177,-218.35005));
#230411=CARTESIAN_POINT('',(48.892180948596,32.9413696007177,-218.35005));
#230412=CARTESIAN_POINT('Origin',(48.1334350484927,-61.7961505568785,-218.35005));
#230413=CARTESIAN_POINT('',(48.1334350484927,-65.1461505568793,-218.35005));
#230414=CARTESIAN_POINT('Origin',(48.1334350484927,-61.7961505568785,-218.35005));
#230415=CARTESIAN_POINT('Origin',(48.1334350484927,-61.7961505568785,-218.35005));
#230416=CARTESIAN_POINT('',(48.1334350484927,-65.1461505568793,-218.35005));
#230417=CARTESIAN_POINT('Origin',(0.127542579976414,-12.8706479699377,-228.35005));
#230418=CARTESIAN_POINT('Origin',(55.2047656166361,-61.9923285455256,-228.35005));
#230419=CARTESIAN_POINT('Origin',(48.1954151687739,-68.8699303295103,-228.35005));
#230420=CARTESIAN_POINT('Origin',(0.127542579976414,-12.8706479699377,-228.35005));
#230421=CARTESIAN_POINT('Origin',(0.128459562639233,-12.6359082483571,-228.35005));
#230422=CARTESIAN_POINT('Origin',(48.6323674899383,42.9861279943057,-228.35005));
#230423=CARTESIAN_POINT('Origin',(55.5877717798047,36.0539745652106,-228.35005));
#230424=CARTESIAN_POINT('Origin',(0.128459562639233,-12.6359082483571,-228.35005));
#230425=CARTESIAN_POINT('Origin',(51.397926952212,-43.6786252257833,-167.906149834141));
#230426=CARTESIAN_POINT('Origin',(51.7304496786285,-70.1559157828803,-167.906149834141));
#230427=CARTESIAN_POINT('Origin',(0.,-12.9675000200281,-167.906149834141));
#230428=CARTESIAN_POINT('Origin',(51.3278340104563,17.8606293780317,-167.906149834141));
#230429=CARTESIAN_POINT('Origin',(51.6000409161409,44.3386087195339,-167.906149834141));
#230430=CARTESIAN_POINT('Origin',(0.,-12.9675000200281,-167.906149834141));
#230431=CARTESIAN_POINT('Ctrl Pts',(-43.8493461424558,-78.8521074299086,
-211.864982076876));
#230432=CARTESIAN_POINT('Ctrl Pts',(-21.0752244585295,-62.961249057474,
-239.042379319384));
#230433=CARTESIAN_POINT('Ctrl Pts',(-40.4601948759454,-78.0802943160701,
-211.86498207687));
#230434=CARTESIAN_POINT('Ctrl Pts',(-19.8470357167519,-61.333671538836,
-239.042379319393));
#230435=CARTESIAN_POINT('Ctrl Pts',(-36.4842840549755,-77.5339017897621,
-211.864982076872));
#230436=CARTESIAN_POINT('Ctrl Pts',(-17.4751640410206,-60.0398805476777,
-239.042379319393));
#230437=CARTESIAN_POINT('Ctrl Pts',(-31.6477754280485,-77.4599324799423,
-211.864982076871));
#230438=CARTESIAN_POINT('Ctrl Pts',(-14.5387717509043,-59.7364199365376,
-239.042379319393));
#230439=CARTESIAN_POINT('Ctrl Pts',(-29.3183793276549,-77.5317048145231,
-211.864982076871));
#230440=CARTESIAN_POINT('Ctrl Pts',(-13.1728997877445,-59.8076087424511,
-239.042379319393));
#230441=CARTESIAN_POINT('Ctrl Pts',(-27.7276393867415,-77.6574160379369,
-211.864982076871));
#230442=CARTESIAN_POINT('Ctrl Pts',(-12.3078514256087,-59.9884330330066,
-239.042379319393));
#230443=CARTESIAN_POINT('Ctrl Pts',(-26.1251285606442,-77.8260872807418,
-211.864982076871));
#230444=CARTESIAN_POINT('Ctrl Pts',(-11.4850984575113,-60.2258797863292,
-239.042379319393));
#230445=CARTESIAN_POINT('Ctrl Pts',(-24.504034109899,-77.9574724885703,
-211.864982076871));
#230446=CARTESIAN_POINT('Ctrl Pts',(-10.6757840293104,-60.3962257939897,
-239.042379319393));
#230447=CARTESIAN_POINT('Ctrl Pts',(-21.9997405622719,-78.0300903453287,
-211.864982076871));
#230448=CARTESIAN_POINT('Ctrl Pts',(-9.48446360027414,-60.4742901256445,
-239.042379319393));
#230449=CARTESIAN_POINT('Ctrl Pts',(-19.4557251513172,-77.9671468699367,
-211.864982076871));
#230450=CARTESIAN_POINT('Ctrl Pts',(-8.31856484927211,-60.385504961024,
-239.042379319393));
#230451=CARTESIAN_POINT('Ctrl Pts',(-17.7580995848034,-77.8323435614113,
-211.864982076871));
#230452=CARTESIAN_POINT('Ctrl Pts',(-7.55969975399382,-60.2185931298735,
-239.042379319393));
#230453=CARTESIAN_POINT('Ctrl Pts',(-16.0218744898441,-77.6472898528508,
-211.864982076871));
#230454=CARTESIAN_POINT('Ctrl Pts',(-6.78854926351807,-59.9912329899662,
-239.042379319393));
#230455=CARTESIAN_POINT('Ctrl Pts',(-14.2242428743346,-77.5073035049326,
-211.864982076871));
#230456=CARTESIAN_POINT('Ctrl Pts',(-5.98348432758041,-59.8179657745908,
-239.042379319393));
#230457=CARTESIAN_POINT('Ctrl Pts',(-11.5028152109754,-77.4528279485756,
-211.864982076871));
#230458=CARTESIAN_POINT('Ctrl Pts',(-4.76588582139345,-59.7403137615462,
-239.042379319393));
#230459=CARTESIAN_POINT('Ctrl Pts',(-8.76522200381794,-77.5576352824452,
-211.864982076872));
#230460=CARTESIAN_POINT('Ctrl Pts',(-3.56229847767841,-59.8420012365378,
-239.042379319393));
#230461=CARTESIAN_POINT('Ctrl Pts',(-6.93562803804477,-77.7358880723896,
-211.864982076871));
#230462=CARTESIAN_POINT('Ctrl Pts',(-2.78461998053008,-60.0255540781957,
-239.042379319393));
#230463=CARTESIAN_POINT('Ctrl Pts',(-5.53332725337535,-77.9148333735951,
-211.864982076871));
#230464=CARTESIAN_POINT('Ctrl Pts',(-2.20326121884502,-60.2085554263816,
-239.042379319393));
#230465=CARTESIAN_POINT('Ctrl Pts',(-4.54456283515166,-78.025500619718,
-211.864982076871));
#230466=CARTESIAN_POINT('Ctrl Pts',(-1.80191868227511,-60.318198378429,
-239.042379319393));
#230467=CARTESIAN_POINT('Ctrl Pts',(-3.03559134111532,-78.1451797699688,
-211.864982076871));
#230468=CARTESIAN_POINT('Ctrl Pts',(-1.20446149167326,-60.4340132220253,
-239.042379319393));
#230469=CARTESIAN_POINT('Ctrl Pts',(-1.5148280855032,-78.2155854299247,
-211.864982076871));
#230470=CARTESIAN_POINT('Ctrl Pts',(-0.606254863140601,-60.5036064966923,
-239.042379319393));
#230471=CARTESIAN_POINT('Ctrl Pts',(-0.502991918578145,-78.2289825342829,
-211.864982076871));
#230472=CARTESIAN_POINT('Ctrl Pts',(-0.203385156708754,-60.5196440064212,
-239.042379319393));
#230473=CARTESIAN_POINT('Ctrl Pts',(0.502991918602468,-78.2289825342829,
-211.864982076871));
#230474=CARTESIAN_POINT('Ctrl Pts',(0.203385156705297,-60.5196440064212,
-239.042379319393));
#230475=CARTESIAN_POINT('Ctrl Pts',(1.51482689495333,-78.2155855032342,
-211.864982076871));
#230476=CARTESIAN_POINT('Ctrl Pts',(0.606259313960994,-60.5036065477656,
-239.042379319393));
#230477=CARTESIAN_POINT('Ctrl Pts',(3.0355887465281,-78.1451799566583,-211.864982076871));
#230478=CARTESIAN_POINT('Ctrl Pts',(1.204456703078,-60.434013319996,-239.042379319393));
#230479=CARTESIAN_POINT('Ctrl Pts',(4.54456624804472,-78.0255001346635,
-211.864982076871));
#230480=CARTESIAN_POINT('Ctrl Pts',(1.80191683140721,-60.3181991676866,
-239.042379319393));
#230481=CARTESIAN_POINT('Ctrl Pts',(5.5333272533997,-77.9148333735951,-211.864982076871));
#230482=CARTESIAN_POINT('Ctrl Pts',(2.20326121884159,-60.2085554263816,
-239.042379319393));
#230483=CARTESIAN_POINT('Ctrl Pts',(6.93562803806916,-77.7358880723894,
-211.864982076871));
#230484=CARTESIAN_POINT('Ctrl Pts',(2.78461998052664,-60.0255540781959,
-239.042379319393));
#230485=CARTESIAN_POINT('Ctrl Pts',(8.76522200384232,-77.5576352824453,
-211.864982076871));
#230486=CARTESIAN_POINT('Ctrl Pts',(3.56229847767494,-59.8420012365377,
-239.042379319393));
#230487=CARTESIAN_POINT('Ctrl Pts',(11.5028152109998,-77.4528279485751,
-211.864982076871));
#230488=CARTESIAN_POINT('Ctrl Pts',(4.7658858213899,-59.7403137615466,-239.042379319393));
#230489=CARTESIAN_POINT('Ctrl Pts',(14.2242428743589,-77.5073035049326,
-211.864982076871));
#230490=CARTESIAN_POINT('Ctrl Pts',(5.98348432757681,-59.8179657745909,
-239.042379319393));
#230491=CARTESIAN_POINT('Ctrl Pts',(16.0218744898684,-77.6472898528505,
-211.864982076871));
#230492=CARTESIAN_POINT('Ctrl Pts',(6.78854926351442,-59.9912329899664,
-239.042379319393));
#230493=CARTESIAN_POINT('Ctrl Pts',(17.7580995848278,-77.832343561411,-211.864982076871));
#230494=CARTESIAN_POINT('Ctrl Pts',(7.55969975399014,-60.2185931298737,
-239.042379319393));
#230495=CARTESIAN_POINT('Ctrl Pts',(19.4557251513416,-77.9671468699364,
-211.864982076871));
#230496=CARTESIAN_POINT('Ctrl Pts',(8.31856484926843,-60.3855049610241,
-239.042379319393));
#230497=CARTESIAN_POINT('Ctrl Pts',(21.9997405622963,-78.0300903453282,
-211.864982076871));
#230498=CARTESIAN_POINT('Ctrl Pts',(9.48446360027046,-60.4742901256449,
-239.042379319393));
#230499=CARTESIAN_POINT('Ctrl Pts',(24.5040341099234,-77.9574724885699,
-211.864982076871));
#230500=CARTESIAN_POINT('Ctrl Pts',(10.6757840293067,-60.39622579399,-239.042379319393));
#230501=CARTESIAN_POINT('Ctrl Pts',(26.1251285606686,-77.8260872807413,
-211.864982076871));
#230502=CARTESIAN_POINT('Ctrl Pts',(11.4850984575076,-60.2258797863295,
-239.042379319393));
#230503=CARTESIAN_POINT('Ctrl Pts',(27.7276393867659,-77.6574160379364,
-211.864982076871));
#230504=CARTESIAN_POINT('Ctrl Pts',(12.307851425605,-59.9884330330069,-239.042379319393));
#230505=CARTESIAN_POINT('Ctrl Pts',(29.3183793276793,-77.5317048145225,
-211.864982076871));
#230506=CARTESIAN_POINT('Ctrl Pts',(13.1728997877408,-59.8076087424512,
-239.042379319393));
#230507=CARTESIAN_POINT('Ctrl Pts',(31.6477754280729,-77.4599324799418,
-211.864982076871));
#230508=CARTESIAN_POINT('Ctrl Pts',(14.5387717509006,-59.7364199365383,
-239.042379319393));
#230509=CARTESIAN_POINT('Ctrl Pts',(36.4842840550008,-77.5339017897612,
-211.864982076871));
#230510=CARTESIAN_POINT('Ctrl Pts',(17.4751640410175,-60.0398805476776,
-239.042379319393));
#230511=CARTESIAN_POINT('Ctrl Pts',(40.4601948759724,-78.0802943160702,
-211.864982076872));
#230512=CARTESIAN_POINT('Ctrl Pts',(19.8470357167496,-61.3336715388389,
-239.042379319392));
#230513=CARTESIAN_POINT('Ctrl Pts',(43.8493461424807,-78.8521074299069,
-211.864982076868));
#230514=CARTESIAN_POINT('Ctrl Pts',(21.0752244585277,-62.9612490574688,
-239.0423793194));
#230515=CARTESIAN_POINT('Ctrl Pts',(25.5478248690252,37.5021404050027,-238.870094813919));
#230516=CARTESIAN_POINT('Ctrl Pts',(31.0974823253722,43.1081780439896,-229.864162540276));
#230517=CARTESIAN_POINT('Ctrl Pts',(36.6471397817123,48.7142156829799,-220.858230266689));
#230518=CARTESIAN_POINT('Ctrl Pts',(42.1967972380602,54.3202533219665,-211.852297993045));
#230519=CARTESIAN_POINT('Ctrl Pts',(23.7340150363558,36.8170136325857,-238.870094813938));
#230520=CARTESIAN_POINT('Ctrl Pts',(28.8928311974199,42.3227771550256,-229.864162540312));
#230521=CARTESIAN_POINT('Ctrl Pts',(34.0516473584841,47.8285406774658,-220.858230266679));
#230522=CARTESIAN_POINT('Ctrl Pts',(39.2104635195483,53.3343041999057,-211.852297993053));
#230523=CARTESIAN_POINT('Ctrl Pts',(21.2241728789609,36.320693756165,-238.870094813932));
#230524=CARTESIAN_POINT('Ctrl Pts',(25.8876894275506,41.7749009515431,-229.864162540305));
#230525=CARTESIAN_POINT('Ctrl Pts',(30.5512059761403,47.2291081469212,-220.858230266679));
#230526=CARTESIAN_POINT('Ctrl Pts',(35.21472252473,52.6833153422993,-211.852297993052));
#230527=CARTESIAN_POINT('Ctrl Pts',(18.1531449537935,36.3323039390022,-238.870094813935));
#230528=CARTESIAN_POINT('Ctrl Pts',(22.2007701700553,41.8486188105145,-229.864162540308));
#230529=CARTESIAN_POINT('Ctrl Pts',(26.2483953863169,47.3649336820266,-220.85823026668));
#230530=CARTESIAN_POINT('Ctrl Pts',(30.2960206025786,52.8812485535388,-211.852297993052));
#230531=CARTESIAN_POINT('Ctrl Pts',(16.4944071585121,36.4865308984241,-238.870094813934));
#230532=CARTESIAN_POINT('Ctrl Pts',(20.2017948578975,42.0687249742654,-229.864162540306));
#230533=CARTESIAN_POINT('Ctrl Pts',(23.9091825572828,47.6509190501065,-220.858230266679));
#230534=CARTESIAN_POINT('Ctrl Pts',(27.6165702566681,53.2331131259477,-211.852297993052));
#230535=CARTESIAN_POINT('Ctrl Pts',(15.4128369679802,36.6843043274095,-238.870094813934));
#230536=CARTESIAN_POINT('Ctrl Pts',(18.8901600859934,42.3335714329084,-229.864162540306));
#230537=CARTESIAN_POINT('Ctrl Pts',(22.3674832040067,47.9828385384071,-220.858230266679));
#230538=CARTESIAN_POINT('Ctrl Pts',(25.8448063220201,53.632105643906,-211.852297993052));
#230539=CARTESIAN_POINT('Ctrl Pts',(14.3520270002835,36.9260614299673,-238.870094813935));
#230540=CARTESIAN_POINT('Ctrl Pts',(17.5982791985805,42.6550627945494,-229.864162540306));
#230541=CARTESIAN_POINT('Ctrl Pts',(20.8445313968775,48.3840641591314,-220.858230266679));
#230542=CARTESIAN_POINT('Ctrl Pts',(24.0907835951745,54.1130655237135,-211.852297993052));
#230543=CARTESIAN_POINT('Ctrl Pts',(13.2987772727661,37.1178867569915,-238.870094813935));
#230544=CARTESIAN_POINT('Ctrl Pts',(16.2995186126252,42.9177482501692,-229.864162540307));
#230545=CARTESIAN_POINT('Ctrl Pts',(19.3002599524843,48.7176097433469,-220.858230266679));
#230546=CARTESIAN_POINT('Ctrl Pts',(22.3010012923435,54.5174712365246,-211.852297993051));
#230547=CARTESIAN_POINT('Ctrl Pts',(11.7222378941044,37.2692384770327,-238.870094813934));
#230548=CARTESIAN_POINT('Ctrl Pts',(14.3287171552671,43.1379437466391,-229.864162540307));
#230549=CARTESIAN_POINT('Ctrl Pts',(16.9351964164299,49.0066490162454,-220.858230266679));
#230550=CARTESIAN_POINT('Ctrl Pts',(19.5416756775926,54.8753542858517,-211.852297993052));
#230551=CARTESIAN_POINT('Ctrl Pts',(10.1381417281494,37.288217650217,-238.870094813935));
#230552=CARTESIAN_POINT('Ctrl Pts',(12.3460138186247,43.1833567383484,-229.864162540307));
#230553=CARTESIAN_POINT('Ctrl Pts',(14.5538859091001,49.0784958264797,-220.858230266679));
#230554=CARTESIAN_POINT('Ctrl Pts',(16.7617579995755,54.973634914611,-211.852297993051));
#230555=CARTESIAN_POINT('Ctrl Pts',(9.0694859968433,37.2108732070893,-238.870094813934));
#230556=CARTESIAN_POINT('Ctrl Pts',(11.0234698129422,43.0965115564161,-229.864162540306));
#230557=CARTESIAN_POINT('Ctrl Pts',(12.9774536290411,48.9821499057428,-220.858230266679));
#230558=CARTESIAN_POINT('Ctrl Pts',(14.93143744514,54.8677882550696,-211.852297993052));
#230559=CARTESIAN_POINT('Ctrl Pts',(8.09600002160285,37.0974623895316,-238.870094813934));
#230560=CARTESIAN_POINT('Ctrl Pts',(9.83246501086473,42.9648667488742,-229.864162540306));
#230561=CARTESIAN_POINT('Ctrl Pts',(11.5689300001266,48.8322711082166,-220.858230266679));
#230562=CARTESIAN_POINT('Ctrl Pts',(13.3053949893885,54.6996754675592,-211.852297993052));
#230563=CARTESIAN_POINT('Ctrl Pts',(7.21039615408183,37.0252028273246,-238.870094813934));
#230564=CARTESIAN_POINT('Ctrl Pts',(8.76313299670731,42.8850718970782,-229.864162540307));
#230565=CARTESIAN_POINT('Ctrl Pts',(10.3158698393328,48.7449409668318,-220.858230266679));
#230566=CARTESIAN_POINT('Ctrl Pts',(11.8686066819583,54.6048100365855,-211.852297993052));
#230567=CARTESIAN_POINT('Ctrl Pts',(5.85470835560891,37.0124469887412,-238.870094813934));
#230568=CARTESIAN_POINT('Ctrl Pts',(7.14898080710293,42.8806994061336,-229.864162540306));
#230569=CARTESIAN_POINT('Ctrl Pts',(8.44325325859696,48.7489518235258,-220.858230266679));
#230570=CARTESIAN_POINT('Ctrl Pts',(9.73752571009099,54.6172042409181,-211.852297993051));
#230571=CARTESIAN_POINT('Ctrl Pts',(4.4991133918818,37.0982029765426,-238.870094813934));
#230572=CARTESIAN_POINT('Ctrl Pts',(5.53799235246699,42.9924849109515,-229.864162540307));
#230573=CARTESIAN_POINT('Ctrl Pts',(6.57687131305217,48.8867668453602,-220.858230266679));
#230574=CARTESIAN_POINT('Ctrl Pts',(7.61575027363735,54.7810487797691,-211.852297993052));
#230575=CARTESIAN_POINT('Ctrl Pts',(3.61373337750269,37.2187456251595,-238.870094813934));
#230576=CARTESIAN_POINT('Ctrl Pts',(4.47509554657543,43.143583333024,-229.864162540306));
#230577=CARTESIAN_POINT('Ctrl Pts',(5.33645771564818,49.0684210408883,-220.858230266679));
#230578=CARTESIAN_POINT('Ctrl Pts',(6.19781988472092,54.9932587487528,-211.852297993052));
#230579=CARTESIAN_POINT('Ctrl Pts',(2.91021678336389,37.3395607013659,-238.870094813934));
#230580=CARTESIAN_POINT('Ctrl Pts',(3.621152681702,43.2962952860814,-229.864162540307));
#230581=CARTESIAN_POINT('Ctrl Pts',(4.33208858004011,49.2530298707968,-220.858230266679));
#230582=CARTESIAN_POINT('Ctrl Pts',(5.04302447837822,55.2097644555123,-211.852297993052));
#230583=CARTESIAN_POINT('Ctrl Pts',(2.37632997378629,37.4191211557246,-238.870094813935));
#230584=CARTESIAN_POINT('Ctrl Pts',(2.9659120800303,43.3985012706933,-229.864162540306));
#230585=CARTESIAN_POINT('Ctrl Pts',(3.5554941862743,49.3778813856621,-220.858230266679));
#230586=CARTESIAN_POINT('Ctrl Pts',(4.14507629251831,55.3572615006307,-211.852297993052));
#230587=CARTESIAN_POINT('Ctrl Pts',(1.58453082874124,37.5028233147248,-238.870094813934));
#230588=CARTESIAN_POINT('Ctrl Pts',(1.98012592383798,43.5079032854707,-229.864162540307));
#230589=CARTESIAN_POINT('Ctrl Pts',(2.37572101893471,49.5129832562166,-220.858230266679));
#230590=CARTESIAN_POINT('Ctrl Pts',(2.77131611403145,55.5180632269626,-211.852297993052));
#230591=CARTESIAN_POINT('Ctrl Pts',(0.79519346259745,37.5528208103196,-238.870094813934));
#230592=CARTESIAN_POINT('Ctrl Pts',(0.991502132242674,43.5735821125591,
-229.864162540306));
#230593=CARTESIAN_POINT('Ctrl Pts',(1.1878108018879,49.5943434147985,-220.858230266679));
#230594=CARTESIAN_POINT('Ctrl Pts',(1.38411947153312,55.615104717038,-211.852297993052));
#230595=CARTESIAN_POINT('Ctrl Pts',(0.266260901836723,37.5640986908796,
-238.870094813934));
#230596=CARTESIAN_POINT('Ctrl Pts',(0.330758472424439,43.5882172364105,
-229.864162540306));
#230597=CARTESIAN_POINT('Ctrl Pts',(0.395256043012154,49.6123357819414,
-220.858230266679));
#230598=CARTESIAN_POINT('Ctrl Pts',(0.45975361359987,55.6364543274722,-211.852297993052));
#230599=CARTESIAN_POINT('Ctrl Pts',(-0.266261156428491,37.5640986908796,
-238.870094813935));
#230600=CARTESIAN_POINT('Ctrl Pts',(-0.330758075650379,43.5882172364105,
-229.864162540306));
#230601=CARTESIAN_POINT('Ctrl Pts',(-0.395254994872268,49.6123357819414,
-220.858230266679));
#230602=CARTESIAN_POINT('Ctrl Pts',(-0.459751914094156,55.6364543274723,
-211.852297993052));
#230603=CARTESIAN_POINT('Ctrl Pts',(-0.795196360647825,37.5528209283231,
-238.870094813934));
#230604=CARTESIAN_POINT('Ctrl Pts',(-0.991503022362771,43.5735822101004,
-229.864162540306));
#230605=CARTESIAN_POINT('Ctrl Pts',(-1.18780968407772,49.5943434918777,
-220.858230266679));
#230606=CARTESIAN_POINT('Ctrl Pts',(-1.38411634579266,55.6151047736551,
-211.852297993051));
#230607=CARTESIAN_POINT('Ctrl Pts',(-1.58452896877659,37.5028231831529,
-238.870094813935));
#230608=CARTESIAN_POINT('Ctrl Pts',(-1.98012255687567,43.5079033550423,
-229.864162540307));
#230609=CARTESIAN_POINT('Ctrl Pts',(-2.37571614497474,49.5129835269317,
-220.858230266679));
#230610=CARTESIAN_POINT('Ctrl Pts',(-2.77130973307382,55.5180636988211,
-211.852297993052));
#230611=CARTESIAN_POINT('Ctrl Pts',(-2.37632882947295,37.4191215872896,
-238.870094813934));
#230612=CARTESIAN_POINT('Ctrl Pts',(-2.96591227679258,43.3985013387235,
-229.864162540306));
#230613=CARTESIAN_POINT('Ctrl Pts',(-3.5554957241122,49.3778810901573,-220.858230266679));
#230614=CARTESIAN_POINT('Ctrl Pts',(-4.14507917143183,55.3572608415911,
-211.852297993052));
#230615=CARTESIAN_POINT('Ctrl Pts',(-2.91021703795575,37.3395607013659,
-238.870094813934));
#230616=CARTESIAN_POINT('Ctrl Pts',(-3.62115228492807,43.2962952860814,
-229.864162540307));
#230617=CARTESIAN_POINT('Ctrl Pts',(-4.33208753190037,49.2530298707968,
-220.858230266679));
#230618=CARTESIAN_POINT('Ctrl Pts',(-5.0430227788727,55.2097644555124,-211.852297993052));
#230619=CARTESIAN_POINT('Ctrl Pts',(-3.61373363209456,37.2187456251595,
-238.870094813934));
#230620=CARTESIAN_POINT('Ctrl Pts',(-4.47509514980151,43.143583333024,-229.864162540306));
#230621=CARTESIAN_POINT('Ctrl Pts',(-5.33645666750845,49.0684210408883,
-220.858230266679));
#230622=CARTESIAN_POINT('Ctrl Pts',(-6.1978181852154,54.9932587487528,-211.852297993052));
#230623=CARTESIAN_POINT('Ctrl Pts',(-4.49911364647367,37.0982029765426,
-238.870094813935));
#230624=CARTESIAN_POINT('Ctrl Pts',(-5.53799195569307,42.9924849109514,
-229.864162540306));
#230625=CARTESIAN_POINT('Ctrl Pts',(-6.57687026491244,48.8867668453602,
-220.858230266679));
#230626=CARTESIAN_POINT('Ctrl Pts',(-7.61574857413184,54.781048779769,-211.852297993052));
#230627=CARTESIAN_POINT('Ctrl Pts',(-5.85470861020079,37.0124469887413,
-238.870094813934));
#230628=CARTESIAN_POINT('Ctrl Pts',(-7.14898041032902,42.8806994061337,
-229.864162540306));
#230629=CARTESIAN_POINT('Ctrl Pts',(-8.44325221045725,48.7489518235258,
-220.858230266679));
#230630=CARTESIAN_POINT('Ctrl Pts',(-9.73752401058548,54.6172042409182,
-211.852297993052));
#230631=CARTESIAN_POINT('Ctrl Pts',(-7.21039640867369,37.0252028273246,
-238.870094813935));
#230632=CARTESIAN_POINT('Ctrl Pts',(-8.7631325999334,42.8850718970782,-229.864162540307));
#230633=CARTESIAN_POINT('Ctrl Pts',(-10.3158687911931,48.7449409668318,
-220.858230266679));
#230634=CARTESIAN_POINT('Ctrl Pts',(-11.8686049824528,54.6048100365855,
-211.852297993051));
#230635=CARTESIAN_POINT('Ctrl Pts',(-8.09600027619472,37.0974623895316,
-238.870094813934));
#230636=CARTESIAN_POINT('Ctrl Pts',(-9.83246461409083,42.9648667488742,
-229.864162540306));
#230637=CARTESIAN_POINT('Ctrl Pts',(-11.5689289519869,48.8322711082166,
-220.858230266679));
#230638=CARTESIAN_POINT('Ctrl Pts',(-13.305393289883,54.6996754675591,-211.852297993052));
#230639=CARTESIAN_POINT('Ctrl Pts',(-9.06948625143518,37.2108732070893,
-238.870094813935));
#230640=CARTESIAN_POINT('Ctrl Pts',(-11.0234694161683,43.0965115564161,
-229.864162540306));
#230641=CARTESIAN_POINT('Ctrl Pts',(-12.9774525809014,48.9821499057428,
-220.858230266679));
#230642=CARTESIAN_POINT('Ctrl Pts',(-14.9314357456345,54.8677882550697,
-211.852297993052));
#230643=CARTESIAN_POINT('Ctrl Pts',(-10.1381419827413,37.288217650217,-238.870094813934));
#230644=CARTESIAN_POINT('Ctrl Pts',(-12.3460134218509,43.1833567383484,
-229.864162540306));
#230645=CARTESIAN_POINT('Ctrl Pts',(-14.5538848609604,49.0784958264796,
-220.858230266679));
#230646=CARTESIAN_POINT('Ctrl Pts',(-16.76175630007,54.9736349146109,-211.852297993052));
#230647=CARTESIAN_POINT('Ctrl Pts',(-11.7222381486963,37.2692384770326,
-238.870094813935));
#230648=CARTESIAN_POINT('Ctrl Pts',(-14.3287167584933,43.1379437466391,
-229.864162540307));
#230649=CARTESIAN_POINT('Ctrl Pts',(-16.9351953682902,49.0066490162454,
-220.858230266679));
#230650=CARTESIAN_POINT('Ctrl Pts',(-19.5416739780872,54.8753542858518,
-211.852297993052));
#230651=CARTESIAN_POINT('Ctrl Pts',(-13.2987775273579,37.1178867569916,
-238.870094813934));
#230652=CARTESIAN_POINT('Ctrl Pts',(-16.2995182158513,42.9177482501693,
-229.864162540306));
#230653=CARTESIAN_POINT('Ctrl Pts',(-19.3002589043446,48.7176097433469,
-220.858230266679));
#230654=CARTESIAN_POINT('Ctrl Pts',(-22.300999592838,54.5174712365245,-211.852297993052));
#230655=CARTESIAN_POINT('Ctrl Pts',(-14.3520272548754,36.9260614299673,
-238.870094813934));
#230656=CARTESIAN_POINT('Ctrl Pts',(-17.5982788018066,42.6550627945494,
-229.864162540306));
#230657=CARTESIAN_POINT('Ctrl Pts',(-20.8445303487378,48.3840641591314,
-220.858230266679));
#230658=CARTESIAN_POINT('Ctrl Pts',(-24.0907818956689,54.1130655237136,
-211.852297993052));
#230659=CARTESIAN_POINT('Ctrl Pts',(-15.4128372225721,36.6843043274095,
-238.870094813934));
#230660=CARTESIAN_POINT('Ctrl Pts',(-18.8901596892196,42.3335714329084,
-229.864162540306));
#230661=CARTESIAN_POINT('Ctrl Pts',(-22.367482155867,47.9828385384072,-220.858230266679));
#230662=CARTESIAN_POINT('Ctrl Pts',(-25.8448046225145,53.632105643906,-211.852297993052));
#230663=CARTESIAN_POINT('Ctrl Pts',(-16.494407413104,36.4865308984241,-238.870094813934));
#230664=CARTESIAN_POINT('Ctrl Pts',(-20.2017944611236,42.0687249742654,
-229.864162540306));
#230665=CARTESIAN_POINT('Ctrl Pts',(-23.9091815091431,47.6509190501066,
-220.858230266679));
#230666=CARTESIAN_POINT('Ctrl Pts',(-27.6165685571627,53.2331131259478,
-211.852297993052));
#230667=CARTESIAN_POINT('Ctrl Pts',(-18.1531452083854,36.3323039390022,
-238.870094813935));
#230668=CARTESIAN_POINT('Ctrl Pts',(-22.2007697732813,41.8486188105144,
-229.864162540307));
#230669=CARTESIAN_POINT('Ctrl Pts',(-26.2483943381771,47.3649336820265,
-220.858230266679));
#230670=CARTESIAN_POINT('Ctrl Pts',(-30.2960189030729,52.8812485535387,
-211.852297993051));
#230671=CARTESIAN_POINT('Ctrl Pts',(-21.2241730962565,36.3206937563061,
-238.870094813934));
#230672=CARTESIAN_POINT('Ctrl Pts',(-25.8876889860007,41.7749009524383,
-229.864162540306));
#230673=CARTESIAN_POINT('Ctrl Pts',(-30.5512048757446,47.2291081485709,
-220.85823026668));
#230674=CARTESIAN_POINT('Ctrl Pts',(-35.2147207654887,52.6833153447033,
-211.852297993052));
#230675=CARTESIAN_POINT('Ctrl Pts',(-23.7340152164193,36.8170136178475,
-238.870094813936));
#230676=CARTESIAN_POINT('Ctrl Pts',(-28.8928307114097,42.3227771387571,
-229.864162540307));
#230677=CARTESIAN_POINT('Ctrl Pts',(-34.0516462064001,47.8285406596655,
-220.858230266679));
#230678=CARTESIAN_POINT('Ctrl Pts',(-39.2104617013909,53.3343041805747,
-211.85229799305));
#230679=CARTESIAN_POINT('Ctrl Pts',(-25.547825019704,37.5021403657523,-238.870094813925));
#230680=CARTESIAN_POINT('Ctrl Pts',(-31.0974818022918,43.1081779989934,
-229.864162540309));
#230681=CARTESIAN_POINT('Ctrl Pts',(-36.6471385848807,48.7142156322395,
-220.858230266681));
#230682=CARTESIAN_POINT('Ctrl Pts',(-42.1967953674649,54.320253265481,-211.852297993061));
#230683=CARTESIAN_POINT('Ctrl Pts',(48.9714493645238,-32.4976365372143,
-239.032601429863));
#230684=CARTESIAN_POINT('Ctrl Pts',(68.1913744168868,-58.588595799019,-211.730755606268));
#230685=CARTESIAN_POINT('Ctrl Pts',(47.6504140161628,-30.9809716432943,
-239.032601429841));
#230686=CARTESIAN_POINT('Ctrl Pts',(66.0438929094031,-54.9590042342752,
-211.730755606272));
#230687=CARTESIAN_POINT('Ctrl Pts',(46.5919797891444,-28.6187972486599,
-239.032601429843));
#230688=CARTESIAN_POINT('Ctrl Pts',(64.3781819143446,-49.9473558418611,
-211.730755606271));
#230689=CARTESIAN_POINT('Ctrl Pts',(46.3023719972087,-25.6595919193811,
-239.032601429843));
#230690=CARTESIAN_POINT('Ctrl Pts',(63.9692632136205,-43.762285990858,-211.730755606272));
#230691=CARTESIAN_POINT('Ctrl Pts',(46.3453291243135,-24.2216224913335,
-239.032601429843));
#230692=CARTESIAN_POINT('Ctrl Pts',(64.0706036090694,-40.7439486410264,
-211.730755606272));
#230693=CARTESIAN_POINT('Ctrl Pts',(46.4942182564745,-23.2800468285249,
-239.032601429843));
#230694=CARTESIAN_POINT('Ctrl Pts',(64.3397924421248,-38.7400276918009,
-211.730755606272));
#230695=CARTESIAN_POINT('Ctrl Pts',(46.6823308842909,-22.4376754428628,
-239.032601429843));
#230696=CARTESIAN_POINT('Ctrl Pts',(64.6771567767455,-36.9265599675944,
-211.730755606272));
#230697=CARTESIAN_POINT('Ctrl Pts',(46.8110566085946,-21.6771313665435,
-239.032601429843));
#230698=CARTESIAN_POINT('Ctrl Pts',(64.9159602271999,-35.2663729129392,
-211.730755606272));
#230699=CARTESIAN_POINT('Ctrl Pts',(46.8864232013851,-20.5344885406242,
-239.032601429843));
#230700=CARTESIAN_POINT('Ctrl Pts',(65.0656320382587,-32.7370789599851,
-211.730755606271));
#230701=CARTESIAN_POINT('Ctrl Pts',(46.845613352649,-19.389471894004,-239.032601429842));
#230702=CARTESIAN_POINT('Ctrl Pts',(65.0024851991802,-30.205094760215,-211.730755606272));
#230703=CARTESIAN_POINT('Ctrl Pts',(46.739717205202,-18.6241517464968,-239.032601429843));
#230704=CARTESIAN_POINT('Ctrl Pts',(64.8208630220631,-28.539554521699,-211.730755606272));
#230705=CARTESIAN_POINT('Ctrl Pts',(46.5950583390951,-17.8704826264274,
-239.032601429843));
#230706=CARTESIAN_POINT('Ctrl Pts',(64.5773028603203,-26.9236650389039,
-211.730755606272));
#230707=CARTESIAN_POINT('Ctrl Pts',(46.4891834572756,-17.1171663742141,
-239.032601429843));
#230708=CARTESIAN_POINT('Ctrl Pts',(64.4023778490554,-25.3332388913667,
-211.730755606272));
#230709=CARTESIAN_POINT('Ctrl Pts',(46.4453565014347,-15.9661997524868,
-239.032601429843));
#230710=CARTESIAN_POINT('Ctrl Pts',(64.3295185111446,-22.9500603856902,
-211.730755606271));
#230711=CARTESIAN_POINT('Ctrl Pts',(46.5193900629931,-14.8111705824743,
-239.032601429843));
#230712=CARTESIAN_POINT('Ctrl Pts',(64.443529180052,-20.5764219053293,-211.730755606272));
#230713=CARTESIAN_POINT('Ctrl Pts',(46.6471770799421,-14.0499533302827,
-239.032601429843));
#230714=CARTESIAN_POINT('Ctrl Pts',(64.6432253119956,-19.0049914961272,
-211.730755606272));
#230715=CARTESIAN_POINT('Ctrl Pts',(46.7740202606564,-13.4754604930206,
-239.032601429843));
#230716=CARTESIAN_POINT('Ctrl Pts',(64.8432542225078,-17.8091893041105,
-211.730755606272));
#230717=CARTESIAN_POINT('Ctrl Pts',(46.8513541209764,-13.0740155121622,
-239.032601429843));
#230718=CARTESIAN_POINT('Ctrl Pts',(64.9641969010104,-16.980210969671,-211.730755606271));
#230719=CARTESIAN_POINT('Ctrl Pts',(46.9348053643729,-12.4640324698742,
-239.032601429843));
#230720=CARTESIAN_POINT('Ctrl Pts',(65.0935448562552,-15.7339405894364,
-211.730755606272));
#230721=CARTESIAN_POINT('Ctrl Pts',(46.9850328086675,-11.8494593400854,
-239.032601429843));
#230722=CARTESIAN_POINT('Ctrl Pts',(65.171164912913,-14.4848476258101,-211.730755606272));
#230723=CARTESIAN_POINT('Ctrl Pts',(46.9961709729731,-11.4388750292095,
-239.032601429843));
#230724=CARTESIAN_POINT('Ctrl Pts',(65.1884659210897,-13.6502250547399,
-211.730755606272));
#230725=CARTESIAN_POINT('Ctrl Pts',(46.9961709729731,-11.0289590886771,
-239.032601429843));
#230726=CARTESIAN_POINT('Ctrl Pts',(65.1884659210897,-12.8146289801201,
-211.730755606272));
#230727=CARTESIAN_POINT('Ctrl Pts',(46.9850328086376,-10.6183760206315,
-239.032601429842));
#230728=CARTESIAN_POINT('Ctrl Pts',(65.1711648319807,-11.980003483899,-211.730755606272));
#230729=CARTESIAN_POINT('Ctrl Pts',(46.9348056898163,-10.0038043022318,
-239.032601429843));
#230730=CARTESIAN_POINT('Ctrl Pts',(65.093544987819,-10.7309166067835,-211.730755606272));
#230731=CARTESIAN_POINT('Ctrl Pts',(46.8513537675148,-9.39381595500219,
-239.032601429843));
#230732=CARTESIAN_POINT('Ctrl Pts',(64.9641971936048,-9.48464435696854,
-211.730755606272));
#230733=CARTESIAN_POINT('Ctrl Pts',(46.7740202606564,-8.99237362486574,
-239.032601429843));
#230734=CARTESIAN_POINT('Ctrl Pts',(64.8432542225078,-8.65566473074882,
-211.730755606272));
#230735=CARTESIAN_POINT('Ctrl Pts',(46.6471770799421,-8.41788078760364,
-239.032601429843));
#230736=CARTESIAN_POINT('Ctrl Pts',(64.6432253119957,-7.45986253873205,
-211.730755606272));
#230737=CARTESIAN_POINT('Ctrl Pts',(46.5193900629931,-7.65666353541205,
-239.032601429843));
#230738=CARTESIAN_POINT('Ctrl Pts',(64.4435291800518,-5.88843212952995,
-211.730755606271));
#230739=CARTESIAN_POINT('Ctrl Pts',(46.4453565014347,-6.50163436539958,
-239.032601429843));
#230740=CARTESIAN_POINT('Ctrl Pts',(64.3295185111447,-3.51479364916907,
-211.730755606272));
#230741=CARTESIAN_POINT('Ctrl Pts',(46.4891834572756,-5.35066774367227,
-239.032601429843));
#230742=CARTESIAN_POINT('Ctrl Pts',(64.4023778490553,-1.13161514349255,
-211.730755606272));
#230743=CARTESIAN_POINT('Ctrl Pts',(46.5950583390951,-4.59735149145896,
-239.032601429843));
#230744=CARTESIAN_POINT('Ctrl Pts',(64.5773028603203,0.458811004044723,
-211.730755606272));
#230745=CARTESIAN_POINT('Ctrl Pts',(46.739717205202,-3.84368237138963,-239.032601429843));
#230746=CARTESIAN_POINT('Ctrl Pts',(64.8208630220631,2.07470048683978,-211.730755606272));
#230747=CARTESIAN_POINT('Ctrl Pts',(46.8456133526491,-3.07836222388228,
-239.032601429843));
#230748=CARTESIAN_POINT('Ctrl Pts',(65.0024851991801,3.74024072535572,-211.730755606271));
#230749=CARTESIAN_POINT('Ctrl Pts',(46.8864232013849,-1.93334557726219,
-239.032601429842));
#230750=CARTESIAN_POINT('Ctrl Pts',(65.0656320382587,6.27222492512578,-211.730755606272));
#230751=CARTESIAN_POINT('Ctrl Pts',(46.8110566085948,-0.790702751342818,
-239.032601429843));
#230752=CARTESIAN_POINT('Ctrl Pts',(64.9159602271998,8.80151887808002,-211.730755606272));
#230753=CARTESIAN_POINT('Ctrl Pts',(46.6823308842909,-0.0301586750235619,
-239.032601429843));
#230754=CARTESIAN_POINT('Ctrl Pts',(64.6771567767455,10.4617059327352,-211.730755606272));
#230755=CARTESIAN_POINT('Ctrl Pts',(46.4942182564745,0.812212710638539,
-239.032601429843));
#230756=CARTESIAN_POINT('Ctrl Pts',(64.3397924421248,12.2751736569417,-211.730755606272));
#230757=CARTESIAN_POINT('Ctrl Pts',(46.3453291243136,1.75378837344716,-239.032601429843));
#230758=CARTESIAN_POINT('Ctrl Pts',(64.0706036090695,14.2790946061672,-211.730755606272));
#230759=CARTESIAN_POINT('Ctrl Pts',(46.3023719972086,3.1917578014948,-239.032601429843));
#230760=CARTESIAN_POINT('Ctrl Pts',(63.9692632136205,17.2974319559987,-211.730755606272));
#230761=CARTESIAN_POINT('Ctrl Pts',(46.5821989973795,6.05102323992199,-239.032601429842));
#230762=CARTESIAN_POINT('Ctrl Pts',(64.3643716897167,23.2736162661097,-211.730755606271));
#230763=CARTESIAN_POINT('Ctrl Pts',(47.566430740579,8.32255892669279,-239.032601429843));
#230764=CARTESIAN_POINT('Ctrl Pts',(65.9117879843948,28.0899407880831,-211.730755606275));
#230765=CARTESIAN_POINT('Ctrl Pts',(48.7769866795674,9.7996450480234,-239.032601429843));
#230766=CARTESIAN_POINT('Ctrl Pts',(67.8755806199084,31.5767606755659,-211.730755606259));
#230767=CARTESIAN_POINT('Origin',(-296.501483394397,-25.4138432731711,-235.35005));
#230768=CARTESIAN_POINT('Origin',(-6.29739814579425E-15,-11.5034818258363,
-234.75005));
#230769=CARTESIAN_POINT('',(42.9727564520429,17.4202489659096,-234.75005));
#230770=CARTESIAN_POINT('',(42.9727564520429,17.4202489659097,-234.75005));
#230771=CARTESIAN_POINT('',(27.3749781671338,32.4720860539414,-234.75005));
#230772=CARTESIAN_POINT('',(27.3749781671338,32.4720860539414,-234.75005));
#230773=CARTESIAN_POINT('Origin',(-6.29739814579425E-15,-11.5034818258363,
-234.75005));
#230774=CARTESIAN_POINT('Origin',(38.9907249661392,14.740057695632,-234.75005));
#230775=CARTESIAN_POINT('',(43.7871111365364,14.9262825715819,-234.75005));
#230776=CARTESIAN_POINT('',(43.7871111365364,14.9262825715819,-234.75005));
#230777=CARTESIAN_POINT('Origin',(38.9907249661392,14.740057695632,-234.75005));
#230778=CARTESIAN_POINT('Origin',(-636.934816028482,-11.5034818258361,-234.75005));
#230779=CARTESIAN_POINT('',(43.7871111365364,-37.9332462232544,-234.75005));
#230780=CARTESIAN_POINT('',(43.7871111365364,-37.9332462232544,-234.75005));
#230781=CARTESIAN_POINT('Origin',(-636.934816028482,-11.5034818258361,-234.75005));
#230782=CARTESIAN_POINT('Origin',(38.9907249661392,-37.7470213473046,-234.75005));
#230783=CARTESIAN_POINT('',(42.9727564520428,-40.4272126175822,-234.75005));
#230784=CARTESIAN_POINT('',(42.9727564520428,-40.4272126175822,-234.75005));
#230785=CARTESIAN_POINT('Origin',(38.9907249661392,-37.7470213473046,-234.75005));
#230786=CARTESIAN_POINT('Origin',(-6.29739814579425E-15,-11.5034818258363,
-234.75005));
#230787=CARTESIAN_POINT('',(25.258351173106,-56.7279850958119,-234.75005));
#230788=CARTESIAN_POINT('',(25.258351173106,-56.7279850958119,-234.75005));
#230789=CARTESIAN_POINT('Origin',(-6.29739814579425E-15,-11.5034818258363,
-234.75005));
#230790=CARTESIAN_POINT('Origin',(22.9178089794592,-52.5372975341153,-234.75005));
#230791=CARTESIAN_POINT('',(23.0804343803032,-57.3345418450714,-234.75005));
#230792=CARTESIAN_POINT('',(23.0804343803032,-57.3345418450714,-234.75005));
#230793=CARTESIAN_POINT('Origin',(22.9178089794592,-52.5372975341153,-234.75005));
#230794=CARTESIAN_POINT('Origin',(7.14692237356698E-14,623.509175991979,
-234.75005));
#230795=CARTESIAN_POINT('Origin',(7.14692237356698E-14,623.509175991979,
-234.75005));
#230796=CARTESIAN_POINT('Origin',(-2.61456814389029E-14,-173.57701443073,
-234.75005));
#230797=CARTESIAN_POINT('',(25.4241796108136,33.1612401412018,-234.75005));
#230798=CARTESIAN_POINT('Origin',(-2.61456814389029E-14,-173.57701443073,
-234.75005));
#230799=CARTESIAN_POINT('',(25.4241796108136,33.1612401412018,-234.75005));
#230800=CARTESIAN_POINT('Origin',(24.838300653577,28.3971299569735,-234.75005));
#230801=CARTESIAN_POINT('Origin',(24.838300653577,28.3971299569735,-234.75005));
#230802=CARTESIAN_POINT('Origin',(11.4589044897296,-32.0203896799758,-234.75005));
#230803=CARTESIAN_POINT('',(23.121090730514,-58.5338529228103,-234.75005));
#230804=CARTESIAN_POINT('Origin',(7.14692237356698E-14,623.509175991979,
-234.75005));
#230805=CARTESIAN_POINT('',(25.5706493501227,34.3522676872588,-234.75005));
#230806=CARTESIAN_POINT('Origin',(-2.61456814389029E-14,-173.57701443073,
-234.75005));
#230807=CARTESIAN_POINT('',(28.0091475455229,33.4908250781833,-234.75005));
#230808=CARTESIAN_POINT('Origin',(24.838300653577,28.3971299569735,-234.75005));
#230809=CARTESIAN_POINT('',(43.9682643235187,18.0902967834791,-234.75005));
#230810=CARTESIAN_POINT('Origin',(-6.29739814579425E-15,-11.5034818258363,
-234.75005));
#230811=CARTESIAN_POINT('',(44.9862076791357,14.9728387905693,-234.75005));
#230812=CARTESIAN_POINT('Origin',(38.9907249661392,14.740057695632,-234.75005));
#230813=CARTESIAN_POINT('',(44.9862076791357,-37.9798024422418,-234.75005));
#230814=CARTESIAN_POINT('Origin',(-636.934816028482,-11.5034818258361,-234.75005));
#230815=CARTESIAN_POINT('',(43.9682643235187,-41.0972604351516,-234.75005));
#230816=CARTESIAN_POINT('Origin',(38.9907249661392,-37.7470213473046,-234.75005));
#230817=CARTESIAN_POINT('',(25.8434867215177,-57.775656986236,-234.75005));
#230818=CARTESIAN_POINT('Origin',(-6.29739814579425E-15,-11.5034818258363,
-234.75005));
#230819=CARTESIAN_POINT('Origin',(22.9178089794592,-52.5372975341153,-234.75005));
#230820=CARTESIAN_POINT('Origin',(22.9178089794592,-52.5372975341153,-234.75005));
#230821=CARTESIAN_POINT('',(25.8434867215177,-57.775656986236,-234.75005));
#230822=CARTESIAN_POINT('',(23.121090730514,-58.5338529228103,-234.75005));
#230823=CARTESIAN_POINT('Origin',(7.14692237356698E-14,623.509175991979,
-234.75005));
#230824=CARTESIAN_POINT('Origin',(-2.61456814389029E-14,-173.57701443073,
-234.75005));
#230825=CARTESIAN_POINT('',(25.5706493501227,34.3522676872588,-234.75005));
#230826=CARTESIAN_POINT('Origin',(24.838300653577,28.3971299569735,-234.75005));
#230827=CARTESIAN_POINT('',(28.0091475455229,33.4908250781833,-234.75005));
#230828=CARTESIAN_POINT('Origin',(-6.29739814579425E-15,-11.5034818258363,
-234.75005));
#230829=CARTESIAN_POINT('',(43.9682643235187,18.0902967834791,-234.75005));
#230830=CARTESIAN_POINT('Origin',(38.9907249661392,14.740057695632,-234.75005));
#230831=CARTESIAN_POINT('',(44.9862076791357,14.9728387905693,-234.75005));
#230832=CARTESIAN_POINT('Origin',(-636.934816028482,-11.5034818258361,-234.75005));
#230833=CARTESIAN_POINT('',(44.9862076791357,-37.9798024422418,-234.75005));
#230834=CARTESIAN_POINT('Origin',(38.9907249661392,-37.7470213473046,-234.75005));
#230835=CARTESIAN_POINT('',(43.9682643235187,-41.0972604351516,-234.75005));
#230836=CARTESIAN_POINT('Origin',(-6.29739814579425E-15,-11.5034818258363,
-234.75005));
#230837=CARTESIAN_POINT('Ctrl Pts',(48.1560655127274,-41.999274229607,-235.35005));
#230838=CARTESIAN_POINT('Ctrl Pts',(51.9279919200935,-48.6191351285365,
-228.68335));
#230839=CARTESIAN_POINT('Ctrl Pts',(55.7004001286368,-55.2387363218615,
-222.01665));
#230840=CARTESIAN_POINT('Ctrl Pts',(59.4732891526772,-61.8580772083615,
-215.34995));
#230841=CARTESIAN_POINT('Ctrl Pts',(59.5110180429176,-61.9242706172265,
-215.283283));
#230842=CARTESIAN_POINT('Ctrl Pts',(59.548746933158,-61.9904640260915,-215.216616));
#230843=CARTESIAN_POINT('Ctrl Pts',(59.5864758233984,-62.0566574349565,
-215.149949));
#230844=CARTESIAN_POINT('Ctrl Pts',(48.2756382252007,-41.8104563330539,
-235.35005));
#230845=CARTESIAN_POINT('Ctrl Pts',(52.0407670149459,-48.4530353242655,
-228.68335));
#230846=CARTESIAN_POINT('Ctrl Pts',(55.8063647406712,-55.0953754160451,
-222.01665));
#230847=CARTESIAN_POINT('Ctrl Pts',(59.57243049321,-61.7374760219621,-215.34995));
#230848=CARTESIAN_POINT('Ctrl Pts',(59.6100911507354,-61.8038970280213,
-215.283283));
#230849=CARTESIAN_POINT('Ctrl Pts',(59.6477518082608,-61.8703180340805,
-215.216616));
#230850=CARTESIAN_POINT('Ctrl Pts',(59.6854124657861,-61.9367390401396,
-215.149949));
#230851=CARTESIAN_POINT('Ctrl Pts',(48.3910626922776,-41.5900298422911,
-235.35005));
#230852=CARTESIAN_POINT('Ctrl Pts',(52.1903238662186,-48.2138133273298,
-228.68335));
#230853=CARTESIAN_POINT('Ctrl Pts',(55.9900266043744,-54.8373975226491,
-222.01665));
#230854=CARTESIAN_POINT('Ctrl Pts',(59.790170143516,-61.4607818737039,-215.34995));
#230855=CARTESIAN_POINT('Ctrl Pts',(59.8281715789074,-61.5270157172145,
-215.283283));
#230856=CARTESIAN_POINT('Ctrl Pts',(59.8661730142988,-61.593249560725,-215.216616));
#230857=CARTESIAN_POINT('Ctrl Pts',(59.9041744496902,-61.6594834042356,
-215.149949));
#230858=CARTESIAN_POINT('Ctrl Pts',(48.5387172079886,-41.2798109487642,
-235.35005));
#230859=CARTESIAN_POINT('Ctrl Pts',(52.4230972161915,-47.8204177760876,
-228.68335));
#230860=CARTESIAN_POINT('Ctrl Pts',(56.3078726256209,-54.3608781649969,
-222.01665));
#230861=CARTESIAN_POINT('Ctrl Pts',(60.1930428686919,-60.9011916159786,
-215.34995));
#230862=CARTESIAN_POINT('Ctrl Pts',(60.2318945711226,-60.9665947504884,
-215.283283000001));
#230863=CARTESIAN_POINT('Ctrl Pts',(60.2707462735533,-61.0319978849983,
-215.216616));
#230864=CARTESIAN_POINT('Ctrl Pts',(60.309597975984,-61.0974010195081,-215.149949));
#230865=CARTESIAN_POINT('Ctrl Pts',(48.6371642419829,-41.0193984169334,
-235.35005));
#230866=CARTESIAN_POINT('Ctrl Pts',(52.6688606290506,-47.3486283864447,
-228.68335));
#230867=CARTESIAN_POINT('Ctrl Pts',(56.7009009677878,-53.6777576502171,
-222.01665));
#230868=CARTESIAN_POINT('Ctrl Pts',(60.7332848610003,-60.0067857712577,
-215.34995));
#230869=CARTESIAN_POINT('Ctrl Pts',(60.7736086999325,-60.0700760524681,
-215.283283));
#230870=CARTESIAN_POINT('Ctrl Pts',(60.8139325388646,-60.1333663336785,
-215.216616));
#230871=CARTESIAN_POINT('Ctrl Pts',(60.8542563777967,-60.1966566148889,
-215.149949));
#230872=CARTESIAN_POINT('Ctrl Pts',(48.7259447515556,-40.7557132274099,
-235.35005));
#230873=CARTESIAN_POINT('Ctrl Pts',(52.8863489207853,-46.8366038296761,
-228.68335));
#230874=CARTESIAN_POINT('Ctrl Pts',(57.0470401243311,-52.9174317848832,
-222.016650000001));
#230875=CARTESIAN_POINT('Ctrl Pts',(61.2080181081436,-58.9981967263321,
-215.349950000001));
#230876=CARTESIAN_POINT('Ctrl Pts',(61.2496278879817,-59.0590043757466,
-215.283283000001));
#230877=CARTESIAN_POINT('Ctrl Pts',(61.2912376678198,-59.1198120251611,
-215.216616));
#230878=CARTESIAN_POINT('Ctrl Pts',(61.332847447658,-59.1806196745756,-215.149949000001));
#230879=CARTESIAN_POINT('Ctrl Pts',(48.7945150938174,-40.4960542325497,
-235.35005));
#230880=CARTESIAN_POINT('Ctrl Pts',(53.0535779259056,-46.3256171279293,
-228.68335));
#230881=CARTESIAN_POINT('Ctrl Pts',(57.3128652259323,-52.1551472055685,
-222.01665));
#230882=CARTESIAN_POINT('Ctrl Pts',(61.572376853754,-57.9846441771198,-215.34995));
#230883=CARTESIAN_POINT('Ctrl Pts',(61.6149719700322,-58.0429391468354,
-215.283283));
#230884=CARTESIAN_POINT('Ctrl Pts',(61.6575670863105,-58.1012341165509,
-215.216616));
#230885=CARTESIAN_POINT('Ctrl Pts',(61.7001622025887,-58.1595290862664,
-215.149949));
#230886=CARTESIAN_POINT('Ctrl Pts',(48.8537891615446,-40.2227290210882,
-235.35005));
#230887=CARTESIAN_POINT('Ctrl Pts',(53.184407479365,-45.7839380160283,-228.68335));
#230888=CARTESIAN_POINT('Ctrl Pts',(57.5151818684938,-51.3451352378197,
-222.01665));
#230889=CARTESIAN_POINT('Ctrl Pts',(61.8461122714633,-56.9063204848096,
-215.349950000001));
#230890=CARTESIAN_POINT('Ctrl Pts',(61.889421575493,-56.9619323372794,-215.283283000001));
#230891=CARTESIAN_POINT('Ctrl Pts',(61.9327308795227,-57.0175441897493,
-215.216616));
#230892=CARTESIAN_POINT('Ctrl Pts',(61.9760401835524,-57.0731560422192,
-215.149949000001));
#230893=CARTESIAN_POINT('Ctrl Pts',(48.8993219763807,-39.9191637201113,
-235.35005));
#230894=CARTESIAN_POINT('Ctrl Pts',(53.2653672535676,-45.2450247261708,
-228.68335));
#230895=CARTESIAN_POINT('Ctrl Pts',(57.631494193953,-50.5708856635808,-222.01665));
#230896=CARTESIAN_POINT('Ctrl Pts',(61.9977027895214,-55.8967464260103,
-215.34995));
#230897=CARTESIAN_POINT('Ctrl Pts',(62.0413648754771,-55.9500050336346,
-215.283283));
#230898=CARTESIAN_POINT('Ctrl Pts',(62.0850269614327,-56.0032636412589,
-215.216616));
#230899=CARTESIAN_POINT('Ctrl Pts',(62.1286890473884,-56.0565222488832,
-215.149949));
#230900=CARTESIAN_POINT('Ctrl Pts',(48.9214109907111,-39.6817730556917,
-235.35005));
#230901=CARTESIAN_POINT('Ctrl Pts',(53.2924626390134,-44.9053881830262,
-228.68335));
#230902=CARTESIAN_POINT('Ctrl Pts',(57.6635282520289,-50.1290038777392,
-222.01665));
#230903=CARTESIAN_POINT('Ctrl Pts',(62.0346078304961,-55.3526201213579,
-215.34995));
#230904=CARTESIAN_POINT('Ctrl Pts',(62.0783186262807,-55.4048562837941,
-215.283283));
#230905=CARTESIAN_POINT('Ctrl Pts',(62.1220294220654,-55.4570924462303,
-215.216616));
#230906=CARTESIAN_POINT('Ctrl Pts',(62.1657402178501,-55.5093286086665,
-215.149949));
#230907=CARTESIAN_POINT('Ctrl Pts',(48.9276804568491,-39.5283381317121,
-235.35005));
#230908=CARTESIAN_POINT('Ctrl Pts',(53.2999213760692,-44.7204933330714,
-228.68335));
#230909=CARTESIAN_POINT('Ctrl Pts',(57.6721622952894,-49.9126485344307,
-222.01665));
#230910=CARTESIAN_POINT('Ctrl Pts',(62.0444032145095,-55.1048037357899,
-215.34995));
#230911=CARTESIAN_POINT('Ctrl Pts',(62.0881256237017,-55.1567252878035,
-215.283283));
#230912=CARTESIAN_POINT('Ctrl Pts',(62.1318480328939,-55.2086468398171,
-215.216616));
#230913=CARTESIAN_POINT('Ctrl Pts',(62.1755704420861,-55.2605683918307,
-215.149949));
#230914=CARTESIAN_POINT('Ctrl Pts',(48.4015825627194,-42.4301635567086,
-234.916111528175));
#230915=CARTESIAN_POINT('Ctrl Pts',(51.8161020106309,-48.4227195017014,
-228.881144730288));
#230916=CARTESIAN_POINT('Ctrl Pts',(55.2310162579792,-54.4150626175587,
-222.846177932402));
#230917=CARTESIAN_POINT('Ctrl Pts',(58.6463245735781,-60.4071924582901,
-216.811211134516));
#230918=CARTESIAN_POINT('',(55.4860418356793,-47.316570933751,-225.35));
#230919=CARTESIAN_POINT('Ctrl Pts',(24.4127870505286,-62.4913878448826,
-235.35005));
#230920=CARTESIAN_POINT('Ctrl Pts',(30.252655437952,-66.705065059021,-228.68335));
#230921=CARTESIAN_POINT('Ctrl Pts',(36.0925246020991,-70.9187639624533,
-222.01665));
#230922=CARTESIAN_POINT('Ctrl Pts',(41.9323946221365,-75.1324845521997,
-215.34995));
#230923=CARTESIAN_POINT('Ctrl Pts',(41.990793322337,-75.1746217580972,-215.283283));
#230924=CARTESIAN_POINT('Ctrl Pts',(42.0491920225373,-75.2167589639946,
-215.216616));
#230925=CARTESIAN_POINT('Ctrl Pts',(42.1075907227377,-75.2588961698921,
-215.149949));
#230926=CARTESIAN_POINT('Ctrl Pts',(24.4238355020022,-62.4909941277675,
-235.35005));
#230927=CARTESIAN_POINT('Ctrl Pts',(30.2665958673131,-66.7045508406744,
-228.68335));
#230928=CARTESIAN_POINT('Ctrl Pts',(36.1093567495128,-70.9181220131437,
-222.01665));
#230929=CARTESIAN_POINT('Ctrl Pts',(41.9521182016317,-75.1317076431822,
-215.34995));
#230930=CARTESIAN_POINT('Ctrl Pts',(42.0105458161529,-75.1738434994826,
-215.283283));
#230931=CARTESIAN_POINT('Ctrl Pts',(42.0689734306741,-75.215979355783,-215.216616));
#230932=CARTESIAN_POINT('Ctrl Pts',(42.1274010451954,-75.2581152120834,
-215.149949));
#230933=CARTESIAN_POINT('Ctrl Pts',(24.4348839534758,-62.4906004106524,
-235.35005));
#230934=CARTESIAN_POINT('Ctrl Pts',(30.2805362966741,-66.7040366223279,
-228.68335));
#230935=CARTESIAN_POINT('Ctrl Pts',(36.1261888969267,-70.9174800638341,
-222.01665));
#230936=CARTESIAN_POINT('Ctrl Pts',(41.971841781127,-75.1309307341648,-215.34995));
#230937=CARTESIAN_POINT('Ctrl Pts',(42.030298309969,-75.1730652408681,-215.283283));
#230938=CARTESIAN_POINT('Ctrl Pts',(42.088754838811,-75.2151997475714,-215.216616));
#230939=CARTESIAN_POINT('Ctrl Pts',(42.147211367653,-75.2573342542747,-215.149949));
#230940=CARTESIAN_POINT('Ctrl Pts',(24.4459324049493,-62.4902066935372,
-235.35005));
#230941=CARTESIAN_POINT('Ctrl Pts',(30.2944767260352,-66.7035224039813,
-228.68335));
#230942=CARTESIAN_POINT('Ctrl Pts',(36.1430210443405,-70.9168381145244,
-222.01665));
#230943=CARTESIAN_POINT('Ctrl Pts',(41.9915653606222,-75.1301538251473,
-215.34995));
#230944=CARTESIAN_POINT('Ctrl Pts',(42.050050803785,-75.1722869822535,-215.283283));
#230945=CARTESIAN_POINT('Ctrl Pts',(42.1085362469478,-75.2144201393598,
-215.216616));
#230946=CARTESIAN_POINT('Ctrl Pts',(42.1670216901106,-75.256553296466,-215.149949));
#230947=CARTESIAN_POINT('Ctrl Pts',(24.5840380483692,-62.4852852295981,
-235.35005));
#230948=CARTESIAN_POINT('Ctrl Pts',(30.4687320930486,-66.6970946746494,
-228.68335));
#230949=CARTESIAN_POINT('Ctrl Pts',(36.3534228870133,-70.9088137481542,
-222.01665));
#230950=CARTESIAN_POINT('Ctrl Pts',(42.2381101043121,-75.120442462429,-215.34995));
#230951=CARTESIAN_POINT('Ctrl Pts',(42.2969569764852,-75.1625587495718,
-215.283283));
#230952=CARTESIAN_POINT('Ctrl Pts',(42.3558038486582,-75.2046750367146,
-215.216616));
#230953=CARTESIAN_POINT('Ctrl Pts',(42.4146507208312,-75.2467913238573,
-215.149949));
#230954=CARTESIAN_POINT('Ctrl Pts',(24.7878826649652,-62.4682791689329,
-235.35005));
#230955=CARTESIAN_POINT('Ctrl Pts',(30.7858798041607,-66.6737307701245,
-228.68335));
#230956=CARTESIAN_POINT('Ctrl Pts',(36.7838683264116,-70.8789174633912,
-222.01665));
#230957=CARTESIAN_POINT('Ctrl Pts',(42.781847274702,-75.0838392837,-215.34995));
#230958=CARTESIAN_POINT('Ctrl Pts',(42.8418270641849,-75.1258885019031,
-215.283283));
#230959=CARTESIAN_POINT('Ctrl Pts',(42.9018068536678,-75.1679377201062,
-215.216616));
#230960=CARTESIAN_POINT('Ctrl Pts',(42.9617866431507,-75.2099869383093,
-215.149949));
#230961=CARTESIAN_POINT('Ctrl Pts',(25.048207175495,-62.4347017437458,-235.35005));
#230962=CARTESIAN_POINT('Ctrl Pts',(31.2985071141138,-66.6007006042259,
-228.68335));
#230963=CARTESIAN_POINT('Ctrl Pts',(37.5487936188611,-70.7661908933779,
-222.01665));
#230964=CARTESIAN_POINT('Ctrl Pts',(43.7990648514606,-74.9311726743249,
-215.34995));
#230965=CARTESIAN_POINT('Ctrl Pts',(43.8615675637866,-74.9728224921344,
-215.283283));
#230966=CARTESIAN_POINT('Ctrl Pts',(43.9240702761126,-75.0144723099439,
-215.216616));
#230967=CARTESIAN_POINT('Ctrl Pts',(43.9865729884385,-75.0561221277533,
-215.149949));
#230968=CARTESIAN_POINT('Ctrl Pts',(25.2812199560259,-62.390732268219,-235.35005));
#230969=CARTESIAN_POINT('Ctrl Pts',(31.8143029221326,-66.4798048243852,
-228.68335));
#230970=CARTESIAN_POINT('Ctrl Pts',(38.3473707133638,-70.5681428074098,
-222.01665));
#230971=CARTESIAN_POINT('Ctrl Pts',(44.8804206737979,-74.6557463029982,
-215.34995));
#230972=CARTESIAN_POINT('Ctrl Pts',(44.9457511734022,-74.6966223379541,
-215.283283));
#230973=CARTESIAN_POINT('Ctrl Pts',(45.0110816730065,-74.73749837291,-215.216616));
#230974=CARTESIAN_POINT('Ctrl Pts',(45.0764121726109,-74.7783744078659,
-215.149949));
#230975=CARTESIAN_POINT('Ctrl Pts',(25.5015868365187,-62.3415392578964,
-235.35005));
#230976=CARTESIAN_POINT('Ctrl Pts',(32.299209143815,-66.325492796133,-228.68335));
#230977=CARTESIAN_POINT('Ctrl Pts',(39.0968174546589,-70.3085029414293,
-222.01665));
#230978=CARTESIAN_POINT('Ctrl Pts',(45.8944083573785,-74.2905697967455,
-215.34995));
#230979=CARTESIAN_POINT('Ctrl Pts',(45.9623842664057,-74.3303904652987,
-215.283283));
#230980=CARTESIAN_POINT('Ctrl Pts',(46.0303601754329,-74.3702111338518,
-215.216616));
#230981=CARTESIAN_POINT('Ctrl Pts',(46.0983360844601,-74.410031802405,-215.149949));
#230982=CARTESIAN_POINT('Ctrl Pts',(25.7300777644121,-62.275287851211,-235.35005));
#230983=CARTESIAN_POINT('Ctrl Pts',(32.7889564583827,-66.1223030781061,
-228.68335));
#230984=CARTESIAN_POINT('Ctrl Pts',(39.8478250972557,-69.9681827947029,
-222.01665));
#230985=CARTESIAN_POINT('Ctrl Pts',(46.906679573783,-73.8129271161338,-215.34995));
#230986=CARTESIAN_POINT('Ctrl Pts',(46.9772681185483,-73.8513745593482,
-215.283283));
#230987=CARTESIAN_POINT('Ctrl Pts',(47.0478566633135,-73.8898220025625,
-215.216616));
#230988=CARTESIAN_POINT('Ctrl Pts',(47.1184452080788,-73.9282694457768,
-215.149949));
#230989=CARTESIAN_POINT('Ctrl Pts',(25.9496411726737,-62.2064433802863,
-235.35005));
#230990=CARTESIAN_POINT('Ctrl Pts',(33.2328325215974,-65.8962682476017,
-228.68335));
#230991=CARTESIAN_POINT('Ctrl Pts',(40.5160203632138,-69.5847817101261,
-222.01665));
#230992=CARTESIAN_POINT('Ctrl Pts',(47.7991999531534,-73.2719838903286,
-215.34995));
#230993=CARTESIAN_POINT('Ctrl Pts',(47.8720317490528,-73.3088559121307,
-215.283283));
#230994=CARTESIAN_POINT('Ctrl Pts',(47.9448635449522,-73.3457279339327,
-215.216616));
#230995=CARTESIAN_POINT('Ctrl Pts',(48.0176953408516,-73.3825999557347,
-215.149949));
#230996=CARTESIAN_POINT('Ctrl Pts',(26.2296171960789,-62.0929811520229,
-235.35005));
#230997=CARTESIAN_POINT('Ctrl Pts',(33.5992240749579,-65.6911775370676,
-228.68335));
#230998=CARTESIAN_POINT('Ctrl Pts',(40.9688364442604,-69.2879023661194,
-222.01665));
#230999=CARTESIAN_POINT('Ctrl Pts',(48.3384489792287,-72.8831557643943,
-215.34995));
#231000=CARTESIAN_POINT('Ctrl Pts',(48.4121451045784,-72.919108298377,-215.283283));
#231001=CARTESIAN_POINT('Ctrl Pts',(48.485841229928,-72.9550608323598,-215.216616));
#231002=CARTESIAN_POINT('Ctrl Pts',(48.5595373552777,-72.9910133663425,
-215.149949));
#231003=CARTESIAN_POINT('Ctrl Pts',(26.4137508499222,-62.0144582859218,
-235.35005));
#231004=CARTESIAN_POINT('Ctrl Pts',(33.8110251833904,-65.5692400768433,
-228.68335));
#231005=CARTESIAN_POINT('Ctrl Pts',(41.2083125347321,-69.1224537201152,
-222.01665));
#231006=CARTESIAN_POINT('Ctrl Pts',(48.6056072289401,-72.6740993398878,
-215.34995));
#231007=CARTESIAN_POINT('Ctrl Pts',(48.6795801758822,-72.7096157960855,
-215.283283));
#231008=CARTESIAN_POINT('Ctrl Pts',(48.7535531228243,-72.7451322522832,
-215.216616));
#231009=CARTESIAN_POINT('Ctrl Pts',(48.8275260697664,-72.780648708481,-215.149949));
#231010=CARTESIAN_POINT('Ctrl Pts',(26.60131676328,-61.915483833886,-235.35005));
#231011=CARTESIAN_POINT('Ctrl Pts',(33.9746898504281,-65.4717344596898,
-228.68335));
#231012=CARTESIAN_POINT('Ctrl Pts',(41.3480800753329,-69.0263711060389,
-222.01665));
#231013=CARTESIAN_POINT('Ctrl Pts',(48.7214815967444,-72.5793938958684,
-215.34995));
#231014=CARTESIAN_POINT('Ctrl Pts',(48.7952156119585,-72.6149241237667,
-215.283283));
#231015=CARTESIAN_POINT('Ctrl Pts',(48.8689496271726,-72.6504543516649,
-215.216616));
#231016=CARTESIAN_POINT('Ctrl Pts',(48.9426836423867,-72.6859845795632,
-215.149949));
#231017=CARTESIAN_POINT('',(33.2187488845874,-68.8101802592752,-225.35));
#231018=CARTESIAN_POINT('Ctrl Pts',(27.0930165135311,-62.1526330725429,
-234.905475377596));
#231019=CARTESIAN_POINT('Ctrl Pts',(33.75885046978,-65.3675653924474,-228.878503713969));
#231020=CARTESIAN_POINT('Ctrl Pts',(40.424698326436,-68.5811786244384,-222.851532050343));
#231021=CARTESIAN_POINT('Ctrl Pts',(47.0905557676078,-71.7934728593479,
-216.824560386716));
#231022=CARTESIAN_POINT('Ctrl Pts',(29.0709882823152,37.525873057636,-235.35005));
#231023=CARTESIAN_POINT('Ctrl Pts',(35.5332604733831,40.6579014073498,-228.683350000001));
#231024=CARTESIAN_POINT('Ctrl Pts',(41.9930962102693,43.771133049519,-222.01665));
#231025=CARTESIAN_POINT('Ctrl Pts',(48.4493862544499,46.8657485296993,-215.34995));
#231026=CARTESIAN_POINT('Ctrl Pts',(48.5139491548917,46.8966946845011,-215.283283));
#231027=CARTESIAN_POINT('Ctrl Pts',(48.5785120553335,46.9276408393029,-215.216616));
#231028=CARTESIAN_POINT('Ctrl Pts',(48.6430749557753,46.9585869941047,-215.149949));
#231029=CARTESIAN_POINT('Ctrl Pts',(28.9262831839988,37.6116730896339,-235.35005));
#231030=CARTESIAN_POINT('Ctrl Pts',(35.404815368487,40.7403542996618,-228.683350000001));
#231031=CARTESIAN_POINT('Ctrl Pts',(41.8809828830328,43.8508119821702,-222.01665));
#231032=CARTESIAN_POINT('Ctrl Pts',(48.3537103198215,46.9432211795102,-215.34995));
#231033=CARTESIAN_POINT('Ctrl Pts',(48.4184375941894,46.9741452714836,-215.283283));
#231034=CARTESIAN_POINT('Ctrl Pts',(48.4831648685572,47.005069363457,-215.216616));
#231035=CARTESIAN_POINT('Ctrl Pts',(48.5478921429251,47.0359934554304,-215.149949));
#231036=CARTESIAN_POINT('Ctrl Pts',(28.7510590357854,37.7017381212741,-235.35005));
#231037=CARTESIAN_POINT('Ctrl Pts',(35.2153249135404,40.8559840579253,-228.683350000001));
#231038=CARTESIAN_POINT('Ctrl Pts',(41.67737658309,43.9932018113665,-222.01665));
#231039=CARTESIAN_POINT('Ctrl Pts',(48.1362091874323,47.1135549465408,-215.34995));
#231040=CARTESIAN_POINT('Ctrl Pts',(48.2007975134757,47.1447584778926,-215.283283));
#231041=CARTESIAN_POINT('Ctrl Pts',(48.2653858395191,47.1759620092443,-215.216616));
#231042=CARTESIAN_POINT('Ctrl Pts',(48.3299741655626,47.207165540596,-215.149949));
#231043=CARTESIAN_POINT('Ctrl Pts',(28.5095079111441,37.8154098604791,-235.350050000001));
#231044=CARTESIAN_POINT('Ctrl Pts',(34.9092271504532,41.0352703241457,-228.683350000001));
#231045=CARTESIAN_POINT('Ctrl Pts',(41.3069791618872,44.2400465335893,-222.016650000001));
#231046=CARTESIAN_POINT('Ctrl Pts',(47.7018738162952,47.429883386524,-215.34995));
#231047=CARTESIAN_POINT('Ctrl Pts',(47.7658227628392,47.4617817550534,-215.283283));
#231048=CARTESIAN_POINT('Ctrl Pts',(47.8297717093833,47.4936801235827,-215.216616));
#231049=CARTESIAN_POINT('Ctrl Pts',(47.8937206559274,47.525578492112,-215.149949));
#231050=CARTESIAN_POINT('Ctrl Pts',(28.3066649003232,37.8966208237621,-235.35005));
#231051=CARTESIAN_POINT('Ctrl Pts',(34.5530956045189,41.2282169831045,-228.68335));
#231052=CARTESIAN_POINT('Ctrl Pts',(40.7978279568429,44.5468276894782,-222.01665));
#231053=CARTESIAN_POINT('Ctrl Pts',(47.0400956910773,47.8525776841313,-215.34995));
#231054=CARTESIAN_POINT('Ctrl Pts',(47.1025183684196,47.8856351840778,-215.283283));
#231055=CARTESIAN_POINT('Ctrl Pts',(47.1649410457619,47.9186926840244,-215.216616));
#231056=CARTESIAN_POINT('Ctrl Pts',(47.2273637231043,47.9517501839709,-215.149949));
#231057=CARTESIAN_POINT('Ctrl Pts',(28.0997724400839,37.970731452037,-235.35005));
#231058=CARTESIAN_POINT('Ctrl Pts',(34.1684829306694,41.4070992755122,-228.683350000001));
#231059=CARTESIAN_POINT('Ctrl Pts',(40.2357864490083,44.8327392792855,-222.01665));
#231060=CARTESIAN_POINT('Ctrl Pts',(46.3010499603476,48.2477545207809,-215.34995));
#231061=CARTESIAN_POINT('Ctrl Pts',(46.361702595461,48.2819046731959,-215.283283));
#231062=CARTESIAN_POINT('Ctrl Pts',(46.4223552305744,48.3160548256108,-215.216616));
#231063=CARTESIAN_POINT('Ctrl Pts',(46.4830078656878,48.3502049780258,-215.149949));
#231064=CARTESIAN_POINT('Ctrl Pts',(27.9025329741163,38.0324522529201,-235.35005));
#231065=CARTESIAN_POINT('Ctrl Pts',(33.7896008939784,41.5559827385479,-228.683350000001));
#231066=CARTESIAN_POINT('Ctrl Pts',(39.6755763327887,45.0712058294971,-222.01665));
#231067=CARTESIAN_POINT('Ctrl Pts',(45.5599690892415,48.5782013338904,-215.349950000001));
#231068=CARTESIAN_POINT('Ctrl Pts',(45.618813016806,48.6132712889344,-215.283283000001));
#231069=CARTESIAN_POINT('Ctrl Pts',(45.6776569443706,48.6483412439783,-215.216616));
#231070=CARTESIAN_POINT('Ctrl Pts',(45.7365008719351,48.6834111990222,-215.149949000001));
#231071=CARTESIAN_POINT('Ctrl Pts',(27.6836295517497,38.0888474954169,-235.35005));
#231072=CARTESIAN_POINT('Ctrl Pts',(33.3812146101381,41.6857034969331,-228.68335));
#231073=CARTESIAN_POINT('Ctrl Pts',(39.0780453981879,45.2768392802963,-222.01665));
#231074=CARTESIAN_POINT('Ctrl Pts',(44.773784383473,48.8623098007285,-215.34995));
#231075=CARTESIAN_POINT('Ctrl Pts',(44.8307417733259,48.8981645059328,-215.283283));
#231076=CARTESIAN_POINT('Ctrl Pts',(44.8876991631787,48.9340192111371,-215.216616));
#231077=CARTESIAN_POINT('Ctrl Pts',(44.9446565530316,48.9698739163414,-215.149949));
#231078=CARTESIAN_POINT('Ctrl Pts',(27.4619512217085,38.1391172889764,-235.35005));
#231079=CARTESIAN_POINT('Ctrl Pts',(32.9867338744792,41.7852023290646,-228.683350000001));
#231080=CARTESIAN_POINT('Ctrl Pts',(38.511124795091,45.4283250387717,-222.016650000001));
#231081=CARTESIAN_POINT('Ctrl Pts',(44.0349491888799,49.0685138787004,-215.349950000001));
#231082=CARTESIAN_POINT('Ctrl Pts',(44.0901874328179,49.1049157670997,-215.283283000001));
#231083=CARTESIAN_POINT('Ctrl Pts',(44.1454256767557,49.141317655499,-215.216616));
#231084=CARTESIAN_POINT('Ctrl Pts',(44.2006639206936,49.1777195438983,-215.149949000001));
#231085=CARTESIAN_POINT('Ctrl Pts',(27.272251770635,38.1696450547512,-235.35005));
#231086=CARTESIAN_POINT('Ctrl Pts',(32.7234828694691,41.832799228952,-228.68335));
#231087=CARTESIAN_POINT('Ctrl Pts',(38.1745805518739,45.4949461119472,-222.01665));
#231088=CARTESIAN_POINT('Ctrl Pts',(43.625485383249,49.1560953813671,-215.34995));
#231089=CARTESIAN_POINT('Ctrl Pts',(43.6799944315629,49.1927068740612,-215.283283));
#231090=CARTESIAN_POINT('Ctrl Pts',(43.7345034798766,49.2293183667554,-215.216616));
#231091=CARTESIAN_POINT('Ctrl Pts',(43.7890125281904,49.2659298594496,-215.149949));
#231092=CARTESIAN_POINT('Ctrl Pts',(27.1569075795172,38.1844371310006,-235.35005));
#231093=CARTESIAN_POINT('Ctrl Pts',(32.5837764342019,41.8536056393876,-228.68335));
#231094=CARTESIAN_POINT('Ctrl Pts',(38.0106452875494,45.5227741479461,-222.01665));
#231095=CARTESIAN_POINT('Ctrl Pts',(43.4375141409548,49.1919426564936,-215.34995));
#231096=CARTESIAN_POINT('Ctrl Pts',(43.4917828294889,49.2286343415791,-215.283283));
#231097=CARTESIAN_POINT('Ctrl Pts',(43.5460515180229,49.2653260266646,-215.216616));
#231098=CARTESIAN_POINT('Ctrl Pts',(43.600320206557,49.30201771175,-215.149949));
#231099=CARTESIAN_POINT('Ctrl Pts',(29.5524353619882,37.7591803693089,-234.853368133768));
#231100=CARTESIAN_POINT('Ctrl Pts',(35.3897707041939,40.5875346064766,-228.831260854445));
#231101=CARTESIAN_POINT('Ctrl Pts',(41.225095491082,43.4005549188572,-222.809153575121));
#231102=CARTESIAN_POINT('Ctrl Pts',(47.0575921287078,46.1983743823903,-216.787046295788));
#231103=CARTESIAN_POINT('',(35.2972108607157,43.6881898936869,-225.35));
#231104=CARTESIAN_POINT('Ctrl Pts',(48.9291851287222,16.4845500982845,-235.35005));
#231105=CARTESIAN_POINT('Ctrl Pts',(53.3017114728827,20.6931427899333,-228.68335));
#231106=CARTESIAN_POINT('Ctrl Pts',(57.6742344655836,24.9017353436595,-222.01665));
#231107=CARTESIAN_POINT('Ctrl Pts',(62.0467541066728,29.1103277631972,-215.34995));
#231108=CARTESIAN_POINT('Ctrl Pts',(62.0904793030837,29.1524136873926,-215.283283));
#231109=CARTESIAN_POINT('Ctrl Pts',(62.1342044994946,29.194499611588,-215.216616));
#231110=CARTESIAN_POINT('Ctrl Pts',(62.1779296959055,29.2365855357833,-215.149949));
#231111=CARTESIAN_POINT('Ctrl Pts',(48.9286835714312,16.4968248922029,-235.35005));
#231112=CARTESIAN_POINT('Ctrl Pts',(53.3011147739234,20.7079343778016,-228.68335));
#231113=CARTESIAN_POINT('Ctrl Pts',(57.6735437421284,24.9190437709811,-222.01665));
#231114=CARTESIAN_POINT('Ctrl Pts',(62.0459704759518,29.1301530740427,-215.34995));
#231115=CARTESIAN_POINT('Ctrl Pts',(62.08969474329,29.1722641670733,-215.283283));
#231116=CARTESIAN_POINT('Ctrl Pts',(62.1334190106282,29.2143752601038,-215.216616));
#231117=CARTESIAN_POINT('Ctrl Pts',(62.1771432779665,29.2564863531345,-215.149949));
#231118=CARTESIAN_POINT('Ctrl Pts',(48.9281820141402,16.5090996861212,-235.35005));
#231119=CARTESIAN_POINT('Ctrl Pts',(53.3005180749641,20.72272596567,-228.68335));
#231120=CARTESIAN_POINT('Ctrl Pts',(57.6728530186733,24.9363521983027,-222.01665));
#231121=CARTESIAN_POINT('Ctrl Pts',(62.0451868452307,29.1499783848881,-215.34995));
#231122=CARTESIAN_POINT('Ctrl Pts',(62.0889101834963,29.1921146467539,-215.283283));
#231123=CARTESIAN_POINT('Ctrl Pts',(62.1326335217618,29.2342509086198,-215.216616));
#231124=CARTESIAN_POINT('Ctrl Pts',(62.1763568600274,29.2763871704856,-215.149949));
#231125=CARTESIAN_POINT('Ctrl Pts',(48.9276804568491,16.5213744800396,-235.35005));
#231126=CARTESIAN_POINT('Ctrl Pts',(53.2999213760048,20.7375175535383,-228.68335));
#231127=CARTESIAN_POINT('Ctrl Pts',(57.6721622952182,24.9536606256242,-222.01665));
#231128=CARTESIAN_POINT('Ctrl Pts',(62.0444032145096,29.1698036957335,-215.34995));
#231129=CARTESIAN_POINT('Ctrl Pts',(62.0881256237025,29.2119651264346,-215.283283));
#231130=CARTESIAN_POINT('Ctrl Pts',(62.1318480328954,29.2541265571357,-215.216616));
#231131=CARTESIAN_POINT('Ctrl Pts',(62.1755704420884,29.2962879878368,-215.149949));
#231132=CARTESIAN_POINT('Ctrl Pts',(48.9214109907111,16.6748094040191,-235.35005));
#231133=CARTESIAN_POINT('Ctrl Pts',(53.2924626390134,20.9224124018924,-228.68335));
#231134=CARTESIAN_POINT('Ctrl Pts',(57.663528252029,25.170015967144,-222.01665));
#231135=CARTESIAN_POINT('Ctrl Pts',(62.0346078304961,29.4176200813015,-215.34995));
#231136=CARTESIAN_POINT('Ctrl Pts',(62.0783186262808,29.4600961224431,-215.283283));
#231137=CARTESIAN_POINT('Ctrl Pts',(62.1220294220655,29.5025721635847,-215.216616));
#231138=CARTESIAN_POINT('Ctrl Pts',(62.1657402178502,29.5450482047262,-215.149949));
#231139=CARTESIAN_POINT('Ctrl Pts',(48.8992712925998,16.9131404133547,-235.35005));
#231140=CARTESIAN_POINT('Ctrl Pts',(53.2652870417935,21.2619501899207,-228.68335));
#231141=CARTESIAN_POINT('Ctrl Pts',(57.6313776897902,25.6107124643303,-222.01665));
#231142=CARTESIAN_POINT('Ctrl Pts',(61.9975402416511,29.9594276183431,-215.34995));
#231143=CARTESIAN_POINT('Ctrl Pts',(62.0412018671697,30.0029147698833,-215.283283));
#231144=CARTESIAN_POINT('Ctrl Pts',(62.0848634926883,30.0464019214233,-215.216616));
#231145=CARTESIAN_POINT('Ctrl Pts',(62.1285251182069,30.0898890729635,-215.149949));
#231146=CARTESIAN_POINT('Ctrl Pts',(48.8533444192211,17.2181014412188,-235.35005));
#231147=CARTESIAN_POINT('Ctrl Pts',(53.1855995667747,21.7941761255924,-228.68335));
#231148=CARTESIAN_POINT('Ctrl Pts',(57.5179747573295,26.3699864363254,-222.01665));
#231149=CARTESIAN_POINT('Ctrl Pts',(61.8504540244681,30.9455347714532,-215.34995));
#231150=CARTESIAN_POINT('Ctrl Pts',(61.8937788171395,30.9912902548045,-215.283283));
#231151=CARTESIAN_POINT('Ctrl Pts',(61.9371036098109,31.0370457381558,-215.216616));
#231152=CARTESIAN_POINT('Ctrl Pts',(61.9804284024823,31.082801221507,-215.149949));
#231153=CARTESIAN_POINT('Ctrl Pts',(48.793774157437,17.4925774935122,-235.35005));
#231154=CARTESIAN_POINT('Ctrl Pts',(53.0569741223029,22.3329163118503,-228.68335));
#231155=CARTESIAN_POINT('Ctrl Pts',(57.3203153214379,27.1726388120429,-222.01665));
#231156=CARTESIAN_POINT('Ctrl Pts',(61.5837608612094,32.0117507116806,-215.34995));
#231157=CARTESIAN_POINT('Ctrl Pts',(61.6263953166071,32.060141830677,-215.283283));
#231158=CARTESIAN_POINT('Ctrl Pts',(61.6690297720048,32.1085329496734,-215.216616));
#231159=CARTESIAN_POINT('Ctrl Pts',(61.7116642274025,32.1569240686698,-215.149949));
#231160=CARTESIAN_POINT('Ctrl Pts',(48.7243271460874,17.7538206185435,-235.35005));
#231161=CARTESIAN_POINT('Ctrl Pts',(52.8915700395936,22.8426678835018,-228.68335));
#231162=CARTESIAN_POINT('Ctrl Pts',(57.0589527628024,27.9304206519508,-222.01665));
#231163=CARTESIAN_POINT('Ctrl Pts',(61.2264100602501,33.0170891792215,-215.34995));
#231164=CARTESIAN_POINT('Ctrl Pts',(61.2680846332245,33.0679558644942,-215.283283));
#231165=CARTESIAN_POINT('Ctrl Pts',(61.309759206199,33.1188225497669,-215.216616));
#231166=CARTESIAN_POINT('Ctrl Pts',(61.3514337791735,33.1696892350396,-215.149949));
#231167=CARTESIAN_POINT('Ctrl Pts',(48.6354732464631,18.0177190827397,-235.35005));
#231168=CARTESIAN_POINT('Ctrl Pts',(52.6780922604543,23.3513726702934,-228.68335));
#231169=CARTESIAN_POINT('Ctrl Pts',(56.7208284608432,28.6833361882777,-222.01665));
#231170=CARTESIAN_POINT('Ctrl Pts',(60.7635813168395,34.0136255628538,-215.34995));
#231171=CARTESIAN_POINT('Ctrl Pts',(60.8040088453995,34.0669284565996,-215.283283));
#231172=CARTESIAN_POINT('Ctrl Pts',(60.8444363739595,34.1202313503453,-215.216616));
#231173=CARTESIAN_POINT('Ctrl Pts',(60.8848639025194,34.1735342440911,-215.149949));
#231174=CARTESIAN_POINT('Ctrl Pts',(48.5352774797299,18.2802794424427,-235.35005));
#231175=CARTESIAN_POINT('Ctrl Pts',(52.4343101169869,23.8247568642913,-228.68335));
#231176=CARTESIAN_POINT('Ctrl Pts',(56.3334174156944,29.3668400879758,-222.016650000001));
#231177=CARTESIAN_POINT('Ctrl Pts',(60.2324571773606,34.9065517584836,-215.349950000001));
#231178=CARTESIAN_POINT('Ctrl Pts',(60.2714475749772,34.9619488751887,-215.283283000001));
#231179=CARTESIAN_POINT('Ctrl Pts',(60.3104379725939,35.0173459918937,-215.216616));
#231180=CARTESIAN_POINT('Ctrl Pts',(60.3494283702106,35.0727431085988,-215.149949000001));
#231181=CARTESIAN_POINT('Ctrl Pts',(48.3890207412154,18.5878255918932,-235.35005));
#231182=CARTESIAN_POINT('Ctrl Pts',(52.1962991404372,24.228375758149,-228.68335));
#231183=CARTESIAN_POINT('Ctrl Pts',(56.0035911516163,29.8657278812732,-222.01665));
#231184=CARTESIAN_POINT('Ctrl Pts',(59.810707037304,35.4999122879811,-215.34995));
#231185=CARTESIAN_POINT('Ctrl Pts',(59.8487781961609,35.5562541320482,-215.283283));
#231186=CARTESIAN_POINT('Ctrl Pts',(59.8868493550178,35.6125959761153,-215.216616));
#231187=CARTESIAN_POINT('Ctrl Pts',(59.9249205138747,35.6689378201824,-215.149949));
#231188=CARTESIAN_POINT('Ctrl Pts',(48.2711217441656,18.8106246802399,-235.35005));
#231189=CARTESIAN_POINT('Ctrl Pts',(52.0406861996216,24.475501377336,-228.68335));
#231190=CARTESIAN_POINT('Ctrl Pts',(55.8102121224059,30.1365835498488,-222.01665));
#231191=CARTESIAN_POINT('Ctrl Pts',(59.5794745156759,35.7939072308497,-215.34995));
#231192=CARTESIAN_POINT('Ctrl Pts',(59.6171671396086,35.8504804676597,-215.283283));
#231193=CARTESIAN_POINT('Ctrl Pts',(59.6548597635413,35.9070537044696,-215.216616));
#231194=CARTESIAN_POINT('Ctrl Pts',(59.692552387474,35.9636269412797,-215.149949));
#231195=CARTESIAN_POINT('Ctrl Pts',(48.1560655143106,18.9923105754345,-235.35005));
#231196=CARTESIAN_POINT('Ctrl Pts',(51.9286217775904,24.6399928719346,-228.68335));
#231197=CARTESIAN_POINT('Ctrl Pts',(55.7011108008251,30.2835687301176,-222.01665));
#231198=CARTESIAN_POINT('Ctrl Pts',(59.4732891526392,35.9230771683515,-215.34995));
#231199=CARTESIAN_POINT('Ctrl Pts',(59.5110109361573,35.9794722527339,-215.283283));
#231200=CARTESIAN_POINT('Ctrl Pts',(59.5487327196755,36.0358673371162,-215.216616));
#231201=CARTESIAN_POINT('Ctrl Pts',(59.5864545031936,36.0922624214986,-215.149949));
#231202=CARTESIAN_POINT('Ctrl Pts',(48.1468610159222,19.00684544705,-235.35005));
#231203=CARTESIAN_POINT('Ctrl Pts',(51.9196566238279,24.6531521915024,-228.68335));
#231204=CARTESIAN_POINT('Ctrl Pts',(55.6923826950986,30.2953275445391,-222.01665));
#231205=CARTESIAN_POINT('Ctrl Pts',(59.4647943235962,35.9334107633517,-215.34995));
#231206=CARTESIAN_POINT('Ctrl Pts',(59.5025184398812,35.9897915955398,-215.283283));
#231207=CARTESIAN_POINT('Ctrl Pts',(59.5402425561662,36.046172427728,-215.216616));
#231208=CARTESIAN_POINT('Ctrl Pts',(59.5779666724512,36.102553259916,-215.149949));
#231209=CARTESIAN_POINT('Ctrl Pts',(48.1376565175338,19.0213803186655,-235.35005));
#231210=CARTESIAN_POINT('Ctrl Pts',(51.9106914700654,24.6663115110703,-228.68335));
#231211=CARTESIAN_POINT('Ctrl Pts',(55.6836545893721,30.3070863589606,-222.01665));
#231212=CARTESIAN_POINT('Ctrl Pts',(59.4562994945533,35.9437443583519,-215.34995));
#231213=CARTESIAN_POINT('Ctrl Pts',(59.4940259436051,36.0001109383457,-215.283283));
#231214=CARTESIAN_POINT('Ctrl Pts',(59.5317523926569,36.0564775183397,-215.216616));
#231215=CARTESIAN_POINT('Ctrl Pts',(59.5694788417088,36.1128440983336,-215.149949));
#231216=CARTESIAN_POINT('Ctrl Pts',(48.1284520191454,19.0359151902811,-235.35005));
#231217=CARTESIAN_POINT('Ctrl Pts',(51.9017263163029,24.6794708306382,-228.68335));
#231218=CARTESIAN_POINT('Ctrl Pts',(55.6749264836457,30.3188451733821,-222.01665));
#231219=CARTESIAN_POINT('Ctrl Pts',(59.4478046655104,35.9540779533519,-215.34995));
#231220=CARTESIAN_POINT('Ctrl Pts',(59.485533447329,36.0104302811517,-215.283283));
#231221=CARTESIAN_POINT('Ctrl Pts',(59.5232622291477,36.0667826089514,-215.216616));
#231222=CARTESIAN_POINT('Ctrl Pts',(59.5609910109663,36.1231349367511,-215.149949));
#231223=CARTESIAN_POINT('',(55.4860418356284,22.8455890891576,-225.35));
#231224=CARTESIAN_POINT('Ctrl Pts',(48.4260896922586,19.3965417854656,-234.872874618363));
#231225=CARTESIAN_POINT('Ctrl Pts',(51.8397102119512,24.5067087698627,-228.840465153427));
#231226=CARTESIAN_POINT('Ctrl Pts',(55.2532709224339,29.6135143043896,-222.808055688492));
#231227=CARTESIAN_POINT('Ctrl Pts',(58.6665914736623,34.7169872964315,-216.775646223556));
#231228=CARTESIAN_POINT('Origin',(41.5452362233251,-63.7990866568863,-205.34995));
#231229=CARTESIAN_POINT('',(48.8319431829163,-72.7145462807723,-205.34995));
#231230=CARTESIAN_POINT('',(41.9984355604289,-75.3045692187324,-205.34995));
#231231=CARTESIAN_POINT('Origin',(0.,-12.9675000200281,-205.34995));
#231232=CARTESIAN_POINT('',(59.6081272922882,-61.9689221688742,-205.34995));
#231233=CARTESIAN_POINT('Origin',(50.7133971693864,-54.6569255427236,-205.34995));
#231234=CARTESIAN_POINT('',(62.2188176672479,-55.1116977796555,-205.34995));
#231235=CARTESIAN_POINT('Origin',(50.7133971693864,28.7219255026674,-205.34995));
#231236=CARTESIAN_POINT('',(59.6081272922883,36.0339221288179,-205.34995));
#231237=CARTESIAN_POINT('',(62.218817667248,29.176697739599,-205.34995));
#231238=CARTESIAN_POINT('Origin',(0.,-12.9675000200281,-205.34995));
#231239=CARTESIAN_POINT('',(48.5592309447134,47.0014027710106,-205.34995));
#231240=CARTESIAN_POINT('Origin',(41.3132181298675,38.0528376956935,-205.34995));
#231241=CARTESIAN_POINT('',(43.4702127313761,49.3634032389879,-205.34995));
#231242=CARTESIAN_POINT('Origin',(0.,990.91999998,-205.34995));
#231243=CARTESIAN_POINT('Origin',(-476.643301415307,-33.8122127813758,-179.64995));
#231244=CARTESIAN_POINT('',(44.0225733573905,52.2597994838836,-179.64995));
#231245=CARTESIAN_POINT('Origin',(0.,-178.58000002,-179.64995));
#231246=CARTESIAN_POINT('',(42.1144903105792,-78.2508795831687,-179.64995));
#231247=CARTESIAN_POINT('Origin',(0.,990.91999998,-179.64995));
#231248=CARTESIAN_POINT('',(50.6979144815776,-74.9976066350312,-179.64995));
#231249=CARTESIAN_POINT('Origin',(41.5452362233251,-63.7990866568863,-179.64995));
#231250=CARTESIAN_POINT('',(61.8858792604563,-63.8413696154326,-179.64995));
#231251=CARTESIAN_POINT('Origin',(0.,-12.9675000200281,-179.64995));
#231252=CARTESIAN_POINT('',(65.1651121384123,-55.2281553161325,-179.64995));
#231253=CARTESIAN_POINT('Origin',(50.7133971693864,-54.6569255427236,-179.64995));
#231254=CARTESIAN_POINT('',(65.1651121384124,29.2931552760762,-179.64995));
#231255=CARTESIAN_POINT('Origin',(-1004.,-12.967500020028,-179.64995));
#231256=CARTESIAN_POINT('',(61.8858792604563,37.9063695753764,-179.64995));
#231257=CARTESIAN_POINT('Origin',(50.7133971693864,28.7219255026673,-179.64995));
#231258=CARTESIAN_POINT('',(50.4147813349261,49.2929407301111,-179.64995));
#231259=CARTESIAN_POINT('Origin',(0.,-12.9675000200281,-179.64995));
#231260=CARTESIAN_POINT('Origin',(41.3132181298675,38.0528376956935,-179.64995));
#231261=CARTESIAN_POINT('Origin',(-476.643301415307,-33.8122127813758,-205.34995));
#231262=CARTESIAN_POINT('Origin',(-1004.,-12.967500020028,-179.64995));
#231263=CARTESIAN_POINT('',(65.1651121384124,-55.2281553161325,-179.64995));
#231264=CARTESIAN_POINT('',(65.1651121384125,29.293155276076,-179.64995));
#231265=CARTESIAN_POINT('Origin',(50.7133971693864,28.7219255026673,-179.64995));
#231266=CARTESIAN_POINT('',(61.8858792604564,37.9063695753764,-179.64995));
#231267=CARTESIAN_POINT('Origin',(0.,-12.9675000200281,-179.64995));
#231268=CARTESIAN_POINT('',(50.4147813349261,49.292940730111,-179.64995));
#231269=CARTESIAN_POINT('Origin',(41.3132181298675,38.0528376956935,-179.64995));
#231270=CARTESIAN_POINT('',(44.0225733573905,52.2597994838836,-179.64995));
#231271=CARTESIAN_POINT('Origin',(0.,-178.58000002,-179.64995));
#231272=CARTESIAN_POINT('Origin',(0.,990.91999998,-179.64995));
#231273=CARTESIAN_POINT('',(42.1144903105791,-78.2508795831687,-179.64995));
#231274=CARTESIAN_POINT('Origin',(41.5452362233251,-63.7990866568863,-179.64995));
#231275=CARTESIAN_POINT('',(50.6979144815776,-74.9976066350312,-179.64995));
#231276=CARTESIAN_POINT('Origin',(0.,-12.9675000200281,-179.64995));
#231277=CARTESIAN_POINT('',(61.8858792604563,-63.8413696154326,-179.64995));
#231278=CARTESIAN_POINT('Origin',(50.7133971693864,-54.6569255427236,-179.64995));
#231279=CARTESIAN_POINT('Ctrl Pts',(48.9276804568491,-39.5283381317121,
-235.35005));
#231280=CARTESIAN_POINT('Ctrl Pts',(53.2999213760692,-44.7204933330714,
-228.68335));
#231281=CARTESIAN_POINT('Ctrl Pts',(57.6721622952894,-49.9126485344307,
-222.01665));
#231282=CARTESIAN_POINT('Ctrl Pts',(62.0444032145095,-55.1048037357899,
-215.34995));
#231283=CARTESIAN_POINT('Ctrl Pts',(49.0194233450359,-37.283081077169,-235.35005));
#231284=CARTESIAN_POINT('Ctrl Pts',(53.4090672042376,-42.0148742220589,
-228.683350000001));
#231285=CARTESIAN_POINT('Ctrl Pts',(57.7985067146479,-46.7466590436653,
-222.016650000001));
#231286=CARTESIAN_POINT('Ctrl Pts',(62.1877418657617,-51.4784358040522,
-215.34995));
#231287=CARTESIAN_POINT('Ctrl Pts',(49.1841844420714,-32.7087365060477,
-235.35005));
#231288=CARTESIAN_POINT('Ctrl Pts',(53.600359505658,-36.5883830285289,-228.68335));
#231289=CARTESIAN_POINT('Ctrl Pts',(58.0165345692446,-40.4680295510101,
-222.01665));
#231290=CARTESIAN_POINT('Ctrl Pts',(62.4327096328312,-44.3476760734913,
-215.34995));
#231291=CARTESIAN_POINT('Ctrl Pts',(49.3659986639477,-25.6715165814334,
-235.35005));
#231292=CARTESIAN_POINT('Ctrl Pts',(53.8070961606803,-28.4006856868431,
-228.68335));
#231293=CARTESIAN_POINT('Ctrl Pts',(58.2481936574129,-31.1298547922528,
-222.01665));
#231294=CARTESIAN_POINT('Ctrl Pts',(62.6892911541455,-33.8590238976625,
-215.34995));
#231295=CARTESIAN_POINT('Ctrl Pts',(49.4760453414413,-18.5583238061847,
-235.35005));
#231296=CARTESIAN_POINT('Ctrl Pts',(53.9314601157808,-20.1883767671888,
-228.68335));
#231297=CARTESIAN_POINT('Ctrl Pts',(58.3868748901203,-21.8184297281929,
-222.01665));
#231298=CARTESIAN_POINT('Ctrl Pts',(62.8422896644598,-23.448482689197,-215.34995));
#231299=CARTESIAN_POINT('Ctrl Pts',(49.5,-13.8395357876534,-235.35005));
#231300=CARTESIAN_POINT('Ctrl Pts',(53.9589513940208,-14.7196423822522,
-228.68335));
#231301=CARTESIAN_POINT('Ctrl Pts',(58.4179027880416,-15.599748976851,-222.01665));
#231302=CARTESIAN_POINT('Ctrl Pts',(62.8768541820624,-16.4798555714498,
-215.34995));
#231303=CARTESIAN_POINT('Ctrl Pts',(49.5,-11.5034818258362,-235.35005));
#231304=CARTESIAN_POINT('Ctrl Pts',(53.9589513940208,-11.9914878905669,
-228.68335));
#231305=CARTESIAN_POINT('Ctrl Pts',(58.4179027880416,-12.4794939552975,
-222.01665));
#231306=CARTESIAN_POINT('Ctrl Pts',(62.8768541820624,-12.9675000200282,
-215.34995));
#231307=CARTESIAN_POINT('Ctrl Pts',(49.5,-11.5034818258362,-235.35005));
#231308=CARTESIAN_POINT('Ctrl Pts',(53.9589513940208,-11.9914878905669,
-228.68335));
#231309=CARTESIAN_POINT('Ctrl Pts',(58.4179027880416,-12.4794939552975,
-222.01665));
#231310=CARTESIAN_POINT('Ctrl Pts',(62.8768541820624,-12.9675000200282,
-215.34995));
#231311=CARTESIAN_POINT('Ctrl Pts',(62.9214436960026,-12.9723800806755,
-215.283283));
#231312=CARTESIAN_POINT('Ctrl Pts',(62.9660332099428,-12.9772601413228,
-215.216616));
#231313=CARTESIAN_POINT('Ctrl Pts',(63.010622723883,-12.9821402019701,-215.149949));
#231314=CARTESIAN_POINT('Ctrl Pts',(49.5,-9.16742786401911,-235.35005));
#231315=CARTESIAN_POINT('Ctrl Pts',(53.9589513940208,-9.26333339888158,
-228.68335));
#231316=CARTESIAN_POINT('Ctrl Pts',(58.4179027880416,-9.35923893374405,
-222.01665));
#231317=CARTESIAN_POINT('Ctrl Pts',(62.8768541820624,-9.45514446860653,
-215.34995));
#231318=CARTESIAN_POINT('Ctrl Pts',(62.9214436960026,-9.45610352395515,
-215.283283));
#231319=CARTESIAN_POINT('Ctrl Pts',(62.9660332099428,-9.45706257930377,
-215.216616));
#231320=CARTESIAN_POINT('Ctrl Pts',(63.010622723883,-9.4580216346524,-215.149949));
#231321=CARTESIAN_POINT('Ctrl Pts',(49.4760453034623,-4.44863709409477,
-235.35005));
#231322=CARTESIAN_POINT('Ctrl Pts',(53.9314600904615,-3.79459717968296,
-228.68335));
#231323=CARTESIAN_POINT('Ctrl Pts',(58.3868748774607,-3.14055726527114,
-222.01665));
#231324=CARTESIAN_POINT('Ctrl Pts',(62.8422896644599,-2.48651735085932,
-215.34995));
#231325=CARTESIAN_POINT('Ctrl Pts',(62.8868438123299,-2.47997695171521,
-215.283283));
#231326=CARTESIAN_POINT('Ctrl Pts',(62.9313979601999,-2.47343655257108,
-215.216616));
#231327=CARTESIAN_POINT('Ctrl Pts',(62.9759521080699,-2.46689615342696,
-215.149949));
#231328=CARTESIAN_POINT('Ctrl Pts',(49.3659992921549,2.6645466712911,-235.350050000001));
#231329=CARTESIAN_POINT('Ctrl Pts',(53.8070965794851,4.41770573339612,-228.683350000001));
#231330=CARTESIAN_POINT('Ctrl Pts',(58.2481938668153,6.17086479550113,-222.016650000001));
#231331=CARTESIAN_POINT('Ctrl Pts',(62.6892911541455,7.92402385760615,-215.349950000001));
#231332=CARTESIAN_POINT('Ctrl Pts',(62.7337021270188,7.9415554482272,-215.283283000001));
#231333=CARTESIAN_POINT('Ctrl Pts',(62.7781130998921,7.95908703884825,-215.216616));
#231334=CARTESIAN_POINT('Ctrl Pts',(62.8225240727654,7.9766186294693,-215.149949000001));
#231335=CARTESIAN_POINT('Ctrl Pts',(49.1841830823307,9.70178317521733,-235.35005));
#231336=CARTESIAN_POINT('Ctrl Pts',(53.6003585991642,12.6054141279565,-228.68335));
#231337=CARTESIAN_POINT('Ctrl Pts',(58.0165341159977,15.5090450806958,-222.01665));
#231338=CARTESIAN_POINT('Ctrl Pts',(62.4327096328312,18.412676033435,-215.34995));
#231339=CARTESIAN_POINT('Ctrl Pts',(62.4768713879996,18.4417123429624,-215.283283));
#231340=CARTESIAN_POINT('Ctrl Pts',(62.5210331431679,18.4707486524898,-215.216616));
#231341=CARTESIAN_POINT('Ctrl Pts',(62.5651948983362,18.4997849620172,-215.149949));
#231342=CARTESIAN_POINT('Ctrl Pts',(49.0194233450359,14.2761174254963,-235.35005));
#231343=CARTESIAN_POINT('Ctrl Pts',(53.4090672042376,18.031898440925,-228.68335));
#231344=CARTESIAN_POINT('Ctrl Pts',(57.7985067146477,21.7876711330703,-222.01665));
#231345=CARTESIAN_POINT('Ctrl Pts',(62.1877418657617,25.5434357639959,-215.34995));
#231346=CARTESIAN_POINT('Ctrl Pts',(62.2316342172729,25.5809934103052,-215.283283));
#231347=CARTESIAN_POINT('Ctrl Pts',(62.275526568784,25.6185510566144,-215.216616));
#231348=CARTESIAN_POINT('Ctrl Pts',(62.3194189202952,25.6561087029237,-215.149949));
#231349=CARTESIAN_POINT('Ctrl Pts',(48.9276804568491,16.5213744800396,-235.35005));
#231350=CARTESIAN_POINT('Ctrl Pts',(53.2999213760048,20.7375175535383,-228.68335));
#231351=CARTESIAN_POINT('Ctrl Pts',(57.6721622952182,24.9536606256242,-222.01665));
#231352=CARTESIAN_POINT('Ctrl Pts',(62.0444032145096,29.1698036957335,-215.34995));
#231353=CARTESIAN_POINT('Ctrl Pts',(62.0881256237025,29.2119651264346,-215.283283));
#231354=CARTESIAN_POINT('Ctrl Pts',(62.1318480328954,29.2541265571357,-215.216616));
#231355=CARTESIAN_POINT('Ctrl Pts',(62.1755704420884,29.2962879878368,-215.149949));
#231356=CARTESIAN_POINT('Origin',(-1004.,-12.967500020028,-205.34995));
#231357=CARTESIAN_POINT('Ctrl Pts',(27.1569075795172,38.1844371310006,-235.35005));
#231358=CARTESIAN_POINT('Ctrl Pts',(32.5837764342019,41.8536056393876,-228.68335));
#231359=CARTESIAN_POINT('Ctrl Pts',(38.0106452875494,45.5227741479461,-222.01665));
#231360=CARTESIAN_POINT('Ctrl Pts',(43.4375141409548,49.1919426564936,-215.34995));
#231361=CARTESIAN_POINT('Ctrl Pts',(43.4917828294889,49.2286343415791,-215.283283));
#231362=CARTESIAN_POINT('Ctrl Pts',(43.5460515180229,49.2653260266646,-215.216616));
#231363=CARTESIAN_POINT('Ctrl Pts',(43.600320206557,49.30201771175,-215.149949));
#231364=CARTESIAN_POINT('Ctrl Pts',(22.7175376169318,38.7537549124104,-235.35005));
#231365=CARTESIAN_POINT('Ctrl Pts',(27.2067518411579,42.6544032575593,-228.68335));
#231366=CARTESIAN_POINT('Ctrl Pts',(31.7011009472754,46.5938202572852,-222.01665));
#231367=CARTESIAN_POINT('Ctrl Pts',(36.2028725106807,50.5716334315145,-215.34995));
#231368=CARTESIAN_POINT('Ctrl Pts',(36.2478902263148,50.6114115632568,-215.283283));
#231369=CARTESIAN_POINT('Ctrl Pts',(36.2929079419489,50.6511896949991,-215.216616));
#231370=CARTESIAN_POINT('Ctrl Pts',(36.3379256575829,50.6909678267414,-215.149949));
#231371=CARTESIAN_POINT('Ctrl Pts',(13.711356444076,39.6240660636921,-235.35005));
#231372=CARTESIAN_POINT('Ctrl Pts',(16.3741503826813,43.8592570013518,-228.68335));
#231373=CARTESIAN_POINT('Ctrl Pts',(19.0446466451262,48.1913695751969,-222.01665));
#231374=CARTESIAN_POINT('Ctrl Pts',(21.7262765934597,52.6194725853171,-215.34995));
#231375=CARTESIAN_POINT('Ctrl Pts',(21.753092892943,52.6637536154183,-215.283283));
#231376=CARTESIAN_POINT('Ctrl Pts',(21.7799091924264,52.7080346455195,-215.216616));
#231377=CARTESIAN_POINT('Ctrl Pts',(21.8067254919097,52.7523156756207,-215.149949));
#231378=CARTESIAN_POINT('Ctrl Pts',(-5.03069808033274E-14,40.0660654363212,
-235.350050000001));
#231379=CARTESIAN_POINT('Ctrl Pts',(-2.50315176572591E-14,44.4636082157172,
-228.683350000001));
#231380=CARTESIAN_POINT('Ctrl Pts',(3.67646180426256E-14,48.9871491221026,
-222.016650000001));
#231381=CARTESIAN_POINT('Ctrl Pts',(-2.42861286636753E-14,53.6354775956494,
-215.34995));
#231382=CARTESIAN_POINT('Ctrl Pts',(-2.48966361307383E-14,53.6819608803848,
-215.283283));
#231383=CARTESIAN_POINT('Ctrl Pts',(-2.55071435978013E-14,53.7284441651203,
-215.216616));
#231384=CARTESIAN_POINT('Ctrl Pts',(-2.61176510648644E-14,53.7749274498558,
-215.149949));
#231385=CARTESIAN_POINT('Ctrl Pts',(-13.7113564440761,39.6240660636921,
-235.35005));
#231386=CARTESIAN_POINT('Ctrl Pts',(-16.3741503826814,43.8592570013518,
-228.68335));
#231387=CARTESIAN_POINT('Ctrl Pts',(-19.0446466451262,48.1913695751964,
-222.01665));
#231388=CARTESIAN_POINT('Ctrl Pts',(-21.7262765934598,52.619472585317,-215.34995));
#231389=CARTESIAN_POINT('Ctrl Pts',(-21.7530928929431,52.6637536154182,
-215.283283));
#231390=CARTESIAN_POINT('Ctrl Pts',(-21.7799091924265,52.7080346455194,
-215.216616));
#231391=CARTESIAN_POINT('Ctrl Pts',(-21.8067254919098,52.7523156756206,
-215.149949));
#231392=CARTESIAN_POINT('Ctrl Pts',(-22.7175376169319,38.7537549124104,
-235.350050000001));
#231393=CARTESIAN_POINT('Ctrl Pts',(-27.206751841158,42.6544032575593,-228.68335));
#231394=CARTESIAN_POINT('Ctrl Pts',(-31.7011009472754,46.5938202572849,
-222.01665));
#231395=CARTESIAN_POINT('Ctrl Pts',(-36.2028725106808,50.5716334315145,
-215.34995));
#231396=CARTESIAN_POINT('Ctrl Pts',(-36.2478902263149,50.6114115632568,
-215.283283));
#231397=CARTESIAN_POINT('Ctrl Pts',(-36.2929079419489,50.6511896949991,
-215.216616));
#231398=CARTESIAN_POINT('Ctrl Pts',(-36.337925657583,50.6909678267414,-215.149949));
#231399=CARTESIAN_POINT('Ctrl Pts',(-27.1569075795173,38.1844371310006,
-235.35005));
#231400=CARTESIAN_POINT('Ctrl Pts',(-32.5837764342019,41.8536056393876,
-228.68335));
#231401=CARTESIAN_POINT('Ctrl Pts',(-38.0106452875494,45.5227741479461,
-222.01665));
#231402=CARTESIAN_POINT('Ctrl Pts',(-43.4375141409549,49.1919426564936,
-215.34995));
#231403=CARTESIAN_POINT('Ctrl Pts',(-43.491782829489,49.2286343415791,-215.283283));
#231404=CARTESIAN_POINT('Ctrl Pts',(-43.546051518023,49.2653260266646,-215.216616));
#231405=CARTESIAN_POINT('Ctrl Pts',(-43.6003202065571,49.30201771175,-215.149949));
#231406=CARTESIAN_POINT('Origin',(0.,-178.58000002,-205.34995));
#231407=CARTESIAN_POINT('Origin',(-296.501483394397,-25.4138432731711,-235.35005));
#231408=CARTESIAN_POINT('Ctrl Pts',(-24.4459324049495,-62.4902066935372,
-235.35005));
#231409=CARTESIAN_POINT('Ctrl Pts',(-30.2944767260349,-66.7035224039814,
-228.68335));
#231410=CARTESIAN_POINT('Ctrl Pts',(-36.1430210443398,-70.9168381145246,
-222.01665));
#231411=CARTESIAN_POINT('Ctrl Pts',(-41.991565360621,-75.1301538251475,
-215.34995));
#231412=CARTESIAN_POINT('Ctrl Pts',(-42.0500508037838,-75.1722869822537,
-215.283283));
#231413=CARTESIAN_POINT('Ctrl Pts',(-42.1085362469466,-75.21442013936,-215.216616));
#231414=CARTESIAN_POINT('Ctrl Pts',(-42.1670216901095,-75.2565532964662,
-215.149949));
#231415=CARTESIAN_POINT('Ctrl Pts',(-20.4621956228808,-62.6321691537996,
-235.35005));
#231416=CARTESIAN_POINT('Ctrl Pts',(-25.267980358079,-66.8889339565476,
-228.68335));
#231417=CARTESIAN_POINT('Ctrl Pts',(-30.0738587790242,-71.1483055815339,
-222.01665));
#231418=CARTESIAN_POINT('Ctrl Pts',(-34.8798403105591,-75.4102836728986,
-215.34995));
#231419=CARTESIAN_POINT('Ctrl Pts',(-34.9279001258744,-75.4529034538122,
-215.283283));
#231420=CARTESIAN_POINT('Ctrl Pts',(-34.9759599411898,-75.4955232347258,
-215.216616));
#231421=CARTESIAN_POINT('Ctrl Pts',(-35.0240197565051,-75.5381430156395,
-215.149949));
#231422=CARTESIAN_POINT('Ctrl Pts',(-12.3633338208145,-62.8510026026509,
-235.35005));
#231423=CARTESIAN_POINT('Ctrl Pts',(-15.1854795229237,-67.1680657809434,
-228.68335));
#231424=CARTESIAN_POINT('Ctrl Pts',(-18.0077657557388,-71.4916460146837,
-222.01665));
#231425=CARTESIAN_POINT('Ctrl Pts',(-20.8302066559562,-75.8217424142497,
-215.34995));
#231426=CARTESIAN_POINT('Ctrl Pts',(-20.8584310649584,-75.8650433782453,
-215.283283));
#231427=CARTESIAN_POINT('Ctrl Pts',(-20.8866554739606,-75.908344342241,
-215.216616));
#231428=CARTESIAN_POINT('Ctrl Pts',(-20.9148798829627,-75.9516453062367,
-215.149949));
#231429=CARTESIAN_POINT('Ctrl Pts',(-1.09287578986539E-13,-62.9629927582852,
-235.35005));
#231430=CARTESIAN_POINT('Ctrl Pts',(1.49836951995733E-13,-67.3083190291539,
-228.683350000001));
#231431=CARTESIAN_POINT('Ctrl Pts',(3.24284869790415E-13,-71.6621174720752,
-222.016650000001));
#231432=CARTESIAN_POINT('Ctrl Pts',(5.36029554076834E-13,-76.0243869305461,
-215.349950000001));
#231433=CARTESIAN_POINT('Ctrl Pts',(5.38147000919697E-13,-76.0680096251308,
-215.283283000001));
#231434=CARTESIAN_POINT('Ctrl Pts',(5.40264447762562E-13,-76.1116323197155,
-215.216616000001));
#231435=CARTESIAN_POINT('Ctrl Pts',(5.42381894605426E-13,-76.1552550143002,
-215.149949000001));
#231436=CARTESIAN_POINT('Ctrl Pts',(12.3633338208143,-62.8510026026509,
-235.35005));
#231437=CARTESIAN_POINT('Ctrl Pts',(15.185479522924,-67.1680657809432,-228.68335));
#231438=CARTESIAN_POINT('Ctrl Pts',(18.0077657557395,-71.4916460146835,
-222.01665));
#231439=CARTESIAN_POINT('Ctrl Pts',(20.8302066559573,-75.8217424142497,
-215.34995));
#231440=CARTESIAN_POINT('Ctrl Pts',(20.8584310649595,-75.8650433782453,
-215.283283));
#231441=CARTESIAN_POINT('Ctrl Pts',(20.8866554739617,-75.908344342241,-215.216616));
#231442=CARTESIAN_POINT('Ctrl Pts',(20.9148798829638,-75.9516453062367,
-215.149949));
#231443=CARTESIAN_POINT('Ctrl Pts',(20.4621956228805,-62.6321691537997,
-235.35005));
#231444=CARTESIAN_POINT('Ctrl Pts',(25.2679803580793,-66.8889339565475,
-228.68335));
#231445=CARTESIAN_POINT('Ctrl Pts',(30.0738587790249,-71.1483055815338,
-222.01665));
#231446=CARTESIAN_POINT('Ctrl Pts',(34.8798403105602,-75.4102836728983,
-215.34995));
#231447=CARTESIAN_POINT('Ctrl Pts',(34.9279001258756,-75.4529034538119,
-215.283283));
#231448=CARTESIAN_POINT('Ctrl Pts',(34.975959941191,-75.4955232347256,-215.216616));
#231449=CARTESIAN_POINT('Ctrl Pts',(35.0240197565063,-75.5381430156392,
-215.149949));
#231450=CARTESIAN_POINT('Ctrl Pts',(24.4459324049493,-62.4902066935372,
-235.35005));
#231451=CARTESIAN_POINT('Ctrl Pts',(30.2944767260352,-66.7035224039813,
-228.68335));
#231452=CARTESIAN_POINT('Ctrl Pts',(36.1430210443405,-70.9168381145244,
-222.01665));
#231453=CARTESIAN_POINT('Ctrl Pts',(41.9915653606222,-75.1301538251473,
-215.34995));
#231454=CARTESIAN_POINT('Ctrl Pts',(42.050050803785,-75.1722869822535,-215.283283));
#231455=CARTESIAN_POINT('Ctrl Pts',(42.1085362469478,-75.2144201393598,
-215.216616));
#231456=CARTESIAN_POINT('Ctrl Pts',(42.1670216901106,-75.256553296466,-215.149949));
#231457=CARTESIAN_POINT('Origin',(0.,-12.9675000200281,-218.35005));
#231458=CARTESIAN_POINT('Ctrl Pts',(7312.83864083626,-22580.9607088348,
-376.75075701007));
#231459=CARTESIAN_POINT('Ctrl Pts',(6830.77747415825,-19700.0678309805,
-349.81728900813));
#231460=CARTESIAN_POINT('Ctrl Pts',(6348.71630748024,-16819.1749531262,
-322.88382100619));
#231461=CARTESIAN_POINT('Ctrl Pts',(5866.65514080223,-13938.2820752719,
-295.95035300425));
#231462=CARTESIAN_POINT('Ctrl Pts',(5625.62455746322,-12497.8356363448,
-282.483619003281));
#231463=CARTESIAN_POINT('Ctrl Pts',(5384.59397412422,-11057.3891974177,
-269.01688500231));
#231464=CARTESIAN_POINT('Ctrl Pts',(5143.56339078521,-9616.94275849054,
-255.55015100134));
#231465=CARTESIAN_POINT('Ctrl Pts',(5023.0480991157,-8896.71953902697,-248.816784000855));
#231466=CARTESIAN_POINT('Ctrl Pts',(4902.5328074462,-8176.49631956341,-242.083417000367));
#231467=CARTESIAN_POINT('Ctrl Pts',(4782.0175157767,-7456.27310009984,-235.350049999879));
#231468=CARTESIAN_POINT('Ctrl Pts',(4662.69544481679,-6743.18080360126,
-228.683349999394));
#231469=CARTESIAN_POINT('Ctrl Pts',(4544.55443977813,-6017.25926759624,
-222.01665));
#231470=CARTESIAN_POINT('Ctrl Pts',(4428.35272571124,-5278.63127980493,
-215.34995));
#231471=CARTESIAN_POINT('Ctrl Pts',(4427.19070857058,-5271.24499992702,
-215.283283));
#231472=CARTESIAN_POINT('Ctrl Pts',(4426.02869142993,-5263.85872004911,
-215.216616));
#231473=CARTESIAN_POINT('Ctrl Pts',(4424.86667428927,-5256.4724401712,-215.149949));
#231474=CARTESIAN_POINT('Ctrl Pts',(5678.44144856441,-17578.5062585325,
-376.75075700783));
#231475=CARTESIAN_POINT('Ctrl Pts',(5307.04370444825,-15333.6138629625,
-349.817289006321));
#231476=CARTESIAN_POINT('Ctrl Pts',(4935.64596033209,-13088.7214673926,
-322.883821004812));
#231477=CARTESIAN_POINT('Ctrl Pts',(4564.24821621593,-10843.8290718226,
-295.950353003305));
#231478=CARTESIAN_POINT('Ctrl Pts',(4378.54934415786,-9721.38287403765,
-282.48361900255));
#231479=CARTESIAN_POINT('Ctrl Pts',(4192.85047209977,-8598.93667625267,
-269.016885001796));
#231480=CARTESIAN_POINT('Ctrl Pts',(4007.1516000417,-7476.4904784677,-255.550151001042));
#231481=CARTESIAN_POINT('Ctrl Pts',(3914.30216401265,-6915.26737957521,
-248.816784000665));
#231482=CARTESIAN_POINT('Ctrl Pts',(3821.45272798362,-6354.04428068272,
-242.083417000286));
#231483=CARTESIAN_POINT('Ctrl Pts',(3728.60329195457,-5792.82118179023,
-235.350049999906));
#231484=CARTESIAN_POINT('Ctrl Pts',(3636.67315727236,-5237.15474724321,
-228.683349999529));
#231485=CARTESIAN_POINT('Ctrl Pts',(3545.66125393428,-4671.51484522691,
-222.01665));
#231486=CARTESIAN_POINT('Ctrl Pts',(3456.15702691661,-4095.9969311378,-215.34995));
#231487=CARTESIAN_POINT('Ctrl Pts',(3455.26198464644,-4090.24175199691,
-215.283283));
#231488=CARTESIAN_POINT('Ctrl Pts',(3454.36694237628,-4084.48657285602,
-215.216616));
#231489=CARTESIAN_POINT('Ctrl Pts',(3453.47190010611,-4078.73139371513,
-215.149949));
#231490=CARTESIAN_POINT('Ctrl Pts',(4044.04425629255,-12576.0518082303,
-376.750757005589));
#231491=CARTESIAN_POINT('Ctrl Pts',(3783.30993473824,-10967.1598949446,
-349.817289004512));
#231492=CARTESIAN_POINT('Ctrl Pts',(3522.57561318394,-9358.26798165898,
-322.883821003436));
#231493=CARTESIAN_POINT('Ctrl Pts',(3261.84129162964,-7749.37606837333,
-295.950353002358));
#231494=CARTESIAN_POINT('Ctrl Pts',(3131.47413085249,-6944.9301117305,-282.483619001821));
#231495=CARTESIAN_POINT('Ctrl Pts',(3001.10697007533,-6140.48415508768,
-269.016885001282));
#231496=CARTESIAN_POINT('Ctrl Pts',(2870.73980929818,-5336.03819844486,
-255.550151000744));
#231497=CARTESIAN_POINT('Ctrl Pts',(2805.5562289096,-4933.81522012345,-248.816784000475));
#231498=CARTESIAN_POINT('Ctrl Pts',(2740.37264852102,-4531.59224180204,
-242.083417000204));
#231499=CARTESIAN_POINT('Ctrl Pts',(2675.18906813245,-4129.36926348062,
-235.350049999933));
#231500=CARTESIAN_POINT('Ctrl Pts',(2610.65086972792,-3731.12869088517,
-228.683349999664));
#231501=CARTESIAN_POINT('Ctrl Pts',(2546.76806809043,-3325.77042285759,
-222.01665));
#231502=CARTESIAN_POINT('Ctrl Pts',(2483.96132812197,-2913.36258247067,
-215.34995));
#231503=CARTESIAN_POINT('Ctrl Pts',(2483.3332607223,-2909.2385040668,-215.283283));
#231504=CARTESIAN_POINT('Ctrl Pts',(2482.70519332262,-2905.11442566293,
-215.216616));
#231505=CARTESIAN_POINT('Ctrl Pts',(2482.07712592294,-2900.99034725906,
-215.149949));
#231506=CARTESIAN_POINT('Ctrl Pts',(2409.6470640207,-7573.59735792804,-376.750757003348));
#231507=CARTESIAN_POINT('Ctrl Pts',(2259.57616502824,-6600.7059269267,-349.817289002703));
#231508=CARTESIAN_POINT('Ctrl Pts',(2109.5052660358,-5627.81449592536,-322.883821002058));
#231509=CARTESIAN_POINT('Ctrl Pts',(1959.43436704334,-4654.92306492402,
-295.950353001413));
#231510=CARTESIAN_POINT('Ctrl Pts',(1884.39891754712,-4168.47734942335,
-282.483619001091));
#231511=CARTESIAN_POINT('Ctrl Pts',(1809.36346805089,-3682.03163392268,
-269.016885000768));
#231512=CARTESIAN_POINT('Ctrl Pts',(1734.32801855467,-3195.58591842202,
-255.550151000446));
#231513=CARTESIAN_POINT('Ctrl Pts',(1696.81029380655,-2952.36306067169,
-248.816784000284));
#231514=CARTESIAN_POINT('Ctrl Pts',(1659.29256905844,-2709.14020292135,
-242.083417000122));
#231515=CARTESIAN_POINT('Ctrl Pts',(1621.77484431033,-2465.91734517101,
-235.35004999996));
#231516=CARTESIAN_POINT('Ctrl Pts',(1584.62858218348,-2225.10263452712,
-228.683349999799));
#231517=CARTESIAN_POINT('Ctrl Pts',(1547.87488224658,-1980.02600048826,
-222.01665));
#231518=CARTESIAN_POINT('Ctrl Pts',(1511.76562932734,-1730.72823380353,
-215.34995));
#231519=CARTESIAN_POINT('Ctrl Pts',(1511.40453679815,-1728.23525613669,
-215.283283));
#231520=CARTESIAN_POINT('Ctrl Pts',(1511.04344426897,-1725.74227846985,
-215.216616));
#231521=CARTESIAN_POINT('Ctrl Pts',(1510.68235173978,-1723.249300803,-215.149949));
#231522=CARTESIAN_POINT('Ctrl Pts',(1864.84799993008,-5906.11254116062,
-376.750757002601));
#231523=CARTESIAN_POINT('Ctrl Pts',(1751.66490845825,-5145.22127092072,
-349.8172890021));
#231524=CARTESIAN_POINT('Ctrl Pts',(1638.48181698641,-4384.33000068082,
-322.883821001599));
#231525=CARTESIAN_POINT('Ctrl Pts',(1525.29872551458,-3623.43873044092,
-295.950353001097));
#231526=CARTESIAN_POINT('Ctrl Pts',(1468.70717977866,-3242.99309532097,
-282.483619000847));
#231527=CARTESIAN_POINT('Ctrl Pts',(1412.11563404274,-2862.54746020102,
-269.016885000597));
#231528=CARTESIAN_POINT('Ctrl Pts',(1355.52408830682,-2482.10182508107,
-255.550151000346));
#231529=CARTESIAN_POINT('Ctrl Pts',(1327.22831543887,-2291.87900752109,
-248.816784000221));
#231530=CARTESIAN_POINT('Ctrl Pts',(1298.93254257091,-2101.65618996112,
-242.083417000095));
#231531=CARTESIAN_POINT('Ctrl Pts',(1270.63676970295,-1911.43337240115,
-235.350049999969));
#231532=CARTESIAN_POINT('Ctrl Pts',(1242.621153002,-1723.09394907444,-228.683349999844));
#231533=CARTESIAN_POINT('Ctrl Pts',(1214.91048696529,-1531.44452636515,
-222.01665));
#231534=CARTESIAN_POINT('Ctrl Pts',(1187.70039639579,-1336.51678424783,
-215.34995));
#231535=CARTESIAN_POINT('Ctrl Pts',(1187.4282954901,-1334.56750682665,-215.283283));
#231536=CARTESIAN_POINT('Ctrl Pts',(1187.15619458441,-1332.61822940548,
-215.216616));
#231537=CARTESIAN_POINT('Ctrl Pts',(1186.88409367872,-1330.66895198431,
-215.149949));
#231538=CARTESIAN_POINT('Ctrl Pts',(1320.04893583946,-4238.62772439321,
-376.750757001854));
#231539=CARTESIAN_POINT('Ctrl Pts',(1243.75365188824,-3689.73661491475,
-349.817289001497));
#231540=CARTESIAN_POINT('Ctrl Pts',(1167.45836793703,-3140.84550543629,
-322.883821001139));
#231541=CARTESIAN_POINT('Ctrl Pts',(1091.16308398581,-2591.95439595782,
-295.950353000782));
#231542=CARTESIAN_POINT('Ctrl Pts',(1053.0154420102,-2317.50884121858,-282.483619000604));
#231543=CARTESIAN_POINT('Ctrl Pts',(1014.86780003459,-2043.06328647936,
-269.016885000425));
#231544=CARTESIAN_POINT('Ctrl Pts',(976.720158058986,-1768.61773174013,
-255.550151000247));
#231545=CARTESIAN_POINT('Ctrl Pts',(957.646337071182,-1631.39495437051,
-248.816784000158));
#231546=CARTESIAN_POINT('Ctrl Pts',(938.572516083378,-1494.17217700089,
-242.083417000068));
#231547=CARTESIAN_POINT('Ctrl Pts',(919.498695095574,-1356.94939963128,
-235.350049999978));
#231548=CARTESIAN_POINT('Ctrl Pts',(900.61372382052,-1221.08526362176,-228.683349999889));
#231549=CARTESIAN_POINT('Ctrl Pts',(881.946091684011,-1082.86305224204,
-222.01665));
#231550=CARTESIAN_POINT('Ctrl Pts',(863.635163464249,-942.305334692116,
-215.34995));
#231551=CARTESIAN_POINT('Ctrl Pts',(863.452054182054,-940.899757516616,
-215.283283));
#231552=CARTESIAN_POINT('Ctrl Pts',(863.268944899859,-939.494180341118,
-215.216616));
#231553=CARTESIAN_POINT('Ctrl Pts',(863.085835617665,-938.088603165619,
-215.149949));
#231554=CARTESIAN_POINT('Ctrl Pts',(775.24987174884,-2571.1429076258,-376.750757001107));
#231555=CARTESIAN_POINT('Ctrl Pts',(735.842395318242,-2234.25195890877,
-349.817289000894));
#231556=CARTESIAN_POINT('Ctrl Pts',(696.434918887644,-1897.36101019174,
-322.883821000681));
#231557=CARTESIAN_POINT('Ctrl Pts',(657.027442457046,-1560.47006147472,
-295.950353000467));
#231558=CARTESIAN_POINT('Ctrl Pts',(637.323704241746,-1392.0245871162,-282.483619000361));
#231559=CARTESIAN_POINT('Ctrl Pts',(617.619966026447,-1223.57911275769,
-269.016885000254));
#231560=CARTESIAN_POINT('Ctrl Pts',(597.916227811148,-1055.13363839918,
-255.550151000147));
#231561=CARTESIAN_POINT('Ctrl Pts',(588.064358703498,-970.910901219922,
-248.816784000094));
#231562=CARTESIAN_POINT('Ctrl Pts',(578.212489595849,-886.688164040665,
-242.083417000041));
#231563=CARTESIAN_POINT('Ctrl Pts',(568.360620488199,-802.465426861409,
-235.350049999987));
#231564=CARTESIAN_POINT('Ctrl Pts',(558.606294639041,-719.076578169076,
-228.683349999934));
#231565=CARTESIAN_POINT('Ctrl Pts',(548.981696402727,-634.281578118933,
-222.01665));
#231566=CARTESIAN_POINT('Ctrl Pts',(539.569930532705,-548.093885136405,
-215.34995));
#231567=CARTESIAN_POINT('Ctrl Pts',(539.475812874006,-547.23200820658,-215.283283));
#231568=CARTESIAN_POINT('Ctrl Pts',(539.381695215308,-546.370131276755,
-215.216616));
#231569=CARTESIAN_POINT('Ctrl Pts',(539.287577556609,-545.50825434693,-215.149949));
#231570=CARTESIAN_POINT('Ctrl Pts',(593.650183718634,-2015.31463536999,
-376.750757000858));
#231571=CARTESIAN_POINT('Ctrl Pts',(566.538643128242,-1749.09040690678,
-349.817289000693));
#231572=CARTESIAN_POINT('Ctrl Pts',(539.427102537849,-1482.86617844356,
-322.883821000528));
#231573=CARTESIAN_POINT('Ctrl Pts',(512.315561947457,-1216.64194998035,
-295.950353000362));
#231574=CARTESIAN_POINT('Ctrl Pts',(498.759791652261,-1083.52983574874,
-282.48361900028));
#231575=CARTESIAN_POINT('Ctrl Pts',(485.204021357065,-950.417721517136,
-269.016885000197));
#231576=CARTESIAN_POINT('Ctrl Pts',(471.648251061869,-817.305607285529,
-255.550151000114));
#231577=CARTESIAN_POINT('Ctrl Pts',(464.87036591427,-750.749550169726,-248.816784000073));
#231578=CARTESIAN_POINT('Ctrl Pts',(458.092480766672,-684.193493053923,
-242.083417000031));
#231579=CARTESIAN_POINT('Ctrl Pts',(451.314595619074,-617.637435938119,
-235.35004999999));
#231580=CARTESIAN_POINT('Ctrl Pts',(444.603818245215,-551.740349684848,
-228.683349999949));
#231581=CARTESIAN_POINT('Ctrl Pts',(437.993564642299,-484.754420077896,
-222.01665));
#231582=CARTESIAN_POINT('Ctrl Pts',(431.54818622219,-416.690068617835,-215.34995));
#231583=CARTESIAN_POINT('Ctrl Pts',(431.48373243799,-416.009425103234,-215.283283));
#231584=CARTESIAN_POINT('Ctrl Pts',(431.419278653791,-415.328781588633,
-215.216616));
#231585=CARTESIAN_POINT('Ctrl Pts',(431.354824869591,-414.648138074033,
-215.149949));
#231586=CARTESIAN_POINT('Ctrl Pts',(412.050495688428,-1459.48636311419,
-376.750757000609));
#231587=CARTESIAN_POINT('Ctrl Pts',(397.234890938242,-1263.92885490479,
-349.817289000492));
#231588=CARTESIAN_POINT('Ctrl Pts',(382.419286188055,-1068.37134669538,
-322.883821000374));
#231589=CARTESIAN_POINT('Ctrl Pts',(367.603681437869,-872.813838485983,
-295.950353000257));
#231590=CARTESIAN_POINT('Ctrl Pts',(360.195879062775,-775.035084381282,
-282.483619000199));
#231591=CARTESIAN_POINT('Ctrl Pts',(352.788076687683,-677.256330276581,
-269.016885000139));
#231592=CARTESIAN_POINT('Ctrl Pts',(345.380274312589,-579.477576171881,
-255.550151000081));
#231593=CARTESIAN_POINT('Ctrl Pts',(341.676373125042,-530.58819911953,-248.816784000052));
#231594=CARTESIAN_POINT('Ctrl Pts',(337.972471937496,-481.69882206718,-242.083417000022));
#231595=CARTESIAN_POINT('Ctrl Pts',(334.26857074995,-432.80944501483,-235.350049999993));
#231596=CARTESIAN_POINT('Ctrl Pts',(330.601341851388,-384.404121200621,
-228.683349999963));
#231597=CARTESIAN_POINT('Ctrl Pts',(327.005432881871,-335.22726203686,-222.01665));
#231598=CARTESIAN_POINT('Ctrl Pts',(323.526441911676,-285.286252099265,
-215.34995));
#231599=CARTESIAN_POINT('Ctrl Pts',(323.491652001974,-284.786841999889,
-215.283283));
#231600=CARTESIAN_POINT('Ctrl Pts',(323.456862092273,-284.287431900513,
-215.216616));
#231601=CARTESIAN_POINT('Ctrl Pts',(323.422072182572,-283.788021801137,
-215.149949));
#231602=CARTESIAN_POINT('Ctrl Pts',(230.450807658222,-903.658090858384,
-376.75075700036));
#231603=CARTESIAN_POINT('Ctrl Pts',(227.931138748241,-778.767302902795,
-349.817289000291));
#231604=CARTESIAN_POINT('Ctrl Pts',(225.411469838261,-653.876514947205,
-322.883821000222));
#231605=CARTESIAN_POINT('Ctrl Pts',(222.891800928281,-528.985726991616,
-295.950353000152));
#231606=CARTESIAN_POINT('Ctrl Pts',(221.63196647329,-466.540333013821,-282.483619000117));
#231607=CARTESIAN_POINT('Ctrl Pts',(220.3721320183,-404.094939036027,-269.016885000082));
#231608=CARTESIAN_POINT('Ctrl Pts',(219.11229756331,-341.649545058231,-255.550151000048));
#231609=CARTESIAN_POINT('Ctrl Pts',(218.482380335815,-310.426848069334,
-248.816784000031));
#231610=CARTESIAN_POINT('Ctrl Pts',(217.85246310832,-279.204151080437,-242.083417000013));
#231611=CARTESIAN_POINT('Ctrl Pts',(217.222545880824,-247.981454091539,
-235.350049999996));
#231612=CARTESIAN_POINT('Ctrl Pts',(216.598865457562,-217.067892716394,
-228.683349999979));
#231613=CARTESIAN_POINT('Ctrl Pts',(216.017301121443,-185.700103995824,
-222.01665));
#231614=CARTESIAN_POINT('Ctrl Pts',(215.504697601161,-153.882435580695,
-215.34995));
#231615=CARTESIAN_POINT('Ctrl Pts',(215.499571565958,-153.564258896543,
-215.283283));
#231616=CARTESIAN_POINT('Ctrl Pts',(215.494445530756,-153.246082212392,
-215.216616));
#231617=CARTESIAN_POINT('Ctrl Pts',(215.489319495554,-152.92790552824,-215.149949));
#231618=CARTESIAN_POINT('Ctrl Pts',(169.91757831482,-718.38200010645,-376.750757000277));
#231619=CARTESIAN_POINT('Ctrl Pts',(171.496554684908,-617.046785568798,
-349.817289000224));
#231620=CARTESIAN_POINT('Ctrl Pts',(173.075531054996,-515.711571031146,
-322.883821000171));
#231621=CARTESIAN_POINT('Ctrl Pts',(174.654507425084,-414.376356493494,
-295.950353000117));
#231622=CARTESIAN_POINT('Ctrl Pts',(175.443995610129,-363.708749224667,
-282.48361900009));
#231623=CARTESIAN_POINT('Ctrl Pts',(176.233483795173,-313.041141955842,
-269.016885000063));
#231624=CARTESIAN_POINT('Ctrl Pts',(177.022971980217,-262.373534687016,
-255.550151000037));
#231625=CARTESIAN_POINT('Ctrl Pts',(177.417716072739,-237.039731052603,
-248.816784000024));
#231626=CARTESIAN_POINT('Ctrl Pts',(177.812460165261,-211.70592741819,-242.08341700001));
#231627=CARTESIAN_POINT('Ctrl Pts',(178.207204257783,-186.372123783777,
-235.350049999997));
#231628=CARTESIAN_POINT('Ctrl Pts',(178.598039992953,-161.289149888318,
-228.683349999984));
#231629=CARTESIAN_POINT('Ctrl Pts',(179.021257201301,-135.857717982145,
-222.01665));
#231630=CARTESIAN_POINT('Ctrl Pts',(179.497449497656,-110.081163407838,
-215.34995));
#231631=CARTESIAN_POINT('Ctrl Pts',(179.50221142062,-109.823397862094,-215.283283));
#231632=CARTESIAN_POINT('Ctrl Pts',(179.506973343583,-109.565632316351,
-215.216616));
#231633=CARTESIAN_POINT('Ctrl Pts',(179.511735266547,-109.307866770608,
-215.149949));
#231634=CARTESIAN_POINT('Ctrl Pts',(109.384348971418,-533.105909354515,
-376.750757000194));
#231635=CARTESIAN_POINT('Ctrl Pts',(115.061970621574,-455.3262682348,-349.817289000156));
#231636=CARTESIAN_POINT('Ctrl Pts',(120.739592271731,-377.546627115086,
-322.883821000119));
#231637=CARTESIAN_POINT('Ctrl Pts',(126.417213921888,-299.766985995371,
-295.950353000081));
#231638=CARTESIAN_POINT('Ctrl Pts',(129.256024746967,-260.877165435514,
-282.483619000063));
#231639=CARTESIAN_POINT('Ctrl Pts',(132.094835572045,-221.987344875657,
-269.016885000044));
#231640=CARTESIAN_POINT('Ctrl Pts',(134.933646397123,-183.097524315799,
-255.550151000025));
#231641=CARTESIAN_POINT('Ctrl Pts',(136.353051809663,-163.652614035871,
-248.816784000016));
#231642=CARTESIAN_POINT('Ctrl Pts',(137.772457222202,-144.207703755942,
-242.083417000007));
#231643=CARTESIAN_POINT('Ctrl Pts',(139.191862634741,-124.762793476013,
-235.350049999998));
#231644=CARTESIAN_POINT('Ctrl Pts',(140.597214528344,-105.510407060242,
-228.683349999989));
#231645=CARTESIAN_POINT('Ctrl Pts',(142.025213281158,-86.0153319684663,
-222.01665));
#231646=CARTESIAN_POINT('Ctrl Pts',(143.490201394151,-66.2798912349809,
-215.34995));
#231647=CARTESIAN_POINT('Ctrl Pts',(143.504851275281,-66.082536827646,-215.283283));
#231648=CARTESIAN_POINT('Ctrl Pts',(143.519501156411,-65.8851824203112,
-215.216616));
#231649=CARTESIAN_POINT('Ctrl Pts',(143.534151037541,-65.6878280129763,
-215.149949));
#231650=CARTESIAN_POINT('Ctrl Pts',(48.8511196280154,-347.82981860258,-376.750757000109));
#231651=CARTESIAN_POINT('Ctrl Pts',(58.6273865582409,-293.605750900803,
-349.817289000088));
#231652=CARTESIAN_POINT('Ctrl Pts',(68.4036534884664,-239.381683199026,
-322.883821000067));
#231653=CARTESIAN_POINT('Ctrl Pts',(78.179920418692,-185.157615497249,-295.950353000046));
#231654=CARTESIAN_POINT('Ctrl Pts',(83.0680538838047,-158.04558164636,-282.483619000036));
#231655=CARTESIAN_POINT('Ctrl Pts',(87.9561873489175,-130.933547795471,
-269.016885000025));
#231656=CARTESIAN_POINT('Ctrl Pts',(92.8443208140303,-103.821513944583,
-255.550151000015));
#231657=CARTESIAN_POINT('Ctrl Pts',(95.2883875465867,-90.2654970191385,
-248.816784000009));
#231658=CARTESIAN_POINT('Ctrl Pts',(97.7324542791431,-76.7094800936942,
-242.083417000004));
#231659=CARTESIAN_POINT('Ctrl Pts',(100.176521011699,-63.1534631682499,
-235.350049999999));
#231660=CARTESIAN_POINT('Ctrl Pts',(102.596389063735,-49.7316642321664,
-228.683349999994));
#231661=CARTESIAN_POINT('Ctrl Pts',(105.029169361015,-36.1729459547875,
-222.01665));
#231662=CARTESIAN_POINT('Ctrl Pts',(107.482953290646,-22.4786190621241,
-215.34995));
#231663=CARTESIAN_POINT('Ctrl Pts',(107.507491129942,-22.3416757931975,
-215.283283));
#231664=CARTESIAN_POINT('Ctrl Pts',(107.532028969239,-22.2047325242709,
-215.216616));
#231665=CARTESIAN_POINT('Ctrl Pts',(107.556566808535,-22.0677892553443,
-215.149949));
#231666=CARTESIAN_POINT('Ctrl Pts',(28.673376513548,-286.071121685269,-376.750757000082));
#231667=CARTESIAN_POINT('Ctrl Pts',(39.8158585371298,-239.698911789471,
-349.817289000066));
#231668=CARTESIAN_POINT('Ctrl Pts',(50.9583405607115,-193.326701893672,
-322.88382100005));
#231669=CARTESIAN_POINT('Ctrl Pts',(62.1008225842933,-146.954491997874,
-295.950353000034));
#231670=CARTESIAN_POINT('Ctrl Pts',(67.6720635960841,-123.768387049975,
-282.483619000027));
#231671=CARTESIAN_POINT('Ctrl Pts',(73.243304607875,-100.582282102076,-269.016885000018));
#231672=CARTESIAN_POINT('Ctrl Pts',(78.8145456196659,-77.3961771541774,
-255.550151000011));
#231673=CARTESIAN_POINT('Ctrl Pts',(81.6001661255613,-65.8031246802278,
-248.816784000007));
#231674=CARTESIAN_POINT('Ctrl Pts',(84.3857866314568,-54.2100722062783,
-242.083417000003));
#231675=CARTESIAN_POINT('Ctrl Pts',(87.1714071373522,-42.6170197323288,
-235.350049999999));
#231676=CARTESIAN_POINT('Ctrl Pts',(89.9294472421992,-31.1387499561412,
-228.683349999995));
#231677=CARTESIAN_POINT('Ctrl Pts',(92.6971547209677,-19.5588172835613,
-222.01665));
#231678=CARTESIAN_POINT('Ctrl Pts',(95.4805372561441,-7.8781950045052,-215.34995));
#231679=CARTESIAN_POINT('Ctrl Pts',(95.508371081496,-7.76138878171465,-215.283283));
#231680=CARTESIAN_POINT('Ctrl Pts',(95.5362049068479,-7.64458255892409,
-215.216616));
#231681=CARTESIAN_POINT('Ctrl Pts',(95.5640387321998,-7.52777633613354,
-215.149949));
#231682=CARTESIAN_POINT('Ctrl Pts',(8.49563339908065,-224.312424767957,
-376.750757000054));
#231683=CARTESIAN_POINT('Ctrl Pts',(21.0043305160186,-185.792072678138,
-349.817289000044));
#231684=CARTESIAN_POINT('Ctrl Pts',(33.5130276329566,-147.271720588319,
-322.883821000033));
#231685=CARTESIAN_POINT('Ctrl Pts',(46.0217247498946,-108.7513684985,-295.950353000022));
#231686=CARTESIAN_POINT('Ctrl Pts',(52.2760733083635,-89.4911924535907,
-282.483619000017));
#231687=CARTESIAN_POINT('Ctrl Pts',(58.5304218668325,-70.2310164086813,
-269.016885000012));
#231688=CARTESIAN_POINT('Ctrl Pts',(64.7847704253015,-50.9708403637719,
-255.550151000007));
#231689=CARTESIAN_POINT('Ctrl Pts',(67.911944704536,-41.3407523413171,-248.816784000005));
#231690=CARTESIAN_POINT('Ctrl Pts',(71.0391189837705,-31.7106643188625,
-242.083417000002));
#231691=CARTESIAN_POINT('Ctrl Pts',(74.166293263005,-22.0805762964077,-235.35005));
#231692=CARTESIAN_POINT('Ctrl Pts',(77.2625054206629,-12.5458356801159,
-228.683349999997));
#231693=CARTESIAN_POINT('Ctrl Pts',(80.3651400809202,-2.94468861233498,
-222.01665));
#231694=CARTESIAN_POINT('Ctrl Pts',(83.4781212216425,6.72222905311371,-215.34995));
#231695=CARTESIAN_POINT('Ctrl Pts',(83.5092510330498,6.81889822976819,-215.283283));
#231696=CARTESIAN_POINT('Ctrl Pts',(83.5403808444571,6.91556740642268,-215.216616));
#231697=CARTESIAN_POINT('Ctrl Pts',(83.5715106558644,7.01223658307716,-215.149949));
#231698=CARTESIAN_POINT('Ctrl Pts',(-11.6821097153867,-162.553727850645,
-376.750757000025));
#231699=CARTESIAN_POINT('Ctrl Pts',(2.1928024949075,-131.885233566805,-349.81728900002));
#231700=CARTESIAN_POINT('Ctrl Pts',(16.0677147052017,-101.216739282966,
-322.883821000016));
#231701=CARTESIAN_POINT('Ctrl Pts',(29.9426269154959,-70.548244999126,-295.95035300001));
#231702=CARTESIAN_POINT('Ctrl Pts',(36.880083020643,-55.2139978572062,-282.483619000008));
#231703=CARTESIAN_POINT('Ctrl Pts',(43.81753912579,-39.8797507152863,-269.016885000005));
#231704=CARTESIAN_POINT('Ctrl Pts',(50.7549952309371,-24.5455035733664,
-255.550151000003));
#231705=CARTESIAN_POINT('Ctrl Pts',(54.2237232835107,-16.8783800024065,
-248.816784000002));
#231706=CARTESIAN_POINT('Ctrl Pts',(57.6924513360842,-9.21125643144658,
-242.083417000001));
#231707=CARTESIAN_POINT('Ctrl Pts',(61.1611793886578,-1.54413286048666,
-235.35005));
#231708=CARTESIAN_POINT('Ctrl Pts',(64.5955635991267,6.04707859590932,-228.683349999999));
#231709=CARTESIAN_POINT('Ctrl Pts',(68.0331254408726,13.6694400588913,-222.01665));
#231710=CARTESIAN_POINT('Ctrl Pts',(71.4757051871408,21.3226531107326,-215.34995));
#231711=CARTESIAN_POINT('Ctrl Pts',(71.5101309846035,21.3991852412511,-215.283283));
#231712=CARTESIAN_POINT('Ctrl Pts',(71.5445567820663,21.4757173717695,-215.216616));
#231713=CARTESIAN_POINT('Ctrl Pts',(71.578982579529,21.5522495022879,-215.149949));
#231714=CARTESIAN_POINT('Ctrl Pts',(-18.4080240868758,-141.967495544875,
-376.750757000016));
#231715=CARTESIAN_POINT('Ctrl Pts',(-4.07770684546288,-113.916287196361,
-349.817289000013));
#231716=CARTESIAN_POINT('Ctrl Pts',(10.25261039595,-85.865078847848,-322.88382100001));
#231717=CARTESIAN_POINT('Ctrl Pts',(24.582927637363,-57.8138704993346,-295.950353000006));
#231718=CARTESIAN_POINT('Ctrl Pts',(31.7480862580694,-43.7882663250779,
-282.483619000005));
#231719=CARTESIAN_POINT('Ctrl Pts',(38.9132448787759,-29.7626621508213,
-269.016885000003));
#231720=CARTESIAN_POINT('Ctrl Pts',(46.0784034994824,-15.7370579765646,
-255.550151000002));
#231721=CARTESIAN_POINT('Ctrl Pts',(49.6609828098356,-8.72425588943629,
-248.816784000002));
#231722=CARTESIAN_POINT('Ctrl Pts',(53.2435621201888,-1.71145380230796,
-242.083417000001));
#231723=CARTESIAN_POINT('Ctrl Pts',(56.826141430542,5.30134828482038,-235.35005));
#231724=CARTESIAN_POINT('Ctrl Pts',(60.3732496586146,12.2447166879177,-228.683349999999));
#231725=CARTESIAN_POINT('Ctrl Pts',(63.9224538941901,19.2074829493001,-222.01665));
#231726=CARTESIAN_POINT('Ctrl Pts',(67.4748998423069,26.1894611299389,-215.34995));
#231727=CARTESIAN_POINT('Ctrl Pts',(67.5104243017881,26.2592809117453,-215.283283));
#231728=CARTESIAN_POINT('Ctrl Pts',(67.5459487612693,26.3291006935517,-215.216616));
#231729=CARTESIAN_POINT('Ctrl Pts',(67.5814732207505,26.3989204753581,-215.149949));
#231730=CARTESIAN_POINT('Ctrl Pts',(-25.1339384583649,-121.381263239104,
-376.750757000007));
#231731=CARTESIAN_POINT('Ctrl Pts',(-10.3482161858333,-95.9473408259171,
-349.817289000005));
#231732=CARTESIAN_POINT('Ctrl Pts',(4.4375060866984,-70.5134184127302,-322.883821000004));
#231733=CARTESIAN_POINT('Ctrl Pts',(19.22322835923,-45.0794959995432,-295.950353000003));
#231734=CARTESIAN_POINT('Ctrl Pts',(26.6160894954959,-32.3625347929498,
-282.483619000002));
#231735=CARTESIAN_POINT('Ctrl Pts',(34.0089506317617,-19.6455735863562,
-269.016885000001));
#231736=CARTESIAN_POINT('Ctrl Pts',(41.4018117680275,-6.9286123797628,-255.550151000001));
#231737=CARTESIAN_POINT('Ctrl Pts',(45.0982423361605,-0.570131776466063,
-248.816784000001));
#231738=CARTESIAN_POINT('Ctrl Pts',(48.7946729042934,5.78834882683067,-242.083417));
#231739=CARTESIAN_POINT('Ctrl Pts',(52.4911034724263,12.1468294301274,-235.35005));
#231740=CARTESIAN_POINT('Ctrl Pts',(56.1509357181025,18.4423547799261,-228.68335));
#231741=CARTESIAN_POINT('Ctrl Pts',(59.8117823475076,24.7455258397088,-222.01665));
#231742=CARTESIAN_POINT('Ctrl Pts',(63.4740944974731,31.0562691491453,-215.34995));
#231743=CARTESIAN_POINT('Ctrl Pts',(63.5107176189727,31.1193765822396,-215.283283));
#231744=CARTESIAN_POINT('Ctrl Pts',(63.5473407404724,31.1824840153339,-215.216616));
#231745=CARTESIAN_POINT('Ctrl Pts',(63.5839638619721,31.2455914484283,-215.149949));
#231746=CARTESIAN_POINT('Ctrl Pts',(-31.859852829854,-100.795030933333,
-376.750756999998));
#231747=CARTESIAN_POINT('Ctrl Pts',(-16.6187255262036,-77.9783944554729,
-349.817288999998));
#231748=CARTESIAN_POINT('Ctrl Pts',(-1.37759822255324,-55.1617579776124,
-322.883820999999));
#231749=CARTESIAN_POINT('Ctrl Pts',(13.8635290810972,-32.3451214997519,
-295.950352999999));
#231750=CARTESIAN_POINT('Ctrl Pts',(21.4840927329223,-20.9368032608216,
-282.483618999999));
#231751=CARTESIAN_POINT('Ctrl Pts',(29.1046563847475,-9.52848502189127,
-269.016885));
#231752=CARTESIAN_POINT('Ctrl Pts',(36.7252200365728,1.87983321703902,-255.550151));
#231753=CARTESIAN_POINT('Ctrl Pts',(40.5355018624854,7.58399233650416,-248.816784));
#231754=CARTESIAN_POINT('Ctrl Pts',(44.345783688398,13.2881514559693,-242.083417));
#231755=CARTESIAN_POINT('Ctrl Pts',(48.1560655143106,18.9923105754345,-235.35005));
#231756=CARTESIAN_POINT('Ctrl Pts',(51.9286217775904,24.6399928719346,-228.68335));
#231757=CARTESIAN_POINT('Ctrl Pts',(55.7011108008251,30.2835687301176,-222.01665));
#231758=CARTESIAN_POINT('Ctrl Pts',(59.4732891526392,35.9230771683515,-215.34995));
#231759=CARTESIAN_POINT('Ctrl Pts',(59.5110109361573,35.9794722527339,-215.283283));
#231760=CARTESIAN_POINT('Ctrl Pts',(59.5487327196755,36.0358673371162,-215.216616));
#231761=CARTESIAN_POINT('Ctrl Pts',(59.5864545031936,36.0922624214986,-215.149949));
#231762=CARTESIAN_POINT('Ctrl Pts',(-33.5413314227263,-95.6484728568909,
-376.750756999995));
#231763=CARTESIAN_POINT('Ctrl Pts',(-18.1863528612963,-73.4861578628619,
-349.817288999997));
#231764=CARTESIAN_POINT('Ctrl Pts',(-2.83137429986615,-51.3238428688329,
-322.883820999997));
#231765=CARTESIAN_POINT('Ctrl Pts',(12.5236042615639,-29.161527874804,-295.950352999998));
#231766=CARTESIAN_POINT('Ctrl Pts',(20.201093542279,-18.0803703777895,-282.483618999998));
#231767=CARTESIAN_POINT('Ctrl Pts',(27.878582822994,-6.99921288077501,-269.016884999999));
#231768=CARTESIAN_POINT('Ctrl Pts',(35.556072103709,4.08194461623947,-255.550151));
#231769=CARTESIAN_POINT('Ctrl Pts',(39.3948167440666,9.62252336474671,-248.816784));
#231770=CARTESIAN_POINT('Ctrl Pts',(43.2335613844241,15.163102113254,-242.083417));
#231771=CARTESIAN_POINT('Ctrl Pts',(47.0723060247816,20.7036808617612,-235.35005));
#231772=CARTESIAN_POINT('Ctrl Pts',(50.8730432924624,26.1894023949367,-228.683350000001));
#231773=CARTESIAN_POINT('Ctrl Pts',(54.6734429141545,31.6680794527198,-222.01665));
#231774=CARTESIAN_POINT('Ctrl Pts',(58.4730878164307,37.1397791731531,-215.34995));
#231775=CARTESIAN_POINT('Ctrl Pts',(58.5110842654535,37.1944961703575,-215.283283));
#231776=CARTESIAN_POINT('Ctrl Pts',(58.5490807144762,37.2492131675618,-215.216616));
#231777=CARTESIAN_POINT('Ctrl Pts',(58.587077163499,37.3039301647661,-215.149949));
#231778=CARTESIAN_POINT('Ctrl Pts',(-41.2301579830855,-81.5182387771612,
-376.750756999989));
#231779=CARTESIAN_POINT('Ctrl Pts',(-24.8836555508694,-61.3775485896441,
-349.817288999991));
#231780=CARTESIAN_POINT('Ctrl Pts',(-8.53715311865333,-41.2368584021269,
-322.883820999993));
#231781=CARTESIAN_POINT('Ctrl Pts',(7.80934931356275,-21.0961682146096,
-295.950352999996));
#231782=CARTESIAN_POINT('Ctrl Pts',(15.9826005296708,-11.025823120851,-282.483618999996));
#231783=CARTESIAN_POINT('Ctrl Pts',(24.1558517457789,-0.955478027092413,
-269.016884999998));
#231784=CARTESIAN_POINT('Ctrl Pts',(32.3291029618869,9.1148670666662,-255.550150999998));
#231785=CARTESIAN_POINT('Ctrl Pts',(36.4157285699409,14.1500396135455,-248.816783999999));
#231786=CARTESIAN_POINT('Ctrl Pts',(40.5023541779949,19.1852121604248,-242.083416999999));
#231787=CARTESIAN_POINT('Ctrl Pts',(44.588979786049,24.2203847073041,-235.35005));
#231788=CARTESIAN_POINT('Ctrl Pts',(48.6351437544193,29.2057040606499,-228.683350000001));
#231789=CARTESIAN_POINT('Ctrl Pts',(52.6799616741893,34.1756765917424,-222.01665));
#231790=CARTESIAN_POINT('Ctrl Pts',(56.7225263698862,39.1304491224114,-215.34995));
#231791=CARTESIAN_POINT('Ctrl Pts',(56.7629520168432,39.1799968477181,-215.283283));
#231792=CARTESIAN_POINT('Ctrl Pts',(56.8033776638002,39.2295445730248,-215.216616));
#231793=CARTESIAN_POINT('Ctrl Pts',(56.8438033107571,39.2790922983315,-215.149949));
#231794=CARTESIAN_POINT('Ctrl Pts',(-61.5202391452974,-58.1759617860395,
-376.750756999982));
#231795=CARTESIAN_POINT('Ctrl Pts',(-42.2054487986876,-41.4892341751692,
-349.817288999985));
#231796=CARTESIAN_POINT('Ctrl Pts',(-22.8906584520777,-24.8025065642989,
-322.883820999989));
#231797=CARTESIAN_POINT('Ctrl Pts',(-3.5758681054679,-8.11577895342853,
-295.950352999993));
#231798=CARTESIAN_POINT('Ctrl Pts',(6.08152706783702,0.227584852006628,
-282.483618999994));
#231799=CARTESIAN_POINT('Ctrl Pts',(15.738922241142,8.57094865744179,-269.016884999996));
#231800=CARTESIAN_POINT('Ctrl Pts',(25.3963174144469,16.9143124628769,-255.550150999997));
#231801=CARTESIAN_POINT('Ctrl Pts',(30.2250150010993,21.0859943655945,-248.816783999999));
#231802=CARTESIAN_POINT('Ctrl Pts',(35.0537125877518,25.2576762683121,-242.083416999999));
#231803=CARTESIAN_POINT('Ctrl Pts',(39.8824101744042,29.4293581710297,-235.35005));
#231804=CARTESIAN_POINT('Ctrl Pts',(44.6632988740601,33.5597362925323,-228.683350000001));
#231805=CARTESIAN_POINT('Ctrl Pts',(49.4410603210161,37.6624224459266,-222.01665));
#231806=CARTESIAN_POINT('Ctrl Pts',(54.214059251162,41.7376821955923,-215.34995));
#231807=CARTESIAN_POINT('Ctrl Pts',(54.2617892404634,41.778434793089,-215.283283));
#231808=CARTESIAN_POINT('Ctrl Pts',(54.3095192297649,41.8191873905857,-215.216616));
#231809=CARTESIAN_POINT('Ctrl Pts',(54.3572492190663,41.8599399880823,-215.149949));
#231810=CARTESIAN_POINT('Ctrl Pts',(-86.4308715045652,-38.5465561709931,
-376.75075699998));
#231811=CARTESIAN_POINT('Ctrl Pts',(-63.394599877538,-24.7210691437011,
-349.817288999984));
#231812=CARTESIAN_POINT('Ctrl Pts',(-40.3583282505107,-10.8955821164091,
-322.883820999988));
#231813=CARTESIAN_POINT('Ctrl Pts',(-17.3220566234834,2.92990491088294,
-295.950352999991));
#231814=CARTESIAN_POINT('Ctrl Pts',(-5.80392080996978,9.84264842452895,
-282.483618999993));
#231815=CARTESIAN_POINT('Ctrl Pts',(5.71421500354386,16.755391938175,-269.016884999996));
#231816=CARTESIAN_POINT('Ctrl Pts',(17.2323508170575,23.668135451821,-255.550150999997));
#231817=CARTESIAN_POINT('Ctrl Pts',(22.9914187238143,27.1245072086439,-248.816783999998));
#231818=CARTESIAN_POINT('Ctrl Pts',(28.7504866305711,30.580878965467,-242.083416999999));
#231819=CARTESIAN_POINT('Ctrl Pts',(34.509554537328,34.03725072229,-235.35005));
#231820=CARTESIAN_POINT('Ctrl Pts',(40.2116019697604,37.4594009765702,-228.683350000001));
#231821=CARTESIAN_POINT('Ctrl Pts',(45.9096065172025,40.8490096838924,-222.01665));
#231822=CARTESIAN_POINT('Ctrl Pts',(51.6016474095961,44.2063892516083,-215.34995));
#231823=CARTESIAN_POINT('Ctrl Pts',(51.65856781852,44.2399630472854,-215.283283));
#231824=CARTESIAN_POINT('Ctrl Pts',(51.715488227444,44.2735368429626,-215.216616));
#231825=CARTESIAN_POINT('Ctrl Pts',(51.7724086363679,44.3071106386397,-215.149949));
#231826=CARTESIAN_POINT('Ctrl Pts',(-101.966904434915,-30.8346247983327,
-376.750756999984));
#231827=CARTESIAN_POINT('Ctrl Pts',(-76.6679969066201,-18.0147641121609,
-349.817288999987));
#231828=CARTESIAN_POINT('Ctrl Pts',(-51.3690893783256,-5.19490342598898,
-322.88382099999));
#231829=CARTESIAN_POINT('Ctrl Pts',(-26.070181850031,7.62495726018286,-295.950352999994));
#231830=CARTESIAN_POINT('Ctrl Pts',(-13.4207280858838,14.0348876032688,
-282.483618999995));
#231831=CARTESIAN_POINT('Ctrl Pts',(-0.771274321736487,20.4448179463547,
-269.016884999996));
#231832=CARTESIAN_POINT('Ctrl Pts',(11.8781794424108,26.8547482894406,-255.550150999998));
#231833=CARTESIAN_POINT('Ctrl Pts',(18.2029063244844,30.0597134609836,-248.816783999999));
#231834=CARTESIAN_POINT('Ctrl Pts',(24.5276332065581,33.2646786325266,-242.083416999999));
#231835=CARTESIAN_POINT('Ctrl Pts',(30.8523600886317,36.4696438040695,-235.35005));
#231836=CARTESIAN_POINT('Ctrl Pts',(37.1144659124669,39.6428766471814,-228.683350000001));
#231837=CARTESIAN_POINT('Ctrl Pts',(43.3732515923186,42.7902567304839,-222.01665));
#231838=CARTESIAN_POINT('Ctrl Pts',(49.6271914214616,45.9120323459617,-215.34995));
#231839=CARTESIAN_POINT('Ctrl Pts',(49.6897308197531,45.9432501021165,-215.283283));
#231840=CARTESIAN_POINT('Ctrl Pts',(49.7522702180445,45.9744678582713,-215.216616));
#231841=CARTESIAN_POINT('Ctrl Pts',(49.8148096163359,46.005685614426,-215.149949));
#231842=CARTESIAN_POINT('Ctrl Pts',(-107.993804890233,-28.9044482397935,
-376.750756999988));
#231843=CARTESIAN_POINT('Ctrl Pts',(-81.8862252383193,-16.2510537069498,
-349.81728899999));
#231844=CARTESIAN_POINT('Ctrl Pts',(-55.7786455864053,-3.5976591741061,
-322.883820999992));
#231845=CARTESIAN_POINT('Ctrl Pts',(-29.6710659344913,9.05573535873763,
-295.950352999994));
#231846=CARTESIAN_POINT('Ctrl Pts',(-16.6172761085343,15.3824326251595,
-282.483618999996));
#231847=CARTESIAN_POINT('Ctrl Pts',(-3.5634862825773,21.7091298915814,-269.016884999997));
#231848=CARTESIAN_POINT('Ctrl Pts',(9.49030354337971,28.0358271580032,-255.550150999998));
#231849=CARTESIAN_POINT('Ctrl Pts',(16.0171984563582,31.1991757912142,-248.816783999999));
#231850=CARTESIAN_POINT('Ctrl Pts',(22.5440933693367,34.3625244244251,-242.083416999999));
#231851=CARTESIAN_POINT('Ctrl Pts',(29.0709882823152,37.525873057636,-235.35005));
#231852=CARTESIAN_POINT('Ctrl Pts',(35.5332604733831,40.6579014073498,-228.683350000001));
#231853=CARTESIAN_POINT('Ctrl Pts',(41.9930962102693,43.771133049519,-222.01665));
#231854=CARTESIAN_POINT('Ctrl Pts',(48.4493862544499,46.8657485296993,-215.34995));
#231855=CARTESIAN_POINT('Ctrl Pts',(48.5139491548917,46.8966946845011,-215.283283));
#231856=CARTESIAN_POINT('Ctrl Pts',(48.5785120553335,46.9276408393029,-215.216616));
#231857=CARTESIAN_POINT('Ctrl Pts',(48.6430749557753,46.9585869941047,-215.149949));
#231858=CARTESIAN_POINT('Ctrl Pts',(-132.101406711508,-21.1837420056372,
-376.750756999997));
#231859=CARTESIAN_POINT('Ctrl Pts',(-102.759138565116,-9.1962120861059,
-349.817288999997));
#231860=CARTESIAN_POINT('Ctrl Pts',(-73.4168704187245,2.79131783342537,
-322.883820999998));
#231861=CARTESIAN_POINT('Ctrl Pts',(-44.0746022723325,14.7788477529567,
-295.950352999998));
#231862=CARTESIAN_POINT('Ctrl Pts',(-29.4034681991366,20.7726127127223,
-282.483618999999));
#231863=CARTESIAN_POINT('Ctrl Pts',(-14.7323341259406,26.766377672488,-269.016884999999));
#231864=CARTESIAN_POINT('Ctrl Pts',(-0.0612000527446133,32.7601426322536,
-255.550151));
#231865=CARTESIAN_POINT('Ctrl Pts',(7.27436698385337,35.7570251121364,-248.816784));
#231866=CARTESIAN_POINT('Ctrl Pts',(14.6099340204513,38.7539075920192,-242.083417));
#231867=CARTESIAN_POINT('Ctrl Pts',(21.9455010570494,41.7507900719021,-235.35005));
#231868=CARTESIAN_POINT('Ctrl Pts',(29.2084387170473,44.7180004480236,-228.68335));
#231869=CARTESIAN_POINT('Ctrl Pts',(36.4724746820719,47.694638325659,-222.016650000001));
#231870=CARTESIAN_POINT('Ctrl Pts',(43.7381655864028,50.6806132646498,-215.34995));
#231871=CARTESIAN_POINT('Ctrl Pts',(43.810822495446,50.7104730140397,-215.283283));
#231872=CARTESIAN_POINT('Ctrl Pts',(43.8834794044894,50.7403327634296,-215.216616));
#231873=CARTESIAN_POINT('Ctrl Pts',(43.9561363135327,50.7701925128195,-215.149949));
#231874=CARTESIAN_POINT('Ctrl Pts',(-156.209008532784,-13.4630357714808,
-376.750757000006));
#231875=CARTESIAN_POINT('Ctrl Pts',(-123.632051891913,-2.14137046526198,
-349.817289000005));
#231876=CARTESIAN_POINT('Ctrl Pts',(-91.0550952510435,9.18029484095685,
-322.883821000004));
#231877=CARTESIAN_POINT('Ctrl Pts',(-58.4781386101737,20.5019601471757,
-295.950353000003));
#231878=CARTESIAN_POINT('Ctrl Pts',(-42.1896602897388,26.1627928002851,
-282.483619000002));
#231879=CARTESIAN_POINT('Ctrl Pts',(-25.9011819693039,31.8236254533946,
-269.016885000001));
#231880=CARTESIAN_POINT('Ctrl Pts',(-9.61270364886893,37.484458106504,-255.550151000001));
#231881=CARTESIAN_POINT('Ctrl Pts',(-1.46846448865147,40.3148744330587,
-248.816784000001));
#231882=CARTESIAN_POINT('Ctrl Pts',(6.67577467156599,43.1452907596133,-242.083417));
#231883=CARTESIAN_POINT('Ctrl Pts',(14.8200138317834,45.9757070861681,-235.35005));
#231884=CARTESIAN_POINT('Ctrl Pts',(22.8836169607117,48.7780994886975,-228.68335));
#231885=CARTESIAN_POINT('Ctrl Pts',(30.9518531538746,51.6181436017991,-222.016650000001));
#231886=CARTESIAN_POINT('Ctrl Pts',(39.0269449183556,54.4954779996004,-215.349950000001));
#231887=CARTESIAN_POINT('Ctrl Pts',(39.1076958360005,54.5242513435783,-215.283283000001));
#231888=CARTESIAN_POINT('Ctrl Pts',(39.1884467536454,54.5530246875563,-215.216616));
#231889=CARTESIAN_POINT('Ctrl Pts',(39.2691976712902,54.5817980315343,-215.149949000001));
#231890=CARTESIAN_POINT('Ctrl Pts',(-180.316610354058,-5.74232953732446,
-376.750757000015));
#231891=CARTESIAN_POINT('Ctrl Pts',(-144.50496521871,4.91347115558193,-349.817289000013));
#231892=CARTESIAN_POINT('Ctrl Pts',(-108.693320083363,15.5692718484884,
-322.88382100001));
#231893=CARTESIAN_POINT('Ctrl Pts',(-72.8816749480149,26.2250725413947,
-295.950353000006));
#231894=CARTESIAN_POINT('Ctrl Pts',(-54.975852380341,31.5529728878479,-282.483619000005));
#231895=CARTESIAN_POINT('Ctrl Pts',(-37.0700298126672,36.8808732343011,
-269.016885000003));
#231896=CARTESIAN_POINT('Ctrl Pts',(-19.1642072449932,42.2087735807543,
-255.550151000002));
#231897=CARTESIAN_POINT('Ctrl Pts',(-10.2112959611563,44.8727237539809,
-248.816784000002));
#231898=CARTESIAN_POINT('Ctrl Pts',(-1.25838467731937,47.5366739272075,
-242.083417000001));
#231899=CARTESIAN_POINT('Ctrl Pts',(7.69452660651757,50.2006241004341,-235.35005));
#231900=CARTESIAN_POINT('Ctrl Pts',(16.558795204376,52.8381985293713,-228.68335));
#231901=CARTESIAN_POINT('Ctrl Pts',(25.4312316256772,55.5416488779391,-222.016650000001));
#231902=CARTESIAN_POINT('Ctrl Pts',(34.3157242503085,58.3103427345509,-215.349950000001));
#231903=CARTESIAN_POINT('Ctrl Pts',(34.4045691765549,58.3380296731169,-215.283283000001));
#231904=CARTESIAN_POINT('Ctrl Pts',(34.4934141028013,58.365716611683,-215.216616));
#231905=CARTESIAN_POINT('Ctrl Pts',(34.5822590290476,58.3934035502491,-215.149949000001));
#231906=CARTESIAN_POINT('Ctrl Pts',(-252.639415817883,17.4197891651448,
-376.750757000044));
#231907=CARTESIAN_POINT('Ctrl Pts',(-207.123705199102,26.0779960181138,
-349.817289000036));
#231908=CARTESIAN_POINT('Ctrl Pts',(-161.60799458032,34.7362028710828,-322.883821000027));
#231909=CARTESIAN_POINT('Ctrl Pts',(-116.092283961538,43.3944097240518,
-295.950353000018));
#231910=CARTESIAN_POINT('Ctrl Pts',(-93.3344286521477,47.7235131505364,
-282.483619000015));
#231911=CARTESIAN_POINT('Ctrl Pts',(-70.576573342757,52.0526165770209,-269.01688500001));
#231912=CARTESIAN_POINT('Ctrl Pts',(-47.8187180333662,56.3817200035054,
-255.550151000006));
#231913=CARTESIAN_POINT('Ctrl Pts',(-36.4397903786708,58.5462717167477,
-248.816784000004));
#231914=CARTESIAN_POINT('Ctrl Pts',(-25.0608627239755,60.7108234299899,
-242.083417000002));
#231915=CARTESIAN_POINT('Ctrl Pts',(-13.6819350692801,62.8753751432322,
-235.35005));
#231916=CARTESIAN_POINT('Ctrl Pts',(-2.41567006463117,65.0184956513928,
-228.683349999998));
#231917=CARTESIAN_POINT('Ctrl Pts',(8.86936704108513,67.3121647063593,-222.016650000002));
#231918=CARTESIAN_POINT('Ctrl Pts',(20.1820622461672,69.7549369394024,-215.349950000001));
#231919=CARTESIAN_POINT('Ctrl Pts',(20.2951891982182,69.7793646617328,-215.283283000001));
#231920=CARTESIAN_POINT('Ctrl Pts',(20.4083161502691,69.8037923840631,-215.216616));
#231921=CARTESIAN_POINT('Ctrl Pts',(20.5214431023201,69.8282201063935,-215.149949000001));
#231922=CARTESIAN_POINT('Ctrl Pts',(-324.962221281708,40.581907867614,-376.750757000072));
#231923=CARTESIAN_POINT('Ctrl Pts',(-269.742445179492,47.2425208806457,
-349.817289000059));
#231924=CARTESIAN_POINT('Ctrl Pts',(-214.522669077277,53.9031338936774,
-322.883821000045));
#231925=CARTESIAN_POINT('Ctrl Pts',(-159.302892975062,60.563746906709,-295.950353000031));
#231926=CARTESIAN_POINT('Ctrl Pts',(-131.693004923954,63.8940534132249,
-282.483619000024));
#231927=CARTESIAN_POINT('Ctrl Pts',(-104.083116872847,67.2243599197407,
-269.016885000017));
#231928=CARTESIAN_POINT('Ctrl Pts',(-76.4732288217392,70.5546664262565,
-255.55015100001));
#231929=CARTESIAN_POINT('Ctrl Pts',(-62.6682847961853,72.2198196795144,
-248.816784000007));
#231930=CARTESIAN_POINT('Ctrl Pts',(-48.8633407706315,73.8849729327724,
-242.083417000003));
#231931=CARTESIAN_POINT('Ctrl Pts',(-35.0583967450777,75.5501261860303,
-235.35005));
#231932=CARTESIAN_POINT('Ctrl Pts',(-21.3901353336382,77.1987927734144,
-228.683349999997));
#231933=CARTESIAN_POINT('Ctrl Pts',(-7.69249754350693,79.0826805347794,
-222.016650000002));
#231934=CARTESIAN_POINT('Ctrl Pts',(6.0484002420259,81.199531144254,-215.349950000001));
#231935=CARTESIAN_POINT('Ctrl Pts',(6.18580921988141,81.2206996503486,-215.283283000001));
#231936=CARTESIAN_POINT('Ctrl Pts',(6.32321819773692,81.2418681564432,-215.216616000001));
#231937=CARTESIAN_POINT('Ctrl Pts',(6.46062717559243,81.2630366625378,-215.149949000001));
#231938=CARTESIAN_POINT('Ctrl Pts',(-397.285026745533,63.7440265700833,
-376.750757000099));
#231939=CARTESIAN_POINT('Ctrl Pts',(-332.361185159884,68.4070457431775,
-349.81728900008));
#231940=CARTESIAN_POINT('Ctrl Pts',(-267.437343574235,73.0700649162719,
-322.883821000062));
#231941=CARTESIAN_POINT('Ctrl Pts',(-202.513501988586,77.7330840893662,
-295.950353000043));
#231942=CARTESIAN_POINT('Ctrl Pts',(-170.051581195761,80.0645936759133,
-282.483619000033));
#231943=CARTESIAN_POINT('Ctrl Pts',(-137.589660402937,82.3961032624605,
-269.016885000024));
#231944=CARTESIAN_POINT('Ctrl Pts',(-105.127739610112,84.7276128490076,
-255.550151000015));
#231945=CARTESIAN_POINT('Ctrl Pts',(-88.8967792136999,85.8933676422812,
-248.81678400001));
#231946=CARTESIAN_POINT('Ctrl Pts',(-72.6658188172876,87.0591224355548,
-242.083417000005));
#231947=CARTESIAN_POINT('Ctrl Pts',(-56.4348584208753,88.2248772288284,
-235.35005));
#231948=CARTESIAN_POINT('Ctrl Pts',(-40.3646006026454,89.3790898954359,
-228.683349999995));
#231949=CARTESIAN_POINT('Ctrl Pts',(-24.254362128099,90.8531963631996,-222.016650000002));
#231950=CARTESIAN_POINT('Ctrl Pts',(-8.08526176211542,92.6441253491055,
-215.349950000002));
#231951=CARTESIAN_POINT('Ctrl Pts',(-7.92357075845534,92.6620346389644,
-215.283283000002));
#231952=CARTESIAN_POINT('Ctrl Pts',(-7.76187975479526,92.6799439288233,
-215.216616000002));
#231953=CARTESIAN_POINT('Ctrl Pts',(-7.60018875113518,92.6978532186822,
-215.149949000001));
#231954=CARTESIAN_POINT('Ctrl Pts',(-614.253443137008,133.230382677491,
-376.750757000185));
#231955=CARTESIAN_POINT('Ctrl Pts',(-520.217405101058,131.900620330773,
-349.81728900015));
#231956=CARTESIAN_POINT('Ctrl Pts',(-426.181367065107,130.570857984055,
-322.883821000115));
#231957=CARTESIAN_POINT('Ctrl Pts',(-332.145329029157,129.241095637338,
-295.950353000079));
#231958=CARTESIAN_POINT('Ctrl Pts',(-285.127310011182,128.576214463979,
-282.483619000062));
#231959=CARTESIAN_POINT('Ctrl Pts',(-238.109290993206,127.91133329062,-269.016885000044));
#231960=CARTESIAN_POINT('Ctrl Pts',(-191.091271975231,127.246452117261,
-255.550151000026));
#231961=CARTESIAN_POINT('Ctrl Pts',(-167.582262466243,126.914011530581,
-248.816784000018));
#231962=CARTESIAN_POINT('Ctrl Pts',(-144.073252957256,126.581570943902,
-242.083417000009));
#231963=CARTESIAN_POINT('Ctrl Pts',(-120.564243448268,126.249130357223,
-235.35005));
#231964=CARTESIAN_POINT('Ctrl Pts',(-97.2879964096667,125.9199812615,-228.683349999992));
#231965=CARTESIAN_POINT('Ctrl Pts',(-73.9399558818752,126.16474384846,-222.016650000005));
#231966=CARTESIAN_POINT('Ctrl Pts',(-50.4862477745394,126.97790796366,-215.349950000003));
#231967=CARTESIAN_POINT('Ctrl Pts',(-50.2517106934656,126.986039604812,
-215.283283000003));
#231968=CARTESIAN_POINT('Ctrl Pts',(-50.0171736123918,126.994171245964,
-215.216616000002));
#231969=CARTESIAN_POINT('Ctrl Pts',(-49.782636531318,127.002302887115,-215.149949000002));
#231970=CARTESIAN_POINT('Ctrl Pts',(-831.221859528483,202.716738784898,
-376.75075700027));
#231971=CARTESIAN_POINT('Ctrl Pts',(-708.073625042231,195.394194918369,
-349.817289000218));
#231972=CARTESIAN_POINT('Ctrl Pts',(-584.92539055598,188.071651051839,-322.883821000167));
#231973=CARTESIAN_POINT('Ctrl Pts',(-461.777156069728,180.749107185309,
-295.950353000116));
#231974=CARTESIAN_POINT('Ctrl Pts',(-400.203038826602,177.087835252044,
-282.48361900009));
#231975=CARTESIAN_POINT('Ctrl Pts',(-338.628921583476,173.426563318779,
-269.016885000064));
#231976=CARTESIAN_POINT('Ctrl Pts',(-277.05480434035,169.765291385514,-255.550151000039));
#231977=CARTESIAN_POINT('Ctrl Pts',(-246.267745718787,167.934655418882,
-248.816784000026));
#231978=CARTESIAN_POINT('Ctrl Pts',(-215.480687097224,166.10401945225,-242.083417000013));
#231979=CARTESIAN_POINT('Ctrl Pts',(-184.693628475661,164.273383485617,
-235.35005));
#231980=CARTESIAN_POINT('Ctrl Pts',(-154.211392216688,162.460872627565,
-228.683349999988));
#231981=CARTESIAN_POINT('Ctrl Pts',(-123.625549635651,161.47629133372,-222.016650000007));
#231982=CARTESIAN_POINT('Ctrl Pts',(-92.8872337869633,161.311690578215,
-215.349950000004));
#231983=CARTESIAN_POINT('Ctrl Pts',(-92.5798506284758,161.31004457066,-215.283283000004));
#231984=CARTESIAN_POINT('Ctrl Pts',(-92.2724674699883,161.308398563104,
-215.216616000004));
#231985=CARTESIAN_POINT('Ctrl Pts',(-91.9650843115009,161.306752555549,
-215.149949000004));
#231986=CARTESIAN_POINT('Ctrl Pts',(-1048.19027591996,272.203094892306,
-376.750757000354));
#231987=CARTESIAN_POINT('Ctrl Pts',(-895.929844983404,258.887769505964,
-349.817289000287));
#231988=CARTESIAN_POINT('Ctrl Pts',(-743.669414046851,245.572444119622,
-322.883821000219));
#231989=CARTESIAN_POINT('Ctrl Pts',(-591.408983110298,232.257118733281,
-295.950353000152));
#231990=CARTESIAN_POINT('Ctrl Pts',(-515.278767642022,225.59945604011,-282.483619000118));
#231991=CARTESIAN_POINT('Ctrl Pts',(-439.148552173745,218.941793346939,
-269.016885000084));
#231992=CARTESIAN_POINT('Ctrl Pts',(-363.018336705469,212.284130653768,
-255.550151000051));
#231993=CARTESIAN_POINT('Ctrl Pts',(-324.953228971331,208.955299307182,
-248.816784000034));
#231994=CARTESIAN_POINT('Ctrl Pts',(-286.888121237192,205.626467960597,
-242.083417000017));
#231995=CARTESIAN_POINT('Ctrl Pts',(-248.823013503054,202.297636614011,
-235.35005));
#231996=CARTESIAN_POINT('Ctrl Pts',(-211.134788023709,199.001763993629,
-228.683349999984));
#231997=CARTESIAN_POINT('Ctrl Pts',(-173.311143389428,196.787838818981,
-222.016650000008));
#231998=CARTESIAN_POINT('Ctrl Pts',(-135.288219799387,195.64547319277,-215.349950000004));
#231999=CARTESIAN_POINT('Ctrl Pts',(-134.907990563486,195.634049536507,
-215.283283000005));
#232000=CARTESIAN_POINT('Ctrl Pts',(-134.527761327585,195.622625880244,
-215.216616000005));
#232001=CARTESIAN_POINT('Ctrl Pts',(-134.147532091684,195.611202223982,
-215.149949000005));
#232002=CARTESIAN_POINT('Ctrl Pts',(-1699.09552509438,480.662163214529,
-376.75075700061));
#232003=CARTESIAN_POINT('Ctrl Pts',(-1459.49850480692,449.368493268751,
-349.817289000493));
#232004=CARTESIAN_POINT('Ctrl Pts',(-1219.90148451947,418.074823322972,
-322.883821000378));
#232005=CARTESIAN_POINT('Ctrl Pts',(-980.30446423201,386.781153377194,-295.950353000261));
#232006=CARTESIAN_POINT('Ctrl Pts',(-860.505954088282,371.134318404306,
-282.483619000203));
#232007=CARTESIAN_POINT('Ctrl Pts',(-740.707443944553,355.487483431416,
-269.016885000145));
#232008=CARTESIAN_POINT('Ctrl Pts',(-620.908933800825,339.840648458528,
-255.550151000087));
#232009=CARTESIAN_POINT('Ctrl Pts',(-561.009678728961,332.017230972083,
-248.816784000058));
#232010=CARTESIAN_POINT('Ctrl Pts',(-501.110423657097,324.193813485639,
-242.083417000029));
#232011=CARTESIAN_POINT('Ctrl Pts',(-441.211168585233,316.370395999194,
-235.35005));
#232012=CARTESIAN_POINT('Ctrl Pts',(-381.904975444773,308.624438091823,
-228.683349999972));
#232013=CARTESIAN_POINT('Ctrl Pts',(-322.367924650756,302.722481274762,
-222.016650000015));
#232014=CARTESIAN_POINT('Ctrl Pts',(-262.491177836659,298.646821036434,
-215.349950000008));
#232015=CARTESIAN_POINT('Ctrl Pts',(-261.892410368517,298.60606443405,-215.283283000008));
#232016=CARTESIAN_POINT('Ctrl Pts',(-261.293642900374,298.565307831665,
-215.216616000008));
#232017=CARTESIAN_POINT('Ctrl Pts',(-260.694875432232,298.524551229281,
-215.149949000007));
#232018=CARTESIAN_POINT('Ctrl Pts',(-2350.0007742688,689.121231536752,-376.750757000865));
#232019=CARTESIAN_POINT('Ctrl Pts',(-2023.06716463044,639.849217031537,
-349.8172890007));
#232020=CARTESIAN_POINT('Ctrl Pts',(-1696.13355499208,590.577202526323,
-322.883821000536));
#232021=CARTESIAN_POINT('Ctrl Pts',(-1369.19994535372,541.305188021109,
-295.95035300037));
#232022=CARTESIAN_POINT('Ctrl Pts',(-1205.73314053454,516.669180768502,
-282.483619000288));
#232023=CARTESIAN_POINT('Ctrl Pts',(-1042.26633571536,492.033173515894,
-269.016885000205));
#232024=CARTESIAN_POINT('Ctrl Pts',(-878.799530896182,467.397166263287,
-255.550151000123));
#232025=CARTESIAN_POINT('Ctrl Pts',(-797.066128486591,455.079162636984,
-248.816784000082));
#232026=CARTESIAN_POINT('Ctrl Pts',(-715.332726077001,442.76115901068,-242.083417000041));
#232027=CARTESIAN_POINT('Ctrl Pts',(-633.599323667412,430.443155384376,
-235.35005));
#232028=CARTESIAN_POINT('Ctrl Pts',(-552.675162865837,418.247112190016,
-228.68334999996));
#232029=CARTESIAN_POINT('Ctrl Pts',(-471.424705912085,408.657123730544,
-222.016650000021));
#232030=CARTESIAN_POINT('Ctrl Pts',(-389.694135873931,401.648168880098,
-215.34995000001));
#232031=CARTESIAN_POINT('Ctrl Pts',(-388.876830173548,401.578079331591,
-215.28328300001));
#232032=CARTESIAN_POINT('Ctrl Pts',(-388.059524473164,401.507989783086,
-215.216616000011));
#232033=CARTESIAN_POINT('Ctrl Pts',(-387.242218772781,401.43790023458,-215.149949000011));
#232034=CARTESIAN_POINT('Ctrl Pts',(-3000.90602344323,897.580299858975,
-376.75075700112));
#232035=CARTESIAN_POINT('Ctrl Pts',(-2586.63582445396,830.329940794324,
-349.817289000906));
#232036=CARTESIAN_POINT('Ctrl Pts',(-2172.36562546469,763.079581729674,
-322.883821000693));
#232037=CARTESIAN_POINT('Ctrl Pts',(-1758.09542647544,695.829222665023,
-295.95035300048));
#232038=CARTESIAN_POINT('Ctrl Pts',(-1550.9603269808,662.204043132698,-282.483619000373));
#232039=CARTESIAN_POINT('Ctrl Pts',(-1343.82522748617,628.578863600373,
-269.016885000266));
#232040=CARTESIAN_POINT('Ctrl Pts',(-1136.69012799154,594.953684068047,
-255.55015100016));
#232041=CARTESIAN_POINT('Ctrl Pts',(-1033.12257824422,578.141094301885,
-248.816784000106));
#232042=CARTESIAN_POINT('Ctrl Pts',(-929.555028496906,561.328504535722,
-242.083417000053));
#232043=CARTESIAN_POINT('Ctrl Pts',(-825.98747874959,544.515914769559,-235.35005));
#232044=CARTESIAN_POINT('Ctrl Pts',(-723.445350286901,527.86978628821,-228.683349999948));
#232045=CARTESIAN_POINT('Ctrl Pts',(-620.481487173413,514.591766186325,
-222.016650000027));
#232046=CARTESIAN_POINT('Ctrl Pts',(-516.897093911203,504.649516723762,
-215.349950000014));
#232047=CARTESIAN_POINT('Ctrl Pts',(-515.861249978578,504.550094229134,
-215.283283000013));
#232048=CARTESIAN_POINT('Ctrl Pts',(-514.825406045954,504.450671734507,
-215.216616000014));
#232049=CARTESIAN_POINT('Ctrl Pts',(-513.789562113329,504.351249239879,
-215.149949000014));
#232050=CARTESIAN_POINT('Ctrl Pts',(-4953.62177096649,1522.95750482565,
-376.750757001886));
#232051=CARTESIAN_POINT('Ctrl Pts',(-4277.34180392452,1401.77211208268,
-349.817289001526));
#232052=CARTESIAN_POINT('Ctrl Pts',(-3601.06183688254,1280.58671933972,
-322.883821001167));
#232053=CARTESIAN_POINT('Ctrl Pts',(-2924.78186984057,1159.40132659677,
-295.950353000808));
#232054=CARTESIAN_POINT('Ctrl Pts',(-2586.64188631958,1098.80863022529,
-282.483619000628));
#232055=CARTESIAN_POINT('Ctrl Pts',(-2248.50190279859,1038.21593385381,
-269.016885000448));
#232056=CARTESIAN_POINT('Ctrl Pts',(-1910.36191927761,977.623237482327,
-255.550151000268));
#232057=CARTESIAN_POINT('Ctrl Pts',(-1741.29192751712,947.326889296587,
-248.816784000179));
#232058=CARTESIAN_POINT('Ctrl Pts',(-1572.22193575662,917.030541110847,
-242.08341700009));
#232059=CARTESIAN_POINT('Ctrl Pts',(-1403.15194399613,886.734192925108,
-235.35005));
#232060=CARTESIAN_POINT('Ctrl Pts',(-1235.75591255009,856.737808582791,
-228.683349999911));
#232061=CARTESIAN_POINT('Ctrl Pts',(-1067.6518309574,832.395693553669,-222.016650000045));
#232062=CARTESIAN_POINT('Ctrl Pts',(-898.505968023019,813.653560254753,
-215.349950000023));
#232063=CARTESIAN_POINT('Ctrl Pts',(-896.814509393671,813.466138921761,
-215.283283000022));
#232064=CARTESIAN_POINT('Ctrl Pts',(-895.123050764323,813.278717588769,
-215.216616000022));
#232065=CARTESIAN_POINT('Ctrl Pts',(-893.431592134975,813.091296255777,
-215.149949000023));
#232066=CARTESIAN_POINT('Ctrl Pts',(-6906.33751848976,2148.33470979231,
-376.750757002651));
#232067=CARTESIAN_POINT('Ctrl Pts',(-5968.04778339507,1973.21428337105,
-349.817289002145));
#232068=CARTESIAN_POINT('Ctrl Pts',(-5029.75804830038,1798.09385694977,
-322.883821001641));
#232069=CARTESIAN_POINT('Ctrl Pts',(-4091.4683132057,1622.97343052851,-295.950353001135));
#232070=CARTESIAN_POINT('Ctrl Pts',(-3622.32344565836,1535.41321731788,
-282.483619000883));
#232071=CARTESIAN_POINT('Ctrl Pts',(-3153.17857811102,1447.85300410724,
-269.01688500063));
#232072=CARTESIAN_POINT('Ctrl Pts',(-2684.03371056368,1360.29279089661,
-255.550151000377));
#232073=CARTESIAN_POINT('Ctrl Pts',(-2449.46127679,1316.51268429129,-248.816784000251));
#232074=CARTESIAN_POINT('Ctrl Pts',(-2214.88884301634,1272.73257768597,
-242.083417000126));
#232075=CARTESIAN_POINT('Ctrl Pts',(-1980.31640924266,1228.95247108066,
-235.35005));
#232076=CARTESIAN_POINT('Ctrl Pts',(-1748.06647481329,1185.60583087737,
-228.683349999876));
#232077=CARTESIAN_POINT('Ctrl Pts',(-1514.82217474138,1150.19962092101,
-222.016650000063));
#232078=CARTESIAN_POINT('Ctrl Pts',(-1280.11484213483,1122.65760378574,
-215.349950000032));
#232079=CARTESIAN_POINT('Ctrl Pts',(-1277.76776880876,1122.38218361439,
-215.283283000032));
#232080=CARTESIAN_POINT('Ctrl Pts',(-1275.42069548269,1122.10676344303,
-215.216616000032));
#232081=CARTESIAN_POINT('Ctrl Pts',(-1273.07362215662,1121.83134327167,
-215.149949000032));
#232082=CARTESIAN_POINT('Ctrl Pts',(-8859.05326601302,2773.71191475898,
-376.750757003417));
#232083=CARTESIAN_POINT('Ctrl Pts',(-7658.75376286563,2544.6564546594,-349.817289002765));
#232084=CARTESIAN_POINT('Ctrl Pts',(-6458.45425971823,2315.60099455983,
-322.883821002114));
#232085=CARTESIAN_POINT('Ctrl Pts',(-5258.15475657084,2086.54553446025,
-295.950353001463));
#232086=CARTESIAN_POINT('Ctrl Pts',(-4658.00500499714,1972.01780441047,
-282.483619001138));
#232087=CARTESIAN_POINT('Ctrl Pts',(-4057.85525342344,1857.49007436067,
-269.016885000812));
#232088=CARTESIAN_POINT('Ctrl Pts',(-3457.70550184975,1742.96234431089,
-255.550151000486));
#232089=CARTESIAN_POINT('Ctrl Pts',(-3157.6306260629,1685.69847928599,-248.816784000324));
#232090=CARTESIAN_POINT('Ctrl Pts',(-2857.55575027604,1628.4346142611,-242.083417000162));
#232091=CARTESIAN_POINT('Ctrl Pts',(-2557.4808744892,1571.17074923621,-235.35005));
#232092=CARTESIAN_POINT('Ctrl Pts',(-2260.37703707648,1514.47385317195,
-228.683349999839));
#232093=CARTESIAN_POINT('Ctrl Pts',(-1961.99251852537,1468.00354828836,
-222.01665000008));
#232094=CARTESIAN_POINT('Ctrl Pts',(-1661.72371624665,1431.66164731674,
-215.349950000041));
#232095=CARTESIAN_POINT('Ctrl Pts',(-1658.72102822386,1431.29822830702,
-215.28328300004));
#232096=CARTESIAN_POINT('Ctrl Pts',(-1655.71834020106,1430.93480929729,
-215.216616000041));
#232097=CARTESIAN_POINT('Ctrl Pts',(-1652.71565217826,1430.57139028757,
-215.149949000041));
#232098=CARTESIAN_POINT('Ctrl Pts',(-14717.2005085828,4649.84352965899,
-376.750757005713));
#232099=CARTESIAN_POINT('Ctrl Pts',(-12730.8717012773,4258.98296852449,
-349.817289004623));
#232100=CARTESIAN_POINT('Ctrl Pts',(-10744.5428939718,3868.12240738999,
-322.883821003535));
#232101=CARTESIAN_POINT('Ctrl Pts',(-8758.21408666624,3477.26184625548,
-295.950353002446));
#232102=CARTESIAN_POINT('Ctrl Pts',(-7765.04968301347,3281.83156568823,
-282.483619001902));
#232103=CARTESIAN_POINT('Ctrl Pts',(-6771.88527936071,3086.40128512098,
-269.016885001358));
#232104=CARTESIAN_POINT('Ctrl Pts',(-5778.72087570795,2890.97100455373,
-255.550151000813));
#232105=CARTESIAN_POINT('Ctrl Pts',(-5282.13867388157,2793.2558642701,-248.816784000541));
#232106=CARTESIAN_POINT('Ctrl Pts',(-4785.55647205519,2695.54072398648,
-242.083417000271));
#232107=CARTESIAN_POINT('Ctrl Pts',(-4288.9742702288,2597.82558370285,-235.35005));
#232108=CARTESIAN_POINT('Ctrl Pts',(-3797.30872386605,2501.0779200557,-228.683349999731));
#232109=CARTESIAN_POINT('Ctrl Pts',(-3303.50354987733,2421.41533039039,
-222.016650000135));
#232110=CARTESIAN_POINT('Ctrl Pts',(-2806.55033858209,2358.67377790971,
-215.349950000068));
#232111=CARTESIAN_POINT('Ctrl Pts',(-2801.58080646913,2358.0463623849,-215.283283000067));
#232112=CARTESIAN_POINT('Ctrl Pts',(-2796.61127435617,2357.41894686008,
-215.216616000068));
#232113=CARTESIAN_POINT('Ctrl Pts',(-2791.64174224321,2356.79153133527,
-215.149949000068));
#232114=CARTESIAN_POINT('Ctrl Pts',(-20575.3477511526,6525.97514455899,
-376.750757008008));
#232115=CARTESIAN_POINT('Ctrl Pts',(-17802.9896396889,5973.30948238956,
-349.817289006482));
#232116=CARTESIAN_POINT('Ctrl Pts',(-15030.6315282253,5420.64382022014,
-322.883821004956));
#232117=CARTESIAN_POINT('Ctrl Pts',(-12258.2734167616,4867.97815805071,
-295.950353003429));
#232118=CARTESIAN_POINT('Ctrl Pts',(-10872.0943610298,4591.645326966,-282.483619002666));
#232119=CARTESIAN_POINT('Ctrl Pts',(-9485.91530529798,4315.31249588128,
-269.016885001903));
#232120=CARTESIAN_POINT('Ctrl Pts',(-8099.73624956616,4038.97966479657,
-255.55015100114));
#232121=CARTESIAN_POINT('Ctrl Pts',(-7406.64672170025,3900.81324925421,
-248.816784000758));
#232122=CARTESIAN_POINT('Ctrl Pts',(-6713.55719383433,3762.64683371185,
-242.083417000379));
#232123=CARTESIAN_POINT('Ctrl Pts',(-6020.46766596842,3624.4804181695,-235.35005));
#232124=CARTESIAN_POINT('Ctrl Pts',(-5334.24041065563,3487.68198693944,
-228.683349999624));
#232125=CARTESIAN_POINT('Ctrl Pts',(-4645.01458122929,3374.82711249242,
-222.016650000188));
#232126=CARTESIAN_POINT('Ctrl Pts',(-3951.37696091755,3285.68590850268,
-215.349950000095));
#232127=CARTESIAN_POINT('Ctrl Pts',(-3944.44058471441,3284.79449646278,
-215.283283000095));
#232128=CARTESIAN_POINT('Ctrl Pts',(-3937.50420851128,3283.90308442287,
-215.216616000095));
#232129=CARTESIAN_POINT('Ctrl Pts',(-3930.56783230814,3283.01167238296,
-215.149949000095));
#232130=CARTESIAN_POINT('Ctrl Pts',(-26433.4949937224,8402.106759459,-376.750757010304));
#232131=CARTESIAN_POINT('Ctrl Pts',(-22875.1075781007,7687.63599625465,
-349.81728900834));
#232132=CARTESIAN_POINT('Ctrl Pts',(-19316.7201624788,6973.16523305029,
-322.883821006377));
#232133=CARTESIAN_POINT('Ctrl Pts',(-15758.332746857,6258.69446984594,-295.950353004413));
#232134=CARTESIAN_POINT('Ctrl Pts',(-13979.1390390461,5901.45908824376,
-282.48361900343));
#232135=CARTESIAN_POINT('Ctrl Pts',(-12199.9453312353,5544.22370664158,
-269.016885002448));
#232136=CARTESIAN_POINT('Ctrl Pts',(-10420.7516234244,5186.98832503941,
-255.550151001467));
#232137=CARTESIAN_POINT('Ctrl Pts',(-9531.15476951892,5008.37063423832,
-248.816784000976));
#232138=CARTESIAN_POINT('Ctrl Pts',(-8641.55791561347,4829.75294343723,
-242.083417000487));
#232139=CARTESIAN_POINT('Ctrl Pts',(-7751.96106170802,4651.13525263614,
-235.35005));
#232140=CARTESIAN_POINT('Ctrl Pts',(-6871.1720974452,4474.28605382318,-228.683349999516));
#232141=CARTESIAN_POINT('Ctrl Pts',(-5986.52561258124,4328.23889459445,
-222.016650000243));
#232142=CARTESIAN_POINT('Ctrl Pts',(-5096.20358325299,4212.69803909567,
-215.349950000122));
#232143=CARTESIAN_POINT('Ctrl Pts',(-5087.30036295968,4211.54263054066,
-215.283283000121));
#232144=CARTESIAN_POINT('Ctrl Pts',(-5078.39714266638,4210.38722198566,
-215.216616000122));
#232145=CARTESIAN_POINT('Ctrl Pts',(-5069.49392237307,4209.23181343066,
-215.149949000122));
#232146=CARTESIAN_POINT('Origin',(0.,-12.9675000200281,-218.35005));
#232147=CARTESIAN_POINT('Ctrl Pts',(-10765.646428189,-1979.29526939781,
-376.750757000846));
#232148=CARTESIAN_POINT('Ctrl Pts',(-9257.10677574949,-1902.78686830728,
-349.817289000686));
#232149=CARTESIAN_POINT('Ctrl Pts',(-7748.56712330994,-1826.27846721676,
-322.883821000524));
#232150=CARTESIAN_POINT('Ctrl Pts',(-6240.0274708704,-1749.77006612623,
-295.950353000363));
#232151=CARTESIAN_POINT('Ctrl Pts',(-5485.75764465062,-1711.51586558096,
-282.483619000282));
#232152=CARTESIAN_POINT('Ctrl Pts',(-4731.48781843085,-1673.2616650357,
-269.016885000202));
#232153=CARTESIAN_POINT('Ctrl Pts',(-3977.21799221108,-1635.00746449044,
-255.550151000121));
#232154=CARTESIAN_POINT('Ctrl Pts',(-3600.08307910119,-1615.8803642178,
-248.816784000081));
#232155=CARTESIAN_POINT('Ctrl Pts',(-3222.9481659913,-1596.75326394517,
-242.083417000041));
#232156=CARTESIAN_POINT('Ctrl Pts',(-2845.81325288141,-1577.62616367254,
-235.35005));
#232157=CARTESIAN_POINT('Ctrl Pts',(-2472.41234881222,-1558.68844063033,
-228.68334999996));
#232158=CARTESIAN_POINT('Ctrl Pts',(-2099.07452015968,-1540.45097924114,
-222.01665));
#232159=CARTESIAN_POINT('Ctrl Pts',(-1725.79722689738,-1522.91379824522,
-215.34994999996));
#232160=CARTESIAN_POINT('Ctrl Pts',(-1722.06445396475,-1522.73842643524,
-215.28328299996));
#232161=CARTESIAN_POINT('Ctrl Pts',(-1718.33168103213,-1522.56305462527,
-215.21661599996));
#232162=CARTESIAN_POINT('Ctrl Pts',(-1714.5989080995,-1522.3876828153,-215.14994899996));
#232163=CARTESIAN_POINT('Ctrl Pts',(-8392.35568812379,-1534.61913504983,
-376.750757000658));
#232164=CARTESIAN_POINT('Ctrl Pts',(-7213.78531733318,-1478.38877237011,
-349.817289000532));
#232165=CARTESIAN_POINT('Ctrl Pts',(-6035.21494654257,-1422.15840969038,
-322.883821000408));
#232166=CARTESIAN_POINT('Ctrl Pts',(-4856.64457575196,-1365.92804701065,
-295.950353000282));
#232167=CARTESIAN_POINT('Ctrl Pts',(-4267.35939035666,-1337.81286567079,
-282.48361900022));
#232168=CARTESIAN_POINT('Ctrl Pts',(-3678.07420496136,-1309.69768433093,
-269.016885000157));
#232169=CARTESIAN_POINT('Ctrl Pts',(-3088.78901956605,-1281.58250299106,
-255.550151000094));
#232170=CARTESIAN_POINT('Ctrl Pts',(-2794.1464268684,-1267.52491232113,
-248.816784000063));
#232171=CARTESIAN_POINT('Ctrl Pts',(-2499.50383417074,-1253.4673216512,
-242.083417000031));
#232172=CARTESIAN_POINT('Ctrl Pts',(-2204.8612414731,-1239.40973098127,
-235.35005));
#232173=CARTESIAN_POINT('Ctrl Pts',(-1913.13590216849,-1225.49132437738,
-228.683349999968));
#232174=CARTESIAN_POINT('Ctrl Pts',(-1621.45955977666,-1212.11656254984,
-222.01665));
#232175=CARTESIAN_POINT('Ctrl Pts',(-1329.83024235737,-1199.28546008462,
-215.349949999969));
#232176=CARTESIAN_POINT('Ctrl Pts',(-1326.91394918317,-1199.15714905996,
-215.283282999969));
#232177=CARTESIAN_POINT('Ctrl Pts',(-1323.99765600898,-1199.02883803529,
-215.216615999969));
#232178=CARTESIAN_POINT('Ctrl Pts',(-1321.08136283478,-1198.90052701063,
-215.149948999969));
#232179=CARTESIAN_POINT('Ctrl Pts',(-6019.06494805854,-1089.94300070186,
-376.750757000469));
#232180=CARTESIAN_POINT('Ctrl Pts',(-5170.46385891687,-1053.99067643293,
-349.817289000379));
#232181=CARTESIAN_POINT('Ctrl Pts',(-4321.8627697752,-1018.03835216401,
-322.88382100029));
#232182=CARTESIAN_POINT('Ctrl Pts',(-3473.26168063352,-982.086027895082,
-295.950353000201));
#232183=CARTESIAN_POINT('Ctrl Pts',(-3048.96113606269,-964.10986576062,
-282.483619000157));
#232184=CARTESIAN_POINT('Ctrl Pts',(-2624.66059149186,-946.133703626157,
-269.016885000112));
#232185=CARTESIAN_POINT('Ctrl Pts',(-2200.36004692103,-928.157541491694,
-255.550151000067));
#232186=CARTESIAN_POINT('Ctrl Pts',(-1988.2097746356,-919.169460424462,
-248.816784000044));
#232187=CARTESIAN_POINT('Ctrl Pts',(-1776.05950235019,-910.181379357231,
-242.083417000023));
#232188=CARTESIAN_POINT('Ctrl Pts',(-1563.90923006478,-901.19329829,-235.35005));
#232189=CARTESIAN_POINT('Ctrl Pts',(-1353.85945552476,-892.294208124424,
-228.683349999978));
#232190=CARTESIAN_POINT('Ctrl Pts',(-1143.84459939364,-883.782145858533,
-222.01665));
#232191=CARTESIAN_POINT('Ctrl Pts',(-933.863257817356,-875.657121924021,
-215.349949999977));
#232192=CARTESIAN_POINT('Ctrl Pts',(-931.763444401592,-875.575871684668,
-215.283282999978));
#232193=CARTESIAN_POINT('Ctrl Pts',(-929.663630985828,-875.494621445315,
-215.216615999977));
#232194=CARTESIAN_POINT('Ctrl Pts',(-927.563817570064,-875.413371205962,
-215.149948999978));
#232195=CARTESIAN_POINT('Ctrl Pts',(-3645.77420799329,-645.266866353884,
-376.75075700028));
#232196=CARTESIAN_POINT('Ctrl Pts',(-3127.14240050056,-629.592580495759,
-349.817289000227));
#232197=CARTESIAN_POINT('Ctrl Pts',(-2608.51059300782,-613.918294637635,
-322.883821000173));
#232198=CARTESIAN_POINT('Ctrl Pts',(-2089.87878551509,-598.24400877951,
-295.95035300012));
#232199=CARTESIAN_POINT('Ctrl Pts',(-1830.56288176873,-590.406865850448,
-282.483619000093));
#232200=CARTESIAN_POINT('Ctrl Pts',(-1571.24697802237,-582.569722921386,
-269.016885000067));
#232201=CARTESIAN_POINT('Ctrl Pts',(-1311.931074276,-574.732579992324,-255.55015100004));
#232202=CARTESIAN_POINT('Ctrl Pts',(-1182.27312240282,-570.814008527792,
-248.816784000027));
#232203=CARTESIAN_POINT('Ctrl Pts',(-1052.61517052964,-566.895437063261,
-242.083417000014));
#232204=CARTESIAN_POINT('Ctrl Pts',(-922.957218656454,-562.97686559873,
-235.35005));
#232205=CARTESIAN_POINT('Ctrl Pts',(-794.583008881026,-559.097091871471,
-228.683349999987));
#232206=CARTESIAN_POINT('Ctrl Pts',(-666.229639010622,-555.447729167229,
-222.01665));
#232207=CARTESIAN_POINT('Ctrl Pts',(-537.896273277345,-552.028783763422,
-215.349949999987));
#232208=CARTESIAN_POINT('Ctrl Pts',(-536.612939620012,-551.994594309379,
-215.283282999987));
#232209=CARTESIAN_POINT('Ctrl Pts',(-535.329605962679,-551.960404855337,
-215.216615999987));
#232210=CARTESIAN_POINT('Ctrl Pts',(-534.046272305346,-551.926215401294,
-215.149948999987));
#232211=CARTESIAN_POINT('Ctrl Pts',(-2854.6772946382,-497.041488237892,
-376.750757000217));
#232212=CARTESIAN_POINT('Ctrl Pts',(-2446.03524769512,-488.126548516702,
-349.817289000176));
#232213=CARTESIAN_POINT('Ctrl Pts',(-2037.39320075203,-479.211608795511,
-322.883821000135));
#232214=CARTESIAN_POINT('Ctrl Pts',(-1628.75115380895,-470.29666907432,
-295.950353000093));
#232215=CARTESIAN_POINT('Ctrl Pts',(-1424.43013033741,-465.839199213724,
-282.483619000073));
#232216=CARTESIAN_POINT('Ctrl Pts',(-1220.10910686587,-461.381729353129,
-269.016885000052));
#232217=CARTESIAN_POINT('Ctrl Pts',(-1015.78808339432,-456.924259492534,
-255.550151000031));
#232218=CARTESIAN_POINT('Ctrl Pts',(-913.627571658554,-454.695524562236,
-248.816784000021));
#232219=CARTESIAN_POINT('Ctrl Pts',(-811.467059922784,-452.466789631938,
-242.083417000011));
#232220=CARTESIAN_POINT('Ctrl Pts',(-709.306548187014,-450.23805470164,
-235.35005));
#232221=CARTESIAN_POINT('Ctrl Pts',(-608.157526666449,-448.03138645382,
-228.68334999999));
#232222=CARTESIAN_POINT('Ctrl Pts',(-507.024652216282,-446.002923603462,
-222.01665));
#232223=CARTESIAN_POINT('Ctrl Pts',(-405.907278430675,-444.152671043223,
-215.34994999999));
#232224=CARTESIAN_POINT('Ctrl Pts',(-404.896104692818,-444.134168517617,
-215.283282999989));
#232225=CARTESIAN_POINT('Ctrl Pts',(-403.884930954962,-444.115665992011,
-215.21661599999));
#232226=CARTESIAN_POINT('Ctrl Pts',(-402.873757217106,-444.097163466405,
-215.14994899999));
#232227=CARTESIAN_POINT('Ctrl Pts',(-2063.58038128312,-348.816110121901,
-376.750757000154));
#232228=CARTESIAN_POINT('Ctrl Pts',(-1764.92809488968,-346.660516537644,
-349.817289000125));
#232229=CARTESIAN_POINT('Ctrl Pts',(-1466.27580849624,-344.504922953386,
-322.883821000096));
#232230=CARTESIAN_POINT('Ctrl Pts',(-1167.6235221028,-342.349329369129,
-295.950353000066));
#232231=CARTESIAN_POINT('Ctrl Pts',(-1018.29737890609,-341.271532577001,
-282.483619000052));
#232232=CARTESIAN_POINT('Ctrl Pts',(-868.971235709368,-340.193735784872,
-269.016885000037));
#232233=CARTESIAN_POINT('Ctrl Pts',(-719.64509251265,-339.115938992743,
-255.550151000022));
#232234=CARTESIAN_POINT('Ctrl Pts',(-644.982020914291,-338.577040596679,
-248.816784000015));
#232235=CARTESIAN_POINT('Ctrl Pts',(-570.318949315933,-338.038142200615,
-242.083417000008));
#232236=CARTESIAN_POINT('Ctrl Pts',(-495.655877717574,-337.49924380455,
-235.35005));
#232237=CARTESIAN_POINT('Ctrl Pts',(-421.732044451872,-336.96568103617,
-228.683349999993));
#232238=CARTESIAN_POINT('Ctrl Pts',(-347.819665421942,-336.558118039694,
-222.01665));
#232239=CARTESIAN_POINT('Ctrl Pts',(-273.918283584005,-336.276558323023,
-215.349949999993));
#232240=CARTESIAN_POINT('Ctrl Pts',(-273.179269765626,-336.273742725853,
-215.283282999993));
#232241=CARTESIAN_POINT('Ctrl Pts',(-272.440255947246,-336.270927128685,
-215.216615999993));
#232242=CARTESIAN_POINT('Ctrl Pts',(-271.701242128866,-336.268111531515,
-215.149948999993));
#232243=CARTESIAN_POINT('Ctrl Pts',(-1272.48346792803,-200.59073200591,
-376.750757000092));
#232244=CARTESIAN_POINT('Ctrl Pts',(-1083.82094208424,-205.194484558586,
-349.817289000074));
#232245=CARTESIAN_POINT('Ctrl Pts',(-895.15841624045,-209.798237111262,
-322.883821000057));
#232246=CARTESIAN_POINT('Ctrl Pts',(-706.49589039666,-214.401989663939,
-295.950353000039));
#232247=CARTESIAN_POINT('Ctrl Pts',(-612.164627474765,-216.703865940277,
-282.483619000031));
#232248=CARTESIAN_POINT('Ctrl Pts',(-517.83336455287,-219.005742216615,
-269.016885000022));
#232249=CARTESIAN_POINT('Ctrl Pts',(-423.502101630976,-221.307618492953,
-255.550151000013));
#232250=CARTESIAN_POINT('Ctrl Pts',(-376.336470170028,-222.458556631122,
-248.816784000009));
#232251=CARTESIAN_POINT('Ctrl Pts',(-329.170838709081,-223.609494769291,
-242.083417000004));
#232252=CARTESIAN_POINT('Ctrl Pts',(-282.005207248134,-224.760432907461,
-235.35005));
#232253=CARTESIAN_POINT('Ctrl Pts',(-235.306562237295,-225.899975618519,
-228.683349999995));
#232254=CARTESIAN_POINT('Ctrl Pts',(-188.614678627603,-227.113312475926,
-222.01665));
#232255=CARTESIAN_POINT('Ctrl Pts',(-141.929288737335,-228.400445602824,
-215.349949999996));
#232256=CARTESIAN_POINT('Ctrl Pts',(-141.462434838432,-228.413316934091,
-215.283282999995));
#232257=CARTESIAN_POINT('Ctrl Pts',(-140.995580939529,-228.426188265358,
-215.216615999995));
#232258=CARTESIAN_POINT('Ctrl Pts',(-140.528727040626,-228.439059596626,
-215.149948999996));
#232259=CARTESIAN_POINT('Ctrl Pts',(-1008.78449680967,-151.182272633913,
-376.750757000071));
#232260=CARTESIAN_POINT('Ctrl Pts',(-856.785224482427,-158.039140565566,
-349.817289000057));
#232261=CARTESIAN_POINT('Ctrl Pts',(-704.785952155186,-164.896008497221,
-322.883821000044));
#232262=CARTESIAN_POINT('Ctrl Pts',(-552.786679827945,-171.752876428875,
-295.95035300003));
#232263=CARTESIAN_POINT('Ctrl Pts',(-476.787043664325,-175.181310394702,
-282.483619000024));
#232264=CARTESIAN_POINT('Ctrl Pts',(-400.787407500704,-178.609744360529,
-269.016885000016));
#232265=CARTESIAN_POINT('Ctrl Pts',(-324.787771337084,-182.038178326357,
-255.55015100001));
#232266=CARTESIAN_POINT('Ctrl Pts',(-286.787953255274,-183.75239530927,
-248.816784000007));
#232267=CARTESIAN_POINT('Ctrl Pts',(-248.788135173463,-185.466612292184,
-242.083417000003));
#232268=CARTESIAN_POINT('Ctrl Pts',(-210.788317091653,-187.180829275097,
-235.35005));
#232269=CARTESIAN_POINT('Ctrl Pts',(-173.164734832436,-188.878073812635,
-228.683349999997));
#232270=CARTESIAN_POINT('Ctrl Pts',(-135.546349696156,-190.631710621336,
-222.01665));
#232271=CARTESIAN_POINT('Ctrl Pts',(-97.932957121778,-192.441741362757,
-215.349949999997));
#232272=CARTESIAN_POINT('Ctrl Pts',(-97.5568231960341,-192.45984167017,
-215.283282999997));
#232273=CARTESIAN_POINT('Ctrl Pts',(-97.1806892702902,-192.477941977583,
-215.216615999996));
#232274=CARTESIAN_POINT('Ctrl Pts',(-96.8045553445463,-192.496042284996,
-215.149948999996));
#232275=CARTESIAN_POINT('Ctrl Pts',(-745.085525691306,-101.773813261915,
-376.75075700005));
#232276=CARTESIAN_POINT('Ctrl Pts',(-629.749506880614,-110.883796572547,
-349.81728900004));
#232277=CARTESIAN_POINT('Ctrl Pts',(-514.413488069922,-119.993779883179,
-322.88382100003));
#232278=CARTESIAN_POINT('Ctrl Pts',(-399.07746925923,-129.103763193811,
-295.950353000021));
#232279=CARTESIAN_POINT('Ctrl Pts',(-341.409459853884,-133.658754849127,
-282.483619000017));
#232280=CARTESIAN_POINT('Ctrl Pts',(-283.741450448538,-138.213746504444,
-269.016885000012));
#232281=CARTESIAN_POINT('Ctrl Pts',(-226.073441043192,-142.76873815976,
-255.550151000007));
#232282=CARTESIAN_POINT('Ctrl Pts',(-197.239436340519,-145.046233987418,
-248.816784000005));
#232283=CARTESIAN_POINT('Ctrl Pts',(-168.405431637847,-147.323729815076,
-242.083417000002));
#232284=CARTESIAN_POINT('Ctrl Pts',(-139.571426935173,-149.601225642734,
-235.35005));
#232285=CARTESIAN_POINT('Ctrl Pts',(-111.022907427576,-151.856172006752,
-228.683349999998));
#232286=CARTESIAN_POINT('Ctrl Pts',(-82.4780207647092,-154.150108766748,
-222.01665));
#232287=CARTESIAN_POINT('Ctrl Pts',(-53.9366255062213,-156.48303712269,
-215.349949999998));
#232288=CARTESIAN_POINT('Ctrl Pts',(-53.6512115536363,-156.506366406249,
-215.283282999997));
#232289=CARTESIAN_POINT('Ctrl Pts',(-53.3657976010514,-156.529695689807,
-215.216615999998));
#232290=CARTESIAN_POINT('Ctrl Pts',(-53.0803836484664,-156.553024973366,
-215.149948999998));
#232291=CARTESIAN_POINT('Ctrl Pts',(-481.386554572944,-52.3653538899179,
-376.750757000028));
#232292=CARTESIAN_POINT('Ctrl Pts',(-402.713789278801,-63.7284525795279,
-349.817289000023));
#232293=CARTESIAN_POINT('Ctrl Pts',(-324.041023984658,-75.0915512691379,
-322.883821000018));
#232294=CARTESIAN_POINT('Ctrl Pts',(-245.368258690515,-86.4546499587479,
-295.950353000012));
#232295=CARTESIAN_POINT('Ctrl Pts',(-206.031876043444,-92.1361993035529,
-282.48361900001));
#232296=CARTESIAN_POINT('Ctrl Pts',(-166.695493396372,-97.8177486483579,
-269.016885000007));
#232297=CARTESIAN_POINT('Ctrl Pts',(-127.359110749301,-103.499297993163,
-255.550151000004));
#232298=CARTESIAN_POINT('Ctrl Pts',(-107.690919425765,-106.340072665565,
-248.816784000003));
#232299=CARTESIAN_POINT('Ctrl Pts',(-88.0227281022291,-109.180847337968,
-242.083417000002));
#232300=CARTESIAN_POINT('Ctrl Pts',(-68.3545367786933,-112.02162201037,
-235.35005));
#232301=CARTESIAN_POINT('Ctrl Pts',(-48.8810800227174,-114.834270200868,
-228.683349999999));
#232302=CARTESIAN_POINT('Ctrl Pts',(-29.4096918332626,-117.668506912158,
-222.01665));
#232303=CARTESIAN_POINT('Ctrl Pts',(-9.94029389066457,-120.524332882624,
-215.349949999999));
#232304=CARTESIAN_POINT('Ctrl Pts',(-9.74559991123855,-120.552891142328,
-215.283282999999));
#232305=CARTESIAN_POINT('Ctrl Pts',(-9.55090593181253,-120.581449402032,
-215.216615999999));
#232306=CARTESIAN_POINT('Ctrl Pts',(-9.3562119523865,-120.610007661736,
-215.149948999999));
#232307=CARTESIAN_POINT('Ctrl Pts',(-393.48689753349,-35.8958674325856,
-376.750757000021));
#232308=CARTESIAN_POINT('Ctrl Pts',(-327.035216744864,-48.0100045818548,
-349.817289000017));
#232309=CARTESIAN_POINT('Ctrl Pts',(-260.583535956237,-60.1241417311241,
-322.883821000013));
#232310=CARTESIAN_POINT('Ctrl Pts',(-194.13185516761,-72.2382788803934,
-295.950353000009));
#232311=CARTESIAN_POINT('Ctrl Pts',(-160.906014773297,-78.2953474550281,
-282.483619000007));
#232312=CARTESIAN_POINT('Ctrl Pts',(-127.680174378983,-84.3524160296627,
-269.016885000005));
#232313=CARTESIAN_POINT('Ctrl Pts',(-94.45433398467,-90.4094846042973,-255.550151000003));
#232314=CARTESIAN_POINT('Ctrl Pts',(-77.8414137875133,-93.4380188916147,
-248.816784000002));
#232315=CARTESIAN_POINT('Ctrl Pts',(-61.2284935903567,-96.466553178932,
-242.083417000001));
#232316=CARTESIAN_POINT('Ctrl Pts',(-44.6155733932,-99.4950874662493,-235.35005));
#232317=CARTESIAN_POINT('Ctrl Pts',(-28.167137554431,-102.493636265573,
-228.683349999999));
#232318=CARTESIAN_POINT('Ctrl Pts',(-11.7202488561137,-105.507972960628,
-222.01665));
#232319=CARTESIAN_POINT('Ctrl Pts',(4.72514998118767,-108.538098135935,
-215.349949999999));
#232320=CARTESIAN_POINT('Ctrl Pts',(4.88960396956071,-108.568399387688,
-215.283282999999));
#232321=CARTESIAN_POINT('Ctrl Pts',(5.05405795793375,-108.59870063944,-215.216615999999));
#232322=CARTESIAN_POINT('Ctrl Pts',(5.2185119463068,-108.629001891193,-215.149948999999));
#232323=CARTESIAN_POINT('Ctrl Pts',(-305.587240494037,-19.4263809752531,
-376.750757000014));
#232324=CARTESIAN_POINT('Ctrl Pts',(-251.356644210927,-32.2915565841817,
-349.817289000011));
#232325=CARTESIAN_POINT('Ctrl Pts',(-197.126047927816,-45.1567321931103,
-322.883821000009));
#232326=CARTESIAN_POINT('Ctrl Pts',(-142.895451644705,-58.0219078020389,
-295.950353000006));
#232327=CARTESIAN_POINT('Ctrl Pts',(-115.78015350315,-64.4544956065032,
-282.483619000005));
#232328=CARTESIAN_POINT('Ctrl Pts',(-88.6648553615948,-70.8870834109675,
-269.016885000003));
#232329=CARTESIAN_POINT('Ctrl Pts',(-61.5495572200395,-77.3196712154318,
-255.550151000002));
#232330=CARTESIAN_POINT('Ctrl Pts',(-47.9919081492619,-80.5359651176639,
-248.816784000002));
#232331=CARTESIAN_POINT('Ctrl Pts',(-34.4342590784842,-83.7522590198961,
-242.083417000001));
#232332=CARTESIAN_POINT('Ctrl Pts',(-20.8766100077067,-86.9685529221282,
-235.35005));
#232333=CARTESIAN_POINT('Ctrl Pts',(-7.45319508614462,-90.1530023302789,
-228.68335));
#232334=CARTESIAN_POINT('Ctrl Pts',(5.96919412103514,-93.3474390090985,
-222.01665));
#232335=CARTESIAN_POINT('Ctrl Pts',(19.3905938530399,-96.5518633892461,
-215.34995));
#232336=CARTESIAN_POINT('Ctrl Pts',(19.52480785036,-96.5839076330473,-215.283283));
#232337=CARTESIAN_POINT('Ctrl Pts',(19.6590218476801,-96.6159518768485,
-215.216616));
#232338=CARTESIAN_POINT('Ctrl Pts',(19.7932358450001,-96.6479961206498,
-215.149949));
#232339=CARTESIAN_POINT('Ctrl Pts',(-217.687583454584,-2.9568945179205,
-376.750757000007));
#232340=CARTESIAN_POINT('Ctrl Pts',(-175.67807167699,-16.5731085865084,
-349.817289000006));
#232341=CARTESIAN_POINT('Ctrl Pts',(-133.668559899395,-30.1893226550964,
-322.883821000005));
#232342=CARTESIAN_POINT('Ctrl Pts',(-91.6590481218006,-43.8055367236842,
-295.950353000003));
#232343=CARTESIAN_POINT('Ctrl Pts',(-70.6542922330034,-50.6136437579782,
-282.483619000003));
#232344=CARTESIAN_POINT('Ctrl Pts',(-49.6495363442062,-57.4217507922722,
-269.016885000001));
#232345=CARTESIAN_POINT('Ctrl Pts',(-28.644780455409,-64.2298578265662,
-255.550151000001));
#232346=CARTESIAN_POINT('Ctrl Pts',(-18.1424025110104,-67.6339113437132,
-248.816784000001));
#232347=CARTESIAN_POINT('Ctrl Pts',(-7.64002456661188,-71.0379648608601,
-242.083417000001));
#232348=CARTESIAN_POINT('Ctrl Pts',(2.8623533777867,-74.4420183780071,-235.35005));
#232349=CARTESIAN_POINT('Ctrl Pts',(13.2607473821417,-77.8123683949843,
-228.68335));
#232350=CARTESIAN_POINT('Ctrl Pts',(23.658637098184,-81.1869050575687,-222.01665));
#232351=CARTESIAN_POINT('Ctrl Pts',(34.0560377248921,-84.5656286425572,
-215.34995));
#232352=CARTESIAN_POINT('Ctrl Pts',(34.1600117311593,-84.599415878407,-215.283283));
#232353=CARTESIAN_POINT('Ctrl Pts',(34.2639857374263,-84.6332031142567,
-215.216616));
#232354=CARTESIAN_POINT('Ctrl Pts',(34.3679597436934,-84.6669903501065,
-215.149949));
#232355=CARTESIAN_POINT('Ctrl Pts',(-188.387697774766,2.53293430119023,
-376.750757000005));
#232356=CARTESIAN_POINT('Ctrl Pts',(-150.451880832343,-11.3336259206174,
-349.817289000004));
#232357=CARTESIAN_POINT('Ctrl Pts',(-112.516063889921,-25.2001861424251,
-322.883821000003));
#232358=CARTESIAN_POINT('Ctrl Pts',(-74.580246947499,-39.0667463642328,
-295.950353000002));
#232359=CARTESIAN_POINT('Ctrl Pts',(-55.6123384762878,-46.0000264751366,
-282.483619000002));
#232360=CARTESIAN_POINT('Ctrl Pts',(-36.6444300050767,-52.9333065860405,
-269.016885000001));
#232361=CARTESIAN_POINT('Ctrl Pts',(-17.6765215338656,-59.8665866969443,
-255.550151000001));
#232362=CARTESIAN_POINT('Ctrl Pts',(-8.19256729825999,-63.3332267523963,
-248.816784000001));
#232363=CARTESIAN_POINT('Ctrl Pts',(1.29138693734558,-66.7998668078482,
-242.083417));
#232364=CARTESIAN_POINT('Ctrl Pts',(10.7753411729511,-70.2665068633001,
-235.35005));
#232365=CARTESIAN_POINT('Ctrl Pts',(20.1653948715705,-73.6988237498861,
-228.68335));
#232366=CARTESIAN_POINT('Ctrl Pts',(29.5551180905669,-77.1333937403921,
-222.01665));
#232367=CARTESIAN_POINT('Ctrl Pts',(38.9445190155095,-80.5702170603276,
-215.34995));
#232368=CARTESIAN_POINT('Ctrl Pts',(39.038413024759,-80.6045852935269,-215.283283));
#232369=CARTESIAN_POINT('Ctrl Pts',(39.1323070340084,-80.6389535267262,
-215.216616));
#232370=CARTESIAN_POINT('Ctrl Pts',(39.2262010432579,-80.6733217599254,
-215.149949));
#232371=CARTESIAN_POINT('Ctrl Pts',(-159.087812094948,8.022763120301,-376.750757000003));
#232372=CARTESIAN_POINT('Ctrl Pts',(-125.225689987698,-6.09414325472644,
-349.817289000002));
#232373=CARTESIAN_POINT('Ctrl Pts',(-91.3635678804476,-20.2110496297539,
-322.883821000001));
#232374=CARTESIAN_POINT('Ctrl Pts',(-57.5014457731974,-34.3279560047813,
-295.950353000001));
#232375=CARTESIAN_POINT('Ctrl Pts',(-40.5703847195723,-41.386409192295,
-282.483619000001));
#232376=CARTESIAN_POINT('Ctrl Pts',(-23.6393236659472,-48.4448623798088,
-269.016885));
#232377=CARTESIAN_POINT('Ctrl Pts',(-6.70826261232206,-55.5033155673225,
-255.550151000001));
#232378=CARTESIAN_POINT('Ctrl Pts',(1.75726791449049,-59.0325421610793,
-248.816784));
#232379=CARTESIAN_POINT('Ctrl Pts',(10.222798441303,-62.5617687548362,-242.083417));
#232380=CARTESIAN_POINT('Ctrl Pts',(18.6883289681156,-66.090995348593,-235.35005));
#232381=CARTESIAN_POINT('Ctrl Pts',(27.0700423609993,-69.585279104788,-228.68335));
#232382=CARTESIAN_POINT('Ctrl Pts',(35.4515990829499,-73.0798824232155,
-222.01665));
#232383=CARTESIAN_POINT('Ctrl Pts',(43.833000306127,-76.574805478098,-215.34995));
#232384=CARTESIAN_POINT('Ctrl Pts',(43.9168143183588,-76.6097547086468,
-215.283283));
#232385=CARTESIAN_POINT('Ctrl Pts',(44.0006283305905,-76.6447039391955,
-215.216616));
#232386=CARTESIAN_POINT('Ctrl Pts',(44.0844423428223,-76.6796531697443,
-215.149949));
#232387=CARTESIAN_POINT('Ctrl Pts',(-129.78792641513,13.512591939412,-376.750757));
#232388=CARTESIAN_POINT('Ctrl Pts',(-99.9994991430521,-0.854660588835203,
-349.817289000001));
#232389=CARTESIAN_POINT('Ctrl Pts',(-70.211071870974,-15.2219131170825,
-322.883821));
#232390=CARTESIAN_POINT('Ctrl Pts',(-40.4226445988958,-29.5891656453297,
-295.950353));
#232391=CARTESIAN_POINT('Ctrl Pts',(-25.5284309628568,-36.7727919094533,
-282.483619));
#232392=CARTESIAN_POINT('Ctrl Pts',(-10.6342173268177,-43.9564181735769,
-269.016885));
#232393=CARTESIAN_POINT('Ctrl Pts',(4.25999630922143,-51.1400444377006,
-255.550151));
#232394=CARTESIAN_POINT('Ctrl Pts',(11.707103127241,-54.7318575697624,-248.816784));
#232395=CARTESIAN_POINT('Ctrl Pts',(19.1542099452605,-58.3236707018242,
-242.083417));
#232396=CARTESIAN_POINT('Ctrl Pts',(26.60131676328,-61.915483833886,-235.35005));
#232397=CARTESIAN_POINT('Ctrl Pts',(33.9746898504281,-65.4717344596898,
-228.68335));
#232398=CARTESIAN_POINT('Ctrl Pts',(41.3480800753329,-69.0263711060389,
-222.01665));
#232399=CARTESIAN_POINT('Ctrl Pts',(48.7214815967444,-72.5793938958684,
-215.34995));
#232400=CARTESIAN_POINT('Ctrl Pts',(48.7952156119585,-72.6149241237667,
-215.283283));
#232401=CARTESIAN_POINT('Ctrl Pts',(48.8689496271726,-72.6504543516649,
-215.216616));
#232402=CARTESIAN_POINT('Ctrl Pts',(48.9426836423867,-72.6859845795632,
-215.149949));
#232403=CARTESIAN_POINT('Ctrl Pts',(-122.462954995176,14.8850491441897,
-376.750756999999));
#232404=CARTESIAN_POINT('Ctrl Pts',(-93.6929514318907,0.455210077637512,
-349.817289));
#232405=CARTESIAN_POINT('Ctrl Pts',(-64.9229478686056,-13.9746289889147,
-322.883821));
#232406=CARTESIAN_POINT('Ctrl Pts',(-36.1529443053205,-28.4044680554669,
-295.950353));
#232407=CARTESIAN_POINT('Ctrl Pts',(-21.7679425236779,-35.619387588743,
-282.483619));
#232408=CARTESIAN_POINT('Ctrl Pts',(-7.38294074203528,-42.834307122019,
-269.016885));
#232409=CARTESIAN_POINT('Ctrl Pts',(7.00206103960729,-50.0492266552951,
-255.550151));
#232410=CARTESIAN_POINT('Ctrl Pts',(14.1945619304286,-53.6566864219332,
-248.816784));
#232411=CARTESIAN_POINT('Ctrl Pts',(21.3870628212499,-57.2641461885712,
-242.083417));
#232412=CARTESIAN_POINT('Ctrl Pts',(28.5795637120712,-60.8716059552093,
-235.35005));
#232413=CARTESIAN_POINT('Ctrl Pts',(35.7008517227853,-64.4433482984152,
-228.68335));
#232414=CARTESIAN_POINT('Ctrl Pts',(42.8222003234286,-68.0129932767448,
-222.01665));
#232415=CARTESIAN_POINT('Ctrl Pts',(49.9436019193987,-71.5805410003109,
-215.34995));
#232416=CARTESIAN_POINT('Ctrl Pts',(50.0148159353584,-71.6162164775466,
-215.283283));
#232417=CARTESIAN_POINT('Ctrl Pts',(50.0860299513181,-71.6518919547823,
-215.216616));
#232418=CARTESIAN_POINT('Ctrl Pts',(50.1572439672778,-71.687567432018,-215.149949));
#232419=CARTESIAN_POINT('Ctrl Pts',(-103.0219124536,22.8222305961756,-376.750757000007));
#232420=CARTESIAN_POINT('Ctrl Pts',(-77.174697282254,7.34909250165779,-349.817289000007));
#232421=CARTESIAN_POINT('Ctrl Pts',(-51.3274821109085,-8.12404559286004,
-322.883821000005));
#232422=CARTESIAN_POINT('Ctrl Pts',(-25.480266939563,-23.5971836873778,
-295.950353000003));
#232423=CARTESIAN_POINT('Ctrl Pts',(-12.5566593538902,-31.3337527346368,
-282.483619000003));
#232424=CARTESIAN_POINT('Ctrl Pts',(0.366948231782582,-39.0703217818957,
-269.016885000003));
#232425=CARTESIAN_POINT('Ctrl Pts',(13.2905558174553,-46.8068908291546,
-255.550151000002));
#232426=CARTESIAN_POINT('Ctrl Pts',(19.7523596102917,-50.6751753527841,
-248.816784000002));
#232427=CARTESIAN_POINT('Ctrl Pts',(26.2141634031281,-54.5434598764135,
-242.083417000001));
#232428=CARTESIAN_POINT('Ctrl Pts',(32.6759671959645,-58.411744400043,-235.350050000001));
#232429=CARTESIAN_POINT('Ctrl Pts',(39.0737927334262,-62.2417290769038,
-228.683350000001));
#232430=CARTESIAN_POINT('Ctrl Pts',(45.4718450018044,-66.0691978041651,
-222.01665));
#232431=CARTESIAN_POINT('Ctrl Pts',(51.8701148758579,-69.894150514329,-215.34995));
#232432=CARTESIAN_POINT('Ctrl Pts',(51.9340975745985,-69.9324000414307,
-215.283283));
#232433=CARTESIAN_POINT('Ctrl Pts',(51.998080273339,-69.9706495685323,-215.216616));
#232434=CARTESIAN_POINT('Ctrl Pts',(52.0620629720796,-70.0088990956339,
-215.149949));
#232435=CARTESIAN_POINT('Ctrl Pts',(-71.4332298554826,45.3676034181815,
-376.750756999996));
#232436=CARTESIAN_POINT('Ctrl Pts',(-50.4371334176971,26.5324811107851,
-349.817288999997));
#232437=CARTESIAN_POINT('Ctrl Pts',(-29.4410369799117,7.69735880338874,
-322.883820999997));
#232438=CARTESIAN_POINT('Ctrl Pts',(-8.44494054212614,-11.1377635040076,
-295.950352999998));
#232439=CARTESIAN_POINT('Ctrl Pts',(2.05310767676661,-20.5553246577058,
-282.483618999998));
#232440=CARTESIAN_POINT('Ctrl Pts',(12.5511558956594,-29.972885811404,-269.016884999999));
#232441=CARTESIAN_POINT('Ctrl Pts',(23.0492041145521,-39.3904469651022,
-255.550150999999));
#232442=CARTESIAN_POINT('Ctrl Pts',(28.2982282239985,-44.0992275419513,
-248.816783999999));
#232443=CARTESIAN_POINT('Ctrl Pts',(33.5472523334448,-48.8080081188004,
-242.083416999999));
#232444=CARTESIAN_POINT('Ctrl Pts',(38.7962764428913,-53.5167886956495,
-235.35005));
#232445=CARTESIAN_POINT('Ctrl Pts',(43.9933300166005,-58.1789476826288,
-228.68335));
#232446=CARTESIAN_POINT('Ctrl Pts',(49.1909136386903,-62.839044754287,-222.01665));
#232447=CARTESIAN_POINT('Ctrl Pts',(54.3890197977427,-67.4970794092701,
-215.34995));
#232448=CARTESIAN_POINT('Ctrl Pts',(54.4410008593333,-67.5436597558199,
-215.283283));
#232449=CARTESIAN_POINT('Ctrl Pts',(54.4929819209238,-67.5902401023698,
-215.216616));
#232450=CARTESIAN_POINT('Ctrl Pts',(54.5449629825143,-67.6368204489196,
-215.149949));
#232451=CARTESIAN_POINT('Ctrl Pts',(-45.0390725903934,73.7599134480721,
-376.750757000003));
#232452=CARTESIAN_POINT('Ctrl Pts',(-28.0469137085574,50.6061693294573,
-349.817289000002));
#232453=CARTESIAN_POINT('Ctrl Pts',(-11.0547548267215,27.4524252108426,
-322.883821000002));
#232454=CARTESIAN_POINT('Ctrl Pts',(5.93740405511448,4.29868109222778,-295.950353000001));
#232455=CARTESIAN_POINT('Ctrl Pts',(14.4334834960324,-7.2781909670796,-282.483619000001));
#232456=CARTESIAN_POINT('Ctrl Pts',(22.9295629369504,-18.855063026387,-269.016885000001));
#232457=CARTESIAN_POINT('Ctrl Pts',(31.4256423778684,-30.4319350856944,
-255.550151000001));
#232458=CARTESIAN_POINT('Ctrl Pts',(35.6736820983274,-36.2203711153481,
-248.816784000001));
#232459=CARTESIAN_POINT('Ctrl Pts',(39.9217218187864,-42.0088071450018,
-242.083417000001));
#232460=CARTESIAN_POINT('Ctrl Pts',(44.1697615392454,-47.7972431746554,
-235.35005));
#232461=CARTESIAN_POINT('Ctrl Pts',(48.3757414604919,-53.5283679564908,
-228.68335));
#232462=CARTESIAN_POINT('Ctrl Pts',(52.582425249623,-59.2584041216488,-222.01665));
#232463=CARTESIAN_POINT('Ctrl Pts',(56.7898089004066,-64.9873508559399,
-215.34995));
#232464=CARTESIAN_POINT('Ctrl Pts',(56.8318827369145,-65.0446403232828,
-215.283283));
#232465=CARTESIAN_POINT('Ctrl Pts',(56.8739565734223,-65.1019297906258,
-215.216616));
#232466=CARTESIAN_POINT('Ctrl Pts',(56.9160304099302,-65.1592192579687,
-215.149949));
#232467=CARTESIAN_POINT('Ctrl Pts',(-34.4954719600033,91.6721063226136,
-376.750757));
#232468=CARTESIAN_POINT('Ctrl Pts',(-18.9810705532065,65.8496728858911,
-349.817289000001));
#232469=CARTESIAN_POINT('Ctrl Pts',(-3.46666914640964,40.0272394491684,
-322.883821));
#232470=CARTESIAN_POINT('Ctrl Pts',(12.0477322603872,14.2048060124459,-295.950353));
#232471=CARTESIAN_POINT('Ctrl Pts',(19.8049329637856,1.2935892940846,-282.483619));
#232472=CARTESIAN_POINT('Ctrl Pts',(27.562133667184,-11.6176274242767,-269.016885));
#232473=CARTESIAN_POINT('Ctrl Pts',(35.3193343705824,-24.528844142638,-255.550151));
#232474=CARTESIAN_POINT('Ctrl Pts',(39.1979347222817,-30.9844525018186,
-248.816784));
#232475=CARTESIAN_POINT('Ctrl Pts',(43.0765350739809,-37.4400608609993,
-242.083417));
#232476=CARTESIAN_POINT('Ctrl Pts',(46.9551354256801,-43.8956692201799,
-235.35005));
#232477=CARTESIAN_POINT('Ctrl Pts',(50.7953337936991,-50.2873606649132,
-228.68335));
#232478=CARTESIAN_POINT('Ctrl Pts',(54.6361431746697,-56.6785834369767,
-222.01665));
#232479=CARTESIAN_POINT('Ctrl Pts',(58.477561814447,-63.069336786611,-215.34995));
#232480=CARTESIAN_POINT('Ctrl Pts',(58.5159760008448,-63.1332443201074,
-215.283283));
#232481=CARTESIAN_POINT('Ctrl Pts',(58.5543901872426,-63.1971518536037,
-215.216616));
#232482=CARTESIAN_POINT('Ctrl Pts',(58.5928043736403,-63.2610593871,-215.149949));
#232483=CARTESIAN_POINT('Ctrl Pts',(-31.8464935875069,98.4079754366887,
-376.750756999999));
#232484=CARTESIAN_POINT('Ctrl Pts',(-16.6079109017479,71.6637374050134,
-349.817289));
#232485=CARTESIAN_POINT('Ctrl Pts',(-1.36932821598904,44.919499373338,-322.883821));
#232486=CARTESIAN_POINT('Ctrl Pts',(13.8692544697699,18.1752613416626,-295.950353));
#232487=CARTESIAN_POINT('Ctrl Pts',(21.4885458126493,4.80314232582491,-282.483619));
#232488=CARTESIAN_POINT('Ctrl Pts',(29.1078371555287,-8.56897669001278,
-269.016885));
#232489=CARTESIAN_POINT('Ctrl Pts',(36.7271284984082,-21.9410957058504,
-255.550151));
#232490=CARTESIAN_POINT('Ctrl Pts',(40.5367741698479,-28.6271552137693,
-248.816784));
#232491=CARTESIAN_POINT('Ctrl Pts',(44.3464198412877,-35.3132147216881,
-242.083417));
#232492=CARTESIAN_POINT('Ctrl Pts',(48.1560655127274,-41.999274229607,-235.35005));
#232493=CARTESIAN_POINT('Ctrl Pts',(51.9279919200935,-48.6191351285365,
-228.68335));
#232494=CARTESIAN_POINT('Ctrl Pts',(55.7004001286368,-55.2387363218615,
-222.01665));
#232495=CARTESIAN_POINT('Ctrl Pts',(59.4732891526772,-61.8580772083615,
-215.34995));
#232496=CARTESIAN_POINT('Ctrl Pts',(59.5110180429176,-61.9242706172265,
-215.283283));
#232497=CARTESIAN_POINT('Ctrl Pts',(59.548746933158,-61.9904640260915,-215.216616));
#232498=CARTESIAN_POINT('Ctrl Pts',(59.5864758233984,-62.0566574349565,
-215.149949));
#232499=CARTESIAN_POINT('Ctrl Pts',(-21.2505800975213,125.351451892989,
-376.750756999997));
#232500=CARTESIAN_POINT('Ctrl Pts',(-7.11527229591406,94.9199954815027,
-349.817288999997));
#232501=CARTESIAN_POINT('Ctrl Pts',(7.02003550569317,64.4885390700161,-322.883820999998));
#232502=CARTESIAN_POINT('Ctrl Pts',(21.1553433073004,34.0570826585295,-295.950352999998));
#232503=CARTESIAN_POINT('Ctrl Pts',(28.222997208104,18.8413544527863,-282.483618999999));
#232504=CARTESIAN_POINT('Ctrl Pts',(35.2906511089077,3.62562624704296,-269.016884999999));
#232505=CARTESIAN_POINT('Ctrl Pts',(42.3583050097113,-11.5901019587003,
-255.550151));
#232506=CARTESIAN_POINT('Ctrl Pts',(45.8921319601131,-19.197966061572,-248.816784));
#232507=CARTESIAN_POINT('Ctrl Pts',(49.4259589105149,-26.8058301644436,
-242.083417));
#232508=CARTESIAN_POINT('Ctrl Pts',(52.9597858609167,-34.4136942673153,
-235.35005));
#232509=CARTESIAN_POINT('Ctrl Pts',(56.458624425671,-41.9462329830297,-228.68335));
#232510=CARTESIAN_POINT('Ctrl Pts',(59.957427944505,-49.4793478614006,-222.01665));
#232511=CARTESIAN_POINT('Ctrl Pts',(63.4561985055979,-57.0130388953633,
-215.34995));
#232512=CARTESIAN_POINT('Ctrl Pts',(63.4911862112088,-57.0883758057029,
-215.283283));
#232513=CARTESIAN_POINT('Ctrl Pts',(63.5261739168198,-57.1637127160426,
-215.216616));
#232514=CARTESIAN_POINT('Ctrl Pts',(63.5611616224307,-57.2390496263822,
-215.149949));
#232515=CARTESIAN_POINT('Ctrl Pts',(-10.6546666075359,152.29492834929,-376.750756999995));
#232516=CARTESIAN_POINT('Ctrl Pts',(2.37736630991967,118.176253557992,-349.817288999995));
#232517=CARTESIAN_POINT('Ctrl Pts',(15.4093992273753,84.0575787666943,-322.883820999996));
#232518=CARTESIAN_POINT('Ctrl Pts',(28.4414321448309,49.9389039753965,-295.950352999998));
#232519=CARTESIAN_POINT('Ctrl Pts',(34.9574486035587,32.8795665797476,-282.483618999998));
#232520=CARTESIAN_POINT('Ctrl Pts',(41.4734650622865,15.8202291840987,-269.016884999999));
#232521=CARTESIAN_POINT('Ctrl Pts',(47.9894815210143,-1.2391082115502,-255.550151));
#232522=CARTESIAN_POINT('Ctrl Pts',(51.2474897503782,-9.76877690937465,
-248.816784));
#232523=CARTESIAN_POINT('Ctrl Pts',(54.5054979797421,-18.2984456071991,
-242.083417));
#232524=CARTESIAN_POINT('Ctrl Pts',(57.763506209106,-26.8281143050236,-235.35005));
#232525=CARTESIAN_POINT('Ctrl Pts',(60.9892569312485,-35.273330837523,-228.683350000001));
#232526=CARTESIAN_POINT('Ctrl Pts',(64.2144557603733,-43.7199594009398,
-222.016650000001));
#232527=CARTESIAN_POINT('Ctrl Pts',(67.4391078585187,-52.1680005823651,
-215.349950000001));
#232528=CARTESIAN_POINT('Ctrl Pts',(67.4713543795001,-52.2524809941794,
-215.283283000001));
#232529=CARTESIAN_POINT('Ctrl Pts',(67.5036009004816,-52.3369614059937,
-215.216616));
#232530=CARTESIAN_POINT('Ctrl Pts',(67.535847421463,-52.4214418178079,-215.149949000001));
#232531=CARTESIAN_POINT('Ctrl Pts',(-0.0587531175507312,179.238404805591,
-376.750756999993));
#232532=CARTESIAN_POINT('Ctrl Pts',(11.8700049157533,141.432511634481,-349.817288999993));
#232533=CARTESIAN_POINT('Ctrl Pts',(23.7987629490573,103.626618463372,-322.883820999995));
#232534=CARTESIAN_POINT('Ctrl Pts',(35.7275209823613,65.8207252922634,-295.950352999997));
#232535=CARTESIAN_POINT('Ctrl Pts',(41.6918999990133,46.9177787067089,-282.483618999997));
#232536=CARTESIAN_POINT('Ctrl Pts',(47.6562790156653,28.0148321211544,-269.016884999998));
#232537=CARTESIAN_POINT('Ctrl Pts',(53.6206580323173,9.11188553559992,-255.550150999999));
#232538=CARTESIAN_POINT('Ctrl Pts',(56.6028475406433,-0.339587757177323,
-248.816784));
#232539=CARTESIAN_POINT('Ctrl Pts',(59.5850370489693,-9.79106104995457,
-242.083416999999));
#232540=CARTESIAN_POINT('Ctrl Pts',(62.5672265572953,-19.2425343427318,
-235.35005));
#232541=CARTESIAN_POINT('Ctrl Pts',(65.519889436826,-28.6004286920162,-228.683350000001));
#232542=CARTESIAN_POINT('Ctrl Pts',(68.4714835762416,-37.9605709404789,
-222.016650000001));
#232543=CARTESIAN_POINT('Ctrl Pts',(71.4220172114394,-47.322962269367,-215.349950000001));
#232544=CARTESIAN_POINT('Ctrl Pts',(71.4515225477914,-47.4165861826559,
-215.283283000001));
#232545=CARTESIAN_POINT('Ctrl Pts',(71.4810278841433,-47.5102100959448,
-215.216616));
#232546=CARTESIAN_POINT('Ctrl Pts',(71.5105332204953,-47.6038340092336,
-215.149949000001));
#232547=CARTESIAN_POINT('Ctrl Pts',(31.728987352405,260.068834174492,-376.750756999986));
#232548=CARTESIAN_POINT('Ctrl Pts',(40.3479207332542,211.20128586395,-349.817288999988));
#232549=CARTESIAN_POINT('Ctrl Pts',(48.9668541141034,162.333737553407,-322.883820999991));
#232550=CARTESIAN_POINT('Ctrl Pts',(57.5857874949526,113.466189242864,-295.950352999994));
#232551=CARTESIAN_POINT('Ctrl Pts',(61.8952541853772,89.0324150875929,-282.483618999995));
#232552=CARTESIAN_POINT('Ctrl Pts',(66.2047208758018,64.5986409323216,-269.016884999996));
#232553=CARTESIAN_POINT('Ctrl Pts',(70.5141875662264,40.1648667770503,-255.550150999998));
#232554=CARTESIAN_POINT('Ctrl Pts',(72.6689209114386,27.9479796994146,-248.816783999999));
#232555=CARTESIAN_POINT('Ctrl Pts',(74.8236542566509,15.731092621779,-242.083416999999));
#232556=CARTESIAN_POINT('Ctrl Pts',(76.9783876018632,3.51420554414337,-235.35005));
#232557=CARTESIAN_POINT('Ctrl Pts',(79.1117869535586,-8.58172225549588,
-228.683350000001));
#232558=CARTESIAN_POINT('Ctrl Pts',(81.2425670238464,-20.6824055590965,
-222.016650000001));
#232559=CARTESIAN_POINT('Ctrl Pts',(83.3707452702016,-32.7878473303725,
-215.349950000001));
#232560=CARTESIAN_POINT('Ctrl Pts',(83.3920270526652,-32.9089017480852,
-215.283283000001));
#232561=CARTESIAN_POINT('Ctrl Pts',(83.4133088351287,-33.0299561657981,
-215.216616));
#232562=CARTESIAN_POINT('Ctrl Pts',(83.4345906175922,-33.1510105835108,
-215.149949000001));
#232563=CARTESIAN_POINT('Ctrl Pts',(63.5167278223608,340.899263543393,-376.750756999979));
#232564=CARTESIAN_POINT('Ctrl Pts',(68.8258365507552,280.970060093418,-349.817288999983));
#232565=CARTESIAN_POINT('Ctrl Pts',(74.1349452791495,221.040856643441,-322.883820999986));
#232566=CARTESIAN_POINT('Ctrl Pts',(79.4440540075439,161.111653193465,-295.950352999991));
#232567=CARTESIAN_POINT('Ctrl Pts',(82.098608371741,131.147051468477,-282.483618999993));
#232568=CARTESIAN_POINT('Ctrl Pts',(84.7531627359382,101.182449743489,-269.016884999995));
#232569=CARTESIAN_POINT('Ctrl Pts',(87.4077171001354,71.2178480185007,-255.550150999997));
#232570=CARTESIAN_POINT('Ctrl Pts',(88.734994282234,56.2355471560066,-248.816783999998));
#232571=CARTESIAN_POINT('Ctrl Pts',(90.0622714643326,41.2532462935126,-242.083416999999));
#232572=CARTESIAN_POINT('Ctrl Pts',(91.3895486464312,26.2709454310185,-235.35005));
#232573=CARTESIAN_POINT('Ctrl Pts',(92.7036844702911,11.4369841810244,-228.683350000001));
#232574=CARTESIAN_POINT('Ctrl Pts',(94.0136504714512,-3.40424017771396,
-222.016650000001));
#232575=CARTESIAN_POINT('Ctrl Pts',(95.3194733289638,-18.252732391378,-215.349950000001));
#232576=CARTESIAN_POINT('Ctrl Pts',(95.3325315575389,-18.4012173135146,
-215.283283000001));
#232577=CARTESIAN_POINT('Ctrl Pts',(95.345589786114,-18.5497022356513,-215.216616000001));
#232578=CARTESIAN_POINT('Ctrl Pts',(95.3586480146891,-18.698187157788,-215.149949000001));
#232579=CARTESIAN_POINT('Ctrl Pts',(95.3044682923166,421.729692912295,-376.750756999971));
#232580=CARTESIAN_POINT('Ctrl Pts',(97.3037523682561,350.738834322885,-349.817288999976));
#232581=CARTESIAN_POINT('Ctrl Pts',(99.3030364441956,279.747975733475,-322.883820999982));
#232582=CARTESIAN_POINT('Ctrl Pts',(101.302320520135,208.757117144065,-295.950352999988));
#232583=CARTESIAN_POINT('Ctrl Pts',(102.301962558105,173.261687849361,-282.48361899999));
#232584=CARTESIAN_POINT('Ctrl Pts',(103.301604596075,137.766258554656,-269.016884999993));
#232585=CARTESIAN_POINT('Ctrl Pts',(104.301246634044,102.270829259951,-255.550150999996));
#232586=CARTESIAN_POINT('Ctrl Pts',(104.801067653029,84.5231146125986,-248.816783999998));
#232587=CARTESIAN_POINT('Ctrl Pts',(105.300888672014,66.7753999652462,-242.083416999998));
#232588=CARTESIAN_POINT('Ctrl Pts',(105.800709690999,49.0276853178937,-235.35005));
#232589=CARTESIAN_POINT('Ctrl Pts',(106.295581987024,31.4556906175448,-228.683350000001));
#232590=CARTESIAN_POINT('Ctrl Pts',(106.784733919056,13.8739252036685,-222.016650000002));
#232591=CARTESIAN_POINT('Ctrl Pts',(107.268201387726,-3.71761745238349,
-215.349950000002));
#232592=CARTESIAN_POINT('Ctrl Pts',(107.273036062413,-3.89353287894403,
-215.283283000002));
#232593=CARTESIAN_POINT('Ctrl Pts',(107.277870737099,-4.06944830550458,
-215.216616000002));
#232594=CARTESIAN_POINT('Ctrl Pts',(107.282705411786,-4.24536373206513,
-215.149949000001));
#232595=CARTESIAN_POINT('Ctrl Pts',(190.667689702184,664.220981018999,-376.750756999951));
#232596=CARTESIAN_POINT('Ctrl Pts',(182.737499820759,560.045157011288,-349.81728899996));
#232597=CARTESIAN_POINT('Ctrl Pts',(174.807309939334,455.869333003578,-322.883820999969));
#232598=CARTESIAN_POINT('Ctrl Pts',(166.877120057909,351.693508995868,-295.950352999979));
#232599=CARTESIAN_POINT('Ctrl Pts',(162.912025117196,299.605596992013,-282.483618999983));
#232600=CARTESIAN_POINT('Ctrl Pts',(158.946930176484,247.517684988157,-269.016884999988));
#232601=CARTESIAN_POINT('Ctrl Pts',(154.981835235771,195.429772984302,-255.550150999993));
#232602=CARTESIAN_POINT('Ctrl Pts',(152.999287765415,169.385816982375,-248.816783999995));
#232603=CARTESIAN_POINT('Ctrl Pts',(151.016740295059,143.341860980447,-242.083416999997));
#232604=CARTESIAN_POINT('Ctrl Pts',(149.034192824703,117.297904978519,-235.35005));
#232605=CARTESIAN_POINT('Ctrl Pts',(147.071274537221,91.5118099271058,-228.683350000003));
#232606=CARTESIAN_POINT('Ctrl Pts',(145.09798426187,65.708421347816,-222.016650000002));
#232607=CARTESIAN_POINT('Ctrl Pts',(143.114385564013,39.8877273646,-215.349950000003));
#232608=CARTESIAN_POINT('Ctrl Pts',(143.094549577034,39.6295204247678,-215.283283000003));
#232609=CARTESIAN_POINT('Ctrl Pts',(143.074713590055,39.3713134849356,-215.216616000002));
#232610=CARTESIAN_POINT('Ctrl Pts',(143.054877603077,39.1131065451034,-215.149949000002));
#232611=CARTESIAN_POINT('Ctrl Pts',(286.030911112051,906.712269125702,-376.750756999929));
#232612=CARTESIAN_POINT('Ctrl Pts',(268.171247273262,769.351479699691,-349.817288999943));
#232613=CARTESIAN_POINT('Ctrl Pts',(250.311583434473,631.990690273681,-322.883820999956));
#232614=CARTESIAN_POINT('Ctrl Pts',(232.451919595683,494.62990084767,-295.95035299997));
#232615=CARTESIAN_POINT('Ctrl Pts',(223.522087676288,425.949506134664,-282.483618999976));
#232616=CARTESIAN_POINT('Ctrl Pts',(214.592255756894,357.269111421658,-269.016884999983));
#232617=CARTESIAN_POINT('Ctrl Pts',(205.662423837499,288.588716708654,-255.55015099999));
#232618=CARTESIAN_POINT('Ctrl Pts',(201.197507877801,254.24851935215,-248.816783999994));
#232619=CARTESIAN_POINT('Ctrl Pts',(196.732591918104,219.908321995647,-242.083416999997));
#232620=CARTESIAN_POINT('Ctrl Pts',(192.267675958407,185.568124639145,-235.35005));
#232621=CARTESIAN_POINT('Ctrl Pts',(187.846967087419,151.567929236667,-228.683350000004));
#232622=CARTESIAN_POINT('Ctrl Pts',(183.411234604685,117.542917491964,-222.016650000003));
#232623=CARTESIAN_POINT('Ctrl Pts',(178.960569740299,83.4930721815835,-215.349950000004));
#232624=CARTESIAN_POINT('Ctrl Pts',(178.916063091656,83.1525737284796,-215.283283000004));
#232625=CARTESIAN_POINT('Ctrl Pts',(178.871556443012,82.8120752753758,-215.216616000004));
#232626=CARTESIAN_POINT('Ctrl Pts',(178.827049794367,82.4715768222719,-215.149949000004));
#232627=CARTESIAN_POINT('Ctrl Pts',(381.394132521918,1149.20355723241,-376.750756999909));
#232628=CARTESIAN_POINT('Ctrl Pts',(353.604994725765,978.657802388094,-349.817288999926));
#232629=CARTESIAN_POINT('Ctrl Pts',(325.815856929611,808.112047543783,-322.883820999944));
#232630=CARTESIAN_POINT('Ctrl Pts',(298.026719133457,637.566292699472,-295.950352999961));
#232631=CARTESIAN_POINT('Ctrl Pts',(284.13215023538,552.293415277316,-282.48361899997));
#232632=CARTESIAN_POINT('Ctrl Pts',(270.237581337303,467.02053785516,-269.016884999978));
#232633=CARTESIAN_POINT('Ctrl Pts',(256.343012439226,381.747660433005,-255.550150999987));
#232634=CARTESIAN_POINT('Ctrl Pts',(249.395727990188,339.111221721927,-248.816783999992));
#232635=CARTESIAN_POINT('Ctrl Pts',(242.448443541149,296.474783010849,-242.083416999996));
#232636=CARTESIAN_POINT('Ctrl Pts',(235.501159092111,253.83834429977,-235.35005));
#232637=CARTESIAN_POINT('Ctrl Pts',(228.622659637617,211.624048546228,-228.683350000005));
#232638=CARTESIAN_POINT('Ctrl Pts',(221.724484947499,169.377413636111,-222.016650000005));
#232639=CARTESIAN_POINT('Ctrl Pts',(214.806753916586,127.098416998567,-215.349950000004));
#232640=CARTESIAN_POINT('Ctrl Pts',(214.737576606277,126.675627032191,-215.283283000005));
#232641=CARTESIAN_POINT('Ctrl Pts',(214.668399295968,126.252837065816,-215.216616000005));
#232642=CARTESIAN_POINT('Ctrl Pts',(214.599221985659,125.83004709944,-215.149949000005));
#232643=CARTESIAN_POINT('Ctrl Pts',(667.483796751521,1876.67742155251,-376.750756999846));
#232644=CARTESIAN_POINT('Ctrl Pts',(609.906237083273,1606.57677045331,-349.817288999875));
#232645=CARTESIAN_POINT('Ctrl Pts',(552.328677415026,1336.47611935409,-322.883820999905));
#232646=CARTESIAN_POINT('Ctrl Pts',(494.751117746779,1066.37546825488,-295.950352999934));
#232647=CARTESIAN_POINT('Ctrl Pts',(465.962337912655,931.325142705271,-282.483618999949));
#232648=CARTESIAN_POINT('Ctrl Pts',(437.173558078531,796.274817155664,-269.016884999963));
#232649=CARTESIAN_POINT('Ctrl Pts',(408.384778244408,661.224491606058,-255.550150999978));
#232650=CARTESIAN_POINT('Ctrl Pts',(393.990388327346,593.699328831254,-248.816783999986));
#232651=CARTESIAN_POINT('Ctrl Pts',(379.595998410284,526.174166056451,-242.083416999993));
#232652=CARTESIAN_POINT('Ctrl Pts',(365.201608493222,458.649003281647,-235.35005));
#232653=CARTESIAN_POINT('Ctrl Pts',(350.94973728821,391.792406474911,-228.683350000008));
#232654=CARTESIAN_POINT('Ctrl Pts',(336.664235975943,324.880902068554,-222.016650000008));
#232655=CARTESIAN_POINT('Ctrl Pts',(322.345306445446,257.914451449517,-215.349950000008));
#232656=CARTESIAN_POINT('Ctrl Pts',(322.202117150141,257.244786943327,-215.283283000008));
#232657=CARTESIAN_POINT('Ctrl Pts',(322.058927854835,256.575122437136,-215.216616000008));
#232658=CARTESIAN_POINT('Ctrl Pts',(321.91573855953,255.905457930946,-215.149949000007));
#232659=CARTESIAN_POINT('Ctrl Pts',(953.573460981123,2604.15128587263,-376.750756999783));
#232660=CARTESIAN_POINT('Ctrl Pts',(866.207479440782,2234.49573851851,-349.817288999824));
#232661=CARTESIAN_POINT('Ctrl Pts',(778.841497900441,1864.8401911644,-322.883820999866));
#232662=CARTESIAN_POINT('Ctrl Pts',(691.4755163601,1495.18464381028,-295.950352999906));
#232663=CARTESIAN_POINT('Ctrl Pts',(647.79252558993,1310.35687013323,-282.483618999927));
#232664=CARTESIAN_POINT('Ctrl Pts',(604.109534819759,1125.52909645617,-269.016884999948));
#232665=CARTESIAN_POINT('Ctrl Pts',(560.426544049589,940.701322779111,-255.550150999969));
#232666=CARTESIAN_POINT('Ctrl Pts',(538.585048664503,848.287435940582,-248.81678399998));
#232667=CARTESIAN_POINT('Ctrl Pts',(516.743553279418,755.873549102053,-242.08341699999));
#232668=CARTESIAN_POINT('Ctrl Pts',(494.902057894333,663.459662263524,-235.35005));
#232669=CARTESIAN_POINT('Ctrl Pts',(473.276814938803,571.960764403594,-228.683350000011));
#232670=CARTESIAN_POINT('Ctrl Pts',(451.603987004386,480.384390500996,-222.016650000011));
#232671=CARTESIAN_POINT('Ctrl Pts',(429.883858974306,388.730485900468,-215.34995000001));
#232672=CARTESIAN_POINT('Ctrl Pts',(429.666657694005,387.813946854463,-215.28328300001));
#232673=CARTESIAN_POINT('Ctrl Pts',(429.449456413704,386.897407808457,-215.216616000011));
#232674=CARTESIAN_POINT('Ctrl Pts',(429.232255133403,385.980868762451,-215.149949000011));
#232675=CARTESIAN_POINT('Ctrl Pts',(1239.66312521072,3331.62515019274,-376.750756999719));
#232676=CARTESIAN_POINT('Ctrl Pts',(1122.50872179829,2862.41470658373,-349.817288999773));
#232677=CARTESIAN_POINT('Ctrl Pts',(1005.35431838586,2393.20426297471,-322.883820999826));
#232678=CARTESIAN_POINT('Ctrl Pts',(888.199914973422,1923.99381936569,-295.95035299988));
#232679=CARTESIAN_POINT('Ctrl Pts',(829.622713267204,1689.38859756118,-282.483618999906));
#232680=CARTESIAN_POINT('Ctrl Pts',(771.045511560987,1454.78337575667,-269.016884999933));
#232681=CARTESIAN_POINT('Ctrl Pts',(712.46830985477,1220.17815395216,-255.55015099996));
#232682=CARTESIAN_POINT('Ctrl Pts',(683.179709001661,1102.87554304991,-248.816783999974));
#232683=CARTESIAN_POINT('Ctrl Pts',(653.891108148553,985.572932147655,-242.083416999987));
#232684=CARTESIAN_POINT('Ctrl Pts',(624.602507295445,868.2703212454,-235.35005));
#232685=CARTESIAN_POINT('Ctrl Pts',(595.603892589396,752.129122332277,-228.683350000014));
#232686=CARTESIAN_POINT('Ctrl Pts',(566.54373803283,635.887878933439,-222.016650000014));
#232687=CARTESIAN_POINT('Ctrl Pts',(537.422411503166,519.546520351418,-215.349950000014));
#232688=CARTESIAN_POINT('Ctrl Pts',(537.131198237869,518.383106765598,-215.283283000013));
#232689=CARTESIAN_POINT('Ctrl Pts',(536.839984972572,517.219693179777,-215.216616000014));
#232690=CARTESIAN_POINT('Ctrl Pts',(536.548771707275,516.056279593957,-215.149949000014));
#232691=CARTESIAN_POINT('Ctrl Pts',(2097.93211789953,5514.04674315307,-376.750756999531));
#232692=CARTESIAN_POINT('Ctrl Pts',(1891.41244887082,4746.17161077935,-349.81728899962));
#232693=CARTESIAN_POINT('Ctrl Pts',(1684.8927798421,3978.29647840563,-322.88382099971));
#232694=CARTESIAN_POINT('Ctrl Pts',(1478.37311081339,3210.42134603191,-295.950352999799));
#232695=CARTESIAN_POINT('Ctrl Pts',(1375.11327629903,2826.48377984504,-282.483618999843));
#232696=CARTESIAN_POINT('Ctrl Pts',(1271.85344178467,2442.54621365819,-269.016884999889));
#232697=CARTESIAN_POINT('Ctrl Pts',(1168.59360727031,2058.60864747133,-255.550150999933));
#232698=CARTESIAN_POINT('Ctrl Pts',(1116.96369001313,1866.6398643779,-248.816783999956));
#232699=CARTESIAN_POINT('Ctrl Pts',(1065.33377275596,1674.67108128446,-242.083416999977));
#232700=CARTESIAN_POINT('Ctrl Pts',(1013.70385549878,1482.70229819103,-235.35005));
#232701=CARTESIAN_POINT('Ctrl Pts',(962.585125541175,1292.63419611833,-228.683350000023));
#232702=CARTESIAN_POINT('Ctrl Pts',(911.362991118159,1102.39834423077,-222.016650000023));
#232703=CARTESIAN_POINT('Ctrl Pts',(860.038069089746,911.99462370427,-215.349950000023));
#232704=CARTESIAN_POINT('Ctrl Pts',(859.524819869462,910.090586499004,-215.283283000022));
#232705=CARTESIAN_POINT('Ctrl Pts',(859.011570649176,908.186549293739,-215.216616000022));
#232706=CARTESIAN_POINT('Ctrl Pts',(858.498321428892,906.282512088474,-215.149949000023));
#232707=CARTESIAN_POINT('Ctrl Pts',(2956.20111058834,7696.4683361134,-376.750756999341));
#232708=CARTESIAN_POINT('Ctrl Pts',(2660.31617594335,6629.92851497498,-349.817288999467));
#232709=CARTESIAN_POINT('Ctrl Pts',(2364.43124129834,5563.38869383655,-322.883820999593));
#232710=CARTESIAN_POINT('Ctrl Pts',(2068.54630665335,4496.84887269812,-295.950352999718));
#232711=CARTESIAN_POINT('Ctrl Pts',(1920.60383933086,3963.57896212891,-282.48361899978));
#232712=CARTESIAN_POINT('Ctrl Pts',(1772.66137200836,3430.3090515597,-269.016884999844));
#232713=CARTESIAN_POINT('Ctrl Pts',(1624.71890468586,2897.03914099049,-255.550150999906));
#232714=CARTESIAN_POINT('Ctrl Pts',(1550.74767102461,2630.40418570588,-248.816783999938));
#232715=CARTESIAN_POINT('Ctrl Pts',(1476.77643736336,2363.76923042127,-242.083416999969));
#232716=CARTESIAN_POINT('Ctrl Pts',(1402.80520370211,2097.13427513666,-235.35005));
#232717=CARTESIAN_POINT('Ctrl Pts',(1329.56635849295,1833.13926990437,-228.683350000032));
#232718=CARTESIAN_POINT('Ctrl Pts',(1256.18224420349,1568.9088095281,-222.016650000032));
#232719=CARTESIAN_POINT('Ctrl Pts',(1182.65372667633,1304.44272705712,-215.349950000032));
#232720=CARTESIAN_POINT('Ctrl Pts',(1181.91844150105,1301.79806623241,-215.283283000032));
#232721=CARTESIAN_POINT('Ctrl Pts',(1181.18315632578,1299.1534054077,-215.216616000032));
#232722=CARTESIAN_POINT('Ctrl Pts',(1180.44787115051,1296.50874458299,-215.149949000032));
#232723=CARTESIAN_POINT('Ctrl Pts',(3814.47010327714,9878.88992907374,-376.750756999153));
#232724=CARTESIAN_POINT('Ctrl Pts',(3429.21990301587,8513.68541917061,-349.817288999315));
#232725=CARTESIAN_POINT('Ctrl Pts',(3043.96970275459,7148.48090926748,-322.883820999476));
#232726=CARTESIAN_POINT('Ctrl Pts',(2658.71950249332,5783.27639936434,-295.950352999637));
#232727=CARTESIAN_POINT('Ctrl Pts',(2466.09440236268,5100.67414441278,-282.483618999717));
#232728=CARTESIAN_POINT('Ctrl Pts',(2273.46930223204,4418.07188946121,-269.016884999799));
#232729=CARTESIAN_POINT('Ctrl Pts',(2080.84420210141,3735.46963450965,-255.550150999879));
#232730=CARTESIAN_POINT('Ctrl Pts',(1984.53165203609,3394.16850703386,-248.81678399992));
#232731=CARTESIAN_POINT('Ctrl Pts',(1888.21910197076,3052.86737955808,-242.08341699996));
#232732=CARTESIAN_POINT('Ctrl Pts',(1791.90655190545,2711.56625208229,-235.35005));
#232733=CARTESIAN_POINT('Ctrl Pts',(1696.54759144473,2373.64434369042,-228.683350000041));
#232734=CARTESIAN_POINT('Ctrl Pts',(1601.00149728882,2035.41927482542,-222.016650000041));
#232735=CARTESIAN_POINT('Ctrl Pts',(1505.26938426291,1696.89083040998,-215.349950000041));
#232736=CARTESIAN_POINT('Ctrl Pts',(1504.31206313264,1693.50554596582,-215.28328300004));
#232737=CARTESIAN_POINT('Ctrl Pts',(1503.35474200239,1690.12026152166,-215.216616000041));
#232738=CARTESIAN_POINT('Ctrl Pts',(1502.39742087213,1686.7349770775,-215.149949000041));
#232739=CARTESIAN_POINT('Origin',(-636.934816028482,-11.5034818258361,-229.35005));
#232740=CARTESIAN_POINT('Origin',(-636.934816028482,-11.5034818258361,-229.35005));
#232741=CARTESIAN_POINT('Origin',(-636.934816028482,-11.5034818258361,-229.35005));
#232742=CARTESIAN_POINT('Origin',(-636.934816028482,-11.5034818258361,-229.35005));
#232743=CARTESIAN_POINT('Origin',(-636.934816028482,-11.5034818258361,-229.35005));
#232744=CARTESIAN_POINT('Origin',(0.,-32.21456093117,-229.35005));
#232745=CARTESIAN_POINT('Origin',(0.,-33.21456093117,-229.35005));
#232746=CARTESIAN_POINT('Origin',(-2.22174260618994E-13,-11.0034818258363,
-229.35005));
#232747=CARTESIAN_POINT('Origin',(-2.22174260618994E-13,-12.0034818258363,
-229.35005));
#232748=CARTESIAN_POINT('Origin',(-1.54373336646987E-15,-42.8201004838369,
-229.35005));
#232749=CARTESIAN_POINT('Origin',(-1.23757166668304E-15,-43.8201004838368,
-229.35005));
#232750=CARTESIAN_POINT('Origin',(-2.8425373731103E-15,9.20759727949731,
-229.35005));
#232751=CARTESIAN_POINT('Origin',(-2.53637567332344E-15,10.2075972794973,
-229.35005));
#232752=CARTESIAN_POINT('Origin',(-1.54373336646988E-15,19.8131368321642,
-229.35005));
#232753=CARTESIAN_POINT('Origin',(-1.23757166668304E-15,20.8131368321642,
-229.35005));
#232754=CARTESIAN_POINT('Origin',(-2.61456814389029E-14,-173.57701443073,
-229.35005));
#232755=CARTESIAN_POINT('Origin',(7.14692237356698E-14,623.509175991979,
-229.35005));
#232756=CARTESIAN_POINT('Origin',(-2.61456814389029E-14,-173.57701443073,
-229.35005));
#232757=CARTESIAN_POINT('Origin',(-2.61456814389029E-14,-173.57701443073,
-232.25005));
#232758=CARTESIAN_POINT('Origin',(-2.61456814389029E-14,-173.57701443073,
-229.35005));
#232759=CARTESIAN_POINT('Origin',(-2.61456814389029E-14,-173.57701443073,
-232.25005));
#232760=CARTESIAN_POINT('Origin',(11.4589044897296,-32.0203896799758,-232.25005));
#232761=CARTESIAN_POINT('Origin',(0.,-32.21456093117,-229.35005));
#232762=CARTESIAN_POINT('Origin',(0.,-33.21456093117,-229.35005));
#232763=CARTESIAN_POINT('Origin',(-3.33261390928491E-13,-21.6090213785032,
-229.35005));
#232764=CARTESIAN_POINT('Origin',(-3.33261390928491E-13,-22.6090213785032,
-229.35005));
#232765=CARTESIAN_POINT('Origin',(-2.22174260618994E-13,-11.0034818258363,
-229.35005));
#232766=CARTESIAN_POINT('Origin',(-2.22174260618994E-13,-12.0034818258363,
-229.35005));
#232767=CARTESIAN_POINT('Origin',(-1.11087130309497E-13,-0.397942273169518,
-229.35005));
#232768=CARTESIAN_POINT('Origin',(-1.11087130309497E-13,-1.3979422731695,
-229.35005));
#232769=CARTESIAN_POINT('Origin',(-1.54373336646987E-15,-42.8201004838369,
-229.35005));
#232770=CARTESIAN_POINT('Origin',(-1.23757166668304E-15,-43.8201004838368,
-229.35005));
#232771=CARTESIAN_POINT('Origin',(-2.8425373731103E-15,9.20759727949731,
-229.35005));
#232772=CARTESIAN_POINT('Origin',(-2.53637567332344E-15,10.2075972794973,
-229.35005));
#232773=CARTESIAN_POINT('Origin',(-1.54373336646988E-15,19.8131368321642,
-229.35005));
#232774=CARTESIAN_POINT('Origin',(-1.23757166668304E-15,20.8131368321642,
-229.35005));
#232775=CARTESIAN_POINT('Origin',(-2.61456814389029E-14,-173.57701443073,
-229.35005));
#232776=CARTESIAN_POINT('Origin',(-2.61456814389029E-14,-173.57701443073,
-229.35005));
#232777=CARTESIAN_POINT('Origin',(7.14692237356698E-14,623.509175991979,
-229.35005));
#232778=CARTESIAN_POINT('Origin',(7.14692237356698E-14,623.509175991979,
-229.35005));
#232779=CARTESIAN_POINT('Origin',(-6.29739814579425E-15,-11.5034818258363,
-229.35005));
#232780=CARTESIAN_POINT('Origin',(-6.29739814579425E-15,-11.5034818258363,
-229.35005));
#232781=CARTESIAN_POINT('Origin',(-6.29739814579425E-15,-11.5034818258363,
-229.35005));
#232782=CARTESIAN_POINT('Origin',(-6.29739814579425E-15,-11.5034818258363,
-229.35005));
#232783=CARTESIAN_POINT('Origin',(0.,-32.21456093117,-229.35005));
#232784=CARTESIAN_POINT('Origin',(0.,-32.21456093117,-229.35005));
#232785=CARTESIAN_POINT('Origin',(0.,-33.21456093117,-229.35005));
#232786=CARTESIAN_POINT('Origin',(0.,-33.21456093117,-229.35005));
#232787=CARTESIAN_POINT('Origin',(-3.33261390928491E-13,-21.6090213785032,
-229.35005));
#232788=CARTESIAN_POINT('Origin',(-3.33261390928491E-13,-21.6090213785032,
-229.35005));
#232789=CARTESIAN_POINT('Origin',(-3.33261390928491E-13,-22.6090213785032,
-229.35005));
#232790=CARTESIAN_POINT('Origin',(-3.33261390928491E-13,-22.6090213785032,
-229.35005));
#232791=CARTESIAN_POINT('Origin',(-2.22174260618994E-13,-11.0034818258363,
-229.35005));
#232792=CARTESIAN_POINT('Origin',(-2.22174260618994E-13,-11.0034818258363,
-229.35005));
#232793=CARTESIAN_POINT('Origin',(-2.22174260618994E-13,-12.0034818258363,
-229.35005));
#232794=CARTESIAN_POINT('Origin',(-2.22174260618994E-13,-12.0034818258363,
-229.35005));
#232795=CARTESIAN_POINT('Origin',(-1.11087130309497E-13,-0.397942273169518,
-229.35005));
#232796=CARTESIAN_POINT('Origin',(-1.11087130309497E-13,-0.397942273169518,
-229.35005));
#232797=CARTESIAN_POINT('Origin',(-1.11087130309497E-13,-1.3979422731695,
-229.35005));
#232798=CARTESIAN_POINT('Origin',(-1.11087130309497E-13,-1.3979422731695,
-229.35005));
#232799=CARTESIAN_POINT('Origin',(-1.54373336646987E-15,-42.8201004838369,
-229.35005));
#232800=CARTESIAN_POINT('Origin',(-1.54373336646987E-15,-42.8201004838369,
-229.35005));
#232801=CARTESIAN_POINT('Origin',(-1.23757166668304E-15,-43.8201004838368,
-229.35005));
#232802=CARTESIAN_POINT('Origin',(-1.23757166668304E-15,-43.8201004838368,
-229.35005));
#232803=CARTESIAN_POINT('Origin',(-2.8425373731103E-15,9.20759727949731,
-229.35005));
#232804=CARTESIAN_POINT('Origin',(-2.8425373731103E-15,9.20759727949731,
-229.35005));
#232805=CARTESIAN_POINT('Origin',(-2.53637567332344E-15,10.2075972794973,
-229.35005));
#232806=CARTESIAN_POINT('Origin',(-2.53637567332344E-15,10.2075972794973,
-229.35005));
#232807=CARTESIAN_POINT('Origin',(-1.54373336646988E-15,19.8131368321642,
-229.35005));
#232808=CARTESIAN_POINT('Origin',(-1.54373336646988E-15,19.8131368321642,
-229.35005));
#232809=CARTESIAN_POINT('Origin',(-1.23757166668304E-15,20.8131368321642,
-229.35005));
#232810=CARTESIAN_POINT('Origin',(-1.23757166668304E-15,20.8131368321642,
-229.35005));
#232811=CARTESIAN_POINT('Origin',(-48.892180948596,36.2913696007177,-227.85005));
#232812=CARTESIAN_POINT('Origin',(-47.392180948596,37.1573950045021,-220.195349461621));
#232813=CARTESIAN_POINT('',(-47.392180948596,37.1573950045021,-221.195349461621));
#232814=CARTESIAN_POINT('',(-47.392180948596,37.1573950045021,-223.85005));
#232815=CARTESIAN_POINT('',(-47.392180948596,37.1573950045021,-220.195349461621));
#232816=CARTESIAN_POINT('',(-48.892180948596,38.0234204082866,-221.195349461621));
#232817=CARTESIAN_POINT('Ctrl Pts',(-48.8921809485959,38.0234204082865,
-221.195349461621));
#232818=CARTESIAN_POINT('Ctrl Pts',(-48.142180948596,37.5904077063944,-220.945349461621));
#232819=CARTESIAN_POINT('Ctrl Pts',(-47.3921809485961,37.1573950045022,
-221.195349461621));
#232820=CARTESIAN_POINT('',(-48.892180948596,38.0234204082866,-223.85005));
#232821=CARTESIAN_POINT('',(-48.892180948596,38.0234204082866,-220.195349461621));
#232822=CARTESIAN_POINT('Ctrl Pts',(-47.3921809485959,37.1573950045021,
-223.85005));
#232823=CARTESIAN_POINT('Ctrl Pts',(-48.142180948596,37.5904077063944,-223.417037298108));
#232824=CARTESIAN_POINT('Ctrl Pts',(-48.892180948596,38.0234204082866,-223.85005));
#232825=CARTESIAN_POINT('Origin',(-47.392180948596,35.4253441969333,-220.195349461621));
#232826=CARTESIAN_POINT('',(-47.392180948596,35.4253441969333,-221.195349461621));
#232827=CARTESIAN_POINT('',(-47.392180948596,35.4253441969333,-223.85005));
#232828=CARTESIAN_POINT('',(-47.392180948596,35.4253441969333,-220.195349461621));
#232829=CARTESIAN_POINT('Ctrl Pts',(-47.392180948596,37.1573950045021,-221.195349461621));
#232830=CARTESIAN_POINT('Ctrl Pts',(-47.392180948596,36.2913696007178,-220.945349461621));
#232831=CARTESIAN_POINT('Ctrl Pts',(-47.392180948596,35.4253441969335,-221.195349461621));
#232832=CARTESIAN_POINT('Ctrl Pts',(-47.392180948596,35.4253441969333,-223.85005));
#232833=CARTESIAN_POINT('Ctrl Pts',(-47.392180948596,36.2913696007177,-223.417037298108));
#232834=CARTESIAN_POINT('Ctrl Pts',(-47.392180948596,37.1573950045021,-223.85005));
#232835=CARTESIAN_POINT('Origin',(-48.892180948596,34.5593187931488,-220.195349461621));
#232836=CARTESIAN_POINT('',(-48.892180948596,34.5593187931488,-221.195349461621));
#232837=CARTESIAN_POINT('',(-48.892180948596,34.5593187931488,-223.85005));
#232838=CARTESIAN_POINT('',(-48.892180948596,34.5593187931488,-220.195349461621));
#232839=CARTESIAN_POINT('Ctrl Pts',(-47.3921809485961,35.4253441969333,
-221.195349461621));
#232840=CARTESIAN_POINT('Ctrl Pts',(-48.1421809485961,34.992331495041,-220.945349461621));
#232841=CARTESIAN_POINT('Ctrl Pts',(-48.8921809485962,34.5593187931488,
-221.195349461621));
#232842=CARTESIAN_POINT('Ctrl Pts',(-48.8921809485961,34.5593187931488,
-223.85005));
#232843=CARTESIAN_POINT('Ctrl Pts',(-48.142180948596,34.9923314950411,-223.417037298108));
#232844=CARTESIAN_POINT('Ctrl Pts',(-47.392180948596,35.4253441969333,-223.85005));
#232845=CARTESIAN_POINT('Origin',(-50.392180948596,35.4253441969333,-220.195349461621));
#232846=CARTESIAN_POINT('',(-50.392180948596,35.4253441969323,-221.19534946162));
#232847=CARTESIAN_POINT('',(-50.392180948596,35.4253441969333,-223.85005));
#232848=CARTESIAN_POINT('',(-50.392180948596,35.4253441969333,-220.195349461621));
#232849=CARTESIAN_POINT('Ctrl Pts',(-48.892180948596,34.5593187931489,-221.195349461621));
#232850=CARTESIAN_POINT('Ctrl Pts',(-49.6421809485958,34.992331495041,-220.945349461621));
#232851=CARTESIAN_POINT('Ctrl Pts',(-50.3921809485955,35.425344196933,-221.195349461621));
#232852=CARTESIAN_POINT('Ctrl Pts',(-50.3921809485959,35.4253441969333,
-223.85005));
#232853=CARTESIAN_POINT('Ctrl Pts',(-49.642180948596,34.9923314950411,-223.417037298108));
#232854=CARTESIAN_POINT('Ctrl Pts',(-48.892180948596,34.5593187931488,-223.85005));
#232855=CARTESIAN_POINT('Origin',(-50.392180948596,37.1573950045021,-220.195349461621));
#232856=CARTESIAN_POINT('',(-50.392180948596,37.1573950045021,-221.195349461621));
#232857=CARTESIAN_POINT('',(-50.392180948596,37.1573950045021,-223.85005));
#232858=CARTESIAN_POINT('',(-50.392180948596,37.1573950045021,-220.195349461621));
#232859=CARTESIAN_POINT('Ctrl Pts',(-50.392180948596,35.4253441969326,-221.195349461621));
#232860=CARTESIAN_POINT('Ctrl Pts',(-50.392180948596,36.2913696007175,-220.945349461621));
#232861=CARTESIAN_POINT('Ctrl Pts',(-50.392180948596,37.1573950045023,-221.195349461621));
#232862=CARTESIAN_POINT('Ctrl Pts',(-50.392180948596,37.1573950045022,-223.85005));
#232863=CARTESIAN_POINT('Ctrl Pts',(-50.392180948596,36.2913696007177,-223.417037298108));
#232864=CARTESIAN_POINT('Ctrl Pts',(-50.392180948596,35.4253441969332,-223.85005));
#232865=CARTESIAN_POINT('Origin',(-48.892180948596,38.0234204082866,-220.195349461621));
#232866=CARTESIAN_POINT('Ctrl Pts',(-50.3921809485959,37.1573950045022,
-221.195349461621));
#232867=CARTESIAN_POINT('Ctrl Pts',(-49.642180948596,37.5904077063944,-220.945349461621));
#232868=CARTESIAN_POINT('Ctrl Pts',(-48.8921809485962,38.0234204082865,
-221.195349461621));
#232869=CARTESIAN_POINT('Ctrl Pts',(-48.892180948596,38.0234204082866,-223.85005));
#232870=CARTESIAN_POINT('Ctrl Pts',(-49.642180948596,37.5904077063944,-223.417037298108));
#232871=CARTESIAN_POINT('Ctrl Pts',(-50.392180948596,37.1573950045022,-223.85005));
#232872=CARTESIAN_POINT('Origin',(-48.892180948596,36.2913696007177,-221.35005));
#232873=CARTESIAN_POINT('',(-48.892180948596,36.2913696007177,-220.195349461621));
#232874=CARTESIAN_POINT('',(-48.892180948596,34.2913696007177,-221.35005));
#232875=CARTESIAN_POINT('Origin',(-48.892180948596,36.2913696007177,-223.85005));
#232876=CARTESIAN_POINT('Origin',(-48.892180948596,36.2913696007177,-223.85005));
#232877=CARTESIAN_POINT('Origin',(-48.892180948596,36.2913696007177,-223.85005));
#232878=CARTESIAN_POINT('Origin',(-48.892180948596,36.2913696007177,-223.85005));
#232879=CARTESIAN_POINT('Origin',(-48.892180948596,36.2913696007177,-223.85005));
#232880=CARTESIAN_POINT('Origin',(-48.892180948596,36.2913696007177,-223.85005));
#232881=CARTESIAN_POINT('Origin',(-48.892180948596,36.2913696007177,-223.85005));
#232882=CARTESIAN_POINT('Origin',(-48.892180948596,36.2913696007177,-223.85005));
#232883=CARTESIAN_POINT('Origin',(-48.892180948596,36.2913696007177,-223.85005));
#232884=CARTESIAN_POINT('Origin',(-48.892180948596,36.2913696007177,-223.85005));
#232885=CARTESIAN_POINT('Origin',(-48.892180948596,36.2913696007177,-223.85005));
#232886=CARTESIAN_POINT('Origin',(-48.892180948596,36.2913696007177,-223.85005));
#232887=CARTESIAN_POINT('Origin',(-48.892180948596,36.2913696007177,-223.60005));
#232888=CARTESIAN_POINT('',(-48.892180948596,33.2913696007177,-223.85005));
#232889=CARTESIAN_POINT('Origin',(-48.892180948596,36.2913696007177,-223.85005));
#232890=CARTESIAN_POINT('',(-48.892180948596,33.0413696007177,-223.60005));
#232891=CARTESIAN_POINT('Origin',(-48.892180948596,33.2913696007177,-223.60005));
#232892=CARTESIAN_POINT('',(-48.892180948596,39.5413696007177,-223.60005));
#232893=CARTESIAN_POINT('Origin',(-48.892180948596,36.2913696007177,-223.60005));
#232894=CARTESIAN_POINT('Origin',(-48.892180948596,36.2913696007177,-223.60005));
#232895=CARTESIAN_POINT('Origin',(-48.892180948596,36.2913696007177,-218.35005));
#232896=CARTESIAN_POINT('',(-48.892180948596,39.5413696007177,-218.35005));
#232897=CARTESIAN_POINT('Origin',(-48.892180948596,36.2913696007177,-218.35005));
#232898=CARTESIAN_POINT('Origin',(-48.892180948596,36.2913696007177,-223.85005));
#232899=CARTESIAN_POINT('Origin',(-48.892180948596,36.2913696007177,-223.85005));
#232900=CARTESIAN_POINT('',(-48.892180948596,39.5413696007177,-223.85005));
#232901=CARTESIAN_POINT('Origin',(-12.9675000200281,-12.9675000200282,-32.54995));
#232902=CARTESIAN_POINT('',(-62.557372991106,-15.4675000200284,-32.54995));
#232903=CARTESIAN_POINT('',(-66.8875000100281,-17.9675000200284,-32.54995));
#232904=CARTESIAN_POINT('Origin',(-66.8875000100282,-12.9675000200284,-32.54995));
#232905=CARTESIAN_POINT('',(-71.2176270289503,-15.4675000200284,-32.54995));
#232906=CARTESIAN_POINT('Origin',(-66.8875000100282,-12.9675000200284,-32.54995));
#232907=CARTESIAN_POINT('',(-71.2176270289504,-10.4675000200284,-32.54995));
#232908=CARTESIAN_POINT('Origin',(-66.8875000100282,-12.9675000200284,-32.54995));
#232909=CARTESIAN_POINT('',(-66.8875000100282,-7.96750002002839,-32.54995));
#232910=CARTESIAN_POINT('Origin',(-66.8875000100282,-12.9675000200284,-32.54995));
#232911=CARTESIAN_POINT('',(-62.557372991106,-10.4675000200284,-32.54995));
#232912=CARTESIAN_POINT('Origin',(-66.8875000100282,-12.9675000200284,-32.54995));
#232913=CARTESIAN_POINT('Origin',(-66.8875000100282,-12.9675000200284,-32.54995));
#232914=CARTESIAN_POINT('Origin',(-66.8875000100282,-12.9675000200284,-32.54995));
#232915=CARTESIAN_POINT('',(-69.7742513559762,-17.9675000200284,-31.7764473081038));
#232916=CARTESIAN_POINT('Ctrl Pts',(-69.7742513559762,-17.9675000200284,
-31.7764473081038));
#232917=CARTESIAN_POINT('Ctrl Pts',(-70.5477540478725,-16.6277540578728,
-32.5499500000001));
#232918=CARTESIAN_POINT('Ctrl Pts',(-71.2176270289503,-15.4675000200284,
-32.5499500000001));
#232919=CARTESIAN_POINT('Ctrl Pts',(-66.8875000100281,-17.9675000200284,
-32.54995));
#232920=CARTESIAN_POINT('Ctrl Pts',(-68.2272459721837,-17.9675000200284,
-32.54995));
#232921=CARTESIAN_POINT('Ctrl Pts',(-69.7742513559762,-17.9675000200284,
-31.7764473081038));
#232922=CARTESIAN_POINT('Origin',(-66.8875000100282,-12.9675000200284,-32.54995));
#232923=CARTESIAN_POINT('',(-72.6610027019244,-12.9675000200284,-31.7764473081038));
#232924=CARTESIAN_POINT('Ctrl Pts',(-71.2176270289503,-15.4675000200284,
-32.5499500000001));
#232925=CARTESIAN_POINT('Ctrl Pts',(-71.8875000100281,-14.307245982184,
-32.5499500000001));
#232926=CARTESIAN_POINT('Ctrl Pts',(-72.6610027019243,-12.9675000200284,
-31.7764473081039));
#232927=CARTESIAN_POINT('Ctrl Pts',(-72.6610027019244,-12.9675000200284,
-31.7764473081038));
#232928=CARTESIAN_POINT('Ctrl Pts',(-71.8875000100282,-11.6277540578728,
-32.5499500000001));
#232929=CARTESIAN_POINT('Ctrl Pts',(-71.2176270289504,-10.4675000200284,
-32.5499500000001));
#232930=CARTESIAN_POINT('Origin',(-66.8875000100282,-12.9675000200284,-32.54995));
#232931=CARTESIAN_POINT('',(-69.7742513559763,-7.96750002002841,-31.7764473081038));
#232932=CARTESIAN_POINT('Ctrl Pts',(-71.2176270289504,-10.4675000200284,
-32.5499500000001));
#232933=CARTESIAN_POINT('Ctrl Pts',(-70.5477540478726,-9.30724598218405,
-32.5499500000001));
#232934=CARTESIAN_POINT('Ctrl Pts',(-69.7742513559763,-7.96750002002843,
-31.7764473081038));
#232935=CARTESIAN_POINT('Ctrl Pts',(-69.7742513559763,-7.96750002002841,
-31.7764473081038));
#232936=CARTESIAN_POINT('Ctrl Pts',(-68.2272459721838,-7.96750002002841,
-32.54995));
#232937=CARTESIAN_POINT('Ctrl Pts',(-66.8875000100282,-7.9675000200284,
-32.54995));
#232938=CARTESIAN_POINT('Origin',(-66.8875000100282,-12.9675000200284,-32.54995));
#232939=CARTESIAN_POINT('',(-64.0007486640801,-7.96750002002838,-31.7764473081038));
#232940=CARTESIAN_POINT('Ctrl Pts',(-66.8875000100282,-7.9675000200284,
-32.54995));
#232941=CARTESIAN_POINT('Ctrl Pts',(-65.5477540478726,-7.9675000200284,
-32.54995));
#232942=CARTESIAN_POINT('Ctrl Pts',(-64.0007486640801,-7.96750002002839,
-31.7764473081038));
#232943=CARTESIAN_POINT('Ctrl Pts',(-64.0007486640801,-7.96750002002838,
-31.7764473081038));
#232944=CARTESIAN_POINT('Ctrl Pts',(-63.2272459721838,-9.30724598218399,
-32.54995));
#232945=CARTESIAN_POINT('Ctrl Pts',(-62.557372991106,-10.4675000200284,
-32.54995));
#232946=CARTESIAN_POINT('Origin',(-66.8875000100282,-12.9675000200284,-32.54995));
#232947=CARTESIAN_POINT('',(-61.1139973181319,-12.9675000200284,-31.7764473081038));
#232948=CARTESIAN_POINT('Ctrl Pts',(-62.557372991106,-10.4675000200284,
-32.54995));
#232949=CARTESIAN_POINT('Ctrl Pts',(-61.8875000100282,-11.6277540578727,
-32.54995));
#232950=CARTESIAN_POINT('Ctrl Pts',(-61.113997318132,-12.9675000200284,
-31.7764473081038));
#232951=CARTESIAN_POINT('Ctrl Pts',(-61.1139973181319,-12.9675000200284,
-31.7764473081037));
#232952=CARTESIAN_POINT('Ctrl Pts',(-61.8875000100282,-14.307245982184,
-32.54995));
#232953=CARTESIAN_POINT('Ctrl Pts',(-62.557372991106,-15.4675000200284,
-32.54995));
#232954=CARTESIAN_POINT('Origin',(-66.8875000100282,-12.9675000200284,-32.54995));
#232955=CARTESIAN_POINT('',(-64.00074866408,-17.9675000200283,-31.7764473081038));
#232956=CARTESIAN_POINT('Ctrl Pts',(-62.557372991106,-15.4675000200284,
-32.54995));
#232957=CARTESIAN_POINT('Ctrl Pts',(-63.2272459721838,-16.6277540578727,
-32.54995));
#232958=CARTESIAN_POINT('Ctrl Pts',(-64.00074866408,-17.9675000200283,-31.7764473081038));
#232959=CARTESIAN_POINT('Ctrl Pts',(-64.00074866408,-17.9675000200283,-31.7764473081038));
#232960=CARTESIAN_POINT('Ctrl Pts',(-65.5477540478725,-17.9675000200283,
-32.54995));
#232961=CARTESIAN_POINT('Ctrl Pts',(-66.8875000100281,-17.9675000200284,
-32.54995));
#232962=CARTESIAN_POINT('Origin',(-12.9675000200281,-12.9675000200282,-28.54995));
#232963=CARTESIAN_POINT('',(-66.8875000100281,-17.9675000200283,-28.54995));
#232964=CARTESIAN_POINT('',(-71.2176270289503,-15.4675000200284,-28.54995));
#232965=CARTESIAN_POINT('Origin',(-66.8875000100282,-12.9675000200284,-28.54995));
#232966=CARTESIAN_POINT('',(-62.557372991106,-15.4675000200284,-28.54995));
#232967=CARTESIAN_POINT('Origin',(-66.8875000100282,-12.9675000200284,-28.54995));
#232968=CARTESIAN_POINT('',(-62.557372991106,-10.4675000200284,-28.54995));
#232969=CARTESIAN_POINT('Origin',(-66.8875000100282,-12.9675000200284,-28.54995));
#232970=CARTESIAN_POINT('',(-66.8875000100282,-7.9675000200284,-28.54995));
#232971=CARTESIAN_POINT('Origin',(-66.8875000100282,-12.9675000200284,-28.54995));
#232972=CARTESIAN_POINT('',(-71.2176270289503,-10.4675000200284,-28.54995));
#232973=CARTESIAN_POINT('Origin',(-66.8875000100282,-12.9675000200284,-28.54995));
#232974=CARTESIAN_POINT('Origin',(-66.8875000100282,-12.9675000200284,-28.54995));
#232975=CARTESIAN_POINT('Origin',(-66.8875000100282,-12.9675000200284,-28.54995));
#232976=CARTESIAN_POINT('',(-64.0007486640798,-17.9675000200283,-28.9965319873851));
#232977=CARTESIAN_POINT('Ctrl Pts',(-64.0007486640717,-17.9675000200283,
-28.9965319873876));
#232978=CARTESIAN_POINT('Ctrl Pts',(-65.5477540478691,-17.9675000200284,
-28.54995));
#232979=CARTESIAN_POINT('Ctrl Pts',(-66.887500010028,-17.9675000200283,
-28.54995));
#232980=CARTESIAN_POINT('Ctrl Pts',(-62.557372991106,-15.4675000200284,
-28.54995));
#232981=CARTESIAN_POINT('Ctrl Pts',(-63.2272459721854,-16.6277540578755,
-28.54995));
#232982=CARTESIAN_POINT('Ctrl Pts',(-64.000748664084,-17.9675000200353,
-28.9965319873875));
#232983=CARTESIAN_POINT('Origin',(-66.8875000100282,-12.9675000200284,-28.54995));
#232984=CARTESIAN_POINT('',(-61.1139973181319,-12.9675000200284,-28.9965319873852));
#232985=CARTESIAN_POINT('Ctrl Pts',(-61.1139973181278,-12.9675000200213,
-28.9965319873876));
#232986=CARTESIAN_POINT('Ctrl Pts',(-61.8875000100265,-14.3072459821811,
-28.54995));
#232987=CARTESIAN_POINT('Ctrl Pts',(-62.557372991106,-15.4675000200284,
-28.54995));
#232988=CARTESIAN_POINT('Ctrl Pts',(-62.557372991106,-10.4675000200284,
-28.54995));
#232989=CARTESIAN_POINT('Ctrl Pts',(-61.8875000100266,-11.6277540578756,
-28.54995));
#232990=CARTESIAN_POINT('Ctrl Pts',(-61.1139973181279,-12.9675000200354,
-28.9965319873876));
#232991=CARTESIAN_POINT('Origin',(-66.8875000100282,-12.9675000200284,-28.54995));
#232992=CARTESIAN_POINT('',(-64.0007486640801,-7.96750002002838,-28.9965319873852));
#232993=CARTESIAN_POINT('Ctrl Pts',(-64.0007486640842,-7.96750002002133,
-28.9965319873875));
#232994=CARTESIAN_POINT('Ctrl Pts',(-63.2272459721855,-9.30724598218116,
-28.54995));
#232995=CARTESIAN_POINT('Ctrl Pts',(-62.557372991106,-10.4675000200284,
-28.54995));
#232996=CARTESIAN_POINT('Ctrl Pts',(-66.8875000100282,-7.9675000200284,
-28.54995));
#232997=CARTESIAN_POINT('Ctrl Pts',(-65.5477540478693,-7.96750002002839,
-28.54995));
#232998=CARTESIAN_POINT('Ctrl Pts',(-64.0007486640719,-7.96750002002839,
-28.9965319873876));
#232999=CARTESIAN_POINT('Origin',(-66.8875000100282,-12.9675000200284,-28.54995));
#233000=CARTESIAN_POINT('',(-69.7742513559763,-7.96750002002841,-28.9965319873852));
#233001=CARTESIAN_POINT('Ctrl Pts',(-69.7742513559845,-7.96750002002841,
-28.9965319873875));
#233002=CARTESIAN_POINT('Ctrl Pts',(-68.2272459721871,-7.9675000200284,
-28.54995));
#233003=CARTESIAN_POINT('Ctrl Pts',(-66.8875000100282,-7.9675000200284,
-28.54995));
#233004=CARTESIAN_POINT('Ctrl Pts',(-71.2176270289503,-10.4675000200284,
-28.54995));
#233005=CARTESIAN_POINT('Ctrl Pts',(-70.5477540478709,-9.30724598218117,
-28.54995));
#233006=CARTESIAN_POINT('Ctrl Pts',(-69.7742513559722,-7.96750002002137,
-28.9965319873875));
#233007=CARTESIAN_POINT('Origin',(-66.8875000100282,-12.9675000200284,-28.54995));
#233008=CARTESIAN_POINT('',(-72.6610027019244,-12.9675000200284,-28.9965319873853));
#233009=CARTESIAN_POINT('Ctrl Pts',(-72.6610027019285,-12.9675000200355,
-28.9965319873875));
#233010=CARTESIAN_POINT('Ctrl Pts',(-71.8875000100298,-11.6277540578756,
-28.54995));
#233011=CARTESIAN_POINT('Ctrl Pts',(-71.2176270289503,-10.4675000200284,
-28.54995));
#233012=CARTESIAN_POINT('Ctrl Pts',(-71.2176270289503,-15.4675000200284,
-28.5499499999999));
#233013=CARTESIAN_POINT('Ctrl Pts',(-71.8875000100297,-14.3072459821812,
-28.5499499999999));
#233014=CARTESIAN_POINT('Ctrl Pts',(-72.6610027019284,-12.9675000200213,
-28.9965319873875));
#233015=CARTESIAN_POINT('Origin',(-66.8875000100282,-12.9675000200284,-28.54995));
#233016=CARTESIAN_POINT('',(-69.7742513559762,-17.9675000200284,-28.9965319873853));
#233017=CARTESIAN_POINT('Ctrl Pts',(-66.887500010028,-17.9675000200283,
-28.54995));
#233018=CARTESIAN_POINT('Ctrl Pts',(-68.227245972187,-17.9675000200284,
-28.54995));
#233019=CARTESIAN_POINT('Ctrl Pts',(-69.7742513559844,-17.9675000200284,
-28.9965319873875));
#233020=CARTESIAN_POINT('Ctrl Pts',(-69.7742513559721,-17.9675000200355,
-28.9965319873875));
#233021=CARTESIAN_POINT('Ctrl Pts',(-70.5477540478708,-16.6277540578756,
-28.5499499999999));
#233022=CARTESIAN_POINT('Ctrl Pts',(-71.2176270289503,-15.4675000200284,
-28.5499499999999));
#233023=CARTESIAN_POINT('Origin',(-64.00074866408,-17.9675000200283,-32.54995));
#233024=CARTESIAN_POINT('',(-64.00074866408,-17.9675000200283,-32.54995));
#233025=CARTESIAN_POINT('',(-69.7742513559762,-17.9675000200284,-32.54995));
#233026=CARTESIAN_POINT('Origin',(-61.1139973181319,-12.9675000200284,-32.54995));
#233027=CARTESIAN_POINT('',(-61.1139973181319,-12.9675000200284,-32.54995));
#233028=CARTESIAN_POINT('Origin',(-64.0007486640801,-7.96750002002838,-32.54995));
#233029=CARTESIAN_POINT('',(-64.0007486640801,-7.96750002002838,-32.54995));
#233030=CARTESIAN_POINT('Origin',(-69.7742513559763,-7.96750002002841,-32.54995));
#233031=CARTESIAN_POINT('',(-69.7742513559763,-7.96750002002841,-32.54995));
#233032=CARTESIAN_POINT('Origin',(-72.6610027019244,-12.9675000200284,-32.54995));
#233033=CARTESIAN_POINT('',(-72.6610027019244,-12.9675000200284,-32.54995));
#233034=CARTESIAN_POINT('Origin',(-69.7742513559762,-17.9675000200284,-32.54995));
#233035=CARTESIAN_POINT('Origin',(0.,8.39884049934975E-16,-32.54995));
#233036=CARTESIAN_POINT('',(-2.5,49.5898729710778,-32.54995));
#233037=CARTESIAN_POINT('',(-5.,53.91999999,-32.54995));
#233038=CARTESIAN_POINT('Origin',(-1.73472347597681E-15,53.91999999,-32.54995));
#233039=CARTESIAN_POINT('',(-2.5,58.2501270089222,-32.54995));
#233040=CARTESIAN_POINT('Origin',(-1.73472347597681E-15,53.91999999,-32.54995));
#233041=CARTESIAN_POINT('',(2.5,58.2501270089222,-32.54995));
#233042=CARTESIAN_POINT('Origin',(-1.73472347597681E-15,53.91999999,-32.54995));
#233043=CARTESIAN_POINT('',(5.,53.91999999,-32.54995));
#233044=CARTESIAN_POINT('Origin',(-1.73472347597681E-15,53.91999999,-32.54995));
#233045=CARTESIAN_POINT('',(2.5,49.5898729710778,-32.54995));
#233046=CARTESIAN_POINT('Origin',(-1.73472347597681E-15,53.91999999,-32.54995));
#233047=CARTESIAN_POINT('Origin',(-1.73472347597681E-15,53.91999999,-32.54995));
#233048=CARTESIAN_POINT('Origin',(-1.73472347597681E-15,53.91999999,-32.54995));
#233049=CARTESIAN_POINT('',(-5.,56.8067513359481,-31.7764473081038));
#233050=CARTESIAN_POINT('Ctrl Pts',(-4.99999999999996,56.8067513359481,
-31.7764473081038));
#233051=CARTESIAN_POINT('Ctrl Pts',(-3.66025403784437,57.5802540278444,
-32.54995));
#233052=CARTESIAN_POINT('Ctrl Pts',(-2.49999999999999,58.2501270089222,
-32.54995));
#233053=CARTESIAN_POINT('Ctrl Pts',(-5.,53.91999999,-32.54995));
#233054=CARTESIAN_POINT('Ctrl Pts',(-5.,55.2597459521556,-32.54995));
#233055=CARTESIAN_POINT('Ctrl Pts',(-5.,56.8067513359481,-31.7764473081038));
#233056=CARTESIAN_POINT('Origin',(-1.73472347597681E-15,53.91999999,-32.54995));
#233057=CARTESIAN_POINT('',(-1.66200633571292E-14,59.6935026818963,-31.7764473081038));
#233058=CARTESIAN_POINT('Ctrl Pts',(-2.49999999999999,58.2501270089222,
-32.54995));
#233059=CARTESIAN_POINT('Ctrl Pts',(-1.33974596215561,58.91999999,-32.54995));
#233060=CARTESIAN_POINT('Ctrl Pts',(-9.88775234870751E-15,59.6935026818962,
-31.7764473081038));
#233061=CARTESIAN_POINT('Ctrl Pts',(1.40342291401011E-14,59.6935026818963,
-31.7764473081037));
#233062=CARTESIAN_POINT('Ctrl Pts',(1.33974596215562,58.91999999,-32.54995));
#233063=CARTESIAN_POINT('Ctrl Pts',(2.5,58.2501270089222,-32.54995));
#233064=CARTESIAN_POINT('Origin',(-1.73472347597681E-15,53.91999999,-32.54995));
#233065=CARTESIAN_POINT('',(5.,56.8067513359482,-31.7764473081038));
#233066=CARTESIAN_POINT('Ctrl Pts',(2.5,58.2501270089222,-32.54995));
#233067=CARTESIAN_POINT('Ctrl Pts',(3.66025403784437,57.5802540278444,-32.54995));
#233068=CARTESIAN_POINT('Ctrl Pts',(4.99999999999995,56.8067513359482,-31.7764473081038));
#233069=CARTESIAN_POINT('Ctrl Pts',(5.,56.8067513359482,-31.7764473081037));
#233070=CARTESIAN_POINT('Ctrl Pts',(5.,55.2597459521556,-32.54995));
#233071=CARTESIAN_POINT('Ctrl Pts',(5.,53.91999999,-32.54995));
#233072=CARTESIAN_POINT('Origin',(-1.73472347597681E-15,53.91999999,-32.54995));
#233073=CARTESIAN_POINT('',(5.,51.0332486440519,-31.7764473081038));
#233074=CARTESIAN_POINT('Ctrl Pts',(5.,53.91999999,-32.54995));
#233075=CARTESIAN_POINT('Ctrl Pts',(5.,52.5802540278444,-32.54995));
#233076=CARTESIAN_POINT('Ctrl Pts',(5.,51.0332486440519,-31.7764473081038));
#233077=CARTESIAN_POINT('Ctrl Pts',(4.99999999999998,51.0332486440519,-31.7764473081038));
#233078=CARTESIAN_POINT('Ctrl Pts',(3.66025403784436,50.2597459521556,-32.54995));
#233079=CARTESIAN_POINT('Ctrl Pts',(2.49999999999997,49.5898729710778,-32.54995));
#233080=CARTESIAN_POINT('Origin',(-1.73472347597681E-15,53.91999999,-32.54995));
#233081=CARTESIAN_POINT('',(-2.79122613421945E-15,48.1464972981038,-31.7764473081038));
#233082=CARTESIAN_POINT('Ctrl Pts',(2.49999999999997,49.5898729710778,-32.54995));
#233083=CARTESIAN_POINT('Ctrl Pts',(1.33974596215561,48.91999999,-32.54995));
#233084=CARTESIAN_POINT('Ctrl Pts',(3.60424521098048E-14,48.1464972981038,
-31.7764473081038));
#233085=CARTESIAN_POINT('Ctrl Pts',(-3.50855728502523E-15,48.1464972981038,
-31.7764473081038));
#233086=CARTESIAN_POINT('Ctrl Pts',(-1.3397459621556,48.9199999900001,-32.5499500000001));
#233087=CARTESIAN_POINT('Ctrl Pts',(-2.49999999999997,49.5898729710779,
-32.5499500000001));
#233088=CARTESIAN_POINT('Origin',(-1.73472347597681E-15,53.91999999,-32.54995));
#233089=CARTESIAN_POINT('',(-5.,51.0332486440519,-31.7764473081037));
#233090=CARTESIAN_POINT('Ctrl Pts',(-2.49999999999997,49.5898729710779,
-32.5499500000001));
#233091=CARTESIAN_POINT('Ctrl Pts',(-3.66025403784436,50.2597459521557,
-32.5499500000001));
#233092=CARTESIAN_POINT('Ctrl Pts',(-4.99999999999998,51.0332486440519,
-31.7764473081038));
#233093=CARTESIAN_POINT('Ctrl Pts',(-5.,51.0332486440519,-31.7764473081038));
#233094=CARTESIAN_POINT('Ctrl Pts',(-5.,52.5802540278444,-32.54995));
#233095=CARTESIAN_POINT('Ctrl Pts',(-5.,53.91999999,-32.54995));
#233096=CARTESIAN_POINT('Origin',(0.,2.17747716649809E-16,-28.54995));
#233097=CARTESIAN_POINT('',(-5.,53.91999999,-28.54995));
#233098=CARTESIAN_POINT('',(-2.5,58.2501270089222,-28.54995));
#233099=CARTESIAN_POINT('Origin',(-1.73472347597681E-15,53.91999999,-28.54995));
#233100=CARTESIAN_POINT('',(-2.5,49.5898729710778,-28.54995));
#233101=CARTESIAN_POINT('Origin',(-1.73472347597681E-15,53.91999999,-28.54995));
#233102=CARTESIAN_POINT('',(2.5,49.5898729710778,-28.54995));
#233103=CARTESIAN_POINT('Origin',(-1.73472347597681E-15,53.91999999,-28.54995));
#233104=CARTESIAN_POINT('',(5.,53.91999999,-28.54995));
#233105=CARTESIAN_POINT('Origin',(-1.73472347597681E-15,53.91999999,-28.54995));
#233106=CARTESIAN_POINT('',(2.5,58.2501270089222,-28.54995));
#233107=CARTESIAN_POINT('Origin',(-1.73472347597681E-15,53.91999999,-28.54995));
#233108=CARTESIAN_POINT('Origin',(-1.73472347597681E-15,53.91999999,-28.54995));
#233109=CARTESIAN_POINT('Origin',(-1.73472347597681E-15,53.91999999,-28.54995));
#233110=CARTESIAN_POINT('',(-5.,51.0332486440517,-28.9965319873851));
#233111=CARTESIAN_POINT('Ctrl Pts',(-5.,51.0332486440436,-28.9965319873876));
#233112=CARTESIAN_POINT('Ctrl Pts',(-5.,52.5802540278411,-28.54995));
#233113=CARTESIAN_POINT('Ctrl Pts',(-5.,53.91999999,-28.54995));
#233114=CARTESIAN_POINT('Ctrl Pts',(-2.49999999999998,49.5898729710779,
-28.54995));
#233115=CARTESIAN_POINT('Ctrl Pts',(-3.66025403784716,50.2597459521573,
-28.54995));
#233116=CARTESIAN_POINT('Ctrl Pts',(-5.00000000000693,51.0332486440559,
-28.9965319873875));
#233117=CARTESIAN_POINT('Origin',(-1.73472347597681E-15,53.91999999,-28.54995));
#233118=CARTESIAN_POINT('',(-3.91685175604228E-15,48.1464972981038,-28.9965319873852));
#233119=CARTESIAN_POINT('Ctrl Pts',(7.06240095952727E-12,48.1464972980997,
-28.9965319873875));
#233120=CARTESIAN_POINT('Ctrl Pts',(-1.33974596215276,48.9199999899984,
-28.54995));
#233121=CARTESIAN_POINT('Ctrl Pts',(-2.49999999999998,49.5898729710779,
-28.54995));
#233122=CARTESIAN_POINT('Ctrl Pts',(2.49999999999996,49.5898729710778,-28.54995));
#233123=CARTESIAN_POINT('Ctrl Pts',(1.33974596215275,48.9199999899984,-28.54995));
#233124=CARTESIAN_POINT('Ctrl Pts',(-7.05906782420426E-12,48.1464972980997,
-28.9965319873875));
#233125=CARTESIAN_POINT('Origin',(-1.73472347597681E-15,53.91999999,-28.54995));
#233126=CARTESIAN_POINT('',(5.,51.0332486440519,-28.9965319873852));
#233127=CARTESIAN_POINT('Ctrl Pts',(5.00000000000706,51.033248644056,-28.9965319873876));
#233128=CARTESIAN_POINT('Ctrl Pts',(3.6602540378472,50.2597459521573,-28.54995));
#233129=CARTESIAN_POINT('Ctrl Pts',(2.49999999999996,49.5898729710778,-28.54995));
#233130=CARTESIAN_POINT('Ctrl Pts',(5.,53.91999999,-28.54995));
#233131=CARTESIAN_POINT('Ctrl Pts',(5.,52.5802540278411,-28.54995));
#233132=CARTESIAN_POINT('Ctrl Pts',(5.,51.0332486440438,-28.9965319873875));
#233133=CARTESIAN_POINT('Origin',(-1.73472347597681E-15,53.91999999,-28.54995));
#233134=CARTESIAN_POINT('',(5.,56.8067513359482,-28.9965319873852));
#233135=CARTESIAN_POINT('Ctrl Pts',(5.,56.8067513359563,-28.9965319873876));
#233136=CARTESIAN_POINT('Ctrl Pts',(5.,55.2597459521589,-28.54995));
#233137=CARTESIAN_POINT('Ctrl Pts',(5.,53.91999999,-28.54995));
#233138=CARTESIAN_POINT('Ctrl Pts',(2.49999999999998,58.2501270089222,-28.54995));
#233139=CARTESIAN_POINT('Ctrl Pts',(3.66025403784719,57.5802540278428,-28.54995));
#233140=CARTESIAN_POINT('Ctrl Pts',(5.000000000007,56.8067513359441,-28.9965319873876));
#233141=CARTESIAN_POINT('Origin',(-1.73472347597681E-15,53.91999999,-28.54995));
#233142=CARTESIAN_POINT('',(-1.57929637069991E-14,59.6935026818963,-28.9965319873852));
#233143=CARTESIAN_POINT('Ctrl Pts',(-7.06778525504927E-12,59.6935026819004,
-28.9965319873876));
#233144=CARTESIAN_POINT('Ctrl Pts',(1.33974596215276,58.9199999900017,-28.54995));
#233145=CARTESIAN_POINT('Ctrl Pts',(2.49999999999998,58.2501270089222,-28.54995));
#233146=CARTESIAN_POINT('Ctrl Pts',(-2.5,58.2501270089222,-28.54995));
#233147=CARTESIAN_POINT('Ctrl Pts',(-1.33974596215277,58.9199999900016,
-28.54995));
#233148=CARTESIAN_POINT('Ctrl Pts',(7.07624629086929E-12,59.6935026819003,
-28.9965319873875));
#233149=CARTESIAN_POINT('Origin',(-1.73472347597681E-15,53.91999999,-28.54995));
#233150=CARTESIAN_POINT('',(-5.,56.8067513359481,-28.9965319873852));
#233151=CARTESIAN_POINT('Ctrl Pts',(-5.,53.91999999,-28.54995));
#233152=CARTESIAN_POINT('Ctrl Pts',(-5.,55.2597459521589,-28.54995));
#233153=CARTESIAN_POINT('Ctrl Pts',(-5.,56.8067513359563,-28.9965319873876));
#233154=CARTESIAN_POINT('Ctrl Pts',(-5.00000000000706,56.806751335944,-28.9965319873876));
#233155=CARTESIAN_POINT('Ctrl Pts',(-3.66025403784722,57.5802540278427,
-28.54995));
#233156=CARTESIAN_POINT('Ctrl Pts',(-2.5,58.2501270089222,-28.54995));
#233157=CARTESIAN_POINT('Origin',(-5.,51.0332486440519,-32.54995));
#233158=CARTESIAN_POINT('',(-5.,51.0332486440519,-32.54995));
#233159=CARTESIAN_POINT('',(-5.,56.8067513359481,-32.54995));
#233160=CARTESIAN_POINT('Origin',(-3.63207727782644E-15,48.1464972981038,
-32.54995));
#233161=CARTESIAN_POINT('',(-3.63207727782644E-15,48.1464972981038,-32.54995));
#233162=CARTESIAN_POINT('Origin',(5.,51.0332486440519,-32.54995));
#233163=CARTESIAN_POINT('',(5.,51.0332486440519,-32.54995));
#233164=CARTESIAN_POINT('Origin',(5.,56.8067513359482,-32.54995));
#233165=CARTESIAN_POINT('',(5.,56.8067513359482,-32.54995));
#233166=CARTESIAN_POINT('Origin',(-1.56125112837912E-14,59.6935026818963,
-32.54995));
#233167=CARTESIAN_POINT('',(-1.56125112837912E-14,59.6935026818963,-32.54995));
#233168=CARTESIAN_POINT('Origin',(-5.,56.8067513359481,-32.54995));
#233169=CARTESIAN_POINT('Origin',(47.392180948596,-60.9300389954978,-220.195349461621));
#233170=CARTESIAN_POINT('',(47.392180948596,-60.9300389954978,-221.195349461621));
#233171=CARTESIAN_POINT('',(47.392180948596,-60.9300389954978,-223.85005));
#233172=CARTESIAN_POINT('',(47.392180948596,-60.9300389954978,-220.195349461621));
#233173=CARTESIAN_POINT('',(48.892180948596,-60.0640135917134,-223.85005));
#233174=CARTESIAN_POINT('Ctrl Pts',(47.392180948596,-60.9300389954978,-223.85005));
#233175=CARTESIAN_POINT('Ctrl Pts',(48.142180948596,-60.4970262936056,-223.417037298108));
#233176=CARTESIAN_POINT('Ctrl Pts',(48.8921809485959,-60.0640135917134,
-223.85005));
#233177=CARTESIAN_POINT('',(48.892180948596,-60.0640135917134,-221.195349461621));
#233178=CARTESIAN_POINT('',(48.892180948596,-60.0640135917134,-220.195349461621));
#233179=CARTESIAN_POINT('Ctrl Pts',(48.892180948596,-60.0640135917134,-221.195349461621));
#233180=CARTESIAN_POINT('Ctrl Pts',(48.142180948596,-60.4970262936056,-220.945349461621));
#233181=CARTESIAN_POINT('Ctrl Pts',(47.392180948596,-60.9300389954978,-221.195349461621));
#233182=CARTESIAN_POINT('Origin',(47.392180948596,-62.6620898030667,-220.195349461621));
#233183=CARTESIAN_POINT('',(47.392180948596,-62.6620898030667,-221.195349461621));
#233184=CARTESIAN_POINT('',(47.392180948596,-62.6620898030667,-223.85005));
#233185=CARTESIAN_POINT('',(47.392180948596,-62.6620898030667,-220.195349461621));
#233186=CARTESIAN_POINT('Ctrl Pts',(47.392180948596,-62.6620898030667,-223.85005));
#233187=CARTESIAN_POINT('Ctrl Pts',(47.392180948596,-61.7960643992823,-223.417037298108));
#233188=CARTESIAN_POINT('Ctrl Pts',(47.392180948596,-60.9300389954978,-223.85005));
#233189=CARTESIAN_POINT('Ctrl Pts',(47.392180948596,-60.9300389954978,-221.195349461621));
#233190=CARTESIAN_POINT('Ctrl Pts',(47.392180948596,-61.7960643992822,-220.945349461621));
#233191=CARTESIAN_POINT('Ctrl Pts',(47.392180948596,-62.6620898030667,-221.195349461621));
#233192=CARTESIAN_POINT('Origin',(48.892180948596,-63.5281152068512,-220.195349461621));
#233193=CARTESIAN_POINT('',(48.892180948596,-63.5281152068512,-221.195349461621));
#233194=CARTESIAN_POINT('',(48.892180948596,-63.5281152068512,-223.85005));
#233195=CARTESIAN_POINT('',(48.892180948596,-63.5281152068512,-220.195349461621));
#233196=CARTESIAN_POINT('Ctrl Pts',(48.892180948596,-63.5281152068512,-223.85005));
#233197=CARTESIAN_POINT('Ctrl Pts',(48.142180948596,-63.095102504959,-223.417037298108));
#233198=CARTESIAN_POINT('Ctrl Pts',(47.3921809485961,-62.6620898030668,
-223.85005));
#233199=CARTESIAN_POINT('Ctrl Pts',(47.392180948596,-62.6620898030667,-221.195349461621));
#233200=CARTESIAN_POINT('Ctrl Pts',(48.142180948596,-63.095102504959,-220.945349461621));
#233201=CARTESIAN_POINT('Ctrl Pts',(48.892180948596,-63.5281152068512,-221.195349461621));
#233202=CARTESIAN_POINT('Origin',(50.392180948596,-62.6620898030667,-220.195349461621));
#233203=CARTESIAN_POINT('',(50.392180948596,-62.6620898030677,-221.19534946162));
#233204=CARTESIAN_POINT('',(50.392180948596,-62.6620898030667,-223.85005));
#233205=CARTESIAN_POINT('',(50.392180948596,-62.6620898030667,-220.195349461621));
#233206=CARTESIAN_POINT('Ctrl Pts',(50.392180948596,-62.6620898030667,-223.85005));
#233207=CARTESIAN_POINT('Ctrl Pts',(49.642180948596,-63.0951025049589,-223.417037298108));
#233208=CARTESIAN_POINT('Ctrl Pts',(48.8921809485959,-63.5281152068512,
-223.85005));
#233209=CARTESIAN_POINT('Ctrl Pts',(48.8921809485958,-63.5281152068512,
-221.195349461621));
#233210=CARTESIAN_POINT('Ctrl Pts',(49.6421809485957,-63.0951025049591,
-220.945349461621));
#233211=CARTESIAN_POINT('Ctrl Pts',(50.3921809485954,-62.662089803067,-221.195349461621));
#233212=CARTESIAN_POINT('Origin',(50.392180948596,-60.9300389954978,-220.195349461621));
#233213=CARTESIAN_POINT('',(50.392180948596,-60.9300389954978,-221.195349461621));
#233214=CARTESIAN_POINT('',(50.392180948596,-60.9300389954978,-223.85005));
#233215=CARTESIAN_POINT('',(50.392180948596,-60.9300389954978,-220.195349461621));
#233216=CARTESIAN_POINT('Ctrl Pts',(50.392180948596,-60.9300389954978,-223.85005));
#233217=CARTESIAN_POINT('Ctrl Pts',(50.392180948596,-61.7960643992822,-223.417037298108));
#233218=CARTESIAN_POINT('Ctrl Pts',(50.392180948596,-62.6620898030667,-223.85005));
#233219=CARTESIAN_POINT('Ctrl Pts',(50.392180948596,-62.6620898030672,-221.195349461621));
#233220=CARTESIAN_POINT('Ctrl Pts',(50.392180948596,-61.7960643992825,-220.945349461621));
#233221=CARTESIAN_POINT('Ctrl Pts',(50.392180948596,-60.9300389954979,-221.195349461621));
#233222=CARTESIAN_POINT('Origin',(48.892180948596,-60.0640135917134,-220.195349461621));
#233223=CARTESIAN_POINT('Ctrl Pts',(48.892180948596,-60.0640135917134,-223.85005));
#233224=CARTESIAN_POINT('Ctrl Pts',(49.642180948596,-60.4970262936056,-223.417037298108));
#233225=CARTESIAN_POINT('Ctrl Pts',(50.392180948596,-60.9300389954978,-223.85005));
#233226=CARTESIAN_POINT('Ctrl Pts',(50.3921809485959,-60.9300389954977,
-221.195349461621));
#233227=CARTESIAN_POINT('Ctrl Pts',(49.642180948596,-60.4970262936056,-220.945349461621));
#233228=CARTESIAN_POINT('Ctrl Pts',(48.8921809485961,-60.0640135917134,
-221.195349461621));
#233229=CARTESIAN_POINT('Origin',(48.892180948596,-61.7960643992823,-221.35005));
#233230=CARTESIAN_POINT('',(48.892180948596,-61.7960643992823,-220.195349461621));
#233231=CARTESIAN_POINT('',(48.892180948596,-63.7960643992823,-221.35005));
#233232=CARTESIAN_POINT('Origin',(48.892180948596,-61.7960643992823,-223.85005));
#233233=CARTESIAN_POINT('Origin',(48.892180948596,-61.7960643992823,-223.85005));
#233234=CARTESIAN_POINT('Origin',(48.892180948596,-61.7960643992823,-223.85005));
#233235=CARTESIAN_POINT('Origin',(48.892180948596,-61.7960643992823,-223.85005));
#233236=CARTESIAN_POINT('Origin',(48.892180948596,-61.7960643992823,-223.85005));
#233237=CARTESIAN_POINT('Origin',(48.892180948596,-61.7960643992823,-223.85005));
#233238=CARTESIAN_POINT('Origin',(48.892180948596,-61.7960643992823,-223.85005));
#233239=CARTESIAN_POINT('Origin',(48.892180948596,-61.7960643992823,-223.85005));
#233240=CARTESIAN_POINT('Origin',(48.892180948596,-61.7960643992823,-223.85005));
#233241=CARTESIAN_POINT('Origin',(48.892180948596,-61.7960643992823,-223.85005));
#233242=CARTESIAN_POINT('Origin',(48.892180948596,-61.7960643992823,-223.85005));
#233243=CARTESIAN_POINT('Origin',(48.892180948596,-61.7960643992823,-223.85005));
#233244=CARTESIAN_POINT('Origin',(48.892180948596,-61.7960643992823,-223.60005));
#233245=CARTESIAN_POINT('',(48.892180948596,-64.7960643992823,-223.85005));
#233246=CARTESIAN_POINT('Origin',(48.892180948596,-61.7960643992823,-223.85005));
#233247=CARTESIAN_POINT('',(48.892180948596,-65.0460643992823,-223.60005));
#233248=CARTESIAN_POINT('Origin',(48.892180948596,-64.7960643992823,-223.60005));
#233249=CARTESIAN_POINT('',(48.892180948596,-58.5460643992823,-223.60005));
#233250=CARTESIAN_POINT('Origin',(48.892180948596,-61.7960643992823,-223.60005));
#233251=CARTESIAN_POINT('Origin',(48.892180948596,-61.7960643992823,-223.60005));
#233252=CARTESIAN_POINT('Origin',(48.892180948596,-61.7960643992823,-218.35005));
#233253=CARTESIAN_POINT('',(48.892180948596,-58.5460643992823,-218.35005));
#233254=CARTESIAN_POINT('Origin',(48.892180948596,-61.7960643992823,-218.35005));
#233255=CARTESIAN_POINT('Origin',(48.892180948596,-61.7960643992823,-223.85005));
#233256=CARTESIAN_POINT('Origin',(48.892180948596,-61.7960643992823,-223.85005));
#233257=CARTESIAN_POINT('',(48.892180948596,-58.5460643992823,-223.85005));
#233258=CARTESIAN_POINT('Origin',(35.64,75.4199999800001,-156.84995));
#233259=CARTESIAN_POINT('',(54.068191350826,75.4199999800001,-165.506240402784));
#233260=CARTESIAN_POINT('Origin',(54.068191350826,75.4199999800001,-156.84995));
#233261=CARTESIAN_POINT('',(55.5347128540504,71.1699999800001,-157.666957010302));
#233262=CARTESIAN_POINT('',(55.5347128540504,79.6699999800001,-157.666957010302));
#233263=CARTESIAN_POINT('Origin',(35.6422492679874,75.4199999800001,-156.798433293361));
#233264=CARTESIAN_POINT('',(55.5347128540504,71.1699999800001,-156.032942989698));
#233265=CARTESIAN_POINT('Ctrl Pts',(55.5347128540504,71.1699999800001,-157.666957010302));
#233266=CARTESIAN_POINT('Ctrl Pts',(55.5128901885938,71.0676625433561,-157.666004212151));
#233267=CARTESIAN_POINT('Ctrl Pts',(55.4895752701877,70.9585129098176,-157.644597099288));
#233268=CARTESIAN_POINT('Ctrl Pts',(55.4465989628004,70.7576504297677,-157.559247888691));
#233269=CARTESIAN_POINT('Ctrl Pts',(55.4269405591479,70.6659422090179,-157.495293401921));
#233270=CARTESIAN_POINT('Ctrl Pts',(55.3963403195744,70.5233317827474,-157.349523662669));
#233271=CARTESIAN_POINT('Ctrl Pts',(55.3831763635442,70.4620669759979,-157.258753516933));
#233272=CARTESIAN_POINT('Ctrl Pts',(55.3656791431848,70.3806748728845,-157.059753990808));
#233273=CARTESIAN_POINT('Ctrl Pts',(55.361351080024,70.3605621082167,-156.951518209892));
#233274=CARTESIAN_POINT('Ctrl Pts',(55.361351080024,70.3605621082167,-156.748381790108));
#233275=CARTESIAN_POINT('Ctrl Pts',(55.3656791431848,70.3806748728845,-156.640146009192));
#233276=CARTESIAN_POINT('Ctrl Pts',(55.3831763635442,70.4620669759979,-156.441146483066));
#233277=CARTESIAN_POINT('Ctrl Pts',(55.3963403195744,70.5233317827474,-156.350376337331));
#233278=CARTESIAN_POINT('Ctrl Pts',(55.4269405591479,70.6659422090179,-156.204606598079));
#233279=CARTESIAN_POINT('Ctrl Pts',(55.4465989628004,70.7576504297677,-156.140652111309));
#233280=CARTESIAN_POINT('Ctrl Pts',(55.4895752701877,70.9585129098176,-156.055302900712));
#233281=CARTESIAN_POINT('Ctrl Pts',(55.5128901885938,71.0676625433561,-156.033895787849));
#233282=CARTESIAN_POINT('Ctrl Pts',(55.5347128540504,71.1699999800001,-156.032942989698));
#233283=CARTESIAN_POINT('',(55.5347128540504,79.6699999800001,-156.032942989698));
#233284=CARTESIAN_POINT('Origin',(35.6422492679874,75.4199999800001,-156.901466706639));
#233285=CARTESIAN_POINT('Ctrl Pts',(55.5347128540504,79.6699999800001,-156.032942989698));
#233286=CARTESIAN_POINT('Ctrl Pts',(55.5128901885938,79.7723374166442,-156.033895787849));
#233287=CARTESIAN_POINT('Ctrl Pts',(55.4895752701877,79.8814870501826,-156.055302900712));
#233288=CARTESIAN_POINT('Ctrl Pts',(55.4465989628004,80.0823495302325,-156.140652111309));
#233289=CARTESIAN_POINT('Ctrl Pts',(55.4269405591479,80.1740577509823,-156.204606598079));
#233290=CARTESIAN_POINT('Ctrl Pts',(55.3963403195744,80.3166681772527,-156.350376337331));
#233291=CARTESIAN_POINT('Ctrl Pts',(55.3831763635442,80.3779329840023,-156.441146483066));
#233292=CARTESIAN_POINT('Ctrl Pts',(55.3656791431848,80.4593250871157,-156.640146009192));
#233293=CARTESIAN_POINT('Ctrl Pts',(55.361351080024,80.4794378517835,-156.748381790108));
#233294=CARTESIAN_POINT('Ctrl Pts',(55.361351080024,80.4794378517835,-156.951518209892));
#233295=CARTESIAN_POINT('Ctrl Pts',(55.3656791431848,80.4593250871157,-157.059753990808));
#233296=CARTESIAN_POINT('Ctrl Pts',(55.3831763635442,80.3779329840023,-157.258753516933));
#233297=CARTESIAN_POINT('Ctrl Pts',(55.3963403195744,80.3166681772527,-157.349523662669));
#233298=CARTESIAN_POINT('Ctrl Pts',(55.4269405591479,80.1740577509823,-157.495293401921));
#233299=CARTESIAN_POINT('Ctrl Pts',(55.4465989628004,80.0823495302325,-157.559247888691));
#233300=CARTESIAN_POINT('Ctrl Pts',(55.4895752701877,79.8814870501826,-157.644597099288));
#233301=CARTESIAN_POINT('Ctrl Pts',(55.5128901885938,79.7723374166442,-157.666004212151));
#233302=CARTESIAN_POINT('Ctrl Pts',(55.5347128540504,79.6699999800001,-157.666957010302));
#233303=CARTESIAN_POINT('Origin',(53.8419119874809,75.4199999800001,-156.84995));
#233304=CARTESIAN_POINT('',(53.8419119874809,75.4199999800001,-148.04995));
#233305=CARTESIAN_POINT('',(53.8419119874809,75.4199999800001,-165.64995));
#233306=CARTESIAN_POINT('Origin',(53.8419119874809,75.4199999800001,-156.84995));
#233307=CARTESIAN_POINT('Origin',(53.8419119874809,75.4199999800001,-156.84995));
#233308=CARTESIAN_POINT('Origin',(53.8419119874809,75.4199999800001,-165.39995));
#233309=CARTESIAN_POINT('Origin',(52.25,75.4199999800001,-156.84995));
#233310=CARTESIAN_POINT('',(52.,75.4199999800001,-165.39995));
#233311=CARTESIAN_POINT('Origin',(52.,75.4199999800001,-156.84995));
#233312=CARTESIAN_POINT('',(52.25,75.4199999800001,-165.64995));
#233313=CARTESIAN_POINT('Origin',(52.25,75.4199999800001,-165.39995));
#233314=CARTESIAN_POINT('',(52.25,75.4199999800001,-148.04995));
#233315=CARTESIAN_POINT('Origin',(52.25,75.4199999800001,-156.84995));
#233316=CARTESIAN_POINT('Origin',(52.25,75.4199999800001,-156.84995));
#233317=CARTESIAN_POINT('Origin',(54.,79.6699999800001,-156.84995));
#233318=CARTESIAN_POINT('',(54.,79.6699999800001,-156.09995));
#233319=CARTESIAN_POINT('',(54.,79.6699999800001,-157.59995));
#233320=CARTESIAN_POINT('Origin',(54.,79.6699999800001,-156.84995));
#233321=CARTESIAN_POINT('',(54.,71.1699999800001,-156.09995));
#233322=CARTESIAN_POINT('',(54.,79.6699999800001,-156.09995));
#233323=CARTESIAN_POINT('',(54.,71.1699999800001,-157.59995));
#233324=CARTESIAN_POINT('Origin',(54.,71.1699999800001,-156.84995));
#233325=CARTESIAN_POINT('',(54.,79.6699999800001,-157.59995));
#233326=CARTESIAN_POINT('Origin',(54.,79.6699999800001,-157.59995));
#233327=CARTESIAN_POINT('',(54.,79.6699999800001,-157.59995));
#233328=CARTESIAN_POINT('',(54.,71.1699999800001,-157.59995));
#233329=CARTESIAN_POINT('Origin',(54.,71.1699999800001,-156.84995));
#233330=CARTESIAN_POINT('',(54.,71.1699999800001,-156.09995));
#233331=CARTESIAN_POINT('Origin',(54.,79.6699999800001,-156.09995));
#233332=CARTESIAN_POINT('',(54.,79.6699999800001,-156.09995));
#233333=CARTESIAN_POINT('Origin',(54.,79.6699999800001,-156.84995));
#233334=CARTESIAN_POINT('Origin',(49.,75.4199999800001,-156.84995));
#233335=CARTESIAN_POINT('',(49.,75.4199999800001,-149.04995));
#233336=CARTESIAN_POINT('Origin',(49.,75.4199999800001,-156.84995));
#233337=CARTESIAN_POINT('Origin',(49.,75.4199999800001,-156.84995));
#233338=CARTESIAN_POINT('',(52.,75.4199999800001,-149.04995));
#233339=CARTESIAN_POINT('Origin',(52.,75.4199999800001,-156.84995));
#233340=CARTESIAN_POINT('',(49.,75.4199999800001,-149.04995));
#233341=CARTESIAN_POINT('Origin',(27.1098413022335,75.4199999800001,-156.84995));
#233342=CARTESIAN_POINT('',(27.1098413022335,75.4199999800001,-148.04995));
#233343=CARTESIAN_POINT('Origin',(52.,92.9199999800001,-126.84995));
#233344=CARTESIAN_POINT('Origin',(-44.5079524583208,-57.4754524783487,-39.8944822890418));
#233345=CARTESIAN_POINT('',(-46.5079524583208,-57.4754524783487,-40.4194822890418));
#233346=CARTESIAN_POINT('Origin',(-44.5079524583208,-57.4754524783487,-40.4194822890418));
#233347=CARTESIAN_POINT('',(-45.9829524583208,-57.4754524783487,-39.8944822890418));
#233348=CARTESIAN_POINT('',(-45.9829524583208,-57.4754524783487,-39.8944822890418));
#233349=CARTESIAN_POINT('Origin',(-44.5079524583208,-57.4754524783487,-39.8944822890418));
#233350=CARTESIAN_POINT('Origin',(-44.5079524583208,-57.4754524783487,-39.8944822890418));
#233351=CARTESIAN_POINT('Origin',(-44.5079524583208,-57.4754524783487,-39.8944822890418));
#233352=CARTESIAN_POINT('',(-46.5079524583208,-57.4754524783487,-55.24995));
#233353=CARTESIAN_POINT('Origin',(-44.5079524583208,-57.4754524783487,-55.24995));
#233354=CARTESIAN_POINT('',(-46.5079524583208,-57.4754524783487,-39.8944822890418));
#233355=CARTESIAN_POINT('Origin',(0.,45.41999998,-55.24995));
#233356=CARTESIAN_POINT('',(-47.0079524583208,-57.4754524783487,-55.24995));
#233357=CARTESIAN_POINT('Origin',(-44.5079524583208,-57.4754524783487,-55.24995));
#233358=CARTESIAN_POINT('Origin',(-44.5079524583208,-57.4754524783487,-48.1788821881345));
#233359=CARTESIAN_POINT('',(-47.0079524583208,-57.4754524783487,-179.64995));
#233360=CARTESIAN_POINT('Origin',(-44.5079524583208,-57.4754524783487,-179.64995));
#233361=CARTESIAN_POINT('',(-47.0079524583208,-57.4754524783487,-48.1788821881345));
#233362=CARTESIAN_POINT('Origin',(-44.5079524583208,-57.4754524783487,-179.64995));
#233363=CARTESIAN_POINT('Origin',(48.,93.4199999800001,-86.84995));
#233364=CARTESIAN_POINT('',(48.,93.4199999800001,-79.84995));
#233365=CARTESIAN_POINT('',(48.,92.9199999800001,-80.34995));
#233366=CARTESIAN_POINT('Origin',(48.,93.4199999800001,-80.34995));
#233367=CARTESIAN_POINT('',(54.5,92.9199999800001,-86.84995));
#233368=CARTESIAN_POINT('Origin',(48.,92.9199999800001,-86.84995));
#233369=CARTESIAN_POINT('',(55.,93.4199999800001,-86.84995));
#233370=CARTESIAN_POINT('Origin',(54.5,93.4199999800001,-86.84995));
#233371=CARTESIAN_POINT('Origin',(48.,93.4199999800001,-86.84995));
#233372=CARTESIAN_POINT('Origin',(54.5,93.4199999800001,-86.84995));
#233373=CARTESIAN_POINT('',(54.5,92.9199999800001,-182.84995));
#233374=CARTESIAN_POINT('',(55.,93.4199999800001,-182.84995));
#233375=CARTESIAN_POINT('Origin',(54.5,93.4199999800001,-182.84995));
#233376=CARTESIAN_POINT('',(55.,93.4199999800001,-86.84995));
#233377=CARTESIAN_POINT('',(54.5,92.9199999800001,-182.84995));
#233378=CARTESIAN_POINT('Origin',(-51.,93.4199999800001,-80.34995));
#233379=CARTESIAN_POINT('',(-51.,93.4199999800001,-79.84995));
#233380=CARTESIAN_POINT('',(-51.,92.9199999800001,-80.34995));
#233381=CARTESIAN_POINT('Origin',(-51.,93.4199999800001,-80.34995));
#233382=CARTESIAN_POINT('',(-51.,92.9199999800001,-80.34995));
#233383=CARTESIAN_POINT('',(-51.,93.4199999800001,-79.84995));
#233384=CARTESIAN_POINT('Origin',(48.,93.4199999800001,-182.84995));
#233385=CARTESIAN_POINT('',(48.,92.9199999800001,-189.34995));
#233386=CARTESIAN_POINT('',(48.,93.4199999800001,-189.84995));
#233387=CARTESIAN_POINT('Origin',(48.,93.4199999800001,-189.34995));
#233388=CARTESIAN_POINT('Origin',(48.,93.4199999800001,-182.84995));
#233389=CARTESIAN_POINT('Origin',(48.,92.9199999800001,-182.84995));
#233390=CARTESIAN_POINT('Origin',(-51.,93.4199999800001,-86.84995));
#233391=CARTESIAN_POINT('',(-58.,93.4199999800001,-86.84995));
#233392=CARTESIAN_POINT('',(-57.5,92.9199999800001,-86.84995));
#233393=CARTESIAN_POINT('Origin',(-57.5,93.4199999800001,-86.84995));
#233394=CARTESIAN_POINT('Origin',(-51.,92.9199999800001,-86.84995));
#233395=CARTESIAN_POINT('Origin',(-51.,93.4199999800001,-86.84995));
#233396=CARTESIAN_POINT('Origin',(48.,93.4199999800001,-189.34995));
#233397=CARTESIAN_POINT('',(-51.,92.9199999800001,-189.34995));
#233398=CARTESIAN_POINT('',(-51.,93.4199999800001,-189.84995));
#233399=CARTESIAN_POINT('Origin',(-51.,93.4199999800001,-189.34995));
#233400=CARTESIAN_POINT('',(48.,93.4199999800001,-189.84995));
#233401=CARTESIAN_POINT('',(-51.,92.9199999800001,-189.34995));
#233402=CARTESIAN_POINT('Origin',(-57.5,93.4199999800001,-182.84995));
#233403=CARTESIAN_POINT('',(-58.,93.4199999800001,-182.84995));
#233404=CARTESIAN_POINT('',(-57.5,92.9199999800001,-182.84995));
#233405=CARTESIAN_POINT('Origin',(-57.5,93.4199999800001,-182.84995));
#233406=CARTESIAN_POINT('',(-57.5,92.9199999800001,-182.84995));
#233407=CARTESIAN_POINT('',(-58.,93.4199999800001,-86.84995));
#233408=CARTESIAN_POINT('Origin',(-51.,93.4199999800001,-182.84995));
#233409=CARTESIAN_POINT('Origin',(-51.,92.9199999800001,-182.84995));
#233410=CARTESIAN_POINT('Origin',(-51.,93.4199999800001,-182.84995));
#233411=CARTESIAN_POINT('Origin',(-58.,105.91999998,-86.84995));
#233412=CARTESIAN_POINT('',(-58.,94.4199999800001,-182.84995));
#233413=CARTESIAN_POINT('',(-58.,105.91999998,-182.84995));
#233414=CARTESIAN_POINT('',(-58.,94.4199999800001,-86.84995));
#233415=CARTESIAN_POINT('',(-58.,105.91999998,-86.84995));
#233416=CARTESIAN_POINT('',(-58.,94.4199999800001,-86.84995));
#233417=CARTESIAN_POINT('Origin',(-51.,105.91999998,-182.84995));
#233418=CARTESIAN_POINT('',(-51.,94.4199999800001,-189.84995));
#233419=CARTESIAN_POINT('',(-51.,105.91999998,-189.84995));
#233420=CARTESIAN_POINT('Origin',(-51.,94.4199999800001,-182.84995));
#233421=CARTESIAN_POINT('Origin',(-51.,105.91999998,-86.84995));
#233422=CARTESIAN_POINT('',(-51.,94.4199999800001,-79.84995));
#233423=CARTESIAN_POINT('',(-51.,105.91999998,-79.84995));
#233424=CARTESIAN_POINT('Origin',(-51.,94.4199999800001,-86.84995));
#233425=CARTESIAN_POINT('Origin',(-55.,92.9199999800001,-82.84995));
#233426=CARTESIAN_POINT('',(-55.,91.9199999800001,-86.84995));
#233427=CARTESIAN_POINT('',(-55.,59.91999998,-86.84995));
#233428=CARTESIAN_POINT('',(-55.,92.9199999800001,-86.84995));
#233429=CARTESIAN_POINT('',(-55.,91.9199999800001,-182.84995));
#233430=CARTESIAN_POINT('',(-55.,91.9199999800001,-86.84995));
#233431=CARTESIAN_POINT('',(-55.,59.91999998,-182.84995));
#233432=CARTESIAN_POINT('',(-55.,92.9199999800001,-182.84995));
#233433=CARTESIAN_POINT('',(-55.,59.91999998,-182.84995));
#233434=CARTESIAN_POINT('',(-55.,75.4199999800001,-120.64995));
#233435=CARTESIAN_POINT('Origin',(-55.,75.4199999800001,-112.84995));
#233436=CARTESIAN_POINT('',(-55.,75.4199999800001,-164.64995));
#233437=CARTESIAN_POINT('Origin',(-55.,75.4199999800001,-156.84995));
#233438=CARTESIAN_POINT('Origin',(-51.,91.9199999800001,-86.84995));
#233439=CARTESIAN_POINT('',(-56.,92.9199999800001,-86.84995));
#233440=CARTESIAN_POINT('Origin',(-56.,91.9199999800001,-86.84995));
#233441=CARTESIAN_POINT('',(-51.,91.9199999800001,-82.84995));
#233442=CARTESIAN_POINT('Origin',(-51.,91.9199999800001,-86.84995));
#233443=CARTESIAN_POINT('',(-51.,92.9199999800001,-81.84995));
#233444=CARTESIAN_POINT('Origin',(-51.,91.9199999800001,-81.84995));
#233445=CARTESIAN_POINT('Origin',(-51.,92.9199999800001,-86.84995));
#233446=CARTESIAN_POINT('Origin',(-56.,91.9199999800001,-182.84995));
#233447=CARTESIAN_POINT('',(-56.,92.9199999800001,-182.84995));
#233448=CARTESIAN_POINT('Origin',(-56.,91.9199999800001,-182.84995));
#233449=CARTESIAN_POINT('',(-56.,92.9199999800001,-182.84995));
#233450=CARTESIAN_POINT('Origin',(-51.,91.9199999800001,-182.84995));
#233451=CARTESIAN_POINT('',(-51.,91.9199999800001,-186.84995));
#233452=CARTESIAN_POINT('',(-51.,92.9199999800001,-187.84995));
#233453=CARTESIAN_POINT('Origin',(-51.,91.9199999800001,-187.84995));
#233454=CARTESIAN_POINT('Origin',(-51.,91.9199999800001,-182.84995));
#233455=CARTESIAN_POINT('Origin',(-51.,92.9199999800001,-182.84995));
#233456=CARTESIAN_POINT('Origin',(-51.,92.9199999800001,-182.84995));
#233457=CARTESIAN_POINT('',(-51.,59.91999998,-186.84995));
#233458=CARTESIAN_POINT('',(-51.,92.9199999800001,-186.84995));
#233459=CARTESIAN_POINT('Origin',(-51.,59.91999998,-182.84995));
#233460=CARTESIAN_POINT('Origin',(-51.,59.91999998,-182.84995));
#233461=CARTESIAN_POINT('',(-51.,58.91999998,-185.84995));
#233462=CARTESIAN_POINT('Origin',(-51.,59.91999998,-185.84995));
#233463=CARTESIAN_POINT('',(-54.,58.91999998,-182.84995));
#233464=CARTESIAN_POINT('Origin',(-51.,58.91999998,-182.84995));
#233465=CARTESIAN_POINT('Origin',(-54.,59.91999998,-182.84995));
#233466=CARTESIAN_POINT('Origin',(-51.,59.91999998,-86.84995));
#233467=CARTESIAN_POINT('',(-54.,58.91999998,-86.84995));
#233468=CARTESIAN_POINT('Origin',(-54.,59.91999998,-86.84995));
#233469=CARTESIAN_POINT('',(-51.,58.91999998,-83.84995));
#233470=CARTESIAN_POINT('Origin',(-51.,58.91999998,-86.84995));
#233471=CARTESIAN_POINT('',(-51.,59.91999998,-82.84995));
#233472=CARTESIAN_POINT('Origin',(-51.,59.91999998,-83.84995));
#233473=CARTESIAN_POINT('Origin',(-51.,59.91999998,-86.84995));
#233474=CARTESIAN_POINT('Origin',(-54.,59.91999998,-82.84995));
#233475=CARTESIAN_POINT('',(-54.,58.91999998,-86.84995));
#233476=CARTESIAN_POINT('Origin',(-51.,92.9199999800001,-86.84995));
#233477=CARTESIAN_POINT('',(-51.,92.9199999800001,-82.84995));
#233478=CARTESIAN_POINT('Origin',(48.,92.9199999800001,-86.84995));
#233479=CARTESIAN_POINT('',(48.,59.91999998,-82.84995));
#233480=CARTESIAN_POINT('',(48.,91.9199999800001,-82.84995));
#233481=CARTESIAN_POINT('',(48.,92.9199999800001,-82.84995));
#233482=CARTESIAN_POINT('',(52.,59.91999998,-86.84995));
#233483=CARTESIAN_POINT('Origin',(48.,59.91999998,-86.84995));
#233484=CARTESIAN_POINT('',(52.,91.9199999800001,-86.84995));
#233485=CARTESIAN_POINT('',(52.,92.9199999800001,-86.84995));
#233486=CARTESIAN_POINT('Origin',(48.,91.9199999800001,-86.84995));
#233487=CARTESIAN_POINT('Origin',(51.,59.91999998,-82.84995));
#233488=CARTESIAN_POINT('',(51.,58.91999998,-182.84995));
#233489=CARTESIAN_POINT('',(52.,59.91999998,-182.84995));
#233490=CARTESIAN_POINT('Origin',(51.,59.91999998,-182.84995));
#233491=CARTESIAN_POINT('',(52.,59.91999998,-182.84995));
#233492=CARTESIAN_POINT('',(51.,58.91999998,-86.84995));
#233493=CARTESIAN_POINT('Origin',(51.,59.91999998,-86.84995));
#233494=CARTESIAN_POINT('',(51.,58.91999998,-86.84995));
#233495=CARTESIAN_POINT('Origin',(48.,59.91999998,-86.84995));
#233496=CARTESIAN_POINT('',(48.,58.91999998,-83.84995));
#233497=CARTESIAN_POINT('Origin',(48.,59.91999998,-83.84995));
#233498=CARTESIAN_POINT('Origin',(48.,58.91999998,-86.84995));
#233499=CARTESIAN_POINT('Origin',(48.,59.91999998,-182.84995));
#233500=CARTESIAN_POINT('',(48.,58.91999998,-185.84995));
#233501=CARTESIAN_POINT('',(48.,59.91999998,-186.84995));
#233502=CARTESIAN_POINT('Origin',(48.,59.91999998,-185.84995));
#233503=CARTESIAN_POINT('Origin',(48.,59.91999998,-182.84995));
#233504=CARTESIAN_POINT('Origin',(48.,58.91999998,-182.84995));
#233505=CARTESIAN_POINT('Origin',(48.,92.9199999800001,-182.84995));
#233506=CARTESIAN_POINT('',(52.,91.9199999800001,-182.84995));
#233507=CARTESIAN_POINT('',(52.,92.9199999800001,-182.84995));
#233508=CARTESIAN_POINT('',(48.,91.9199999800001,-186.84995));
#233509=CARTESIAN_POINT('',(48.,92.9199999800001,-186.84995));
#233510=CARTESIAN_POINT('Origin',(48.,91.9199999800001,-182.84995));
#233511=CARTESIAN_POINT('Origin',(48.,91.9199999800001,-182.84995));
#233512=CARTESIAN_POINT('',(48.,92.9199999800001,-187.84995));
#233513=CARTESIAN_POINT('Origin',(48.,91.9199999800001,-187.84995));
#233514=CARTESIAN_POINT('',(53.,92.9199999800001,-182.84995));
#233515=CARTESIAN_POINT('Origin',(48.,92.9199999800001,-182.84995));
#233516=CARTESIAN_POINT('Origin',(53.,91.9199999800001,-182.84995));
#233517=CARTESIAN_POINT('Origin',(53.,91.9199999800001,-182.84995));
#233518=CARTESIAN_POINT('',(53.,92.9199999800001,-86.84995));
#233519=CARTESIAN_POINT('',(53.,92.9199999800001,-182.84995));
#233520=CARTESIAN_POINT('Origin',(53.,91.9199999800001,-86.84995));
#233521=CARTESIAN_POINT('',(52.,91.9199999800001,-86.84995));
#233522=CARTESIAN_POINT('Origin',(48.,91.9199999800001,-86.84995));
#233523=CARTESIAN_POINT('',(48.,92.9199999800001,-81.84995));
#233524=CARTESIAN_POINT('Origin',(48.,92.9199999800001,-86.84995));
#233525=CARTESIAN_POINT('Origin',(48.,91.9199999800001,-81.84995));
#233526=CARTESIAN_POINT('Origin',(52.,92.9199999800001,-82.84995));
#233527=CARTESIAN_POINT('',(52.,75.4199999800001,-120.64995));
#233528=CARTESIAN_POINT('Origin',(52.,75.4199999800001,-112.84995));
#233529=CARTESIAN_POINT('',(52.,75.4199999800001,-164.64995));
#233530=CARTESIAN_POINT('Origin',(52.,75.4199999800001,-156.84995));
#233531=CARTESIAN_POINT('Origin',(48.,105.91999998,-86.84995));
#233532=CARTESIAN_POINT('',(48.,94.4199999800001,-79.84995));
#233533=CARTESIAN_POINT('',(48.,105.91999998,-79.84995));
#233534=CARTESIAN_POINT('',(55.,94.4199999800001,-86.84995));
#233535=CARTESIAN_POINT('',(55.,105.91999998,-86.84995));
#233536=CARTESIAN_POINT('Origin',(48.,94.4199999800001,-86.84995));
#233537=CARTESIAN_POINT('Origin',(48.,105.91999998,-182.84995));
#233538=CARTESIAN_POINT('',(55.,94.4199999800001,-182.84995));
#233539=CARTESIAN_POINT('',(55.,105.91999998,-182.84995));
#233540=CARTESIAN_POINT('',(48.,94.4199999800001,-189.84995));
#233541=CARTESIAN_POINT('',(48.,105.91999998,-189.84995));
#233542=CARTESIAN_POINT('Origin',(48.,94.4199999800001,-182.84995));
#233543=CARTESIAN_POINT('Origin',(-51.,91.9199999800001,-81.84995));
#233544=CARTESIAN_POINT('',(48.,92.9199999800001,-81.84995));
#233545=CARTESIAN_POINT('',(-1.5,91.9199999800001,-82.84995));
#233546=CARTESIAN_POINT('Origin',(-55.,92.9199999800001,-82.84995));
#233547=CARTESIAN_POINT('',(48.,59.91999998,-82.84995));
#233548=CARTESIAN_POINT('Origin',(-55.,59.91999998,-83.84995));
#233549=CARTESIAN_POINT('',(-1.5,58.91999998,-83.84995));
#233550=CARTESIAN_POINT('Origin',(-1.5,58.91999998,0.));
#233551=CARTESIAN_POINT('',(48.,58.91999998,-185.84995));
#233552=CARTESIAN_POINT('Origin',(-55.,59.91999998,-185.84995));
#233553=CARTESIAN_POINT('',(-1.5,59.91999998,-186.84995));
#233554=CARTESIAN_POINT('Origin',(-55.,92.9199999800001,-186.84995));
#233555=CARTESIAN_POINT('',(48.,91.9199999800001,-186.84995));
#233556=CARTESIAN_POINT('Origin',(-51.,91.9199999800001,-187.84995));
#233557=CARTESIAN_POINT('',(-1.5,92.9199999800001,-187.84995));
#233558=CARTESIAN_POINT('Origin',(-51.,92.9199999800001,-182.84995));
#233559=CARTESIAN_POINT('Origin',(48.,105.91999998,-189.84995));
#233560=CARTESIAN_POINT('',(48.,94.4199999800001,-189.84995));
#233561=CARTESIAN_POINT('Origin',(-51.,105.91999998,-79.84995));
#233562=CARTESIAN_POINT('',(-51.,94.4199999800001,-79.84995));
#233563=CARTESIAN_POINT('Origin',(151.5,75.4199999800001,-112.84995));
#233564=CARTESIAN_POINT('',(151.5,75.4199999800001,-120.64995));
#233565=CARTESIAN_POINT('Origin',(151.5,75.4199999800001,-156.84995));
#233566=CARTESIAN_POINT('',(151.5,75.4199999800001,-164.64995));
#233567=CARTESIAN_POINT('Origin',(55.,105.91999998,-86.84995));
#233568=CARTESIAN_POINT('',(55.,94.4199999800001,-86.84995));
#233569=CARTESIAN_POINT('Origin',(55.01,94.4199999800001,-52.64995));
#233570=CARTESIAN_POINT('Origin',(35.64,75.4199999800001,-112.84995));
#233571=CARTESIAN_POINT('',(54.068191350826,75.4199999800001,-121.506240402785));
#233572=CARTESIAN_POINT('Origin',(54.068191350826,75.4199999800001,-112.84995));
#233573=CARTESIAN_POINT('',(55.5347128540504,71.1699999800001,-113.666957010302));
#233574=CARTESIAN_POINT('',(55.5347128540504,79.6699999800001,-113.666957010302));
#233575=CARTESIAN_POINT('Origin',(35.6422492679874,75.4199999800001,-112.798433293361));
#233576=CARTESIAN_POINT('',(55.5347128540504,71.1699999800001,-112.032942989698));
#233577=CARTESIAN_POINT('Ctrl Pts',(55.5347128540504,71.1699999800001,-113.666957010302));
#233578=CARTESIAN_POINT('Ctrl Pts',(55.5128901885938,71.0676625433561,-113.666004212151));
#233579=CARTESIAN_POINT('Ctrl Pts',(55.4895752701877,70.9585129098177,-113.644597099288));
#233580=CARTESIAN_POINT('Ctrl Pts',(55.4465989628004,70.7576504297677,-113.559247888691));
#233581=CARTESIAN_POINT('Ctrl Pts',(55.4269405591479,70.6659422090179,-113.495293401921));
#233582=CARTESIAN_POINT('Ctrl Pts',(55.3963403195744,70.5233317827474,-113.349523662669));
#233583=CARTESIAN_POINT('Ctrl Pts',(55.3831763635442,70.4620669759979,-113.258753516934));
#233584=CARTESIAN_POINT('Ctrl Pts',(55.3656791431848,70.3806748728845,-113.059753990808));
#233585=CARTESIAN_POINT('Ctrl Pts',(55.361351080024,70.3605621082167,-112.951518209892));
#233586=CARTESIAN_POINT('Ctrl Pts',(55.361351080024,70.3605621082167,-112.748381790108));
#233587=CARTESIAN_POINT('Ctrl Pts',(55.3656791431848,70.3806748728845,-112.640146009192));
#233588=CARTESIAN_POINT('Ctrl Pts',(55.3831763635442,70.4620669759979,-112.441146483067));
#233589=CARTESIAN_POINT('Ctrl Pts',(55.3963403195744,70.5233317827474,-112.350376337331));
#233590=CARTESIAN_POINT('Ctrl Pts',(55.4269405591479,70.6659422090179,-112.204606598079));
#233591=CARTESIAN_POINT('Ctrl Pts',(55.4465989628004,70.7576504297677,-112.140652111309));
#233592=CARTESIAN_POINT('Ctrl Pts',(55.4895752701877,70.9585129098177,-112.055302900712));
#233593=CARTESIAN_POINT('Ctrl Pts',(55.5128901885938,71.0676625433561,-112.033895787849));
#233594=CARTESIAN_POINT('Ctrl Pts',(55.5347128540504,71.1699999800001,-112.032942989698));
#233595=CARTESIAN_POINT('',(55.5347128540504,79.6699999800001,-112.032942989698));
#233596=CARTESIAN_POINT('Origin',(35.6422492679874,75.4199999800001,-112.901466706639));
#233597=CARTESIAN_POINT('Ctrl Pts',(55.5347128540504,79.6699999800001,-112.032942989698));
#233598=CARTESIAN_POINT('Ctrl Pts',(55.5128901885938,79.7723374166442,-112.033895787849));
#233599=CARTESIAN_POINT('Ctrl Pts',(55.4895752701877,79.8814870501826,-112.055302900712));
#233600=CARTESIAN_POINT('Ctrl Pts',(55.4465989628004,80.0823495302325,-112.140652111309));
#233601=CARTESIAN_POINT('Ctrl Pts',(55.4269405591479,80.1740577509823,-112.204606598079));
#233602=CARTESIAN_POINT('Ctrl Pts',(55.3963403195744,80.3166681772527,-112.350376337331));
#233603=CARTESIAN_POINT('Ctrl Pts',(55.3831763635442,80.3779329840023,-112.441146483067));
#233604=CARTESIAN_POINT('Ctrl Pts',(55.3656791431848,80.4593250871157,-112.640146009192));
#233605=CARTESIAN_POINT('Ctrl Pts',(55.361351080024,80.4794378517835,-112.748381790108));
#233606=CARTESIAN_POINT('Ctrl Pts',(55.361351080024,80.4794378517835,-112.951518209892));
#233607=CARTESIAN_POINT('Ctrl Pts',(55.3656791431848,80.4593250871157,-113.059753990808));
#233608=CARTESIAN_POINT('Ctrl Pts',(55.3831763635442,80.3779329840023,-113.258753516933));
#233609=CARTESIAN_POINT('Ctrl Pts',(55.3963403195744,80.3166681772527,-113.349523662669));
#233610=CARTESIAN_POINT('Ctrl Pts',(55.4269405591479,80.1740577509823,-113.495293401921));
#233611=CARTESIAN_POINT('Ctrl Pts',(55.4465989628004,80.0823495302325,-113.559247888691));
#233612=CARTESIAN_POINT('Ctrl Pts',(55.4895752701877,79.8814870501826,-113.644597099288));
#233613=CARTESIAN_POINT('Ctrl Pts',(55.5128901885938,79.7723374166442,-113.666004212151));
#233614=CARTESIAN_POINT('Ctrl Pts',(55.5347128540504,79.6699999800001,-113.666957010302));
#233615=CARTESIAN_POINT('Origin',(53.8419119874809,75.4199999800001,-112.84995));
#233616=CARTESIAN_POINT('',(53.8419119874809,75.4199999800001,-104.04995));
#233617=CARTESIAN_POINT('',(53.8419119874809,75.4199999800001,-121.64995));
#233618=CARTESIAN_POINT('Origin',(53.8419119874809,75.4199999800001,-112.84995));
#233619=CARTESIAN_POINT('Origin',(53.8419119874809,75.4199999800001,-112.84995));
#233620=CARTESIAN_POINT('Origin',(53.8419119874809,75.4199999800001,-121.39995));
#233621=CARTESIAN_POINT('Origin',(52.25,75.4199999800001,-112.84995));
#233622=CARTESIAN_POINT('',(52.,75.4199999800001,-121.39995));
#233623=CARTESIAN_POINT('Origin',(52.,75.4199999800001,-112.84995));
#233624=CARTESIAN_POINT('',(52.25,75.4199999800001,-121.64995));
#233625=CARTESIAN_POINT('Origin',(52.25,75.4199999800001,-121.39995));
#233626=CARTESIAN_POINT('',(52.25,75.4199999800001,-104.04995));
#233627=CARTESIAN_POINT('Origin',(52.25,75.4199999800001,-112.84995));
#233628=CARTESIAN_POINT('Origin',(52.25,75.4199999800001,-112.84995));
#233629=CARTESIAN_POINT('Origin',(54.,79.6699999800001,-112.84995));
#233630=CARTESIAN_POINT('',(54.,79.6699999800001,-112.09995));
#233631=CARTESIAN_POINT('',(54.,79.6699999800001,-113.59995));
#233632=CARTESIAN_POINT('Origin',(54.,79.6699999800001,-112.84995));
#233633=CARTESIAN_POINT('',(54.,71.1699999800001,-112.09995));
#233634=CARTESIAN_POINT('',(54.,79.6699999800001,-112.09995));
#233635=CARTESIAN_POINT('',(54.,71.1699999800001,-113.59995));
#233636=CARTESIAN_POINT('Origin',(54.,71.1699999800001,-112.84995));
#233637=CARTESIAN_POINT('',(54.,79.6699999800001,-113.59995));
#233638=CARTESIAN_POINT('Origin',(54.,79.6699999800001,-113.59995));
#233639=CARTESIAN_POINT('',(54.,79.6699999800001,-113.59995));
#233640=CARTESIAN_POINT('',(54.,71.1699999800001,-113.59995));
#233641=CARTESIAN_POINT('Origin',(54.,71.1699999800001,-112.84995));
#233642=CARTESIAN_POINT('',(54.,71.1699999800001,-112.09995));
#233643=CARTESIAN_POINT('Origin',(54.,79.6699999800001,-112.09995));
#233644=CARTESIAN_POINT('',(54.,79.6699999800001,-112.09995));
#233645=CARTESIAN_POINT('Origin',(54.,79.6699999800001,-112.84995));
#233646=CARTESIAN_POINT('Origin',(49.,75.4199999800001,-112.84995));
#233647=CARTESIAN_POINT('',(49.,75.4199999800001,-105.04995));
#233648=CARTESIAN_POINT('Origin',(49.,75.4199999800001,-112.84995));
#233649=CARTESIAN_POINT('Origin',(49.,75.4199999800001,-112.84995));
#233650=CARTESIAN_POINT('',(52.,75.4199999800001,-105.04995));
#233651=CARTESIAN_POINT('Origin',(52.,75.4199999800001,-112.84995));
#233652=CARTESIAN_POINT('',(49.,75.4199999800001,-105.04995));
#233653=CARTESIAN_POINT('Origin',(27.1098413022335,75.4199999800001,-112.84995));
#233654=CARTESIAN_POINT('',(27.1098413022335,75.4199999800001,-104.04995));
#233655=CARTESIAN_POINT('Origin',(52.,92.9199999800001,-82.84995));
#233656=CARTESIAN_POINT('Origin',(48.6475142708864,46.7952694142692,-180.14995));
#233657=CARTESIAN_POINT('',(41.086116694801,39.9409786193705,-180.14995));
#233658=CARTESIAN_POINT('',(41.4396700853943,39.5874252287771,-179.64995));
#233659=CARTESIAN_POINT('Origin',(41.4396700853943,39.5874252287771,-180.14995));
#233660=CARTESIAN_POINT('',(48.6849040646875,46.8326592080703,-179.64995));
#233661=CARTESIAN_POINT('',(41.4396700853943,39.5874252287771,-179.64995));
#233662=CARTESIAN_POINT('',(48.2939608802931,47.1488228048625,-180.14995));
#233663=CARTESIAN_POINT('Ctrl Pts',(48.2939608802932,47.1488228048625,-180.14995));
#233664=CARTESIAN_POINT('Ctrl Pts',(48.2939608802932,47.1488228048625,-180.087184163359));
#233665=CARTESIAN_POINT('Ctrl Pts',(48.3037994668372,47.1409231885199,-180.020261450625));
#233666=CARTESIAN_POINT('Ctrl Pts',(48.3437200901627,47.1088207011521,-179.897213130352));
#233667=CARTESIAN_POINT('Ctrl Pts',(48.3737972006442,47.0846160842381,-179.84108638012));
#233668=CARTESIAN_POINT('Ctrl Pts',(48.443221456874,47.0286267129769,-179.752211869064));
#233669=CARTESIAN_POINT('Ctrl Pts',(48.4872746644709,46.9930450683611,-179.713637732877));
#233670=CARTESIAN_POINT('Ctrl Pts',(48.5836337459409,46.9149957840453,-179.662507580811));
#233671=CARTESIAN_POINT('Ctrl Pts',(48.6359363487773,46.8725251312072,-179.64995));
#233672=CARTESIAN_POINT('Ctrl Pts',(48.6849040646876,46.8326592080703,-179.64995));
#233673=CARTESIAN_POINT('',(48.2939608802931,47.1488228048625,-180.14995));
#233674=CARTESIAN_POINT('Origin',(40.7325633042078,40.2945320099637,-180.14995));
#233675=CARTESIAN_POINT('',(40.7325633042078,39.7945320099637,-180.14995));
#233676=CARTESIAN_POINT('',(40.7325633042078,39.2945320099637,-179.64995));
#233677=CARTESIAN_POINT('Origin',(40.7325633042078,39.2945320099637,-180.14995));
#233678=CARTESIAN_POINT('Origin',(40.7325633042078,40.2945320099637,-179.64995));
#233679=CARTESIAN_POINT('Origin',(40.7325633042078,40.2945320099637,-180.14995));
#233680=CARTESIAN_POINT('Origin',(39.9396700853943,39.2945320099637,-180.14995));
#233681=CARTESIAN_POINT('',(40.4396700853943,39.7945320099637,-180.14995));
#233682=CARTESIAN_POINT('',(40.4396700853943,39.2945320099637,-179.64995));
#233683=CARTESIAN_POINT('Origin',(40.4396700853943,39.2945320099637,-180.14995));
#233684=CARTESIAN_POINT('',(40.4396700853943,39.2945320099637,-179.64995));
#233685=CARTESIAN_POINT('',(40.7325633042078,39.7945320099637,-180.14995));
#233686=CARTESIAN_POINT('Origin',(40.4396700853943,40.2945320099637,-180.14995));
#233687=CARTESIAN_POINT('',(39.9396700853943,40.2945320099637,-180.14995));
#233688=CARTESIAN_POINT('',(39.4396700853942,40.2945320099637,-179.64995));
#233689=CARTESIAN_POINT('Origin',(39.4396700853942,40.2945320099637,-180.14995));
#233690=CARTESIAN_POINT('Origin',(40.4396700853943,40.2945320099637,-179.64995));
#233691=CARTESIAN_POINT('Origin',(40.4396700853943,40.2945320099637,-180.14995));
#233692=CARTESIAN_POINT('Origin',(39.4396700853942,49.9558747416749,-180.14995));
#233693=CARTESIAN_POINT('',(39.4396700853942,50.0426929113215,-179.64995));
#233694=CARTESIAN_POINT('',(39.9396700853943,49.9558747416749,-180.14995));
#233695=CARTESIAN_POINT('Ctrl Pts',(39.4396700853942,50.0426929113213,-179.64995));
#233696=CARTESIAN_POINT('Ctrl Pts',(39.5025092537829,50.0318525348131,-179.64995));
#233697=CARTESIAN_POINT('Ctrl Pts',(39.5695953475419,50.0202501005871,-179.662513814803));
#233698=CARTESIAN_POINT('Ctrl Pts',(39.6931562106457,49.9988279173233,-179.713808517639));
#233699=CARTESIAN_POINT('Ctrl Pts',(39.7496292333555,49.9890099683669,-179.752544364656));
#233700=CARTESIAN_POINT('Ctrl Pts',(39.8381537765163,49.973597171116,-179.841586696561));
#233701=CARTESIAN_POINT('Ctrl Pts',(39.8763752988257,49.9669287636703,-179.897554483501));
#233702=CARTESIAN_POINT('Ctrl Pts',(39.9271363480647,49.9580662763262,-180.020367660125));
#233703=CARTESIAN_POINT('Ctrl Pts',(39.9396700853942,49.9558747416746,-180.087215626338));
#233704=CARTESIAN_POINT('Ctrl Pts',(39.9396700853942,49.9558747416746,-180.14995));
#233705=CARTESIAN_POINT('',(39.4396700853942,49.9558747416749,-179.64995));
#233706=CARTESIAN_POINT('',(39.9396700853943,40.2945320099637,-180.14995));
#233707=CARTESIAN_POINT('Origin',(39.4396700853942,-64.8856746638358,-180.14995));
#233708=CARTESIAN_POINT('',(39.9396700853942,-65.3856746638358,-180.14995));
#233709=CARTESIAN_POINT('',(39.4396700853942,-65.3856746638358,-179.64995));
#233710=CARTESIAN_POINT('Origin',(39.4396700853942,-65.3856746638358,-180.14995));
#233711=CARTESIAN_POINT('',(39.4396700853942,-75.2524362554308,-179.64995));
#233712=CARTESIAN_POINT('',(39.4396700853942,-65.3856746638358,-179.64995));
#233713=CARTESIAN_POINT('',(39.9396700853942,-75.2524362554308,-180.14995));
#233714=CARTESIAN_POINT('Origin',(39.4396700853942,-75.2524362554308,-180.14995));
#233715=CARTESIAN_POINT('',(39.9396700853942,-75.2524362554308,-180.14995));
#233716=CARTESIAN_POINT('Origin',(40.4396700853942,-65.3856746638358,-180.14995));
#233717=CARTESIAN_POINT('',(40.4396700853942,-64.8856746638358,-180.14995));
#233718=CARTESIAN_POINT('',(40.4396700853943,-64.3856746638358,-179.64995));
#233719=CARTESIAN_POINT('Origin',(40.4396700853943,-64.3856746638358,-180.14995));
#233720=CARTESIAN_POINT('Origin',(40.4396700853942,-65.3856746638358,-179.64995));
#233721=CARTESIAN_POINT('Origin',(40.4396700853942,-65.3856746638358,-180.14995));
#233722=CARTESIAN_POINT('Origin',(39.9396700853942,-64.3856746638358,-180.14995));
#233723=CARTESIAN_POINT('',(40.7325633042077,-64.8856746638358,-180.14995));
#233724=CARTESIAN_POINT('',(40.7325633042078,-64.3856746638358,-179.64995));
#233725=CARTESIAN_POINT('Origin',(40.7325633042078,-64.3856746638358,-180.14995));
#233726=CARTESIAN_POINT('',(40.7325633042078,-64.3856746638358,-179.64995));
#233727=CARTESIAN_POINT('',(40.4396700853942,-64.8856746638358,-180.14995));
#233728=CARTESIAN_POINT('Origin',(40.7325633042077,-65.3856746638358,-180.14995));
#233729=CARTESIAN_POINT('',(41.086116694801,-65.0321212732425,-180.14995));
#233730=CARTESIAN_POINT('',(41.4396700853943,-64.6785678826493,-179.64995));
#233731=CARTESIAN_POINT('Origin',(41.4396700853943,-64.6785678826493,-180.14995));
#233732=CARTESIAN_POINT('Origin',(40.7325633042077,-65.3856746638358,-179.64995));
#233733=CARTESIAN_POINT('Origin',(40.7325633042077,-65.3856746638358,-180.14995));
#233734=CARTESIAN_POINT('Origin',(49.1137948708872,-72.3526926681422,-180.14995));
#233735=CARTESIAN_POINT('',(49.1484061576371,-72.3873039548922,-179.64995));
#233736=CARTESIAN_POINT('',(48.7602414802939,-72.7062460587355,-180.14995));
#233737=CARTESIAN_POINT('Ctrl Pts',(49.1484061576372,-72.3873039548922,
-179.64995));
#233738=CARTESIAN_POINT('Ctrl Pts',(49.0997901061269,-72.4275161617186,
-179.64995));
#233739=CARTESIAN_POINT('Ctrl Pts',(49.0478648385672,-72.470354734769,-179.662506414177));
#233740=CARTESIAN_POINT('Ctrl Pts',(48.9522061528442,-72.5490766792219,
-179.713622094328));
#233741=CARTESIAN_POINT('Ctrl Pts',(48.9084759486685,-72.5849631007156,
-179.752182677537));
#233742=CARTESIAN_POINT('Ctrl Pts',(48.8395335697769,-72.6414546742699,
-179.841043950726));
#233743=CARTESIAN_POINT('Ctrl Pts',(48.8096591731515,-72.6658815244501,
-179.89718443088));
#233744=CARTESIAN_POINT('Ctrl Pts',(48.7700107976248,-72.6982762551188,
-180.020252853856));
#233745=CARTESIAN_POINT('Ctrl Pts',(48.760241480294,-72.7062460587355,-180.087181792204));
#233746=CARTESIAN_POINT('Ctrl Pts',(48.760241480294,-72.7062460587355,-180.14995));
#233747=CARTESIAN_POINT('',(49.1137948708872,-72.3526926681422,-179.64995));
#233748=CARTESIAN_POINT('',(41.086116694801,-65.0321212732425,-180.14995));
#233749=CARTESIAN_POINT('Origin',(61.6666822880186,-45.93000002,-189.64995));
#233750=CARTESIAN_POINT('',(62.1666822880186,-45.93000002,-182.64995));
#233751=CARTESIAN_POINT('',(61.6666822880186,-46.43000002,-182.64995));
#233752=CARTESIAN_POINT('Origin',(61.6666822880186,-45.93000002,-182.64995));
#233753=CARTESIAN_POINT('',(61.6666822880186,-46.43000002,-189.64995));
#233754=CARTESIAN_POINT('',(61.6666822880186,-46.43000002,-236.10005));
#233755=CARTESIAN_POINT('',(62.1666822880186,-45.93000002,-189.64995));
#233756=CARTESIAN_POINT('Origin',(61.6666822880186,-45.93000002,-189.64995));
#233757=CARTESIAN_POINT('',(62.1666822880186,-45.93000002,-189.64995));
#233758=CARTESIAN_POINT('Origin',(59.1666822880186,-45.93000002,-182.64995));
#233759=CARTESIAN_POINT('',(59.1666822880186,-45.93000002,-179.64995));
#233760=CARTESIAN_POINT('',(59.1666822880186,-46.43000002,-180.14995));
#233761=CARTESIAN_POINT('Origin',(59.1666822880186,-45.93000002,-180.14995));
#233762=CARTESIAN_POINT('Origin',(59.1666822880186,-46.43000002,-182.64995));
#233763=CARTESIAN_POINT('Origin',(59.1666822880186,-45.93000002,-182.64995));
#233764=CARTESIAN_POINT('Origin',(51.5042290374232,-45.93000002,-180.14995));
#233765=CARTESIAN_POINT('',(51.9388724063314,-45.93000002,-179.64995));
#233766=CARTESIAN_POINT('',(51.9388724063314,-46.43000002,-180.14995));
#233767=CARTESIAN_POINT('Origin',(51.9388724063314,-45.93000002,-180.14995));
#233768=CARTESIAN_POINT('',(51.9388724063314,-46.43000002,-180.14995));
#233769=CARTESIAN_POINT('',(59.1666822880186,-45.93000002,-179.64995));
#233770=CARTESIAN_POINT('Origin',(51.9388724063314,-46.93000002,-180.14995));
#233771=CARTESIAN_POINT('',(50.9486043375898,-46.7908269190399,-179.64995));
#233772=CARTESIAN_POINT('',(51.4437383719606,-46.8604134695199,-180.14995));
#233773=CARTESIAN_POINT('Origin',(50.9486043375898,-46.7908269190399,-180.14995));
#233774=CARTESIAN_POINT('Origin',(51.9388724063314,-46.93000002,-180.14995));
#233775=CARTESIAN_POINT('Origin',(51.9388724063314,-46.93000002,-179.64995));
#233776=CARTESIAN_POINT('Origin',(52.1173462765794,-38.4747959130728,-180.14995));
#233777=CARTESIAN_POINT('',(50.1545486215213,-52.4408269190399,-179.64995));
#233778=CARTESIAN_POINT('',(50.6496826558921,-52.51041346952,-180.14995));
#233779=CARTESIAN_POINT('Origin',(50.1545486215213,-52.4408269190399,-180.14995));
#233780=CARTESIAN_POINT('',(52.6124803109501,-38.5443824635529,-180.14995));
#233781=CARTESIAN_POINT('',(50.0744984522816,-53.0104134695199,-179.64995));
#233782=CARTESIAN_POINT('Origin',(51.1448166902628,-52.58000002,-180.14995));
#233783=CARTESIAN_POINT('',(51.1448166902628,-53.58000002,-179.64995));
#233784=CARTESIAN_POINT('',(51.1448166902628,-53.08000002,-180.14995));
#233785=CARTESIAN_POINT('Origin',(51.1448166902628,-53.58000002,-180.14995));
#233786=CARTESIAN_POINT('Origin',(51.1448166902628,-52.58000002,-180.14995));
#233787=CARTESIAN_POINT('Origin',(51.1448166902628,-52.58000002,-179.64995));
#233788=CARTESIAN_POINT('Origin',(50.5696324866523,-53.58000002,-180.14995));
#233789=CARTESIAN_POINT('',(59.1666822880186,-53.58000002,-179.64995));
#233790=CARTESIAN_POINT('',(59.1666822880186,-53.08000002,-180.14995));
#233791=CARTESIAN_POINT('Origin',(59.1666822880186,-53.58000002,-180.14995));
#233792=CARTESIAN_POINT('',(59.1666822880186,-53.08000002,-180.14995));
#233793=CARTESIAN_POINT('',(51.1448166902628,-53.58000002,-179.64995));
#233794=CARTESIAN_POINT('Origin',(59.1666822880186,-53.58000002,-182.64995));
#233795=CARTESIAN_POINT('',(62.1666822880186,-53.58000002,-182.64995));
#233796=CARTESIAN_POINT('',(61.6666822880186,-53.08000002,-182.64995));
#233797=CARTESIAN_POINT('Origin',(61.6666822880186,-53.58000002,-182.64995));
#233798=CARTESIAN_POINT('Origin',(59.1666822880186,-53.08000002,-182.64995));
#233799=CARTESIAN_POINT('Origin',(59.1666822880186,-53.58000002,-182.64995));
#233800=CARTESIAN_POINT('Origin',(61.6666822880186,-53.58000002,-189.64995));
#233801=CARTESIAN_POINT('',(61.6666822880186,-53.08000002,-189.64995));
#233802=CARTESIAN_POINT('',(62.1666822880186,-53.58000002,-189.64995));
#233803=CARTESIAN_POINT('Origin',(61.6666822880186,-53.58000002,-189.64995));
#233804=CARTESIAN_POINT('',(61.6666822880186,-53.08000002,-236.10005));
#233805=CARTESIAN_POINT('',(62.1666822880186,-53.58000002,-189.64995));
#233806=CARTESIAN_POINT('Origin',(61.6666822880186,-53.9537553161325,-189.64995));
#233807=CARTESIAN_POINT('',(62.1666822880186,-53.9537553161325,-189.64995));
#233808=CARTESIAN_POINT('',(61.6666822880186,-54.4537553161325,-189.64995));
#233809=CARTESIAN_POINT('Origin',(61.6666822880186,-53.9537553161325,-189.64995));
#233810=CARTESIAN_POINT('',(62.1666822880186,-53.9537553161325,-182.64995));
#233811=CARTESIAN_POINT('',(62.1666822880186,-53.9537553161325,-189.64995));
#233812=CARTESIAN_POINT('',(61.6666822880186,-54.4537553161325,-182.64995));
#233813=CARTESIAN_POINT('Origin',(61.6666822880186,-53.9537553161325,-182.64995));
#233814=CARTESIAN_POINT('',(61.6666822880186,-54.4537553161325,-189.64995));
#233815=CARTESIAN_POINT('Origin',(59.1666822880186,-53.9537553161325,-182.64995));
#233816=CARTESIAN_POINT('',(59.1666822880186,-53.9537553161325,-179.64995));
#233817=CARTESIAN_POINT('',(59.1666822880186,-54.4537553161325,-180.14995));
#233818=CARTESIAN_POINT('Origin',(59.1666822880186,-53.9537553161325,-180.14995));
#233819=CARTESIAN_POINT('Origin',(59.1666822880186,-54.4537553161325,-182.64995));
#233820=CARTESIAN_POINT('Origin',(59.1666822880186,-53.9537553161325,-182.64995));
#233821=CARTESIAN_POINT('Origin',(62.1666822880186,-53.9537553161325,-180.14995));
#233822=CARTESIAN_POINT('',(53.361677340714,-53.9537553161325,-179.64995));
#233823=CARTESIAN_POINT('',(53.361677340714,-54.4537553161325,-180.14995));
#233824=CARTESIAN_POINT('Origin',(53.361677340714,-53.9537553161325,-180.14995));
#233825=CARTESIAN_POINT('',(53.361677340714,-54.4537553161325,-180.14995));
#233826=CARTESIAN_POINT('',(59.1666822880186,-53.9537553161325,-179.64995));
#233827=CARTESIAN_POINT('Origin',(53.361677340714,-54.9537553161325,-180.14995));
#233828=CARTESIAN_POINT('',(52.6545705595274,-55.6608620973191,-179.64995));
#233829=CARTESIAN_POINT('',(53.0081239501207,-55.3073087067258,-180.14995));
#233830=CARTESIAN_POINT('Origin',(52.6545705595274,-55.6608620973191,-180.14995));
#233831=CARTESIAN_POINT('Origin',(53.361677340714,-54.9537553161325,-180.14995));
#233832=CARTESIAN_POINT('Origin',(53.361677340714,-54.9537553161325,-179.64995));
#233833=CARTESIAN_POINT('Origin',(59.2455673951362,-62.2518589329279,-180.14995));
#233834=CARTESIAN_POINT('',(59.5991207857295,-61.8983055423346,-180.14995));
#233835=CARTESIAN_POINT('',(59.2791589653485,-62.2854505031402,-179.64995));
#233836=CARTESIAN_POINT('Ctrl Pts',(59.5991207857295,-61.8983055423347,
-180.14995));
#233837=CARTESIAN_POINT('Ctrl Pts',(59.5991207857295,-61.8983055423347,
-180.087180970045));
#233838=CARTESIAN_POINT('Ctrl Pts',(59.591125231612,-61.9080494267527,-180.020249867196));
#233839=CARTESIAN_POINT('Ctrl Pts',(59.558623384557,-61.947597642818,-179.89717444851));
#233840=CARTESIAN_POINT('Ctrl Pts',(59.5341151062373,-61.9773974043459,
-179.841029188496));
#233841=CARTESIAN_POINT('Ctrl Pts',(59.4774393533586,-62.0461626981974,
-179.752172507515));
#233842=CARTESIAN_POINT('Ctrl Pts',(59.4414409519271,-62.0897745954456,
-179.713616638591));
#233843=CARTESIAN_POINT('Ctrl Pts',(59.3624719505921,-62.1851765785503,
-179.662506000476));
#233844=CARTESIAN_POINT('Ctrl Pts',(59.3194982880101,-62.2369634695716,
-179.64995));
#233845=CARTESIAN_POINT('Ctrl Pts',(59.2791589653485,-62.2854505031402,
-179.64995));
#233846=CARTESIAN_POINT('',(59.5991207857295,-61.8983055423346,-180.14995));
#233847=CARTESIAN_POINT('',(52.6545705595274,-55.6608620973191,-179.64995));
#233848=CARTESIAN_POINT('Origin',(61.6666822880186,-37.78000002,-189.64995));
#233849=CARTESIAN_POINT('',(62.1666822880186,-37.78000002,-182.64995));
#233850=CARTESIAN_POINT('',(61.6666822880186,-38.28000002,-182.64995));
#233851=CARTESIAN_POINT('Origin',(61.6666822880186,-37.78000002,-182.64995));
#233852=CARTESIAN_POINT('',(61.6666822880186,-38.28000002,-189.64995));
#233853=CARTESIAN_POINT('',(61.6666822880186,-38.28000002,-236.10005));
#233854=CARTESIAN_POINT('',(62.1666822880186,-37.78000002,-189.64995));
#233855=CARTESIAN_POINT('Origin',(61.6666822880186,-37.78000002,-189.64995));
#233856=CARTESIAN_POINT('',(62.1666822880186,-37.78000002,-189.64995));
#233857=CARTESIAN_POINT('Origin',(59.1666822880186,-37.78000002,-182.64995));
#233858=CARTESIAN_POINT('',(59.1666822880186,-37.78000002,-179.64995));
#233859=CARTESIAN_POINT('',(59.1666822880186,-38.28000002,-180.14995));
#233860=CARTESIAN_POINT('Origin',(59.1666822880186,-37.78000002,-180.14995));
#233861=CARTESIAN_POINT('Origin',(59.1666822880186,-38.28000002,-182.64995));
#233862=CARTESIAN_POINT('Origin',(59.1666822880186,-37.78000002,-182.64995));
#233863=CARTESIAN_POINT('Origin',(52.7401871797155,-37.78000002,-180.14995));
#233864=CARTESIAN_POINT('',(53.1262583325313,-37.78000002,-179.64995));
#233865=CARTESIAN_POINT('',(53.1262583325313,-38.28000002,-180.14995));
#233866=CARTESIAN_POINT('Origin',(53.1262583325313,-37.78000002,-180.14995));
#233867=CARTESIAN_POINT('',(53.1262583325313,-38.28000002,-180.14995));
#233868=CARTESIAN_POINT('',(59.1666822880186,-37.78000002,-179.64995));
#233869=CARTESIAN_POINT('Origin',(53.1262583325313,-38.78000002,-180.14995));
#233870=CARTESIAN_POINT('',(52.1640112991968,-38.5078224183517,-179.64995));
#233871=CARTESIAN_POINT('',(52.6451348158641,-38.6439112191758,-180.14995));
#233872=CARTESIAN_POINT('Origin',(52.1640112991968,-38.5078224183517,-180.14995));
#233873=CARTESIAN_POINT('Origin',(53.1262583325313,-38.78000002,-180.14995));
#233874=CARTESIAN_POINT('Origin',(53.1262583325313,-38.78000002,-179.64995));
#233875=CARTESIAN_POINT('Origin',(57.4563699825363,-40.0047992274175,-180.14995));
#233876=CARTESIAN_POINT('',(52.0098956044577,-39.2393471721372,-179.64995));
#233877=CARTESIAN_POINT('',(52.5050296388285,-39.3089337226171,-180.14995));
#233878=CARTESIAN_POINT('Origin',(52.0098956044577,-39.2393471721372,-180.14995));
#233879=CARTESIAN_POINT('Origin',(57.4563699825363,-40.0047992274175,-180.14995));
#233880=CARTESIAN_POINT('Origin',(57.4563699825363,-40.0047992274175,-179.64995));
#233881=CARTESIAN_POINT('Origin',(52.1173462765794,-38.4747959130728,-180.14995));
#233882=CARTESIAN_POINT('',(51.2999564243458,-44.2908269190399,-179.64995));
#233883=CARTESIAN_POINT('',(51.7950904587165,-44.36041346952,-180.14995));
#233884=CARTESIAN_POINT('Origin',(51.2999564243458,-44.2908269190399,-180.14995));
#233885=CARTESIAN_POINT('',(52.6124803109501,-38.5443824635529,-180.14995));
#233886=CARTESIAN_POINT('',(50.0744984522816,-53.0104134695199,-179.64995));
#233887=CARTESIAN_POINT('Origin',(52.2902244930873,-44.43000002,-180.14995));
#233888=CARTESIAN_POINT('',(52.2902244930873,-45.43000002,-179.64995));
#233889=CARTESIAN_POINT('',(52.2902244930873,-44.93000002,-180.14995));
#233890=CARTESIAN_POINT('Origin',(52.2902244930873,-45.43000002,-180.14995));
#233891=CARTESIAN_POINT('Origin',(52.2902244930873,-44.43000002,-180.14995));
#233892=CARTESIAN_POINT('Origin',(52.2902244930873,-44.43000002,-179.64995));
#233893=CARTESIAN_POINT('Origin',(51.7150402894768,-45.43000002,-180.14995));
#233894=CARTESIAN_POINT('',(59.1666822880186,-45.43000002,-179.64995));
#233895=CARTESIAN_POINT('',(59.1666822880186,-44.93000002,-180.14995));
#233896=CARTESIAN_POINT('Origin',(59.1666822880186,-45.43000002,-180.14995));
#233897=CARTESIAN_POINT('',(59.1666822880186,-44.93000002,-180.14995));
#233898=CARTESIAN_POINT('',(52.2902244930873,-45.43000002,-179.64995));
#233899=CARTESIAN_POINT('Origin',(59.1666822880186,-45.43000002,-182.64995));
#233900=CARTESIAN_POINT('',(62.1666822880186,-45.43000002,-182.64995));
#233901=CARTESIAN_POINT('',(61.6666822880186,-44.93000002,-182.64995));
#233902=CARTESIAN_POINT('Origin',(61.6666822880186,-45.43000002,-182.64995));
#233903=CARTESIAN_POINT('Origin',(59.1666822880186,-44.93000002,-182.64995));
#233904=CARTESIAN_POINT('Origin',(59.1666822880186,-45.43000002,-182.64995));
#233905=CARTESIAN_POINT('Origin',(61.6666822880186,-45.43000002,-189.64995));
#233906=CARTESIAN_POINT('',(61.6666822880186,-44.93000002,-189.64995));
#233907=CARTESIAN_POINT('',(62.1666822880186,-45.43000002,-189.64995));
#233908=CARTESIAN_POINT('Origin',(61.6666822880186,-45.43000002,-189.64995));
#233909=CARTESIAN_POINT('',(61.6666822880186,-44.93000002,-236.10005));
#233910=CARTESIAN_POINT('',(62.1666822880186,-45.43000002,-189.64995));
#233911=CARTESIAN_POINT('Origin',(61.6666822880186,-29.63000002,-189.64995));
#233912=CARTESIAN_POINT('',(62.1666822880186,-29.63000002,-182.64995));
#233913=CARTESIAN_POINT('',(61.6666822880186,-30.13000002,-182.64995));
#233914=CARTESIAN_POINT('Origin',(61.6666822880186,-29.63000002,-182.64995));
#233915=CARTESIAN_POINT('',(61.6666822880186,-30.13000002,-189.64995));
#233916=CARTESIAN_POINT('',(61.6666822880186,-30.13000002,-236.10005));
#233917=CARTESIAN_POINT('',(62.1666822880186,-29.63000002,-189.64995));
#233918=CARTESIAN_POINT('Origin',(61.6666822880186,-29.63000002,-189.64995));
#233919=CARTESIAN_POINT('',(62.1666822880186,-29.63000002,-189.64995));
#233920=CARTESIAN_POINT('Origin',(59.1666822880186,-29.63000002,-182.64995));
#233921=CARTESIAN_POINT('',(59.1666822880186,-29.63000002,-179.64995));
#233922=CARTESIAN_POINT('',(59.1666822880186,-30.13000002,-180.14995));
#233923=CARTESIAN_POINT('Origin',(59.1666822880186,-29.63000002,-180.14995));
#233924=CARTESIAN_POINT('Origin',(59.1666822880186,-30.13000002,-182.64995));
#233925=CARTESIAN_POINT('Origin',(59.1666822880186,-29.63000002,-182.64995));
#233926=CARTESIAN_POINT('Origin',(55.9258311851596,-29.63000002,-180.14995));
#233927=CARTESIAN_POINT('',(56.294192362543,-29.63000002,-179.64995));
#233928=CARTESIAN_POINT('',(56.294192362543,-30.13000002,-180.14995));
#233929=CARTESIAN_POINT('Origin',(56.294192362543,-29.63000002,-180.14995));
#233930=CARTESIAN_POINT('',(56.294192362543,-30.13000002,-180.14995));
#233931=CARTESIAN_POINT('',(59.1666822880186,-29.63000002,-179.64995));
#233932=CARTESIAN_POINT('Origin',(56.294192362543,-30.63000002,-180.14995));
#233933=CARTESIAN_POINT('',(55.3400535089406,-30.3306356132208,-179.64995));
#233934=CARTESIAN_POINT('',(55.8171229357418,-30.4803178166104,-180.14995));
#233935=CARTESIAN_POINT('Origin',(55.3400535089406,-30.3306356132208,-180.14995));
#233936=CARTESIAN_POINT('Origin',(56.294192362543,-30.63000002,-180.14995));
#233937=CARTESIAN_POINT('Origin',(56.294192362543,-30.63000002,-179.64995));
#233938=CARTESIAN_POINT('Origin',(0.,-12.9675000200281,-180.14995));
#233939=CARTESIAN_POINT('',(53.2803342727705,-35.8848729013564,-179.64995));
#233940=CARTESIAN_POINT('',(53.7396474992599,-36.0824364606782,-180.14995));
#233941=CARTESIAN_POINT('Origin',(53.2803342727705,-35.8848729013564,-180.14995));
#233942=CARTESIAN_POINT('Origin',(0.,-12.9675000200281,-180.14995));
#233943=CARTESIAN_POINT('Origin',(0.,-12.9675000200281,-179.64995));
#233944=CARTESIAN_POINT('Origin',(54.1989607257493,-36.28000002,-180.14995));
#233945=CARTESIAN_POINT('',(54.1989607257493,-37.28000002,-179.64995));
#233946=CARTESIAN_POINT('',(54.1989607257493,-36.78000002,-180.14995));
#233947=CARTESIAN_POINT('Origin',(54.1989607257493,-37.28000002,-180.14995));
#233948=CARTESIAN_POINT('Origin',(54.1989607257493,-36.28000002,-180.14995));
#233949=CARTESIAN_POINT('Origin',(54.1989607257493,-36.28000002,-179.64995));
#233950=CARTESIAN_POINT('Origin',(53.4342104250764,-37.28000002,-180.14995));
#233951=CARTESIAN_POINT('',(59.1666822880186,-37.28000002,-179.64995));
#233952=CARTESIAN_POINT('',(59.1666822880186,-36.78000002,-180.14995));
#233953=CARTESIAN_POINT('Origin',(59.1666822880186,-37.28000002,-180.14995));
#233954=CARTESIAN_POINT('',(59.1666822880186,-36.78000002,-180.14995));
#233955=CARTESIAN_POINT('',(54.1989607257493,-37.28000002,-179.64995));
#233956=CARTESIAN_POINT('Origin',(59.1666822880186,-37.28000002,-182.64995));
#233957=CARTESIAN_POINT('',(62.1666822880186,-37.28000002,-182.64995));
#233958=CARTESIAN_POINT('',(61.6666822880186,-36.78000002,-182.64995));
#233959=CARTESIAN_POINT('Origin',(61.6666822880186,-37.28000002,-182.64995));
#233960=CARTESIAN_POINT('Origin',(59.1666822880186,-36.78000002,-182.64995));
#233961=CARTESIAN_POINT('Origin',(59.1666822880186,-37.28000002,-182.64995));
#233962=CARTESIAN_POINT('Origin',(61.6666822880186,-37.28000002,-189.64995));
#233963=CARTESIAN_POINT('',(61.6666822880186,-36.78000002,-189.64995));
#233964=CARTESIAN_POINT('',(62.1666822880186,-37.28000002,-189.64995));
#233965=CARTESIAN_POINT('Origin',(61.6666822880186,-37.28000002,-189.64995));
#233966=CARTESIAN_POINT('',(61.6666822880186,-36.78000002,-236.10005));
#233967=CARTESIAN_POINT('',(62.1666822880186,-37.28000002,-189.64995));
#233968=CARTESIAN_POINT('Origin',(61.6666822880186,-21.48000002,-189.64995));
#233969=CARTESIAN_POINT('',(62.1666822880186,-21.48000002,-182.64995));
#233970=CARTESIAN_POINT('',(61.6666822880186,-21.98000002,-182.64995));
#233971=CARTESIAN_POINT('Origin',(61.6666822880186,-21.48000002,-182.64995));
#233972=CARTESIAN_POINT('',(61.6666822880186,-21.98000002,-189.64995));
#233973=CARTESIAN_POINT('',(61.6666822880186,-21.98000002,-236.10005));
#233974=CARTESIAN_POINT('',(62.1666822880186,-21.48000002,-189.64995));
#233975=CARTESIAN_POINT('Origin',(61.6666822880186,-21.48000002,-189.64995));
#233976=CARTESIAN_POINT('',(62.1666822880186,-21.48000002,-189.64995));
#233977=CARTESIAN_POINT('Origin',(59.1666822880186,-21.48000002,-182.64995));
#233978=CARTESIAN_POINT('',(59.1666822880186,-21.48000002,-179.64995));
#233979=CARTESIAN_POINT('',(59.1666822880186,-21.98000002,-180.14995));
#233980=CARTESIAN_POINT('Origin',(59.1666822880186,-21.48000002,-180.14995));
#233981=CARTESIAN_POINT('Origin',(59.1666822880186,-21.98000002,-182.64995));
#233982=CARTESIAN_POINT('Origin',(59.1666822880186,-21.48000002,-182.64995));
#233983=CARTESIAN_POINT('Origin',(57.8015989722647,-21.48000002,-180.14995));
#233984=CARTESIAN_POINT('',(58.2281061322669,-21.48000002,-179.64995));
#233985=CARTESIAN_POINT('',(58.2281061322669,-21.98000002,-180.14995));
#233986=CARTESIAN_POINT('Origin',(58.2281061322669,-21.48000002,-180.14995));
#233987=CARTESIAN_POINT('',(58.2281061322669,-21.98000002,-180.14995));
#233988=CARTESIAN_POINT('',(59.1666822880186,-21.48000002,-179.64995));
#233989=CARTESIAN_POINT('Origin',(58.2281061322669,-22.48000002,-180.14995));
#233990=CARTESIAN_POINT('',(57.2411890791776,-22.3187712064411,-179.64995));
#233991=CARTESIAN_POINT('',(57.7346476057223,-22.3993856132206,-180.14995));
#233992=CARTESIAN_POINT('Origin',(57.2411890791776,-22.3187712064411,-180.14995));
#233993=CARTESIAN_POINT('Origin',(58.2281061322669,-22.48000002,-180.14995));
#233994=CARTESIAN_POINT('Origin',(58.2281061322669,-22.48000002,-179.64995));
#233995=CARTESIAN_POINT('Origin',(0.,-12.9675000200281,-180.14995));
#233996=CARTESIAN_POINT('',(56.051992088731,-27.8730084945768,-179.64995));
#233997=CARTESIAN_POINT('',(56.5351989170821,-28.0015042572884,-180.14995));
#233998=CARTESIAN_POINT('Origin',(56.051992088731,-27.8730084945768,-180.14995));
#233999=CARTESIAN_POINT('Origin',(0.,-12.9675000200281,-180.14995));
#234000=CARTESIAN_POINT('Origin',(0.,-12.9675000200281,-179.64995));
#234001=CARTESIAN_POINT('Origin',(57.0184057454332,-28.13000002,-180.14995));
#234002=CARTESIAN_POINT('',(57.0184057454332,-29.13000002,-179.64995));
#234003=CARTESIAN_POINT('',(57.0184057454332,-28.63000002,-180.14995));
#234004=CARTESIAN_POINT('Origin',(57.0184057454332,-29.13000002,-180.14995));
#234005=CARTESIAN_POINT('Origin',(57.0184057454332,-28.13000002,-180.14995));
#234006=CARTESIAN_POINT('Origin',(57.0184057454332,-28.13000002,-179.64995));
#234007=CARTESIAN_POINT('Origin',(56.3643157835779,-29.13000002,-180.14995));
#234008=CARTESIAN_POINT('',(59.1666822880186,-29.13000002,-179.64995));
#234009=CARTESIAN_POINT('',(59.1666822880186,-28.63000002,-180.14995));
#234010=CARTESIAN_POINT('Origin',(59.1666822880186,-29.13000002,-180.14995));
#234011=CARTESIAN_POINT('',(59.1666822880186,-28.63000002,-180.14995));
#234012=CARTESIAN_POINT('',(57.0184057454332,-29.13000002,-179.64995));
#234013=CARTESIAN_POINT('Origin',(59.1666822880186,-29.13000002,-182.64995));
#234014=CARTESIAN_POINT('',(62.1666822880186,-29.13000002,-182.64995));
#234015=CARTESIAN_POINT('',(61.6666822880186,-28.63000002,-182.64995));
#234016=CARTESIAN_POINT('Origin',(61.6666822880186,-29.13000002,-182.64995));
#234017=CARTESIAN_POINT('Origin',(59.1666822880186,-28.63000002,-182.64995));
#234018=CARTESIAN_POINT('Origin',(59.1666822880186,-29.13000002,-182.64995));
#234019=CARTESIAN_POINT('Origin',(61.6666822880186,-29.13000002,-189.64995));
#234020=CARTESIAN_POINT('',(61.6666822880186,-28.63000002,-189.64995));
#234021=CARTESIAN_POINT('',(62.1666822880186,-29.13000002,-189.64995));
#234022=CARTESIAN_POINT('Origin',(61.6666822880186,-29.13000002,-189.64995));
#234023=CARTESIAN_POINT('',(61.6666822880186,-28.63000002,-236.10005));
#234024=CARTESIAN_POINT('',(62.1666822880186,-29.13000002,-189.64995));
#234025=CARTESIAN_POINT('Origin',(61.6666822880186,-13.33000002,-189.64995));
#234026=CARTESIAN_POINT('',(62.1666822880186,-13.33000002,-182.64995));
#234027=CARTESIAN_POINT('',(61.6666822880186,-13.83000002,-182.64995));
#234028=CARTESIAN_POINT('Origin',(61.6666822880186,-13.33000002,-182.64995));
#234029=CARTESIAN_POINT('',(61.6666822880186,-13.83000002,-189.64995));
#234030=CARTESIAN_POINT('',(61.6666822880186,-13.83000002,-236.10005));
#234031=CARTESIAN_POINT('',(62.1666822880186,-13.33000002,-189.64995));
#234032=CARTESIAN_POINT('Origin',(61.6666822880186,-13.33000002,-189.64995));
#234033=CARTESIAN_POINT('',(62.1666822880186,-13.33000002,-189.64995));
#234034=CARTESIAN_POINT('Origin',(59.1666822880186,-13.33000002,-182.64995));
#234035=CARTESIAN_POINT('',(59.1666822880186,-13.33000002,-179.64995));
#234036=CARTESIAN_POINT('',(59.1666822880186,-13.83000002,-180.14995));
#234037=CARTESIAN_POINT('Origin',(59.1666822880186,-13.33000002,-180.14995));
#234038=CARTESIAN_POINT('Origin',(59.1666822880186,-13.83000002,-182.64995));
#234039=CARTESIAN_POINT('Origin',(59.1666822880186,-13.33000002,-182.64995));
#234040=CARTESIAN_POINT('Origin',(58.4936414813615,-13.33000002,-180.14995));
#234041=CARTESIAN_POINT('',(58.9842656455946,-13.33000002,-179.64995));
#234042=CARTESIAN_POINT('',(58.9842656455946,-13.83000002,-180.14995));
#234043=CARTESIAN_POINT('Origin',(58.9842656455946,-13.33000002,-180.14995));
#234044=CARTESIAN_POINT('',(58.9842656455946,-13.83000002,-180.14995));
#234045=CARTESIAN_POINT('',(59.1666822880186,-13.33000002,-179.64995));
#234046=CARTESIAN_POINT('Origin',(58.9842656455946,-14.33000002,-180.14995));
#234047=CARTESIAN_POINT('',(57.9845323295676,-14.3069067996615,-179.64995));
#234048=CARTESIAN_POINT('',(58.4843989875811,-14.3184534098307,-180.14995));
#234049=CARTESIAN_POINT('Origin',(57.9845323295676,-14.3069067996615,-180.14995));
#234050=CARTESIAN_POINT('Origin',(58.9842656455946,-14.33000002,-180.14995));
#234051=CARTESIAN_POINT('Origin',(58.9842656455946,-14.33000002,-179.64995));
#234052=CARTESIAN_POINT('Origin',(0.,-12.9675000200281,-180.14995));
#234053=CARTESIAN_POINT('',(57.588867600144,-19.8611440877971,-179.64995));
#234054=CARTESIAN_POINT('',(58.0853233553177,-19.9205720538985,-180.14995));
#234055=CARTESIAN_POINT('Origin',(57.588867600144,-19.8611440877971,-180.14995));
#234056=CARTESIAN_POINT('Origin',(0.,-12.9675000200281,-180.14995));
#234057=CARTESIAN_POINT('Origin',(0.,-12.9675000200281,-179.64995));
#234058=CARTESIAN_POINT('Origin',(58.5817791104913,-19.98000002,-180.14995));
#234059=CARTESIAN_POINT('',(58.5817791104913,-20.98000002,-179.64995));
#234060=CARTESIAN_POINT('',(58.5817791104913,-20.48000002,-180.14995));
#234061=CARTESIAN_POINT('Origin',(58.5817791104913,-20.98000002,-180.14995));
#234062=CARTESIAN_POINT('Origin',(58.5817791104913,-19.98000002,-180.14995));
#234063=CARTESIAN_POINT('Origin',(58.5817791104913,-19.98000002,-179.64995));
#234064=CARTESIAN_POINT('Origin',(58.0156215492899,-20.98000002,-180.14995));
#234065=CARTESIAN_POINT('',(59.1666822880186,-20.98000002,-179.64995));
#234066=CARTESIAN_POINT('',(59.1666822880186,-20.48000002,-180.14995));
#234067=CARTESIAN_POINT('Origin',(59.1666822880186,-20.98000002,-180.14995));
#234068=CARTESIAN_POINT('',(59.1666822880186,-20.48000002,-180.14995));
#234069=CARTESIAN_POINT('',(58.5817791104913,-20.98000002,-179.64995));
#234070=CARTESIAN_POINT('Origin',(59.1666822880186,-20.98000002,-182.64995));
#234071=CARTESIAN_POINT('',(62.1666822880186,-20.98000002,-182.64995));
#234072=CARTESIAN_POINT('',(61.6666822880186,-20.48000002,-182.64995));
#234073=CARTESIAN_POINT('Origin',(61.6666822880186,-20.98000002,-182.64995));
#234074=CARTESIAN_POINT('Origin',(59.1666822880186,-20.48000002,-182.64995));
#234075=CARTESIAN_POINT('Origin',(59.1666822880186,-20.98000002,-182.64995));
#234076=CARTESIAN_POINT('Origin',(61.6666822880186,-20.98000002,-189.64995));
#234077=CARTESIAN_POINT('',(61.6666822880186,-20.48000002,-189.64995));
#234078=CARTESIAN_POINT('',(62.1666822880186,-20.98000002,-189.64995));
#234079=CARTESIAN_POINT('Origin',(61.6666822880186,-20.98000002,-189.64995));
#234080=CARTESIAN_POINT('',(61.6666822880186,-20.48000002,-236.10005));
#234081=CARTESIAN_POINT('',(62.1666822880186,-20.98000002,-189.64995));
#234082=CARTESIAN_POINT('Origin',(61.6666822880186,-5.18000001999998,-189.64995));
#234083=CARTESIAN_POINT('',(62.1666822880186,-5.18000001999998,-182.64995));
#234084=CARTESIAN_POINT('',(61.6666822880186,-5.68000001999998,-182.64995));
#234085=CARTESIAN_POINT('Origin',(61.6666822880186,-5.18000001999998,-182.64995));
#234086=CARTESIAN_POINT('',(61.6666822880186,-5.68000001999998,-189.64995));
#234087=CARTESIAN_POINT('',(61.6666822880186,-5.68000001999998,-236.10005));
#234088=CARTESIAN_POINT('',(62.1666822880186,-5.18000001999998,-189.64995));
#234089=CARTESIAN_POINT('Origin',(61.6666822880186,-5.18000001999998,-189.64995));
#234090=CARTESIAN_POINT('',(62.1666822880186,-5.18000001999998,-189.64995));
#234091=CARTESIAN_POINT('Origin',(59.1666822880186,-5.18000001999998,-182.64995));
#234092=CARTESIAN_POINT('',(59.1666822880186,-5.18000001999998,-179.64995));
#234093=CARTESIAN_POINT('',(59.1666822880186,-5.68000001999998,-180.14995));
#234094=CARTESIAN_POINT('Origin',(59.1666822880186,-5.18000001999998,-180.14995));
#234095=CARTESIAN_POINT('Origin',(59.1666822880186,-5.68000001999998,-182.64995));
#234096=CARTESIAN_POINT('Origin',(59.1666822880186,-5.18000001999998,-182.64995));
#234097=CARTESIAN_POINT('Origin',(58.0443136211429,-5.18000001999998,-180.14995));
#234098=CARTESIAN_POINT('',(58.6082745331205,-5.18000001999998,-179.64995));
#234099=CARTESIAN_POINT('',(58.6082745331205,-5.68000001999998,-180.14995));
#234100=CARTESIAN_POINT('Origin',(58.6082745331205,-5.18000001999998,-180.14995));
#234101=CARTESIAN_POINT('',(58.6082745331205,-5.68000001999998,-180.14995));
#234102=CARTESIAN_POINT('',(59.1666822880186,-5.18000001999998,-179.64995));
#234103=CARTESIAN_POINT('Origin',(58.6082745331205,-6.18000001999998,-180.14995));
#234104=CARTESIAN_POINT('',(57.6149139478134,-6.29504239288181,-179.64995));
#234105=CARTESIAN_POINT('',(58.1115942404669,-6.2375212064409,-180.14995));
#234106=CARTESIAN_POINT('Origin',(57.6149139478134,-6.29504239288181,-180.14995));
#234107=CARTESIAN_POINT('Origin',(58.6082745331205,-6.18000001999998,-180.14995));
#234108=CARTESIAN_POINT('Origin',(58.6082745331205,-6.18000001999998,-179.64995));
#234109=CARTESIAN_POINT('Origin',(0.,-12.9675000200281,-180.14995));
#234110=CARTESIAN_POINT('',(57.9892195435792,-11.8492796810174,-179.64995));
#234111=CARTESIAN_POINT('',(58.48912660861,-11.8396398505087,-180.14995));
#234112=CARTESIAN_POINT('Origin',(57.9892195435792,-11.8492796810174,-180.14995));
#234113=CARTESIAN_POINT('Origin',(0.,-12.9675000200281,-180.14995));
#234114=CARTESIAN_POINT('Origin',(0.,-12.9675000200281,-179.64995));
#234115=CARTESIAN_POINT('Origin',(58.9890336736409,-11.83000002,-180.14995));
#234116=CARTESIAN_POINT('',(58.9890336736409,-12.83000002,-179.64995));
#234117=CARTESIAN_POINT('',(58.9890336736409,-12.33000002,-180.14995));
#234118=CARTESIAN_POINT('Origin',(58.9890336736409,-12.83000002,-180.14995));
#234119=CARTESIAN_POINT('Origin',(58.9890336736409,-11.83000002,-180.14995));
#234120=CARTESIAN_POINT('Origin',(58.9890336736409,-11.83000002,-179.64995));
#234121=CARTESIAN_POINT('Origin',(58.4965263391765,-12.83000002,-180.14995));
#234122=CARTESIAN_POINT('',(59.1666822880186,-12.83000002,-179.64995));
#234123=CARTESIAN_POINT('',(59.1666822880186,-12.33000002,-180.14995));
#234124=CARTESIAN_POINT('Origin',(59.1666822880186,-12.83000002,-180.14995));
#234125=CARTESIAN_POINT('',(59.1666822880186,-12.33000002,-180.14995));
#234126=CARTESIAN_POINT('',(58.9890336736409,-12.83000002,-179.64995));
#234127=CARTESIAN_POINT('Origin',(59.1666822880186,-12.83000002,-182.64995));
#234128=CARTESIAN_POINT('',(62.1666822880186,-12.83000002,-182.64995));
#234129=CARTESIAN_POINT('',(61.6666822880186,-12.33000002,-182.64995));
#234130=CARTESIAN_POINT('Origin',(61.6666822880186,-12.83000002,-182.64995));
#234131=CARTESIAN_POINT('Origin',(59.1666822880186,-12.33000002,-182.64995));
#234132=CARTESIAN_POINT('Origin',(59.1666822880186,-12.83000002,-182.64995));
#234133=CARTESIAN_POINT('Origin',(61.6666822880186,-12.83000002,-189.64995));
#234134=CARTESIAN_POINT('',(61.6666822880186,-12.33000002,-189.64995));
#234135=CARTESIAN_POINT('',(62.1666822880186,-12.83000002,-189.64995));
#234136=CARTESIAN_POINT('Origin',(61.6666822880186,-12.83000002,-189.64995));
#234137=CARTESIAN_POINT('',(61.6666822880186,-12.33000002,-236.10005));
#234138=CARTESIAN_POINT('',(62.1666822880186,-12.83000002,-189.64995));
#234139=CARTESIAN_POINT('Origin',(61.6666822880186,2.96999998000002,-189.64995));
#234140=CARTESIAN_POINT('',(62.1666822880186,2.96999998000002,-182.64995));
#234141=CARTESIAN_POINT('',(61.6666822880186,2.46999998000002,-182.64995));
#234142=CARTESIAN_POINT('Origin',(61.6666822880186,2.96999998000002,-182.64995));
#234143=CARTESIAN_POINT('',(61.6666822880186,2.46999998000002,-189.64995));
#234144=CARTESIAN_POINT('',(61.6666822880186,2.46999998000002,-236.10005));
#234145=CARTESIAN_POINT('',(62.1666822880186,2.96999998000002,-189.64995));
#234146=CARTESIAN_POINT('Origin',(61.6666822880186,2.96999998000002,-189.64995));
#234147=CARTESIAN_POINT('',(62.1666822880186,2.96999998000002,-189.64995));
#234148=CARTESIAN_POINT('Origin',(59.1666822880186,2.96999998000002,-182.64995));
#234149=CARTESIAN_POINT('',(59.1666822880186,2.96999998000002,-179.64995));
#234150=CARTESIAN_POINT('',(59.1666822880186,2.46999998000002,-180.14995));
#234151=CARTESIAN_POINT('Origin',(59.1666822880186,2.96999998000002,-180.14995));
#234152=CARTESIAN_POINT('Origin',(59.1666822880186,2.46999998000002,-182.64995));
#234153=CARTESIAN_POINT('Origin',(59.1666822880186,2.96999998000002,-182.64995));
#234154=CARTESIAN_POINT('Origin',(56.4263554888062,2.96999998000002,-180.14995));
#234155=CARTESIAN_POINT('',(57.077763566464,2.96999998000002,-179.64995));
#234156=CARTESIAN_POINT('',(57.077763566464,2.46999998000002,-180.14995));
#234157=CARTESIAN_POINT('Origin',(57.077763566464,2.96999998000002,-180.14995));
#234158=CARTESIAN_POINT('',(57.077763566464,2.46999998000002,-180.14995));
#234159=CARTESIAN_POINT('',(59.1666822880186,2.96999998000002,-179.64995));
#234160=CARTESIAN_POINT('Origin',(57.077763566464,1.96999998000002,-180.14995));
#234161=CARTESIAN_POINT('',(56.1103438449985,1.71682201389785,-179.64995));
#234162=CARTESIAN_POINT('',(56.5940537057312,1.84341099694893,-180.14995));
#234163=CARTESIAN_POINT('Origin',(56.1103438449985,1.71682201389785,-180.14995));
#234164=CARTESIAN_POINT('Origin',(57.077763566464,1.96999998000002,-180.14995));
#234165=CARTESIAN_POINT('Origin',(57.077763566464,1.96999998000002,-179.64995));
#234166=CARTESIAN_POINT('Origin',(0.,-12.9675000200281,-180.14995));
#234167=CARTESIAN_POINT('',(57.276884975832,-3.83741527423775,-179.64995));
#234168=CARTESIAN_POINT('',(57.7706512256236,-3.75870764711887,-180.14995));
#234169=CARTESIAN_POINT('Origin',(57.276884975832,-3.83741527423775,-180.14995));
#234170=CARTESIAN_POINT('Origin',(0.,-12.9675000200281,-180.14995));
#234171=CARTESIAN_POINT('Origin',(0.,-12.9675000200281,-179.64995));
#234172=CARTESIAN_POINT('Origin',(58.2644174754153,-3.68000001999999,-180.14995));
#234173=CARTESIAN_POINT('',(58.2644174754153,-4.68000001999999,-179.64995));
#234174=CARTESIAN_POINT('',(58.2644174754153,-4.18000001999998,-180.14995));
#234175=CARTESIAN_POINT('Origin',(58.2644174754153,-4.68000001999999,-180.14995));
#234176=CARTESIAN_POINT('Origin',(58.2644174754153,-3.68000001999999,-180.14995));
#234177=CARTESIAN_POINT('Origin',(58.2644174754153,-3.68000001999999,-179.64995));
#234178=CARTESIAN_POINT('Origin',(57.8362329664502,-4.68000001999999,-180.14995));
#234179=CARTESIAN_POINT('',(59.1666822880186,-4.68000001999999,-179.64995));
#234180=CARTESIAN_POINT('',(59.1666822880186,-4.18000001999998,-180.14995));
#234181=CARTESIAN_POINT('Origin',(59.1666822880186,-4.68000001999999,-180.14995));
#234182=CARTESIAN_POINT('',(59.1666822880186,-4.18000001999998,-180.14995));
#234183=CARTESIAN_POINT('',(58.2644174754153,-4.68000001999999,-179.64995));
#234184=CARTESIAN_POINT('Origin',(59.1666822880186,-4.68000001999999,-182.64995));
#234185=CARTESIAN_POINT('',(62.1666822880186,-4.68000001999999,-182.64995));
#234186=CARTESIAN_POINT('',(61.6666822880186,-4.18000001999998,-182.64995));
#234187=CARTESIAN_POINT('Origin',(61.6666822880186,-4.68000001999999,-182.64995));
#234188=CARTESIAN_POINT('Origin',(59.1666822880186,-4.18000001999998,-182.64995));
#234189=CARTESIAN_POINT('Origin',(59.1666822880186,-4.68000001999999,-182.64995));
#234190=CARTESIAN_POINT('Origin',(61.6666822880186,-4.68000001999999,-189.64995));
#234191=CARTESIAN_POINT('',(61.6666822880186,-4.18000001999998,-189.64995));
#234192=CARTESIAN_POINT('',(62.1666822880186,-4.68000001999999,-189.64995));
#234193=CARTESIAN_POINT('Origin',(61.6666822880186,-4.68000001999999,-189.64995));
#234194=CARTESIAN_POINT('',(61.6666822880186,-4.18000001999998,-236.10005));
#234195=CARTESIAN_POINT('',(62.1666822880186,-4.68000001999999,-189.64995));
#234196=CARTESIAN_POINT('Origin',(61.6666822880186,11.11999998,-189.64995));
#234197=CARTESIAN_POINT('',(62.1666822880186,11.11999998,-182.64995));
#234198=CARTESIAN_POINT('',(61.6666822880186,10.61999998,-182.64995));
#234199=CARTESIAN_POINT('Origin',(61.6666822880186,11.11999998,-182.64995));
#234200=CARTESIAN_POINT('',(61.6666822880186,10.61999998,-189.64995));
#234201=CARTESIAN_POINT('',(61.6666822880186,10.61999998,-236.10005));
#234202=CARTESIAN_POINT('',(62.1666822880186,11.11999998,-189.64995));
#234203=CARTESIAN_POINT('Origin',(61.6666822880186,11.11999998,-189.64995));
#234204=CARTESIAN_POINT('',(62.1666822880186,11.11999998,-189.64995));
#234205=CARTESIAN_POINT('Origin',(59.1666822880186,11.11999998,-182.64995));
#234206=CARTESIAN_POINT('',(59.1666822880186,11.11999998,-179.64995));
#234207=CARTESIAN_POINT('',(59.1666822880186,10.61999998,-180.14995));
#234208=CARTESIAN_POINT('Origin',(59.1666822880186,11.11999998,-180.14995));
#234209=CARTESIAN_POINT('Origin',(59.1666822880186,10.61999998,-182.64995));
#234210=CARTESIAN_POINT('Origin',(59.1666822880186,11.11999998,-182.64995));
#234211=CARTESIAN_POINT('Origin',(53.533913024817,11.11999998,-180.14995));
#234212=CARTESIAN_POINT('',(54.2951871140408,11.11999998,-179.64995));
#234213=CARTESIAN_POINT('',(54.2951871140408,10.61999998,-180.14995));
#234214=CARTESIAN_POINT('Origin',(54.2951871140408,11.11999998,-180.14995));
#234215=CARTESIAN_POINT('',(54.2951871140408,10.61999998,-180.14995));
#234216=CARTESIAN_POINT('',(59.1666822880186,11.11999998,-179.64995));
#234217=CARTESIAN_POINT('Origin',(54.2951871140408,10.11999998,-180.14995));
#234218=CARTESIAN_POINT('',(53.3749297053282,9.72868642067751,-179.64995));
#234219=CARTESIAN_POINT('',(53.8350584096845,9.92434320033877,-180.14995));
#234220=CARTESIAN_POINT('Origin',(53.3749297053282,9.72868642067751,-180.14995));
#234221=CARTESIAN_POINT('Origin',(54.2951871140408,10.11999998,-180.14995));
#234222=CARTESIAN_POINT('Origin',(54.2951871140408,10.11999998,-179.64995));
#234223=CARTESIAN_POINT('Origin',(0.,-12.9675000200281,-180.14995));
#234224=CARTESIAN_POINT('',(55.4089665961269,4.1744491325419,-179.64995));
#234225=CARTESIAN_POINT('',(55.8866301012659,4.32222455627096,-180.14995));
#234226=CARTESIAN_POINT('Origin',(55.4089665961269,4.1744491325419,-180.14995));
#234227=CARTESIAN_POINT('Origin',(0.,-12.9675000200281,-180.14995));
#234228=CARTESIAN_POINT('Origin',(0.,-12.9675000200281,-179.64995));
#234229=CARTESIAN_POINT('Origin',(56.3642936064049,4.46999998000001,-180.14995));
#234230=CARTESIAN_POINT('',(56.3642936064049,3.46999998000002,-179.64995));
#234231=CARTESIAN_POINT('',(56.3642936064049,3.96999998000001,-180.14995));
#234232=CARTESIAN_POINT('Origin',(56.3642936064049,3.46999998000002,-180.14995));
#234233=CARTESIAN_POINT('Origin',(56.3642936064049,4.46999998000001,-180.14995));
#234234=CARTESIAN_POINT('Origin',(56.3642936064049,4.46999998000001,-179.64995));
#234235=CARTESIAN_POINT('Origin',(55.9943844840627,3.46999998000002,-180.14995));
#234236=CARTESIAN_POINT('',(59.1666822880186,3.46999998000002,-179.64995));
#234237=CARTESIAN_POINT('',(59.1666822880186,3.96999998000001,-180.14995));
#234238=CARTESIAN_POINT('Origin',(59.1666822880186,3.46999998000002,-180.14995));
#234239=CARTESIAN_POINT('',(59.1666822880186,3.96999998000001,-180.14995));
#234240=CARTESIAN_POINT('',(56.3642936064049,3.46999998000002,-179.64995));
#234241=CARTESIAN_POINT('Origin',(59.1666822880186,3.46999998000002,-182.64995));
#234242=CARTESIAN_POINT('',(62.1666822880186,3.46999998000002,-182.64995));
#234243=CARTESIAN_POINT('',(61.6666822880186,3.96999998000001,-182.64995));
#234244=CARTESIAN_POINT('Origin',(61.6666822880186,3.46999998000002,-182.64995));
#234245=CARTESIAN_POINT('Origin',(59.1666822880186,3.96999998000001,-182.64995));
#234246=CARTESIAN_POINT('Origin',(59.1666822880186,3.46999998000002,-182.64995));
#234247=CARTESIAN_POINT('Origin',(61.6666822880186,3.46999998000002,-189.64995));
#234248=CARTESIAN_POINT('',(61.6666822880186,3.96999998000001,-189.64995));
#234249=CARTESIAN_POINT('',(62.1666822880186,3.46999998000002,-189.64995));
#234250=CARTESIAN_POINT('Origin',(61.6666822880186,3.46999998000002,-189.64995));
#234251=CARTESIAN_POINT('',(61.6666822880186,3.96999998000001,-236.10005));
#234252=CARTESIAN_POINT('',(62.1666822880186,3.46999998000002,-189.64995));
#234253=CARTESIAN_POINT('Origin',(61.6666822880186,19.26999998,-189.64995));
#234254=CARTESIAN_POINT('',(62.1666822880186,19.26999998,-182.64995));
#234255=CARTESIAN_POINT('',(61.6666822880186,18.76999998,-182.64995));
#234256=CARTESIAN_POINT('Origin',(61.6666822880186,19.26999998,-182.64995));
#234257=CARTESIAN_POINT('',(61.6666822880186,18.76999998,-189.64995));
#234258=CARTESIAN_POINT('',(61.6666822880186,18.76999998,-236.10005));
#234259=CARTESIAN_POINT('',(62.1666822880186,19.26999998,-189.64995));
#234260=CARTESIAN_POINT('Origin',(61.6666822880186,19.26999998,-189.64995));
#234261=CARTESIAN_POINT('',(62.1666822880186,19.26999998,-189.64995));
#234262=CARTESIAN_POINT('Origin',(59.1666822880186,19.26999998,-182.64995));
#234263=CARTESIAN_POINT('',(59.1666822880186,19.26999998,-179.64995));
#234264=CARTESIAN_POINT('',(59.1666822880186,18.76999998,-180.14995));
#234265=CARTESIAN_POINT('Origin',(59.1666822880186,19.26999998,-180.14995));
#234266=CARTESIAN_POINT('Origin',(59.1666822880186,18.76999998,-182.64995));
#234267=CARTESIAN_POINT('Origin',(59.1666822880186,19.26999998,-182.64995));
#234268=CARTESIAN_POINT('Origin',(51.746661977277,19.26999998,-180.14995));
#234269=CARTESIAN_POINT('',(52.3218461808875,19.26999998,-179.64995));
#234270=CARTESIAN_POINT('',(52.3218461808875,18.76999998,-180.14995));
#234271=CARTESIAN_POINT('Origin',(52.3218461808875,19.26999998,-180.14995));
#234272=CARTESIAN_POINT('',(52.3218461808875,18.76999998,-180.14995));
#234273=CARTESIAN_POINT('',(59.1666822880186,19.26999998,-179.64995));
#234274=CARTESIAN_POINT('Origin',(52.3218461808875,18.26999998,-180.14995));
#234275=CARTESIAN_POINT('',(51.3315781121459,18.1308268790399,-179.64995));
#234276=CARTESIAN_POINT('',(51.8267121465167,18.20041342952,-180.14995));
#234277=CARTESIAN_POINT('Origin',(51.3315781121459,18.1308268790399,-180.14995));
#234278=CARTESIAN_POINT('Origin',(52.3218461808875,18.26999998,-180.14995));
#234279=CARTESIAN_POINT('Origin',(52.3218461808875,18.26999998,-179.64995));
#234280=CARTESIAN_POINT('Origin',(52.1173462765794,12.5397958730165,-180.14995));
#234281=CARTESIAN_POINT('',(52.0098956044578,13.3043471320808,-179.64995));
#234282=CARTESIAN_POINT('',(52.5050296388285,13.3739336825608,-180.14995));
#234283=CARTESIAN_POINT('Origin',(52.0098956044578,13.3043471320808,-180.14995));
#234284=CARTESIAN_POINT('',(52.6124803109502,12.6093824234965,-180.14995));
#234285=CARTESIAN_POINT('',(61.1310018874833,-51.5956963488069,-179.64995));
#234286=CARTESIAN_POINT('Origin',(57.4563699825364,14.0697991873612,-180.14995));
#234287=CARTESIAN_POINT('',(52.2496341347737,12.2978223783642,-179.64995));
#234288=CARTESIAN_POINT('',(52.7229737572976,12.4589111791821,-180.14995));
#234289=CARTESIAN_POINT('Origin',(52.2496341347737,12.2978223783642,-180.14995));
#234290=CARTESIAN_POINT('Origin',(57.4563699825364,14.0697991873612,-180.14995));
#234291=CARTESIAN_POINT('Origin',(57.4563699825364,14.0697991873612,-179.64995));
#234292=CARTESIAN_POINT('Origin',(53.1963133798215,12.61999998,-180.14995));
#234293=CARTESIAN_POINT('',(53.1963133798215,11.61999998,-179.64995));
#234294=CARTESIAN_POINT('',(53.1963133798215,12.11999998,-180.14995));
#234295=CARTESIAN_POINT('Origin',(53.1963133798215,11.61999998,-180.14995));
#234296=CARTESIAN_POINT('Origin',(53.1963133798215,12.61999998,-180.14995));
#234297=CARTESIAN_POINT('Origin',(53.1963133798215,12.61999998,-179.64995));
#234298=CARTESIAN_POINT('Origin',(52.8475859784398,11.61999998,-180.14995));
#234299=CARTESIAN_POINT('',(59.1666822880186,11.61999998,-179.64995));
#234300=CARTESIAN_POINT('',(59.1666822880186,12.11999998,-180.14995));
#234301=CARTESIAN_POINT('Origin',(59.1666822880186,11.61999998,-180.14995));
#234302=CARTESIAN_POINT('',(59.1666822880186,12.11999998,-180.14995));
#234303=CARTESIAN_POINT('',(53.1963133798215,11.61999998,-179.64995));
#234304=CARTESIAN_POINT('Origin',(59.1666822880186,11.61999998,-182.64995));
#234305=CARTESIAN_POINT('',(62.1666822880186,11.61999998,-182.64995));
#234306=CARTESIAN_POINT('',(61.6666822880186,12.11999998,-182.64995));
#234307=CARTESIAN_POINT('Origin',(61.6666822880186,11.61999998,-182.64995));
#234308=CARTESIAN_POINT('Origin',(59.1666822880186,12.11999998,-182.64995));
#234309=CARTESIAN_POINT('Origin',(59.1666822880186,11.61999998,-182.64995));
#234310=CARTESIAN_POINT('Origin',(61.6666822880186,11.61999998,-189.64995));
#234311=CARTESIAN_POINT('',(61.6666822880186,12.11999998,-189.64995));
#234312=CARTESIAN_POINT('',(62.1666822880186,11.61999998,-189.64995));
#234313=CARTESIAN_POINT('Origin',(61.6666822880186,11.61999998,-189.64995));
#234314=CARTESIAN_POINT('',(61.6666822880186,12.11999998,-236.10005));
#234315=CARTESIAN_POINT('',(62.1666822880186,11.61999998,-189.64995));
#234316=CARTESIAN_POINT('Origin',(61.6666822880186,27.41999998,-189.64995));
#234317=CARTESIAN_POINT('',(62.1666822880186,27.41999998,-182.64995));
#234318=CARTESIAN_POINT('',(61.6666822880186,26.91999998,-182.64995));
#234319=CARTESIAN_POINT('Origin',(61.6666822880186,27.41999998,-182.64995));
#234320=CARTESIAN_POINT('',(61.6666822880186,26.91999998,-189.64995));
#234321=CARTESIAN_POINT('',(61.6666822880186,26.91999998,-236.10005));
#234322=CARTESIAN_POINT('',(62.1666822880186,27.41999998,-189.64995));
#234323=CARTESIAN_POINT('Origin',(61.6666822880186,27.41999998,-189.64995));
#234324=CARTESIAN_POINT('',(62.1666822880186,27.41999998,-189.64995));
#234325=CARTESIAN_POINT('Origin',(59.1666822880186,27.41999998,-182.64995));
#234326=CARTESIAN_POINT('',(59.1666822880186,27.41999998,-179.64995));
#234327=CARTESIAN_POINT('',(59.1666822880186,26.91999998,-180.14995));
#234328=CARTESIAN_POINT('Origin',(59.1666822880186,27.41999998,-180.14995));
#234329=CARTESIAN_POINT('Origin',(59.1666822880186,26.91999998,-182.64995));
#234330=CARTESIAN_POINT('Origin',(59.1666822880186,27.41999998,-182.64995));
#234331=CARTESIAN_POINT('Origin',(50.6012541744525,27.41999998,-180.14995));
#234332=CARTESIAN_POINT('',(51.176438378063,27.41999998,-179.64995));
#234333=CARTESIAN_POINT('',(51.176438378063,26.91999998,-180.14995));
#234334=CARTESIAN_POINT('Origin',(51.176438378063,27.41999998,-180.14995));
#234335=CARTESIAN_POINT('',(51.176438378063,26.91999998,-180.14995));
#234336=CARTESIAN_POINT('',(59.1666822880186,27.41999998,-179.64995));
#234337=CARTESIAN_POINT('Origin',(51.176438378063,26.41999998,-180.14995));
#234338=CARTESIAN_POINT('',(50.1861703093214,26.28082687904,-179.64995));
#234339=CARTESIAN_POINT('',(50.6813043436922,26.35041342952,-180.14995));
#234340=CARTESIAN_POINT('Origin',(50.1861703093214,26.28082687904,-180.14995));
#234341=CARTESIAN_POINT('Origin',(51.176438378063,26.41999998,-180.14995));
#234342=CARTESIAN_POINT('Origin',(51.176438378063,26.41999998,-179.64995));
#234343=CARTESIAN_POINT('Origin',(52.1173462765794,12.5397958730165,-180.14995));
#234344=CARTESIAN_POINT('',(50.9802260253899,20.63082687904,-179.64995));
#234345=CARTESIAN_POINT('',(51.4753600597607,20.70041342952,-180.14995));
#234346=CARTESIAN_POINT('Origin',(50.9802260253899,20.63082687904,-180.14995));
#234347=CARTESIAN_POINT('',(52.6124803109502,12.6093824234965,-180.14995));
#234348=CARTESIAN_POINT('',(61.1310018874833,-51.5956963488069,-179.64995));
#234349=CARTESIAN_POINT('Origin',(51.9704940941315,20.76999998,-180.14995));
#234350=CARTESIAN_POINT('',(51.9704940941315,19.76999998,-179.64995));
#234351=CARTESIAN_POINT('',(51.9704940941315,20.26999998,-180.14995));
#234352=CARTESIAN_POINT('Origin',(51.9704940941315,19.76999998,-180.14995));
#234353=CARTESIAN_POINT('Origin',(51.9704940941315,20.76999998,-180.14995));
#234354=CARTESIAN_POINT('Origin',(51.9704940941315,20.76999998,-179.64995));
#234355=CARTESIAN_POINT('Origin',(51.5358507252234,19.76999998,-180.14995));
#234356=CARTESIAN_POINT('',(59.1666822880186,19.76999998,-179.64995));
#234357=CARTESIAN_POINT('',(59.1666822880186,20.26999998,-180.14995));
#234358=CARTESIAN_POINT('Origin',(59.1666822880186,19.76999998,-180.14995));
#234359=CARTESIAN_POINT('',(59.1666822880186,20.26999998,-180.14995));
#234360=CARTESIAN_POINT('',(51.9704940941315,19.76999998,-179.64995));
#234361=CARTESIAN_POINT('Origin',(59.1666822880186,19.76999998,-182.64995));
#234362=CARTESIAN_POINT('',(62.1666822880186,19.76999998,-182.64995));
#234363=CARTESIAN_POINT('',(61.6666822880186,20.26999998,-182.64995));
#234364=CARTESIAN_POINT('Origin',(61.6666822880186,19.76999998,-182.64995));
#234365=CARTESIAN_POINT('Origin',(59.1666822880186,20.26999998,-182.64995));
#234366=CARTESIAN_POINT('Origin',(59.1666822880186,19.76999998,-182.64995));
#234367=CARTESIAN_POINT('Origin',(61.6666822880186,19.76999998,-189.64995));
#234368=CARTESIAN_POINT('',(61.6666822880186,20.26999998,-189.64995));
#234369=CARTESIAN_POINT('',(62.1666822880186,19.76999998,-189.64995));
#234370=CARTESIAN_POINT('Origin',(61.6666822880186,19.76999998,-189.64995));
#234371=CARTESIAN_POINT('',(61.6666822880186,20.26999998,-236.10005));
#234372=CARTESIAN_POINT('',(62.1666822880186,19.76999998,-189.64995));
#234373=CARTESIAN_POINT('Origin',(59.4002474757908,36.1278445718973,-180.14995));
#234374=CARTESIAN_POINT('',(59.4349689580299,36.1625660541364,-179.64995));
#234375=CARTESIAN_POINT('',(59.7538008663841,35.7742911813041,-180.14995));
#234376=CARTESIAN_POINT('Ctrl Pts',(59.4349689580299,36.1625660541365,-179.64995));
#234377=CARTESIAN_POINT('Ctrl Pts',(59.4751674290521,36.1139360589365,-179.64995));
#234378=CARTESIAN_POINT('Ctrl Pts',(59.517991405701,36.0619958343442,-179.662506459348));
#234379=CARTESIAN_POINT('Ctrl Pts',(59.5966866581669,35.9663093970947,-179.713622693033));
#234380=CARTESIAN_POINT('Ctrl Pts',(59.6325609826829,35.9225664005524,-179.752183794052));
#234381=CARTESIAN_POINT('Ctrl Pts',(59.689032648704,35.8536048925318,-179.841045572058));
#234382=CARTESIAN_POINT('Ctrl Pts',(59.7134506950769,35.8237224381175,-179.89718552734));
#234383=CARTESIAN_POINT('Ctrl Pts',(59.7458338457619,35.7840632466862,-180.020253182031));
#234384=CARTESIAN_POINT('Ctrl Pts',(59.7538008663841,35.7742911813041,-180.0871818826));
#234385=CARTESIAN_POINT('Ctrl Pts',(59.7538008663841,35.7742911813041,-180.14995));
#234386=CARTESIAN_POINT('',(52.8995100714853,29.6271071675918,-179.64995));
#234387=CARTESIAN_POINT('',(59.4002474757908,36.1278445718973,-179.64995));
#234388=CARTESIAN_POINT('',(53.2530634620785,29.2735537769986,-180.14995));
#234389=CARTESIAN_POINT('Origin',(52.8995100714853,29.6271071675918,-180.14995));
#234390=CARTESIAN_POINT('',(53.2530634620785,29.2735537769986,-180.14995));
#234391=CARTESIAN_POINT('Origin',(53.6066168526718,28.9200003864052,-180.14995));
#234392=CARTESIAN_POINT('',(53.6066168526718,27.9200003864053,-179.64995));
#234393=CARTESIAN_POINT('',(53.6066168526718,28.4200003864053,-180.14995));
#234394=CARTESIAN_POINT('Origin',(53.6066168526718,27.9200003864053,-180.14995));
#234395=CARTESIAN_POINT('Origin',(53.6066168526718,28.9200003864052,-180.14995));
#234396=CARTESIAN_POINT('Origin',(53.6066168526718,28.9200003864052,-179.64995));
#234397=CARTESIAN_POINT('Origin',(52.3995100714852,27.9200003864053,-180.14995));
#234398=CARTESIAN_POINT('',(59.1666822880186,27.9200003864053,-179.64995));
#234399=CARTESIAN_POINT('',(59.1666822880186,28.4200003864053,-180.14995));
#234400=CARTESIAN_POINT('Origin',(59.1666822880186,27.9200003864053,-180.14995));
#234401=CARTESIAN_POINT('',(59.1666822880186,28.4200003864053,-180.14995));
#234402=CARTESIAN_POINT('',(53.6066168526718,27.9200003864053,-179.64995));
#234403=CARTESIAN_POINT('Origin',(59.1666822880186,27.9200003864053,-182.64995));
#234404=CARTESIAN_POINT('',(62.1666822880186,27.9200003864053,-182.64995));
#234405=CARTESIAN_POINT('',(61.6666822880186,28.4200003864053,-182.64995));
#234406=CARTESIAN_POINT('Origin',(61.6666822880186,27.9200003864053,-182.64995));
#234407=CARTESIAN_POINT('Origin',(59.1666822880186,28.4200003864053,-182.64995));
#234408=CARTESIAN_POINT('Origin',(59.1666822880186,27.9200003864053,-182.64995));
#234409=CARTESIAN_POINT('Origin',(61.6666822880186,27.9200003864053,-189.64995));
#234410=CARTESIAN_POINT('',(61.6666822880186,28.4200003864053,-189.64995));
#234411=CARTESIAN_POINT('',(62.1666822880186,27.9200003864053,-189.64995));
#234412=CARTESIAN_POINT('Origin',(61.6666822880186,27.9200003864053,-189.64995));
#234413=CARTESIAN_POINT('',(61.6666822880186,28.4200003864053,-189.64995));
#234414=CARTESIAN_POINT('',(62.1666822880186,27.9200003864053,-189.64995));
#234415=CARTESIAN_POINT('Origin',(53.361677340714,-54.9537553161325,-189.64995));
#234416=CARTESIAN_POINT('',(53.361677340714,-54.4537553161325,-189.64995));
#234417=CARTESIAN_POINT('',(53.361677340714,-54.4537553161325,-189.64995));
#234418=CARTESIAN_POINT('',(53.0081239501207,-55.3073087067258,-189.64995));
#234419=CARTESIAN_POINT('',(53.0081239501207,-55.3073087067258,-179.64995));
#234420=CARTESIAN_POINT('Origin',(53.361677340714,-54.9537553161325,-189.64995));
#234421=CARTESIAN_POINT('Origin',(40.7325633042077,-65.3856746638358,-189.64995));
#234422=CARTESIAN_POINT('',(41.086116694801,-65.0321212732425,-189.64995));
#234423=CARTESIAN_POINT('',(41.086116694801,-65.0321212732425,-189.64995));
#234424=CARTESIAN_POINT('',(40.7325633042077,-64.8856746638358,-189.64995));
#234425=CARTESIAN_POINT('',(40.7325633042077,-64.8856746638358,-179.64995));
#234426=CARTESIAN_POINT('Origin',(40.7325633042077,-65.3856746638358,-189.64995));
#234427=CARTESIAN_POINT('Origin',(53.6066168526718,28.9200003864052,-189.64995));
#234428=CARTESIAN_POINT('',(53.2530634620785,29.2735537769986,-189.64995));
#234429=CARTESIAN_POINT('',(53.2530634620785,29.2735537769986,-189.64995));
#234430=CARTESIAN_POINT('',(53.6066168526718,28.4200003864053,-189.64995));
#234431=CARTESIAN_POINT('',(53.6066168526718,28.4200003864053,-179.64995));
#234432=CARTESIAN_POINT('Origin',(53.6066168526718,28.9200003864052,-189.64995));
#234433=CARTESIAN_POINT('Origin',(40.7325633042078,40.2945320099637,-189.64995));
#234434=CARTESIAN_POINT('',(40.7325633042078,39.7945320099637,-189.64995));
#234435=CARTESIAN_POINT('',(40.7325633042078,39.7945320099637,-189.64995));
#234436=CARTESIAN_POINT('',(41.086116694801,39.9409786193705,-189.64995));
#234437=CARTESIAN_POINT('',(41.086116694801,39.9409786193705,-179.64995));
#234438=CARTESIAN_POINT('Origin',(40.7325633042078,40.2945320099637,-189.64995));
#234439=CARTESIAN_POINT('Origin',(40.4396700853943,40.2945320099637,-189.64995));
#234440=CARTESIAN_POINT('',(39.9396700853943,40.2945320099637,-189.64995));
#234441=CARTESIAN_POINT('',(39.9396700853943,40.2945320099637,-189.64995));
#234442=CARTESIAN_POINT('',(40.4396700853943,39.7945320099637,-189.64995));
#234443=CARTESIAN_POINT('',(40.4396700853943,39.7945320099637,-179.64995));
#234444=CARTESIAN_POINT('Origin',(40.4396700853943,40.2945320099637,-189.64995));
#234445=CARTESIAN_POINT('Origin',(51.176438378063,26.41999998,-171.64995));
#234446=CARTESIAN_POINT('',(51.176438378063,26.91999998,-189.64995));
#234447=CARTESIAN_POINT('',(51.176438378063,26.91999998,-236.10005));
#234448=CARTESIAN_POINT('',(50.6813043436922,26.35041342952,-189.64995));
#234449=CARTESIAN_POINT('',(50.6813043436922,26.35041342952,-171.64995));
#234450=CARTESIAN_POINT('Origin',(51.176438378063,26.41999998,-189.64995));
#234451=CARTESIAN_POINT('Origin',(52.3218461808875,18.26999998,-171.64995));
#234452=CARTESIAN_POINT('',(52.3218461808875,18.76999998,-189.64995));
#234453=CARTESIAN_POINT('',(52.3218461808875,18.76999998,-236.10005));
#234454=CARTESIAN_POINT('',(51.8267121465167,18.20041342952,-189.64995));
#234455=CARTESIAN_POINT('',(51.8267121465167,18.20041342952,-171.64995));
#234456=CARTESIAN_POINT('Origin',(52.3218461808875,18.26999998,-189.64995));
#234457=CARTESIAN_POINT('Origin',(54.2951871140408,10.11999998,-179.64995));
#234458=CARTESIAN_POINT('',(54.2951871140408,10.61999998,-189.64995));
#234459=CARTESIAN_POINT('',(54.2951871140408,10.61999998,-189.64995));
#234460=CARTESIAN_POINT('',(53.8350584096845,9.92434320033877,-189.64995));
#234461=CARTESIAN_POINT('',(53.8350584096845,9.92434320033877,-179.64995));
#234462=CARTESIAN_POINT('Origin',(54.2951871140408,10.11999998,-189.64995));
#234463=CARTESIAN_POINT('Origin',(57.077763566464,1.96999998000002,-179.64995));
#234464=CARTESIAN_POINT('',(57.077763566464,2.46999998000002,-189.64995));
#234465=CARTESIAN_POINT('',(57.077763566464,2.46999998000002,-189.64995));
#234466=CARTESIAN_POINT('',(56.5940537057312,1.84341099694893,-189.64995));
#234467=CARTESIAN_POINT('',(56.5940537057312,1.84341099694893,-179.64995));
#234468=CARTESIAN_POINT('Origin',(57.077763566464,1.96999998000002,-189.64995));
#234469=CARTESIAN_POINT('Origin',(58.6082745331205,-6.18000001999998,-179.64995));
#234470=CARTESIAN_POINT('',(58.6082745331205,-5.68000001999998,-189.64995));
#234471=CARTESIAN_POINT('',(58.6082745331205,-5.68000001999998,-189.64995));
#234472=CARTESIAN_POINT('',(58.1115942404669,-6.2375212064409,-189.64995));
#234473=CARTESIAN_POINT('',(58.1115942404669,-6.2375212064409,-179.64995));
#234474=CARTESIAN_POINT('Origin',(58.6082745331205,-6.18000001999998,-189.64995));
#234475=CARTESIAN_POINT('Origin',(58.9842656455946,-14.33000002,-179.64995));
#234476=CARTESIAN_POINT('',(58.9842656455946,-13.83000002,-189.64995));
#234477=CARTESIAN_POINT('',(58.9842656455946,-13.83000002,-189.64995));
#234478=CARTESIAN_POINT('',(58.4843989875811,-14.3184534098307,-189.64995));
#234479=CARTESIAN_POINT('',(58.4843989875811,-14.3184534098307,-179.64995));
#234480=CARTESIAN_POINT('Origin',(58.9842656455946,-14.33000002,-189.64995));
#234481=CARTESIAN_POINT('Origin',(58.9890336736409,-11.83000002,-179.64995));
#234482=CARTESIAN_POINT('',(58.48912660861,-11.8396398505087,-189.64995));
#234483=CARTESIAN_POINT('',(58.48912660861,-11.8396398505087,-179.64995));
#234484=CARTESIAN_POINT('',(58.9890336736409,-12.33000002,-189.64995));
#234485=CARTESIAN_POINT('',(58.9890336736409,-12.33000002,-179.64995));
#234486=CARTESIAN_POINT('Origin',(58.9890336736409,-11.83000002,-189.64995));
#234487=CARTESIAN_POINT('Origin',(58.2644174754153,-3.68000001999999,-179.64995));
#234488=CARTESIAN_POINT('',(57.7706512256236,-3.75870764711887,-189.64995));
#234489=CARTESIAN_POINT('',(57.7706512256236,-3.75870764711887,-179.64995));
#234490=CARTESIAN_POINT('',(58.2644174754153,-4.18000001999998,-189.64995));
#234491=CARTESIAN_POINT('',(58.2644174754153,-4.18000001999998,-179.64995));
#234492=CARTESIAN_POINT('Origin',(58.2644174754153,-3.68000001999999,-189.64995));
#234493=CARTESIAN_POINT('Origin',(56.3642936064049,4.46999998000001,-179.64995));
#234494=CARTESIAN_POINT('',(55.8866301012659,4.32222455627096,-189.64995));
#234495=CARTESIAN_POINT('',(55.8866301012659,4.32222455627096,-179.64995));
#234496=CARTESIAN_POINT('',(56.3642936064049,3.96999998000001,-189.64995));
#234497=CARTESIAN_POINT('',(56.3642936064049,3.96999998000001,-179.64995));
#234498=CARTESIAN_POINT('Origin',(56.3642936064049,4.46999998000001,-189.64995));
#234499=CARTESIAN_POINT('Origin',(53.1963133798215,12.61999998,-179.64995));
#234500=CARTESIAN_POINT('',(52.7229737572976,12.4589111791821,-189.64995));
#234501=CARTESIAN_POINT('',(52.7229737572976,12.4589111791821,-179.64995));
#234502=CARTESIAN_POINT('',(53.1963133798215,12.11999998,-189.64995));
#234503=CARTESIAN_POINT('',(53.1963133798215,12.11999998,-179.64995));
#234504=CARTESIAN_POINT('Origin',(53.1963133798215,12.61999998,-189.64995));
#234505=CARTESIAN_POINT('Origin',(51.9704940941315,20.76999998,-236.10005));
#234506=CARTESIAN_POINT('',(51.4753600597607,20.70041342952,-189.64995));
#234507=CARTESIAN_POINT('',(51.4753600597607,20.70041342952,-171.64995));
#234508=CARTESIAN_POINT('',(51.9704940941315,20.26999998,-189.64995));
#234509=CARTESIAN_POINT('',(51.9704940941315,20.26999998,-236.10005));
#234510=CARTESIAN_POINT('Origin',(51.9704940941315,20.76999998,-189.64995));
#234511=CARTESIAN_POINT('Origin',(58.5817791104913,-19.98000002,-179.64995));
#234512=CARTESIAN_POINT('',(58.0853233553177,-19.9205720538985,-189.64995));
#234513=CARTESIAN_POINT('',(58.0853233553177,-19.9205720538985,-179.64995));
#234514=CARTESIAN_POINT('',(58.5817791104913,-20.48000002,-189.64995));
#234515=CARTESIAN_POINT('',(58.5817791104913,-20.48000002,-179.64995));
#234516=CARTESIAN_POINT('Origin',(58.5817791104913,-19.98000002,-189.64995));
#234517=CARTESIAN_POINT('Origin',(58.2281061322669,-22.48000002,-179.64995));
#234518=CARTESIAN_POINT('',(58.2281061322669,-21.98000002,-189.64995));
#234519=CARTESIAN_POINT('',(58.2281061322669,-21.98000002,-189.64995));
#234520=CARTESIAN_POINT('',(57.7346476057223,-22.3993856132206,-189.64995));
#234521=CARTESIAN_POINT('',(57.7346476057223,-22.3993856132206,-179.64995));
#234522=CARTESIAN_POINT('Origin',(58.2281061322669,-22.48000002,-189.64995));
#234523=CARTESIAN_POINT('Origin',(57.0184057454332,-28.13000002,-179.64995));
#234524=CARTESIAN_POINT('',(56.5351989170821,-28.0015042572884,-189.64995));
#234525=CARTESIAN_POINT('',(56.5351989170821,-28.0015042572884,-179.64995));
#234526=CARTESIAN_POINT('',(57.0184057454332,-28.63000002,-189.64995));
#234527=CARTESIAN_POINT('',(57.0184057454332,-28.63000002,-179.64995));
#234528=CARTESIAN_POINT('Origin',(57.0184057454332,-28.13000002,-189.64995));
#234529=CARTESIAN_POINT('Origin',(56.294192362543,-30.63000002,-179.64995));
#234530=CARTESIAN_POINT('',(56.294192362543,-30.13000002,-189.64995));
#234531=CARTESIAN_POINT('',(56.294192362543,-30.13000002,-189.64995));
#234532=CARTESIAN_POINT('',(55.8171229357418,-30.4803178166104,-189.64995));
#234533=CARTESIAN_POINT('',(55.8171229357418,-30.4803178166104,-179.64995));
#234534=CARTESIAN_POINT('Origin',(56.294192362543,-30.63000002,-189.64995));
#234535=CARTESIAN_POINT('Origin',(53.1262583325313,-38.78000002,-179.64995));
#234536=CARTESIAN_POINT('',(53.1262583325313,-38.28000002,-189.64995));
#234537=CARTESIAN_POINT('',(53.1262583325313,-38.28000002,-189.64995));
#234538=CARTESIAN_POINT('',(52.6451348158641,-38.6439112191758,-189.64995));
#234539=CARTESIAN_POINT('',(52.6451348158641,-38.6439112191758,-179.64995));
#234540=CARTESIAN_POINT('Origin',(53.1262583325313,-38.78000002,-189.64995));
#234541=CARTESIAN_POINT('Origin',(54.1989607257493,-36.28000002,-179.64995));
#234542=CARTESIAN_POINT('',(53.7396474992599,-36.0824364606782,-189.64995));
#234543=CARTESIAN_POINT('',(53.7396474992599,-36.0824364606782,-179.64995));
#234544=CARTESIAN_POINT('',(54.1989607257493,-36.78000002,-189.64995));
#234545=CARTESIAN_POINT('',(54.1989607257493,-36.78000002,-179.64995));
#234546=CARTESIAN_POINT('Origin',(54.1989607257493,-36.28000002,-189.64995));
#234547=CARTESIAN_POINT('Origin',(52.2902244930873,-44.43000002,-236.10005));
#234548=CARTESIAN_POINT('',(51.7950904587165,-44.36041346952,-189.64995));
#234549=CARTESIAN_POINT('',(51.7950904587165,-44.36041346952,-171.64995));
#234550=CARTESIAN_POINT('',(52.2902244930873,-44.93000002,-189.64995));
#234551=CARTESIAN_POINT('',(52.2902244930873,-44.93000002,-236.10005));
#234552=CARTESIAN_POINT('Origin',(52.2902244930873,-44.43000002,-189.64995));
#234553=CARTESIAN_POINT('Origin',(51.9388724063314,-46.93000002,-171.64995));
#234554=CARTESIAN_POINT('',(51.9388724063314,-46.43000002,-189.64995));
#234555=CARTESIAN_POINT('',(51.9388724063314,-46.43000002,-236.10005));
#234556=CARTESIAN_POINT('',(51.4437383719606,-46.86041346952,-189.64995));
#234557=CARTESIAN_POINT('',(51.4437383719606,-46.8604134695199,-171.64995));
#234558=CARTESIAN_POINT('Origin',(51.9388724063314,-46.93000002,-189.64995));
#234559=CARTESIAN_POINT('Origin',(51.1448166902628,-52.58000002,-236.10005));
#234560=CARTESIAN_POINT('',(50.6496826558921,-52.51041346952,-189.64995));
#234561=CARTESIAN_POINT('',(50.6496826558921,-52.51041346952,-171.64995));
#234562=CARTESIAN_POINT('',(51.1448166902628,-53.08000002,-189.64995));
#234563=CARTESIAN_POINT('',(51.1448166902628,-53.08000002,-236.10005));
#234564=CARTESIAN_POINT('Origin',(51.1448166902628,-52.58000002,-189.64995));
#234565=CARTESIAN_POINT('Origin',(40.4396700853942,-65.3856746638358,-189.64995));
#234566=CARTESIAN_POINT('',(40.4396700853942,-64.8856746638358,-189.64995));
#234567=CARTESIAN_POINT('',(40.4396700853942,-64.8856746638358,-189.64995));
#234568=CARTESIAN_POINT('',(39.9396700853942,-65.3856746638358,-189.64995));
#234569=CARTESIAN_POINT('',(39.9396700853942,-65.3856746638358,-179.64995));
#234570=CARTESIAN_POINT('Origin',(40.4396700853942,-65.3856746638358,-189.64995));
#234571=CARTESIAN_POINT('Origin',(50.5696324866523,-53.08000002,-179.64995));
#234572=CARTESIAN_POINT('Origin',(0.,-12.9675000200281,-179.64995));
#234573=CARTESIAN_POINT('',(8.67557705647162E-17,53.4196191598902,-179.64995));
#234574=CARTESIAN_POINT('Origin',(0.,-178.58000002,-179.64995));
#234575=CARTESIAN_POINT('',(-1.57577820804084E-14,-75.2524362554308,-179.64995));
#234576=CARTESIAN_POINT('',(8.67557705647162E-17,53.4196191598902,-179.64995));
#234577=CARTESIAN_POINT('',(-1.57577820804084E-14,-75.2524362554308,-179.64995));
#234578=CARTESIAN_POINT('Origin',(0.,-12.9675000200281,-179.64995));
#234579=CARTESIAN_POINT('',(59.1666822880186,28.4200003864053,-179.64995));
#234580=CARTESIAN_POINT('',(59.1666822880186,28.4200003864053,-179.64995));
#234581=CARTESIAN_POINT('',(59.1666822880186,28.4200003864053,-179.64995));
#234582=CARTESIAN_POINT('',(59.1666822880186,28.4200003864053,-179.64995));
#234583=CARTESIAN_POINT('',(59.1666822880186,28.4200003864053,-179.64995));
#234584=CARTESIAN_POINT('',(59.1666822880186,28.4200003864053,-179.64995));
#234585=CARTESIAN_POINT('',(59.1666822880186,28.4200003864053,-179.64995));
#234586=CARTESIAN_POINT('',(59.1666822880186,28.4200003864053,-179.64995));
#234587=CARTESIAN_POINT('',(59.1666822880186,28.4200003864053,-179.64995));
#234588=CARTESIAN_POINT('',(59.1666822880186,28.4200003864053,-179.64995));
#234589=CARTESIAN_POINT('',(59.1666822880186,28.4200003864053,-179.64995));
#234590=CARTESIAN_POINT('Origin',(62.1666822880186,-54.4537553161325,-189.64995));
#234591=CARTESIAN_POINT('',(62.1666822880186,-54.4537553161325,-189.64995));
#234592=CARTESIAN_POINT('Origin',(0.,-178.58000002,-189.64995));
#234593=CARTESIAN_POINT('',(39.9396700853943,49.9558747416749,-189.64995));
#234594=CARTESIAN_POINT('',(39.9396700853943,49.9558747416749,-189.64995));
#234595=CARTESIAN_POINT('',(8.67557705647162E-17,53.4196191598902,-189.64995));
#234596=CARTESIAN_POINT('Origin',(0.,-178.58000002,-189.64995));
#234597=CARTESIAN_POINT('',(8.67557705647162E-17,53.4196191598902,-189.64995));
#234598=CARTESIAN_POINT('Origin',(39.9396700853943,49.9558747416749,-189.64995));
#234599=CARTESIAN_POINT('',(39.9396700853943,49.9558747416749,-189.64995));
#234600=CARTESIAN_POINT('Origin',(39.9396700853942,-64.8856746638358,-189.64995));
#234601=CARTESIAN_POINT('',(39.9396700853942,-64.8856746638358,-189.64995));
#234602=CARTESIAN_POINT('Origin',(39.9396700853942,-64.8856746638358,-189.64995));
#234603=CARTESIAN_POINT('',(39.9396700853942,-75.2524362554308,-189.64995));
#234604=CARTESIAN_POINT('',(39.9396700853942,-75.2524362554308,-189.64995));
#234605=CARTESIAN_POINT('',(39.9396700853942,-64.8856746638358,-189.64995));
#234606=CARTESIAN_POINT('Origin',(50.5696324866523,-53.08000002,-236.10005));
#234607=CARTESIAN_POINT('',(0.,-53.08000002,-189.64995));
#234608=CARTESIAN_POINT('Origin',(51.5042290374232,-46.43000002,-236.10005));
#234609=CARTESIAN_POINT('',(0.,-46.43000002,-189.64995));
#234610=CARTESIAN_POINT('Origin',(57.8362329664502,-4.18000001999998,-236.10005));
#234611=CARTESIAN_POINT('',(0.,-4.18000001999998,-189.64995));
#234612=CARTESIAN_POINT('Origin',(56.4263554888062,2.46999998000002,-236.10005));
#234613=CARTESIAN_POINT('',(0.,2.46999998000002,-189.64995));
#234614=CARTESIAN_POINT('Origin',(55.9943844840627,3.96999998000001,-236.10005));
#234615=CARTESIAN_POINT('',(2.25916865206423E-15,3.96999998000003,-189.64995));
#234616=CARTESIAN_POINT('Origin',(53.533913024817,10.61999998,-236.10005));
#234617=CARTESIAN_POINT('',(2.64564592552133E-15,10.61999998,-189.64995));
#234618=CARTESIAN_POINT('Origin',(51.746661977277,18.76999998,-236.10005));
#234619=CARTESIAN_POINT('',(0.,18.76999998,-189.64995));
#234620=CARTESIAN_POINT('Origin',(51.7150402894768,-44.93000002,-236.10005));
#234621=CARTESIAN_POINT('',(0.,-44.93000002,-189.64995));
#234622=CARTESIAN_POINT('Origin',(58.4965263391765,-12.33000002,-236.10005));
#234623=CARTESIAN_POINT('',(0.,-12.33000002,-189.64995));
#234624=CARTESIAN_POINT('Origin',(58.0443136211429,-5.68000001999998,-236.10005));
#234625=CARTESIAN_POINT('',(-1.15390281302924E-15,-5.68000001999999,-189.64995));
#234626=CARTESIAN_POINT('Origin',(62.1666822880186,28.4200003864053,-189.64995));
#234627=CARTESIAN_POINT('',(62.1666822880186,28.4200003864053,-189.64995));
#234628=CARTESIAN_POINT('',(62.1666822880186,-54.4537553161326,-182.64995));
#234629=CARTESIAN_POINT('Origin',(59.1666822880186,28.4200003864053,-182.64995));
#234630=CARTESIAN_POINT('Origin',(0.,-12.9675000200281,-179.64995));
#234631=CARTESIAN_POINT('Origin',(0.,-12.9675000200281,-189.64995));
#234632=CARTESIAN_POINT('Origin',(58.0156215492899,-20.48000002,-236.10005));
#234633=CARTESIAN_POINT('',(0.,-20.48000002,-189.64995));
#234634=CARTESIAN_POINT('Origin',(58.4936414813615,-13.83000002,-236.10005));
#234635=CARTESIAN_POINT('',(0.,-13.83000002,-189.64995));
#234636=CARTESIAN_POINT('Origin',(62.1666822880186,28.4200003864053,-189.64995));
#234637=CARTESIAN_POINT('',(62.1666822880186,28.4200003864053,-189.64995));
#234638=CARTESIAN_POINT('',(62.1666822880186,-54.4537553161326,-182.64995));
#234639=CARTESIAN_POINT('Origin',(59.1666822880186,28.4200003864053,-182.64995));
#234640=CARTESIAN_POINT('Origin',(0.,-12.9675000200281,-179.64995));
#234641=CARTESIAN_POINT('Origin',(0.,-12.9675000200281,-189.64995));
#234642=CARTESIAN_POINT('Origin',(56.3643157835779,-28.63000002,-236.10005));
#234643=CARTESIAN_POINT('',(4.30053584389595E-15,-28.63000002,-189.64995));
#234644=CARTESIAN_POINT('Origin',(57.8015989722647,-21.98000002,-236.10005));
#234645=CARTESIAN_POINT('',(0.,-21.98000002,-189.64995));
#234646=CARTESIAN_POINT('Origin',(62.1666822880186,28.4200003864053,-189.64995));
#234647=CARTESIAN_POINT('',(62.1666822880186,28.4200003864053,-189.64995));
#234648=CARTESIAN_POINT('',(62.1666822880186,-54.4537553161326,-182.64995));
#234649=CARTESIAN_POINT('Origin',(59.1666822880186,28.4200003864053,-182.64995));
#234650=CARTESIAN_POINT('Origin',(0.,-12.9675000200281,-179.64995));
#234651=CARTESIAN_POINT('Origin',(0.,-12.9675000200281,-189.64995));
#234652=CARTESIAN_POINT('Origin',(53.4342104250764,-36.78000002,-236.10005));
#234653=CARTESIAN_POINT('',(0.,-36.78000002,-189.64995));
#234654=CARTESIAN_POINT('Origin',(55.9258311851596,-30.13000002,-236.10005));
#234655=CARTESIAN_POINT('',(4.55435325611026E-15,-30.13000002,-189.64995));
#234656=CARTESIAN_POINT('Origin',(62.1666822880186,28.4200003864053,-189.64995));
#234657=CARTESIAN_POINT('',(62.1666822880186,28.4200003864053,-189.64995));
#234658=CARTESIAN_POINT('',(62.1666822880186,-54.4537553161326,-182.64995));
#234659=CARTESIAN_POINT('Origin',(59.1666822880186,28.4200003864053,-182.64995));
#234660=CARTESIAN_POINT('Origin',(0.,-12.9675000200281,-179.64995));
#234661=CARTESIAN_POINT('Origin',(0.,-12.9675000200281,-189.64995));
#234662=CARTESIAN_POINT('Origin',(51.5358507252234,20.26999998,-236.10005));
#234663=CARTESIAN_POINT('',(-6.60299801904499E-15,20.26999998,-189.64995));
#234664=CARTESIAN_POINT('Origin',(50.6012541744525,26.91999998,-236.10005));
#234665=CARTESIAN_POINT('',(0.,26.91999998,-189.64995));
#234666=CARTESIAN_POINT('Origin',(62.1666822880186,28.4200003864053,-189.64995));
#234667=CARTESIAN_POINT('',(62.1666822880186,28.4200003864053,-189.64995));
#234668=CARTESIAN_POINT('',(62.1666822880186,-54.4537553161326,-182.64995));
#234669=CARTESIAN_POINT('Origin',(59.1666822880186,28.4200003864053,-182.64995));
#234670=CARTESIAN_POINT('Origin',(52.6124803109502,12.6093824234965,-171.64995));
#234671=CARTESIAN_POINT('',(55.1183933044755,-5.22111501756238,-189.64995));
#234672=CARTESIAN_POINT('Origin',(57.4563699825363,-40.0047992274175,-179.64995));
#234673=CARTESIAN_POINT('',(52.5050296388285,-39.3089337226172,-189.64995));
#234674=CARTESIAN_POINT('',(52.5050296388285,-39.3089337226171,-171.64995));
#234675=CARTESIAN_POINT('Origin',(57.4563699825363,-40.0047992274175,-189.64995));
#234676=CARTESIAN_POINT('Origin',(52.6124803109501,-38.5443824635529,-171.64995));
#234677=CARTESIAN_POINT('',(55.1183933044754,-20.7138850224938,-189.64995));
#234678=CARTESIAN_POINT('Origin',(57.4563699825364,14.0697991873612,-179.64995));
#234679=CARTESIAN_POINT('',(52.5050296388285,13.3739336825608,-189.64995));
#234680=CARTESIAN_POINT('',(52.5050296388285,13.3739336825608,-171.64995));
#234681=CARTESIAN_POINT('Origin',(57.4563699825364,14.0697991873612,-189.64995));
#234682=CARTESIAN_POINT('Origin',(52.8475859784398,12.11999998,-236.10005));
#234683=CARTESIAN_POINT('',(0.,12.11999998,-189.64995));
#234684=CARTESIAN_POINT('Origin',(0.,-12.9675000200281,-189.64995));
#234685=CARTESIAN_POINT('',(52.3995100714852,28.4200003864053,-189.64995));
#234686=CARTESIAN_POINT('',(62.1666822880186,28.4200003864053,-189.64995));
#234687=CARTESIAN_POINT('',(55.1183933044755,-5.22111501756237,-189.64995));
#234688=CARTESIAN_POINT('',(62.1666822880186,28.4200003864053,-189.64995));
#234689=CARTESIAN_POINT('Origin',(0.,-12.9675000200281,-189.64995));
#234690=CARTESIAN_POINT('',(62.1666822880186,28.4200003864053,-189.64995));
#234691=CARTESIAN_POINT('Origin',(0.,-12.9675000200281,-189.64995));
#234692=CARTESIAN_POINT('',(62.1666822880186,28.4200003864053,-189.64995));
#234693=CARTESIAN_POINT('',(0.,-38.28000002,-189.64995));
#234694=CARTESIAN_POINT('',(62.1666822880186,28.4200003864053,-189.64995));
#234695=CARTESIAN_POINT('',(55.1183933044754,-20.7138850224938,-189.64995));
#234696=CARTESIAN_POINT('',(62.1666822880186,28.4200003864053,-189.64995));
#234697=CARTESIAN_POINT('',(59.5991207857295,-61.8983055423346,-189.64995));
#234698=CARTESIAN_POINT('',(59.5991207857295,-61.8983055423346,-189.64995));
#234699=CARTESIAN_POINT('',(48.7602414802939,-72.7062460587355,-189.64995));
#234700=CARTESIAN_POINT('Origin',(0.,-12.9675000200281,-189.64995));
#234701=CARTESIAN_POINT('',(48.7602414802939,-72.7062460587355,-189.64995));
#234702=CARTESIAN_POINT('',(-1.57577820804084E-14,-75.2524362554308,-189.64995));
#234703=CARTESIAN_POINT('',(-1.57577820804084E-14,-75.2524362554308,-189.64995));
#234704=CARTESIAN_POINT('',(8.67557705647162E-17,53.4196191598902,-189.64995));
#234705=CARTESIAN_POINT('',(39.9396700853943,39.7945320099637,-189.64995));
#234706=CARTESIAN_POINT('',(48.2939608802931,47.1488228048625,-189.64995));
#234707=CARTESIAN_POINT('',(48.2939608802931,47.1488228048625,-189.64995));
#234708=CARTESIAN_POINT('',(59.7538008663841,35.7742911813041,-189.64995));
#234709=CARTESIAN_POINT('Origin',(0.,-12.9675000200281,-189.64995));
#234710=CARTESIAN_POINT('',(59.7538008663841,35.7742911813041,-189.64995));
#234711=CARTESIAN_POINT('Origin',(52.6124803109502,12.6093824234965,-171.64995));
#234712=CARTESIAN_POINT('Origin',(52.7401871797155,-38.28000002,-236.10005));
#234713=CARTESIAN_POINT('Origin',(59.1666822880186,28.4200003864053,-182.64995));
#234714=CARTESIAN_POINT('',(62.1666822880186,-54.4537553161326,-182.64995));
#234715=CARTESIAN_POINT('Origin',(62.1666822880186,28.4200003864053,-189.64995));
#234716=CARTESIAN_POINT('Origin',(59.1666822880186,28.4200003864053,-182.64995));
#234717=CARTESIAN_POINT('',(62.1666822880186,-54.4537553161326,-182.64995));
#234718=CARTESIAN_POINT('Origin',(62.1666822880186,28.4200003864053,-189.64995));
#234719=CARTESIAN_POINT('Origin',(59.1666822880186,28.4200003864053,-182.64995));
#234720=CARTESIAN_POINT('',(62.1666822880186,-54.4537553161326,-182.64995));
#234721=CARTESIAN_POINT('Origin',(62.1666822880186,28.4200003864053,-189.64995));
#234722=CARTESIAN_POINT('Origin',(59.1666822880186,28.4200003864053,-182.64995));
#234723=CARTESIAN_POINT('',(62.1666822880186,-54.4537553161326,-182.64995));
#234724=CARTESIAN_POINT('Origin',(62.1666822880186,28.4200003864053,-189.64995));
#234725=CARTESIAN_POINT('Origin',(0.,-12.9675000200281,-179.64995));
#234726=CARTESIAN_POINT('Origin',(59.1666822880186,28.4200003864053,-182.64995));
#234727=CARTESIAN_POINT('',(62.1666822880186,-54.4537553161326,-182.64995));
#234728=CARTESIAN_POINT('Origin',(62.1666822880186,28.4200003864053,-189.64995));
#234729=CARTESIAN_POINT('Origin',(0.,-12.9675000200281,-179.64995));
#234730=CARTESIAN_POINT('Origin',(52.6124803109501,-38.5443824635529,-171.64995));
#234731=CARTESIAN_POINT('Origin',(59.1666822880186,28.4200003864053,-182.64995));
#234732=CARTESIAN_POINT('',(62.1666822880186,-54.4537553161326,-182.64995));
#234733=CARTESIAN_POINT('Origin',(62.1666822880186,28.4200003864053,-189.64995));
#234734=CARTESIAN_POINT('Origin',(48.7602414802939,-72.7062460587355,-189.64995));
#234735=CARTESIAN_POINT('',(48.7602414802939,-72.7062460587355,-189.64995));
#234736=CARTESIAN_POINT('Origin',(-1.57577820804084E-14,-75.2524362554308,
-189.64995));
#234737=CARTESIAN_POINT('',(-1.57577820804084E-14,-75.2524362554308,-189.64995));
#234738=CARTESIAN_POINT('Origin',(0.,-120.,224.35005));
#234739=CARTESIAN_POINT('Origin',(39.9396700853943,39.7945320099637,-189.64995));
#234740=CARTESIAN_POINT('Origin',(48.2939608802931,47.1488228048625,-189.64995));
#234741=CARTESIAN_POINT('',(48.2939608802931,47.1488228048625,-189.64995));
#234742=CARTESIAN_POINT('Origin',(0.,-12.9675000200281,-189.64995));
#234743=CARTESIAN_POINT('',(59.7538008663841,35.7742911813041,-189.64995));
#234744=CARTESIAN_POINT('Origin',(59.7538008663841,35.7742911813041,-189.64995));
#234745=CARTESIAN_POINT('Origin',(52.3995100714852,28.4200003864053,-189.64995));
#234746=CARTESIAN_POINT('Origin',(59.5991207857295,-61.8983055423346,-189.64995));
#234747=CARTESIAN_POINT('',(59.5991207857295,-61.8983055423346,-189.64995));
#234748=CARTESIAN_POINT('Origin',(0.,-12.9675000200281,-189.64995));
#234749=CARTESIAN_POINT('Origin',(12.9675000200281,-12.967500020028,-32.54995));
#234750=CARTESIAN_POINT('',(62.5573729911059,-10.4675000200275,-32.54995));
#234751=CARTESIAN_POINT('',(66.8875000100281,-7.96750002002744,-32.54995));
#234752=CARTESIAN_POINT('Origin',(66.8875000100282,-12.9675000200274,-32.54995));
#234753=CARTESIAN_POINT('',(71.2176270289503,-10.4675000200274,-32.54995));
#234754=CARTESIAN_POINT('Origin',(66.8875000100282,-12.9675000200274,-32.54995));
#234755=CARTESIAN_POINT('',(71.2176270289504,-15.4675000200274,-32.54995));
#234756=CARTESIAN_POINT('Origin',(66.8875000100282,-12.9675000200274,-32.54995));
#234757=CARTESIAN_POINT('',(66.8875000100282,-17.9675000200275,-32.54995));
#234758=CARTESIAN_POINT('Origin',(66.8875000100282,-12.9675000200274,-32.54995));
#234759=CARTESIAN_POINT('',(62.557372991106,-15.4675000200275,-32.54995));
#234760=CARTESIAN_POINT('Origin',(66.8875000100282,-12.9675000200274,-32.54995));
#234761=CARTESIAN_POINT('Origin',(66.8875000100282,-12.9675000200274,-32.54995));
#234762=CARTESIAN_POINT('Origin',(66.8875000100282,-12.9675000200274,-32.54995));
#234763=CARTESIAN_POINT('',(69.7742513559762,-7.96750002002741,-31.7764473081038));
#234764=CARTESIAN_POINT('Ctrl Pts',(69.7742513559762,-7.96750002002744,
-31.7764473081038));
#234765=CARTESIAN_POINT('Ctrl Pts',(70.5477540478725,-9.30724598218304,
-32.5499500000001));
#234766=CARTESIAN_POINT('Ctrl Pts',(71.2176270289503,-10.4675000200274,
-32.5499500000001));
#234767=CARTESIAN_POINT('Ctrl Pts',(66.8875000100281,-7.96750002002744,
-32.54995));
#234768=CARTESIAN_POINT('Ctrl Pts',(68.2272459721837,-7.96750002002743,
-32.54995));
#234769=CARTESIAN_POINT('Ctrl Pts',(69.7742513559762,-7.96750002002741,
-31.7764473081038));
#234770=CARTESIAN_POINT('Origin',(66.8875000100282,-12.9675000200274,-32.54995));
#234771=CARTESIAN_POINT('',(72.6610027019244,-12.9675000200274,-31.7764473081038));
#234772=CARTESIAN_POINT('Ctrl Pts',(71.2176270289503,-10.4675000200274,
-32.5499500000001));
#234773=CARTESIAN_POINT('Ctrl Pts',(71.8875000100281,-11.6277540578718,
-32.5499500000001));
#234774=CARTESIAN_POINT('Ctrl Pts',(72.6610027019244,-12.9675000200274,
-31.7764473081038));
#234775=CARTESIAN_POINT('Ctrl Pts',(72.6610027019244,-12.9675000200274,
-31.7764473081038));
#234776=CARTESIAN_POINT('Ctrl Pts',(71.8875000100282,-14.307245982183,-32.5499500000001));
#234777=CARTESIAN_POINT('Ctrl Pts',(71.2176270289504,-15.4675000200274,
-32.5499500000001));
#234778=CARTESIAN_POINT('Origin',(66.8875000100282,-12.9675000200274,-32.54995));
#234779=CARTESIAN_POINT('',(69.7742513559763,-17.9675000200274,-31.7764473081038));
#234780=CARTESIAN_POINT('Ctrl Pts',(71.2176270289504,-15.4675000200274,
-32.5499500000001));
#234781=CARTESIAN_POINT('Ctrl Pts',(70.5477540478726,-16.6277540578718,
-32.5499500000001));
#234782=CARTESIAN_POINT('Ctrl Pts',(69.7742513559763,-17.9675000200274,
-31.7764473081038));
#234783=CARTESIAN_POINT('Ctrl Pts',(69.7742513559763,-17.9675000200274,
-31.7764473081038));
#234784=CARTESIAN_POINT('Ctrl Pts',(68.2272459721838,-17.9675000200274,
-32.54995));
#234785=CARTESIAN_POINT('Ctrl Pts',(66.8875000100282,-17.9675000200274,
-32.54995));
#234786=CARTESIAN_POINT('Origin',(66.8875000100282,-12.9675000200274,-32.54995));
#234787=CARTESIAN_POINT('',(64.0007486640801,-17.9675000200275,-31.7764473081038));
#234788=CARTESIAN_POINT('Ctrl Pts',(66.8875000100282,-17.9675000200274,
-32.54995));
#234789=CARTESIAN_POINT('Ctrl Pts',(65.5477540478726,-17.9675000200274,
-32.54995));
#234790=CARTESIAN_POINT('Ctrl Pts',(64.0007486640801,-17.9675000200275,
-31.7764473081038));
#234791=CARTESIAN_POINT('Ctrl Pts',(64.0007486640801,-17.9675000200274,
-31.7764473081038));
#234792=CARTESIAN_POINT('Ctrl Pts',(63.2272459721838,-16.6277540578719,
-32.54995));
#234793=CARTESIAN_POINT('Ctrl Pts',(62.557372991106,-15.4675000200275,-32.54995));
#234794=CARTESIAN_POINT('Origin',(66.8875000100282,-12.9675000200274,-32.54995));
#234795=CARTESIAN_POINT('',(61.1139973181319,-12.9675000200275,-31.7764473081038));
#234796=CARTESIAN_POINT('Ctrl Pts',(62.557372991106,-15.4675000200275,-32.54995));
#234797=CARTESIAN_POINT('Ctrl Pts',(61.8875000100282,-14.3072459821831,
-32.54995));
#234798=CARTESIAN_POINT('Ctrl Pts',(61.1139973181319,-12.9675000200275,
-31.7764473081037));
#234799=CARTESIAN_POINT('Ctrl Pts',(61.1139973181319,-12.9675000200275,
-31.7764473081037));
#234800=CARTESIAN_POINT('Ctrl Pts',(61.8875000100281,-11.6277540578719,
-32.5499499999999));
#234801=CARTESIAN_POINT('Ctrl Pts',(62.5573729911059,-10.4675000200275,
-32.5499499999999));
#234802=CARTESIAN_POINT('Origin',(66.8875000100282,-12.9675000200274,-32.54995));
#234803=CARTESIAN_POINT('',(64.00074866408,-7.96750002002747,-31.7764473081038));
#234804=CARTESIAN_POINT('Ctrl Pts',(62.5573729911059,-10.4675000200275,
-32.5499499999999));
#234805=CARTESIAN_POINT('Ctrl Pts',(63.2272459721837,-9.3072459821831,-32.54995));
#234806=CARTESIAN_POINT('Ctrl Pts',(64.00074866408,-7.9675000200275,-31.7764473081037));
#234807=CARTESIAN_POINT('Ctrl Pts',(64.00074866408,-7.96750002002747,-31.7764473081038));
#234808=CARTESIAN_POINT('Ctrl Pts',(65.5477540478725,-7.96750002002745,
-32.54995));
#234809=CARTESIAN_POINT('Ctrl Pts',(66.8875000100281,-7.96750002002744,
-32.54995));
#234810=CARTESIAN_POINT('Origin',(12.9675000200281,-12.967500020028,-28.54995));
#234811=CARTESIAN_POINT('',(66.8875000100281,-7.96750002002746,-28.54995));
#234812=CARTESIAN_POINT('',(71.2176270289503,-10.4675000200274,-28.54995));
#234813=CARTESIAN_POINT('Origin',(66.8875000100282,-12.9675000200274,-28.54995));
#234814=CARTESIAN_POINT('',(62.5573729911059,-10.4675000200275,-28.54995));
#234815=CARTESIAN_POINT('Origin',(66.8875000100282,-12.9675000200274,-28.54995));
#234816=CARTESIAN_POINT('',(62.557372991106,-15.4675000200275,-28.54995));
#234817=CARTESIAN_POINT('Origin',(66.8875000100282,-12.9675000200274,-28.54995));
#234818=CARTESIAN_POINT('',(66.8875000100282,-17.9675000200275,-28.54995));
#234819=CARTESIAN_POINT('Origin',(66.8875000100282,-12.9675000200274,-28.54995));
#234820=CARTESIAN_POINT('',(71.2176270289504,-15.4675000200274,-28.54995));
#234821=CARTESIAN_POINT('Origin',(66.8875000100282,-12.9675000200274,-28.54995));
#234822=CARTESIAN_POINT('Origin',(66.8875000100282,-12.9675000200274,-28.54995));
#234823=CARTESIAN_POINT('Origin',(66.8875000100282,-12.9675000200274,-28.54995));
#234824=CARTESIAN_POINT('',(64.0007486640797,-7.96750002002747,-28.9965319873851));
#234825=CARTESIAN_POINT('Ctrl Pts',(64.0007486640716,-7.96750002002748,
-28.9965319873876));
#234826=CARTESIAN_POINT('Ctrl Pts',(65.5477540478691,-7.96750002002746,
-28.54995));
#234827=CARTESIAN_POINT('Ctrl Pts',(66.8875000100281,-7.96750002002745,
-28.54995));
#234828=CARTESIAN_POINT('Ctrl Pts',(62.5573729911059,-10.4675000200275,
-28.54995));
#234829=CARTESIAN_POINT('Ctrl Pts',(63.2272459721853,-9.30724598218033,
-28.54995));
#234830=CARTESIAN_POINT('Ctrl Pts',(64.000748664084,-7.96750002002055,-28.9965319873875));
#234831=CARTESIAN_POINT('Origin',(66.8875000100282,-12.9675000200274,-28.54995));
#234832=CARTESIAN_POINT('',(61.1139973181319,-12.9675000200275,-28.9965319873852));
#234833=CARTESIAN_POINT('Ctrl Pts',(61.1139973181278,-12.9675000200346,
-28.9965319873876));
#234834=CARTESIAN_POINT('Ctrl Pts',(61.8875000100265,-11.6277540578747,
-28.54995));
#234835=CARTESIAN_POINT('Ctrl Pts',(62.5573729911059,-10.4675000200275,
-28.54995));
#234836=CARTESIAN_POINT('Ctrl Pts',(62.557372991106,-15.4675000200275,-28.54995));
#234837=CARTESIAN_POINT('Ctrl Pts',(61.8875000100266,-14.3072459821803,
-28.54995));
#234838=CARTESIAN_POINT('Ctrl Pts',(61.1139973181278,-12.9675000200204,
-28.9965319873876));
#234839=CARTESIAN_POINT('Origin',(66.8875000100282,-12.9675000200274,-28.54995));
#234840=CARTESIAN_POINT('',(64.0007486640801,-17.9675000200275,-28.9965319873852));
#234841=CARTESIAN_POINT('Ctrl Pts',(64.0007486640842,-17.9675000200345,
-28.9965319873876));
#234842=CARTESIAN_POINT('Ctrl Pts',(63.2272459721855,-16.6277540578747,
-28.54995));
#234843=CARTESIAN_POINT('Ctrl Pts',(62.557372991106,-15.4675000200275,-28.54995));
#234844=CARTESIAN_POINT('Ctrl Pts',(66.8875000100282,-17.9675000200274,
-28.54995));
#234845=CARTESIAN_POINT('Ctrl Pts',(65.5477540478693,-17.9675000200274,
-28.54995));
#234846=CARTESIAN_POINT('Ctrl Pts',(64.000748664072,-17.9675000200275,-28.9965319873876));
#234847=CARTESIAN_POINT('Origin',(66.8875000100282,-12.9675000200274,-28.54995));
#234848=CARTESIAN_POINT('',(69.7742513559763,-17.9675000200274,-28.9965319873852));
#234849=CARTESIAN_POINT('Ctrl Pts',(69.7742513559845,-17.9675000200274,
-28.9965319873875));
#234850=CARTESIAN_POINT('Ctrl Pts',(68.2272459721871,-17.9675000200274,
-28.54995));
#234851=CARTESIAN_POINT('Ctrl Pts',(66.8875000100282,-17.9675000200274,
-28.54995));
#234852=CARTESIAN_POINT('Ctrl Pts',(71.2176270289503,-15.4675000200274,
-28.54995));
#234853=CARTESIAN_POINT('Ctrl Pts',(70.5477540478709,-16.6277540578746,
-28.54995));
#234854=CARTESIAN_POINT('Ctrl Pts',(69.7742513559722,-17.9675000200345,
-28.9965319873875));
#234855=CARTESIAN_POINT('Origin',(66.8875000100282,-12.9675000200274,-28.54995));
#234856=CARTESIAN_POINT('',(72.6610027019244,-12.9675000200274,-28.9965319873853));
#234857=CARTESIAN_POINT('Ctrl Pts',(72.6610027019285,-12.9675000200203,
-28.9965319873875));
#234858=CARTESIAN_POINT('Ctrl Pts',(71.8875000100298,-14.3072459821802,
-28.54995));
#234859=CARTESIAN_POINT('Ctrl Pts',(71.2176270289503,-15.4675000200274,
-28.54995));
#234860=CARTESIAN_POINT('Ctrl Pts',(71.2176270289503,-10.4675000200274,
-28.54995));
#234861=CARTESIAN_POINT('Ctrl Pts',(71.8875000100298,-11.6277540578746,
-28.54995));
#234862=CARTESIAN_POINT('Ctrl Pts',(72.6610027019285,-12.9675000200345,
-28.9965319873875));
#234863=CARTESIAN_POINT('Origin',(66.8875000100282,-12.9675000200274,-28.54995));
#234864=CARTESIAN_POINT('',(69.7742513559762,-7.96750002002741,-28.9965319873852));
#234865=CARTESIAN_POINT('Ctrl Pts',(66.8875000100281,-7.96750002002745,
-28.54995));
#234866=CARTESIAN_POINT('Ctrl Pts',(68.227245972187,-7.96750002002743,-28.54995));
#234867=CARTESIAN_POINT('Ctrl Pts',(69.7742513559844,-7.96750002002742,
-28.9965319873875));
#234868=CARTESIAN_POINT('Ctrl Pts',(69.7742513559721,-7.96750002002036,
-28.9965319873875));
#234869=CARTESIAN_POINT('Ctrl Pts',(70.5477540478708,-9.3072459821802,-28.54995));
#234870=CARTESIAN_POINT('Ctrl Pts',(71.2176270289503,-10.4675000200274,
-28.54995));
#234871=CARTESIAN_POINT('Origin',(64.00074866408,-7.96750002002747,-32.54995));
#234872=CARTESIAN_POINT('',(64.00074866408,-7.96750002002747,-32.54995));
#234873=CARTESIAN_POINT('',(69.7742513559762,-7.96750002002741,-32.54995));
#234874=CARTESIAN_POINT('Origin',(61.1139973181319,-12.9675000200275,-32.54995));
#234875=CARTESIAN_POINT('',(61.1139973181319,-12.9675000200275,-32.54995));
#234876=CARTESIAN_POINT('Origin',(64.0007486640801,-17.9675000200275,-32.54995));
#234877=CARTESIAN_POINT('',(64.0007486640801,-17.9675000200275,-32.54995));
#234878=CARTESIAN_POINT('Origin',(69.7742513559763,-17.9675000200274,-32.54995));
#234879=CARTESIAN_POINT('',(69.7742513559763,-17.9675000200274,-32.54995));
#234880=CARTESIAN_POINT('Origin',(72.6610027019244,-12.9675000200274,-32.54995));
#234881=CARTESIAN_POINT('',(72.6610027019244,-12.9675000200274,-32.54995));
#234882=CARTESIAN_POINT('Origin',(69.7742513559762,-7.96750002002741,-32.54995));
#234883=CARTESIAN_POINT('Origin',(0.,-25.9350000400563,-32.54995));
#234884=CARTESIAN_POINT('',(2.5,-75.5248730111341,-32.54995));
#234885=CARTESIAN_POINT('',(5.,-79.8550000300563,-32.54995));
#234886=CARTESIAN_POINT('Origin',(1.73472347597681E-15,-79.8550000300563,
-32.54995));
#234887=CARTESIAN_POINT('',(2.5,-84.1851270489785,-32.54995));
#234888=CARTESIAN_POINT('Origin',(1.73472347597681E-15,-79.8550000300563,
-32.54995));
#234889=CARTESIAN_POINT('',(-2.5,-84.1851270489785,-32.54995));
#234890=CARTESIAN_POINT('Origin',(1.73472347597681E-15,-79.8550000300563,
-32.54995));
#234891=CARTESIAN_POINT('',(-5.,-79.8550000300563,-32.54995));
#234892=CARTESIAN_POINT('Origin',(1.73472347597681E-15,-79.8550000300563,
-32.54995));
#234893=CARTESIAN_POINT('',(-2.5,-75.5248730111341,-32.54995));
#234894=CARTESIAN_POINT('Origin',(1.73472347597681E-15,-79.8550000300563,
-32.54995));
#234895=CARTESIAN_POINT('Origin',(1.73472347597681E-15,-79.8550000300563,
-32.54995));
#234896=CARTESIAN_POINT('Origin',(1.73472347597681E-15,-79.8550000300563,
-32.54995));
#234897=CARTESIAN_POINT('',(5.,-82.7417513760044,-31.7764473081038));
#234898=CARTESIAN_POINT('Ctrl Pts',(4.99999999999997,-82.7417513760044,
-31.7764473081038));
#234899=CARTESIAN_POINT('Ctrl Pts',(3.66025403784437,-83.5152540679007,
-32.54995));
#234900=CARTESIAN_POINT('Ctrl Pts',(2.49999999999999,-84.1851270489785,
-32.54995));
#234901=CARTESIAN_POINT('Ctrl Pts',(5.,-79.8550000300563,-32.54995));
#234902=CARTESIAN_POINT('Ctrl Pts',(5.,-81.1947459922119,-32.54995));
#234903=CARTESIAN_POINT('Ctrl Pts',(5.,-82.7417513760044,-31.7764473081038));
#234904=CARTESIAN_POINT('Origin',(1.73472347597681E-15,-79.8550000300563,
-32.54995));
#234905=CARTESIAN_POINT('',(1.66200633571292E-14,-85.6285027219525,-31.7764473081038));
#234906=CARTESIAN_POINT('Ctrl Pts',(2.49999999999999,-84.1851270489785,
-32.54995));
#234907=CARTESIAN_POINT('Ctrl Pts',(1.33974596215563,-84.8550000300563,
-32.54995));
#234908=CARTESIAN_POINT('Ctrl Pts',(6.04428732283895E-14,-85.6285027219525,
-31.7764473081038));
#234909=CARTESIAN_POINT('Ctrl Pts',(-1.4353188893285E-15,-85.6285027219525,
-31.7764473081038));
#234910=CARTESIAN_POINT('Ctrl Pts',(-1.33974596215561,-84.8550000300562,
-32.5499500000001));
#234911=CARTESIAN_POINT('Ctrl Pts',(-2.5,-84.1851270489784,-32.5499500000001));
#234912=CARTESIAN_POINT('Origin',(1.73472347597681E-15,-79.8550000300563,
-32.54995));
#234913=CARTESIAN_POINT('',(-5.,-82.7417513760044,-31.7764473081038));
#234914=CARTESIAN_POINT('Ctrl Pts',(-2.5,-84.1851270489784,-32.5499500000001));
#234915=CARTESIAN_POINT('Ctrl Pts',(-3.66025403784436,-83.5152540679006,
-32.5499500000001));
#234916=CARTESIAN_POINT('Ctrl Pts',(-4.99999999999996,-82.7417513760044,
-31.7764473081038));
#234917=CARTESIAN_POINT('Ctrl Pts',(-5.,-82.7417513760044,-31.7764473081038));
#234918=CARTESIAN_POINT('Ctrl Pts',(-5.,-81.1947459922119,-32.54995));
#234919=CARTESIAN_POINT('Ctrl Pts',(-5.,-79.8550000300563,-32.54995));
#234920=CARTESIAN_POINT('Origin',(1.73472347597681E-15,-79.8550000300563,
-32.54995));
#234921=CARTESIAN_POINT('',(-5.,-76.9682486841082,-31.7764473081038));
#234922=CARTESIAN_POINT('Ctrl Pts',(-5.,-79.8550000300563,-32.54995));
#234923=CARTESIAN_POINT('Ctrl Pts',(-5.,-78.5152540679007,-32.54995));
#234924=CARTESIAN_POINT('Ctrl Pts',(-5.,-76.9682486841082,-31.7764473081038));
#234925=CARTESIAN_POINT('Ctrl Pts',(-4.99999999999992,-76.9682486841082,
-31.7764473081038));
#234926=CARTESIAN_POINT('Ctrl Pts',(-3.66025403784435,-76.1947459922119,
-32.54995));
#234927=CARTESIAN_POINT('Ctrl Pts',(-2.5,-75.5248730111341,-32.54995));
#234928=CARTESIAN_POINT('Origin',(1.73472347597681E-15,-79.8550000300563,
-32.54995));
#234929=CARTESIAN_POINT('',(2.79122613421945E-15,-74.0814973381601,-31.7764473081038));
#234930=CARTESIAN_POINT('Ctrl Pts',(-2.50000000000003,-75.5248730111342,
-32.54995));
#234931=CARTESIAN_POINT('Ctrl Pts',(-1.33974596215564,-74.8550000300563,
-32.54995));
#234932=CARTESIAN_POINT('Ctrl Pts',(-3.65208917395811E-14,-74.0814973381601,
-31.7764473081038));
#234933=CARTESIAN_POINT('Ctrl Pts',(4.00294490246061E-14,-74.0814973381601,
-31.7764473081038));
#234934=CARTESIAN_POINT('Ctrl Pts',(1.33974596215562,-74.8550000300563,
-32.54995));
#234935=CARTESIAN_POINT('Ctrl Pts',(2.49999999999998,-75.5248730111341,
-32.54995));
#234936=CARTESIAN_POINT('Origin',(1.73472347597681E-15,-79.8550000300563,
-32.54995));
#234937=CARTESIAN_POINT('',(5.,-76.9682486841082,-31.7764473081038));
#234938=CARTESIAN_POINT('Ctrl Pts',(2.49999999999997,-75.5248730111341,
-32.5499500000001));
#234939=CARTESIAN_POINT('Ctrl Pts',(3.66025403784435,-76.194745992212,-32.5499500000001));
#234940=CARTESIAN_POINT('Ctrl Pts',(4.99999999999997,-76.9682486841082,
-31.7764473081038));
#234941=CARTESIAN_POINT('Ctrl Pts',(5.,-76.9682486841082,-31.7764473081038));
#234942=CARTESIAN_POINT('Ctrl Pts',(5.,-78.5152540679007,-32.54995));
#234943=CARTESIAN_POINT('Ctrl Pts',(5.,-79.8550000300563,-32.54995));
#234944=CARTESIAN_POINT('Origin',(0.,-25.9350000400563,-28.54995));
#234945=CARTESIAN_POINT('',(5.,-79.8550000300563,-28.54995));
#234946=CARTESIAN_POINT('',(2.5,-84.1851270489785,-28.54995));
#234947=CARTESIAN_POINT('Origin',(1.73472347597681E-15,-79.8550000300563,
-28.54995));
#234948=CARTESIAN_POINT('',(2.5,-75.5248730111341,-28.54995));
#234949=CARTESIAN_POINT('Origin',(1.73472347597681E-15,-79.8550000300563,
-28.54995));
#234950=CARTESIAN_POINT('',(-2.5,-75.5248730111341,-28.54995));
#234951=CARTESIAN_POINT('Origin',(1.73472347597681E-15,-79.8550000300563,
-28.54995));
#234952=CARTESIAN_POINT('',(-5.,-79.8550000300563,-28.54995));
#234953=CARTESIAN_POINT('Origin',(1.73472347597681E-15,-79.8550000300563,
-28.54995));
#234954=CARTESIAN_POINT('',(-2.5,-84.1851270489785,-28.54995));
#234955=CARTESIAN_POINT('Origin',(1.73472347597681E-15,-79.8550000300563,
-28.54995));
#234956=CARTESIAN_POINT('Origin',(1.73472347597681E-15,-79.8550000300563,
-28.54995));
#234957=CARTESIAN_POINT('Origin',(1.73472347597681E-15,-79.8550000300563,
-28.54995));
#234958=CARTESIAN_POINT('',(5.,-76.9682486841079,-28.9965319873851));
#234959=CARTESIAN_POINT('Ctrl Pts',(5.,-76.9682486840998,-28.9965319873876));
#234960=CARTESIAN_POINT('Ctrl Pts',(5.,-78.5152540678973,-28.54995));
#234961=CARTESIAN_POINT('Ctrl Pts',(5.,-79.8550000300563,-28.54995));
#234962=CARTESIAN_POINT('Ctrl Pts',(2.49999999999998,-75.5248730111342,
-28.54995));
#234963=CARTESIAN_POINT('Ctrl Pts',(3.66025403784715,-76.1947459922136,
-28.54995));
#234964=CARTESIAN_POINT('Ctrl Pts',(5.00000000000691,-76.9682486841122,
-28.9965319873875));
#234965=CARTESIAN_POINT('Origin',(1.73472347597681E-15,-79.8550000300563,
-28.54995));
#234966=CARTESIAN_POINT('',(3.91685175604228E-15,-74.0814973381601,-28.9965319873853));
#234967=CARTESIAN_POINT('Ctrl Pts',(-7.07188757544677E-12,-74.081497338156,
-28.9965319873875));
#234968=CARTESIAN_POINT('Ctrl Pts',(1.33974596215276,-74.8550000300547,
-28.54995));
#234969=CARTESIAN_POINT('Ctrl Pts',(2.49999999999998,-75.5248730111342,
-28.54995));
#234970=CARTESIAN_POINT('Ctrl Pts',(-2.49999999999996,-75.5248730111341,
-28.54995));
#234971=CARTESIAN_POINT('Ctrl Pts',(-1.33974596215275,-74.8550000300547,
-28.54995));
#234972=CARTESIAN_POINT('Ctrl Pts',(7.06804165007405E-12,-74.081497338156,
-28.9965319873876));
#234973=CARTESIAN_POINT('Origin',(1.73472347597681E-15,-79.8550000300563,
-28.54995));
#234974=CARTESIAN_POINT('',(-5.,-76.9682486841082,-28.9965319873852));
#234975=CARTESIAN_POINT('Ctrl Pts',(-5.00000000000705,-76.9682486841123,
-28.9965319873875));
#234976=CARTESIAN_POINT('Ctrl Pts',(-3.6602540378472,-76.1947459922136,
-28.54995));
#234977=CARTESIAN_POINT('Ctrl Pts',(-2.49999999999996,-75.5248730111341,
-28.54995));
#234978=CARTESIAN_POINT('Ctrl Pts',(-5.,-79.8550000300563,-28.54995));
#234979=CARTESIAN_POINT('Ctrl Pts',(-5.,-78.5152540678974,-28.54995));
#234980=CARTESIAN_POINT('Ctrl Pts',(-5.,-76.9682486841001,-28.9965319873875));
#234981=CARTESIAN_POINT('Origin',(1.73472347597681E-15,-79.8550000300563,
-28.54995));
#234982=CARTESIAN_POINT('',(-5.,-82.7417513760044,-28.9965319873853));
#234983=CARTESIAN_POINT('Ctrl Pts',(-5.,-82.7417513760125,-28.9965319873876));
#234984=CARTESIAN_POINT('Ctrl Pts',(-5.,-81.1947459922152,-28.54995));
#234985=CARTESIAN_POINT('Ctrl Pts',(-5.,-79.8550000300563,-28.54995));
#234986=CARTESIAN_POINT('Ctrl Pts',(-2.49999999999998,-84.1851270489784,
-28.5499499999999));
#234987=CARTESIAN_POINT('Ctrl Pts',(-3.66025403784722,-83.515254067899,
-28.54995));
#234988=CARTESIAN_POINT('Ctrl Pts',(-5.00000000000709,-82.7417513760002,
-28.9965319873875));
#234989=CARTESIAN_POINT('Origin',(1.73472347597681E-15,-79.8550000300563,
-28.54995));
#234990=CARTESIAN_POINT('',(1.57929637069991E-14,-85.6285027219525,-28.9965319873853));
#234991=CARTESIAN_POINT('Ctrl Pts',(7.10342416350341E-12,-85.6285027219566,
-28.9965319873875));
#234992=CARTESIAN_POINT('Ctrl Pts',(-1.33974596215273,-84.8550000300579,
-28.54995));
#234993=CARTESIAN_POINT('Ctrl Pts',(-2.49999999999995,-84.1851270489784,
-28.5499499999999));
#234994=CARTESIAN_POINT('Ctrl Pts',(2.49999999999998,-84.1851270489785,
-28.54995));
#234995=CARTESIAN_POINT('Ctrl Pts',(1.33974596215279,-84.8550000300579,
-28.54995));
#234996=CARTESIAN_POINT('Ctrl Pts',(-7.00830160928372E-12,-85.6285027219566,
-28.9965319873875));
#234997=CARTESIAN_POINT('Origin',(1.73472347597681E-15,-79.8550000300563,
-28.54995));
#234998=CARTESIAN_POINT('',(5.,-82.7417513760044,-28.9965319873853));
#234999=CARTESIAN_POINT('Ctrl Pts',(5.,-79.8550000300563,-28.54995));
#235000=CARTESIAN_POINT('Ctrl Pts',(5.,-81.1947459922152,-28.54995));
#235001=CARTESIAN_POINT('Ctrl Pts',(5.,-82.7417513760126,-28.9965319873876));
#235002=CARTESIAN_POINT('Ctrl Pts',(5.00000000000707,-82.7417513760004,
-28.9965319873876));
#235003=CARTESIAN_POINT('Ctrl Pts',(3.66025403784723,-83.515254067899,-28.54995));
#235004=CARTESIAN_POINT('Ctrl Pts',(2.50000000000001,-84.1851270489785,
-28.54995));
#235005=CARTESIAN_POINT('Origin',(5.,-76.9682486841082,-32.54995));
#235006=CARTESIAN_POINT('',(5.,-76.9682486841082,-32.54995));
#235007=CARTESIAN_POINT('',(5.,-82.7417513760044,-32.54995));
#235008=CARTESIAN_POINT('Origin',(3.63207727782644E-15,-74.0814973381601,
-32.54995));
#235009=CARTESIAN_POINT('',(3.63207727782644E-15,-74.0814973381601,-32.54995));
#235010=CARTESIAN_POINT('Origin',(-5.,-76.9682486841082,-32.54995));
#235011=CARTESIAN_POINT('',(-5.,-76.9682486841082,-32.54995));
#235012=CARTESIAN_POINT('Origin',(-5.,-82.7417513760044,-32.54995));
#235013=CARTESIAN_POINT('',(-5.,-82.7417513760044,-32.54995));
#235014=CARTESIAN_POINT('Origin',(1.56125112837912E-14,-85.6285027219525,
-32.54995));
#235015=CARTESIAN_POINT('',(1.56125112837912E-14,-85.6285027219525,-32.54995));
#235016=CARTESIAN_POINT('Origin',(5.,-82.7417513760044,-32.54995));
#235017=CARTESIAN_POINT('Origin',(-47.392180948596,-60.9300389954978,-220.195349461621));
#235018=CARTESIAN_POINT('',(-47.392180948596,-60.9300389954978,-221.195349461621));
#235019=CARTESIAN_POINT('',(-47.392180948596,-60.9300389954978,-223.85005));
#235020=CARTESIAN_POINT('',(-47.392180948596,-60.9300389954978,-220.195349461621));
#235021=CARTESIAN_POINT('',(-48.892180948596,-60.0640135917134,-221.195349461621));
#235022=CARTESIAN_POINT('Ctrl Pts',(-48.8921809485959,-60.0640135917134,
-221.195349461621));
#235023=CARTESIAN_POINT('Ctrl Pts',(-48.142180948596,-60.4970262936056,
-220.945349461621));
#235024=CARTESIAN_POINT('Ctrl Pts',(-47.3921809485963,-60.9300389954976,
-221.195349461621));
#235025=CARTESIAN_POINT('',(-48.892180948596,-60.0640135917134,-223.85005));
#235026=CARTESIAN_POINT('',(-48.892180948596,-60.0640135917134,-220.195349461621));
#235027=CARTESIAN_POINT('Ctrl Pts',(-47.392180948596,-60.9300389954978,
-223.85005));
#235028=CARTESIAN_POINT('Ctrl Pts',(-48.142180948596,-60.4970262936056,
-223.417037298108));
#235029=CARTESIAN_POINT('Ctrl Pts',(-48.892180948596,-60.0640135917134,
-223.85005));
#235030=CARTESIAN_POINT('Origin',(-47.392180948596,-62.6620898030667,-220.195349461621));
#235031=CARTESIAN_POINT('',(-47.392180948596,-62.6620898030667,-221.195349461621));
#235032=CARTESIAN_POINT('',(-47.392180948596,-62.6620898030667,-223.85005));
#235033=CARTESIAN_POINT('',(-47.392180948596,-62.6620898030667,-220.195349461621));
#235034=CARTESIAN_POINT('Ctrl Pts',(-47.392180948596,-60.9300389954979,
-221.195349461621));
#235035=CARTESIAN_POINT('Ctrl Pts',(-47.392180948596,-61.7960643992822,
-220.945349461621));
#235036=CARTESIAN_POINT('Ctrl Pts',(-47.392180948596,-62.6620898030664,
-221.195349461621));
#235037=CARTESIAN_POINT('Ctrl Pts',(-47.392180948596,-62.6620898030667,
-223.85005));
#235038=CARTESIAN_POINT('Ctrl Pts',(-47.392180948596,-61.7960643992823,
-223.417037298108));
#235039=CARTESIAN_POINT('Ctrl Pts',(-47.392180948596,-60.9300389954978,
-223.85005));
#235040=CARTESIAN_POINT('Origin',(-48.892180948596,-63.5281152068512,-220.195349461621));
#235041=CARTESIAN_POINT('',(-48.892180948596,-63.5281152068512,-221.195349461621));
#235042=CARTESIAN_POINT('',(-48.892180948596,-63.5281152068512,-223.85005));
#235043=CARTESIAN_POINT('',(-48.892180948596,-63.5281152068512,-220.195349461621));
#235044=CARTESIAN_POINT('Ctrl Pts',(-47.392180948596,-62.6620898030668,
-221.195349461621));
#235045=CARTESIAN_POINT('Ctrl Pts',(-48.142180948596,-63.095102504959,-220.945349461621));
#235046=CARTESIAN_POINT('Ctrl Pts',(-48.8921809485959,-63.5281152068512,
-221.195349461621));
#235047=CARTESIAN_POINT('Ctrl Pts',(-48.892180948596,-63.5281152068512,
-223.85005));
#235048=CARTESIAN_POINT('Ctrl Pts',(-48.142180948596,-63.095102504959,-223.417037298108));
#235049=CARTESIAN_POINT('Ctrl Pts',(-47.392180948596,-62.6620898030667,
-223.85005));
#235050=CARTESIAN_POINT('Origin',(-50.392180948596,-62.6620898030667,-220.195349461621));
#235051=CARTESIAN_POINT('',(-50.392180948596,-62.6620898030677,-221.19534946162));
#235052=CARTESIAN_POINT('',(-50.392180948596,-62.6620898030667,-223.85005));
#235053=CARTESIAN_POINT('',(-50.392180948596,-62.6620898030667,-220.195349461621));
#235054=CARTESIAN_POINT('Ctrl Pts',(-48.892180948596,-63.5281152068511,
-221.195349461621));
#235055=CARTESIAN_POINT('Ctrl Pts',(-49.6421809485958,-63.095102504959,
-220.945349461621));
#235056=CARTESIAN_POINT('Ctrl Pts',(-50.3921809485956,-62.662089803067,
-221.195349461621));
#235057=CARTESIAN_POINT('Ctrl Pts',(-50.392180948596,-62.6620898030667,
-223.85005));
#235058=CARTESIAN_POINT('Ctrl Pts',(-49.642180948596,-63.0951025049589,
-223.417037298108));
#235059=CARTESIAN_POINT('Ctrl Pts',(-48.892180948596,-63.5281152068512,
-223.85005));
#235060=CARTESIAN_POINT('Origin',(-50.392180948596,-60.9300389954978,-220.195349461621));
#235061=CARTESIAN_POINT('',(-50.392180948596,-60.9300389954978,-221.195349461621));
#235062=CARTESIAN_POINT('',(-50.392180948596,-60.9300389954978,-223.85005));
#235063=CARTESIAN_POINT('',(-50.392180948596,-60.9300389954978,-220.195349461621));
#235064=CARTESIAN_POINT('Ctrl Pts',(-50.392180948596,-62.6620898030674,
-221.195349461621));
#235065=CARTESIAN_POINT('Ctrl Pts',(-50.392180948596,-61.7960643992827,
-220.945349461621));
#235066=CARTESIAN_POINT('Ctrl Pts',(-50.392180948596,-60.9300389954982,
-221.195349461621));
#235067=CARTESIAN_POINT('Ctrl Pts',(-50.392180948596,-60.9300389954978,
-223.85005));
#235068=CARTESIAN_POINT('Ctrl Pts',(-50.392180948596,-61.7960643992823,
-223.417037298108));
#235069=CARTESIAN_POINT('Ctrl Pts',(-50.392180948596,-62.6620898030667,
-223.85005));
#235070=CARTESIAN_POINT('Origin',(-48.892180948596,-60.0640135917134,-220.195349461621));
#235071=CARTESIAN_POINT('Ctrl Pts',(-50.392180948596,-60.9300389954978,
-221.195349461621));
#235072=CARTESIAN_POINT('Ctrl Pts',(-49.642180948596,-60.4970262936056,
-220.945349461621));
#235073=CARTESIAN_POINT('Ctrl Pts',(-48.8921809485959,-60.0640135917133,
-221.195349461621));
#235074=CARTESIAN_POINT('Ctrl Pts',(-48.892180948596,-60.0640135917134,
-223.85005));
#235075=CARTESIAN_POINT('Ctrl Pts',(-49.642180948596,-60.4970262936056,
-223.417037298108));
#235076=CARTESIAN_POINT('Ctrl Pts',(-50.392180948596,-60.9300389954978,
-223.85005));
#235077=CARTESIAN_POINT('Origin',(-48.892180948596,-61.7960643992823,-221.35005));
#235078=CARTESIAN_POINT('',(-48.892180948596,-61.7960643992823,-220.195349461621));
#235079=CARTESIAN_POINT('',(-48.892180948596,-63.7960643992823,-221.35005));
#235080=CARTESIAN_POINT('Origin',(-48.892180948596,-61.7960643992823,-223.85005));
#235081=CARTESIAN_POINT('Origin',(-48.892180948596,-61.7960643992823,-223.85005));
#235082=CARTESIAN_POINT('Origin',(-48.892180948596,-61.7960643992823,-223.85005));
#235083=CARTESIAN_POINT('Origin',(-48.892180948596,-61.7960643992823,-223.85005));
#235084=CARTESIAN_POINT('Origin',(-48.892180948596,-61.7960643992823,-223.85005));
#235085=CARTESIAN_POINT('Origin',(-48.892180948596,-61.7960643992823,-223.85005));
#235086=CARTESIAN_POINT('Origin',(-48.892180948596,-61.7960643992823,-223.85005));
#235087=CARTESIAN_POINT('Origin',(-48.892180948596,-61.7960643992823,-223.85005));
#235088=CARTESIAN_POINT('Origin',(-48.892180948596,-61.7960643992823,-223.85005));
#235089=CARTESIAN_POINT('Origin',(-48.892180948596,-61.7960643992823,-223.85005));
#235090=CARTESIAN_POINT('Origin',(-48.892180948596,-61.7960643992823,-223.85005));
#235091=CARTESIAN_POINT('Origin',(-48.892180948596,-61.7960643992823,-223.85005));
#235092=CARTESIAN_POINT('Origin',(-48.892180948596,-61.7960643992823,-223.60005));
#235093=CARTESIAN_POINT('',(-48.892180948596,-64.7960643992823,-223.85005));
#235094=CARTESIAN_POINT('Origin',(-48.892180948596,-61.7960643992823,-223.85005));
#235095=CARTESIAN_POINT('',(-48.892180948596,-65.0460643992823,-223.60005));
#235096=CARTESIAN_POINT('Origin',(-48.892180948596,-64.7960643992823,-223.60005));
#235097=CARTESIAN_POINT('',(-48.892180948596,-58.5460643992823,-223.60005));
#235098=CARTESIAN_POINT('Origin',(-48.892180948596,-61.7960643992823,-223.60005));
#235099=CARTESIAN_POINT('Origin',(-48.892180948596,-61.7960643992823,-223.60005));
#235100=CARTESIAN_POINT('Origin',(-48.892180948596,-61.7960643992823,-218.35005));
#235101=CARTESIAN_POINT('',(-48.892180948596,-58.5460643992823,-218.35005));
#235102=CARTESIAN_POINT('Origin',(-48.892180948596,-61.7960643992823,-218.35005));
#235103=CARTESIAN_POINT('Origin',(-48.892180948596,-61.7960643992823,-223.85005));
#235104=CARTESIAN_POINT('Origin',(-48.892180948596,-61.7960643992823,-223.85005));
#235105=CARTESIAN_POINT('',(-48.892180948596,-58.5460643992823,-223.85005));
#235106=CARTESIAN_POINT('Origin',(-14.75,97.3100982187845,-189.413464213672));
#235107=CARTESIAN_POINT('',(-14.,96.9977203019102,-189.84995));
#235108=CARTESIAN_POINT('',(-14.75,97.9199999800001,-189.84995));
#235109=CARTESIAN_POINT('Origin',(-14.7499999999998,96.9977203019109,-189.84995));
#235110=CARTESIAN_POINT('',(-14.,97.9199999800002,-188.561248242419));
#235111=CARTESIAN_POINT('Origin',(-14.7499999999994,97.9199999800002,-188.56124824242));
#235112=CARTESIAN_POINT('',(-14.,-43.3014970868467,-385.890101736374));
#235113=CARTESIAN_POINT('Origin',(-14.75,97.3100982187848,-80.2864357863281));
#235114=CARTESIAN_POINT('',(-14.,97.5344695959176,-80.59995));
#235115=CARTESIAN_POINT('',(-14.,97.9199999800001,-81.1386517575809));
#235116=CARTESIAN_POINT('',(-14.,-43.3014970868374,116.19020173637));
#235117=CARTESIAN_POINT('',(-14.1688463988223,97.9199999800001,-80.3240391180339));
#235118=CARTESIAN_POINT('Origin',(-14.7500000000031,97.9199999800002,-81.138651757583));
#235119=CARTESIAN_POINT('Origin',(-14.75,97.5344695959176,-80.59995));
#235120=CARTESIAN_POINT('Origin',(-14.75,97.5344695959176,-80.59995));
#235121=CARTESIAN_POINT('',(-14.75,97.9199999800001,-79.9566255694448));
#235122=CARTESIAN_POINT('Origin',(-14.75,97.9199999800001,-80.59995));
#235123=CARTESIAN_POINT('',(-14.75,97.5344695959176,-79.84995));
#235124=CARTESIAN_POINT('Origin',(-14.75,97.5344695959176,-80.59995));
#235125=CARTESIAN_POINT('Origin',(-14.75,97.5344695959176,-80.59995));
#235126=CARTESIAN_POINT('Origin',(48.,97.5344695959176,-80.59995));
#235127=CARTESIAN_POINT('',(-40.9309791607344,97.9199999800001,-79.9566255694448));
#235128=CARTESIAN_POINT('',(48.,97.9199999800001,-79.9566255694448));
#235129=CARTESIAN_POINT('',(-40.9309791607344,97.5344695959176,-79.84995));
#235130=CARTESIAN_POINT('Origin',(-40.9309791607344,97.5344695959176,-80.59995));
#235131=CARTESIAN_POINT('',(48.,97.5344695959176,-79.84995));
#235132=CARTESIAN_POINT('Origin',(-40.9309791607344,97.5344695959176,-80.59995));
#235133=CARTESIAN_POINT('',(-41.2284392666181,97.9199999800001,-80.0295257645779));
#235134=CARTESIAN_POINT('Origin',(-40.9309791607344,97.9199999800001,-80.59995));
#235135=CARTESIAN_POINT('Origin',(-40.9309791607344,97.5344695959176,-80.59995));
#235136=CARTESIAN_POINT('Origin',(-57.25,98.9199999800001,-173.84995));
#235137=CARTESIAN_POINT('',(-57.8072469207768,97.9199999800001,-173.103241263434));
#235138=CARTESIAN_POINT('',(-58.,97.5177878719661,-172.802905968413));
#235139=CARTESIAN_POINT('Origin',(-57.25,97.5177878719661,-172.802905968413));
#235140=CARTESIAN_POINT('',(-57.25,97.9199999800001,-173.84995));
#235141=CARTESIAN_POINT('Ctrl Pts',(-57.8072469207768,97.9199999800001,
-173.103241263434));
#235142=CARTESIAN_POINT('Ctrl Pts',(-57.6651860234659,97.9199999800001,
-173.36682332955));
#235143=CARTESIAN_POINT('Ctrl Pts',(-57.4409434098566,97.9199999800001,
-173.629467541839));
#235144=CARTESIAN_POINT('Ctrl Pts',(-57.25,97.9199999800001,-173.84995));
#235145=CARTESIAN_POINT('',(-58.,97.1699999800001,-173.84995));
#235146=CARTESIAN_POINT('Origin',(-57.25,97.1699999800001,-173.84995));
#235147=CARTESIAN_POINT('Origin',(-58.,98.9199999800001,-173.84995));
#235148=CARTESIAN_POINT('Origin',(-57.25,97.5177878719661,-172.802905968413));
#235149=CARTESIAN_POINT('',(-57.8822667063023,97.9199999800001,-172.833958057747));
#235150=CARTESIAN_POINT('Origin',(-57.25,97.5177878719661,-172.802905968413));
#235151=CARTESIAN_POINT('Origin',(-57.25,97.9199999800001,-172.802905968413));
#235152=CARTESIAN_POINT('Origin',(-57.25,-394.08000002,-134.84995));
#235153=CARTESIAN_POINT('',(-58.,97.9199999800001,-167.173500656049));
#235154=CARTESIAN_POINT('Origin',(-58.,-394.08000002,-134.84995));
#235155=CARTESIAN_POINT('Ctrl Pts',(-58.,97.9199999800002,-167.173500656049));
#235156=CARTESIAN_POINT('Ctrl Pts',(-58.,97.9199999800002,-168.594527486982));
#235157=CARTESIAN_POINT('Ctrl Pts',(-57.9835908722536,97.9199999800001,
-170.15643772184));
#235158=CARTESIAN_POINT('Ctrl Pts',(-57.9159202399799,97.9199999800001,
-172.088208331578));
#235159=CARTESIAN_POINT('Ctrl Pts',(-57.9005229085552,97.9199999800001,
-172.462234637024));
#235160=CARTESIAN_POINT('Ctrl Pts',(-57.8822667063024,97.9199999800001,
-172.833958057747));
#235161=CARTESIAN_POINT('Origin',(-57.25,-394.08000002,-134.84995));
#235162=CARTESIAN_POINT('',(-57.8822667063027,97.9199999800001,-96.8659419422532));
#235163=CARTESIAN_POINT('',(-58.,97.5177878719661,-96.8969940315874));
#235164=CARTESIAN_POINT('Origin',(-57.25,97.5177878719661,-96.8969940315874));
#235165=CARTESIAN_POINT('',(-58.,97.9199999800001,-102.526399343951));
#235166=CARTESIAN_POINT('Ctrl Pts',(-57.8822667063024,97.9199999800001,
-96.8659419422532));
#235167=CARTESIAN_POINT('Ctrl Pts',(-57.9005229085552,97.9199999800001,
-97.2376653629762));
#235168=CARTESIAN_POINT('Ctrl Pts',(-57.9159202399799,97.9199999800001,
-97.6116916684221));
#235169=CARTESIAN_POINT('Ctrl Pts',(-57.9835908722536,97.9199999800001,
-99.5434622781595));
#235170=CARTESIAN_POINT('Ctrl Pts',(-58.,97.9199999800002,-101.105372513018));
#235171=CARTESIAN_POINT('Ctrl Pts',(-58.,97.9199999800002,-102.526399343951));
#235172=CARTESIAN_POINT('Origin',(-58.,-394.08000002,-134.84995));
#235173=CARTESIAN_POINT('Origin',(-57.25,97.5177878719661,-96.8969940315875));
#235174=CARTESIAN_POINT('',(-57.8072469207768,97.9199999800001,-96.5966587365659));
#235175=CARTESIAN_POINT('Origin',(-57.25,97.5177878719662,-96.8969940315876));
#235176=CARTESIAN_POINT('Origin',(-57.25,97.9199999800001,-96.8969940315875));
#235177=CARTESIAN_POINT('Origin',(-57.25,98.9199999800001,-95.84995));
#235178=CARTESIAN_POINT('',(-57.25,97.9199999800001,-95.84995));
#235179=CARTESIAN_POINT('',(-58.,97.1699999800001,-95.84995));
#235180=CARTESIAN_POINT('Origin',(-57.25,97.1699999800001,-95.84995));
#235181=CARTESIAN_POINT('Ctrl Pts',(-57.25,97.9199999800001,-95.84995));
#235182=CARTESIAN_POINT('Ctrl Pts',(-57.4409434098566,97.9199999800001,
-96.0704324581614));
#235183=CARTESIAN_POINT('Ctrl Pts',(-57.6651860234659,97.9199999800001,
-96.3330766704501));
#235184=CARTESIAN_POINT('Ctrl Pts',(-57.8072469207768,97.9199999800001,
-96.5966587365659));
#235185=CARTESIAN_POINT('Origin',(-58.,98.9199999800001,-95.84995));
#235186=CARTESIAN_POINT('Origin',(-42.,98.9199999800001,-189.09995));
#235187=CARTESIAN_POINT('',(-42.,97.1699999800001,-189.84995));
#235188=CARTESIAN_POINT('',(-42.,97.9199999800001,-189.09995));
#235189=CARTESIAN_POINT('Origin',(-42.,97.1699999800001,-189.09995));
#235190=CARTESIAN_POINT('',(-40.5638593383655,97.9199999800001,-189.84995));
#235191=CARTESIAN_POINT('Ctrl Pts',(-42.,97.9199999800001,-189.09995));
#235192=CARTESIAN_POINT('Ctrl Pts',(-41.7587302410591,97.9199999800001,
-189.308895740408));
#235193=CARTESIAN_POINT('Ctrl Pts',(-41.4659359584444,97.9199999800001,
-189.555803560147));
#235194=CARTESIAN_POINT('Ctrl Pts',(-40.9977084033149,97.9199999800001,
-189.783413418928));
#235195=CARTESIAN_POINT('Ctrl Pts',(-40.7653076296235,97.9199999800001,
-189.84995));
#235196=CARTESIAN_POINT('Ctrl Pts',(-40.5638593383655,97.9199999800001,
-189.84995));
#235197=CARTESIAN_POINT('Origin',(-42.,98.9199999800001,-189.84995));
#235198=CARTESIAN_POINT('Origin',(-42.,98.9199999800001,-80.59995));
#235199=CARTESIAN_POINT('',(-42.,97.9199999800001,-80.59995));
#235200=CARTESIAN_POINT('Ctrl Pts',(-41.2284392666181,97.9199999800001,
-80.0295257645779));
#235201=CARTESIAN_POINT('Ctrl Pts',(-41.500014913968,97.9199999800001,-80.1711447838968));
#235202=CARTESIAN_POINT('Ctrl Pts',(-41.7725853995754,97.9199999800001,
-80.4030031788408));
#235203=CARTESIAN_POINT('Ctrl Pts',(-42.,97.9199999800001,-80.59995));
#235204=CARTESIAN_POINT('',(-42.,97.1699999800001,-79.84995));
#235205=CARTESIAN_POINT('Origin',(-42.,97.1699999800001,-80.59995));
#235206=CARTESIAN_POINT('Origin',(-42.,98.9199999800001,-79.84995));
#235207=CARTESIAN_POINT('Origin',(-13.5,-43.9113988480613,-385.453615950046));
#235208=CARTESIAN_POINT('',(-13.5,97.9199999800001,-186.413411979785));
#235209=CARTESIAN_POINT('',(-14.,97.9199999800001,-187.272546484838));
#235210=CARTESIAN_POINT('Origin',(-13.5000000000102,97.9199999800001,-187.272546484832));
#235211=CARTESIAN_POINT('',(-13.5,95.460587505094,-189.84995));
#235212=CARTESIAN_POINT('',(-13.5,91.2935952834256,-195.672489873167));
#235213=CARTESIAN_POINT('',(-14.,96.0754406238205,-189.84995));
#235214=CARTESIAN_POINT('Origin',(-13.4999999999996,96.0754406238209,-189.84995));
#235215=CARTESIAN_POINT('',(-14.,-43.9113988480614,-385.453615950046));
#235216=CARTESIAN_POINT('Origin',(-13.5,-43.9113988480525,115.753715950042));
#235217=CARTESIAN_POINT('',(-14.,97.9199999800001,-82.4273535151615));
#235218=CARTESIAN_POINT('',(-13.5,97.9199999800001,-83.2864880202152));
#235219=CARTESIAN_POINT('Origin',(-13.5000000000003,97.9199999800001,-82.4273535151615));
#235220=CARTESIAN_POINT('',(-14.,96.612189917828,-80.59995));
#235221=CARTESIAN_POINT('',(-14.,-43.9113988480525,115.753715950042));
#235222=CARTESIAN_POINT('',(-13.5,95.6849588822271,-80.1634642136719));
#235223=CARTESIAN_POINT('Ctrl Pts',(-13.5,95.6849588822271,-80.1634642136719));
#235224=CARTESIAN_POINT('Ctrl Pts',(-13.5654616428729,95.6849588822324,
-80.1634642136793));
#235225=CARTESIAN_POINT('Ctrl Pts',(-13.6308739481793,95.7090922288018,
-80.1748247725308));
#235226=CARTESIAN_POINT('Ctrl Pts',(-13.7518094841857,95.8019880554524,
-80.2185546590279));
#235227=CARTESIAN_POINT('Ctrl Pts',(-13.8072733639181,95.8707140107035,
-80.2509067929251));
#235228=CARTESIAN_POINT('Ctrl Pts',(-13.8998334172684,96.0423631189524,
-80.3317090882667));
#235229=CARTESIAN_POINT('Ctrl Pts',(-13.9368931960372,96.1452187774359,
-80.3801274772601));
#235230=CARTESIAN_POINT('Ctrl Pts',(-13.9869863364741,96.3694891476217,
-80.4857007649587));
#235231=CARTESIAN_POINT('Ctrl Pts',(-14.,96.4907937818967,-80.542803845684));
#235232=CARTESIAN_POINT('Ctrl Pts',(-14.,96.612189917828,-80.59995));
#235233=CARTESIAN_POINT('',(-13.5,91.2935952834259,-74.0274101268328));
#235234=CARTESIAN_POINT('Origin',(-14.,-394.08000002,-134.84995));
#235235=CARTESIAN_POINT('',(-14.,97.9199999800001,-134.84995));
#235236=CARTESIAN_POINT('',(-14.,-394.08000002,-80.59995));
#235237=CARTESIAN_POINT('Origin',(-14.,-394.08000002,-134.84995));
#235238=CARTESIAN_POINT('',(-14.,97.9199999800001,-134.84995));
#235239=CARTESIAN_POINT('',(-14.,105.91999998,-189.84995));
#235240=CARTESIAN_POINT('Origin',(-58.,105.91999998,-86.84995));
#235241=CARTESIAN_POINT('',(-58.,97.9199999800001,-182.84995));
#235242=CARTESIAN_POINT('',(-58.,97.1699999800001,-182.84995));
#235243=CARTESIAN_POINT('',(-58.,97.1699999800001,-173.84995));
#235244=CARTESIAN_POINT('',(-58.,94.4199999800001,-182.84995));
#235245=CARTESIAN_POINT('',(-58.,105.91999998,-182.84995));
#235246=CARTESIAN_POINT('',(-58.,94.4199999800001,-86.84995));
#235247=CARTESIAN_POINT('',(-58.,94.4199999800001,-86.84995));
#235248=CARTESIAN_POINT('',(-58.,97.1699999800001,-86.84995));
#235249=CARTESIAN_POINT('',(-58.,105.91999998,-86.84995));
#235250=CARTESIAN_POINT('',(-58.,97.1699999800001,-86.84995));
#235251=CARTESIAN_POINT('Origin',(11.75,97.3100982187845,-189.413464213672));
#235252=CARTESIAN_POINT('',(11.,97.9199999800002,-188.561248242419));
#235253=CARTESIAN_POINT('',(11.,96.9977203019102,-189.84995));
#235254=CARTESIAN_POINT('',(11.,-43.3014970868467,-385.890101736374));
#235255=CARTESIAN_POINT('',(11.75,97.9199999800001,-189.84995));
#235256=CARTESIAN_POINT('Origin',(11.7499999999996,97.9199999800003,-188.56124824242));
#235257=CARTESIAN_POINT('Origin',(11.7499999999998,96.9977203019108,-189.84995));
#235258=CARTESIAN_POINT('Origin',(11.75,97.3100982187848,-80.2864357863281));
#235259=CARTESIAN_POINT('',(11.,97.5344695959176,-80.59995));
#235260=CARTESIAN_POINT('',(11.1688463988223,97.9199999800001,-80.3240391180339));
#235261=CARTESIAN_POINT('Origin',(11.75,97.5344695959176,-80.59995));
#235262=CARTESIAN_POINT('',(11.,97.9199999800001,-81.1386517575809));
#235263=CARTESIAN_POINT('Origin',(11.7500000000205,97.9199999800002,-81.1386517575926));
#235264=CARTESIAN_POINT('',(11.,-43.3014970868374,116.19020173637));
#235265=CARTESIAN_POINT('Origin',(11.75,97.5344695959176,-80.59995));
#235266=CARTESIAN_POINT('',(11.75,97.5344695959176,-79.84995));
#235267=CARTESIAN_POINT('',(11.75,97.9199999800001,-79.9566255694448));
#235268=CARTESIAN_POINT('Origin',(11.75,97.5344695959176,-80.59995));
#235269=CARTESIAN_POINT('Origin',(11.75,97.9199999800001,-80.59995));
#235270=CARTESIAN_POINT('Origin',(11.75,97.5344695959176,-80.59995));
#235271=CARTESIAN_POINT('Origin',(-51.,97.5344695959176,-80.59995));
#235272=CARTESIAN_POINT('',(37.9309791607343,97.5344695959176,-79.84995));
#235273=CARTESIAN_POINT('',(37.9309791607343,97.9199999800001,-79.9566255694448));
#235274=CARTESIAN_POINT('Origin',(37.9309791607343,97.5344695959176,-80.59995));
#235275=CARTESIAN_POINT('',(-51.,97.9199999800001,-79.9566255694448));
#235276=CARTESIAN_POINT('',(-51.,97.5344695959176,-79.84995));
#235277=CARTESIAN_POINT('Origin',(37.9309791607343,97.5344695959176,-80.59995));
#235278=CARTESIAN_POINT('',(38.2284392666181,97.9199999800001,-80.0295257645779));
#235279=CARTESIAN_POINT('Origin',(37.9309791607343,97.5344695959176,-80.59995));
#235280=CARTESIAN_POINT('Origin',(37.9309791607343,97.9199999800001,-80.59995));
#235281=CARTESIAN_POINT('Origin',(54.25,98.9199999800001,-173.84995));
#235282=CARTESIAN_POINT('',(55.,97.1699999800001,-173.84995));
#235283=CARTESIAN_POINT('',(54.25,97.9199999800001,-173.84995));
#235284=CARTESIAN_POINT('Origin',(54.25,97.1699999800001,-173.84995));
#235285=CARTESIAN_POINT('',(54.8072469207768,97.9199999800001,-173.103241263434));
#235286=CARTESIAN_POINT('Ctrl Pts',(54.25,97.9199999800001,-173.84995));
#235287=CARTESIAN_POINT('Ctrl Pts',(54.4409434098567,97.9199999800001,-173.629467541839));
#235288=CARTESIAN_POINT('Ctrl Pts',(54.6651860234659,97.9199999800001,-173.36682332955));
#235289=CARTESIAN_POINT('Ctrl Pts',(54.8072469207768,97.9199999800001,-173.103241263434));
#235290=CARTESIAN_POINT('',(55.,97.5177878719661,-172.802905968413));
#235291=CARTESIAN_POINT('Origin',(54.25,97.5177878719661,-172.802905968413));
#235292=CARTESIAN_POINT('Origin',(55.,98.9199999800001,-173.84995));
#235293=CARTESIAN_POINT('Origin',(54.25,97.5177878719661,-172.802905968413));
#235294=CARTESIAN_POINT('',(54.8822667063023,97.9199999800001,-172.833958057747));
#235295=CARTESIAN_POINT('Origin',(54.25,97.9199999800001,-172.802905968413));
#235296=CARTESIAN_POINT('Origin',(54.25,97.5177878719661,-172.802905968413));
#235297=CARTESIAN_POINT('Origin',(54.25,-394.08000002,-134.84995));
#235298=CARTESIAN_POINT('',(55.,97.9199999800001,-167.173500656049));
#235299=CARTESIAN_POINT('Ctrl Pts',(54.8822667063024,97.9199999800001,-172.833958057747));
#235300=CARTESIAN_POINT('Ctrl Pts',(54.9005229085552,97.9199999800001,-172.462234637024));
#235301=CARTESIAN_POINT('Ctrl Pts',(54.9159202399799,97.9199999800001,-172.088208331578));
#235302=CARTESIAN_POINT('Ctrl Pts',(54.9835908722536,97.9199999800001,-170.15643772184));
#235303=CARTESIAN_POINT('Ctrl Pts',(55.,97.9199999800002,-168.594527486982));
#235304=CARTESIAN_POINT('Ctrl Pts',(55.,97.9199999800002,-167.173500656049));
#235305=CARTESIAN_POINT('Origin',(55.,-394.08000002,-134.84995));
#235306=CARTESIAN_POINT('Origin',(54.25,-394.08000002,-134.84995));
#235307=CARTESIAN_POINT('',(55.,97.9199999800001,-102.526399343951));
#235308=CARTESIAN_POINT('',(55.,97.5177878719661,-96.8969940315874));
#235309=CARTESIAN_POINT('Origin',(55.,-394.08000002,-134.84995));
#235310=CARTESIAN_POINT('',(54.8822667063027,97.9199999800001,-96.8659419422532));
#235311=CARTESIAN_POINT('Ctrl Pts',(55.,97.9199999800002,-102.526399343951));
#235312=CARTESIAN_POINT('Ctrl Pts',(55.,97.9199999800002,-101.105372513018));
#235313=CARTESIAN_POINT('Ctrl Pts',(54.9835908722536,97.9199999800001,-99.5434622781595));
#235314=CARTESIAN_POINT('Ctrl Pts',(54.9159202399799,97.9199999800001,-97.6116916684221));
#235315=CARTESIAN_POINT('Ctrl Pts',(54.9005229085552,97.9199999800001,-97.2376653629761));
#235316=CARTESIAN_POINT('Ctrl Pts',(54.8822667063024,97.9199999800001,-96.8659419422532));
#235317=CARTESIAN_POINT('Origin',(54.25,97.5177878719661,-96.8969940315874));
#235318=CARTESIAN_POINT('Origin',(54.25,97.5177878719661,-96.8969940315875));
#235319=CARTESIAN_POINT('',(54.8072469207768,97.9199999800001,-96.5966587365659));
#235320=CARTESIAN_POINT('Origin',(54.25,97.9199999800001,-96.8969940315875));
#235321=CARTESIAN_POINT('Origin',(54.25,97.5177878719662,-96.8969940315876));
#235322=CARTESIAN_POINT('Origin',(54.25,98.9199999800001,-95.84995));
#235323=CARTESIAN_POINT('',(54.25,97.9199999800001,-95.84995));
#235324=CARTESIAN_POINT('Ctrl Pts',(54.8072469207768,97.9199999800001,-96.5966587365659));
#235325=CARTESIAN_POINT('Ctrl Pts',(54.6651860234659,97.9199999800001,-96.3330766704501));
#235326=CARTESIAN_POINT('Ctrl Pts',(54.4409434098566,97.9199999800001,-96.0704324581614));
#235327=CARTESIAN_POINT('Ctrl Pts',(54.25,97.9199999800001,-95.84995));
#235328=CARTESIAN_POINT('',(55.,97.1699999800001,-95.84995));
#235329=CARTESIAN_POINT('Origin',(54.25,97.1699999800001,-95.84995));
#235330=CARTESIAN_POINT('Origin',(55.,98.9199999800001,-95.84995));
#235331=CARTESIAN_POINT('Origin',(39.,98.9199999800001,-189.09995));
#235332=CARTESIAN_POINT('',(37.5638593383657,97.9199999800001,-189.84995));
#235333=CARTESIAN_POINT('',(39.,97.1699999800001,-189.84995));
#235334=CARTESIAN_POINT('Origin',(39.,98.9199999800001,-189.84995));
#235335=CARTESIAN_POINT('',(39.,97.9199999800001,-189.09995));
#235336=CARTESIAN_POINT('Ctrl Pts',(37.5638593383655,97.9199999800001,-189.84995));
#235337=CARTESIAN_POINT('Ctrl Pts',(37.7653076296235,97.9199999800001,-189.84995));
#235338=CARTESIAN_POINT('Ctrl Pts',(37.9977084033149,97.9199999800001,-189.783413418928));
#235339=CARTESIAN_POINT('Ctrl Pts',(38.4659359584444,97.9199999800001,-189.555803560147));
#235340=CARTESIAN_POINT('Ctrl Pts',(38.7587302410591,97.9199999800001,-189.308895740408));
#235341=CARTESIAN_POINT('Ctrl Pts',(39.,97.9199999800001,-189.09995));
#235342=CARTESIAN_POINT('Origin',(39.,97.1699999800001,-189.09995));
#235343=CARTESIAN_POINT('Origin',(39.,98.9199999800001,-80.59995));
#235344=CARTESIAN_POINT('',(39.,97.9199999800001,-80.59995));
#235345=CARTESIAN_POINT('',(39.,97.1699999800001,-79.84995));
#235346=CARTESIAN_POINT('Origin',(39.,97.1699999800001,-80.59995));
#235347=CARTESIAN_POINT('Ctrl Pts',(39.,97.9199999800001,-80.59995));
#235348=CARTESIAN_POINT('Ctrl Pts',(38.7725853995754,97.9199999800001,-80.4030031788408));
#235349=CARTESIAN_POINT('Ctrl Pts',(38.5000149139681,97.9199999800001,-80.1711447838968));
#235350=CARTESIAN_POINT('Ctrl Pts',(38.2284392666181,97.9199999800001,-80.0295257645779));
#235351=CARTESIAN_POINT('Origin',(39.,98.9199999800001,-79.84995));
#235352=CARTESIAN_POINT('Origin',(10.5,-43.9113988480613,-385.453615950046));
#235353=CARTESIAN_POINT('',(11.,97.9199999800001,-187.272546484838));
#235354=CARTESIAN_POINT('',(10.5,97.9199999800001,-186.413411979785));
#235355=CARTESIAN_POINT('Origin',(10.5000000000105,97.9199999800001,-187.272546484831));
#235356=CARTESIAN_POINT('',(11.,96.0754406238205,-189.84995));
#235357=CARTESIAN_POINT('',(11.,-43.9113988480614,-385.453615950046));
#235358=CARTESIAN_POINT('',(10.5,95.460587505094,-189.84995));
#235359=CARTESIAN_POINT('Origin',(10.4999999999996,96.0754406238209,-189.84995));
#235360=CARTESIAN_POINT('',(10.5,91.2935952834256,-195.672489873167));
#235361=CARTESIAN_POINT('Origin',(10.5,-43.9113988480525,115.753715950042));
#235362=CARTESIAN_POINT('',(10.5,97.9199999800001,-83.2864880202152));
#235363=CARTESIAN_POINT('',(11.,97.9199999800001,-82.4273535151615));
#235364=CARTESIAN_POINT('Origin',(10.5,97.9199999800001,-82.427353515161));
#235365=CARTESIAN_POINT('',(10.5,95.6849588822271,-80.1634642136719));
#235366=CARTESIAN_POINT('',(10.5,91.2935952834259,-74.0274101268328));
#235367=CARTESIAN_POINT('',(11.,96.612189917828,-80.59995));
#235368=CARTESIAN_POINT('Ctrl Pts',(10.5,95.6849588822271,-80.1634642136719));
#235369=CARTESIAN_POINT('Ctrl Pts',(10.5156818609759,95.6849588822271,-80.163464213672));
#235370=CARTESIAN_POINT('Ctrl Pts',(10.5313200885977,95.6863393578606,-80.1641136250356));
#235371=CARTESIAN_POINT('Ctrl Pts',(10.5469160042521,95.6890782080141,-80.1654023178236));
#235372=CARTESIAN_POINT('Ctrl Pts',(10.5625645383606,95.6918262986678,-80.1666953584821));
#235373=CARTESIAN_POINT('Ctrl Pts',(10.5781708749757,95.6959420414388,-80.1686320420268));
#235374=CARTESIAN_POINT('Ctrl Pts',(10.5937322749933,95.7014506402686,-80.171224518524));
#235375=CARTESIAN_POINT('Ctrl Pts',(10.6092044253496,95.7069276455028,-80.1738021263301));
#235376=CARTESIAN_POINT('Ctrl Pts',(10.6246325584921,95.7137816788003,-80.1770280703136));
#235377=CARTESIAN_POINT('Ctrl Pts',(10.6400039678108,95.7220828322891,-80.1809357042478));
#235378=CARTESIAN_POINT('Ctrl Pts',(10.6547456182153,95.7300438916917,-80.1846832443837));
#235379=CARTESIAN_POINT('Ctrl Pts',(10.6694353917173,95.7393362069862,-80.1890578912298));
#235380=CARTESIAN_POINT('Ctrl Pts',(10.6840479045028,95.7500602195997,-80.1941073705498));
#235381=CARTESIAN_POINT('Ctrl Pts',(10.6864825086507,95.7518469571701,-80.1949486689273));
#235382=CARTESIAN_POINT('Ctrl Pts',(10.6889141998357,95.753672947647,-80.1958084301768));
#235383=CARTESIAN_POINT('Ctrl Pts',(10.6913425626005,95.7555384804021,-80.1966867914439));
#235384=CARTESIAN_POINT('Ctrl Pts',(10.7116040791809,95.7711039154339,-80.2040155693498));
#235385=CARTESIAN_POINT('Ctrl Pts',(10.7316297878809,95.7894211341418,-80.2126387195569));
#235386=CARTESIAN_POINT('Ctrl Pts',(10.7511868500182,95.8105123565252,-80.222567351155));
#235387=CARTESIAN_POINT('Ctrl Pts',(10.7583837688949,95.8182738400976,-80.2262210469743));
#235388=CARTESIAN_POINT('Ctrl Pts',(10.7655169157189,95.826410619207,-80.2300513643091));
#235389=CARTESIAN_POINT('Ctrl Pts',(10.772573602495,95.8349225100514,-80.2340582614315));
#235390=CARTESIAN_POINT('Ctrl Pts',(10.7920381169864,95.8584009253402,-80.2451105171968));
#235391=CARTESIAN_POINT('Ctrl Pts',(10.8109248100544,95.8847366103483,-80.2575078073411));
#235392=CARTESIAN_POINT('Ctrl Pts',(10.82895296563,95.9139165491847,-80.2712440047493));
#235393=CARTESIAN_POINT('Ctrl Pts',(10.8307439624858,95.9168154136021,-80.2726086194636));
#235394=CARTESIAN_POINT('Ctrl Pts',(10.8325264536709,95.9197423235926,-80.2739864363826));
#235395=CARTESIAN_POINT('Ctrl Pts',(10.834300140239,95.9226972461615,-80.2753774399745));
#235396=CARTESIAN_POINT('Ctrl Pts',(10.8371855095635,95.9275042075999,-80.2776402744384));
#235397=CARTESIAN_POINT('Ctrl Pts',(10.8402295435766,95.9326948651965,-80.2800837305874));
#235398=CARTESIAN_POINT('Ctrl Pts',(10.8431864058672,95.9378670615211,-80.2825184800336));
#235399=CARTESIAN_POINT('Ctrl Pts',(10.8462781372091,95.9432751731987,-80.2850642838054));
#235400=CARTESIAN_POINT('Ctrl Pts',(10.8492744231064,95.9486629966847,-80.2876005193099));
#235401=CARTESIAN_POINT('Ctrl Pts',(10.851919307303,95.9535221815782,-80.2898878650167));
#235402=CARTESIAN_POINT('Ctrl Pts',(10.8524805367969,95.9545532731783,-80.2903732268616));
#235403=CARTESIAN_POINT('Ctrl Pts',(10.8530260296046,95.9555604073977,-80.2908473092743));
#235404=CARTESIAN_POINT('Ctrl Pts',(10.8535534680192,95.956538501865,-80.2913077195793));
#235405=CARTESIAN_POINT('Ctrl Pts',(10.8649452601285,95.9776637148284,-80.3012518160527));
#235406=CARTESIAN_POINT('Ctrl Pts',(10.8761385017745,96.0004894960687,-80.3119968950234));
#235407=CARTESIAN_POINT('Ctrl Pts',(10.8869673939531,96.0250580069767,-80.3235624691653));
#235408=CARTESIAN_POINT('Ctrl Pts',(10.896634247271,96.0469900926667,-80.3338869517554));
#235409=CARTESIAN_POINT('Ctrl Pts',(10.9060105373242,96.0703106233711,-80.3448651281021));
#235410=CARTESIAN_POINT('Ctrl Pts',(10.9149649031813,96.0950201938376,-80.3564969392479));
#235411=CARTESIAN_POINT('Ctrl Pts',(10.9252600821156,96.123429737674,-80.3698704800424));
#235412=CARTESIAN_POINT('Ctrl Pts',(10.9350002950485,96.1536806995305,-80.384110852038));
#235413=CARTESIAN_POINT('Ctrl Pts',(10.9439706013777,96.1857608028677,-80.3992122761633));
#235414=CARTESIAN_POINT('Ctrl Pts',(10.9503835439419,96.2086951211178,-80.4100084030734));
#235415=CARTESIAN_POINT('Ctrl Pts',(10.9564026291807,96.2325638261801,-80.4212443842883));
#235416=CARTESIAN_POINT('Ctrl Pts',(10.9619397662556,96.2573539625288,-80.4329141211094));
#235417=CARTESIAN_POINT('Ctrl Pts',(10.9620475507384,96.2578365209317,-80.4331412811977));
#235418=CARTESIAN_POINT('Ctrl Pts',(10.9621551520677,96.2583194268068,-80.4333686048555));
#235419=CARTESIAN_POINT('Ctrl Pts',(10.9622625697312,96.2588026800681,-80.4335960920423));
#235420=CARTESIAN_POINT('Ctrl Pts',(10.9629080222422,96.2617064579087,-80.434963019707));
#235421=CARTESIAN_POINT('Ctrl Pts',(10.9637502581113,96.265559008235,-80.4367764944774));
#235422=CARTESIAN_POINT('Ctrl Pts',(10.9643453109648,96.2683234584993,-80.4380777533962));
#235423=CARTESIAN_POINT('Ctrl Pts',(10.9645704310761,96.2693693040028,-80.4385700450488));
#235424=CARTESIAN_POINT('Ctrl Pts',(10.9647607130506,96.270259013439,-80.4389888367266));
#235425=CARTESIAN_POINT('Ctrl Pts',(10.9648934963716,96.2708812896082,-80.4392817405416));
#235426=CARTESIAN_POINT('Ctrl Pts',(10.9684360128225,96.287482949737,-80.4470960998693));
#235427=CARTESIAN_POINT('Ctrl Pts',(10.9721210866807,96.306152102166,-80.4558840299471));
#235428=CARTESIAN_POINT('Ctrl Pts',(10.9757459570284,96.3269794923422,-80.4656881571978));
#235429=CARTESIAN_POINT('Ctrl Pts',(10.978979634052,96.3455592059914,-80.4744342302948));
#235430=CARTESIAN_POINT('Ctrl Pts',(10.9821648967382,96.3658572091196,-80.4839893529887));
#235431=CARTESIAN_POINT('Ctrl Pts',(10.9851264759707,96.3879150163117,-80.4943729948297));
#235432=CARTESIAN_POINT('Ctrl Pts',(10.9879212507746,96.4087304660878,-80.5041718009102));
#235433=CARTESIAN_POINT('Ctrl Pts',(10.9905166776936,96.4311137231632,-80.5147087337626));
#235434=CARTESIAN_POINT('Ctrl Pts',(10.9927398924504,96.4550683413436,-80.5259853943057));
#235435=CARTESIAN_POINT('Ctrl Pts',(10.9949001524002,96.478344636227,-80.5369427334761));
#235436=CARTESIAN_POINT('Ctrl Pts',(10.9967089624194,96.5031052705477,-80.5485988343262));
#235437=CARTESIAN_POINT('Ctrl Pts',(10.9979838985217,96.529313066776,-80.5609361188393));
#235438=CARTESIAN_POINT('Ctrl Pts',(10.9991586792015,96.5534620516668,-80.5723042207089));
#235439=CARTESIAN_POINT('Ctrl Pts',(10.9998799817883,96.5788399156019,-80.5842507595581));
#235440=CARTESIAN_POINT('Ctrl Pts',(10.9999863449063,96.6053774356702,-80.5967430818542));
#235441=CARTESIAN_POINT('Ctrl Pts',(10.9999954128483,96.6076398805487,-80.5978081094274));
#235442=CARTESIAN_POINT('Ctrl Pts',(11.,96.6099107273809,-80.5988770913113));
#235443=CARTESIAN_POINT('Ctrl Pts',(11.,96.612189917828,-80.59995));
#235444=CARTESIAN_POINT('',(11.,-43.9113988480525,115.753715950042));
#235445=CARTESIAN_POINT('Origin',(11.,-394.08000002,-134.84995));
#235446=CARTESIAN_POINT('',(11.,97.9199999800001,-134.84995));
#235447=CARTESIAN_POINT('',(11.,105.91999998,-189.84995));
#235448=CARTESIAN_POINT('Origin',(11.,-394.08000002,-134.84995));
#235449=CARTESIAN_POINT('',(11.,97.9199999800001,-134.84995));
#235450=CARTESIAN_POINT('',(11.,-394.08000002,-80.59995));
#235451=CARTESIAN_POINT('Origin',(-14.,91.2935952834256,-195.672489873167));
#235452=CARTESIAN_POINT('',(-14.,97.9199999800001,-186.413411979785));
#235453=CARTESIAN_POINT('',(48.,95.460587505094,-189.84995));
#235454=CARTESIAN_POINT('Origin',(-14.,91.2935952834259,-74.0274101268328));
#235455=CARTESIAN_POINT('',(-14.,97.9199999800001,-83.2864880202152));
#235456=CARTESIAN_POINT('',(10.5,95.6849588822271,-80.1634642136719));
#235457=CARTESIAN_POINT('Origin',(55.,105.91999998,-86.84995));
#235458=CARTESIAN_POINT('',(55.,97.9199999800001,-86.84995));
#235459=CARTESIAN_POINT('',(55.,97.1699999800001,-86.84995));
#235460=CARTESIAN_POINT('',(55.,97.1699999800001,-86.84995));
#235461=CARTESIAN_POINT('',(55.,94.4199999800001,-86.84995));
#235462=CARTESIAN_POINT('',(55.,105.91999998,-86.84995));
#235463=CARTESIAN_POINT('',(55.,94.4199999800001,-182.84995));
#235464=CARTESIAN_POINT('',(55.,94.4199999800001,-86.84995));
#235465=CARTESIAN_POINT('',(55.,97.1699999800001,-182.84995));
#235466=CARTESIAN_POINT('',(55.,105.91999998,-182.84995));
#235467=CARTESIAN_POINT('',(55.,97.1699999800001,-173.84995));
#235468=CARTESIAN_POINT('Origin',(-14.75,105.91999998,-80.59995));
#235469=CARTESIAN_POINT('',(-14.75,96.612189917828,-79.84995));
#235470=CARTESIAN_POINT('Origin',(-14.75,96.612189917828,-80.59995));
#235471=CARTESIAN_POINT('',(-14.75,105.91999998,-79.84995));
#235472=CARTESIAN_POINT('Ctrl Pts',(-14.75,96.612189917828,-79.84995));
#235473=CARTESIAN_POINT('Ctrl Pts',(-14.,96.612189917828,-79.84995));
#235474=CARTESIAN_POINT('Ctrl Pts',(-14.,96.612189917828,-80.59995));
#235475=CARTESIAN_POINT('Ctrl Pts',(-14.7499999999888,96.4109434379512,
-79.84995));
#235476=CARTESIAN_POINT('Ctrl Pts',(-14.0551300101178,96.4950766906307,
-79.8499500000001));
#235477=CARTESIAN_POINT('Ctrl Pts',(-14.,96.4907937818967,-80.542803845684));
#235478=CARTESIAN_POINT('Ctrl Pts',(-14.717465841188,96.2098486464843,-79.84995));
#235479=CARTESIAN_POINT('Ctrl Pts',(-14.087399369873,96.3554456062245,-79.8499500000001));
#235480=CARTESIAN_POINT('Ctrl Pts',(-13.9869863364741,96.3694891476217,
-80.4857007649587));
#235481=CARTESIAN_POINT('Ctrl Pts',(-14.5922329900902,95.8380606797986,
-79.84995));
#235482=CARTESIAN_POINT('Ctrl Pts',(-14.0888617253033,96.0821031793196,
-79.84995));
#235483=CARTESIAN_POINT('Ctrl Pts',(-13.9368931960372,96.1452187774359,
-80.3801274772601));
#235484=CARTESIAN_POINT('Ctrl Pts',(-14.4995835431726,95.6675499872971,
-79.84995));
#235485=CARTESIAN_POINT('Ctrl Pts',(-14.0613642943088,95.9469647180508,
-79.84995));
#235486=CARTESIAN_POINT('Ctrl Pts',(-13.8998334172684,96.0423631189524,
-80.3317090882667));
#235487=CARTESIAN_POINT('Ctrl Pts',(-14.2681834097938,95.3829957999329,
-79.84995));
#235488=CARTESIAN_POINT('Ctrl Pts',(-13.956965021564,95.7189955144651,-79.8499500000001));
#235489=CARTESIAN_POINT('Ctrl Pts',(-13.8072733639181,95.8707140107035,
-80.2509067929251));
#235490=CARTESIAN_POINT('Ctrl Pts',(-14.129523710464,95.2690641952365,-79.84995));
#235491=CARTESIAN_POINT('Ctrl Pts',(-13.8811942932893,95.6232014564904,
-79.8499499999988));
#235492=CARTESIAN_POINT('Ctrl Pts',(-13.7518094841857,95.8019880554524,
-80.2185546590279));
#235493=CARTESIAN_POINT('Ctrl Pts',(-13.8271848704487,95.1150645809588,
-79.84995));
#235494=CARTESIAN_POINT('Ctrl Pts',(-13.7038891791878,95.49503291722,-79.8499500000011));
#235495=CARTESIAN_POINT('Ctrl Pts',(-13.6308739481793,95.7090922288018,
-80.1748247725308));
#235496=CARTESIAN_POINT('Ctrl Pts',(-13.6636541071819,95.0750571210368,
-79.84995));
#235497=CARTESIAN_POINT('Ctrl Pts',(-13.6016004447884,95.4605875051159,
-79.84995));
#235498=CARTESIAN_POINT('Ctrl Pts',(-13.5654616428729,95.6849588822324,
-80.1634642136793));
#235499=CARTESIAN_POINT('Ctrl Pts',(-13.5,95.0750571210118,-79.84995));
#235500=CARTESIAN_POINT('Ctrl Pts',(-13.5,95.4605875050944,-79.84995));
#235501=CARTESIAN_POINT('Ctrl Pts',(-13.5,95.6849588822271,-80.1634642136719));
#235502=CARTESIAN_POINT('',(-13.5,95.0750571210118,-79.84995));
#235503=CARTESIAN_POINT('Origin',(-13.5,95.0750571210117,-80.59995));
#235504=CARTESIAN_POINT('Ctrl Pts',(-14.75,96.612189917828,-79.84995));
#235505=CARTESIAN_POINT('Ctrl Pts',(-14.7499999999888,96.4109434379512,
-79.84995));
#235506=CARTESIAN_POINT('Ctrl Pts',(-14.717465841188,96.2098486464843,-79.84995));
#235507=CARTESIAN_POINT('Ctrl Pts',(-14.5922329900902,95.8380606797986,
-79.84995));
#235508=CARTESIAN_POINT('Ctrl Pts',(-14.4995835431726,95.6675499872971,
-79.84995));
#235509=CARTESIAN_POINT('Ctrl Pts',(-14.2681834097938,95.3829957999329,
-79.84995));
#235510=CARTESIAN_POINT('Ctrl Pts',(-14.129523710464,95.2690641952365,-79.84995));
#235511=CARTESIAN_POINT('Ctrl Pts',(-13.8271848704487,95.1150645809588,
-79.84995));
#235512=CARTESIAN_POINT('Ctrl Pts',(-13.6636541071819,95.0750571210368,
-79.84995));
#235513=CARTESIAN_POINT('Ctrl Pts',(-13.5,95.0750571210118,-79.84995));
#235514=CARTESIAN_POINT('Origin',(-57.25,97.1699999800001,-86.84995));
#235515=CARTESIAN_POINT('',(-57.25,97.9199999800001,-182.84995));
#235516=CARTESIAN_POINT('Origin',(-57.25,97.1699999800001,-182.84995));
#235517=CARTESIAN_POINT('',(-57.25,97.9199999800001,-182.84995));
#235518=CARTESIAN_POINT('Origin',(-51.,97.1699999800001,-182.84995));
#235519=CARTESIAN_POINT('',(-51.,97.1699999800001,-189.84995));
#235520=CARTESIAN_POINT('',(-51.,97.9199999800001,-189.09995));
#235521=CARTESIAN_POINT('Origin',(-51.,97.1699999800001,-189.09995));
#235522=CARTESIAN_POINT('Origin',(-51.,97.1699999800001,-182.84995));
#235523=CARTESIAN_POINT('Origin',(-51.,97.9199999800001,-182.84995));
#235524=CARTESIAN_POINT('Origin',(-51.,97.1699999800001,-189.09995));
#235525=CARTESIAN_POINT('',(-51.,97.1699999800001,-189.84995));
#235526=CARTESIAN_POINT('',(-42.,97.9199999800001,-189.09995));
#235527=CARTESIAN_POINT('Origin',(-57.25,97.1699999800001,-86.84995));
#235528=CARTESIAN_POINT('',(-57.25,97.9199999800001,-86.84995));
#235529=CARTESIAN_POINT('Origin',(-57.25,97.1699999800001,-86.84995));
#235530=CARTESIAN_POINT('',(-57.25,97.9199999800001,-89.84995));
#235531=CARTESIAN_POINT('Origin',(-51.,97.1699999800001,-86.84995));
#235532=CARTESIAN_POINT('',(-51.,97.9199999800001,-80.59995));
#235533=CARTESIAN_POINT('',(-51.,97.1699999800001,-79.84995));
#235534=CARTESIAN_POINT('Origin',(-51.,97.1699999800001,-80.59995));
#235535=CARTESIAN_POINT('Origin',(-51.,97.9199999800001,-86.84995));
#235536=CARTESIAN_POINT('Origin',(-51.,97.1699999800001,-86.84995));
#235537=CARTESIAN_POINT('Origin',(48.,97.1699999800001,-80.59995));
#235538=CARTESIAN_POINT('',(-48.,97.9199999800001,-80.59995));
#235539=CARTESIAN_POINT('',(48.,97.1699999800001,-79.84995));
#235540=CARTESIAN_POINT('Origin',(-51.,105.91999998,-86.84995));
#235541=CARTESIAN_POINT('',(-51.,94.4199999800001,-79.84995));
#235542=CARTESIAN_POINT('Origin',(-51.,94.4199999800001,-86.84995));
#235543=CARTESIAN_POINT('',(-51.,105.91999998,-79.84995));
#235544=CARTESIAN_POINT('Origin',(-51.,105.91999998,-182.84995));
#235545=CARTESIAN_POINT('',(-51.,94.4199999800001,-189.84995));
#235546=CARTESIAN_POINT('Origin',(-51.,94.4199999800001,-182.84995));
#235547=CARTESIAN_POINT('',(-51.,105.91999998,-189.84995));
#235548=CARTESIAN_POINT('Origin',(55.01,94.4199999800001,-52.64995));
#235549=CARTESIAN_POINT('',(48.,94.4199999800001,-189.84995));
#235550=CARTESIAN_POINT('',(48.,94.4199999800001,-189.84995));
#235551=CARTESIAN_POINT('Origin',(48.,94.4199999800001,-182.84995));
#235552=CARTESIAN_POINT('',(48.,94.4199999800001,-79.84995));
#235553=CARTESIAN_POINT('Origin',(48.,94.4199999800001,-86.84995));
#235554=CARTESIAN_POINT('',(-51.,94.4199999800001,-79.84995));
#235555=CARTESIAN_POINT('Origin',(11.75,105.91999998,-80.59995));
#235556=CARTESIAN_POINT('',(11.75,96.612189917828,-79.84995));
#235557=CARTESIAN_POINT('Origin',(11.75,96.612189917828,-80.59995));
#235558=CARTESIAN_POINT('',(11.75,105.91999998,-79.84995));
#235559=CARTESIAN_POINT('Ctrl Pts',(11.,96.612189917828,-80.59995));
#235560=CARTESIAN_POINT('Ctrl Pts',(11.,96.6121899178279,-79.8499500000001));
#235561=CARTESIAN_POINT('Ctrl Pts',(11.75,96.612189917828,-79.84995));
#235562=CARTESIAN_POINT('Ctrl Pts',(11.,96.4907937818966,-80.542803845684));
#235563=CARTESIAN_POINT('Ctrl Pts',(11.0551300101177,96.4950766906306,-79.8499500000013));
#235564=CARTESIAN_POINT('Ctrl Pts',(11.7499999999888,96.4109434379512,-79.84995));
#235565=CARTESIAN_POINT('Ctrl Pts',(10.9869863364741,96.3694891476217,-80.4857007649587));
#235566=CARTESIAN_POINT('Ctrl Pts',(11.087399369873,96.3554456062245,-79.8499500000001));
#235567=CARTESIAN_POINT('Ctrl Pts',(11.717465841188,96.2098486464843,-79.84995));
#235568=CARTESIAN_POINT('Ctrl Pts',(10.9368931960372,96.1452187774359,-80.3801274772601));
#235569=CARTESIAN_POINT('Ctrl Pts',(11.0888617253033,96.0821031793196,-79.84995));
#235570=CARTESIAN_POINT('Ctrl Pts',(11.5922329900902,95.8380606797986,-79.84995));
#235571=CARTESIAN_POINT('Ctrl Pts',(10.8998334172684,96.0423631189524,-80.3317090882667));
#235572=CARTESIAN_POINT('Ctrl Pts',(11.061364294309,95.9469647180509,-79.84995));
#235573=CARTESIAN_POINT('Ctrl Pts',(11.4995835431726,95.6675499872971,-79.84995));
#235574=CARTESIAN_POINT('Ctrl Pts',(10.8072733639181,95.8707140107035,-80.2509067929251));
#235575=CARTESIAN_POINT('Ctrl Pts',(10.9569650215639,95.7189955144651,-79.84995));
#235576=CARTESIAN_POINT('Ctrl Pts',(11.2681834097938,95.3829957999329,-79.84995));
#235577=CARTESIAN_POINT('Ctrl Pts',(10.7518094841857,95.8019880554524,-80.2185546590279));
#235578=CARTESIAN_POINT('Ctrl Pts',(10.8811942932896,95.6232014564902,-79.8499499999989));
#235579=CARTESIAN_POINT('Ctrl Pts',(11.129523710464,95.2690641952365,-79.84995));
#235580=CARTESIAN_POINT('Ctrl Pts',(10.6308739481793,95.7090922288018,-80.1748247725308));
#235581=CARTESIAN_POINT('Ctrl Pts',(10.7038891791875,95.4950329172199,-79.8499500000012));
#235582=CARTESIAN_POINT('Ctrl Pts',(10.8271848704487,95.1150645809588,-79.84995));
#235583=CARTESIAN_POINT('Ctrl Pts',(10.5654616428729,95.6849588822324,-80.1634642136793));
#235584=CARTESIAN_POINT('Ctrl Pts',(10.6016004447886,95.4605875051159,-79.84995));
#235585=CARTESIAN_POINT('Ctrl Pts',(10.6636541071819,95.0750571210368,-79.84995));
#235586=CARTESIAN_POINT('Ctrl Pts',(10.5,95.6849588822271,-80.1634642136719));
#235587=CARTESIAN_POINT('Ctrl Pts',(10.5,95.4605875050944,-79.84995));
#235588=CARTESIAN_POINT('Ctrl Pts',(10.5,95.0750571210118,-79.84995));
#235589=CARTESIAN_POINT('',(10.5,95.0750571210118,-79.84995));
#235590=CARTESIAN_POINT('Origin',(10.5,95.0750571210117,-80.59995));
#235591=CARTESIAN_POINT('Ctrl Pts',(11.75,96.612189917828,-79.84995));
#235592=CARTESIAN_POINT('Ctrl Pts',(11.7499999999888,96.4109434379512,-79.84995));
#235593=CARTESIAN_POINT('Ctrl Pts',(11.717465841188,96.2098486464843,-79.84995));
#235594=CARTESIAN_POINT('Ctrl Pts',(11.5922329900902,95.8380606797986,-79.84995));
#235595=CARTESIAN_POINT('Ctrl Pts',(11.4995835431726,95.6675499872971,-79.84995));
#235596=CARTESIAN_POINT('Ctrl Pts',(11.2681834097938,95.3829957999329,-79.84995));
#235597=CARTESIAN_POINT('Ctrl Pts',(11.129523710464,95.2690641952365,-79.84995));
#235598=CARTESIAN_POINT('Ctrl Pts',(10.8271848704487,95.1150645809588,-79.84995));
#235599=CARTESIAN_POINT('Ctrl Pts',(10.6636541071819,95.0750571210368,-79.84995));
#235600=CARTESIAN_POINT('Ctrl Pts',(10.5,95.0750571210118,-79.84995));
#235601=CARTESIAN_POINT('Origin',(-14.,95.0750571210117,-80.59995));
#235602=CARTESIAN_POINT('',(-1.5,95.0750571210117,-79.84995));
#235603=CARTESIAN_POINT('Origin',(54.25,97.1699999800001,-86.84995));
#235604=CARTESIAN_POINT('',(54.25,97.9199999800001,-182.84995));
#235605=CARTESIAN_POINT('Origin',(54.25,97.1699999800001,-182.84995));
#235606=CARTESIAN_POINT('',(54.25,97.9199999800001,-182.84995));
#235607=CARTESIAN_POINT('Origin',(48.,97.1699999800001,-182.84995));
#235608=CARTESIAN_POINT('',(48.,97.1699999800001,-189.84995));
#235609=CARTESIAN_POINT('',(48.,97.9199999800001,-189.09995));
#235610=CARTESIAN_POINT('Origin',(48.,97.1699999800001,-189.09995));
#235611=CARTESIAN_POINT('Origin',(48.,97.9199999800001,-182.84995));
#235612=CARTESIAN_POINT('Origin',(48.,97.1699999800001,-182.84995));
#235613=CARTESIAN_POINT('Origin',(48.,97.1699999800001,-189.09995));
#235614=CARTESIAN_POINT('',(39.,97.9199999800001,-189.09995));
#235615=CARTESIAN_POINT('',(48.,97.1699999800001,-189.84995));
#235616=CARTESIAN_POINT('Origin',(54.25,97.1699999800001,-86.84995));
#235617=CARTESIAN_POINT('',(54.25,97.9199999800001,-86.84995));
#235618=CARTESIAN_POINT('Origin',(54.25,97.1699999800001,-86.84995));
#235619=CARTESIAN_POINT('',(54.25,97.9199999800001,-89.84995));
#235620=CARTESIAN_POINT('Origin',(48.,97.1699999800001,-86.84995));
#235621=CARTESIAN_POINT('',(48.,97.9199999800001,-80.59995));
#235622=CARTESIAN_POINT('',(48.,97.1699999800001,-79.84995));
#235623=CARTESIAN_POINT('Origin',(48.,97.1699999800001,-80.59995));
#235624=CARTESIAN_POINT('Origin',(48.,97.1699999800001,-86.84995));
#235625=CARTESIAN_POINT('Origin',(48.,97.9199999800001,-86.84995));
#235626=CARTESIAN_POINT('Origin',(-51.,97.1699999800001,-80.59995));
#235627=CARTESIAN_POINT('',(-51.,97.1699999800001,-79.84995));
#235628=CARTESIAN_POINT('',(45.,97.9199999800001,-80.59995));
#235629=CARTESIAN_POINT('Origin',(45.,97.9199999800001,-179.84995));
#235630=CARTESIAN_POINT('',(48.,97.9199999799999,-189.84995));
#235631=CARTESIAN_POINT('',(-51.,97.9199999799999,-189.84995));
#235632=CARTESIAN_POINT('Origin',(48.,105.91999998,-189.84995));
#235633=CARTESIAN_POINT('',(48.,105.91999998,-189.84995));
#235634=CARTESIAN_POINT('Origin',(-51.,105.91999998,-79.84995));
#235635=CARTESIAN_POINT('',(48.,105.91999998,-79.84995));
#235636=CARTESIAN_POINT('Origin',(48.,105.91999998,-86.84995));
#235637=CARTESIAN_POINT('Origin',(48.,105.91999998,-182.84995));
#235638=CARTESIAN_POINT('Origin',(44.5079524583208,31.5404524382925,235.35105));
#235639=CARTESIAN_POINT('',(44.507952458321,29.5404524382925,-52.1412));
#235640=CARTESIAN_POINT('',(44.5079524583209,29.5404524382925,-52.29995));
#235641=CARTESIAN_POINT('',(44.5079524583208,29.5404524382925,235.35105));
#235642=CARTESIAN_POINT('',(44.5079524583208,33.5404524382925,-52.64995));
#235643=CARTESIAN_POINT('Ctrl Pts',(44.5079524583208,33.5404524382925,-52.64995));
#235644=CARTESIAN_POINT('Ctrl Pts',(44.3548545542709,33.5404524382925,-52.6422157773399));
#235645=CARTESIAN_POINT('Ctrl Pts',(44.20228357332,33.522873307937,-52.6339954492238));
#235646=CARTESIAN_POINT('Ctrl Pts',(43.8989259410511,33.4520476875708,-52.6166046360311));
#235647=CARTESIAN_POINT('Ctrl Pts',(43.7494532049307,33.3978112619257,-52.6074716543951));
#235648=CARTESIAN_POINT('Ctrl Pts',(43.3701659866181,33.2066898065316,-52.5827363905734));
#235649=CARTESIAN_POINT('Ctrl Pts',(43.1586558164617,33.0405619760126,-52.56720589332));
#235650=CARTESIAN_POINT('Ctrl Pts',(42.8201807947071,32.6434822936339,-52.5385252711531));
#235651=CARTESIAN_POINT('Ctrl Pts',(42.6932650854895,32.4191782753192,-52.52620900716));
#235652=CARTESIAN_POINT('Ctrl Pts',(42.5294572327396,31.9312855999297,-52.4977486010956));
#235653=CARTESIAN_POINT('Ctrl Pts',(42.4955147520946,31.6718569742787,-52.4826152645993));
#235654=CARTESIAN_POINT('Ctrl Pts',(42.5288723018669,31.1486243083691,-52.4520933590879));
#235655=CARTESIAN_POINT('Ctrl Pts',(42.5981844499906,30.889977401297,-52.437005622842));
#235656=CARTESIAN_POINT('Ctrl Pts',(42.8283842527865,30.425478719589,-52.4099098664091));
#235657=CARTESIAN_POINT('Ctrl Pts',(42.9828916680193,30.2219875462947,-52.3968713548753));
#235658=CARTESIAN_POINT('Ctrl Pts',(43.3663701864947,29.8774589096907,-52.3674499782107));
#235659=CARTESIAN_POINT('Ctrl Pts',(43.5939982252634,29.7422747167445,-52.3520077588389));
#235660=CARTESIAN_POINT('Ctrl Pts',(44.0556467980409,29.5790367525449,-52.3239250203703));
#235661=CARTESIAN_POINT('Ctrl Pts',(44.2811108622566,29.5404524382925,-52.3114096174482));
#235662=CARTESIAN_POINT('Ctrl Pts',(44.507952458321,29.5404524382925,-52.29995));
#235663=CARTESIAN_POINT('',(46.4884569292028,31.8190238668641,-52.64995));
#235664=CARTESIAN_POINT('Origin',(44.5079524583208,31.5404524382925,-52.64995));
#235665=CARTESIAN_POINT('Ctrl Pts',(44.5079524583211,29.5404524382925,-52.1412));
#235666=CARTESIAN_POINT('Ctrl Pts',(44.3247135465072,29.5404524382925,-52.1504568905679));
#235667=CARTESIAN_POINT('Ctrl Pts',(44.1420161231988,29.5656268611773,-52.1604206801398));
#235668=CARTESIAN_POINT('Ctrl Pts',(43.7109798879774,29.6872198414568,-52.1857422946277));
#235669=CARTESIAN_POINT('Ctrl Pts',(43.4736864604903,29.8084243584665,-52.2012650509945));
#235670=CARTESIAN_POINT('Ctrl Pts',(43.0674816021137,30.1299064414062,-52.2311623291258));
#235671=CARTESIAN_POINT('Ctrl Pts',(42.9001540986214,30.3241179882545,-52.245247157081));
#235672=CARTESIAN_POINT('Ctrl Pts',(42.6416335239846,30.774204283096,-52.2715021909468));
#235673=CARTESIAN_POINT('Ctrl Pts',(42.5566346319212,31.0280187184028,-52.2863080330063));
#235674=CARTESIAN_POINT('Ctrl Pts',(42.4910511170322,31.549641664286,-52.3167360381829));
#235675=CARTESIAN_POINT('Ctrl Pts',(42.5094203902604,31.8122183820464,-52.3320530133855));
#235676=CARTESIAN_POINT('Ctrl Pts',(42.6440633687565,32.3087595709814,-52.3610179160734));
#235677=CARTESIAN_POINT('Ctrl Pts',(42.7564335035464,32.5387234706583,-52.3734994103579));
#235678=CARTESIAN_POINT('Ctrl Pts',(43.0697411860967,32.9558560535547,-52.4014935014093));
#235679=CARTESIAN_POINT('Ctrl Pts',(43.2721028320881,33.1355884690471,-52.416958632555));
#235680=CARTESIAN_POINT('Ctrl Pts',(43.7266339026704,33.3994643576703,-52.447617080786));
#235681=CARTESIAN_POINT('Ctrl Pts',(43.972394781555,33.4845697527202,-52.4625147060633));
#235682=CARTESIAN_POINT('Ctrl Pts',(44.4834801603881,33.556936973569,-52.490444503763));
#235683=CARTESIAN_POINT('Ctrl Pts',(44.743966207421,33.5432294366744,-52.5030419818516));
#235684=CARTESIAN_POINT('Ctrl Pts',(45.2513765607801,33.4159146504311,-52.5323887613926));
#235685=CARTESIAN_POINT('Ctrl Pts',(45.4927345544246,33.3011989232752,-52.5479275957456));
#235686=CARTESIAN_POINT('Ctrl Pts',(45.9088031766997,32.9904464827263,-52.5780102250637));
#235687=CARTESIAN_POINT('Ctrl Pts',(46.0819169579592,32.8004312724763,-52.5922977230811));
#235688=CARTESIAN_POINT('Ctrl Pts',(46.2845268385021,32.4687376590909,-52.612207596182));
#235689=CARTESIAN_POINT('Ctrl Pts',(46.3426893780983,32.3477280723218,-52.6191089213483));
#235690=CARTESIAN_POINT('Ctrl Pts',(46.4355872980842,32.0913303618597,-52.6340654544586));
#235691=CARTESIAN_POINT('Ctrl Pts',(46.4691386827723,31.9563670022371,-52.6419383171033));
#235692=CARTESIAN_POINT('Ctrl Pts',(46.4884569292029,31.8190238668635,-52.6499500000001));
#235693=CARTESIAN_POINT('Origin',(44.5079524583208,31.5404524382925,235.35105));
#235694=CARTESIAN_POINT('',(44.5079524583209,29.5404524382925,-51.4412));
#235695=CARTESIAN_POINT('',(44.507952458193,29.5404524382925,-51.5999500000129));
#235696=CARTESIAN_POINT('',(44.5079524583208,29.5404524382925,235.35105));
#235697=CARTESIAN_POINT('Ctrl Pts',(44.507952458321,29.5404524382925,-52.29995));
#235698=CARTESIAN_POINT('Ctrl Pts',(44.5456351337306,29.5404524382925,-52.2980463410057));
#235699=CARTESIAN_POINT('Ctrl Pts',(44.5833527227913,29.5415174066421,-52.2961098566617));
#235700=CARTESIAN_POINT('Ctrl Pts',(44.8762306266861,29.5581074238872,-52.2808303317015));
#235701=CARTESIAN_POINT('Ctrl Pts',(45.1262365572094,29.6213370764521,-52.2663562967642));
#235702=CARTESIAN_POINT('Ctrl Pts',(45.597903751345,29.8426585978762,-52.2360733323412));
#235703=CARTESIAN_POINT('Ctrl Pts',(45.8134393435507,30.0021996411661,-52.2205315928461));
#235704=CARTESIAN_POINT('Ctrl Pts',(46.1636689240197,30.389587657716,-52.1915398257226));
#235705=CARTESIAN_POINT('Ctrl Pts',(46.2975269516407,30.6113093304199,-52.179150014626));
#235706=CARTESIAN_POINT('Ctrl Pts',(46.4747895814738,31.0950501116668,-52.1509318023866));
#235707=CARTESIAN_POINT('Ctrl Pts',(46.5158274230668,31.3527181233366,-52.1359011683725));
#235708=CARTESIAN_POINT('Ctrl Pts',(46.4973503317335,31.8760198349414,-52.1053752351956));
#235709=CARTESIAN_POINT('Ctrl Pts',(46.4353859646996,32.1365641269858,-52.0901768181597));
#235710=CARTESIAN_POINT('Ctrl Pts',(46.2183725159575,32.607519480871,-52.0627044225164));
#235711=CARTESIAN_POINT('Ctrl Pts',(46.0696264259219,32.8153523985847,-52.0499916286466));
#235712=CARTESIAN_POINT('Ctrl Pts',(45.6964971586862,33.1700942756708,-52.0207951908128));
#235713=CARTESIAN_POINT('Ctrl Pts',(45.4734934122146,33.3113546790648,-52.0054093593214));
#235714=CARTESIAN_POINT('Ctrl Pts',(44.9798457017477,33.5023539189302,-51.9749003797879));
#235715=CARTESIAN_POINT('Ctrl Pts',(44.7132445891919,33.5478172614533,-51.9605357857066));
#235716=CARTESIAN_POINT('Ctrl Pts',(44.1908699228379,33.5315455130639,-51.9336717920495));
#235717=CARTESIAN_POINT('Ctrl Pts',(43.9399556743881,33.4749621780699,-51.9193457215013));
#235718=CARTESIAN_POINT('Ctrl Pts',(43.4638587352539,33.266716276669,-51.8892203468131));
#235719=CARTESIAN_POINT('Ctrl Pts',(43.2447120691995,33.1134614667662,-51.8736795310267));
#235720=CARTESIAN_POINT('Ctrl Pts',(42.883495283233,32.7353393673502,-51.8444029665401));
#235721=CARTESIAN_POINT('Ctrl Pts',(42.7430457982723,32.5160099599919,-51.8318575220992));
#235722=CARTESIAN_POINT('Ctrl Pts',(42.5532874534621,32.036216321252,-51.8038695598394));
#235723=CARTESIAN_POINT('Ctrl Pts',(42.5057248801028,31.7803536661032,-51.788944238289));
#235724=CARTESIAN_POINT('Ctrl Pts',(42.5104063276564,31.2573688010795,-51.7584367878293));
#235725=CARTESIAN_POINT('Ctrl Pts',(42.5654998955738,30.9952548269627,-51.7431468060059));
#235726=CARTESIAN_POINT('Ctrl Pts',(42.7701978299134,30.5184201146716,-51.7153314477889));
#235727=CARTESIAN_POINT('Ctrl Pts',(42.9136660376696,30.306512587328,-51.7028338192499));
#235728=CARTESIAN_POINT('Ctrl Pts',(43.2772642491842,29.9425079270756,-51.6738487081959));
#235729=CARTESIAN_POINT('Ctrl Pts',(43.4958968886054,29.795817128197,-51.6585253104048));
#235730=CARTESIAN_POINT('Ctrl Pts',(43.9809674611855,29.5930189970377,-51.6281054976679));
#235731=CARTESIAN_POINT('Ctrl Pts',(44.2432162131644,29.5404524383263,-51.6133239849614));
#235732=CARTESIAN_POINT('Ctrl Pts',(44.5079524580651,29.5404524382925,-51.5999500000129));
#235733=CARTESIAN_POINT('Ctrl Pts',(44.507952458321,29.5404524382925,-51.4412));
#235734=CARTESIAN_POINT('Ctrl Pts',(44.2835205459591,29.5404524382925,-51.452537884689));
#235735=CARTESIAN_POINT('Ctrl Pts',(44.060408947064,29.5782209797479,-51.4649106520451));
#235736=CARTESIAN_POINT('Ctrl Pts',(43.600354723926,29.7390446890627,-51.4928424311542));
#235737=CARTESIAN_POINT('Ctrl Pts',(43.3721726577259,29.8734763513654,-51.5082906901557));
#235738=CARTESIAN_POINT('Ctrl Pts',(42.9874338287575,30.2167497384021,-51.5377391239273));
#235739=CARTESIAN_POINT('Ctrl Pts',(42.8322220836105,30.4197176397976,-51.5508238034211));
#235740=CARTESIAN_POINT('Ctrl Pts',(42.6004293202525,30.8834252224738,-51.5778734124105));
#235741=CARTESIAN_POINT('Ctrl Pts',(42.5302307820271,31.1418277220128,-51.5929468915503));
#235742=CARTESIAN_POINT('Ctrl Pts',(42.4950690952893,31.6650230748981,-51.6234666204686));
#235743=CARTESIAN_POINT('Ctrl Pts',(42.5281472402474,31.9246519959457,-51.638611640863));
#235744=CARTESIAN_POINT('Ctrl Pts',(42.6903245105921,32.4130413675739,-51.6671010208747));
#235745=CARTESIAN_POINT('Ctrl Pts',(42.8164088542485,32.637658525451,-51.6794148597991));
#235746=CARTESIAN_POINT('Ctrl Pts',(43.1534652959873,33.0358936686857,-51.7080575188717));
#235747=CARTESIAN_POINT('Ctrl Pts',(43.364478565968,33.2028067206776,-51.7235858159412));
#235748=CARTESIAN_POINT('Ctrl Pts',(43.830419889728,33.4395637991918,-51.7540297237424));
#235749=CARTESIAN_POINT('Ctrl Pts',(44.0791181973968,33.5106841931608,-51.7686678466185));
#235750=CARTESIAN_POINT('Ctrl Pts',(44.5959203541677,33.5556751071966,-51.79608796974));
#235751=CARTESIAN_POINT('Ctrl Pts',(44.8592765093109,33.5267715625772,-51.8093472661401));
#235752=CARTESIAN_POINT('Ctrl Pts',(45.3605005505186,33.3686702778741,-51.8392794641832));
#235753=CARTESIAN_POINT('Ctrl Pts',(45.5933401003551,33.2407902593983,-51.8547719210234));
#235754=CARTESIAN_POINT('Ctrl Pts',(45.9888671080995,32.9083686699532,-51.8844488428499));
#235755=CARTESIAN_POINT('Ctrl Pts',(46.1501372598996,32.7098359294834,-51.8979859630138));
#235756=CARTESIAN_POINT('Ctrl Pts',(46.3954557319109,32.2529402210043,-51.924638212675));
#235757=CARTESIAN_POINT('Ctrl Pts',(46.4731638382971,31.996744828296,-51.9395829439163));
#235758=CARTESIAN_POINT('Ctrl Pts',(46.5236902380054,31.4741208800458,-51.9700693408976));
#235759=CARTESIAN_POINT('Ctrl Pts',(46.4980090848323,31.212901646118,-51.9853071295434));
#235760=CARTESIAN_POINT('Ctrl Pts',(46.3497242517928,30.7203434272596,-52.0140396923102));
#235761=CARTESIAN_POINT('Ctrl Pts',(46.2306336465384,30.4930439305853,-52.026389417297));
#235762=CARTESIAN_POINT('Ctrl Pts',(45.9056096715121,30.0851316905039,-52.0547064670867));
#235763=CARTESIAN_POINT('Ctrl Pts',(45.6989028260139,29.9116459531387,-52.0702089148879));
#235764=CARTESIAN_POINT('Ctrl Pts',(45.238573056588,29.6610301989817,-52.1007735487266));
#235765=CARTESIAN_POINT('Ctrl Pts',(44.9912718473802,29.5827827275061,-52.1155489658689));
#235766=CARTESIAN_POINT('Ctrl Pts',(44.6600861713746,29.5447870978041,-52.1333880589147));
#235767=CARTESIAN_POINT('Ctrl Pts',(44.5839791314037,29.5404524382925,-52.1373592732352));
#235768=CARTESIAN_POINT('Ctrl Pts',(44.5079524583211,29.5404524382925,-52.1412));
#235769=CARTESIAN_POINT('Origin',(44.5079524583208,31.5404524382925,235.35105));
#235770=CARTESIAN_POINT('',(44.5079524426195,29.5404524382925,-50.7412000015864));
#235771=CARTESIAN_POINT('',(44.5079524583207,29.5404524382925,-50.89995));
#235772=CARTESIAN_POINT('',(44.5079524583208,29.5404524382925,235.35105));
#235773=CARTESIAN_POINT('Ctrl Pts',(44.5079524580651,29.5404524382925,-51.5999500000129));
#235774=CARTESIAN_POINT('Ctrl Pts',(44.5081493673179,29.5404524382924,-51.599940052522));
#235775=CARTESIAN_POINT('Ctrl Pts',(44.5083462778614,29.5404524673725,-51.5999301041178));
#235776=CARTESIAN_POINT('Ctrl Pts',(44.7627038634985,29.5405275958781,-51.5870782385727));
#235777=CARTESIAN_POINT('Ctrl Pts',(45.0144847350904,29.5890492353315,-51.5729435206145));
#235778=CARTESIAN_POINT('Ctrl Pts',(45.4954760302278,29.7813442718332,-51.5430361256822));
#235779=CARTESIAN_POINT('Ctrl Pts',(45.7187617861315,29.9268804692804,-51.5275113369366));
#235780=CARTESIAN_POINT('Ctrl Pts',(46.0931857907529,30.2935768625855,-51.4979008179775));
#235781=CARTESIAN_POINT('Ctrl Pts',(46.241707454404,30.5100447027299,-51.4850571179078));
#235782=CARTESIAN_POINT('Ctrl Pts',(46.4463995242366,30.985003637967,-51.457351180019));
#235783=CARTESIAN_POINT('Ctrl Pts',(46.5016652543187,31.238498615233,-51.4425639730119));
#235784=CARTESIAN_POINT('Ctrl Pts',(46.5134570330975,31.7626294411718,-51.4119896748321));
#235785=CARTESIAN_POINT('Ctrl Pts',(46.465862850225,32.0283350076239,-51.3964901834558));
#235786=CARTESIAN_POINT('Ctrl Pts',(46.2738235919859,32.513261598713,-51.3682027989756));
#235787=CARTESIAN_POINT('Ctrl Pts',(46.135997236833,32.7296270969305,-51.3558448804301));
#235788=CARTESIAN_POINT('Ctrl Pts',(45.782620463481,33.1034209671638,-51.3270906188832));
#235789=CARTESIAN_POINT('Ctrl Pts',(45.5687864590191,33.2557554890865,-51.3118450306571));
#235790=CARTESIAN_POINT('Ctrl Pts',(45.0902866126965,33.4720690956454,-51.2813629574795));
#235791=CARTESIAN_POINT('Ctrl Pts',(44.8294053642904,33.5321786562759,-51.2664305242991));
#235792=CARTESIAN_POINT('Ctrl Pts',(44.3109920276729,33.5468055245127,-51.2398146253572));
#235793=CARTESIAN_POINT('Ctrl Pts',(44.0584917971278,33.5057281278676,-51.2262312871613));
#235794=CARTESIAN_POINT('Ctrl Pts',(43.5732154725709,33.328054025563,-51.1965338643904));
#235795=CARTESIAN_POINT('Ctrl Pts',(43.3463649249246,33.189685965016,-51.1810380596255));
#235796=CARTESIAN_POINT('Ctrl Pts',(42.9599322942034,32.8336714503139,-51.1511324419018));
#235797=CARTESIAN_POINT('Ctrl Pts',(42.8039167057754,32.6198105770137,-51.1379125580922));
#235798=CARTESIAN_POINT('Ctrl Pts',(42.5857129743017,32.1493364439137,-51.1104682336614));
#235799=CARTESIAN_POINT('Ctrl Pts',(42.5235781282351,31.8981751919542,-51.0958171606304));
#235800=CARTESIAN_POINT('Ctrl Pts',(42.4969894941382,31.3760742307904,-51.0653612712291));
#235801=CARTESIAN_POINT('Ctrl Pts',(42.5367477260569,31.1099059746523,-51.0498347896211));
#235802=CARTESIAN_POINT('Ctrl Pts',(42.7144151204012,30.6193907836024,-51.0212214034765));
#235803=CARTESIAN_POINT('Ctrl Pts',(42.8464254671907,30.398322385025,-51.0089084741443));
#235804=CARTESIAN_POINT('Ctrl Pts',(43.1892525940538,30.0145747762835,-50.9803968438328));
#235805=CARTESIAN_POINT('Ctrl Pts',(43.3980237487336,29.8566145876055,-50.9652429394571));
#235806=CARTESIAN_POINT('Ctrl Pts',(43.8693711210719,29.6266874739172,-50.9347251353981));
#235807=CARTESIAN_POINT('Ctrl Pts',(44.1284296497864,29.5589656500773,-50.9196627582983));
#235808=CARTESIAN_POINT('Ctrl Pts',(44.4314438908588,29.5415490019518,-50.9038470542835));
#235809=CARTESIAN_POINT('Ctrl Pts',(44.4697148774346,29.5404524382925,-50.9018816917915));
#235810=CARTESIAN_POINT('Ctrl Pts',(44.5079524583206,29.5404524382925,-50.89995));
#235811=CARTESIAN_POINT('Ctrl Pts',(44.5079524425794,29.5404524382925,-50.7412000007952));
#235812=CARTESIAN_POINT('Ctrl Pts',(44.2452561334393,29.5404524403601,-50.7544709320253));
#235813=CARTESIAN_POINT('Ctrl Pts',(43.9849786972769,29.5922110211334,-50.7691292914831));
#235814=CARTESIAN_POINT('Ctrl Pts',(43.5010903453052,29.7928033553668,-50.7994250448801));
#235815=CARTESIAN_POINT('Ctrl Pts',(43.2819599179859,29.9388901614813,-50.8147559735385));
#235816=CARTESIAN_POINT('Ctrl Pts',(42.9172875125919,30.3018574876075,-50.8437650952998));
#235817=CARTESIAN_POINT('Ctrl Pts',(42.773225484448,30.5133019264419,-50.8562828868087));
#235818=CARTESIAN_POINT('Ctrl Pts',(42.5671310964014,30.9894774249937,-50.8840597908909));
#235819=CARTESIAN_POINT('Ctrl Pts',(42.5112584037884,31.2514232116598,-50.8993399617797));
#235820=CARTESIAN_POINT('Ctrl Pts',(42.5050182585672,31.7744622727418,-50.9298505736762));
#235821=CARTESIAN_POINT('Ctrl Pts',(42.5518462004841,32.0305372605673,-50.9447882812993));
#235822=CARTESIAN_POINT('Ctrl Pts',(42.7401910787824,32.5107818792282,-50.9728025507212));
#235823=CARTESIAN_POINT('Ctrl Pts',(42.879887657652,32.7303817503275,-50.9853261188118));
#235824=CARTESIAN_POINT('Ctrl Pts',(43.2398585046255,33.1095652093879,-51.0145706970902));
#235825=CARTESIAN_POINT('Ctrl Pts',(43.4586032107541,33.2635390974229,-51.0301121797175));
#235826=CARTESIAN_POINT('Ctrl Pts',(43.9342139565177,33.4732767871518,-51.0602565033097));
#235827=CARTESIAN_POINT('Ctrl Pts',(44.1850336713978,33.5306166599398,-51.0745998638826));
#235828=CARTESIAN_POINT('Ctrl Pts',(44.7071273312422,33.548392843454,-51.1014935409689));
#235829=CARTESIAN_POINT('Ctrl Pts',(44.9735543568746,33.5038140543269,-51.1157899654104));
#235830=CARTESIAN_POINT('Ctrl Pts',(45.4676287468362,33.3145522441628,-51.1462698249691));
#235831=CARTESIAN_POINT('Ctrl Pts',(45.6911698647951,33.1739798064205,-51.1616627378082));
#235832=CARTESIAN_POINT('Ctrl Pts',(46.0654869628404,32.820401770524,-51.1908852372873));
#235833=CARTESIAN_POINT('Ctrl Pts',(46.2148924843005,32.6130713946132,-51.2036305608812));
#235834=CARTESIAN_POINT('Ctrl Pts',(46.4334291012576,32.1428534000483,-51.2310599438975));
#235835=CARTESIAN_POINT('Ctrl Pts',(46.4962429254979,31.8825168140543,-51.2462462447471));
#235836=CARTESIAN_POINT('Ctrl Pts',(46.5164335266262,31.3592013514549,-51.2767729800655));
#235837=CARTESIAN_POINT('Ctrl Pts',(46.4762096777092,31.101320734677,-51.2918160160442));
#235838=CARTESIAN_POINT('Ctrl Pts',(46.3004972586309,30.6170965329672,-51.3200624278106));
#235839=CARTESIAN_POINT('Ctrl Pts',(46.1674469680564,30.3950776435402,-51.332438841346));
#235840=CARTESIAN_POINT('Ctrl Pts',(45.8185759413347,30.0065582653918,-51.3613949748962));
#235841=CARTESIAN_POINT('Ctrl Pts',(45.6034971258212,29.8462486108739,-51.3769360567059));
#235842=CARTESIAN_POINT('Ctrl Pts',(45.1323997288438,29.6233229611646,-51.4072370231063));
#235843=CARTESIAN_POINT('Ctrl Pts',(44.8825177204272,29.5592755503712,-51.42172864901));
#235844=CARTESIAN_POINT('Ctrl Pts',(44.5875246136248,29.541638478946,-51.4371455691851));
#235845=CARTESIAN_POINT('Ctrl Pts',(44.5477195375851,29.5404524382925,-51.4391910407822));
#235846=CARTESIAN_POINT('Ctrl Pts',(44.507952458321,29.5404524382925,-51.4412));
#235847=CARTESIAN_POINT('Origin',(44.5079524583208,31.5404524382925,235.35105));
#235848=CARTESIAN_POINT('',(44.5079524583207,29.5404524382925,-50.0412));
#235849=CARTESIAN_POINT('',(44.5079524583207,29.5404524382925,-50.19995));
#235850=CARTESIAN_POINT('',(44.5079524583208,29.5404524382925,235.35105));
#235851=CARTESIAN_POINT('Ctrl Pts',(44.5079524583206,29.5404524382925,-50.89995));
#235852=CARTESIAN_POINT('Ctrl Pts',(44.7223870492869,29.5404524382924,-50.8891171614784));
#235853=CARTESIAN_POINT('Ctrl Pts',(44.9356705179706,29.5749306382515,-50.8773368613579));
#235854=CARTESIAN_POINT('Ctrl Pts',(45.388596365462,29.7257050768233,-50.8500582983187));
#235855=CARTESIAN_POINT('Ctrl Pts',(45.6188175437727,29.8567602462415,-50.8346055081911));
#235856=CARTESIAN_POINT('Ctrl Pts',(46.0172668306694,30.2017837993482,-50.8044134009588));
#235857=CARTESIAN_POINT('Ctrl Pts',(46.1809412372564,30.4130117124252,-50.7907173756756));
#235858=CARTESIAN_POINT('Ctrl Pts',(46.4126181451152,30.8789081377957,-50.7635400841957));
#235859=CARTESIAN_POINT('Ctrl Pts',(46.481496793499,31.1275673053499,-50.7490349660883));
#235860=CARTESIAN_POINT('Ctrl Pts',(46.5226921292547,31.6472471862232,-50.7187203063708));
#235861=CARTESIAN_POINT('Ctrl Pts',(46.490708585099,31.9136550356356,-50.7031798484884));
#235862=CARTESIAN_POINT('Ctrl Pts',(46.327395781776,32.4095726321365,-50.6742513220259));
#235863=CARTESIAN_POINT('Ctrl Pts',(46.2011360550349,32.6353821888252,-50.6618843827444));
#235864=CARTESIAN_POINT('Ctrl Pts',(45.8687191959684,33.0288137008287,-50.6336162127094));
#235865=CARTESIAN_POINT('Ctrl Pts',(45.6650438756082,33.1921243816843,-50.618563684427));
#235866=CARTESIAN_POINT('Ctrl Pts',(45.2010753834282,33.4351518281971,-50.5880365546913));
#235867=CARTESIAN_POINT('Ctrl Pts',(44.9440229078205,33.5102718024179,-50.5728597402943));
#235868=CARTESIAN_POINT('Ctrl Pts',(44.4274400923127,33.5548169790144,-50.5454636985625));
#235869=CARTESIAN_POINT('Ctrl Pts',(44.1732648218395,33.5284566265293,-50.532692322418));
#235870=CARTESIAN_POINT('Ctrl Pts',(43.6802205162023,33.3798298053096,-50.5034496879898));
#235871=CARTESIAN_POINT('Ctrl Pts',(43.4469659558143,33.2558972613171,-50.4880514002574));
#235872=CARTESIAN_POINT('Ctrl Pts',(43.0370244822471,32.9216899214035,-50.4575942019164));
#235873=CARTESIAN_POINT('Ctrl Pts',(42.8658645972105,32.7130212416766,-50.4433498468641));
#235874=CARTESIAN_POINT('Ctrl Pts',(42.621331652736,32.2515930595891,-50.416433202909));
#235875=CARTESIAN_POINT('Ctrl Pts',(42.5461252697442,32.0054783084443,-50.4020765090922));
#235876=CARTESIAN_POINT('Ctrl Pts',(42.4911498890836,31.4884695511673,-50.3719176649177));
#235877=CARTESIAN_POINT('Ctrl Pts',(42.5157620760352,31.2220369675854,-50.3563757642088));
#235878=CARTESIAN_POINT('Ctrl Pts',(42.6653547852825,30.7211280053138,-50.327156074743));
#235879=CARTESIAN_POINT('Ctrl Pts',(42.7861592882629,30.4907476085359,-50.3146487456099));
#235880=CARTESIAN_POINT('Ctrl Pts',(43.1087425797863,30.0882899618175,-50.2866140869383));
#235881=CARTESIAN_POINT('Ctrl Pts',(43.3075233072641,29.9201112674401,-50.2716668406986));
#235882=CARTESIAN_POINT('Ctrl Pts',(43.7642477394687,29.6650253207538,-50.2411539612058));
#235883=CARTESIAN_POINT('Ctrl Pts',(44.0192236691758,29.5830296156398,-50.225881507912));
#235884=CARTESIAN_POINT('Ctrl Pts',(44.357686330653,29.5446815888122,-50.2076645167837));
#235885=CARTESIAN_POINT('Ctrl Pts',(44.4328567771926,29.5404524382925,-50.203743694775));
#235886=CARTESIAN_POINT('Ctrl Pts',(44.5079524583205,29.5404524382925,-50.19995));
#235887=CARTESIAN_POINT('Ctrl Pts',(44.5079524583206,29.5404524382925,-50.0412));
#235888=CARTESIAN_POINT('Ctrl Pts',(44.4718396769997,29.5404524382925,-50.0430243508515));
#235889=CARTESIAN_POINT('Ctrl Pts',(44.4356964143001,29.5414305218481,-50.0448787690027));
#235890=CARTESIAN_POINT('Ctrl Pts',(44.1347625162448,29.5577637409606,-50.0605577779271));
#235891=CARTESIAN_POINT('Ctrl Pts',(43.8754935925516,29.6246561249279,-50.0756065917954));
#235892=CARTESIAN_POINT('Ctrl Pts',(43.4033453825172,29.8531064654309,-50.1061217801408));
#235893=CARTESIAN_POINT('Ctrl Pts',(43.1940137605603,30.0104595756638,-50.121286291831));
#235894=CARTESIAN_POINT('Ctrl Pts',(42.8500294412034,30.3931225943627,-50.1498247474887));
#235895=CARTESIAN_POINT('Ctrl Pts',(42.7173810615116,30.6136699299704,-50.1621376870145));
#235896=CARTESIAN_POINT('Ctrl Pts',(42.5381287939439,31.1035777460775,-50.1907156429541));
#235897=CARTESIAN_POINT('Ctrl Pts',(42.4975087939038,31.3697059799194,-50.2062397899282));
#235898=CARTESIAN_POINT('Ctrl Pts',(42.5224738071396,31.8920503217537,-50.2367098765352));
#235899=CARTESIAN_POINT('Ctrl Pts',(42.5838567543876,32.1434774629151,-50.2513764597696));
#235900=CARTESIAN_POINT('Ctrl Pts',(42.8005716030855,32.6144509620887,-50.2788499138881));
#235901=CARTESIAN_POINT('Ctrl Pts',(42.9557523429832,32.8286004468419,-50.292023374237));
#235902=CARTESIAN_POINT('Ctrl Pts',(43.3408593825313,33.1858084919308,-50.3218968368519));
#235903=CARTESIAN_POINT('Ctrl Pts',(43.5673259416073,33.3249747315708,-50.3373965234486));
#235904=CARTESIAN_POINT('Ctrl Pts',(44.0521514345071,33.5042740140904,-50.3671185721286));
#235905=CARTESIAN_POINT('Ctrl Pts',(44.3045692693176,33.5461702783005,-50.3807586875109));
#235906=CARTESIAN_POINT('Ctrl Pts',(44.8230662180689,33.5331907529982,-50.4073307628807));
#235907=CARTESIAN_POINT('Ctrl Pts',(45.0841320350819,33.4739130629318,-50.4222482572339));
#235908=CARTESIAN_POINT('Ctrl Pts',(45.5633868399102,33.2590953146877,-50.4527248403166));
#235909=CARTESIAN_POINT('Ctrl Pts',(45.7777631848714,33.1073829098469,-50.4679796814991));
#235910=CARTESIAN_POINT('Ctrl Pts',(46.1322836598823,32.7346771640365,-50.4967599837739));
#235911=CARTESIAN_POINT('Ctrl Pts',(46.2707407253182,32.5188152061094,-50.509128838544));
#235912=CARTESIAN_POINT('Ctrl Pts',(46.4643277872029,32.0345012181195,-50.5373804878434));
#235913=CARTESIAN_POINT('Ctrl Pts',(46.512768475601,31.7688589176576,-50.5528762887036));
#235914=CARTESIAN_POINT('Ctrl Pts',(46.5025796737736,31.2445334353493,-50.5834619418383));
#235915=CARTESIAN_POINT('Ctrl Pts',(46.4480603283826,30.9907976408417,-50.5982631965179));
#235916=CARTESIAN_POINT('Ctrl Pts',(46.2448247752994,30.5153615378464,-50.6259969691926));
#235917=CARTESIAN_POINT('Ctrl Pts',(46.0971000007615,30.298613993033,-50.6388061630299));
#235918=CARTESIAN_POINT('Ctrl Pts',(45.7239673879505,29.9307859133832,-50.6683844507841));
#235919=CARTESIAN_POINT('Ctrl Pts',(45.5010763917506,29.7844873078777,-50.683911533902));
#235920=CARTESIAN_POINT('Ctrl Pts',(45.0205425114124,29.5906216983497,-50.7138416294655));
#235921=CARTESIAN_POINT('Ctrl Pts',(44.7688353612694,29.5413084976514,-50.7279957103556));
#235922=CARTESIAN_POINT('Ctrl Pts',(44.5123839247908,29.5404561201211,-50.7409760231318));
#235923=CARTESIAN_POINT('Ctrl Pts',(44.5101681030411,29.540452438275,-50.7410880697314));
#235924=CARTESIAN_POINT('Ctrl Pts',(44.5079524425794,29.5404524382925,-50.7412000007953));
#235925=CARTESIAN_POINT('Origin',(44.5079524583208,31.5404524382925,235.35105));
#235926=CARTESIAN_POINT('',(44.5079524583207,29.5404524382925,-49.3412));
#235927=CARTESIAN_POINT('',(44.5079524583208,29.5404524382925,-49.49995));
#235928=CARTESIAN_POINT('',(44.5079524583208,29.5404524382925,235.35105));
#235929=CARTESIAN_POINT('Ctrl Pts',(44.5079524583205,29.5404524382925,-50.19995));
#235930=CARTESIAN_POINT('Ctrl Pts',(44.6854903835516,29.5404524382924,-50.1909811127192));
#235931=CARTESIAN_POINT('Ctrl Pts',(44.8625403587716,29.56408467282,-50.1813476022625));
#235932=CARTESIAN_POINT('Ctrl Pts',(45.28620891383,29.6796980413921,-50.156572594677));
#235933=CARTESIAN_POINT('Ctrl Pts',(45.5220741830687,29.7969970368165,-50.141235897267));
#235934=CARTESIAN_POINT('Ctrl Pts',(45.9387949613059,30.1181270424578,-50.1108176432552));
#235935=CARTESIAN_POINT('Ctrl Pts',(46.1144794508713,30.3200935055919,-50.0961376044075));
#235936=CARTESIAN_POINT('Ctrl Pts',(46.3715502505798,30.7712516860386,-50.0698200438814));
#235937=CARTESIAN_POINT('Ctrl Pts',(46.4541344793749,31.0141498381624,-50.0556509850076));
#235938=CARTESIAN_POINT('Ctrl Pts',(46.5252715707204,31.5275366066112,-50.0257034235147));
#235939=CARTESIAN_POINT('Ctrl Pts',(46.5093512265501,31.7937439167226,-50.0101746637582));
#235940=CARTESIAN_POINT('Ctrl Pts',(46.3761051620342,32.3003689583257,-49.9806215363314));
#235941=CARTESIAN_POINT('Ctrl Pts',(46.2617604432823,32.5362486897881,-49.9678384083179));
#235942=CARTESIAN_POINT('Ctrl Pts',(45.9507500216637,32.949176749041,-49.9400830025751));
#235943=CARTESIAN_POINT('Ctrl Pts',(45.7578157806442,33.1228486696454,-49.9252708909085));
#235944=CARTESIAN_POINT('Ctrl Pts',(45.3080776926849,33.3928271136546,-49.8946765840869));
#235945=CARTESIAN_POINT('Ctrl Pts',(45.0535188148037,33.4831006191545,-49.8791837636346));
#235946=CARTESIAN_POINT('Ctrl Pts',(44.5371087550905,33.556323037186,-49.8509600296639));
#235947=CARTESIAN_POINT('Ctrl Pts',(44.2810316527491,33.543724827296,-49.8385818257136));
#235948=CARTESIAN_POINT('Ctrl Pts',(43.7812887351337,33.4218568125833,-49.8097812550002));
#235949=CARTESIAN_POINT('Ctrl Pts',(43.5429243093868,33.3114488625768,-49.7945192936551));
#235950=CARTESIAN_POINT('Ctrl Pts',(43.1179787815527,33.0027190464296,-49.764047212715));
#235951=CARTESIAN_POINT('Ctrl Pts',(42.9366013104539,32.8058204339529,-49.7491414824884));
#235952=CARTESIAN_POINT('Ctrl Pts',(42.6671935620064,32.3625804136743,-49.7226036679059));
#235953=CARTESIAN_POINT('Ctrl Pts',(42.5778537182236,32.1227672258342,-49.7089183626068));
#235954=CARTESIAN_POINT('Ctrl Pts',(42.4919955194013,31.6129175222094,-49.6791771298953));
#235955=CARTESIAN_POINT('Ctrl Pts',(42.4999743107404,31.3471585975877,-49.6636745259591));
#235956=CARTESIAN_POINT('Ctrl Pts',(42.6180965880014,30.835474477271,-49.6338262856073));
#235957=CARTESIAN_POINT('Ctrl Pts',(42.7264862189083,30.5944607914065,-49.6206882864261));
#235958=CARTESIAN_POINT('Ctrl Pts',(43.0269238084561,30.1721073775051,-49.5931920944073));
#235959=CARTESIAN_POINT('Ctrl Pts',(43.2144480637339,29.9936415728931,-49.5785134635872));
#235960=CARTESIAN_POINT('Ctrl Pts',(43.6551267556531,29.7118567137799,-49.5480324669067));
#235961=CARTESIAN_POINT('Ctrl Pts',(43.9062190856509,29.6145713201919,-49.5325102566327));
#235962=CARTESIAN_POINT('Ctrl Pts',(44.281221150398,29.5500864982108,-49.51168503931));
#235963=CARTESIAN_POINT('Ctrl Pts',(44.3946043832944,29.5404524382925,-49.5056761348925));
#235964=CARTESIAN_POINT('Ctrl Pts',(44.5079524583208,29.5404524382925,-49.49995));
#235965=CARTESIAN_POINT('Ctrl Pts',(44.5079524583205,29.5404524382924,-49.3412));
#235966=CARTESIAN_POINT('Ctrl Pts',(44.4347306017759,29.5404524382925,-49.3448990326264));
#235967=CARTESIAN_POINT('Ctrl Pts',(44.36143495477,29.5444731844207,-49.3487190647722));
#235968=CARTESIAN_POINT('Ctrl Pts',(44.0247419395233,29.5816604188695,-49.366812800205));
#235969=CARTESIAN_POINT('Ctrl Pts',(43.769538862732,29.6629362233144,-49.3820757314461));
#235970=CARTESIAN_POINT('Ctrl Pts',(43.3120382640791,29.9167649498573,-49.4125911525099));
#235971=CARTESIAN_POINT('Ctrl Pts',(43.1127377910696,30.0844387239051,-49.4275499284887));
#235972=CARTESIAN_POINT('Ctrl Pts',(42.7891170628562,30.485949790652,-49.4556093879586));
#235973=CARTESIAN_POINT('Ctrl Pts',(42.6677358253903,30.7158435078294,-49.4680978123896));
#235974=CARTESIAN_POINT('Ctrl Pts',(42.516688318219,31.2162315094823,-49.497287112486));
#235975=CARTESIAN_POINT('Ctrl Pts',(42.491297617099,31.4826708114347,-49.5128294050999));
#235976=CARTESIAN_POINT('Ctrl Pts',(42.5448208218008,31.9999789945987,-49.5430057157845));
#235977=CARTESIAN_POINT('Ctrl Pts',(42.619361967759,32.2463704050013,-49.557378548058));
#235978=CARTESIAN_POINT('Ctrl Pts',(42.8625328016231,32.7082767065792,-49.5843230823167));
#235979=CARTESIAN_POINT('Ctrl Pts',(43.0328912932333,32.9172191858626,-49.5985050044065));
#235980=CARTESIAN_POINT('Ctrl Pts',(43.4416143774102,33.2525880935964,-49.6289345310327));
#235981=CARTESIAN_POINT('Ctrl Pts',(43.6745563136385,33.3772816950055,-49.6443392230793));
#235982=CARTESIAN_POINT('Ctrl Pts',(44.1672080797862,33.5274255373187,-49.6736062735878));
#235983=CARTESIAN_POINT('Ctrl Pts',(44.4212860495018,33.5545592635309,-49.6864103244151));
#235984=CARTESIAN_POINT('Ctrl Pts',(44.9379811137366,33.5115991391739,-49.7137658060544));
#235985=CARTESIAN_POINT('Ctrl Pts',(45.1952589178849,33.437268907295,-49.7289309694805));
#235986=CARTESIAN_POINT('Ctrl Pts',(45.6600354667484,33.1956337283898,-49.7594583129385));
#235987=CARTESIAN_POINT('Ctrl Pts',(45.864263122286,33.0328886673496,-49.7745222469268));
#235988=CARTESIAN_POINT('Ctrl Pts',(46.1977991581386,32.6404921391706,-49.8028167686727));
#235989=CARTESIAN_POINT('Ctrl Pts',(46.3246783953422,32.415196790911,-49.8151732460972));
#235990=CARTESIAN_POINT('Ctrl Pts',(46.4895428970062,31.9198546302735,-49.8440682054677));
#235991=CARTESIAN_POINT('Ctrl Pts',(46.5223640304513,31.6534620717256,-49.859607771383));
#235992=CARTESIAN_POINT('Ctrl Pts',(46.4827387391494,31.1335018402801,-49.889938784884));
#235993=CARTESIAN_POINT('Ctrl Pts',(46.4145831811994,30.8845641698543,-49.9044601489922));
#235994=CARTESIAN_POINT('Ctrl Pts',(46.1843616608845,30.418168117697,-49.9316665853681));
#235995=CARTESIAN_POINT('Ctrl Pts',(46.021523674798,30.2066536689454,-49.9453063152114));
#235996=CARTESIAN_POINT('Ctrl Pts',(45.6243740475149,29.8604261174862,-49.9754678826649));
#235997=CARTESIAN_POINT('Ctrl Pts',(45.394507714501,29.7285733411811,-49.9909260101993));
#235998=CARTESIAN_POINT('Ctrl Pts',(44.9399504315824,29.5756303575526,-50.0183502395666));
#235999=CARTESIAN_POINT('Ctrl Pts',(44.7245509498906,29.5404524382924,-50.0302578452263));
#236000=CARTESIAN_POINT('Ctrl Pts',(44.5079524583206,29.5404524382925,-50.0412));
#236001=CARTESIAN_POINT('Origin',(44.5079524583208,31.5404524382925,235.35105));
#236002=CARTESIAN_POINT('',(44.5079524583208,29.5404524382925,-48.6412));
#236003=CARTESIAN_POINT('',(44.5079524583208,29.5404524382925,-48.79995));
#236004=CARTESIAN_POINT('',(44.5079524583208,29.5404524382925,235.35105));
#236005=CARTESIAN_POINT('Ctrl Pts',(44.5079524583208,29.5404524382925,-49.49995));
#236006=CARTESIAN_POINT('Ctrl Pts',(44.6484656327225,29.5404524382925,-49.4928515345818));
#236007=CARTESIAN_POINT('Ctrl Pts',(44.7888806723387,29.5552566461249,-49.4853262373563));
#236008=CARTESIAN_POINT('Ctrl Pts',(45.1806504006529,29.6391837124542,-49.4630868832543));
#236009=CARTESIAN_POINT('Ctrl Pts',(45.4213938027402,29.7424116308721,-49.4479141580171));
#236010=CARTESIAN_POINT('Ctrl Pts',(45.854619835414,30.0381992846698,-49.4174012410385));
#236011=CARTESIAN_POINT('Ctrl Pts',(46.041702894108,30.2297530025382,-49.4023631678496));
#236012=CARTESIAN_POINT('Ctrl Pts',(46.323783766141,30.66472907859,-49.3754261622338));
#236013=CARTESIAN_POINT('Ctrl Pts',(46.4199950666918,30.9014832349083,-49.3622232035309));
#236014=CARTESIAN_POINT('Ctrl Pts',(46.520718713886,31.4074374884758,-49.3327092054061));
#236015=CARTESIAN_POINT('Ctrl Pts',(46.520782148984,31.6725038366582,-49.3172470017622));
#236016=CARTESIAN_POINT('Ctrl Pts',(46.4181877781362,32.1891466636479,-49.2871095035211));
#236017=CARTESIAN_POINT('Ctrl Pts',(46.3159074025737,32.4354702613398,-49.2735131832809));
#236018=CARTESIAN_POINT('Ctrl Pts',(46.0261962946597,32.8672514390045,-49.2462838968116));
#236019=CARTESIAN_POINT('Ctrl Pts',(45.8442148432103,33.050360574315,-49.2317498476999));
#236020=CARTESIAN_POINT('Ctrl Pts',(45.4129231573035,33.3436961542053,-49.201406169161));
#236021=CARTESIAN_POINT('Ctrl Pts',(45.1654925444267,33.4478912620257,-49.1858674087248));
#236022=CARTESIAN_POINT('Ctrl Pts',(44.653864715571,33.5515029361511,-49.1569989109002));
#236023=CARTESIAN_POINT('Ctrl Pts',(44.3954195531985,33.5536463187043,-49.144649867494));
#236024=CARTESIAN_POINT('Ctrl Pts',(43.8890919987703,33.4598239728255,-49.1163346517942));
#236025=CARTESIAN_POINT('Ctrl Pts',(43.6462066668259,33.3637312842641,-49.101261831097));
#236026=CARTESIAN_POINT('Ctrl Pts',(43.2051904152028,33.0809433095534,-49.070734523987));
#236027=CARTESIAN_POINT('Ctrl Pts',(43.0126306470048,32.8948361340484,-49.0555786350594));
#236028=CARTESIAN_POINT('Ctrl Pts',(42.7181155625902,32.4681458225661,-49.0282551441886));
#236029=CARTESIAN_POINT('Ctrl Pts',(42.6151406296482,32.2343021242018,-49.0154245650115));
#236030=CARTESIAN_POINT('Ctrl Pts',(42.5000340017128,31.732252165234,-48.9861383174051));
#236031=CARTESIAN_POINT('Ctrl Pts',(42.4921940754199,31.4680869181564,-48.9707286779922));
#236032=CARTESIAN_POINT('Ctrl Pts',(42.579542595888,30.9468134144484,-48.9403210569426));
#236033=CARTESIAN_POINT('Ctrl Pts',(42.6758149910805,30.6952460162276,-48.9261876720982));
#236034=CARTESIAN_POINT('Ctrl Pts',(42.9551155629621,30.2544432760503,-48.8992211777281));
#236035=CARTESIAN_POINT('Ctrl Pts',(43.1316771331268,30.0670398204614,-48.8848356799762));
#236036=CARTESIAN_POINT('Ctrl Pts',(43.5536933825864,29.7629099787529,-48.8546457466773));
#236037=CARTESIAN_POINT('Ctrl Pts',(43.7974425359341,29.6522098012248,-48.8391032355606));
#236038=CARTESIAN_POINT('Ctrl Pts',(44.2043250364462,29.5577537492186,-48.8157933167722));
#236039=CARTESIAN_POINT('Ctrl Pts',(44.3560483031499,29.5404524382925,-48.8076239166769));
#236040=CARTESIAN_POINT('Ctrl Pts',(44.5079524583209,29.5404524382925,-48.79995));
#236041=CARTESIAN_POINT('Ctrl Pts',(44.5079524583208,29.5404524382925,-48.6412));
#236042=CARTESIAN_POINT('Ctrl Pts',(44.3966865670165,29.5404524382925,-48.6468209468259));
#236043=CARTESIAN_POINT('Ctrl Pts',(44.2853796577939,29.5497358422582,-48.6527147317501));
#236044=CARTESIAN_POINT('Ctrl Pts',(43.912159951728,29.6127135730367,-48.6734059507855));
#236045=CARTESIAN_POINT('Ctrl Pts',(43.6606906762901,29.7092600291355,-48.6889256513018));
#236046=CARTESIAN_POINT('Ctrl Pts',(43.2190355200071,29.9898046404431,-48.7194198032597));
#236047=CARTESIAN_POINT('Ctrl Pts',(43.0309311224372,30.1677690648216,-48.7341131182042));
#236048=CARTESIAN_POINT('Ctrl Pts',(42.7293651132697,30.5891228335877,-48.7616371595765));
#236049=CARTESIAN_POINT('Ctrl Pts',(42.6203370049354,30.829583738668,-48.7747326591886));
#236050=CARTESIAN_POINT('Ctrl Pts',(42.5005919680911,31.3407357668696,-48.8045498608337));
#236051=CARTESIAN_POINT('Ctrl Pts',(42.4917660124846,31.6065536272709,-48.8200559026904));
#236052=CARTESIAN_POINT('Ctrl Pts',(42.5760576785285,32.1168053340831,-48.8498205855878));
#236053=CARTESIAN_POINT('Ctrl Pts',(42.6646798040309,32.3569439318746,-48.863562280121));
#236054=CARTESIAN_POINT('Ctrl Pts',(42.9327627204454,32.8010377406691,-48.8900580688071));
#236055=CARTESIAN_POINT('Ctrl Pts',(43.1135369753961,32.9984829249773,-48.9049492673491));
#236056=CARTESIAN_POINT('Ctrl Pts',(43.5375977426921,33.3085472673299,-48.9354155755059));
#236057=CARTESIAN_POINT('Ctrl Pts',(43.775702314129,33.4197000986306,-48.9506861351968));
#236058=CARTESIAN_POINT('Ctrl Pts',(44.2750891658946,33.5430335850107,-48.9795114610464));
#236059=CARTESIAN_POINT('Ctrl Pts',(44.5310529398885,33.5563922254494,-48.9919020831007));
#236060=CARTESIAN_POINT('Ctrl Pts',(45.0476916794559,33.4847389964617,-49.0200916015405));
#236061=CARTESIAN_POINT('Ctrl Pts',(45.3025978489709,33.3951962331301,-49.0355806532099));
#236062=CARTESIAN_POINT('Ctrl Pts',(45.7532539199965,33.1264529365426,-49.0661853097033));
#236063=CARTESIAN_POINT('Ctrl Pts',(45.9467399201863,32.9532851912744,-49.0810105901076));
#236064=CARTESIAN_POINT('Ctrl Pts',(46.2588354661981,32.5413320142359,-49.1087923802611));
#236065=CARTESIAN_POINT('Ctrl Pts',(46.3737882052089,32.3059733464028,-49.1215446136935));
#236066=CARTESIAN_POINT('Ctrl Pts',(46.508576223429,31.7998765958748,-49.151066924141));
#236067=CARTESIAN_POINT('Ctrl Pts',(46.5253118626813,31.5336364010089,-49.1665976021749));
#236068=CARTESIAN_POINT('Ctrl Pts',(46.4556867208825,31.01988806246,-49.1965662552569));
#236069=CARTESIAN_POINT('Ctrl Pts',(46.3737906753047,30.7766781966533,-49.210753497429));
#236070=CARTESIAN_POINT('Ctrl Pts',(46.1179762369941,30.3247075715368,-49.2371184505608));
#236071=CARTESIAN_POINT('Ctrl Pts',(45.9428653239357,30.1222324920566,-49.2517422737912));
#236072=CARTESIAN_POINT('Ctrl Pts',(45.5270038822513,29.7998629835924,-49.282153267877));
#236073=CARTESIAN_POINT('Ctrl Pts',(45.2914026904891,29.6818687965638,-49.2974969010036));
#236074=CARTESIAN_POINT('Ctrl Pts',(44.8662072647484,29.5645788470108,-49.3223979435477));
#236075=CARTESIAN_POINT('Ctrl Pts',(44.6873370504399,29.5404524382924,-49.332137822527));
#236076=CARTESIAN_POINT('Ctrl Pts',(44.5079524583205,29.5404524382924,-49.3412));
#236077=CARTESIAN_POINT('Origin',(44.5079524583208,31.5404524382925,235.35105));
#236078=CARTESIAN_POINT('',(44.5079524583208,29.5404524382925,-47.9412));
#236079=CARTESIAN_POINT('',(44.507952458321,29.5404524382925,-48.09995));
#236080=CARTESIAN_POINT('',(44.5079524583208,29.5404524382925,235.35105));
#236081=CARTESIAN_POINT('Ctrl Pts',(44.5079524583209,29.5404524382925,-48.79995));
#236082=CARTESIAN_POINT('Ctrl Pts',(44.6124054576492,29.5404524382925,-48.794673227863));
#236083=CARTESIAN_POINT('Ctrl Pts',(44.7169196208853,29.5486339379085,-48.7891547387667));
#236084=CARTESIAN_POINT('Ctrl Pts',(45.0755021322027,29.6053773611856,-48.7693847976788));
#236085=CARTESIAN_POINT('Ctrl Pts',(45.3202204921733,29.6946948534938,-48.7544169856902));
#236086=CARTESIAN_POINT('Ctrl Pts',(45.7682363932305,29.9650144896715,-48.7238997291241));
#236087=CARTESIAN_POINT('Ctrl Pts',(45.9658206989812,30.1458278721843,-48.7086444121576));
#236088=CARTESIAN_POINT('Ctrl Pts',(46.2720123503269,30.5645670818025,-48.6809629498817));
#236089=CARTESIAN_POINT('Ctrl Pts',(46.3813725344836,30.7957537575501,-48.6683907563767));
#236090=CARTESIAN_POINT('Ctrl Pts',(46.5098146029957,31.2940686287568,-48.6393223888897));
#236091=CARTESIAN_POINT('Ctrl Pts',(46.5248478732476,31.5571950157847,-48.6239733496464));
#236092=CARTESIAN_POINT('Ctrl Pts',(46.4524088657759,32.0784249813983,-48.593568268319));
#236093=CARTESIAN_POINT('Ctrl Pts',(46.3640405764904,32.3311197494686,-48.5789883387074));
#236094=CARTESIAN_POINT('Ctrl Pts',(46.0994768902361,32.7781044399352,-48.5525860176312));
#236095=CARTESIAN_POINT('Ctrl Pts',(45.9293137744679,32.9702837029562,-48.5383844635656));
#236096=CARTESIAN_POINT('Ctrl Pts',(45.5183631917647,33.2865592546567,-48.5083992973889));
#236097=CARTESIAN_POINT('Ctrl Pts',(45.2790807684743,33.4046389462523,-48.4928672013779));
#236098=CARTESIAN_POINT('Ctrl Pts',(44.773147586514,33.539691527979,-48.4633693600995));
#236099=CARTESIAN_POINT('Ctrl Pts',(44.5119607294398,33.5571963467212,-48.4506408544318));
#236100=CARTESIAN_POINT('Ctrl Pts',(43.9993908098511,33.49175967849,-48.4228382015996));
#236101=CARTESIAN_POINT('Ctrl Pts',(43.7528090648274,33.4102014134541,-48.4080025656435));
#236102=CARTESIAN_POINT('Ctrl Pts',(43.2952295341215,33.1531748205669,-48.3773898859768));
#236103=CARTESIAN_POINT('Ctrl Pts',(43.0905955767037,32.9766637978301,-48.3619039191536));
#236104=CARTESIAN_POINT('Ctrl Pts',(42.7712099849039,32.5642902218657,-48.3337415877487));
#236105=CARTESIAN_POINT('Ctrl Pts',(42.6553637021866,32.3357155711247,-48.3213403494153));
#236106=CARTESIAN_POINT('Ctrl Pts',(42.513629119446,31.8412311006041,-48.2924954219683));
#236107=CARTESIAN_POINT('Ctrl Pts',(42.4914536380871,31.5793346839613,-48.2772181309975));
#236108=CARTESIAN_POINT('Ctrl Pts',(42.549215271666,31.0571371659685,-48.2467566091145));
#236109=CARTESIAN_POINT('Ctrl Pts',(42.6304352239428,30.8020589290332,-48.2318770452933));
#236110=CARTESIAN_POINT('Ctrl Pts',(42.8821025646091,30.348418307425,-48.2054146756995));
#236111=CARTESIAN_POINT('Ctrl Pts',(43.0462671530581,30.1519640435191,-48.1916273905432));
#236112=CARTESIAN_POINT('Ctrl Pts',(43.4469111430654,29.824759237847,-48.1618441244399));
#236113=CARTESIAN_POINT('Ctrl Pts',(43.6819049491589,29.7000547860285,-48.1463354592563));
#236114=CARTESIAN_POINT('Ctrl Pts',(44.1207881906624,29.5686522320205,-48.1203313159722));
#236115=CARTESIAN_POINT('Ctrl Pts',(44.314015955622,29.5404524382925,-48.1097473130534));
#236116=CARTESIAN_POINT('Ctrl Pts',(44.5079524583212,29.5404524382925,-48.09995));
#236117=CARTESIAN_POINT('Ctrl Pts',(44.5079524583209,29.5404524382925,-47.9412));
#236118=CARTESIAN_POINT('Ctrl Pts',(44.3579755816972,29.5404524382925,-47.948776554133));
#236119=CARTESIAN_POINT('Ctrl Pts',(44.2081632822339,29.5573175881789,-47.9568366943373));
#236120=CARTESIAN_POINT('Ctrl Pts',(43.8028204437651,29.6501842668025,-47.9800224755263));
#236121=CARTESIAN_POINT('Ctrl Pts',(43.5586882082148,29.7602263932128,-47.995565146089));
#236122=CARTESIAN_POINT('Ctrl Pts',(43.1357136992404,30.0632679431852,-48.0257717470421));
#236123=CARTESIAN_POINT('Ctrl Pts',(42.9585946709616,30.2502405021384,-48.0401728387275));
#236124=CARTESIAN_POINT('Ctrl Pts',(42.6782261972195,30.6901236343595,-48.0671664596237));
#236125=CARTESIAN_POINT('Ctrl Pts',(42.5813335727787,30.9411492814144,-48.0812406491822));
#236126=CARTESIAN_POINT('Ctrl Pts',(42.4924132920601,31.4619564662418,-48.1116210682971));
#236127=CARTESIAN_POINT('Ctrl Pts',(42.4994572444471,31.7262244829687,-48.1270367026061));
#236128=CARTESIAN_POINT('Ctrl Pts',(42.613090509591,32.2286803782218,-48.1563466298292));
#236129=CARTESIAN_POINT('Ctrl Pts',(42.7153669457972,32.4628200369277,-48.1692109537427));
#236130=CARTESIAN_POINT('Ctrl Pts',(43.0086006049266,32.8903727011717,-48.1964948613361));
#236131=CARTESIAN_POINT('Ctrl Pts',(43.2006018186943,33.077050333196,-48.2116391714431));
#236132=CARTESIAN_POINT('Ctrl Pts',(43.6408310230128,33.3611914449707,-48.2421661848781));
#236133=CARTESIAN_POINT('Ctrl Pts',(43.8835045846324,33.4580233813017,-48.2572498687238));
#236134=CARTESIAN_POINT('Ctrl Pts',(44.3895029349291,33.5532900725682,-48.2855905803808));
#236135=CARTESIAN_POINT('Ctrl Pts',(44.6478181814517,33.551915588119,-48.2979314155088));
#236136=CARTESIAN_POINT('Ctrl Pts',(45.1597114761688,33.4498857052435,-48.326767188599));
#236137=CARTESIAN_POINT('Ctrl Pts',(45.4075316399209,33.3464037142673,-48.342304829183));
#236138=CARTESIAN_POINT('Ctrl Pts',(45.8398138956164,33.0542562520053,-48.3726638960428));
#236139=CARTESIAN_POINT('Ctrl Pts',(46.0223774204,32.8716225014001,-48.3872134850344));
#236140=CARTESIAN_POINT('Ctrl Pts',(46.3132107316458,32.4408213495401,-48.4144708790523));
#236141=CARTESIAN_POINT('Ctrl Pts',(46.4161338763291,32.1950578421958,-48.4280146847723));
#236142=CARTESIAN_POINT('Ctrl Pts',(46.5203614144427,31.6789251427172,-48.4581224255752));
#236143=CARTESIAN_POINT('Ctrl Pts',(46.5211382052541,31.4137751212621,-48.4735895101601));
#236144=CARTESIAN_POINT('Ctrl Pts',(46.4219675984017,30.9074071567246,-48.5031276414248));
#236145=CARTESIAN_POINT('Ctrl Pts',(46.3264795719479,30.6703358570656,-48.5163764440766));
#236146=CARTESIAN_POINT('Ctrl Pts',(46.0457312332532,30.2344824504535,-48.5432717213833));
#236147=CARTESIAN_POINT('Ctrl Pts',(45.8592424108637,30.0423568721471,-48.5582964541171));
#236148=CARTESIAN_POINT('Ctrl Pts',(45.4268711694178,29.7451935799646,-48.5888063114116));
#236149=CARTESIAN_POINT('Ctrl Pts',(45.1863687115451,29.6412061835209,-48.6039890160356));
#236150=CARTESIAN_POINT('Ctrl Pts',(44.7928315447917,29.5556772904819,-48.6263643778008));
#236151=CARTESIAN_POINT('Ctrl Pts',(44.6504483170862,29.5404524382925,-48.6340013730386));
#236152=CARTESIAN_POINT('Ctrl Pts',(44.5079524583208,29.5404524382925,-48.6412));
#236153=CARTESIAN_POINT('Origin',(44.5079524583208,31.5404524382925,235.35105));
#236154=CARTESIAN_POINT('',(44.507952458321,29.5404524382925,-47.2412));
#236155=CARTESIAN_POINT('',(44.5079524583209,29.5404524382925,-47.39995));
#236156=CARTESIAN_POINT('',(44.5079524583208,29.5404524382925,235.35105));
#236157=CARTESIAN_POINT('Ctrl Pts',(44.5079524583212,29.5404524382925,-48.09995));
#236158=CARTESIAN_POINT('Ctrl Pts',(44.5744456140837,29.5404524382925,-48.0965908888793));
#236159=CARTESIAN_POINT('Ctrl Pts',(44.6410122894404,29.5437682233701,-48.0931313532869));
#236160=CARTESIAN_POINT('Ctrl Pts',(44.9628032820804,29.5760206257622,-48.0759343730476));
#236161=CARTESIAN_POINT('Ctrl Pts',(45.2108608454448,29.6505409254038,-48.061229455472));
#236162=CARTESIAN_POINT('Ctrl Pts',(45.6741776139309,29.893919033943,-48.0307250219683));
#236163=CARTESIAN_POINT('Ctrl Pts',(45.8831629699355,30.0639777429019,-48.0152074230301));
#236164=CARTESIAN_POINT('Ctrl Pts',(46.2144966875535,30.4668425681303,-47.9867188329934));
#236165=CARTESIAN_POINT('Ctrl Pts',(46.3372422045201,30.6927293159444,-47.9744005154704));
#236166=CARTESIAN_POINT('Ctrl Pts',(46.4928262269163,31.1831112717244,-47.9457949013833));
#236167=CARTESIAN_POINT('Ctrl Pts',(46.5224008360514,31.4435209456006,-47.9306043370738));
#236168=CARTESIAN_POINT('Ctrl Pts',(46.4799450428868,31.9665016465536,-47.9000971295182));
#236169=CARTESIAN_POINT('Ctrl Pts',(46.4061727093305,32.2238843914121,-47.8850831360681));
#236170=CARTESIAN_POINT('Ctrl Pts',(46.1679504623852,32.6843749522474,-47.8582211866861));
#236171=CARTESIAN_POINT('Ctrl Pts',(46.0098765849212,32.8852330176666,-47.8449349925796));
#236172=CARTESIAN_POINT('Ctrl Pts',(45.620028909405,33.2233916342008,-47.8153776501455));
#236173=CARTESIAN_POINT('Ctrl Pts',(45.389622047513,33.3547451495957,-47.7999067778695));
#236174=CARTESIAN_POINT('Ctrl Pts',(44.8902269731069,33.5212152492233,-47.7698228854077));
#236175=CARTESIAN_POINT('Ctrl Pts',(44.6260583212529,33.554295754968,-47.7563202529318));
#236176=CARTESIAN_POINT('Ctrl Pts',(44.1077875119566,33.5166594429613,-47.7290404454297));
#236177=CARTESIAN_POINT('Ctrl Pts',(43.8584383109475,33.4492787656594,-47.7144785156966));
#236178=CARTESIAN_POINT('Ctrl Pts',(43.3897198382266,33.2198251838446,-47.6841073301254));
#236179=CARTESIAN_POINT('Ctrl Pts',(43.1765312949804,33.0563936078188,-47.6685706853269));
#236180=CARTESIAN_POINT('Ctrl Pts',(42.8332139627755,32.663281046047,-47.6397611462857));
#236181=CARTESIAN_POINT('Ctrl Pts',(42.7034498373582,32.4400428806018,-47.6274261091348));
#236182=CARTESIAN_POINT('Ctrl Pts',(42.5340872269857,31.953853028734,-47.5990650344425));
#236183=CARTESIAN_POINT('Ctrl Pts',(42.4972072082159,31.6951280328635,-47.5839727430167));
#236184=CARTESIAN_POINT('Ctrl Pts',(42.5244193618401,31.1718152306882,-47.5534461628898));
#236185=CARTESIAN_POINT('Ctrl Pts',(42.5907049592164,30.9123590996215,-47.5383112219109));
#236186=CARTESIAN_POINT('Ctrl Pts',(42.8154698231011,30.4451792389422,-47.5110590633713));
#236187=CARTESIAN_POINT('Ctrl Pts',(42.9675879904806,30.2399008772353,-47.498166940483));
#236188=CARTESIAN_POINT('Ctrl Pts',(43.3467828590477,29.8911246887345,-47.4688380789505));
#236189=CARTESIAN_POINT('Ctrl Pts',(43.5725128424477,29.7534030632497,-47.4534177373727));
#236190=CARTESIAN_POINT('Ctrl Pts',(44.0394865101384,29.5818720814861,-47.4248241052893));
#236191=CARTESIAN_POINT('Ctrl Pts',(44.2729285172036,29.5404524382925,-47.4118229743711));
#236192=CARTESIAN_POINT('Ctrl Pts',(44.5079524583209,29.5404524382925,-47.39995));
#236193=CARTESIAN_POINT('Ctrl Pts',(44.5079524583212,29.5404524382925,-47.2412));
#236194=CARTESIAN_POINT('Ctrl Pts',(44.3161695932765,29.5404524382925,-47.2508885152664));
#236195=CARTESIAN_POINT('Ctrl Pts',(44.1250598901523,29.5680293419666,-47.2613473499961));
#236196=CARTESIAN_POINT('Ctrl Pts',(43.6877393791654,29.6974352527612,-47.2872143116007));
#236197=CARTESIAN_POINT('Ctrl Pts',(43.4522787886795,29.8214387035994,-47.3027261120056));
#236198=CARTESIAN_POINT('Ctrl Pts',(43.050514532505,30.1474951765375,-47.3325324788435));
#236199=CARTESIAN_POINT('Ctrl Pts',(42.8857142674878,30.3434963463404,-47.3463775613027));
#236200=CARTESIAN_POINT('Ctrl Pts',(42.6326624757846,30.7964223289899,-47.3727982436239));
#236201=CARTESIAN_POINT('Ctrl Pts',(42.5506780675097,31.0512500957407,-47.3876631966844));
#236202=CARTESIAN_POINT('Ctrl Pts',(42.491337179176,31.573341120158,-47.418118506442));
#236203=CARTESIAN_POINT('Ctrl Pts',(42.5127455459109,31.8353792307101,-47.4334040628909));
#236204=CARTESIAN_POINT('Ctrl Pts',(42.6530492798312,32.3302810924118,-47.4622733381568));
#236205=CARTESIAN_POINT('Ctrl Pts',(42.7681912048292,32.5591352929089,-47.4746887324736));
#236206=CARTESIAN_POINT('Ctrl Pts',(43.0863482336752,32.9724749727599,-47.5028171771827));
#236207=CARTESIAN_POINT('Ctrl Pts',(43.2905260064056,33.149640493398,-47.5182991879222));
#236208=CARTESIAN_POINT('Ctrl Pts',(43.7474962882126,33.4080567439264,-47.5489216211438));
#236209=CARTESIAN_POINT('Ctrl Pts',(43.9939158737931,33.4903338565153,-47.563770031492));
#236210=CARTESIAN_POINT('Ctrl Pts',(44.5061868906327,33.5571755127349,-47.591598563127));
#236211=CARTESIAN_POINT('Ctrl Pts',(44.7672301534184,33.5404430936836,-47.6042985016686));
#236212=CARTESIAN_POINT('Ctrl Pts',(45.2734675098934,33.4069622838196,-47.6337658659344));
#236213=CARTESIAN_POINT('Ctrl Pts',(45.5131751696297,33.2895629917125,-47.6492995991183));
#236214=CARTESIAN_POINT('Ctrl Pts',(45.9251710929418,32.9744026848683,-47.6793050459922));
#236215=CARTESIAN_POINT('Ctrl Pts',(46.0959356868371,32.7826593326602,-47.6935242715538));
#236216=CARTESIAN_POINT('Ctrl Pts',(46.361805112398,32.3363515453863,-47.7199728131524));
#236217=CARTESIAN_POINT('Ctrl Pts',(46.4508870206064,32.0838984732078,-47.7344989812965));
#236218=CARTESIAN_POINT('Ctrl Pts',(46.5248028126764,31.5627978865617,-47.7648965155175));
#236219=CARTESIAN_POINT('Ctrl Pts',(46.5104917901831,31.2995581891282,-47.7802521645345));
#236220=CARTESIAN_POINT('Ctrl Pts',(46.3833906627011,30.8008628174555,-47.809342727882));
#236221=CARTESIAN_POINT('Ctrl Pts',(46.2746778676633,30.5694106870498,-47.821937021061));
#236222=CARTESIAN_POINT('Ctrl Pts',(45.969666662751,30.1498598706526,-47.849582521233));
#236223=CARTESIAN_POINT('Ctrl Pts',(45.7725848615113,29.9685035242572,-47.8648282890485));
#236224=CARTESIAN_POINT('Ctrl Pts',(45.3252623113295,29.6969122274837,-47.8953476089128));
#236225=CARTESIAN_POINT('Ctrl Pts',(45.0807212817331,29.6069066929765,-47.9103265303966));
#236226=CARTESIAN_POINT('Ctrl Pts',(44.7204630306518,29.5489141010597,-47.9302175608401));
#236227=CARTESIAN_POINT('Ctrl Pts',(44.6141790638268,29.5404524382925,-47.9358336285627));
#236228=CARTESIAN_POINT('Ctrl Pts',(44.5079524583209,29.5404524382925,-47.9412));
#236229=CARTESIAN_POINT('Origin',(44.5079524583208,31.5404524382925,235.35105));
#236230=CARTESIAN_POINT('',(44.5079524583209,29.5404524382925,-46.5412));
#236231=CARTESIAN_POINT('',(44.5079524583208,29.5404524382925,-46.69995));
#236232=CARTESIAN_POINT('',(44.5079524583208,29.5404524382925,235.35105));
#236233=CARTESIAN_POINT('Ctrl Pts',(44.5079524583209,29.5404524382925,-47.39995));
#236234=CARTESIAN_POINT('Ctrl Pts',(44.5385862697585,29.5404524382925,-47.398402436563));
#236235=CARTESIAN_POINT('Ctrl Pts',(44.5692449150485,29.5411562530311,-47.3968330906359));
#236236=CARTESIAN_POINT('Ctrl Pts',(44.8549461411357,29.5543055640908,-47.3820164720818));
#236237=CARTESIAN_POINT('Ctrl Pts',(45.1053514370633,29.614769287618,-47.3676029348738));
#236238=CARTESIAN_POINT('Ctrl Pts',(45.5789056016243,29.8306574967445,-47.3373831158073));
#236239=CARTESIAN_POINT('Ctrl Pts',(45.7959658777406,29.9875909690999,-47.3218404062562));
#236240=CARTESIAN_POINT('Ctrl Pts',(46.1507794359507,30.3711385593677,-47.2927290774974));
#236241=CARTESIAN_POINT('Ctrl Pts',(46.2873745175777,30.5918599420633,-47.2802845622801));
#236242=CARTESIAN_POINT('Ctrl Pts',(46.4698592437824,31.0739620758806,-47.2521619378074));
#236243=CARTESIAN_POINT('Ctrl Pts',(46.5136319627525,31.3308953616782,-47.2371741628025));
#236244=CARTESIAN_POINT('Ctrl Pts',(46.5009242215487,31.8541092063848,-47.2066533551947));
#236245=CARTESIAN_POINT('Ctrl Pts',(46.4418263610125,32.115332164523,-47.1914153493033));
#236246=CARTESIAN_POINT('Ctrl Pts',(46.2299515253067,32.5887586022814,-47.1637988071007));
#236247=CARTESIAN_POINT('Ctrl Pts',(46.0834190432785,32.7982891123863,-47.1511860853199));
#236248=CARTESIAN_POINT('Ctrl Pts',(45.7142823903956,33.1569274732217,-47.1220776995284));
#236249=CARTESIAN_POINT('Ctrl Pts',(45.4930970597846,33.3004822053262,-47.1067168131189));
#236250=CARTESIAN_POINT('Ctrl Pts',(45.0043512348937,33.4959368190476,-47.076325519365));
#236251=CARTESIAN_POINT('Ctrl Pts',(44.7410622240157,33.5444211633912,-47.0618420282549));
#236252=CARTESIAN_POINT('Ctrl Pts',(44.2215629831072,33.5361425256362,-47.035356428161));
#236253=CARTESIAN_POINT('Ctrl Pts',(43.9701894283288,33.4835330612488,-47.0211230588669));
#236254=CARTESIAN_POINT('Ctrl Pts',(43.4916145031828,33.2831374574593,-46.9911014679269));
#236255=CARTESIAN_POINT('Ctrl Pts',(43.2703946363235,33.1336745971244,-46.9755665164033));
#236256=CARTESIAN_POINT('Ctrl Pts',(42.9026520849897,32.7611573963193,-46.9461237585419));
#236257=CARTESIAN_POINT('Ctrl Pts',(42.7582353334241,32.5432425794276,-46.9334460915678));
#236258=CARTESIAN_POINT('Ctrl Pts',(42.5571969726149,32.0564042935838,-46.9050471915601));
#236259=CARTESIAN_POINT('Ctrl Pts',(42.5057433597907,31.7910081916521,-46.8895657522793));
#236260=CARTESIAN_POINT('Ctrl Pts',(42.5102196649355,31.2660288392693,-46.8589419567237));
#236261=CARTESIAN_POINT('Ctrl Pts',(42.562075607615,31.0114537827581,-46.8440917450939));
#236262=CARTESIAN_POINT('Ctrl Pts',(42.7601309479512,30.534330462305,-46.8162595514008));
#236263=CARTESIAN_POINT('Ctrl Pts',(42.9050384650336,30.3165894795373,-46.803563577602));
#236264=CARTESIAN_POINT('Ctrl Pts',(43.2735836319553,29.9447670489314,-46.7741005372179));
#236265=CARTESIAN_POINT('Ctrl Pts',(43.4950547252714,29.7957735283593,-46.7585665832752));
#236266=CARTESIAN_POINT('Ctrl Pts',(43.9739264157574,29.5963476757081,-46.7285582847079));
#236267=CARTESIAN_POINT('Ctrl Pts',(44.2253522821904,29.5442282597518,-46.714336565805));
#236268=CARTESIAN_POINT('Ctrl Pts',(44.4892092169482,29.540518289395,-46.7008987945092));
#236269=CARTESIAN_POINT('Ctrl Pts',(44.4985822109721,29.5404524382925,-46.7004233675475));
#236270=CARTESIAN_POINT('Ctrl Pts',(44.5079524583208,29.5404524382925,-46.69995));
#236271=CARTESIAN_POINT('Ctrl Pts',(44.5079524583209,29.5404524382925,-46.5412));
#236272=CARTESIAN_POINT('Ctrl Pts',(44.2750206967325,29.5404524382925,-46.5529672813349));
#236273=CARTESIAN_POINT('Ctrl Pts',(44.0436171059898,29.5811375043278,-46.5658440100673));
#236274=CARTESIAN_POINT('Ctrl Pts',(43.5779919124455,29.750534099846,-46.5943072668012));
#236275=CARTESIAN_POINT('Ctrl Pts',(43.3517741508507,29.8876095534671,-46.609733403351));
#236276=CARTESIAN_POINT('Ctrl Pts',(42.9714833604573,30.2353018099163,-46.6390860141403));
#236277=CARTESIAN_POINT('Ctrl Pts',(42.818754593579,30.4401216450187,-46.652014037059));
#236278=CARTESIAN_POINT('Ctrl Pts',(42.5925962041125,30.9066167014663,-46.6792262486851));
#236279=CARTESIAN_POINT('Ctrl Pts',(42.5255342845323,31.165868982169,-46.6943492983927));
#236280=CARTESIAN_POINT('Ctrl Pts',(42.4967479823186,31.689168175235,-46.7248750846549));
#236281=CARTESIAN_POINT('Ctrl Pts',(42.5328765237534,31.9480765534914,-46.7399780733865));
#236282=CARTESIAN_POINT('Ctrl Pts',(42.7008159887872,32.4347037634724,-46.7683646606355));
#236283=CARTESIAN_POINT('Ctrl Pts',(42.829848466505,32.6582156684402,-46.7806933874648));
#236284=CARTESIAN_POINT('Ctrl Pts',(43.1719235907866,33.05234873328,-46.8094699371344));
#236285=CARTESIAN_POINT('Ctrl Pts',(43.384684326379,33.216474148881,-46.8250052068699));
#236286=CARTESIAN_POINT('Ctrl Pts',(43.8528598735983,33.4473812640628,-46.8553913595732));
#236287=CARTESIAN_POINT('Ctrl Pts',(44.1020841695862,33.5155053329076,-46.8699686615892));
#236288=CARTESIAN_POINT('Ctrl Pts',(44.6200649949416,33.5546051745818,-46.8972765059215));
#236289=CARTESIAN_POINT('Ctrl Pts',(44.8840707818497,33.5223592468335,-46.9107285194261));
#236290=CARTESIAN_POINT('Ctrl Pts',(45.3838357237967,33.3575576767724,-46.9407824314656));
#236291=CARTESIAN_POINT('Ctrl Pts',(45.614731468157,33.2268929751676,-46.9562579107765));
#236292=CARTESIAN_POINT('Ctrl Pts',(46.0057124495535,32.8898748150369,-46.9858392424137));
#236293=CARTESIAN_POINT('Ctrl Pts',(46.1644228605177,32.6894824020146,-46.9991732521161));
#236294=CARTESIAN_POINT('Ctrl Pts',(46.4040654050629,32.2297076493302,-47.0259934460227));
#236295=CARTESIAN_POINT('Ctrl Pts',(46.4786262665402,31.9725573608446,-47.0409938795177));
#236296=CARTESIAN_POINT('Ctrl Pts',(46.5226958109817,31.449637970827,-47.0714975106021));
#236297=CARTESIAN_POINT('Ctrl Pts',(46.493898287438,31.189061856118,-47.0866977839601));
#236298=CARTESIAN_POINT('Ctrl Pts',(46.3397733179045,30.6982423831808,-47.1153289198815));
#236299=CARTESIAN_POINT('Ctrl Pts',(46.2177618156812,30.4720738797123,-47.1276513048442));
#236300=CARTESIAN_POINT('Ctrl Pts',(45.8876915650157,30.0681936211219,-47.1561056836762));
#236301=CARTESIAN_POINT('Ctrl Pts',(45.6791589195109,29.8974451963977,-47.171620529228));
#236302=CARTESIAN_POINT('Ctrl Pts',(45.2164325021904,29.6526125191079,-47.2021375642057));
#236303=CARTESIAN_POINT('Ctrl Pts',(44.9685222274539,29.5773440563874,-47.2168568624556));
#236304=CARTESIAN_POINT('Ctrl Pts',(44.6448390387497,29.5439616914782,-47.2341823901768));
#236305=CARTESIAN_POINT('Ctrl Pts',(44.5763581149533,29.5404524382925,-47.2377442728763));
#236306=CARTESIAN_POINT('Ctrl Pts',(44.5079524583212,29.5404524382925,-47.2412));
#236307=CARTESIAN_POINT('Origin',(44.5079524583208,31.5404524382925,235.35105));
#236308=CARTESIAN_POINT('',(44.5079524583208,29.5404524382925,-45.8412));
#236309=CARTESIAN_POINT('',(44.5079524583207,29.5404524382925,-45.99995));
#236310=CARTESIAN_POINT('',(44.5079524583208,29.5404524382925,235.35105));
#236311=CARTESIAN_POINT('Ctrl Pts',(44.5079524583208,29.5404524382925,-46.69995));
#236312=CARTESIAN_POINT('Ctrl Pts',(44.7634221597085,29.5404524382925,-46.6870441436742));
#236313=CARTESIAN_POINT('Ctrl Pts',(45.0167079303015,29.589399365833,-46.6728209967688));
#236314=CARTESIAN_POINT('Ctrl Pts',(45.4963350804654,29.782246040072,-46.642966426481));
#236315=CARTESIAN_POINT('Ctrl Pts',(45.7172167440047,29.9261789443176,-46.6276098507489));
#236316=CARTESIAN_POINT('Ctrl Pts',(46.0856905776233,30.2854618785066,-46.5985161493034));
#236317=CARTESIAN_POINT('Ctrl Pts',(46.2318559769274,30.4952754861833,-46.5859186555397));
#236318=CARTESIAN_POINT('Ctrl Pts',(46.4428749117245,30.9691110291161,-46.5582782488686));
#236319=CARTESIAN_POINT('Ctrl Pts',(46.5014952445848,31.230443724509,-46.5430338416374));
#236320=CARTESIAN_POINT('Ctrl Pts',(46.5132438034276,31.7536367431509,-46.5125142488833));
#236321=CARTESIAN_POINT('Ctrl Pts',(46.4690172667149,32.0104450524192,-46.497533764176));
#236322=CARTESIAN_POINT('Ctrl Pts',(46.2856638918802,32.4922730914056,-46.4694271285685));
#236323=CARTESIAN_POINT('Ctrl Pts',(46.1486110958527,32.7128281891428,-46.4569720773777));
#236324=CARTESIAN_POINT('Ctrl Pts',(45.7930339387648,33.0957325445022,-46.4278409340355));
#236325=CARTESIAN_POINT('Ctrl Pts',(45.5757221827446,33.2522295367099,-46.4122982508562));
#236326=CARTESIAN_POINT('Ctrl Pts',(45.1018590604176,33.4672095852471,-46.3820893118325));
#236327=CARTESIAN_POINT('Ctrl Pts',(44.8513900654416,33.5272115751659,-46.3676860238968));
#236328=CARTESIAN_POINT('Ctrl Pts',(44.330293025855,33.5502718640802,-46.3406885744799));
#236329=CARTESIAN_POINT('Ctrl Pts',(44.0644745713705,33.5087845471091,-46.3266226714005));
#236330=CARTESIAN_POINT('Ctrl Pts',(43.5689284293712,33.3256133365383,-46.2962461041419));
#236331=CARTESIAN_POINT('Ctrl Pts',(43.3435189490481,33.1874693230036,-46.2808296341347));
#236332=CARTESIAN_POINT('Ctrl Pts',(42.9650423651914,32.8379837252207,-46.2515163679118));
#236333=CARTESIAN_POINT('Ctrl Pts',(42.8133241594923,32.6324043451684,-46.2386471945678));
#236334=CARTESIAN_POINT('Ctrl Pts',(42.5894737850909,32.1647760861673,-46.2113688794594));
#236335=CARTESIAN_POINT('Ctrl Pts',(42.5236977456312,31.9051875424995,-46.1962262144121));
#236336=CARTESIAN_POINT('Ctrl Pts',(42.4975180126245,31.3818684021613,-46.1656992645591));
#236337=CARTESIAN_POINT('Ctrl Pts',(42.5348905306986,31.1232648562457,-46.150614057714));
#236338=CARTESIAN_POINT('Ctrl Pts',(42.7051865878793,30.6373624998062,-46.1222697535884));
#236339=CARTESIAN_POINT('Ctrl Pts',(42.8354315571282,30.4143037868051,-46.1099299903446));
#236340=CARTESIAN_POINT('Ctrl Pts',(43.1795641666072,30.0218623401139,-46.0810988391948));
#236341=CARTESIAN_POINT('Ctrl Pts',(43.3930324959205,29.8588870252188,-46.0655613677385));
#236342=CARTESIAN_POINT('Ctrl Pts',(43.8621051556262,29.6303887290692,-46.0352001517952));
#236343=CARTESIAN_POINT('Ctrl Pts',(44.1115351985903,29.5634963830909,-46.0206483810731));
#236344=CARTESIAN_POINT('Ctrl Pts',(44.4138625005384,29.5421105897467,-46.0047516132155));
#236345=CARTESIAN_POINT('Ctrl Pts',(44.4609318630954,29.5404524382925,-46.0023253934147));
#236346=CARTESIAN_POINT('Ctrl Pts',(44.5079524583205,29.5404524382925,-45.99995));
#236347=CARTESIAN_POINT('Ctrl Pts',(44.5079524583208,29.5404524382925,-45.8412));
#236348=CARTESIAN_POINT('Ctrl Pts',(44.5022154716987,29.5404524382925,-45.8414898219425));
#236349=CARTESIAN_POINT('Ctrl Pts',(44.4964774825353,29.5404771230488,-45.8417804145034));
#236350=CARTESIAN_POINT('Ctrl Pts',(44.225628805887,29.5428083781725,-45.8555311831271));
#236351=CARTESIAN_POINT('Ctrl Pts',(43.9636532182773,29.5977804007479,-45.870369055438));
#236352=CARTESIAN_POINT('Ctrl Pts',(43.4805739512511,29.8048301744746,-45.9008122773467));
#236353=CARTESIAN_POINT('Ctrl Pts',(43.2634245578498,29.9532995605386,-45.9161126197545));
#236354=CARTESIAN_POINT('Ctrl Pts',(42.9030110735591,30.3203699883661,-45.9450262625065));
#236355=CARTESIAN_POINT('Ctrl Pts',(42.7613022043802,30.5336564165181,-45.9574702320632));
#236356=CARTESIAN_POINT('Ctrl Pts',(42.5597712766962,31.0147940314356,-45.9855365929333));
#236357=CARTESIAN_POINT('Ctrl Pts',(42.5069794217426,31.2800702513212,-46.0010110390933));
#236358=CARTESIAN_POINT('Ctrl Pts',(42.5089148690073,31.8053205179484,-46.0316506379799));
#236359=CARTESIAN_POINT('Ctrl Pts',(42.5595843952006,32.0602593978939,-46.0465220726434));
#236360=CARTESIAN_POINT('Ctrl Pts',(42.7553405708373,32.538126635987,-46.0743976615322));
#236361=CARTESIAN_POINT('Ctrl Pts',(42.8990060877282,32.7563080204026,-46.0870481293797));
#236362=CARTESIAN_POINT('Ctrl Pts',(43.2655180517756,33.1298881303849,-46.1164597217674));
#236363=CARTESIAN_POINT('Ctrl Pts',(43.4863511240968,33.2800693374361,-46.1319960849263));
#236364=CARTESIAN_POINT('Ctrl Pts',(43.9644676206521,33.4819499974019,-46.1620378310411));
#236365=CARTESIAN_POINT('Ctrl Pts',(44.2157591859519,33.5353102708598,-46.1762889569765));
#236366=CARTESIAN_POINT('Ctrl Pts',(44.7353185376449,33.5450827675422,-46.2028211646412));
#236367=CARTESIAN_POINT('Ctrl Pts',(44.9987537971474,33.4973500700066,-46.2172515273537));
#236368=CARTESIAN_POINT('Ctrl Pts',(45.4881296745936,33.3032641670339,-46.247634729466));
#236369=CARTESIAN_POINT('Ctrl Pts',(45.7097790220382,33.1602900195349,-46.2630021234292));
#236370=CARTESIAN_POINT('Ctrl Pts',(46.0799306317879,32.802639931508,-46.2921329583388));
#236371=CARTESIAN_POINT('Ctrl Pts',(46.2270254294274,32.5935422094754,-46.3047697633476));
#236372=CARTESIAN_POINT('Ctrl Pts',(46.44020931316,32.1207428492108,-46.3323497260297));
#236373=CARTESIAN_POINT('Ctrl Pts',(46.5000374921706,31.8596895511266,-46.3475778350846));
#236374=CARTESIAN_POINT('Ctrl Pts',(46.5142132434518,31.336447266412,-46.378100301693));
#236375=CARTESIAN_POINT('Ctrl Pts',(46.471135563201,31.0793242663112,-46.3930991433656));
#236376=CARTESIAN_POINT('Ctrl Pts',(46.2899800201273,30.5968035588861,-46.421246184632));
#236377=CARTESIAN_POINT('Ctrl Pts',(46.1540839723624,30.3758276835107,-46.4336753723152));
#236378=CARTESIAN_POINT('Ctrl Pts',(45.8004382557608,29.9912982794807,-46.4627563401128));
#236379=CARTESIAN_POINT('Ctrl Pts',(45.5837639785997,29.8336984212671,-46.4782989859655));
#236380=CARTESIAN_POINT('Ctrl Pts',(45.110685309495,29.6164229725457,-46.5085352450368));
#236381=CARTESIAN_POINT('Ctrl Pts',(44.8603789999663,29.5552536172194,-46.5229643625627));
#236382=CARTESIAN_POINT('Ctrl Pts',(44.5728436713501,29.5412413009968,-46.5378988075647));
#236383=CARTESIAN_POINT('Ctrl Pts',(44.5403843976071,29.5404524382925,-46.5395615984733));
#236384=CARTESIAN_POINT('Ctrl Pts',(44.5079524583209,29.5404524382925,-46.5412));
#236385=CARTESIAN_POINT('Origin',(44.5079524583208,31.5404524382925,235.35105));
#236386=CARTESIAN_POINT('',(44.5079524583206,29.5404524382925,-45.1412));
#236387=CARTESIAN_POINT('',(44.5079524583207,29.5404524382925,-45.29995));
#236388=CARTESIAN_POINT('',(44.5079524583208,29.5404524382925,235.35105));
#236389=CARTESIAN_POINT('Ctrl Pts',(44.5079524583205,29.5404524382925,-45.99995));
#236390=CARTESIAN_POINT('Ctrl Pts',(44.7240341783058,29.5404524382924,-45.98903395157));
#236391=CARTESIAN_POINT('Ctrl Pts',(44.938983568184,29.5754617603926,-45.9771540011326));
#236392=CARTESIAN_POINT('Ctrl Pts',(45.3934223399187,29.7280193428665,-45.9497469995979));
#236393=CARTESIAN_POINT('Ctrl Pts',(45.6235066166138,29.8598248835729,-45.9342792396572));
#236394=CARTESIAN_POINT('Ctrl Pts',(46.0126086329668,30.1987326944784,-45.904737715041));
#236395=CARTESIAN_POINT('Ctrl Pts',(46.1702640354104,30.3998975962579,-45.8914823657854));
#236396=CARTESIAN_POINT('Ctrl Pts',(46.4075506261196,30.8608586977112,-45.8645929682006));
#236397=CARTESIAN_POINT('Ctrl Pts',(46.4808032996821,31.1183931583427,-45.8495701246638));
#236398=CARTESIAN_POINT('Ctrl Pts',(46.5221964566864,31.6414114969648,-45.8190607215775));
#236399=CARTESIAN_POINT('Ctrl Pts',(46.4921105345372,31.9017103260244,-45.8038766232157));
#236400=CARTESIAN_POINT('Ctrl Pts',(46.3355658352113,32.3918035295961,-45.7752878530074));
#236401=CARTESIAN_POINT('Ctrl Pts',(46.2123360749619,32.6175049280227,-45.7629716071216));
#236402=CARTESIAN_POINT('Ctrl Pts',(45.8801698696392,33.0196993788101,-45.7344605139352));
#236403=CARTESIAN_POINT('Ctrl Pts',(45.6708872053655,33.1893026908311,-45.7189411779443));
#236404=CARTESIAN_POINT('Ctrl Pts',(45.2071836024942,33.4317209591311,-45.6884451976239));
#236405=CARTESIAN_POINT('Ctrl Pts',(44.9590301385519,33.5057478068633,-45.6737498276761));
#236406=CARTESIAN_POINT('Ctrl Pts',(44.4433865345556,33.556442345961,-45.6462218767648));
#236407=CARTESIAN_POINT('Ctrl Pts',(44.1806495873855,33.5307494348343,-45.6331322606765));
#236408=CARTESIAN_POINT('Ctrl Pts',(43.6780573849142,33.3791104429147,-45.6033194291989));
#236409=CARTESIAN_POINT('Ctrl Pts',(43.443372877091,33.2539440762327,-45.5878129166744));
#236410=CARTESIAN_POINT('Ctrl Pts',(43.0434688824404,32.92598197317,-45.558044945926));
#236411=CARTESIAN_POINT('Ctrl Pts',(42.8797237890234,32.7292280437918,-45.5442952436542));
#236412=CARTESIAN_POINT('Ctrl Pts',(42.62897202752,32.2751157560239,-45.5178053602011));
#236413=CARTESIAN_POINT('Ctrl Pts',(42.5482579097413,32.0198732233237,-45.5029162124602));
#236414=CARTESIAN_POINT('Ctrl Pts',(42.4915404084121,31.4976079376924,-45.4724507374651));
#236415=CARTESIAN_POINT('Ctrl Pts',(42.5142226926513,31.2358064071097,-45.4571789815144));
#236416=CARTESIAN_POINT('Ctrl Pts',(42.6569030502025,30.7415984948477,-45.4283501866325));
#236417=CARTESIAN_POINT('Ctrl Pts',(42.7732157490531,30.5132084208191,-45.4159577362715));
#236418=CARTESIAN_POINT('Ctrl Pts',(43.0934140220219,30.1014750791851,-45.3877730232199));
#236419=CARTESIAN_POINT('Ctrl Pts',(43.2983488591958,29.9253979250698,-45.3722845110099));
#236420=CARTESIAN_POINT('Ctrl Pts',(43.7563294483999,29.6692920033258,-45.3416784235187));
#236421=CARTESIAN_POINT('Ctrl Pts',(44.0030174043805,29.5882097547967,-45.3268513057966));
#236422=CARTESIAN_POINT('Ctrl Pts',(44.3412934170194,29.5456546263191,-45.3085210366905));
#236423=CARTESIAN_POINT('Ctrl Pts',(44.4246638835946,29.5404524382925,-45.3041575845909));
#236424=CARTESIAN_POINT('Ctrl Pts',(44.5079524583205,29.5404524382925,-45.29995));
#236425=CARTESIAN_POINT('Ctrl Pts',(44.5079524583204,29.5404524382925,-45.1412));
#236426=CARTESIAN_POINT('Ctrl Pts',(44.453989401799,29.5404524382925,-45.1439261137058));
#236427=CARTESIAN_POINT('Ctrl Pts',(44.3999676844034,29.5426363555454,-45.1467188884369));
#236428=CARTESIAN_POINT('Ctrl Pts',(44.090661592359,29.5677625605685,-45.16307730719));
#236429=CARTESIAN_POINT('Ctrl Pts',(43.8416942855719,29.6373763353863,-45.1776850763449));
#236430=CARTESIAN_POINT('Ctrl Pts',(43.3746203408012,29.8711936598925,-45.2081004592373));
#236431=CARTESIAN_POINT('Ctrl Pts',(43.1627237662458,30.0367068232225,-45.2236325491326));
#236432=CARTESIAN_POINT('Ctrl Pts',(42.823140996294,30.4328820248057,-45.2523427519976));
#236433=CARTESIAN_POINT('Ctrl Pts',(42.6955750254693,30.6569419248553,-45.2646618867162));
#236434=CARTESIAN_POINT('Ctrl Pts',(42.5304948927697,31.1444459730064,-45.2930996228583));
#236435=CARTESIAN_POINT('Ctrl Pts',(42.4958786190386,31.4037163382607,-45.3082237274982));
#236436=CARTESIAN_POINT('Ctrl Pts',(42.5278284712106,31.9269737719412,-45.3387470777962));
#236437=CARTESIAN_POINT('Ctrl Pts',(42.5964483318677,32.1858092253091,-45.353845812576));
#236438=CARTESIAN_POINT('Ctrl Pts',(42.8254044147858,32.6509239144061,-45.3809775027733));
#236439=CARTESIAN_POINT('Ctrl Pts',(42.9793632085116,32.8548238030901,-45.393980999241));
#236440=CARTESIAN_POINT('Ctrl Pts',(43.3624287974014,33.2008437030265,-45.4234250106547));
#236441=CARTESIAN_POINT('Ctrl Pts',(43.5903791368553,33.3368878869678,-45.4389085952233));
#236442=CARTESIAN_POINT('Ctrl Pts',(44.0769545501717,33.5098428398493,-45.468534003695));
#236443=CARTESIAN_POINT('Ctrl Pts',(44.3297006140375,33.5485402683169,-45.481959151808));
#236444=CARTESIAN_POINT('Ctrl Pts',(44.8478603800196,33.5291141275632,-45.5087022196127));
#236445=CARTESIAN_POINT('Ctrl Pts',(45.1081882037782,33.4665837408536,-45.5236773022318));
#236446=CARTESIAN_POINT('Ctrl Pts',(45.5844612835644,33.2459261732775,-45.5541735821497));
#236447=CARTESIAN_POINT('Ctrl Pts',(45.79670482814,33.091789441947,-45.569391387728));
#236448=CARTESIAN_POINT('Ctrl Pts',(46.146743368762,32.7148297512957,-45.5980693443669));
#236449=CARTESIAN_POINT('Ctrl Pts',(46.2827292336687,32.4969875397012,-45.6104021190845));
#236450=CARTESIAN_POINT('Ctrl Pts',(46.4702393518327,32.0102802668572,-45.6387933766671));
#236451=CARTESIAN_POINT('Ctrl Pts',(46.5153592165028,31.7444046244669,-45.6543027891398));
#236452=CARTESIAN_POINT('Ctrl Pts',(46.4988869912188,31.220870303568,-45.6848422911923));
#236453=CARTESIAN_POINT('Ctrl Pts',(46.4414444257323,30.9680918530516,-45.6995877008058));
#236454=CARTESIAN_POINT('Ctrl Pts',(46.2324918331374,30.4945357045964,-45.7272118094657));
#236455=CARTESIAN_POINT('Ctrl Pts',(46.0816270318465,30.2788872737542,-45.7401631914179));
#236456=CARTESIAN_POINT('Ctrl Pts',(45.7034218547755,29.9155231302639,-45.7698675375889));
#236457=CARTESIAN_POINT('Ctrl Pts',(45.4789928828164,29.7722287266809,-45.7853846938386));
#236458=CARTESIAN_POINT('Ctrl Pts',(45.0018909428738,29.5865698837846,-45.8149020501006));
#236459=CARTESIAN_POINT('Ctrl Pts',(44.7559254591354,29.5404524382925,-45.8286728631075));
#236460=CARTESIAN_POINT('Ctrl Pts',(44.5079524583208,29.5404524382925,-45.8412));
#236461=CARTESIAN_POINT('Origin',(44.5079524583208,31.5404524382925,235.35105));
#236462=CARTESIAN_POINT('',(44.5079524583207,29.5404524382925,-44.4412));
#236463=CARTESIAN_POINT('',(44.5079524583208,29.5404524382925,-44.59995));
#236464=CARTESIAN_POINT('',(44.5079524583208,29.5404524382925,235.35105));
#236465=CARTESIAN_POINT('Ctrl Pts',(44.5079524583205,29.5404524382925,-45.29995));
#236466=CARTESIAN_POINT('Ctrl Pts',(44.6831064556053,29.5404524382924,-45.2911015443453));
#236467=CARTESIAN_POINT('Ctrl Pts',(44.857829962428,29.5634544131417,-45.2816039453387));
#236468=CARTESIAN_POINT('Ctrl Pts',(45.2827974821138,29.6778151885987,-45.2567998504311));
#236469=CARTESIAN_POINT('Ctrl Pts',(45.5217970209404,29.7963450607897,-45.241268914952));
#236470=CARTESIAN_POINT('Ctrl Pts',(45.9320530989472,30.1133579785335,-45.2112973273572));
#236471=CARTESIAN_POINT('Ctrl Pts',(46.1018169346224,30.3058251526975,-45.1971075467743));
#236472=CARTESIAN_POINT('Ctrl Pts',(46.3655141983934,30.7532564348906,-45.1707359701659));
#236473=CARTESIAN_POINT('Ctrl Pts',(46.4534091422272,31.0061103541599,-45.1561199549078));
#236474=CARTESIAN_POINT('Ctrl Pts',(46.524869168667,31.5274239240777,-45.1257099966626));
#236475=CARTESIAN_POINT('Ctrl Pts',(46.5093574179189,31.7904741309232,-45.1103654012633));
#236476=CARTESIAN_POINT('Ctrl Pts',(46.3800267025948,32.2885362423146,-45.0813117780989));
#236477=CARTESIAN_POINT('Ctrl Pts',(46.2702368122052,32.5195472051907,-45.0687537454164));
#236478=CARTESIAN_POINT('Ctrl Pts',(45.9632621065272,32.9377470444799,-45.04104845632));
#236479=CARTESIAN_POINT('Ctrl Pts',(45.7653451545317,33.1181992899511,-45.0257868678448));
#236480=CARTESIAN_POINT('Ctrl Pts',(45.3168711128907,33.3876739989669,-44.9952711105735));
#236481=CARTESIAN_POINT('Ctrl Pts',(45.0720361186089,33.4765347030518,-44.9803107294253));
#236482=CARTESIAN_POINT('Ctrl Pts',(44.5625491782828,33.5562348996007,-44.9522478034216));
#236483=CARTESIAN_POINT('Ctrl Pts',(44.302783322966,33.5465111301388,-44.9397619469871));
#236484=CARTESIAN_POINT('Ctrl Pts',(43.7938723662163,33.4273407412923,-44.9105769046652));
#236485=CARTESIAN_POINT('Ctrl Pts',(43.5503786996964,33.3162040114379,-44.8950345674939));
#236486=CARTESIAN_POINT('Ctrl Pts',(43.1290006863336,33.0113526575919,-44.8648558325969));
#236487=CARTESIAN_POINT('Ctrl Pts',(42.9528100966551,32.8236637893987,-44.850480751558));
#236488=CARTESIAN_POINT('Ctrl Pts',(42.6742198811008,32.3822500725316,-44.823532322921));
#236489=CARTESIAN_POINT('Ctrl Pts',(42.5783605788317,32.1303218393198,-44.8093590483934));
#236490=CARTESIAN_POINT('Ctrl Pts',(42.4920585623774,31.6087392769756,-44.7789333989233));
#236491=CARTESIAN_POINT('Ctrl Pts',(42.5004277129626,31.344643696309,-44.7635278233844));
#236492=CARTESIAN_POINT('Ctrl Pts',(42.6165141486793,30.8428644390454,-44.7342573667107));
#236493=CARTESIAN_POINT('Ctrl Pts',(42.7199543360269,30.6092172883687,-44.7214486628838));
#236494=CARTESIAN_POINT('Ctrl Pts',(43.015322549558,30.1831022028816,-44.6940988509345));
#236495=CARTESIAN_POINT('Ctrl Pts',(43.2082534171648,29.9973759763086,-44.6789353257623));
#236496=CARTESIAN_POINT('Ctrl Pts',(43.6497916133081,29.7154905600108,-44.6484079756019));
#236497=CARTESIAN_POINT('Ctrl Pts',(43.8928167802752,29.619890520246,-44.6333424596215));
#236498=CARTESIAN_POINT('Ctrl Pts',(44.266572491274,29.5513737199171,-44.6124626064141));
#236499=CARTESIAN_POINT('Ctrl Pts',(44.3872684849238,29.5404524382925,-44.6060467308962));
#236500=CARTESIAN_POINT('Ctrl Pts',(44.5079524583208,29.5404524382925,-44.59995));
#236501=CARTESIAN_POINT('Ctrl Pts',(44.5079524583206,29.5404524382925,-44.4412));
#236502=CARTESIAN_POINT('Ctrl Pts',(44.4179560317545,29.5404524382925,-44.4457464528466));
#236503=CARTESIAN_POINT('Ctrl Pts',(44.3278798180189,29.5465262057059,-44.4504740879429));
#236504=CARTESIAN_POINT('Ctrl Pts',(43.9831082131655,29.5934338475753,-44.4692594506486));
#236505=CARTESIAN_POINT('Ctrl Pts',(43.7370151701557,29.6771307723575,-44.4841327758596));
#236506=CARTESIAN_POINT('Ctrl Pts',(43.2812609719127,29.9382893707129,-44.514773759936));
#236507=CARTESIAN_POINT('Ctrl Pts',(43.0779906547877,30.1167451235776,-44.5302475594717));
#236508=CARTESIAN_POINT('Ctrl Pts',(42.7622648760976,30.5319904552972,-44.5583087634371));
#236509=CARTESIAN_POINT('Ctrl Pts',(42.6485142554119,30.7613997407827,-44.5707552593119));
#236510=CARTESIAN_POINT('Ctrl Pts',(42.5110459693418,31.2571251269908,-44.5996725735074));
#236511=CARTESIAN_POINT('Ctrl Pts',(42.4911590580502,31.5194374102933,-44.6149741233667));
#236512=CARTESIAN_POINT('Ctrl Pts',(42.5536279591984,32.0413032991974,-44.6454163002194));
#236513=CARTESIAN_POINT('Ctrl Pts',(42.6371243081353,32.2956279523115,-44.6602519049844));
#236514=CARTESIAN_POINT('Ctrl Pts',(42.8929170649657,32.7471340129964,-44.6865897585244));
#236515=CARTESIAN_POINT('Ctrl Pts',(43.0589807232594,32.9422382092658,-44.7005527156242));
#236516=CARTESIAN_POINT('Ctrl Pts',(43.4629675598221,33.2660096743689,-44.7304047170464));
#236517=CARTESIAN_POINT('Ctrl Pts',(43.699349010087,33.3886162552127,-44.7459222955409));
#236518=CARTESIAN_POINT('Ctrl Pts',(44.2031855128028,33.534217213492,-44.7756218774485));
#236519=CARTESIAN_POINT('Ctrl Pts',(44.4653512181745,33.5569210687365,-44.7885675291671));
#236520=CARTESIAN_POINT('Ctrl Pts',(44.9798927431999,33.5008773729275,-44.81619582216));
#236521=CARTESIAN_POINT('Ctrl Pts',(45.2275032384634,33.4241205406563,-44.8309433868845));
#236522=CARTESIAN_POINT('Ctrl Pts',(45.6890414504843,33.1763967931192,-44.8614847188126));
#236523=CARTESIAN_POINT('Ctrl Pts',(45.8966665366623,33.0042789598065,-44.8769936572313));
#236524=CARTESIAN_POINT('Ctrl Pts',(46.2242186954592,32.598382047906,-44.9053796457791));
#236525=CARTESIAN_POINT('Ctrl Pts',(46.3447705551076,32.3716503365251,-44.9177134559364));
#236526=CARTESIAN_POINT('Ctrl Pts',(46.4959838624084,31.8799614896161,-44.9463953053395));
#236527=CARTESIAN_POINT('Ctrl Pts',(46.5232288432502,31.6190601159817,-44.9616145521348));
#236528=CARTESIAN_POINT('Ctrl Pts',(46.4759396008089,31.0962780192718,-44.9921101744429));
#236529=CARTESIAN_POINT('Ctrl Pts',(46.3998078168068,30.8395989271094,-45.0070831214857));
#236530=CARTESIAN_POINT('Ctrl Pts',(46.1573336640018,30.3812567907015,-45.0338197461095));
#236531=CARTESIAN_POINT('Ctrl Pts',(45.9973494732639,30.1817923541179,-45.0472526727982));
#236532=CARTESIAN_POINT('Ctrl Pts',(45.6041039612921,29.8470594943569,-45.0768817497333));
#236533=CARTESIAN_POINT('Ctrl Pts',(45.3722364681844,29.7177776170265,-45.0923659876171));
#236534=CARTESIAN_POINT('Ctrl Pts',(44.9232662992318,29.5729351996776,-45.1192716998146));
#236535=CARTESIAN_POINT('Ctrl Pts',(44.7160934399501,29.5404524382924,-45.1306851029699));
#236536=CARTESIAN_POINT('Ctrl Pts',(44.5079524583204,29.5404524382925,-45.1412));
#236537=CARTESIAN_POINT('Origin',(44.5079524583208,31.5404524382925,235.35105));
#236538=CARTESIAN_POINT('',(44.5079524242327,29.5404524382925,-43.7412000034441));
#236539=CARTESIAN_POINT('',(44.5079524583208,29.5404524382925,-43.89995));
#236540=CARTESIAN_POINT('',(44.5079524583208,29.5404524382925,235.35105));
#236541=CARTESIAN_POINT('Ctrl Pts',(44.5079524583208,29.5404524382925,-44.59995));
#236542=CARTESIAN_POINT('Ctrl Pts',(44.642339938529,29.5404524382925,-44.593160993311));
#236543=CARTESIAN_POINT('Ctrl Pts',(44.7766721619236,29.5539942657462,-44.5859798081267));
#236544=CARTESIAN_POINT('Ctrl Pts',(45.1693450251753,29.6343535962872,-44.5637988882803));
#236545=CARTESIAN_POINT('Ctrl Pts',(45.4165147170008,29.7390235784544,-44.5482594585907));
#236546=CARTESIAN_POINT('Ctrl Pts',(45.8471439365854,30.0331498249402,-44.5179261855149));
#236547=CARTESIAN_POINT('Ctrl Pts',(46.028736473741,30.2165750271646,-44.503402565015));
#236548=CARTESIAN_POINT('Ctrl Pts',(46.3176982733281,30.6490097610465,-44.4761920701588));
#236549=CARTESIAN_POINT('Ctrl Pts',(46.4195489627073,30.8957079140314,-44.4625600972487));
#236550=CARTESIAN_POINT('Ctrl Pts',(46.5210517322009,31.4126902081891,-44.4324027967562));
#236551=CARTESIAN_POINT('Ctrl Pts',(46.5204274521103,31.6776992107825,-44.4169439382716));
#236552=CARTESIAN_POINT('Ctrl Pts',(46.4186671045854,32.1833764457246,-44.3874460995666));
#236553=CARTESIAN_POINT('Ctrl Pts',(46.3219722630003,32.4199192153922,-44.3742731409743));
#236554=CARTESIAN_POINT('Ctrl Pts',(46.0390007857604,32.8543077978268,-44.3473082788628));
#236555=CARTESIAN_POINT('Ctrl Pts',(45.8515213356259,33.0454780259863,-44.3322613658288));
#236556=CARTESIAN_POINT('Ctrl Pts',(45.4177261184771,33.3403443524165,-44.3017465667526));
#236557=CARTESIAN_POINT('Ctrl Pts',(45.1768228991778,33.4430640954207,-44.2865805896286));
#236558=CARTESIAN_POINT('Ctrl Pts',(44.6734851563212,33.5498467323824,-44.258038405184));
#236559=CARTESIAN_POINT('Ctrl Pts',(44.4161796862212,33.5545630193631,-44.2457253680806));
#236560=CARTESIAN_POINT('Ctrl Pts',(43.9022440434096,33.4650792961969,-44.2171523490041));
#236561=CARTESIAN_POINT('Ctrl Pts',(43.6514052987463,33.3672998390698,-44.2016285392052));
#236562=CARTESIAN_POINT('Ctrl Pts',(43.2113823922517,33.0846862629223,-44.1711565006768));
#236563=CARTESIAN_POINT('Ctrl Pts',(43.0242473671213,32.9058857393626,-44.1564877704071));
#236564=CARTESIAN_POINT('Ctrl Pts',(42.7245661986959,32.4828630659587,-44.1290102713141));
#236565=CARTESIAN_POINT('Ctrl Pts',(42.6166049835928,32.2414781966625,-44.1158431692384));
#236566=CARTESIAN_POINT('Ctrl Pts',(42.4995716529647,31.7294384786342,-44.0859741856868));
#236567=CARTESIAN_POINT('Ctrl Pts',(42.4921606566817,31.463720544598,-44.070473972868));
#236568=CARTESIAN_POINT('Ctrl Pts',(42.5790686739269,30.9541411633263,-44.0407485089605));
#236569=CARTESIAN_POINT('Ctrl Pts',(42.6688901519482,30.7145457254872,-44.0271004103369));
#236570=CARTESIAN_POINT('Ctrl Pts',(42.9391868848949,30.2718796653486,-44.0005344264075));
#236571=CARTESIAN_POINT('Ctrl Pts',(43.1209684281317,30.0753491108694,-43.9856190182295));
#236572=CARTESIAN_POINT('Ctrl Pts',(43.5465056506158,29.7675167644448,-43.9551432221714));
#236573=CARTESIAN_POINT('Ctrl Pts',(43.7850432714683,29.6576092639034,-43.939887107773));
#236574=CARTESIAN_POINT('Ctrl Pts',(44.1921841661629,29.5591720533483,-43.9164480182645));
#236575=CARTESIAN_POINT('Ctrl Pts',(44.3499432647089,29.5404524382925,-43.9079323319158));
#236576=CARTESIAN_POINT('Ctrl Pts',(44.5079524583209,29.5404524382925,-43.89995));
#236577=CARTESIAN_POINT('Ctrl Pts',(44.5079524241436,29.5404524382925,-43.7412000017266));
#236578=CARTESIAN_POINT('Ctrl Pts',(44.3803294603659,29.5404524404734,-43.7476472776332));
#236579=CARTESIAN_POINT('Ctrl Pts',(44.2527261738062,29.552665552809,-43.754449775196));
#236580=CARTESIAN_POINT('Ctrl Pts',(43.8725994012209,29.6264475978516,-43.7758050522766));
#236581=CARTESIAN_POINT('Ctrl Pts',(43.6303461307986,29.7247231950921,-43.7909096105657));
#236582=CARTESIAN_POINT('Ctrl Pts',(43.1916672495306,30.0115026419363,-43.8214352559901));
#236583=CARTESIAN_POINT('Ctrl Pts',(43.0007627119394,30.1992902156302,-43.8365565373459));
#236584=CARTESIAN_POINT('Ctrl Pts',(42.7100359367441,30.6285242246839,-43.8637628410279));
#236585=CARTESIAN_POINT('Ctrl Pts',(42.6091249039369,30.8632454746232,-43.8766962604526));
#236586=CARTESIAN_POINT('Ctrl Pts',(42.4983798358489,31.3664931807484,-43.9060523766432));
#236587=CARTESIAN_POINT('Ctrl Pts',(42.4928967333233,31.6309557211211,-43.9214793581649));
#236588=CARTESIAN_POINT('Ctrl Pts',(42.5848914825434,32.150843351761,-43.9518061366189));
#236589=CARTESIAN_POINT('Ctrl Pts',(42.6829966663639,32.4008099978702,-43.9657670410182));
#236590=CARTESIAN_POINT('Ctrl Pts',(42.9654575479,32.8388874305972,-43.9928137002469));
#236591=CARTESIAN_POINT('Ctrl Pts',(43.1436679299149,33.0250093423903,-44.00724511456));
#236592=CARTESIAN_POINT('Ctrl Pts',(43.5685156767946,33.3259059398677,-44.0374837869095));
#236593=CARTESIAN_POINT('Ctrl Pts',(43.8133949851612,33.4346525615901,-44.0530264126543));
#236594=CARTESIAN_POINT('Ctrl Pts',(44.3232693350104,33.5484317331885,-44.0821028799755));
#236595=CARTESIAN_POINT('Ctrl Pts',(44.5825690326208,33.5555248442344,-44.094529879345));
#236596=CARTESIAN_POINT('Ctrl Pts',(45.0909771812048,33.4709483696994,-44.1226805315619));
#236597=CARTESIAN_POINT('Ctrl Pts',(45.3351637700046,33.3795900699776,-44.1376810030051));
#236598=CARTESIAN_POINT('Ctrl Pts',(45.7811116310906,33.1055021349579,-44.1682036947369));
#236599=CARTESIAN_POINT('Ctrl Pts',(45.977200356899,32.9230817842003,-44.1834303276808));
#236600=CARTESIAN_POINT('Ctrl Pts',(46.2798872528161,32.5019380996975,-44.2110048667188));
#236601=CARTESIAN_POINT('Ctrl Pts',(46.3873266523313,32.2699612592433,-44.2236453187778));
#236602=CARTESIAN_POINT('Ctrl Pts',(46.5117827927508,31.7705185615192,-44.2527794761451));
#236603=CARTESIAN_POINT('Ctrl Pts',(46.5246684048428,31.5070611576783,-44.2681478247025));
#236604=CARTESIAN_POINT('Ctrl Pts',(46.4478414140236,30.986227172029,-44.2985298071987));
#236605=CARTESIAN_POINT('Ctrl Pts',(46.3573542415884,30.7342562999992,-44.3129523666769));
#236606=CARTESIAN_POINT('Ctrl Pts',(46.0889152695432,30.2892942828932,-44.3394914653767));
#236607=CARTESIAN_POINT('Ctrl Pts',(45.916967928119,30.0984158729122,-44.353745213672));
#236608=CARTESIAN_POINT('Ctrl Pts',(45.502919501942,29.7854643750258,-44.3837899255959));
#236609=CARTESIAN_POINT('Ctrl Pts',(45.2623788433696,29.6694109472359,-44.3993264859628));
#236610=CARTESIAN_POINT('Ctrl Pts',(44.8430821442132,29.5615471791281,-44.4236546054688));
#236611=CARTESIAN_POINT('Ctrl Pts',(44.6756872488009,29.5404524382924,-44.4327263489368));
#236612=CARTESIAN_POINT('Ctrl Pts',(44.5079524583206,29.5404524382925,-44.4412));
#236613=CARTESIAN_POINT('Origin',(44.5079524583208,31.5404524382925,235.35105));
#236614=CARTESIAN_POINT('',(44.5079524583209,29.5404524382925,-43.0412));
#236615=CARTESIAN_POINT('',(44.507952458321,29.5404524382925,-43.19995));
#236616=CARTESIAN_POINT('',(44.5079524583208,29.5404524382925,235.35105));
#236617=CARTESIAN_POINT('Ctrl Pts',(44.5079524583209,29.5404524382925,-43.89995));
#236618=CARTESIAN_POINT('Ctrl Pts',(44.603059908934,29.5404524382925,-43.8951453476813));
#236619=CARTESIAN_POINT('Ctrl Pts',(44.6982377848346,29.547235565763,-43.8901392963898));
#236620=CARTESIAN_POINT('Ctrl Pts',(45.0574337791752,29.5989155974678,-43.8704860455296));
#236621=CARTESIAN_POINT('Ctrl Pts',(45.3117580344694,29.689679706868,-43.8549907684955));
#236622=CARTESIAN_POINT('Ctrl Pts',(45.7608770804952,29.9604869064725,-43.8244035624881));
#236623=CARTESIAN_POINT('Ctrl Pts',(45.9534396256205,30.1344968411654,-43.8096003694657));
#236624=CARTESIAN_POINT('Ctrl Pts',(46.2637198088779,30.5480801576235,-43.7818627423445));
#236625=CARTESIAN_POINT('Ctrl Pts',(46.3776550531411,30.7843111631185,-43.769058241052));
#236626=CARTESIAN_POINT('Ctrl Pts',(46.5098623795721,31.291290795844,-43.739484429143));
#236627=CARTESIAN_POINT('Ctrl Pts',(46.5252340649997,31.5574746018566,-43.7239570404589));
#236628=CARTESIAN_POINT('Ctrl Pts',(46.4530799665626,32.0706154970375,-43.6940238215734));
#236629=CARTESIAN_POINT('Ctrl Pts',(46.3700330713194,32.3133027105304,-43.679867067453));
#236630=CARTESIAN_POINT('Ctrl Pts',(46.1121178894357,32.76391200395,-43.6535815253368));
#236631=CARTESIAN_POINT('Ctrl Pts',(45.9360480411527,32.9655352087732,-43.6388631639973));
#236632=CARTESIAN_POINT('Ctrl Pts',(45.5187506415874,33.2858295266088,-43.6084401543713));
#236633=CARTESIAN_POINT('Ctrl Pts',(45.2827087082266,33.4026601704208,-43.5931081924722));
#236634=CARTESIAN_POINT('Ctrl Pts',(44.7860837297113,33.5371928248204,-43.5640957489453));
#236635=CARTESIAN_POINT('Ctrl Pts',(44.5309508061643,33.5563352546136,-43.5515750827623));
#236636=CARTESIAN_POINT('Ctrl Pts',(44.0155060442822,33.4969435221183,-43.5238035088456));
#236637=CARTESIAN_POINT('Ctrl Pts',(43.7606844094674,33.4144629094121,-43.508524707106));
#236638=CARTESIAN_POINT('Ctrl Pts',(43.3044851377979,33.1585308360496,-43.4780136790564));
#236639=CARTESIAN_POINT('Ctrl Pts',(43.1060554657483,32.9900126717666,-43.4630742662814));
#236640=CARTESIAN_POINT('Ctrl Pts',(42.7841720446195,32.5869171958619,-43.4350563604152));
#236641=CARTESIAN_POINT('Ctrl Pts',(42.6637568048127,32.3562078867747,-43.4225357344948));
#236642=CARTESIAN_POINT('Ctrl Pts',(42.5151465049839,31.8549482478058,-43.3932955888883));
#236643=CARTESIAN_POINT('Ctrl Pts',(42.4910596025346,31.5885214446032,-43.3777540253681));
#236644=CARTESIAN_POINT('Ctrl Pts',(42.5470143797582,31.0717170336357,-43.347607101395));
#236645=CARTESIAN_POINT('Ctrl Pts',(42.6226692072067,30.8257900127035,-43.3332613585073));
#236646=CARTESIAN_POINT('Ctrl Pts',(42.8681218263821,30.3646852855505,-43.3063635827567));
#236647=CARTESIAN_POINT('Ctrl Pts',(43.0398239167052,30.1562018617983,-43.2920764939474));
#236648=CARTESIAN_POINT('Ctrl Pts',(43.4505880991027,29.8227809092919,-43.2616006701789));
#236649=CARTESIAN_POINT('Ctrl Pts',(43.6840525405724,29.6993630562494,-43.2462067914622));
#236650=CARTESIAN_POINT('Ctrl Pts',(44.1209885676691,29.5686285361039,-43.2203205021658));
#236651=CARTESIAN_POINT('Ctrl Pts',(44.3140975965614,29.5404524382925,-43.2097431887043));
#236652=CARTESIAN_POINT('Ctrl Pts',(44.5079524583211,29.5404524382925,-43.19995));
#236653=CARTESIAN_POINT('Ctrl Pts',(44.507952458321,29.5404524382925,-43.0412));
#236654=CARTESIAN_POINT('Ctrl Pts',(44.3428859486929,29.5404524382925,-43.0495388544547));
#236655=CARTESIAN_POINT('Ctrl Pts',(44.1781468636118,29.5608813377326,-43.0584570109277));
#236656=CARTESIAN_POINT('Ctrl Pts',(43.7649541967093,29.6654079696292,-43.0823794328861));
#236657=CARTESIAN_POINT('Ctrl Pts',(43.5273568621061,29.7779947973286,-43.0976661928062));
#236658=CARTESIAN_POINT('Ctrl Pts',(43.1050131171097,30.0906239217968,-43.1281205663205));
#236659=CARTESIAN_POINT('Ctrl Pts',(42.9254061612222,30.2891170907883,-43.1429833612949));
#236660=CARTESIAN_POINT('Ctrl Pts',(42.6598793539486,30.7348529120131,-43.1693979121089));
#236661=CARTESIAN_POINT('Ctrl Pts',(42.5726418801136,30.9756224182398,-43.1832515821635));
#236662=CARTESIAN_POINT('Ctrl Pts',(42.4913795134358,31.486646825032,-43.2130613392264));
#236663=CARTESIAN_POINT('Ctrl Pts',(42.5018432963734,31.7525710885968,-43.2285735879343));
#236664=CARTESIAN_POINT('Ctrl Pts',(42.624719030887,32.2626892444508,-43.2583304803591));
#236665=CARTESIAN_POINT('Ctrl Pts',(42.7349791408251,32.5020849505867,-43.2713469521728));
#236666=CARTESIAN_POINT('Ctrl Pts',(43.0387262026938,32.9215023104342,-43.298924697696));
#236667=CARTESIAN_POINT('Ctrl Pts',(43.2279501527227,33.0984906909758,-43.3136461024127));
#236668=CARTESIAN_POINT('Ctrl Pts',(43.6714863524154,33.3766246271964,-43.3441649698443));
#236669=CARTESIAN_POINT('Ctrl Pts',(43.9236795714655,33.4717364109192,-43.3596793980406));
#236670=CARTESIAN_POINT('Ctrl Pts',(44.4385215547572,33.555409714008,-43.3881287331745));
#236671=CARTESIAN_POINT('Ctrl Pts',(44.6953769497797,33.5478762279429,-43.4004518111039));
#236672=CARTESIAN_POINT('Ctrl Pts',(45.197449818442,33.4357242928857,-43.4290867009739));
#236673=CARTESIAN_POINT('Ctrl Pts',(45.4374779135517,33.3302642656819,-43.4442883933999));
#236674=CARTESIAN_POINT('Ctrl Pts',(45.8681775614868,33.03043806965,-43.4747914729141));
#236675=CARTESIAN_POINT('Ctrl Pts',(46.053507925471,32.8372080082199,-43.4897898965651));
#236676=CARTESIAN_POINT('Ctrl Pts',(46.3316672499433,32.3996557394439,-43.5166039318131));
#236677=CARTESIAN_POINT('Ctrl Pts',(46.4257506445691,32.1619652677515,-43.5299450849482));
#236678=CARTESIAN_POINT('Ctrl Pts',(46.5218971753613,31.6547961984845,-43.5595299473221));
#236679=CARTESIAN_POINT('Ctrl Pts',(46.5194842072782,31.3894908419828,-43.575006093118));
#236680=CARTESIAN_POINT('Ctrl Pts',(46.4120838797738,30.8743568889704,-43.6050555737104));
#236681=CARTESIAN_POINT('Ctrl Pts',(46.3079122710583,30.6296804578189,-43.6185002122192));
#236682=CARTESIAN_POINT('Ctrl Pts',(46.014894866714,30.200790903147,-43.6458121876587));
#236683=CARTESIAN_POINT('Ctrl Pts',(45.8311998526572,30.0190893402774,-43.6603917485845));
#236684=CARTESIAN_POINT('Ctrl Pts',(45.396995209647,29.7292679042007,-43.6907800884619));
#236685=CARTESIAN_POINT('Ctrl Pts',(45.1484211192914,29.6271804045484,-43.7063151433583));
#236686=CARTESIAN_POINT('Ctrl Pts',(44.7618975791812,29.5525429758403,-43.7280185219813));
#236687=CARTESIAN_POINT('Ctrl Pts',(44.6349332753986,29.5404524361225,-43.7347851641561));
#236688=CARTESIAN_POINT('Ctrl Pts',(44.5079524241435,29.5404524382925,-43.7412000017266));
#236689=CARTESIAN_POINT('Origin',(44.5079524583208,31.5404524382925,235.35105));
#236690=CARTESIAN_POINT('',(44.507952458321,29.5404524382925,-42.3412));
#236691=CARTESIAN_POINT('',(44.5079524583208,29.5404524382925,-42.49995));
#236692=CARTESIAN_POINT('',(44.5079524583208,29.5404524382925,235.35105));
#236693=CARTESIAN_POINT('Ctrl Pts',(44.5079524583211,29.5404524382925,-43.19995));
#236694=CARTESIAN_POINT('Ctrl Pts',(44.5665991045952,29.5404524382925,-43.1969872800113));
#236695=CARTESIAN_POINT('Ctrl Pts',(44.6253064126613,29.5430318780239,-43.1939462618424));
#236696=CARTESIAN_POINT('Ctrl Pts',(44.9481088323641,29.5715417421349,-43.176807343547));
#236697=CARTESIAN_POINT('Ctrl Pts',(45.2050074234444,29.6471957029399,-43.1616227285026));
#236698=CARTESIAN_POINT('Ctrl Pts',(45.6684267639518,29.8911636944158,-43.1310959083313));
#236699=CARTESIAN_POINT('Ctrl Pts',(45.8717274789806,30.0548560670756,-43.1160511717391));
#236700=CARTESIAN_POINT('Ctrl Pts',(46.203386444063,30.4489875554122,-43.0878008731286));
#236701=CARTESIAN_POINT('Ctrl Pts',(46.3292265161237,30.6751460267372,-43.0754262073408));
#236702=CARTESIAN_POINT('Ctrl Pts',(46.4914873929182,31.1714524684933,-43.0464749982383));
#236703=CARTESIAN_POINT('Ctrl Pts',(46.5229035490332,31.437869230895,-43.0309340204315));
#236704=CARTESIAN_POINT('Ctrl Pts',(46.480645147573,31.9573565188901,-43.0006305952985));
#236705=CARTESIAN_POINT('Ctrl Pts',(46.4112771461008,32.2058257980606,-42.9861365540135));
#236706=CARTESIAN_POINT('Ctrl Pts',(46.1786137650572,32.6713828596358,-42.958979058755));
#236707=CARTESIAN_POINT('Ctrl Pts',(46.0143711622087,32.8824162231044,-42.9452442068107));
#236708=CARTESIAN_POINT('Ctrl Pts',(45.6150407712465,33.2266213567624,-42.9150314583995));
#236709=CARTESIAN_POINT('Ctrl Pts',(45.3845803766436,33.3571348728264,-42.8995823817306));
#236710=CARTESIAN_POINT('Ctrl Pts',(44.8949905975828,33.5189286620772,-42.8701302270217));
#236711=CARTESIAN_POINT('Ctrl Pts',(44.6416231755321,33.5519820788101,-42.8570390783313));
#236712=CARTESIAN_POINT('Ctrl Pts',(44.1241290834013,33.5211110601426,-42.829995830198));
#236713=CARTESIAN_POINT('Ctrl Pts',(43.8652150613394,33.4528260772934,-42.8149243278356));
#236714=CARTESIAN_POINT('Ctrl Pts',(43.3944144468747,33.221897208872,-42.7844049271258));
#236715=CARTESIAN_POINT('Ctrl Pts',(43.1860250669658,33.0635256619809,-42.7692583113568));
#236716=CARTESIAN_POINT('Ctrl Pts',(42.8439847575439,32.6790416055694,-42.7407649498819));
#236717=CARTESIAN_POINT('Ctrl Pts',(42.7124082776733,32.4576181754678,-42.7284513346686));
#236718=CARTESIAN_POINT('Ctrl Pts',(42.5358196918728,31.9666908278183,-42.6998139060558));
#236719=CARTESIAN_POINT('Ctrl Pts',(42.4966476923776,31.7004968805927,-42.6842859258009));
#236720=CARTESIAN_POINT('Ctrl Pts',(42.524340301447,31.178564329912,-42.6538398603445));
#236721=CARTESIAN_POINT('Ctrl Pts',(42.5869861387273,30.9275852584862,-42.6391994145114));
#236722=CARTESIAN_POINT('Ctrl Pts',(42.8062031762079,30.4574517210543,-42.6117749581612));
#236723=CARTESIAN_POINT('Ctrl Pts',(42.9627882462913,30.2437875024397,-42.5985227745748));
#236724=CARTESIAN_POINT('Ctrl Pts',(43.3501233460486,29.8885876489612,-42.5685953267386));
#236725=CARTESIAN_POINT('Ctrl Pts',(43.5772339468994,29.7507639672093,-42.5531022622821));
#236726=CARTESIAN_POINT('Ctrl Pts',(44.0437613891552,29.5811257564053,-42.5245863785012));
#236727=CARTESIAN_POINT('Ctrl Pts',(44.2750608700149,29.5404524382925,-42.511715251855));
#236728=CARTESIAN_POINT('Ctrl Pts',(44.5079524583208,29.5404524382925,-42.49995));
#236729=CARTESIAN_POINT('Ctrl Pts',(44.5079524583211,29.5404524382925,-42.3412));
#236730=CARTESIAN_POINT('Ctrl Pts',(44.3067852482428,29.5404524382925,-42.3513625950029));
#236731=CARTESIAN_POINT('Ctrl Pts',(44.1064975352776,29.5707947521519,-42.3623657435942));
#236732=CARTESIAN_POINT('Ctrl Pts',(43.6637830034297,29.7085277257708,-42.3887480738117));
#236733=CARTESIAN_POINT('Ctrl Pts',(43.4314436034151,29.8346697873297,-42.4041645735987));
#236734=CARTESIAN_POINT('Ctrl Pts',(43.02504561223,30.1722454089543,-42.4345410033202));
#236735=CARTESIAN_POINT('Ctrl Pts',(42.8562112397984,30.3817086260739,-42.4486066109538));
#236736=CARTESIAN_POINT('Ctrl Pts',(42.6156402274143,30.8445243871565,-42.4756041970169));
#236737=CARTESIAN_POINT('Ctrl Pts',(42.5423722700094,31.091439238053,-42.4900075633192));
#236738=CARTESIAN_POINT('Ctrl Pts',(42.4916260697972,31.6093081936101,-42.5202165857267));
#236739=CARTESIAN_POINT('Ctrl Pts',(42.5185044057893,31.8757541979105,-42.5357592693109));
#236740=CARTESIAN_POINT('Ctrl Pts',(42.6723278910724,32.3751426374909,-42.5648902616198));
#236741=CARTESIAN_POINT('Ctrl Pts',(42.7948106555084,32.6041089980684,-42.5773452309046));
#236742=CARTESIAN_POINT('Ctrl Pts',(43.120414414186,33.0038070068886,-42.6054519885459));
#236743=CARTESIAN_POINT('Ctrl Pts',(43.3207062234586,33.1705099476173,-42.6204325290254));
#236744=CARTESIAN_POINT('Ctrl Pts',(43.7796827487293,33.4219256547043,-42.6509521314353));
#236745=CARTESIAN_POINT('Ctrl Pts',(44.0353147676662,33.5018217336608,-42.666196490046));
#236746=CARTESIAN_POINT('Ctrl Pts',(44.5511784166266,33.5559845339382,-42.6938367148393));
#236747=CARTESIAN_POINT('Ctrl Pts',(44.8059645593044,33.5343048854853,-42.7064343232118));
#236748=CARTESIAN_POINT('Ctrl Pts',(45.3013478971403,33.3948318195729,-42.7355281366863));
#236749=CARTESIAN_POINT('Ctrl Pts',(45.5364369445363,33.2755056929497,-42.7508847454659));
#236750=CARTESIAN_POINT('Ctrl Pts',(45.9506404016502,32.9507645573285,-42.7812811536996));
#236751=CARTESIAN_POINT('Ctrl Pts',(46.1246470852223,32.7473180417129,-42.795799506467));
#236752=CARTESIAN_POINT('Ctrl Pts',(46.3780443384741,32.2937985562453,-42.822254809786));
#236753=CARTESIAN_POINT('Ctrl Pts',(46.4586171008651,32.0499961352609,-42.8364766176767));
#236754=CARTESIAN_POINT('Ctrl Pts',(46.5253375612345,31.5355664158354,-42.8664850179766));
#236755=CARTESIAN_POINT('Ctrl Pts',(46.5070368788851,31.2692699282744,-42.8820189797509));
#236756=CARTESIAN_POINT('Ctrl Pts',(46.3692941445005,30.764191883341,-42.9114818657054));
#236757=CARTESIAN_POINT('Ctrl Pts',(46.2531756622305,30.5298303795275,-42.9241776983054));
#236758=CARTESIAN_POINT('Ctrl Pts',(45.9389970183727,30.1197526296116,-42.9520100227475));
#236759=CARTESIAN_POINT('Ctrl Pts',(45.7444537874955,29.9475590727496,-42.9668602986604));
#236760=CARTESIAN_POINT('Ctrl Pts',(45.2920419459663,29.6811989986307,-42.9974841427735));
#236761=CARTESIAN_POINT('Ctrl Pts',(45.0364736653742,29.5930647429175,-43.0129655615965));
#236762=CARTESIAN_POINT('Ctrl Pts',(44.6836956983711,29.5462378354539,-43.0321530361411));
#236763=CARTESIAN_POINT('Ctrl Pts',(44.5957863231696,29.5404524382925,-43.0367627957675));
#236764=CARTESIAN_POINT('Ctrl Pts',(44.507952458321,29.5404524382925,-43.0412));
#236765=CARTESIAN_POINT('Origin',(44.5079524583208,31.5404524382925,235.35105));
#236766=CARTESIAN_POINT('',(44.5079524583208,29.5404524382925,-41.6412));
#236767=CARTESIAN_POINT('',(44.5079524583208,29.5404524382925,-41.79995));
#236768=CARTESIAN_POINT('',(44.5079524583208,29.5404524382925,235.35105));
#236769=CARTESIAN_POINT('Ctrl Pts',(44.5079524583208,29.5404524382925,-42.49995));
#236770=CARTESIAN_POINT('Ctrl Pts',(44.5281915482536,29.5404524382925,-42.4989275586482));
#236771=CARTESIAN_POINT('Ctrl Pts',(44.5484417718872,29.540759652605,-42.497895594425));
#236772=CARTESIAN_POINT('Ctrl Pts',(44.8337286956703,29.5494283529019,-42.4832305901368));
#236773=CARTESIAN_POINT('Ctrl Pts',(45.0944824477049,29.610105155334,-42.4682880532845));
#236774=CARTESIAN_POINT('Ctrl Pts',(45.5724645023405,29.8274378483818,-42.4378024146283));
#236775=CARTESIAN_POINT('Ctrl Pts',(45.7859274646337,29.9801957566941,-42.422563221996));
#236776=CARTESIAN_POINT('Ctrl Pts',(46.1385233715512,30.354731520291,-42.3938267698192));
#236777=CARTESIAN_POINT('Ctrl Pts',(46.2759191572335,30.5714415107971,-42.3814756374373));
#236778=CARTESIAN_POINT('Ctrl Pts',(46.4669005030961,31.0567856226139,-42.3531638975813));
#236779=CARTESIAN_POINT('Ctrl Pts',(46.5139163692276,31.3225329220241,-42.3376619717824));
#236780=CARTESIAN_POINT('Ctrl Pts',(46.5010299700797,31.8465280017547,-42.3070955921314));
#236781=CARTESIAN_POINT('Ctrl Pts',(46.4452548083671,32.0998571912959,-42.2923180560748));
#236782=CARTESIAN_POINT('Ctrl Pts',(46.23956736931,32.5744893336426,-42.2646311811046));
#236783=CARTESIAN_POINT('Ctrl Pts',(46.0904999084609,32.7907659112026,-42.2517632242203));
#236784=CARTESIAN_POINT('Ctrl Pts',(45.7151930054219,33.1566867337951,-42.2221307236802));
#236785=CARTESIAN_POINT('Ctrl Pts',(45.4916386210013,33.3017007381006,-42.2066075949526));
#236786=CARTESIAN_POINT('Ctrl Pts',(45.0101917985323,33.4929784639923,-42.1767068591824));
#236787=CARTESIAN_POINT('Ctrl Pts',(44.7583465761211,33.5409006655415,-42.162612520535));
#236788=CARTESIAN_POINT('Ctrl Pts',(44.2392900816279,33.5399780585633,-42.136363838068));
#236789=CARTESIAN_POINT('Ctrl Pts',(43.9769576015324,33.486801213419,-42.1215602955512));
#236790=CARTESIAN_POINT('Ctrl Pts',(43.4923247293002,33.2830028017046,-42.0911334197759));
#236791=CARTESIAN_POINT('Ctrl Pts',(43.2740359223536,33.1358969078494,-42.0758152848281));
#236792=CARTESIAN_POINT('Ctrl Pts',(42.9111780813867,32.7711782445811,-42.0468467508355));
#236793=CARTESIAN_POINT('Ctrl Pts',(42.7681190298049,32.5589509546727,-42.0343624134556));
#236794=CARTESIAN_POINT('Ctrl Pts',(42.5643848417266,32.081662414282,-42.0065205819328));
#236795=CARTESIAN_POINT('Ctrl Pts',(42.5098289559704,31.8194338258323,-41.9912239142732));
#236796=CARTESIAN_POINT('Ctrl Pts',(42.5062223419112,31.2964890670197,-41.9607188033425));
#236797=CARTESIAN_POINT('Ctrl Pts',(42.5542911162574,31.0407740716014,-41.9458020952764));
#236798=CARTESIAN_POINT('Ctrl Pts',(42.7450244417216,30.5612921769914,-41.9178323180909));
#236799=CARTESIAN_POINT('Ctrl Pts',(42.8859943698823,30.3421493374886,-41.9052711458869));
#236800=CARTESIAN_POINT('Ctrl Pts',(43.2480710190736,29.9647613371827,-41.8759725539261));
#236801=CARTESIAN_POINT('Ctrl Pts',(43.467493951482,29.8120037073267,-41.8604322827597));
#236802=CARTESIAN_POINT('Ctrl Pts',(43.9439239948383,29.6047886635623,-41.830320146944));
#236803=CARTESIAN_POINT('Ctrl Pts',(44.1949022099252,29.5487278530391,-41.8160060852168));
#236804=CARTESIAN_POINT('Ctrl Pts',(44.4691115548922,29.5407351434851,-41.8019204160975));
#236805=CARTESIAN_POINT('Ctrl Pts',(44.4885374707127,29.5404524382925,-41.8009308092281));
#236806=CARTESIAN_POINT('Ctrl Pts',(44.5079524583208,29.5404524382925,-41.79995));
#236807=CARTESIAN_POINT('Ctrl Pts',(44.5079524583208,29.5404524382925,-41.6412));
#236808=CARTESIAN_POINT('Ctrl Pts',(44.2672514934039,29.5404524382925,-41.6533597671028));
#236809=CARTESIAN_POINT('Ctrl Pts',(44.0283515184313,29.5839018714322,-41.6666958266611));
#236810=CARTESIAN_POINT('Ctrl Pts',(43.5562868000569,29.7617686632792,-41.69573144366));
#236811=CARTESIAN_POINT('Ctrl Pts',(43.3305491677514,29.9024320466283,-41.7112379729174));
#236812=CARTESIAN_POINT('Ctrl Pts',(42.9479362256659,30.2618758672077,-41.7410506484646));
#236813=CARTESIAN_POINT('Ctrl Pts',(42.7943210334294,30.4765676682521,-41.7541400550808));
#236814=CARTESIAN_POINT('Ctrl Pts',(42.5804091612362,30.9484777886012,-41.7816681454345));
#236815=CARTESIAN_POINT('Ctrl Pts',(42.5204451959738,31.2003996722857,-41.7963635886494));
#236816=CARTESIAN_POINT('Ctrl Pts',(42.4985416134286,31.7231890228391,-41.8268596340984));
#236817=CARTESIAN_POINT('Ctrl Pts',(42.5407852138562,31.9892345588435,-41.842378957032));
#236818=CARTESIAN_POINT('Ctrl Pts',(42.7230203528376,32.4779932068023,-41.8708898781629));
#236819=CARTESIAN_POINT('Ctrl Pts',(42.8568716981678,32.6975615073306,-41.8832061380639));
#236820=CARTESIAN_POINT('Ctrl Pts',(43.2030381015716,33.0781745372596,-41.9117950372284));
#236821=CARTESIAN_POINT('Ctrl Pts',(43.4134232315287,33.2343761643763,-41.9269791852681));
#236822=CARTESIAN_POINT('Ctrl Pts',(43.8870707998596,33.4600306290821,-41.9574885720412));
#236823=CARTESIAN_POINT('Ctrl Pts',(44.1467295085273,33.5253551614776,-41.9725113481206));
#236824=CARTESIAN_POINT('Ctrl Pts',(44.664577292091,33.5503314990797,-41.9994005358924));
#236825=CARTESIAN_POINT('Ctrl Pts',(44.9176184749323,33.5143764221844,-42.0126561191544));
#236826=CARTESIAN_POINT('Ctrl Pts',(45.4056701495064,33.3468502962067,-42.0421977648269));
#236827=CARTESIAN_POINT('Ctrl Pts',(45.634857478873,33.2134903728229,-42.0576655488106));
#236828=CARTESIAN_POINT('Ctrl Pts',(46.029544062124,32.8649914031207,-42.0877689375386));
#236829=CARTESIAN_POINT('Ctrl Pts',(46.1908023739995,32.6529352518331,-42.10130516921));
#236830=CARTESIAN_POINT('Ctrl Pts',(46.4182646419594,32.1855953946261,-42.1285666608804));
#236831=CARTESIAN_POINT('Ctrl Pts',(46.4850456536318,31.9361351339568,-42.1431185094195));
#236832=CARTESIAN_POINT('Ctrl Pts',(46.5216889813397,31.4156558332057,-42.1734798019633));
#236833=CARTESIAN_POINT('Ctrl Pts',(46.4872782951218,31.1492992840176,-42.1890172673326));
#236834=CARTESIAN_POINT('Ctrl Pts',(46.31947278005,30.6550538068162,-42.2178482535027));
#236835=CARTESIAN_POINT('Ctrl Pts',(46.1914177283946,30.4307314959853,-42.2301879788846));
#236836=CARTESIAN_POINT('Ctrl Pts',(45.8557565048388,30.0403046812106,-42.2585324112043));
#236837=CARTESIAN_POINT('Ctrl Pts',(45.6504828371936,29.8786401490778,-42.2736176723612));
#236838=CARTESIAN_POINT('Ctrl Pts',(45.1841813937079,29.6396597414361,-42.3041446198437));
#236839=CARTESIAN_POINT('Ctrl Pts',(44.9264820266832,29.5668330656511,-42.3192872261264));
#236840=CARTESIAN_POINT('Ctrl Pts',(44.6107093301824,29.5424301869479,-42.3359512287464));
#236841=CARTESIAN_POINT('Ctrl Pts',(44.5593051412479,29.5404524382925,-42.3386057575353));
#236842=CARTESIAN_POINT('Ctrl Pts',(44.5079524583211,29.5404524382925,-42.3412));
#236843=CARTESIAN_POINT('Origin',(44.5079524583208,31.5404524382925,235.35105));
#236844=CARTESIAN_POINT('',(44.5079524583208,29.5404524382925,-40.9412));
#236845=CARTESIAN_POINT('',(44.5079524583206,29.5404524382925,-41.09995));
#236846=CARTESIAN_POINT('',(44.5079524583208,29.5404524382925,235.35105));
#236847=CARTESIAN_POINT('Ctrl Pts',(44.5079524583208,29.5404524382925,-41.79995));
#236848=CARTESIAN_POINT('Ctrl Pts',(44.753283869434,29.5404524382925,-41.7875563113284));
#236849=CARTESIAN_POINT('Ctrl Pts',(44.9967396162526,29.58558799845,-41.7739409239064));
#236850=CARTESIAN_POINT('Ctrl Pts',(45.4701984701951,29.7677506117743,-41.7447095829667));
#236851=CARTESIAN_POINT('Ctrl Pts',(45.693504501057,29.908624585447,-41.7293197514945));
#236852=CARTESIAN_POINT('Ctrl Pts',(46.0673014950109,30.2627124837551,-41.7001086557242));
#236853=CARTESIAN_POINT('Ctrl Pts',(46.2164182255828,30.4702627635807,-41.6873777310249));
#236854=CARTESIAN_POINT('Ctrl Pts',(46.4342882217952,30.9408037405067,-41.6599295073709));
#236855=CARTESIAN_POINT('Ctrl Pts',(46.4967302934578,31.2012315980501,-41.6447378823475));
#236856=CARTESIAN_POINT('Ctrl Pts',(46.5161707857634,31.7245417365144,-41.6142114576038));
#236857=CARTESIAN_POINT('Ctrl Pts',(46.4755905046121,31.9823295990548,-41.5991738322889));
#236858=CARTESIAN_POINT('Ctrl Pts',(46.2991994999433,32.4663423599117,-41.5709397545723));
#236859=CARTESIAN_POINT('Ctrl Pts',(46.1657958992151,32.6882311279318,-41.5585576361121));
#236860=CARTESIAN_POINT('Ctrl Pts',(45.8163303102628,33.0762557531885,-41.5295858966716));
#236861=CARTESIAN_POINT('Ctrl Pts',(45.6010513151848,33.2362292669554,-41.5140445062661));
#236862=CARTESIAN_POINT('Ctrl Pts',(45.1297039593719,33.4584532284062,-41.4837513783156));
#236863=CARTESIAN_POINT('Ctrl Pts',(44.8797674055392,33.5221428655078,-41.4692674319445));
#236864=CARTESIAN_POINT('Ctrl Pts',(44.3600710535679,33.5524997240187,-41.4421279260594));
#236865=CARTESIAN_POINT('Ctrl Pts',(44.095084372802,33.5152425638956,-41.4283573807194));
#236866=CARTESIAN_POINT('Ctrl Pts',(43.5975734914173,33.340450392492,-41.3981259471071));
#236867=CARTESIAN_POINT('Ctrl Pts',(43.369633415828,33.2056893646584,-41.3826803065285));
#236868=CARTESIAN_POINT('Ctrl Pts',(42.9854456376923,32.8618668253909,-41.3532436938847));
#236869=CARTESIAN_POINT('Ctrl Pts',(42.8305419303208,32.6586702709936,-41.3401793735744));
#236870=CARTESIAN_POINT('Ctrl Pts',(42.5994453267602,32.1946166682982,-41.3131095800838));
#236871=CARTESIAN_POINT('Ctrl Pts',(42.5296341191085,31.9361069541665,-41.2980298467594));
#236872=CARTESIAN_POINT('Ctrl Pts',(42.495261037926,31.412894521579,-41.2675091215251));
#236873=CARTESIAN_POINT('Ctrl Pts',(42.5287171011554,31.1533528012335,-41.2523691878383));
#236874=CARTESIAN_POINT('Ctrl Pts',(42.6916071169511,30.6651803505833,-41.2238924615504));
#236875=CARTESIAN_POINT('Ctrl Pts',(42.8180545809363,30.4407001078993,-41.2115777357079));
#236876=CARTESIAN_POINT('Ctrl Pts',(43.1557309418803,30.042969513371,-41.1829184754688));
#236877=CARTESIAN_POINT('Ctrl Pts',(43.3669616425938,29.8763993374101,-41.1673891947521));
#236878=CARTESIAN_POINT('Ctrl Pts',(43.8331823775542,29.6403626770763,-41.1369521838113));
#236879=CARTESIAN_POINT('Ctrl Pts',(44.0819474833038,29.5696116631542,-41.1223214600046));
#236880=CARTESIAN_POINT('Ctrl Pts',(44.3941587347587,29.5428775963385,-41.1057693820078));
#236881=CARTESIAN_POINT('Ctrl Pts',(44.4510868615659,29.5404524382925,-41.1028227446645));
#236882=CARTESIAN_POINT('Ctrl Pts',(44.5079524583204,29.5404524382924,-41.09995));
#236883=CARTESIAN_POINT('Ctrl Pts',(44.5079524583207,29.5404524382925,-40.9412));
#236884=CARTESIAN_POINT('Ctrl Pts',(44.4816990227574,29.5404524382925,-40.9425262749579));
#236885=CARTESIAN_POINT('Ctrl Pts',(44.4554265546438,29.5409693663035,-40.9438685884719));
#236886=CARTESIAN_POINT('Ctrl Pts',(44.1742025575873,29.5520585347067,-40.9583989382106));
#236887=CARTESIAN_POINT('Ctrl Pts',(43.9235644051612,29.6108031890804,-40.9727740993808));
#236888=CARTESIAN_POINT('Ctrl Pts',(43.448868722049,29.8233085901873,-41.0029529206172));
#236889=CARTESIAN_POINT('Ctrl Pts',(43.230876575762,29.978615301625,-41.0184952593305));
#236890=CARTESIAN_POINT('Ctrl Pts',(42.8732223925083,30.3597649017264,-41.0476801498274));
#236891=CARTESIAN_POINT('Ctrl Pts',(42.7349219704941,30.5798681249784,-41.0601659150567));
#236892=CARTESIAN_POINT('Ctrl Pts',(42.5492075747699,31.0609489748742,-41.0882289646339));
#236893=CARTESIAN_POINT('Ctrl Pts',(42.5037491863373,31.3174136321222,-41.1031894029734));
#236894=CARTESIAN_POINT('Ctrl Pts',(42.5128914807453,31.8405411036034,-41.1337051721431));
#236895=CARTESIAN_POINT('Ctrl Pts',(42.5702129101642,32.1021675131214,-41.1489667126983));
#236896=CARTESIAN_POINT('Ctrl Pts',(42.7789038315715,32.5771121942379,-41.1766718190968));
#236897=CARTESIAN_POINT('Ctrl Pts',(42.9240730637951,32.7876963277406,-41.1892299588978));
#236898=CARTESIAN_POINT('Ctrl Pts',(43.2907472347089,33.148726136872,-41.2182836952346));
#236899=CARTESIAN_POINT('Ctrl Pts',(43.5108018640736,33.2936819270355,-41.233628324904));
#236900=CARTESIAN_POINT('Ctrl Pts',(43.9980058766551,33.4924456941335,-41.2640382461281));
#236901=CARTESIAN_POINT('Ctrl Pts',(44.260932027402,33.5427496462346,-41.2786539832764));
#236902=CARTESIAN_POINT('Ctrl Pts',(44.7802678792263,33.5380892918405,-41.3050257959915));
#236903=CARTESIAN_POINT('Ctrl Pts',(45.0318308817501,33.4872993287206,-41.3192156670481));
#236904=CARTESIAN_POINT('Ctrl Pts',(45.5114979339958,33.2905061605134,-41.3491873591893));
#236905=CARTESIAN_POINT('Ctrl Pts',(45.7336456823359,33.1427878180178,-41.364718303797));
#236906=CARTESIAN_POINT('Ctrl Pts',(46.1043659850929,32.7728543315175,-41.3942361338133));
#236907=CARTESIAN_POINT('Ctrl Pts',(46.2506066901437,32.5555843884028,-41.4069839695767));
#236908=CARTESIAN_POINT('Ctrl Pts',(46.4511194586139,32.0792595436652,-41.4347695855198));
#236909=CARTESIAN_POINT('Ctrl Pts',(46.5042405839542,31.82507926019,-41.4495967687225));
#236910=CARTESIAN_POINT('Ctrl Pts',(46.5114289970589,31.3004026013653,-41.4802029071539));
#236911=CARTESIAN_POINT('Ctrl Pts',(46.4614050940075,31.0348855798487,-41.4956914000758));
#236912=CARTESIAN_POINT('Ctrl Pts',(46.2649253314838,30.5517220087559,-41.5238759417228));
#236913=CARTESIAN_POINT('Ctrl Pts',(46.1252870630233,30.3367996096282,-41.5362684576805));
#236914=CARTESIAN_POINT('Ctrl Pts',(45.7686251759153,29.9661360534585,-41.5650973762653));
#236915=CARTESIAN_POINT('Ctrl Pts',(45.5532369682635,29.8155948501023,-41.5803691748342));
#236916=CARTESIAN_POINT('Ctrl Pts',(45.0725796557155,29.6035881876034,-41.6108346200093));
#236917=CARTESIAN_POINT('Ctrl Pts',(44.8111752277478,29.545871382327,-41.6257236945546));
#236918=CARTESIAN_POINT('Ctrl Pts',(44.533371567733,29.5405735432228,-41.6399123414273));
#236919=CARTESIAN_POINT('Ctrl Pts',(44.5206596789984,29.5404524382925,-41.6405580547381));
#236920=CARTESIAN_POINT('Ctrl Pts',(44.5079524583208,29.5404524382925,-41.6412));
#236921=CARTESIAN_POINT('Origin',(44.5079524583208,31.5404524382925,235.35105));
#236922=CARTESIAN_POINT('',(44.5079524583206,29.5404524382925,-40.2412));
#236923=CARTESIAN_POINT('',(44.5079524583207,29.5404524382925,-40.39995));
#236924=CARTESIAN_POINT('',(44.5079524583208,29.5404524382925,235.35105));
#236925=CARTESIAN_POINT('Ctrl Pts',(44.5079524583204,29.5404524382925,-41.09995));
#236926=CARTESIAN_POINT('Ctrl Pts',(44.7127884447251,29.5404524382924,-41.0896020652096));
#236927=CARTESIAN_POINT('Ctrl Pts',(44.9167205496817,29.5719115854782,-41.078382234377));
#236928=CARTESIAN_POINT('Ctrl Pts',(45.3633783085636,29.7135852641125,-41.0516857624007));
#236929=CARTESIAN_POINT('Ctrl Pts',(45.5959805326658,29.8418092860262,-41.0361952613837));
#236930=CARTESIAN_POINT('Ctrl Pts',(45.9909489883467,30.1747975453953,-41.0065300287005));
#236931=CARTESIAN_POINT('Ctrl Pts',(46.1519040618263,30.3735580889598,-40.9930188370445));
#236932=CARTESIAN_POINT('Ctrl Pts',(46.3965269748775,30.8308081927069,-40.9663459143259));
#236933=CARTESIAN_POINT('Ctrl Pts',(46.473849762942,31.0871228318008,-40.9513942270455));
#236934=CARTESIAN_POINT('Ctrl Pts',(46.5235842739099,31.6097873306858,-40.9209054646105));
#236935=CARTESIAN_POINT('Ctrl Pts',(46.4975203039116,31.8709296573216,-40.9056721622234));
#236936=CARTESIAN_POINT('Ctrl Pts',(46.3485189858338,32.363275640451,-40.8769519798742));
#236937=CARTESIAN_POINT('Ctrl Pts',(46.2290714930095,32.5904360952347,-40.8646065570797));
#236938=CARTESIAN_POINT('Ctrl Pts',(45.9034293848198,32.9978564570087,-40.8362726267976));
#236939=CARTESIAN_POINT('Ctrl Pts',(45.6964973846956,33.1710083951975,-40.8207685404109));
#236940=CARTESIAN_POINT('Ctrl Pts',(45.2358707299797,33.4209180536095,-40.7902095029363));
#236941=CARTESIAN_POINT('Ctrl Pts',(44.9884931356865,33.4988014136315,-40.7754408468782));
#236942=CARTESIAN_POINT('Ctrl Pts',(44.4744103511585,33.557050459181,-40.7477714059051));
#236943=CARTESIAN_POINT('Ctrl Pts',(44.212477323953,33.5355728713584,-40.7348808225659));
#236944=CARTESIAN_POINT('Ctrl Pts',(43.7081385544689,33.3924547954086,-40.7052282844723));
#236945=CARTESIAN_POINT('Ctrl Pts',(43.4710669440809,33.2709075220833,-40.6897067368354));
#236946=CARTESIAN_POINT('Ctrl Pts',(43.0654031441697,32.9488661305975,-40.6598204788102));
#236947=CARTESIAN_POINT('Ctrl Pts',(42.8983842260015,32.7544370551136,-40.6457657693148));
#236948=CARTESIAN_POINT('Ctrl Pts',(42.64052838135,32.30400417371,-40.6194905178995));
#236949=CARTESIAN_POINT('Ctrl Pts',(42.5558954333463,32.0500645319282,-40.6046773721289));
#236950=CARTESIAN_POINT('Ctrl Pts',(42.4910710393704,31.5283806464918,-40.5742458121451));
#236951=CARTESIAN_POINT('Ctrl Pts',(42.5098104533401,31.2658675908542,-40.5589325505662));
#236952=CARTESIAN_POINT('Ctrl Pts',(42.645142236704,30.7695248525269,-40.5299792241638));
#236953=CARTESIAN_POINT('Ctrl Pts',(42.7578483998159,30.539696308703,-40.5175066296998));
#236954=CARTESIAN_POINT('Ctrl Pts',(43.0717451965258,30.1230227740392,-40.4894961665986));
#236955=CARTESIAN_POINT('Ctrl Pts',(43.2743287784446,29.9436007811549,-40.4740288776534));
#236956=CARTESIAN_POINT('Ctrl Pts',(43.7291590812721,29.6803859546179,-40.4433745937409));
#236957=CARTESIAN_POINT('Ctrl Pts',(43.9750015604766,29.5956233620597,-40.4284828445726));
#236958=CARTESIAN_POINT('Ctrl Pts',(44.3224079897582,29.5469011967279,-40.409511451814));
#236959=CARTESIAN_POINT('Ctrl Pts',(44.4152191380681,29.5404524382925,-40.4046347156484));
#236960=CARTESIAN_POINT('Ctrl Pts',(44.5079524583206,29.5404524382925,-40.39995));
#236961=CARTESIAN_POINT('Ctrl Pts',(44.5079524583204,29.5404524382925,-40.2412));
#236962=CARTESIAN_POINT('Ctrl Pts',(44.4461937530077,29.5404524382925,-40.2443199354495));
#236963=CARTESIAN_POINT('Ctrl Pts',(44.3843665227043,29.5433128801535,-40.2475267622089));
#236964=CARTESIAN_POINT('Ctrl Pts',(44.0672753494251,29.5728160956729,-40.2644061316585));
#236965=CARTESIAN_POINT('Ctrl Pts',(43.818862770905,29.6454834042868,-40.2790749383708));
#236966=CARTESIAN_POINT('Ctrl Pts',(43.3541037750594,29.885255197537,-40.3095470463346));
#236967=CARTESIAN_POINT('Ctrl Pts',(43.1440072234425,30.0536017892691,-40.3250708440654));
#236968=CARTESIAN_POINT('Ctrl Pts',(42.8095507615993,30.4539465413159,-40.3536436872243));
#236969=CARTESIAN_POINT('Ctrl Pts',(42.6849862659914,30.679139208081,-40.3659567282376));
#236970=CARTESIAN_POINT('Ctrl Pts',(42.5258014009256,31.1684360756242,-40.394499045511));
#236971=CARTESIAN_POINT('Ctrl Pts',(42.4943116988828,31.4284251490941,-40.4096650747967));
#236972=CARTESIAN_POINT('Ctrl Pts',(42.5327841504894,31.9515357506962,-40.4401798598902));
#236973=CARTESIAN_POINT('Ctrl Pts',(42.6046067820175,32.2094816692934,-40.4552267051417));
#236974=CARTESIAN_POINT('Ctrl Pts',(42.8393199349264,32.6717327757373,-40.4821913530176));
#236975=CARTESIAN_POINT('Ctrl Pts',(42.995827829265,32.8737419397183,-40.4953645404819));
#236976=CARTESIAN_POINT('Ctrl Pts',(43.3828828207437,33.2147017651451,-40.524862503615));
#236977=CARTESIAN_POINT('Ctrl Pts',(43.612077751551,33.3477433963758,-40.5403213880883));
#236978=CARTESIAN_POINT('Ctrl Pts',(44.1105508779273,33.5183219887893,-40.5704785364822));
#236979=CARTESIAN_POINT('Ctrl Pts',(44.3751222469798,33.5534614761425,-40.5841102333803));
#236980=CARTESIAN_POINT('Ctrl Pts',(44.8941011422762,33.5194230807133,-40.6113208728427));
#236981=CARTESIAN_POINT('Ctrl Pts',(45.143747689986,33.4538681268884,-40.6258445737125));
#236982=CARTESIAN_POINT('Ctrl Pts',(45.6137803908419,33.227987954367,-40.6561779272182));
#236983=CARTESIAN_POINT('Ctrl Pts',(45.8280099452777,33.0662641489134,-40.6717173519996));
#236984=CARTESIAN_POINT('Ctrl Pts',(46.1743724328927,32.6756638086287,-40.7006074535274));
#236985=CARTESIAN_POINT('Ctrl Pts',(46.3059352902341,32.4530950791237,-40.7129625126182));
#236986=CARTESIAN_POINT('Ctrl Pts',(46.4787821253612,31.9679809190841,-40.7412608386205));
#236987=CARTESIAN_POINT('Ctrl Pts',(46.5174988314685,31.7097139650406,-40.7563264109397));
#236988=CARTESIAN_POINT('Ctrl Pts',(46.4941399869417,31.186387959989,-40.7868537612344));
#236989=CARTESIAN_POINT('Ctrl Pts',(46.4297578284954,30.926442816073,-40.8020172279628));
#236990=CARTESIAN_POINT('Ctrl Pts',(46.2084083392178,30.4575923617246,-40.8293668377998));
#236991=CARTESIAN_POINT('Ctrl Pts',(46.0577809710145,30.2511892981575,-40.842175707883));
#236992=CARTESIAN_POINT('Ctrl Pts',(45.6812650408056,29.8997713426122,-40.8714462859484));
#236993=CARTESIAN_POINT('Ctrl Pts',(45.4567336356385,29.7604789049286,-40.8868518929288));
#236994=CARTESIAN_POINT('Ctrl Pts',(44.9865042082021,29.5836942426894,-40.9157632323138));
#236995=CARTESIAN_POINT('Ctrl Pts',(44.74808715979,29.5404524382924,-40.9290688394782));
#236996=CARTESIAN_POINT('Ctrl Pts',(44.5079524583207,29.5404524382925,-40.9412));
#236997=CARTESIAN_POINT('Origin',(44.5079524583208,31.5404524382925,235.35105));
#236998=CARTESIAN_POINT('',(44.5079524583208,29.5404524382925,-39.5412));
#236999=CARTESIAN_POINT('',(44.5079524583208,29.5404524382925,-39.69995));
#237000=CARTESIAN_POINT('',(44.5079524583208,29.5404524382925,235.35105));
#237001=CARTESIAN_POINT('',(45.8699699536314,30.0759011606612,-39.4567768040287));
#237002=CARTESIAN_POINT('Ctrl Pts',(45.8699695685728,30.075901520304,-39.4567761523991));
#237003=CARTESIAN_POINT('Ctrl Pts',(45.7701107830075,29.9830338890879,-39.4645294726065));
#237004=CARTESIAN_POINT('Ctrl Pts',(45.6610194473437,29.9006263473464,-39.4724441182083));
#237005=CARTESIAN_POINT('Ctrl Pts',(45.4275260895439,29.7591440756338,-39.4883663366023));
#237006=CARTESIAN_POINT('Ctrl Pts',(45.3036963603113,29.7004880778269,-39.4963327851952));
#237007=CARTESIAN_POINT('Ctrl Pts',(44.9604389072844,29.5790802543851,-39.5172145777165));
#237008=CARTESIAN_POINT('Ctrl Pts',(44.7349169043735,29.5404524382924,-39.5297341763978));
#237009=CARTESIAN_POINT('Ctrl Pts',(44.5079524583207,29.5404524382925,-39.5412));
#237010=CARTESIAN_POINT('',(46.1726017293051,30.4318753540615,-39.5898550790525));
#237011=CARTESIAN_POINT('Ctrl Pts',(45.8699698689079,30.0759017996126,-39.4567779390767));
#237012=CARTESIAN_POINT('Ctrl Pts',(45.9271083068064,30.129039973996,-39.4791532819239));
#237013=CARTESIAN_POINT('Ctrl Pts',(45.981085284682,30.1854725512665,-39.5015086752499));
#237014=CARTESIAN_POINT('Ctrl Pts',(46.0821973535923,30.3043921848593,-39.5459690352455));
#237015=CARTESIAN_POINT('Ctrl Pts',(46.129270885215,30.3668095284313,-39.5680428991861));
#237016=CARTESIAN_POINT('Ctrl Pts',(46.1726016483627,30.4318753890564,-39.5898550650905));
#237017=CARTESIAN_POINT('Ctrl Pts',(44.5079524583208,29.5404524382925,-39.69995));
#237018=CARTESIAN_POINT('Ctrl Pts',(44.6319808972993,29.5404524382925,-39.6936843128947));
#237019=CARTESIAN_POINT('Ctrl Pts',(44.7560060404353,29.5519873437279,-39.6870823575476));
#237020=CARTESIAN_POINT('Ctrl Pts',(45.1400567254562,29.6243843292702,-39.6655692492444));
#237021=CARTESIAN_POINT('Ctrl Pts',(45.3891835300754,29.7254372108916,-39.6500364486059));
#237022=CARTESIAN_POINT('Ctrl Pts',(45.8337542537958,30.019451126976,-39.6190021528564));
#237023=CARTESIAN_POINT('Ctrl Pts',(46.024657531644,30.2097211747746,-39.6038085296457));
#237024=CARTESIAN_POINT('Ctrl Pts',(46.1726016676276,30.4318754179848,-39.5898551670461));
#237025=CARTESIAN_POINT('Origin',(-44.5079524583208,31.5404524382925,235.35105));
#237026=CARTESIAN_POINT('',(-44.5079524583208,29.5404524382925,-52.3162000000004));
#237027=CARTESIAN_POINT('',(-44.5079524583208,29.5404524382925,-52.4749499999996));
#237028=CARTESIAN_POINT('',(-44.5079524583208,29.5404524382925,235.35105));
#237029=CARTESIAN_POINT('',(-46.5079524583208,31.5404524382925,-52.64995));
#237030=CARTESIAN_POINT('Ctrl Pts',(-46.5079524583208,31.5404524382925,
-52.6499499999996));
#237031=CARTESIAN_POINT('Ctrl Pts',(-46.5079524583208,31.2923954725884,
-52.6374186213562));
#237032=CARTESIAN_POINT('Ctrl Pts',(-46.4618041379609,31.0465391623049,
-52.6236524230731));
#237033=CARTESIAN_POINT('Ctrl Pts',(-46.2794036058753,30.577598336436,-52.5946423852496));
#237034=CARTESIAN_POINT('Ctrl Pts',(-46.1422160174819,30.3596409234275,
-52.5796302756193));
#237035=CARTESIAN_POINT('Ctrl Pts',(-45.7889072840913,29.9823693960786,
-52.5502663784982));
#237036=CARTESIAN_POINT('Ctrl Pts',(-45.5743499468127,29.8283664394868,
-52.5371565201615));
#237037=CARTESIAN_POINT('Ctrl Pts',(-45.1026718366126,29.6137589726646,
-52.5096419637332));
#237038=CARTESIAN_POINT('Ctrl Pts',(-44.8508720180615,29.5534424514737,
-52.4949536409844));
#237039=CARTESIAN_POINT('Ctrl Pts',(-44.5657020983325,29.5410772302566,
-52.4783187290003));
#237040=CARTESIAN_POINT('Ctrl Pts',(-44.5368153039993,29.5404524382925,
-52.4766336659975));
#237041=CARTESIAN_POINT('Ctrl Pts',(-44.5079524583208,29.5404524382925,
-52.4749499999996));
#237042=CARTESIAN_POINT('',(-44.7865238868864,33.5209569091754,-52.64995));
#237043=CARTESIAN_POINT('Origin',(-44.5079524583208,31.5404524382925,-52.64995));
#237044=CARTESIAN_POINT('Ctrl Pts',(-44.5079524583208,29.5404524382925,
-52.3162000000005));
#237045=CARTESIAN_POINT('Ctrl Pts',(-44.7127351905467,29.5404524382925,
-52.3281456593803));
#237046=CARTESIAN_POINT('Ctrl Pts',(-44.9166514162594,29.5719068831819,
-52.3400407725471));
#237047=CARTESIAN_POINT('Ctrl Pts',(-45.3553832799493,29.7110280003146,
-52.3656334645957));
#237048=CARTESIAN_POINT('Ctrl Pts',(-45.581284963268,29.8337345445251,-52.3779519699644));
#237049=CARTESIAN_POINT('Ctrl Pts',(-45.9842037250954,30.1650012258081,
-52.4064387466005));
#237050=CARTESIAN_POINT('Ctrl Pts',(-46.1542990722659,30.3739626070849,
-52.4219562029942));
#237051=CARTESIAN_POINT('Ctrl Pts',(-46.3977544226486,30.8372481514485,
-52.4524613120001));
#237052=CARTESIAN_POINT('Ctrl Pts',(-46.4723144406481,31.0852979527207,
-52.4671669959012));
#237053=CARTESIAN_POINT('Ctrl Pts',(-46.5240542552125,31.6007273814734,
-52.4947146142767));
#237054=CARTESIAN_POINT('Ctrl Pts',(-46.4989470904135,31.8633519585254,
-52.5077749424954));
#237055=CARTESIAN_POINT('Ctrl Pts',(-46.3484897234824,32.3661902348615,
-52.5375657411067));
#237056=CARTESIAN_POINT('Ctrl Pts',(-46.2238224665166,32.6012088871632,
-52.5530745766248));
#237057=CARTESIAN_POINT('Ctrl Pts',(-45.899615045655,32.9983157068768,-52.5825917277099));
#237058=CARTESIAN_POINT('Ctrl Pts',(-45.707401438058,33.1601177057035,-52.5962321428486));
#237059=CARTESIAN_POINT('Ctrl Pts',(-45.2727931896581,33.405262303546,-52.6215842906718));
#237060=CARTESIAN_POINT('Ctrl Pts',(-45.0339917549731,33.4861488698347,
-52.6355143743617));
#237061=CARTESIAN_POINT('Ctrl Pts',(-44.7865238868852,33.5209569091755,
-52.6499500000001));
#237062=CARTESIAN_POINT('Origin',(-44.5079524583208,31.5404524382925,235.35105));
#237063=CARTESIAN_POINT('',(-44.5079524583208,29.5404524382925,-51.6162000000004));
#237064=CARTESIAN_POINT('',(-44.5079524583208,29.5404524382925,-51.7749499999997));
#237065=CARTESIAN_POINT('',(-44.5079524583208,29.5404524382925,235.35105));
#237066=CARTESIAN_POINT('Ctrl Pts',(-44.5079524583208,29.5404524382925,
-52.4749499999996));
#237067=CARTESIAN_POINT('Ctrl Pts',(-44.2706710647853,29.5404524382925,
-52.4611085853768));
#237068=CARTESIAN_POINT('Ctrl Pts',(-44.0350082364426,29.5826825426037,
-52.4473615870568));
#237069=CARTESIAN_POINT('Ctrl Pts',(-43.5730800140031,29.754114096945,-52.4204157740813));
#237070=CARTESIAN_POINT('Ctrl Pts',(-43.3532689868484,29.8876666859978,
-52.4081007415779));
#237071=CARTESIAN_POINT('Ctrl Pts',(-42.9721462304376,30.233291144132,-52.3795243534628));
#237072=CARTESIAN_POINT('Ctrl Pts',(-42.8156577993954,30.443415036027,-52.3643450375719));
#237073=CARTESIAN_POINT('Ctrl Pts',(-42.5893075901103,30.916691541608,-52.3338341036518));
#237074=CARTESIAN_POINT('Ctrl Pts',(-42.5235932041223,31.176254293647,-52.3188048043939));
#237075=CARTESIAN_POINT('Ctrl Pts',(-42.4978414783645,31.6940568751854,
-52.2918952846569));
#237076=CARTESIAN_POINT('Ctrl Pts',(-42.5334142479843,31.9471402165956,
-52.2786622508692));
#237077=CARTESIAN_POINT('Ctrl Pts',(-42.7001843791251,32.4353959452518,
-52.2491323466117));
#237078=CARTESIAN_POINT('Ctrl Pts',(-42.8331696097481,32.6647531256922,
-52.2336669106051));
#237079=CARTESIAN_POINT('Ctrl Pts',(-43.1811043150024,33.0600529371203,
-52.203549000438));
#237080=CARTESIAN_POINT('Ctrl Pts',(-43.3930257525339,33.2217038791566,
-52.1899873911714));
#237081=CARTESIAN_POINT('Ctrl Pts',(-43.8601310007166,33.4498532621196,
-52.1627395850274));
#237082=CARTESIAN_POINT('Ctrl Pts',(-44.1094617907247,33.5169770097097,
-52.1481952889435));
#237083=CARTESIAN_POINT('Ctrl Pts',(-44.6298133586672,33.5543635583677,
-52.1178414474801));
#237084=CARTESIAN_POINT('Ctrl Pts',(-44.8961797354773,33.5203488950871,
-52.1023034088328));
#237085=CARTESIAN_POINT('Ctrl Pts',(-45.3906990097786,33.3532756557018,
-52.0734564511651));
#237086=CARTESIAN_POINT('Ctrl Pts',(-45.615263401957,33.2255135713542,-52.0611129327868));
#237087=CARTESIAN_POINT('Ctrl Pts',(-46.006181641077,32.8903819778783,-52.0327809231879));
#237088=CARTESIAN_POINT('Ctrl Pts',(-46.1681162515263,32.6853686448247,
-52.0177009363683));
#237089=CARTESIAN_POINT('Ctrl Pts',(-46.407759615724,32.2194460560125,-51.9871737916894));
#237090=CARTESIAN_POINT('Ctrl Pts',(-46.4809614792731,31.9618509727281,
-51.9720255106516));
#237091=CARTESIAN_POINT('Ctrl Pts',(-46.5216593348524,31.4449987360713,
-51.9447280717919));
#237092=CARTESIAN_POINT('Ctrl Pts',(-46.493420758581,31.1910579788034,-51.9318753975487));
#237093=CARTESIAN_POINT('Ctrl Pts',(-46.3411075770592,30.6989699950747,
-51.9025735558905));
#237094=CARTESIAN_POINT('Ctrl Pts',(-46.2153268957618,30.4664793382221,
-51.8871599551457));
#237095=CARTESIAN_POINT('Ctrl Pts',(-45.8783013478925,30.0595004846572,
-51.8567702251501));
#237096=CARTESIAN_POINT('Ctrl Pts',(-45.6689680127052,29.8902859884014,
-51.8426759073385));
#237097=CARTESIAN_POINT('Ctrl Pts',(-45.2063790954135,29.6490654181459,
-51.8156915538299));
#237098=CARTESIAN_POINT('Ctrl Pts',(-44.9595944554625,29.5754789339219,
-51.8012957831661));
#237099=CARTESIAN_POINT('Ctrl Pts',(-44.6398630971928,29.5437110434508,
-51.7826447872671));
#237100=CARTESIAN_POINT('Ctrl Pts',(-44.5738684804503,29.5404524382925,
-51.7787951012905));
#237101=CARTESIAN_POINT('Ctrl Pts',(-44.5079524583208,29.5404524382925,
-51.7749499999997));
#237102=CARTESIAN_POINT('Ctrl Pts',(-44.5079524583208,29.5404524382925,
-51.6162000000004));
#237103=CARTESIAN_POINT('Ctrl Pts',(-44.7495896327406,29.5404524382925,
-51.6302955018416));
#237104=CARTESIAN_POINT('Ctrl Pts',(-44.9894048430363,29.5842459600337,
-51.6442847224424));
#237105=CARTESIAN_POINT('Ctrl Pts',(-45.456284003817,29.7608924187297,-51.6715193401547));
#237106=CARTESIAN_POINT('Ctrl Pts',(-45.6770188246547,29.897450543898,-51.6839630219098));
#237107=CARTESIAN_POINT('Ctrl Pts',(-46.0606183380932,30.2522024107171,
-51.7130727485595));
#237108=CARTESIAN_POINT('Ctrl Pts',(-46.2175870475827,30.4692423383284,
-51.7286154578915));
#237109=CARTESIAN_POINT('Ctrl Pts',(-46.433548589117,30.9427714748038,-51.7588361514474));
#237110=CARTESIAN_POINT('Ctrl Pts',(-46.4940496040989,31.1931715890985,
-51.7732505145562));
#237111=CARTESIAN_POINT('Ctrl Pts',(-46.5180988052615,31.7140804531209,
-51.8002673009658));
#237112=CARTESIAN_POINT('Ctrl Pts',(-46.4771874157357,31.9797855580725,
-51.8142916095523));
#237113=CARTESIAN_POINT('Ctrl Pts',(-46.2951539687465,32.4756025332761,
-51.8446486740316));
#237114=CARTESIAN_POINT('Ctrl Pts',(-46.1574664721582,32.7013583560729,
-51.8600693255417));
#237115=CARTESIAN_POINT('Ctrl Pts',(-45.8087475736808,33.0806111959291,
-51.8893994447173));
#237116=CARTESIAN_POINT('Ctrl Pts',(-45.6034934894683,33.2327616514278,
-51.9022934398498));
#237117=CARTESIAN_POINT('Ctrl Pts',(-45.1363498331127,33.4576002820923,
-51.9295434864704));
#237118=CARTESIAN_POINT('Ctrl Pts',(-44.8769044300919,33.5239269792106,
-51.9446778016465));
#237119=CARTESIAN_POINT('Ctrl Pts',(-44.3535922286762,33.551222433402,-51.975204346729));
#237120=CARTESIAN_POINT('Ctrl Pts',(-44.0948574742939,33.5143821643818,
-51.9902972074012));
#237121=CARTESIAN_POINT('Ctrl Pts',(-43.6086444486617,33.3450948666379,
-52.0186596338964));
#237122=CARTESIAN_POINT('Ctrl Pts',(-43.3853918009882,33.2153695035301,
-52.0309943100544));
#237123=CARTESIAN_POINT('Ctrl Pts',(-42.9922251533322,32.8721179323723,
-52.0598021044742));
#237124=CARTESIAN_POINT('Ctrl Pts',(-42.8287568054832,32.6589519911188,
-52.0753386799734));
#237125=CARTESIAN_POINT('Ctrl Pts',(-42.599226214873,32.1902621614667,-52.1057106646397));
#237126=CARTESIAN_POINT('Ctrl Pts',(-42.5318061633352,31.9409195204642,
-52.1202734113886));
#237127=CARTESIAN_POINT('Ctrl Pts',(-42.4940923139192,31.4226640461013,
-52.1475547057062));
#237128=CARTESIAN_POINT('Ctrl Pts',(-42.527128561288,31.1585040368843,-52.1610546290855));
#237129=CARTESIAN_POINT('Ctrl Pts',(-42.6935102234801,30.6590892925398,
-52.1911369358111));
#237130=CARTESIAN_POINT('Ctrl Pts',(-42.8248272762757,30.4286564703355,
-52.2066080560616));
#237131=CARTESIAN_POINT('Ctrl Pts',(-43.1629254864012,30.0387487135716,
-52.2361666718356));
#237132=CARTESIAN_POINT('Ctrl Pts',(-43.3637588445647,29.8806411062191,
-52.2494553725313));
#237133=CARTESIAN_POINT('Ctrl Pts',(-43.8242114769924,29.6423435096061,
-52.276315109423));
#237134=CARTESIAN_POINT('Ctrl Pts',(-44.0815819548725,29.5685293338514,
-52.2913283872994));
#237135=CARTESIAN_POINT('Ctrl Pts',(-44.3998220308925,29.5426422323627,
-52.309892391734));
#237136=CARTESIAN_POINT('Ctrl Pts',(-44.4539174098103,29.5404524382925,
-52.313047955504));
#237137=CARTESIAN_POINT('Ctrl Pts',(-44.5079524583208,29.5404524382925,
-52.3162000000005));
#237138=CARTESIAN_POINT('Origin',(-44.5079524583208,31.5404524382925,235.35105));
#237139=CARTESIAN_POINT('',(-44.5079524583208,29.5404524382925,-50.9162000000005));
#237140=CARTESIAN_POINT('',(-44.5079524583208,29.5404524382925,-51.0749499999997));
#237141=CARTESIAN_POINT('',(-44.5079524583208,29.5404524382925,235.35105));
#237142=CARTESIAN_POINT('Ctrl Pts',(-44.5079524583208,29.5404524382925,
-51.7749499999996));
#237143=CARTESIAN_POINT('Ctrl Pts',(-44.3097004477224,29.5404524382925,
-51.7633852993815));
#237144=CARTESIAN_POINT('Ctrl Pts',(-44.1121593984864,29.5699326646355,
-51.7518620715094));
#237145=CARTESIAN_POINT('Ctrl Pts',(-43.675780382826,29.7036747192049,-51.7264066289293));
#237146=CARTESIAN_POINT('Ctrl Pts',(-43.4465825171116,29.8258821762405,
-51.7139436252528));
#237147=CARTESIAN_POINT('Ctrl Pts',(-43.0464307373388,30.1509901224479,
-51.6858486801536));
#237148=CARTESIAN_POINT('Ctrl Pts',(-42.8794843611898,30.3510343371154,
-51.6708735474952));
#237149=CARTESIAN_POINT('Ctrl Pts',(-42.6274641193755,30.8096427930648,
-51.6403549070032));
#237150=CARTESIAN_POINT('Ctrl Pts',(-42.5472226233,31.0651682126213,-51.6251058589299));
#237151=CARTESIAN_POINT('Ctrl Pts',(-42.4923620277257,31.5809771092096,
-51.5974480477624));
#237152=CARTESIAN_POINT('Ctrl Pts',(-42.5137028025219,31.8358089353058,
-51.5848614182352));
#237153=CARTESIAN_POINT('Ctrl Pts',(-42.6525151090392,32.3313591732875,
-51.5557784454235));
#237154=CARTESIAN_POINT('Ctrl Pts',(-42.7715078345278,32.5665771817518,
-51.5404250459692));
#237155=CARTESIAN_POINT('Ctrl Pts',(-43.0956557171075,32.9811970848786,
-51.5100249028677));
#237156=CARTESIAN_POINT('Ctrl Pts',(-43.2988594490325,33.1554808273183,
-51.4954804255421));
#237157=CARTESIAN_POINT('Ctrl Pts',(-43.7519921956795,33.4094843772839,
-51.4690476819877));
#237158=CARTESIAN_POINT('Ctrl Pts',(-43.995646870312,33.4903889620451,-51.4548344926341));
#237159=CARTESIAN_POINT('Ctrl Pts',(-44.5099074369239,33.5578374719646,
-51.4248359595817));
#237160=CARTESIAN_POINT('Ctrl Pts',(-44.776190663482,33.539928907508,-51.4093027713657));
#237161=CARTESIAN_POINT('Ctrl Pts',(-45.2815245090258,33.4029258337993,
-51.3798249637089));
#237162=CARTESIAN_POINT('Ctrl Pts',(-45.5161354722425,33.2870992589641,
-51.3671153589855));
#237163=CARTESIAN_POINT('Ctrl Pts',(-45.9266836109983,32.9734425472894,
-51.3392956819162));
#237164=CARTESIAN_POINT('Ctrl Pts',(-46.0991220374941,32.7791639643163,
-51.3244516334945));
#237165=CARTESIAN_POINT('Ctrl Pts',(-46.366080736808,32.3271912353577,-51.2938325126338));
#237166=CARTESIAN_POINT('Ctrl Pts',(-46.4545686056881,32.0717882815627,
-51.2783491320971));
#237167=CARTESIAN_POINT('Ctrl Pts',(-46.5239606482487,31.5548230770405,
-51.2502090725229));
#237168=CARTESIAN_POINT('Ctrl Pts',(-46.5095061620318,31.2990209657207,
-51.2377986453606));
#237169=CARTESIAN_POINT('Ctrl Pts',(-46.3840578706243,30.8001501121403,
-51.2089377049707));
#237170=CARTESIAN_POINT('Ctrl Pts',(-46.2718308375706,30.5624246444881,
-51.1936549660167));
#237171=CARTESIAN_POINT('Ctrl Pts',(-45.9598446851843,30.1396483898485,
-51.1631974962684));
#237172=CARTESIAN_POINT('Ctrl Pts',(-45.7616139336562,29.959747807885,-51.1483275216909));
#237173=CARTESIAN_POINT('Ctrl Pts',(-45.3162899010547,29.6935789602594,
-51.1218925466886));
#237174=CARTESIAN_POINT('Ctrl Pts',(-45.0756792469387,29.6059936984791,
-51.1080673960021));
#237175=CARTESIAN_POINT('Ctrl Pts',(-44.7199342861136,29.5488717075795,
-51.0873156066207));
#237176=CARTESIAN_POINT('Ctrl Pts',(-44.6139049131048,29.5404524382925,
-51.081130559862));
#237177=CARTESIAN_POINT('Ctrl Pts',(-44.5079524583208,29.5404524382925,
-51.0749499999997));
#237178=CARTESIAN_POINT('Ctrl Pts',(-44.5079524583208,29.5404524382925,
-50.9162000000005));
#237179=CARTESIAN_POINT('Ctrl Pts',(-44.5308414227161,29.5404524382925,
-50.9175351895902));
#237180=CARTESIAN_POINT('Ctrl Pts',(-44.5537463650632,29.5408453642649,
-50.9188713112273));
#237181=CARTESIAN_POINT('Ctrl Pts',(-44.8332472937377,29.5504525720521,
-50.9351755320667));
#237182=CARTESIAN_POINT('Ctrl Pts',(-45.0857893570274,29.6085994744155,
-50.9499071524252));
#237183=CARTESIAN_POINT('Ctrl Pts',(-45.5588880169674,29.8189347221883,
-50.9775045742551));
#237184=CARTESIAN_POINT('Ctrl Pts',(-45.7742700740383,29.9705638419848,
-50.9904930651375));
#237185=CARTESIAN_POINT('Ctrl Pts',(-46.1365457455234,30.3499972378686,
-51.0202277115488));
#237186=CARTESIAN_POINT('Ctrl Pts',(-46.2791089307299,30.5747934763861,
-51.0357420942224));
#237187=CARTESIAN_POINT('Ctrl Pts',(-46.4653506019942,31.0576728823897,
-51.0655683165337));
#237188=CARTESIAN_POINT('Ctrl Pts',(-46.510741168321,31.3097515187281,-51.0794640792994));
#237189=CARTESIAN_POINT('Ctrl Pts',(-46.5047676255909,31.8285847441161,
-51.1058488015839));
#237190=CARTESIAN_POINT('Ctrl Pts',(-46.4490325421369,32.0904046450506,
-51.1207010648344));
#237191=CARTESIAN_POINT('Ctrl Pts',(-46.2406029881886,32.5728162555197,
-51.1511508015596));
#237192=CARTESIAN_POINT('Ctrl Pts',(-46.0915560582926,32.7894783483111,
-51.1664433714712));
#237193=CARTESIAN_POINT('Ctrl Pts',(-45.723486432103,33.1488506286628,-51.1953335578133));
#237194=CARTESIAN_POINT('Ctrl Pts',(-45.5097472355858,33.2899846489231,
-51.2077619713262));
#237195=CARTESIAN_POINT('Ctrl Pts',(-45.0280460202198,33.4901158075745,
-51.2358612088891));
#237196=CARTESIAN_POINT('Ctrl Pts',(-44.7627002581642,33.5421402081724,
-51.2513397116756));
#237197=CARTESIAN_POINT('Ctrl Pts',(-44.2376038870666,33.5387473638364,
-51.2819703333228));
#237198=CARTESIAN_POINT('Ctrl Pts',(-43.982872978989,33.4873971949234,-51.296829636294));
#237199=CARTESIAN_POINT('Ctrl Pts',(-43.5054319540045,33.2903226125284,
-51.3246803627514));
#237200=CARTESIAN_POINT('Ctrl Pts',(-43.2875030771622,33.1459455249636,
-51.3373565686951));
#237201=CARTESIAN_POINT('Ctrl Pts',(-42.9149297381558,32.7782678865303,
-51.3667976846411));
#237202=CARTESIAN_POINT('Ctrl Pts',(-42.7654289473987,32.55706837429,-51.382332714191));
#237203=CARTESIAN_POINT('Ctrl Pts',(-42.5649549535069,32.0785175276322,
-51.4123553751084));
#237204=CARTESIAN_POINT('Ctrl Pts',(-42.5123058678244,31.8271482438344,
-51.4265896842617));
#237205=CARTESIAN_POINT('Ctrl Pts',(-42.5039484084957,31.3076457237372,
-51.4530777489767));
#237206=CARTESIAN_POINT('Ctrl Pts',(-42.5523930990478,31.0443489439623,
-51.4675584153792));
#237207=CARTESIAN_POINT('Ctrl Pts',(-42.7477755310645,30.5555697799855,
-51.4979492880624));
#237208=CARTESIAN_POINT('Ctrl Pts',(-42.8912996606656,30.3343599251892,
-51.5133105208154));
#237209=CARTESIAN_POINT('Ctrl Pts',(-43.2498858906573,29.965169694845,-51.5424200927582));
#237210=CARTESIAN_POINT('Ctrl Pts',(-43.459393533305,29.8186075358262,-51.5550340627078));
#237211=CARTESIAN_POINT('Ctrl Pts',(-43.9327868878355,29.60666355077,-51.5826486750555));
#237212=CARTESIAN_POINT('Ctrl Pts',(-44.1940009390038,29.5475271107708,
-51.5978861613737));
#237213=CARTESIAN_POINT('Ctrl Pts',(-44.4753868222998,29.5406511842867,
-51.6143003378994));
#237214=CARTESIAN_POINT('Ctrl Pts',(-44.4916737747902,29.5404524382925,
-51.6152504101278));
#237215=CARTESIAN_POINT('Ctrl Pts',(-44.5079524583208,29.5404524382925,
-51.6162000000005));
#237216=CARTESIAN_POINT('Origin',(-44.5079524583208,31.5404524382925,235.35105));
#237217=CARTESIAN_POINT('',(-44.5079524583208,29.5404524382925,-50.2162000000005));
#237218=CARTESIAN_POINT('',(-44.5079524583208,29.5404524382925,-50.3749499999996));
#237219=CARTESIAN_POINT('',(-44.5079524583208,29.5404524382925,235.35105));
#237220=CARTESIAN_POINT('Ctrl Pts',(-44.5079524583208,29.5404524382925,
-51.0749499999997));
#237221=CARTESIAN_POINT('Ctrl Pts',(-44.3516039912595,29.5404524382925,
-51.0658296727544));
#237222=CARTESIAN_POINT('Ctrl Pts',(-44.1954230163498,29.5587866319509,
-51.0567191158846));
#237223=CARTESIAN_POINT('Ctrl Pts',(-43.788571375697,29.6561109667705,-51.0329861035133));
#237224=CARTESIAN_POINT('Ctrl Pts',(-43.5489082807268,29.7660616018213,
-51.0199501513565));
#237225=CARTESIAN_POINT('Ctrl Pts',(-43.1290035764768,30.0692603440578,
-50.9923858917143));
#237226=CARTESIAN_POINT('Ctrl Pts',(-42.9517689545595,30.2582030606817,
-50.9776715123485));
#237227=CARTESIAN_POINT('Ctrl Pts',(-42.6730273018941,30.7012671538275,
-50.9471587698027));
#237228=CARTESIAN_POINT('Ctrl Pts',(-42.5775540444165,30.9532789509942,
-50.9316429637197));
#237229=CARTESIAN_POINT('Ctrl Pts',(-42.493095495297,31.4679999066779,-50.9031768396673));
#237230=CARTESIAN_POINT('Ctrl Pts',(-42.5002483396806,31.7249154109233,
-50.8908559756066));
#237231=CARTESIAN_POINT('Ctrl Pts',(-42.6116732973496,32.2271604777061,
-50.8622335901137));
#237232=CARTESIAN_POINT('Ctrl Pts',(-42.7167625248647,32.4673089076121,
-50.8470366335875));
#237233=CARTESIAN_POINT('Ctrl Pts',(-43.0159187736098,32.8984312146818,
-50.8165317422456));
#237234=CARTESIAN_POINT('Ctrl Pts',(-43.2088712752572,33.0840540472864,
-50.8015266391149));
#237235=CARTESIAN_POINT('Ctrl Pts',(-43.6459960586556,33.3628659269626,
-50.7746921063096));
#237236=CARTESIAN_POINT('Ctrl Pts',(-43.8835300958586,33.4573032823413,
-50.7613746378106));
#237237=CARTESIAN_POINT('Ctrl Pts',(-44.3904975881245,33.5542128545749,
-50.7318015340951));
#237238=CARTESIAN_POINT('Ctrl Pts',(-44.6557646955364,33.5522127365159,
-50.716327619496));
#237239=CARTESIAN_POINT('Ctrl Pts',(-45.1711513253888,33.4456120628235,
-50.6862633994211));
#237240=CARTESIAN_POINT('Ctrl Pts',(-45.4161016075001,33.3417550836486,
-50.6727941244446));
#237241=CARTESIAN_POINT('Ctrl Pts',(-45.8454739110283,33.0492886426713,
-50.6454959024792));
#237242=CARTESIAN_POINT('Ctrl Pts',(-46.0274114976107,32.8658788848522,
-50.6309238681454));
#237243=CARTESIAN_POINT('Ctrl Pts',(-46.3178214003599,32.4321584913588,
-50.6005428280456));
#237244=CARTESIAN_POINT('Ctrl Pts',(-46.4202614959123,32.1837740555559,
-50.5850070700988));
#237245=CARTESIAN_POINT('Ctrl Pts',(-46.5199855615089,31.6714972722088,
-50.5562191768769));
#237246=CARTESIAN_POINT('Ctrl Pts',(-46.5202396738285,31.4133698957995,
-50.5438884023581));
#237247=CARTESIAN_POINT('Ctrl Pts',(-46.4228646160598,30.9078541416314,
-50.515510576541));
#237248=CARTESIAN_POINT('Ctrl Pts',(-46.3249538074677,30.6654938288931,
-50.5004112503412));
#237249=CARTESIAN_POINT('Ctrl Pts',(-46.0388405005334,30.2264215419042,
-50.4698851598688));
#237250=CARTESIAN_POINT('Ctrl Pts',(-45.8513328786031,30.0352391567394,
-50.4547580074278));
#237251=CARTESIAN_POINT('Ctrl Pts',(-45.422523382229,29.7438783769635,-50.4275320566281));
#237252=CARTESIAN_POINT('Ctrl Pts',(-45.1879495468724,29.6426221565203,
-50.4146164968316));
#237253=CARTESIAN_POINT('Ctrl Pts',(-44.798241208485,29.5562621223149,-50.3918835104257));
#237254=CARTESIAN_POINT('Ctrl Pts',(-44.6531392944108,29.5404524382925,
-50.3834192321049));
#237255=CARTESIAN_POINT('Ctrl Pts',(-44.5079524583208,29.5404524382925,
-50.3749499999996));
#237256=CARTESIAN_POINT('Ctrl Pts',(-44.5079524583208,29.5404524382925,
-50.2162000000005));
#237257=CARTESIAN_POINT('Ctrl Pts',(-44.5682680746908,29.5404524382925,
-50.2197184109554));
#237258=CARTESIAN_POINT('Ctrl Pts',(-44.6286552888035,29.543180850818,-50.2232409984454));
#237259=CARTESIAN_POINT('Ctrl Pts',(-44.9432382652611,29.5717642544572,
-50.2415916720722));
#237260=CARTESIAN_POINT('Ctrl Pts',(-45.1908258060872,29.6433670029181,
-50.2560342786204));
#237261=CARTESIAN_POINT('Ctrl Pts',(-45.6548201389246,29.8805514677881,
-50.2831006147026));
#237262=CARTESIAN_POINT('Ctrl Pts',(-45.864958208498,30.0474112649116,-50.2970203252533));
#237263=CARTESIAN_POINT('Ctrl Pts',(-46.2053881098655,30.4507815490265,
-50.3273270506451));
#237264=CARTESIAN_POINT('Ctrl Pts',(-46.3334086716835,30.68232470417,-50.3427581152063));
#237265=CARTESIAN_POINT('Ctrl Pts',(-46.4902011678538,31.1732393682324,
-50.3721313296043));
#237266=CARTESIAN_POINT('Ctrl Pts',(-46.5207172683144,31.426903935316,-50.3850914329009));
#237267=CARTESIAN_POINT('Ctrl Pts',(-46.4846744327701,31.9440684483801,
-50.4122688759687));
#237268=CARTESIAN_POINT('Ctrl Pts',(-46.4137986858253,32.2023003552664,
-50.427381483088));
#237269=CARTESIAN_POINT('Ctrl Pts',(-46.1782709362098,32.6705540875203,
-50.4579063540587));
#237270=CARTESIAN_POINT('Ctrl Pts',(-46.0180155913664,32.8771741937101,
-50.4730185335019));
#237271=CARTESIAN_POINT('Ctrl Pts',(-45.6301427936608,33.2155827944716,
-50.5014272660668));
#237272=CARTESIAN_POINT('Ctrl Pts',(-45.4070728232207,33.345156025004,-50.5137513120474));
#237273=CARTESIAN_POINT('Ctrl Pts',(-44.9142518287101,33.5167525737318,
-50.5424992033937));
#237274=CARTESIAN_POINT('Ctrl Pts',(-44.647955317031,33.5532158781841,-50.558033166575));
#237275=CARTESIAN_POINT('Ctrl Pts',(-44.1268308510684,33.520427817413,-50.588432093756));
#237276=CARTESIAN_POINT('Ctrl Pts',(-43.8767072715789,33.4554262072406,
-50.6030226358928));
#237277=CARTESIAN_POINT('Ctrl Pts',(-43.4081569945764,33.2315219641398,
-50.6303547353846));
#237278=CARTESIAN_POINT('Ctrl Pts',(-43.1954050869066,33.0722889103156,
-50.6437637558782));
#237279=CARTESIAN_POINT('Ctrl Pts',(-42.8439986947426,32.6807763605484,
-50.673791598133));
#237280=CARTESIAN_POINT('Ctrl Pts',(-42.7087051457558,32.452476521955,-50.6892709451393));
#237281=CARTESIAN_POINT('Ctrl Pts',(-42.5372706610271,31.9654857010376,
-50.7188729922463));
#237282=CARTESIAN_POINT('Ctrl Pts',(-42.4993407797864,31.7126583229252,
-50.7322493035807));
#237283=CARTESIAN_POINT('Ctrl Pts',(-42.5203182212263,31.194583721686,-50.7590333152903));
#237284=CARTESIAN_POINT('Ctrl Pts',(-42.5836301971647,30.9344397801151,
-50.7740219048743));
#237285=CARTESIAN_POINT('Ctrl Pts',(-42.8056873490928,30.4588951271366,
-50.804522207229));
#237286=CARTESIAN_POINT('Ctrl Pts',(-42.9604033279121,30.2471689693533,
-50.819730770103));
#237287=CARTESIAN_POINT('Ctrl Pts',(-43.3383849810633,29.8982114541963,
-50.8483839225765));
#237288=CARTESIAN_POINT('Ctrl Pts',(-43.5567076480399,29.7628215150986,
-50.8607107194007));
#237289=CARTESIAN_POINT('Ctrl Pts',(-44.0225681142928,29.584960108793,-50.8878859132655));
#237290=CARTESIAN_POINT('Ctrl Pts',(-44.2643554233246,29.5404524382925,
-50.901990172959));
#237291=CARTESIAN_POINT('Ctrl Pts',(-44.5079524583208,29.5404524382925,
-50.9162000000005));
#237292=CARTESIAN_POINT('Origin',(-44.5079524583208,31.5404524382925,235.35105));
#237293=CARTESIAN_POINT('',(-44.5079524583208,29.5404524382925,-49.5162000000005));
#237294=CARTESIAN_POINT('',(-44.5079524583208,29.5404524382925,-49.6749499999997));
#237295=CARTESIAN_POINT('',(-44.5079524583208,29.5404524382925,235.35105));
#237296=CARTESIAN_POINT('Ctrl Pts',(-44.5079524583208,29.5404524382925,
-50.3749499999996));
#237297=CARTESIAN_POINT('Ctrl Pts',(-44.3924091245316,29.5404524382925,
-50.3682099721953));
#237298=CARTESIAN_POINT('Ctrl Pts',(-44.2768120064326,29.5504650026777,
-50.3614668069728));
#237299=CARTESIAN_POINT('Ctrl Pts',(-43.9003665379152,29.6164848585984,
-50.339507487976));
#237300=CARTESIAN_POINT('Ctrl Pts',(-43.6501321722007,29.7142834763753,
-50.3255182498909));
#237301=CARTESIAN_POINT('Ctrl Pts',(-43.2115972335477,29.9962147682009,
-50.2984850006312));
#237302=CARTESIAN_POINT('Ctrl Pts',(-43.0252592255953,30.1741490453239,
-50.2840612318214));
#237303=CARTESIAN_POINT('Ctrl Pts',(-42.723818163838,30.5985232252024,-50.253830602992));
#237304=CARTESIAN_POINT('Ctrl Pts',(-42.614742881212,30.843213893845,-50.2382879210339));
#237305=CARTESIAN_POINT('Ctrl Pts',(-42.5002245589074,31.3529575529645,
-50.2091964974042));
#237306=CARTESIAN_POINT('Ctrl Pts',(-42.4927710519953,31.6123206435822,
-50.196762142347));
#237307=CARTESIAN_POINT('Ctrl Pts',(-42.5766779131083,32.1208776863805,
-50.1686234986617));
#237308=CARTESIAN_POINT('Ctrl Pts',(-42.6676932477752,32.3651548635337,
-50.1536284540101));
#237309=CARTESIAN_POINT('Ctrl Pts',(-42.9411486631884,32.8114526906639,
-50.1231065311302));
#237310=CARTESIAN_POINT('Ctrl Pts',(-43.1232997004361,33.0077938297902,
-50.1078750017102));
#237311=CARTESIAN_POINT('Ctrl Pts',(-43.5440398982312,33.3110704390746,
-50.080282439807));
#237312=CARTESIAN_POINT('Ctrl Pts',(-43.7758833547215,33.4188327572136,
-50.0676540310437));
#237313=CARTESIAN_POINT('Ctrl Pts',(-44.2751366816049,33.5439605610322,
-50.0385309203087));
#237314=CARTESIAN_POINT('Ctrl Pts',(-44.5385395304028,33.5572082346637,
-50.0231657541288));
#237315=CARTESIAN_POINT('Ctrl Pts',(-45.0594426530212,33.4811202826094,
-49.9927797386426));
#237316=CARTESIAN_POINT('Ctrl Pts',(-45.3115366621747,33.3909896609665,
-49.978331175041));
#237317=CARTESIAN_POINT('Ctrl Pts',(-45.7568417506746,33.1232024289028,
-49.9518149947893));
#237318=CARTESIAN_POINT('Ctrl Pts',(-45.9479404421206,32.9515549679649,
-49.9375699710248));
#237319=CARTESIAN_POINT('Ctrl Pts',(-46.2614539645297,32.5380265596496,
-49.9075351370584));
#237320=CARTESIAN_POINT('Ctrl Pts',(-46.3778496296041,32.2976967025486,
-49.8919992440707));
#237321=CARTESIAN_POINT('Ctrl Pts',(-46.5090182683512,31.7910157173607,
-49.8625769068278));
#237322=CARTESIAN_POINT('Ctrl Pts',(-46.5246154445457,31.5301825592137,
-49.8499171884875));
#237323=CARTESIAN_POINT('Ctrl Pts',(-46.4557043772846,31.0183536933514,
-49.822050635679));
#237324=CARTESIAN_POINT('Ctrl Pts',(-46.372368230767,30.7721768865771,-49.8071836015771));
#237325=CARTESIAN_POINT('Ctrl Pts',(-46.1119061688116,30.3161120727555,
-49.7765472414218));
#237326=CARTESIAN_POINT('Ctrl Pts',(-45.9337779549868,30.1126103578477,
-49.7610713053205));
#237327=CARTESIAN_POINT('Ctrl Pts',(-45.5190165437163,29.7962661962156,
-49.7329929761403));
#237328=CARTESIAN_POINT('Ctrl Pts',(-45.2897486819327,29.6821620200328,
-49.7205547797102));
#237329=CARTESIAN_POINT('Ctrl Pts',(-44.8699416127025,29.565085884589,-49.6960660340051));
#237330=CARTESIAN_POINT('Ctrl Pts',(-44.6891776833351,29.5404524382925,
-49.6855214714588));
#237331=CARTESIAN_POINT('Ctrl Pts',(-44.5079524583208,29.5404524382925,
-49.6749499999997));
#237332=CARTESIAN_POINT('Ctrl Pts',(-44.5079524583208,29.5404524382925,
-49.5162000000005));
#237333=CARTESIAN_POINT('Ctrl Pts',(-44.6075826695198,29.5404524382925,
-49.5220117623204));
#237334=CARTESIAN_POINT('Ctrl Pts',(-44.7072983762974,29.5478968952994,
-49.5278285118826));
#237335=CARTESIAN_POINT('Ctrl Pts',(-45.0574846297731,29.600719504041,-49.5482560433354));
#237336=CARTESIAN_POINT('Ctrl Pts',(-45.29909581334,29.6861235028605,-49.5622644165605));
#237337=CARTESIAN_POINT('Ctrl Pts',(-45.7469953257586,29.9482656497159,
-49.5885710882564));
#237338=CARTESIAN_POINT('Ctrl Pts',(-45.9468628369225,30.1263200493847,
-49.6033955359452));
#237339=CARTESIAN_POINT('Ctrl Pts',(-46.2628676237101,30.5463702077689,
-49.6338324985279));
#237340=CARTESIAN_POINT('Ctrl Pts',(-46.3773467568928,30.783284056148,-49.6491399222326));
#237341=CARTESIAN_POINT('Ctrl Pts',(-46.5072346558957,31.2810633104478,
-49.6780752056027));
#237342=CARTESIAN_POINT('Ctrl Pts',(-46.5239839945915,31.5365332692116,
-49.6905344243601));
#237343=CARTESIAN_POINT('Ctrl Pts',(-46.459326200111,32.0541703938326,-49.7185703458577));
#237344=CARTESIAN_POINT('Ctrl Pts',(-46.3730540890751,32.3105994108117,
-49.7340409349361));
#237345=CARTESIAN_POINT('Ctrl Pts',(-46.1098497512395,32.765305155933,-49.7646886205033));
#237346=CARTESIAN_POINT('Ctrl Pts',(-45.9389489246245,32.9612335178118,
-49.7795711660375));
#237347=CARTESIAN_POINT('Ctrl Pts',(-45.5313434501067,33.2781493688681,
-49.807469661087));
#237348=CARTESIAN_POINT('Ctrl Pts',(-45.2982859569776,33.3957968842558,
-49.8200972125782));
#237349=CARTESIAN_POINT('Ctrl Pts',(-44.7945554557703,33.5374114466433,
-49.8494814918152));
#237350=CARTESIAN_POINT('Ctrl Pts',(-44.5281986460667,33.55776831581,-49.8650189723812));
#237351=CARTESIAN_POINT('Ctrl Pts',(-44.0128990377119,33.4948687514879,
-49.8950781162018));
#237352=CARTESIAN_POINT('Ctrl Pts',(-43.7683297027054,33.4160390242073,
-49.9093446607438));
#237353=CARTESIAN_POINT('Ctrl Pts',(-43.3127967774858,33.1658285001609,
-49.935917414715));
#237354=CARTESIAN_POINT('Ctrl Pts',(-43.1080838362608,32.9932790555579,
-49.9503020572687));
#237355=CARTESIAN_POINT('Ctrl Pts',(-42.7802422051094,32.5812708563266,
-49.9806779962582));
#237356=CARTESIAN_POINT('Ctrl Pts',(-42.6591711818348,32.3468651094646,
-49.996050978779));
#237357=CARTESIAN_POINT('Ctrl Pts',(-42.5162361847141,31.8523604660051,
-50.025201375234));
#237358=CARTESIAN_POINT('Ctrl Pts',(-42.4927833343748,31.5978101679999,
-50.0378599609079));
#237359=CARTESIAN_POINT('Ctrl Pts',(-42.5432979860439,31.0816659714257,
-50.0654079541129));
#237360=CARTESIAN_POINT('Ctrl Pts',(-42.6213856920525,30.8254844179476,
-50.0806273299803));
#237361=CARTESIAN_POINT('Ctrl Pts',(-42.8696317804171,30.3645964810192,
-50.1111510461556));
#237362=CARTESIAN_POINT('Ctrl Pts',(-43.0350560656012,30.1630148227299,
-50.1261594532995));
#237363=CARTESIAN_POINT('Ctrl Pts',(-43.4323797711602,29.8348222084344,
-50.1543277446218));
#237364=CARTESIAN_POINT('Ctrl Pts',(-43.660141244683,29.7109029976232,-50.1667443458715));
#237365=CARTESIAN_POINT('Ctrl Pts',(-44.1005015496996,29.5717085211214,
-50.1924320303309));
#237366=CARTESIAN_POINT('Ctrl Pts',(-44.3038169444646,29.5404524382925,
-50.2042920950255));
#237367=CARTESIAN_POINT('Ctrl Pts',(-44.5079524583208,29.5404524382925,
-50.2162000000005));
#237368=CARTESIAN_POINT('Origin',(-44.5079524583208,31.5404524382925,235.35105));
#237369=CARTESIAN_POINT('',(-44.5079524583208,29.5404524382925,-48.8162000000004));
#237370=CARTESIAN_POINT('',(-44.5079524583208,29.5404524382925,-48.9749499999996));
#237371=CARTESIAN_POINT('',(-44.5079524583208,29.5404524382925,235.35105));
#237372=CARTESIAN_POINT('Ctrl Pts',(-44.5079524583208,29.5404524382925,
-49.6749499999997));
#237373=CARTESIAN_POINT('Ctrl Pts',(-44.4296713573153,29.5404524382925,
-49.670383602441));
#237374=CARTESIAN_POINT('Ctrl Pts',(-44.3513041854955,29.5450482640994,
-49.6658121840848));
#237375=CARTESIAN_POINT('Ctrl Pts',(-44.0100641429768,29.5853706921466,
-49.645906514938));
#237376=CARTESIAN_POINT('Ctrl Pts',(-43.755610585112,29.6684825954307,-49.6310633907293));
#237377=CARTESIAN_POINT('Ctrl Pts',(-43.3037426519632,29.9235780366005,
-49.6047044279624));
#237378=CARTESIAN_POINT('Ctrl Pts',(-43.108410266594,30.0893196633568,-49.5907718938373));
#237379=CARTESIAN_POINT('Ctrl Pts',(-42.7840560257168,30.4927404792281,
-49.5609314891058));
#237380=CARTESIAN_POINT('Ctrl Pts',(-42.6610929378257,30.7288880785963,
-49.5454153262035));
#237381=CARTESIAN_POINT('Ctrl Pts',(-42.5146543172607,31.2325538999191,
-49.5156999349872));
#237382=CARTESIAN_POINT('Ctrl Pts',(-42.4915363829144,31.4947984047003,
-49.5027351594508));
#237383=CARTESIAN_POINT('Ctrl Pts',(-42.5468368096406,32.0094939633745,
-49.4751207636448));
#237384=CARTESIAN_POINT('Ctrl Pts',(-42.623214093632,32.2571817619078,-49.4603803638605));
#237385=CARTESIAN_POINT('Ctrl Pts',(-42.8702009197475,32.7190247217399,
-49.4298451301786));
#237386=CARTESIAN_POINT('Ctrl Pts',(-43.0419698811053,32.9268821241792,
-49.4143346310045));
#237387=CARTESIAN_POINT('Ctrl Pts',(-43.4473529517607,33.2550770068072,
-49.3859311602751));
#237388=CARTESIAN_POINT('Ctrl Pts',(-43.6739406933817,33.3760010232055,
-49.3736006862886));
#237389=CARTESIAN_POINT('Ctrl Pts',(-44.1654079682929,33.5279579915564,
-49.3449317619187));
#237390=CARTESIAN_POINT('Ctrl Pts',(-44.4262271418543,33.5555997274517,
-49.3297173101275));
#237391=CARTESIAN_POINT('Ctrl Pts',(-44.9490461965395,33.509132724569,-49.2992195319375));
#237392=CARTESIAN_POINT('Ctrl Pts',(-45.2058465600757,33.4334018254037,
-49.2842395107311));
#237393=CARTESIAN_POINT('Ctrl Pts',(-45.6645551224534,33.191650543762,-49.257481511259));
#237394=CARTESIAN_POINT('Ctrl Pts',(-45.8642564135317,33.0319921369332,
-49.2440742920432));
#237395=CARTESIAN_POINT('Ctrl Pts',(-46.1995741557137,32.639325372177,-49.2144573932752));
#237396=CARTESIAN_POINT('Ctrl Pts',(-46.3292102598113,32.4077055769673,
-49.1989753370165));
#237397=CARTESIAN_POINT('Ctrl Pts',(-46.491528560328,31.9073949943738,-49.1689662889167));
#237398=CARTESIAN_POINT('Ctrl Pts',(-46.5225340672254,31.6436308176897,
-49.1555876776239));
#237399=CARTESIAN_POINT('Ctrl Pts',(-46.4812535020921,31.1260841753774,
-49.1282381629808));
#237400=CARTESIAN_POINT('Ctrl Pts',(-46.4120209946098,30.8770502457702,
-49.1136381484616));
#237401=CARTESIAN_POINT('Ctrl Pts',(-46.178948166395,30.4096926314201,-49.0832301495823));
#237402=CARTESIAN_POINT('Ctrl Pts',(-46.0137898376405,30.1975740153553,
-49.0676971919029));
#237403=CARTESIAN_POINT('Ctrl Pts',(-45.6181367783471,29.8573528393903,
-49.0389699670982));
#237404=CARTESIAN_POINT('Ctrl Pts',(-45.3942174077798,29.7294116890116,
-49.0266487887179));
#237405=CARTESIAN_POINT('Ctrl Pts',(-44.9445050686823,29.5763822844598,
-49.0004155689373));
#237406=CARTESIAN_POINT('Ctrl Pts',(-44.7268193952234,29.5404524382925,
-48.9877172379856));
#237407=CARTESIAN_POINT('Ctrl Pts',(-44.5079524583208,29.5404524382925,
-48.9749499999996));
#237408=CARTESIAN_POINT('Ctrl Pts',(-44.5079524583208,29.5404524382925,
-48.8162000000004));
#237409=CARTESIAN_POINT('Ctrl Pts',(-44.6469069524102,29.5404524382925,
-48.8243056788223));
#237410=CARTESIAN_POINT('Ctrl Pts',(-44.7858169909055,29.5549338421087,
-48.8324087644013));
#237411=CARTESIAN_POINT('Ctrl Pts',(-45.1702021228419,29.6363555489129,
-48.854831230431));
#237412=CARTESIAN_POINT('Ctrl Pts',(-45.405715723631,29.7354215086392,-48.8678646079231));
#237413=CARTESIAN_POINT('Ctrl Pts',(-45.8372124491951,30.0227568965869,
-48.8949655808986));
#237414=CARTESIAN_POINT('Ctrl Pts',(-46.0264887799817,30.212169595963,-48.9100549194317));
#237415=CARTESIAN_POINT('Ctrl Pts',(-46.3168186695098,30.648729018531,-48.9405770483049));
#237416=CARTESIAN_POINT('Ctrl Pts',(-46.4170418320557,30.890401137655,-48.9557090518944));
#237417=CARTESIAN_POINT('Ctrl Pts',(-46.5189384190221,31.3948760227152,
-48.9841661728661));
#237418=CARTESIAN_POINT('Ctrl Pts',(-46.5210788733626,31.6526032984413,
-48.9964828000418));
#237419=CARTESIAN_POINT('Ctrl Pts',(-46.4262861046215,32.1656887343397,
-49.0251677154016));
#237420=CARTESIAN_POINT('Ctrl Pts',(-46.3260837074216,32.4152656781251,
-49.0406984504417));
#237421=CARTESIAN_POINT('Ctrl Pts',(-46.0394122132731,32.8520385101669,
-49.0711246571677));
#237422=CARTESIAN_POINT('Ctrl Pts',(-45.8589761702092,33.0372490386676,
-49.0857438680829));
#237423=CARTESIAN_POINT('Ctrl Pts',(-45.4326608595628,33.3331976238984,
-49.1131288392364));
#237424=CARTESIAN_POINT('Ctrl Pts',(-45.189437010449,33.4390396738555,-49.126446734459));
#237425=CARTESIAN_POINT('Ctrl Pts',(-44.6756555075747,33.550686055685,-49.1564173221266));
#237426=CARTESIAN_POINT('Ctrl Pts',(-44.4101572833061,33.5552965078418,
-49.1719047185422));
#237427=CARTESIAN_POINT('Ctrl Pts',(-43.9019216507782,33.4632115008325,
-49.2015517971062));
#237428=CARTESIAN_POINT('Ctrl Pts',(-43.6633961901834,33.3710070719332,
-49.2150233269016));
#237429=CARTESIAN_POINT('Ctrl Pts',(-43.2235817281476,33.0963130838346,
-49.2417282804086));
#237430=CARTESIAN_POINT('Ctrl Pts',(-43.0288870275621,32.9125412104799,
-49.2566906906406));
#237431=CARTESIAN_POINT('Ctrl Pts',(-42.7255171362445,32.4841010351062,
-49.2871829835634));
#237432=CARTESIAN_POINT('Ctrl Pts',(-42.6180922873079,32.2447206477794,
-49.302409262292));
#237433=CARTESIAN_POINT('Ctrl Pts',(-42.5020856709242,31.7435657778012,
-49.3311102047735));
#237434=CARTESIAN_POINT('Ctrl Pts',(-42.4925379086377,31.4870247470635,
-49.3434494770097));
#237435=CARTESIAN_POINT('Ctrl Pts',(-42.5720552127493,30.9715497267348,
-49.371809575366));
#237436=CARTESIAN_POINT('Ctrl Pts',(-42.6652490010032,30.718404833557,-49.3873161388427));
#237437=CARTESIAN_POINT('Ctrl Pts',(-42.9401546415722,30.2723841156141,
-49.4178663609134));
#237438=CARTESIAN_POINT('Ctrl Pts',(-43.1158328585487,30.0816773705056,
-49.4326244605883));
#237439=CARTESIAN_POINT('Ctrl Pts',(-43.5326703382316,29.7750342823307,
-49.460273261494));
#237440=CARTESIAN_POINT('Ctrl Pts',(-43.7706583326269,29.6631423424877,
-49.4731911760016));
#237441=CARTESIAN_POINT('Ctrl Pts',(-44.1822860790587,29.5603671423784,
-49.4972027945435));
#237442=CARTESIAN_POINT('Ctrl Pts',(-44.3450049210616,29.5404524382925,
-49.5066947269937));
#237443=CARTESIAN_POINT('Ctrl Pts',(-44.5079524583208,29.5404524382925,
-49.5162000000005));
#237444=CARTESIAN_POINT('Origin',(-44.5079524583208,31.5404524382925,235.35105));
#237445=CARTESIAN_POINT('',(-44.5079524583208,29.5404524382925,-48.1162000000004));
#237446=CARTESIAN_POINT('',(-44.5079524583208,29.5404524382925,-48.2749499999996));
#237447=CARTESIAN_POINT('',(-44.5079524583208,29.5404524382925,235.35105));
#237448=CARTESIAN_POINT('Ctrl Pts',(-44.5079524583208,29.5404524382925,
-48.9749499999996));
#237449=CARTESIAN_POINT('Ctrl Pts',(-44.4683714928986,29.5404524382925,
-48.97264111035));
#237450=CARTESIAN_POINT('Ctrl Pts',(-44.4287518944074,29.5416274112108,
-48.9703299671047));
#237451=CARTESIAN_POINT('Ctrl Pts',(-44.1244892411486,29.5597336396126,
-48.9525813123313));
#237452=CARTESIAN_POINT('Ctrl Pts',(-43.8655460451714,29.6279544839446,
-48.9374762925661));
#237453=CARTESIAN_POINT('Ctrl Pts',(-43.400077042296,29.8561938741588,-48.9103239340652));
#237454=CARTESIAN_POINT('Ctrl Pts',(-43.1959415636786,30.0098370335365,
-48.8973402053029));
#237455=CARTESIAN_POINT('Ctrl Pts',(-42.8498745701799,30.3917675000002,
-48.8679521646172));
#237456=CARTESIAN_POINT('Ctrl Pts',(-42.7137697510356,30.61871226316,-48.8525176114667));
#237457=CARTESIAN_POINT('Ctrl Pts',(-42.5356635853209,31.1154542836193,
-48.8222283611175));
#237458=CARTESIAN_POINT('Ctrl Pts',(-42.496736437211,31.3807690747112,-48.8083440418324));
#237459=CARTESIAN_POINT('Ctrl Pts',(-42.524203596213,31.9010235360147,-48.7812606241996));
#237460=CARTESIAN_POINT('Ctrl Pts',(-42.5864312605022,32.1511776656024,
-48.7668083271779));
#237461=CARTESIAN_POINT('Ctrl Pts',(-42.8057858625377,32.6235356115091,
-48.7365478357366));
#237462=CARTESIAN_POINT('Ctrl Pts',(-42.9643836875725,32.8396271517157,
-48.7210055213103));
#237463=CARTESIAN_POINT('Ctrl Pts',(-43.350382955504,33.1915192885072,-48.6919702700874));
#237464=CARTESIAN_POINT('Ctrl Pts',(-43.5717413988538,33.326367924112,-48.6795623118027));
#237465=CARTESIAN_POINT('Ctrl Pts',(-44.0548892019584,33.5055260564065,
-48.6513786899549));
#237466=CARTESIAN_POINT('Ctrl Pts',(-44.3122938236924,33.5475578917467,
-48.6363634203537));
#237467=CARTESIAN_POINT('Ctrl Pts',(-44.8355710464731,33.5311754888667,
-48.6058389156914));
#237468=CARTESIAN_POINT('Ctrl Pts',(-45.0963654311893,33.4702507280505,
-48.5906259099162));
#237469=CARTESIAN_POINT('Ctrl Pts',(-45.5682200277731,33.2551011217427,
-48.5631010584487));
#237470=CARTESIAN_POINT('Ctrl Pts',(-45.7766682854539,33.1071598903678,
-48.5504262815134));
#237471=CARTESIAN_POINT('Ctrl Pts',(-46.132828773842,32.7354814161378,-48.5212617588931));
#237472=CARTESIAN_POINT('Ctrl Pts',(-46.2749260998083,32.5131362704431,
-48.5058847884518));
#237473=CARTESIAN_POINT('Ctrl Pts',(-46.4669477216483,32.0228186329689,
-48.4755142185661));
#237474=CARTESIAN_POINT('Ctrl Pts',(-46.5135478681275,31.7591670652899,
-48.4611622574699));
#237475=CARTESIAN_POINT('Ctrl Pts',(-46.5015253869323,31.2395253140083,
-48.4345602625822));
#237476=CARTESIAN_POINT('Ctrl Pts',(-46.4470347162938,30.9883613969714,
-48.4202826152829));
#237477=CARTESIAN_POINT('Ctrl Pts',(-46.242919821103,30.5109436639625,-48.3902110042146));
#237478=CARTESIAN_POINT('Ctrl Pts',(-46.0916587682423,30.2906972496676,
-48.3746727824303));
#237479=CARTESIAN_POINT('Ctrl Pts',(-45.7164818762461,29.9260400811427,
-48.3453083180696));
#237480=CARTESIAN_POINT('Ctrl Pts',(-45.4978985777791,29.7835041007128,
-48.3326968569679));
#237481=CARTESIAN_POINT('Ctrl Pts',(-45.0198102819191,29.59003151068,-48.3048083730428));
#237482=CARTESIAN_POINT('Ctrl Pts',(-44.7650619789425,29.5404524382925,
-48.2899480553692));
#237483=CARTESIAN_POINT('Ctrl Pts',(-44.5079524583208,29.5404524382925,
-48.2749499999996));
#237484=CARTESIAN_POINT('Ctrl Pts',(-44.5079524583208,29.5404524382925,
-48.1162000000004));
#237485=CARTESIAN_POINT('Ctrl Pts',(-44.6829574575485,29.5404524382925,
-48.1264086249554));
#237486=CARTESIAN_POINT('Ctrl Pts',(-44.8575854482278,29.5634237494144,
-48.1365952577451));
#237487=CARTESIAN_POINT('Ctrl Pts',(-45.2722893575364,29.6749367761027,
-48.1607863191215));
#237488=CARTESIAN_POINT('Ctrl Pts',(-45.5024584683471,29.786798548748,-48.1732817442552));
#237489=CARTESIAN_POINT('Ctrl Pts',(-45.9180503088427,30.0975433635833,
-48.2011014256546));
#237490=CARTESIAN_POINT('Ctrl Pts',(-46.0967531377997,30.2970540722592,
-48.2163925031182));
#237491=CARTESIAN_POINT('Ctrl Pts',(-46.3621447032057,30.7477137033057,
-48.246899580631));
#237492=CARTESIAN_POINT('Ctrl Pts',(-46.4488020510829,30.99309905767,-48.2618235003955));
#237493=CARTESIAN_POINT('Ctrl Pts',(-46.5242001097123,31.5035272387935,
-48.2898084971189));
#237494=CARTESIAN_POINT('Ctrl Pts',(-46.5121432671305,31.7637128885449,
-48.3023564726688));
#237495=CARTESIAN_POINT('Ctrl Pts',(-46.3882000551431,32.271751121424,-48.3316366339381));
#237496=CARTESIAN_POINT('Ctrl Pts',(-46.2749612510384,32.5139993733863,
-48.3471773655706));
#237497=CARTESIAN_POINT('Ctrl Pts',(-45.9666409067441,32.9322757248042,
-48.3773005891367));
#237498=CARTESIAN_POINT('Ctrl Pts',(-45.7775827427436,33.1066668926727,
-48.3916247045115));
#237499=CARTESIAN_POINT('Ctrl Pts',(-45.3332167323945,33.381814914463,-48.4184853484524));
#237500=CARTESIAN_POINT('Ctrl Pts',(-45.0795347991248,33.4756664295537,
-48.4328576967862));
#237501=CARTESIAN_POINT('Ctrl Pts',(-44.5564675923915,33.5568862540778,
-48.4633699505122));
#237502=CARTESIAN_POINT('Ctrl Pts',(-44.2927243429971,33.5459555958065,
-48.4787549733934));
#237503=CARTESIAN_POINT('Ctrl Pts',(-43.7922644434613,33.4251241785786,
-48.507948467533));
#237504=CARTESIAN_POINT('Ctrl Pts',(-43.5595661090824,33.3194223032443,
-48.5206576712748));
#237505=CARTESIAN_POINT('Ctrl Pts',(-43.1362566519627,33.0199117609383,
-48.5481349151771));
#237506=CARTESIAN_POINT('Ctrl Pts',(-42.9523932251493,32.825187863206,-48.5633346892518));
#237507=CARTESIAN_POINT('Ctrl Pts',(-42.6749091578537,32.381138797746,-48.5938605112022));
#237508=CARTESIAN_POINT('Ctrl Pts',(-42.5817065529211,32.1374478458307,
-48.6088897362229));
#237509=CARTESIAN_POINT('Ctrl Pts',(-42.4935289496987,31.6298445702235,
-48.6371047606673));
#237510=CARTESIAN_POINT('Ctrl Pts',(-42.4986884027967,31.3708823477966,
-48.6494961654023));
#237511=CARTESIAN_POINT('Ctrl Pts',(-42.6084989238686,30.860313793874,-48.6784919503211));
#237512=CARTESIAN_POINT('Ctrl Pts',(-42.7154756982118,30.6144289468359,
-48.6940337534694));
#237513=CARTESIAN_POINT('Ctrl Pts',(-43.0134368174215,30.1870502854352,
-48.7243146648186));
#237514=CARTESIAN_POINT('Ctrl Pts',(-43.1983916540592,30.0073619324355,
-48.7387867037976));
#237515=CARTESIAN_POINT('Ctrl Pts',(-43.634012144625,29.7220634423569,-48.7659050529433));
#237516=CARTESIAN_POINT('Ctrl Pts',(-43.8825480054977,29.6223194049305,
-48.7797180735857));
#237517=CARTESIAN_POINT('Ctrl Pts',(-44.2639012978467,29.5516168955097,
-48.8019636823061));
#237518=CARTESIAN_POINT('Ctrl Pts',(-44.385944014934,29.5404524382925,-48.8090828408029));
#237519=CARTESIAN_POINT('Ctrl Pts',(-44.5079524583208,29.5404524382925,
-48.8162000000004));
#237520=CARTESIAN_POINT('Origin',(-44.5079524583208,31.5404524382925,235.35105));
#237521=CARTESIAN_POINT('',(-44.5079524583208,29.5404524382925,-47.4162000000004));
#237522=CARTESIAN_POINT('',(-44.5079524583208,29.5404524382925,-47.5749499999997));
#237523=CARTESIAN_POINT('',(-44.5079524583208,29.5404524382925,235.35105));
#237524=CARTESIAN_POINT('Ctrl Pts',(-44.5079524583208,29.5404524382925,
-48.2749499999996));
#237525=CARTESIAN_POINT('Ctrl Pts',(-44.5074611740721,29.5404524382925,
-48.2749213417518));
#237526=CARTESIAN_POINT('Ctrl Pts',(-44.5069698812021,29.5404526193126,
-48.2748926830011));
#237527=CARTESIAN_POINT('Ctrl Pts',(-44.2386011496059,29.5406503908197,
-48.2592378403247));
#237528=CARTESIAN_POINT('Ctrl Pts',(-43.9734400904005,29.5946645805173,
-48.2437701118711));
#237529=CARTESIAN_POINT('Ctrl Pts',(-43.4932031097656,29.798423853582,-48.2157562880009));
#237530=CARTESIAN_POINT('Ctrl Pts',(-43.2806365401203,29.9410495527583,
-48.2032854916218));
#237531=CARTESIAN_POINT('Ctrl Pts',(-42.9151623196074,30.3031230496922,
-48.1743345441514));
#237532=CARTESIAN_POINT('Ctrl Pts',(-42.7676177442234,30.5210469482816,
-48.1590220488203));
#237533=CARTESIAN_POINT('Ctrl Pts',(-42.5627741871192,31.0051834192762,
-48.1285897669094));
#237534=CARTESIAN_POINT('Ctrl Pts',(-42.50902073151,31.2674026979878,-48.1137751253118));
#237535=CARTESIAN_POINT('Ctrl Pts',(-42.5069602194121,31.7864102811206,
-48.0874957248569));
#237536=CARTESIAN_POINT('Ctrl Pts',(-42.5543111330295,32.0383072839409,
-48.0734471669374));
#237537=CARTESIAN_POINT('Ctrl Pts',(-42.7444520332751,32.5200790493857,
-48.0435631730643));
#237538=CARTESIAN_POINT('Ctrl Pts',(-42.8889138044954,32.743915970668,-48.0280418778959));
#237539=CARTESIAN_POINT('Ctrl Pts',(-43.2540140322781,33.1201551487533,
-47.9983862145619));
#237540=CARTESIAN_POINT('Ctrl Pts',(-43.4700886114566,33.2697998012266,
-47.9854920577344));
#237541=CARTESIAN_POINT('Ctrl Pts',(-43.9443751863956,33.4765379120186,
-47.9578253408628));
#237542=CARTESIAN_POINT('Ctrl Pts',(-44.1975283092354,33.5328502398106,
-47.9430580753638));
#237543=CARTESIAN_POINT('Ctrl Pts',(-44.7213777085793,33.5468913257583,
-47.9125001937353));
#237544=CARTESIAN_POINT('Ctrl Pts',(-44.9871677370191,33.5004857452827,
-47.8969957754096));
#237545=CARTESIAN_POINT('Ctrl Pts',(-45.4729515719845,33.3106212295625,
-47.8686583850365));
#237546=CARTESIAN_POINT('Ctrl Pts',(-45.6900255288811,33.1736795453411,
-47.8563138117252));
#237547=CARTESIAN_POINT('Ctrl Pts',(-46.0653428964289,32.821907248863,-47.8275961700409));
#237548=CARTESIAN_POINT('Ctrl Pts',(-46.2185461635087,32.6088362993964,
-47.8123637915399));
#237549=CARTESIAN_POINT('Ctrl Pts',(-46.4369517705266,32.1314024279935,
-47.7818745527615));
#237550=CARTESIAN_POINT('Ctrl Pts',(-46.4982262257139,31.8707844500243,
-47.7669214434249));
#237551=CARTESIAN_POINT('Ctrl Pts',(-46.5151614667972,31.3524912152932,
-47.7402442842664));
#237552=CARTESIAN_POINT('Ctrl Pts',(-46.4752298333033,31.0998738211168,
-47.7267383740709));
#237553=CARTESIAN_POINT('Ctrl Pts',(-46.2998284515804,30.6139700091309,
-47.6970755394804));
#237554=CARTESIAN_POINT('Ctrl Pts',(-46.1625784307328,30.3865869735557,
-47.6815854439025));
#237555=CARTESIAN_POINT('Ctrl Pts',(-45.808237634687,29.9983022717098,-47.6516350797687));
#237556=CARTESIAN_POINT('Ctrl Pts',(-45.5947804975627,29.8411169979924,
-47.6383483022886));
#237557=CARTESIAN_POINT('Ctrl Pts',(-45.1250058936745,29.620834015134,-47.6109447837285));
#237558=CARTESIAN_POINT('Ctrl Pts',(-44.874219530905,29.5576512913066,-47.5963155792336));
#237559=CARTESIAN_POINT('Ctrl Pts',(-44.5815654461517,29.5414674752469,
-47.5792440909564));
#237560=CARTESIAN_POINT('Ctrl Pts',(-44.5447410599504,29.5404524382925,
-47.5770960017614));
#237561=CARTESIAN_POINT('Ctrl Pts',(-44.5079524583208,29.5404524382925,
-47.5749499999996));
#237562=CARTESIAN_POINT('Ctrl Pts',(-44.5079524583208,29.5404524382925,
-47.4162000000004));
#237563=CARTESIAN_POINT('Ctrl Pts',(-44.7203615317488,29.5404524382925,
-47.4285905292838));
#237564=CARTESIAN_POINT('Ctrl Pts',(-44.9317409055993,29.5742933371907,
-47.4409209927584));
#237565=CARTESIAN_POINT('Ctrl Pts',(-45.3764514988243,29.7208785666382,
-47.4668624440298));
#237566=CARTESIAN_POINT('Ctrl Pts',(-45.6012773747708,29.8464104982827,
-47.4791754476813));
#237567=CARTESIAN_POINT('Ctrl Pts',(-46.000279698641,30.182522922248,-47.5077927928256));
#237568=CARTESIAN_POINT('Ctrl Pts',(-46.1677140915721,30.3932042385524,
-47.5233195259874));
#237569=CARTESIAN_POINT('Ctrl Pts',(-46.4055670380206,30.8587182248351,
-47.5537738083052));
#237570=CARTESIAN_POINT('Ctrl Pts',(-46.4772495247028,31.1073138275644,
-47.5684231370886));
#237571=CARTESIAN_POINT('Ctrl Pts',(-46.5233442630961,31.6238931033201,
-47.5958641955509));
#237572=CARTESIAN_POINT('Ctrl Pts',(-46.4950640003346,31.8871286464186,
-47.6090893535405));
#237573=CARTESIAN_POINT('Ctrl Pts',(-46.33821528632,32.3886208514487,-47.6389985654116));
#237574=CARTESIAN_POINT('Ctrl Pts',(-46.2108591253111,32.6218203074811,
-47.6544939248702));
#237575=CARTESIAN_POINT('Ctrl Pts',(-45.8792998736936,33.0181962783179,
-47.6841885832202));
#237576=CARTESIAN_POINT('Ctrl Pts',(-45.6811130217757,33.1799456474558,
-47.6977656337983));
#237577=CARTESIAN_POINT('Ctrl Pts',(-45.2247563204773,33.4263203586885,
-47.724386441374));
#237578=CARTESIAN_POINT('Ctrl Pts',(-44.9687431979571,33.5046133828753,
-47.7393205401875));
#237579=CARTESIAN_POINT('Ctrl Pts',(-44.44618315351,33.5563426158039,-47.7698032094469));
#237580=CARTESIAN_POINT('Ctrl Pts',(-44.1848481544729,33.5312432690995,
-47.7850477510573));
#237581=CARTESIAN_POINT('Ctrl Pts',(-43.6919680971685,33.3840468816324,
-47.8137990877334));
#237582=CARTESIAN_POINT('Ctrl Pts',(-43.4644572149029,33.26549767212,-47.8261558532141));
#237583=CARTESIAN_POINT('Ctrl Pts',(-43.0557992144319,32.9414122120539,
-47.8544472423104));
#237584=CARTESIAN_POINT('Ctrl Pts',(-42.8818074731782,32.7350480172083,
-47.8699471384817));
#237585=CARTESIAN_POINT('Ctrl Pts',(-42.630120881441,32.2751707661802,-47.9005201446915));
#237586=CARTESIAN_POINT('Ctrl Pts',(-42.5513210079441,32.0279864772773,
-47.9153057669622));
#237587=CARTESIAN_POINT('Ctrl Pts',(-42.4912785014281,31.514278639586,-47.9430085755936));
#237588=CARTESIAN_POINT('Ctrl Pts',(-42.5117614109264,31.2525335670707,
-47.9558562227586));
#237589=CARTESIAN_POINT('Ctrl Pts',(-42.6528631438635,30.7477908955022,
-47.9854703552333));
#237590=CARTESIAN_POINT('Ctrl Pts',(-42.7735473128218,30.5101621105732,
-48.0009948764191));
#237591=CARTESIAN_POINT('Ctrl Pts',(-43.0941807328986,30.1031372910013,
-48.0309088248051));
#237592=CARTESIAN_POINT('Ctrl Pts',(-43.2880628865459,29.9353417761717,
-48.04503977498));
#237593=CARTESIAN_POINT('Ctrl Pts',(-43.7376236282077,29.6758146575417,
-48.071264151577));
#237594=CARTESIAN_POINT('Ctrl Pts',(-43.9912474034753,29.5902619044792,
-48.086058871801));
#237595=CARTESIAN_POINT('Ctrl Pts',(-44.3384685866399,29.5458325820639,
-48.106313440819));
#237596=CARTESIAN_POINT('Ctrl Pts',(-44.4232546759027,29.5404524382925,
-48.1112592960261));
#237597=CARTESIAN_POINT('Ctrl Pts',(-44.5079524583208,29.5404524382925,
-48.1162000000005));
#237598=CARTESIAN_POINT('Origin',(-44.5079524583208,31.5404524382925,235.35105));
#237599=CARTESIAN_POINT('',(-44.5079524583208,29.5404524382925,-46.7162000000005));
#237600=CARTESIAN_POINT('',(-44.5079524583208,29.5404524382925,-46.8749499999997));
#237601=CARTESIAN_POINT('',(-44.5079524583208,29.5404524382925,235.35105));
#237602=CARTESIAN_POINT('Ctrl Pts',(-44.5079524583208,29.5404524382925,
-47.5749499999996));
#237603=CARTESIAN_POINT('Ctrl Pts',(-44.2790401916845,29.5404524382925,
-47.5615967844459));
#237604=CARTESIAN_POINT('Ctrl Pts',(-44.0515134278049,29.5797563843007,
-47.5483243898863));
#237605=CARTESIAN_POINT('Ctrl Pts',(-43.5948870817519,29.7428074112483,
-47.5216878530334));
#237606=CARTESIAN_POINT('Ctrl Pts',(-43.3730898217265,29.8739277980452,
-47.5093729124444));
#237607=CARTESIAN_POINT('Ctrl Pts',(-42.9878325441943,30.2151410676517,
-47.4808987792072));
#237608=CARTESIAN_POINT('Ctrl Pts',(-42.8290298482996,30.4231285580667,
-47.4657598909722));
#237609=CARTESIAN_POINT('Ctrl Pts',(-42.5970500796493,30.893352521703,-47.435238970338));
#237610=CARTESIAN_POINT('Ctrl Pts',(-42.5281738590795,31.1521133878894,
-47.4201579606935));
#237611=CARTESIAN_POINT('Ctrl Pts',(-42.4961237146183,31.6695339342438,
-47.3930840367877));
#237612=CARTESIAN_POINT('Ctrl Pts',(-42.5285979724327,31.9229682037961,
-47.3800238509062));
#237613=CARTESIAN_POINT('Ctrl Pts',(-42.6892492137716,32.412862045555,-47.3505896598269));
#237614=CARTESIAN_POINT('Ctrl Pts',(-42.8191939761698,32.6435720986671,
-47.3351445595209));
#237615=CARTESIAN_POINT('Ctrl Pts',(-43.1625390471162,33.0438263860826,
-47.3049102227339));
#237616=CARTESIAN_POINT('Ctrl Pts',(-43.3733681478899,33.2086657806137,
-47.2911340847757));
#237617=CARTESIAN_POINT('Ctrl Pts',(-43.8471273660993,33.4466628425882,
-47.2634981303801));
#237618=CARTESIAN_POINT('Ctrl Pts',(-44.1053866322545,33.5173752418216,
-47.248433006521));
#237619=CARTESIAN_POINT('Ctrl Pts',(-44.6285574664938,33.553583731792,-47.2179147078569));
#237620=CARTESIAN_POINT('Ctrl Pts',(-44.8883012981081,33.5210075007997,
-47.202762984346));
#237621=CARTESIAN_POINT('Ctrl Pts',(-45.3769781595273,33.3597763480789,
-47.1742568340965));
#237622=CARTESIAN_POINT('Ctrl Pts',(-45.6017771569532,33.2341733546916,
-47.1619437578205));
#237623=CARTESIAN_POINT('Ctrl Pts',(-46.0006808176217,32.8979394298809,
-47.133323152355));
#237624=CARTESIAN_POINT('Ctrl Pts',(-46.1680481645495,32.6872153317937,
-47.1177962134451));
#237625=CARTESIAN_POINT('Ctrl Pts',(-46.4057601468361,32.2216462196778,
-47.0873432577269));
#237626=CARTESIAN_POINT('Ctrl Pts',(-46.4773703160619,31.9730373316473,
-47.0726953670536));
#237627=CARTESIAN_POINT('Ctrl Pts',(-46.5233230608925,31.4564293490652,
-47.0452569998543));
#237628=CARTESIAN_POINT('Ctrl Pts',(-46.4949626727678,31.1931783110856,
-47.0320274853069));
#237629=CARTESIAN_POINT('Ctrl Pts',(-46.3379528821531,30.691720510442,-47.0021153134141));
#237630=CARTESIAN_POINT('Ctrl Pts',(-46.2105292972496,30.4585672754571,
-46.9866203224269));
#237631=CARTESIAN_POINT('Ctrl Pts',(-45.8788590973917,30.0623004629269,
-46.9569279425619));
#237632=CARTESIAN_POINT('Ctrl Pts',(-45.6806277956508,29.900612732495,-46.9433560613437));
#237633=CARTESIAN_POINT('Ctrl Pts',(-45.2242017661382,29.6543737657247,
-46.9167312096222));
#237634=CARTESIAN_POINT('Ctrl Pts',(-44.9681651385769,29.5761558991475,
-46.9017957396811));
#237635=CARTESIAN_POINT('Ctrl Pts',(-44.6389915185149,29.5436682735582,
-46.8825939451776));
#237636=CARTESIAN_POINT('Ctrl Pts',(-44.5734344131156,29.5404524382925,
-46.878769780696));
#237637=CARTESIAN_POINT('Ctrl Pts',(-44.5079524583208,29.5404524382925,
-46.8749499999997));
#237638=CARTESIAN_POINT('Ctrl Pts',(-44.5079524583208,29.5404524382925,
-46.7162000000005));
#237639=CARTESIAN_POINT('Ctrl Pts',(-44.7564402632578,29.5404524382925,
-46.7306951219552));
#237640=CARTESIAN_POINT('Ctrl Pts',(-45.0028783481848,29.586763517434,-46.7450706769092));
#237641=CARTESIAN_POINT('Ctrl Pts',(-45.4747682115069,29.770783442715,-46.7725975856031));
#237642=CARTESIAN_POINT('Ctrl Pts',(-45.6945496843684,29.9099755438604,
-46.78510707846));
#237643=CARTESIAN_POINT('Ctrl Pts',(-46.0744438759381,30.2691102378815,
-46.8143301455376));
#237644=CARTESIAN_POINT('Ctrl Pts',(-46.2288994520815,30.4875840958792,
-46.8298719946552));
#237645=CARTESIAN_POINT('Ctrl Pts',(-46.4396370053616,30.9628662222822,
-46.8600288796926));
#237646=CARTESIAN_POINT('Ctrl Pts',(-46.4974841926455,31.2136212729569,
-46.8743837702223));
#237647=CARTESIAN_POINT('Ctrl Pts',(-46.5162685102811,31.7355259471015,
-46.9012973040128));
#237648=CARTESIAN_POINT('Ctrl Pts',(-46.4722813752727,32.0018365091121,
-46.9155486756193));
#237649=CARTESIAN_POINT('Ctrl Pts',(-46.2841830000069,32.4961949103054,
-46.9460089493815));
#237650=CARTESIAN_POINT('Ctrl Pts',(-46.1440724337216,32.7200947827809,
-46.9614065145837));
#237651=CARTESIAN_POINT('Ctrl Pts',(-45.7912746217199,33.0952069681266,
-46.9906464238707));
#237652=CARTESIAN_POINT('Ctrl Pts',(-45.5842799981298,33.2450541268618,
-47.0034142268443));
#237653=CARTESIAN_POINT('Ctrl Pts',(-45.1145561139262,33.4646088685245,
-47.030814786756));
#237654=CARTESIAN_POINT('Ctrl Pts',(-44.8543600324493,33.5279904158309,
-47.0459928915088));
#237655=CARTESIAN_POINT('Ctrl Pts',(-44.3310385260286,33.5493271984139,
-47.0765199793832));
#237656=CARTESIAN_POINT('Ctrl Pts',(-44.0730171296042,33.5096482784744,
-47.091571227508));
#237657=CARTESIAN_POINT('Ctrl Pts',(-43.588470387443,33.3349726475461,-47.119836454134));
#237658=CARTESIAN_POINT('Ctrl Pts',(-43.3662526306331,33.2024613684762,
-47.1322046309404));
#237659=CARTESIAN_POINT('Ctrl Pts',(-42.9769787956073,32.8544983659666,
-47.1611368977808));
#237660=CARTESIAN_POINT('Ctrl Pts',(-42.8161564949552,32.6397260889244,
-47.1766774460134));
#237661=CARTESIAN_POINT('Ctrl Pts',(-42.5921602652309,32.1690122033702,
-47.2069902633773));
#237662=CARTESIAN_POINT('Ctrl Pts',(-42.5275667981423,31.9192144321939,
-47.2214935604135));
#237663=CARTESIAN_POINT('Ctrl Pts',(-42.4954253358138,31.3998649668793,
-47.2486675931718));
#237664=CARTESIAN_POINT('Ctrl Pts',(-42.5316545863151,31.1350799987585,
-47.2623699771863));
#237665=CARTESIAN_POINT('Ctrl Pts',(-42.7044030484733,30.6371002695444,
-47.2925654879368));
#237666=CARTESIAN_POINT('Ctrl Pts',(-42.8383316269604,30.4085500582092,
-47.308017671671));
#237667=CARTESIAN_POINT('Ctrl Pts',(-43.1807669366193,30.0229712011951,
-47.3374840981808));
#237668=CARTESIAN_POINT('Ctrl Pts',(-43.3833866896859,29.8672896342856,
-47.3506003301631));
#237669=CARTESIAN_POINT('Ctrl Pts',(-43.8465664256208,29.6344366411589,
-47.3776191480928));
#237670=CARTESIAN_POINT('Ctrl Pts',(-44.1048044388238,29.5636483406197,
-47.3926830321964));
#237671=CARTESIAN_POINT('Ctrl Pts',(-44.4154946330336,29.5420535557601,
-47.4108066268586));
#237672=CARTESIAN_POINT('Ctrl Pts',(-44.4617479071714,29.5404524382925,
-47.4135047345167));
#237673=CARTESIAN_POINT('Ctrl Pts',(-44.5079524583208,29.5404524382925,
-47.4162000000004));
#237674=CARTESIAN_POINT('Origin',(-44.5079524583208,31.5404524382925,235.35105));
#237675=CARTESIAN_POINT('',(-44.5079524583208,29.5404524382925,-46.0162000000005));
#237676=CARTESIAN_POINT('',(-44.5079524583208,29.5404524382925,-46.1749499999996));
#237677=CARTESIAN_POINT('',(-44.5079524583208,29.5404524382925,235.35105));
#237678=CARTESIAN_POINT('Ctrl Pts',(-44.5079524583208,29.5404524382925,
-46.8749499999997));
#237679=CARTESIAN_POINT('Ctrl Pts',(-44.3143021702569,29.5404524382925,
-46.863653733196));
#237680=CARTESIAN_POINT('Ctrl Pts',(-44.1213091244848,29.5685798054682,
-46.852395805526));
#237681=CARTESIAN_POINT('Ctrl Pts',(-43.6914378076858,29.6970917220659,
-46.8273199787128));
#237682=CARTESIAN_POINT('Ctrl Pts',(-43.4639541085933,29.8157104726805,
-46.8149641523025));
#237683=CARTESIAN_POINT('Ctrl Pts',(-43.0553918712656,30.1399165374395,
-46.7866694635722));
#237684=CARTESIAN_POINT('Ctrl Pts',(-42.8814651000635,30.3463248186168,
-46.771169235201));
#237685=CARTESIAN_POINT('Ctrl Pts',(-42.6299160339596,30.8062603392753,
-46.7405972964818));
#237686=CARTESIAN_POINT('Ctrl Pts',(-42.5511871182224,31.0534597168105,
-46.7258129815627));
#237687=CARTESIAN_POINT('Ctrl Pts',(-42.4912834411294,31.567196639013,-46.6981127528274));
#237688=CARTESIAN_POINT('Ctrl Pts',(-42.5118432659359,31.8289562196735,
-46.6852618412255));
#237689=CARTESIAN_POINT('Ctrl Pts',(-42.653100990733,32.3336677708646,-46.6556447311323));
#237690=CARTESIAN_POINT('Ctrl Pts',(-42.7738520231998,32.5712535567185,
-46.6401204319946));
#237691=CARTESIAN_POINT('Ctrl Pts',(-43.0945944652074,32.9781731096842,
-46.6102086216764));
#237692=CARTESIAN_POINT('Ctrl Pts',(-43.2885188885881,33.1459085169591,
-46.5960836249017));
#237693=CARTESIAN_POINT('Ctrl Pts',(-43.738147121595,33.4053064718327,-46.5698553113095));
#237694=CARTESIAN_POINT('Ctrl Pts',(-43.9917954352067,33.4907881687241,
-46.5550591596821));
#237695=CARTESIAN_POINT('Ctrl Pts',(-44.5133362311153,33.557373773589,-46.5246359465874));
#237696=CARTESIAN_POINT('Ctrl Pts',(-44.7759962087206,33.5394933565031,
-46.5093141145603));
#237697=CARTESIAN_POINT('Ctrl Pts',(-45.2727989878659,33.4057598484895,
-46.4803339524434));
#237698=CARTESIAN_POINT('Ctrl Pts',(-45.5029417480266,33.2938328714309,
-46.4678403455768));
#237699=CARTESIAN_POINT('Ctrl Pts',(-45.9184513158687,32.9829695593626,
-46.4400170775355));
#237700=CARTESIAN_POINT('Ctrl Pts',(-46.0970988735073,32.7834089690963,
-46.4247250922264));
#237701=CARTESIAN_POINT('Ctrl Pts',(-46.3623616986635,32.3326811878688,
-46.3942183268163));
#237702=CARTESIAN_POINT('Ctrl Pts',(-46.448949684947,32.0872788365525,-46.3792955714436));
#237703=CARTESIAN_POINT('Ctrl Pts',(-46.5242122990237,31.5768211820417,
-46.3513130362452));
#237704=CARTESIAN_POINT('Ctrl Pts',(-46.5120818147021,31.3166221890583,
-46.3387629497789));
#237705=CARTESIAN_POINT('Ctrl Pts',(-46.3879880918281,30.8086117835772,
-46.3094798043972));
#237706=CARTESIAN_POINT('Ctrl Pts',(-46.2746832139355,30.5664030893519,
-46.293939143996));
#237707=CARTESIAN_POINT('Ctrl Pts',(-45.9662539710802,30.1482250005864,
-46.2638177082691));
#237708=CARTESIAN_POINT('Ctrl Pts',(-45.7771529020937,29.9738907471899,
-46.2494952167125));
#237709=CARTESIAN_POINT('Ctrl Pts',(-45.3326938112695,29.6988515142441,
-46.2226373537353));
#237710=CARTESIAN_POINT('Ctrl Pts',(-45.0789563152446,29.6050636206244,
-46.20825855832));
#237711=CARTESIAN_POINT('Ctrl Pts',(-44.7126485077894,29.5483025272819,
-46.1868906028852));
#237712=CARTESIAN_POINT('Ctrl Pts',(-44.6102608596984,29.5404524382925,
-46.18091799008));
#237713=CARTESIAN_POINT('Ctrl Pts',(-44.5079524583208,29.5404524382925,
-46.1749499999996));
#237714=CARTESIAN_POINT('Ctrl Pts',(-44.5079524583208,29.5404524382925,
-46.0162000000005));
#237715=CARTESIAN_POINT('Ctrl Pts',(-44.5383536771069,29.5404524382925,
-46.0179734044297));
#237716=CARTESIAN_POINT('Ctrl Pts',(-44.5687810503939,29.5411456067265,
-46.0197483345381));
#237717=CARTESIAN_POINT('Ctrl Pts',(-44.8554070412256,29.5542378028698,
-46.0364681840033));
#237718=CARTESIAN_POINT('Ctrl Pts',(-45.1070127036482,29.6151117604346,
-46.051145180978));
#237719=CARTESIAN_POINT('Ctrl Pts',(-45.5783230337682,29.8308201602911,
-46.0786382835683));
#237720=CARTESIAN_POINT('Ctrl Pts',(-45.7926673939301,29.9854378464794,
-46.0917810608028));
#237721=CARTESIAN_POINT('Ctrl Pts',(-46.15067990082,30.3696491201322,-46.1216327344523));
#237722=CARTESIAN_POINT('Ctrl Pts',(-46.2903845425981,30.5958548497405,
-46.137134947823));
#237723=CARTESIAN_POINT('Ctrl Pts',(-46.470781347776,31.0803748758474,-46.1668735759635));
#237724=CARTESIAN_POINT('Ctrl Pts',(-46.5132304133134,31.3327377152465,
-46.1805526964107));
#237725=CARTESIAN_POINT('Ctrl Pts',(-46.5013618106744,31.8512900681338,
-46.2070951687838));
#237726=CARTESIAN_POINT('Ctrl Pts',(-46.4426453630262,32.1124787945741,
-46.2220025027231));
#237727=CARTESIAN_POINT('Ctrl Pts',(-46.2288377388442,32.5922400048864,
-46.2524752065213));
#237728=CARTESIAN_POINT('Ctrl Pts',(-46.0775458753399,32.8069810465109,
-46.2677362057149));
#237729=CARTESIAN_POINT('Ctrl Pts',(-45.705574354989,33.162272184137,-46.2965340255289));
#237730=CARTESIAN_POINT('Ctrl Pts',(-45.4900510161627,33.3011542993969,
-46.308910917459));
#237731=CARTESIAN_POINT('Ctrl Pts',(-45.0061505371029,33.4957832007704,
-46.337138445404));
#237732=CARTESIAN_POINT('Ctrl Pts',(-44.7405522996734,33.5447939295987,
-46.3526316759207));
#237733=CARTESIAN_POINT('Ctrl Pts',(-44.2160984402956,33.5356850725764,
-46.3832248177176));
#237734=CARTESIAN_POINT('Ctrl Pts',(-43.9622017190187,33.4816688204458,
-46.3980354597921));
#237735=CARTESIAN_POINT('Ctrl Pts',(-43.4864450689416,33.2794138062905,
-46.4257879310466));
#237736=CARTESIAN_POINT('Ctrl Pts',(-43.26950932895,33.1322243219307,-46.4385745561242));
#237737=CARTESIAN_POINT('Ctrl Pts',(-42.9009215232177,32.7599607115152,
-46.4681311021637));
#237738=CARTESIAN_POINT('Ctrl Pts',(-42.754110809741,32.5373365857783,-46.4836596399625));
#237739=CARTESIAN_POINT('Ctrl Pts',(-42.5591896442861,32.0571131135749,
-46.5136048413296));
#237740=CARTESIAN_POINT('Ctrl Pts',(-42.509344177805,31.8054569258723,-46.5277718721102));
#237741=CARTESIAN_POINT('Ctrl Pts',(-42.5065609942799,31.2862157253844,
-46.5540841523981));
#237742=CARTESIAN_POINT('Ctrl Pts',(-42.5578084465479,31.0234825992861,
-46.5687704921146));
#237743=CARTESIAN_POINT('Ctrl Pts',(-42.7582857197508,30.5370872462227,
-46.5991895386185));
#237744=CARTESIAN_POINT('Ctrl Pts',(-42.9039655063881,30.3176230386802,
-46.6145254578345));
#237745=CARTESIAN_POINT('Ctrl Pts',(-43.2662348402282,29.9522288050545,
-46.6435506869134));
#237746=CARTESIAN_POINT('Ctrl Pts',(-43.477368658903,29.8077676195006,-46.6560826117008));
#237747=CARTESIAN_POINT('Ctrl Pts',(-43.9531006830822,29.6007360692539,
-46.6838336464447));
#237748=CARTESIAN_POINT('Ctrl Pts',(-44.2149321958984,29.5443404907937,
-46.6991071513591));
#237749=CARTESIAN_POINT('Ctrl Pts',(-44.4893817598351,29.5405170815757,
-46.7151167092554));
#237750=CARTESIAN_POINT('Ctrl Pts',(-44.4986685396741,29.5404524382925,
-46.7156584380794));
#237751=CARTESIAN_POINT('Ctrl Pts',(-44.5079524583208,29.5404524382925,
-46.7162000000005));
#237752=CARTESIAN_POINT('Origin',(-44.5079524583208,31.5404524382925,235.35105));
#237753=CARTESIAN_POINT('',(-44.5079524583208,29.5404524382925,-45.3162000000005));
#237754=CARTESIAN_POINT('',(-44.5079524583208,29.5404524382925,-45.4749499999996));
#237755=CARTESIAN_POINT('',(-44.5079524583208,29.5404524382925,235.35105));
#237756=CARTESIAN_POINT('Ctrl Pts',(-44.5079524583208,29.5404524382925,
-46.1749499999996));
#237757=CARTESIAN_POINT('Ctrl Pts',(-44.3499883457847,29.5404524382925,
-46.1657354267684));
#237758=CARTESIAN_POINT('Ctrl Pts',(-44.1922131522001,29.5591675560845,
-46.1565318738093));
#237759=CARTESIAN_POINT('Ctrl Pts',(-43.7916928277782,29.6559975471492,
-46.1331681882181));
#237760=CARTESIAN_POINT('Ctrl Pts',(-43.5590243839374,29.7617710997056,
-46.1204619525901));
#237761=CARTESIAN_POINT('Ctrl Pts',(-43.1358040936022,30.0614127809282,
-46.0929806844905));
#237762=CARTESIAN_POINT('Ctrl Pts',(-42.9519999941258,30.2561932014292,
-46.0777797853709));
#237763=CARTESIAN_POINT('Ctrl Pts',(-42.6746557778512,30.7003211188648,
-46.047254058953));
#237764=CARTESIAN_POINT('Ctrl Pts',(-42.5815292159222,30.9440327901853,
-46.0322260051473));
#237765=CARTESIAN_POINT('Ctrl Pts',(-42.4935001036119,31.4516693923597,
-46.0040136280915));
#237766=CARTESIAN_POINT('Ctrl Pts',(-42.4987391411722,31.7106454145308,
-45.9916208876941));
#237767=CARTESIAN_POINT('Ctrl Pts',(-42.6087130924422,32.2211856295038,
-45.9626217676926));
#237768=CARTESIAN_POINT('Ctrl Pts',(-42.71576292151,32.46702931215,-45.9470799133305));
#237769=CARTESIAN_POINT('Ctrl Pts',(-43.0138453266327,32.8943041431967,
-45.9168007097928));
#237770=CARTESIAN_POINT('Ctrl Pts',(-43.1988484496968,33.0739317835504,
-45.9023303295503));
#237771=CARTESIAN_POINT('Ctrl Pts',(-43.6345701344869,33.3591136145181,
-45.8752149223088));
#237772=CARTESIAN_POINT('Ctrl Pts',(-43.8831646935248,33.4587903990257,
-45.8613959529469));
#237773=CARTESIAN_POINT('Ctrl Pts',(-44.4018450959186,33.5547728555338,
-45.8311395961405));
#237774=CARTESIAN_POINT('Ctrl Pts',(-44.6665470282396,33.5513217783439,
-45.8156986500884));
#237775=CARTESIAN_POINT('Ctrl Pts',(-45.1708172757467,33.4443351603151,
-45.7862828856504));
#237776=CARTESIAN_POINT('Ctrl Pts',(-45.4062982186259,33.3451934933126,
-45.7732537587104));
#237777=CARTESIAN_POINT('Ctrl Pts',(-45.8377023124348,33.0577188693083,
-45.7461484535465));
#237778=CARTESIAN_POINT('Ctrl Pts',(-46.0269178118715,32.8682447374916,
-45.7310577858079));
#237779=CARTESIAN_POINT('Ctrl Pts',(-46.3171023630338,32.4315978014306,
-45.7005354749506));
#237780=CARTESIAN_POINT('Ctrl Pts',(-46.4172456921539,32.189901539422,-45.6854045801821));
#237781=CARTESIAN_POINT('Ctrl Pts',(-46.5189861151194,31.6853905271185,
-45.656950188912));
#237782=CARTESIAN_POINT('Ctrl Pts',(-46.5210440443298,31.4276495789899,
-45.6446332463212));
#237783=CARTESIAN_POINT('Ctrl Pts',(-46.4260812542442,30.9145917233784,
-45.6159447653103));
#237784=CARTESIAN_POINT('Ctrl Pts',(-46.3258014972443,30.6650555678543,
-45.6004138344901));
#237785=CARTESIAN_POINT('Ctrl Pts',(-46.0390006125387,30.2283874424556,
-45.5699891434584));
#237786=CARTESIAN_POINT('Ctrl Pts',(-45.8585125153081,30.0432387913122,
-45.5553715402261));
#237787=CARTESIAN_POINT('Ctrl Pts',(-45.4320917831814,29.7474100204124,
-45.5279895470776));
#237788=CARTESIAN_POINT('Ctrl Pts',(-45.1888087028346,29.6416361403906,
-45.5146666142627));
#237789=CARTESIAN_POINT('Ctrl Pts',(-44.7923251502757,29.5556220098947,
-45.4915384070302));
#237790=CARTESIAN_POINT('Ctrl Pts',(-44.6501700009571,29.5404524382925,
-45.4832460233201));
#237791=CARTESIAN_POINT('Ctrl Pts',(-44.5079524583208,29.5404524382925,
-45.4749499999996));
#237792=CARTESIAN_POINT('Ctrl Pts',(-44.5079524583208,29.5404524382925,
-45.3162000000005));
#237793=CARTESIAN_POINT('Ctrl Pts',(-44.5752886867944,29.5404524382925,
-45.3201279466614));
#237794=CARTESIAN_POINT('Ctrl Pts',(-44.6427020885513,29.5438529784239,
-45.324060395097));
#237795=CARTESIAN_POINT('Ctrl Pts',(-44.9637283423644,29.5764404651513,
-45.3427869265695));
#237796=CARTESIAN_POINT('Ctrl Pts',(-45.2103073144421,29.6505276104354,
-45.357170699941));
#237797=CARTESIAN_POINT('Ctrl Pts',(-45.6725387562852,29.8927703223525,
-45.3841342007152));
#237798=CARTESIAN_POINT('Ctrl Pts',(-45.8816674111162,30.0625838873391,
-45.3982741697899));
#237799=CARTESIAN_POINT('Ctrl Pts',(-46.2178256572483,30.4704768600807,
-45.4286847830932));
#237800=CARTESIAN_POINT('Ctrl Pts',(-46.3430369784634,30.7032045710331,
-45.4440937530365));
#237801=CARTESIAN_POINT('Ctrl Pts',(-46.4942135996953,31.1955882923935,
-45.473377385137));
#237802=CARTESIAN_POINT('Ctrl Pts',(-46.5218734780736,31.4496006556456,
-45.4862043064054));
#237803=CARTESIAN_POINT('Ctrl Pts',(-46.4799910133021,31.9663710348521,
-45.5135321610796));
#237804=CARTESIAN_POINT('Ctrl Pts',(-46.4061981185894,32.2238006132641,
-45.5286893195264));
#237805=CARTESIAN_POINT('Ctrl Pts',(-46.1655110794876,32.6891241595004,
-45.5592166422012));
#237806=CARTESIAN_POINT('Ctrl Pts',(-46.0031516230724,32.8937264714402,
-45.5742882563357));
#237807=CARTESIAN_POINT('Ctrl Pts',(-45.61145913328,33.2280228330628,-45.6026006538787));
#237808=CARTESIAN_POINT('Ctrl Pts',(-45.3865124168643,33.3553228205668,
-45.6149506690847));
#237809=CARTESIAN_POINT('Ctrl Pts',(-44.8915620166817,33.5212403492853,
-45.6438227757619));
#237810=CARTESIAN_POINT('Ctrl Pts',(-44.625181292559,33.5546303190202,-45.6593616513357));
#237811=CARTESIAN_POINT('Ctrl Pts',(-44.1050333555753,33.5160717933918,
-45.6897036143263));
#237812=CARTESIAN_POINT('Ctrl Pts',(-43.8559077769371,33.4484077857242,
-45.7042359397469));
#237813=CARTESIAN_POINT('Ctrl Pts',(-43.3891733207894,33.2191740955852,
-45.7314621163555));
#237814=CARTESIAN_POINT('Ctrl Pts',(-43.1774647128587,33.0569025576557,
-45.7450643068372));
#237815=CARTESIAN_POINT('Ctrl Pts',(-42.8304222957157,32.6606348682511,
-45.7752050873378));
#237816=CARTESIAN_POINT('Ctrl Pts',(-42.6980291883871,32.4310106793887,
-45.7906667418528));
#237817=CARTESIAN_POINT('Ctrl Pts',(-42.5324528658392,31.9424334735313,
-45.8201780671262));
#237818=CARTESIAN_POINT('Ctrl Pts',(-42.4974840288384,31.6892830248564,
-45.8333760251249));
#237819=CARTESIAN_POINT('Ctrl Pts',(-42.5244614333995,31.1715527096957,
-45.8603176430636));
#237820=CARTESIAN_POINT('Ctrl Pts',(-42.5907918097007,30.9121428759785,
-45.8753571835553));
#237821=CARTESIAN_POINT('Ctrl Pts',(-42.8182406097052,30.439455042982,-45.9058704210559));
#237822=CARTESIAN_POINT('Ctrl Pts',(-42.9751815563657,30.2297448947546,
-45.9210420337551));
#237823=CARTESIAN_POINT('Ctrl Pts',(-43.3571097235158,29.8849776008381,
-45.9495986106678));
#237824=CARTESIAN_POINT('Ctrl Pts',(-43.5773052343559,29.7518975545269,
-45.9619122452689));
#237825=CARTESIAN_POINT('Ctrl Pts',(-44.0382118459221,29.5821060668551,
-45.9887984642771));
#237826=CARTESIAN_POINT('Ctrl Pts',(-44.2722963888769,29.5404524382925,
-46.0024533959495));
#237827=CARTESIAN_POINT('Ctrl Pts',(-44.5079524583208,29.5404524382925,
-46.0162000000005));
#237828=CARTESIAN_POINT('Origin',(-44.5079524583208,31.5404524382925,235.35105));
#237829=CARTESIAN_POINT('',(-44.5079524583208,29.5404524382925,-44.6162000000005));
#237830=CARTESIAN_POINT('',(-44.5079524583208,29.5404524382925,-44.7749499999996));
#237831=CARTESIAN_POINT('',(-44.5079524583208,29.5404524382925,235.35105));
#237832=CARTESIAN_POINT('Ctrl Pts',(-44.5079524583208,29.5404524382925,
-45.4749499999996));
#237833=CARTESIAN_POINT('Ctrl Pts',(-44.3884404302508,29.5404524382925,
-45.4679784650289));
#237834=CARTESIAN_POINT('Ctrl Pts',(-44.2688843411178,29.5511646694685,
-45.4610043598295));
#237835=CARTESIAN_POINT('Ctrl Pts',(-43.9012887286443,29.6178935469937,
-45.4395612824353));
#237836=CARTESIAN_POINT('Ctrl Pts',(-43.6627974894879,29.7101746456848,
-45.4260952254977));
#237837=CARTESIAN_POINT('Ctrl Pts',(-43.2230751000556,29.9850100727128,
-45.3993858122089));
#237838=CARTESIAN_POINT('Ctrl Pts',(-43.0284398716923,30.1688457313581,
-45.3844219142687));
#237839=CARTESIAN_POINT('Ctrl Pts',(-42.7252141543255,30.5973786185983,
-45.3539291427878));
#237840=CARTESIAN_POINT('Ctrl Pts',(-42.6178693581101,30.8367857273349,
-45.3387038490141));
#237841=CARTESIAN_POINT('Ctrl Pts',(-42.5020198797053,31.3379781831177,
-45.3100055909587));
#237842=CARTESIAN_POINT('Ctrl Pts',(-42.4925541004512,31.5945318855494,
-45.2976671252213));
#237843=CARTESIAN_POINT('Ctrl Pts',(-42.5722405742376,32.1099813837036,
-45.2693033820827));
#237844=CARTESIAN_POINT('Ctrl Pts',(-42.6655125922908,32.3630878196491,
-45.2537964796918));
#237845=CARTESIAN_POINT('Ctrl Pts',(-42.9405500282181,32.8090078723666,
-45.2232474990108));
#237846=CARTESIAN_POINT('Ctrl Pts',(-43.1162818009553,32.9996544475994,
-45.2084908769637));
#237847=CARTESIAN_POINT('Ctrl Pts',(-43.533224312882,33.3061798501348,-45.1808449578783));
#237848=CARTESIAN_POINT('Ctrl Pts',(-43.7712693626966,33.4180055638395,
-45.1679231805785));
#237849=CARTESIAN_POINT('Ctrl Pts',(-44.28006033097,33.544858196687,-45.1382437074292));
#237850=CARTESIAN_POINT('Ctrl Pts',(-44.5461058074549,33.5574089118735,
-45.1227243879675));
#237851=CARTESIAN_POINT('Ctrl Pts',(-45.0581062113836,33.4800081747317,
-45.0928576977382));
#237852=CARTESIAN_POINT('Ctrl Pts',(-45.2996831041404,33.3945297789453,
-45.078855744023));
#237853=CARTESIAN_POINT('Ctrl Pts',(-45.7474950569434,33.132250299015,-45.0525446883363));
#237854=CARTESIAN_POINT('Ctrl Pts',(-45.9473071006096,32.9541327539777,
-45.0377186684623));
#237855=CARTESIAN_POINT('Ctrl Pts',(-46.2631753763515,32.5339890935242,
-45.0072809639001));
#237856=CARTESIAN_POINT('Ctrl Pts',(-46.377577875197,32.2970472517023,-44.9919743611866));
#237857=CARTESIAN_POINT('Ctrl Pts',(-46.5073145669426,31.7992306316387,
-44.9630416003788));
#237858=CARTESIAN_POINT('Ctrl Pts',(-46.5239858684761,31.5437495211416,
-44.9505842036502));
#237859=CARTESIAN_POINT('Ctrl Pts',(-46.4591671137971,31.0261349851744,
-44.9225447286169));
#237860=CARTESIAN_POINT('Ctrl Pts',(-46.3728195132755,30.7697405399738,
-44.9070736842639));
#237861=CARTESIAN_POINT('Ctrl Pts',(-46.1094871362041,30.3151271858606,
-44.8764269316416));
#237862=CARTESIAN_POINT('Ctrl Pts',(-45.9385337983681,30.1192546985941,
-44.861545677212));
#237863=CARTESIAN_POINT('Ctrl Pts',(-45.530828254992,29.8024494454341,-44.8336498506883));
#237864=CARTESIAN_POINT('Ctrl Pts',(-45.2977182116059,29.6848636532952,
-44.8210196689411));
#237865=CARTESIAN_POINT('Ctrl Pts',(-44.8722812568097,29.5654047678576,
-44.7962025132447));
#237866=CARTESIAN_POINT('Ctrl Pts',(-44.6903467166921,29.5404524382925,
-44.7855896650713));
#237867=CARTESIAN_POINT('Ctrl Pts',(-44.5079524583208,29.5404524382925,
-44.7749499999996));
#237868=CARTESIAN_POINT('Ctrl Pts',(-44.5079524583208,29.5404524382925,
-44.6162000000005));
#237869=CARTESIAN_POINT('Ctrl Pts',(-44.6122192188551,29.5404524382925,
-44.6222822276983));
#237870=CARTESIAN_POINT('Ctrl Pts',(-44.716562581159,29.5486059400025,-44.6283689238327));
#237871=CARTESIAN_POINT('Ctrl Pts',(-45.0843777019556,29.6067092957952,
-44.6498248058792));
#237872=CARTESIAN_POINT('Ctrl Pts',(-45.3375946885842,29.7010931643449,
-44.6641435400043));
#237873=CARTESIAN_POINT('Ctrl Pts',(-45.7811807138443,29.9771521689784,
-44.6910274555468));
#237874=CARTESIAN_POINT('Ctrl Pts',(-45.9698787058019,30.15201982734,-44.7053651373213));
#237875=CARTESIAN_POINT('Ctrl Pts',(-46.2772853751844,30.5711184567403,
-44.7355032519971));
#237876=CARTESIAN_POINT('Ctrl Pts',(-46.389970016758,30.8136974900051,-44.7510445310149));
#237877=CARTESIAN_POINT('Ctrl Pts',(-46.5126520729056,31.3219681554154,
-44.7802996506334));
#237878=CARTESIAN_POINT('Ctrl Pts',(-46.5240920270596,31.5820422493856,
-44.7928303028339));
#237879=CARTESIAN_POINT('Ctrl Pts',(-46.4475585219114,32.0922229686962,
-44.8208359154349));
#237880=CARTESIAN_POINT('Ctrl Pts',(-46.3603196882749,32.3374650435143,
-44.8357695569832));
#237881=CARTESIAN_POINT('Ctrl Pts',(-46.0938493289167,32.7875517806148,
-44.8662791577781));
#237882=CARTESIAN_POINT('Ctrl Pts',(-45.9146836175038,32.9866436168496,
-44.8815625753197));
#237883=CARTESIAN_POINT('Ctrl Pts',(-45.4984024727998,33.2963945808861,
-44.9093521539228));
#237884=CARTESIAN_POINT('Ctrl Pts',(-45.268012095978,33.4077096809596,-44.9218631878031));
#237885=CARTESIAN_POINT('Ctrl Pts',(-44.7708483802375,33.5401854738332,
-44.9508644045545));
#237886=CARTESIAN_POINT('Ctrl Pts',(-44.5080747570903,33.5573895966803,
-44.9661928659047));
#237887=CARTESIAN_POINT('Ctrl Pts',(-43.9864789169903,33.4893962270578,
-44.9966192899104));
#237888=CARTESIAN_POINT('Ctrl Pts',(-43.7330682428071,33.4031791871255,
-45.0113659496721));
#237889=CARTESIAN_POINT('Ctrl Pts',(-43.2840691961485,33.1425552376921,
-45.0376279945938));
#237890=CARTESIAN_POINT('Ctrl Pts',(-43.0905893083135,32.974208798702,-45.0517757084025));
#237891=CARTESIAN_POINT('Ctrl Pts',(-42.7709778104767,32.5664218049919,
-45.0816983543494));
#237892=CARTESIAN_POINT('Ctrl Pts',(-42.6508593773377,32.3284303032967,
-45.0972246986866));
#237893=CARTESIAN_POINT('Ctrl Pts',(-42.5110760907483,31.8234254495933,
-45.1268136214321));
#237894=CARTESIAN_POINT('Ctrl Pts',(-42.4912430285492,31.5618027775643,
-45.1396340620203));
#237895=CARTESIAN_POINT('Ctrl Pts',(-42.5524594664912,31.048341281544,-45.1673586655931));
#237896=CARTESIAN_POINT('Ctrl Pts',(-42.6318594285012,30.8012854209585,
-45.1821553024847));
#237897=CARTESIAN_POINT('Ctrl Pts',(-42.8847087561168,30.3419026329704,
-45.2127372424671));
#237898=CARTESIAN_POINT('Ctrl Pts',(-43.0592496209379,30.1359121223225,
-45.2282342769088));
#237899=CARTESIAN_POINT('Ctrl Pts',(-43.4687171145355,29.8128472013648,
-45.2564977204751));
#237900=CARTESIAN_POINT('Ctrl Pts',(-43.6964582419797,29.6948860705821,
-45.2688628373804));
#237901=CARTESIAN_POINT('Ctrl Pts',(-44.1248814272467,29.5680588587409,
-45.2938541898544));
#237902=CARTESIAN_POINT('Ctrl Pts',(-44.3161037171375,29.5404524382925,
-45.3050088234314));
#237903=CARTESIAN_POINT('Ctrl Pts',(-44.5079524583208,29.5404524382925,
-45.3162000000005));
#237904=CARTESIAN_POINT('Origin',(-44.5079524583208,31.5404524382925,235.35105));
#237905=CARTESIAN_POINT('',(-44.5079524583208,29.5404524382925,-43.9162000000005));
#237906=CARTESIAN_POINT('',(-44.5079524583208,29.5404524382925,-44.0749499999996));
#237907=CARTESIAN_POINT('',(-44.5079524583208,29.5404524382925,235.35105));
#237908=CARTESIAN_POINT('Ctrl Pts',(-44.5079524583208,29.5404524382925,
-44.7749499999996));
#237909=CARTESIAN_POINT('Ctrl Pts',(-44.4269158891708,29.5404524382925,
-44.7702228667993));
#237910=CARTESIAN_POINT('Ctrl Pts',(-44.3457885731801,29.5453774932786,
-44.7654904400331));
#237911=CARTESIAN_POINT('Ctrl Pts',(-44.0123133744175,29.5861855354304,
-44.7460377201053));
#237912=CARTESIAN_POINT('Ctrl Pts',(-43.7677747684345,29.6650857813368,
-44.7317729680897));
#237913=CARTESIAN_POINT('Ctrl Pts',(-43.3123227136843,29.9154252946429,
-44.7052049315628));
#237914=CARTESIAN_POINT('Ctrl Pts',(-43.1076607188679,30.0880337573836,
-44.6908149936175));
#237915=CARTESIAN_POINT('Ctrl Pts',(-42.7799440122894,30.5001310234453,
-44.6604381987701));
#237916=CARTESIAN_POINT('Ctrl Pts',(-42.658943374774,30.7345646059895,-44.6450658629603));
#237917=CARTESIAN_POINT('Ctrl Pts',(-42.5161481504766,31.2291048648655,
-44.6159177439879));
#237918=CARTESIAN_POINT('Ctrl Pts',(-42.4927668196029,31.4836645710956,
-44.6032617323741));
#237919=CARTESIAN_POINT('Ctrl Pts',(-42.5434285080603,31.9997976447559,
-44.5757100125053));
#237920=CARTESIAN_POINT('Ctrl Pts',(-42.6215891793797,32.2559573025136,
-44.5604896146143));
#237921=CARTESIAN_POINT('Ctrl Pts',(-42.8699633092896,32.7167686211005,
-44.5299660345109));
#237922=CARTESIAN_POINT('Ctrl Pts',(-43.035439322463,32.9182984430415,-44.5149587373105));
#237923=CARTESIAN_POINT('Ctrl Pts',(-43.4328587864362,33.2463868218929,
-44.4867929188162));
#237924=CARTESIAN_POINT('Ctrl Pts',(-43.6606686457498,33.3702482293867,
-44.4743748890671));
#237925=CARTESIAN_POINT('Ctrl Pts',(-44.1587978262492,33.5275409238952,
-44.4453173535379));
#237926=CARTESIAN_POINT('Ctrl Pts',(-44.4252408746356,33.5562821846605,
-44.429774842382));
#237927=CARTESIAN_POINT('Ctrl Pts',(-44.9437910037961,33.5090174220985,
-44.3995260848475));
#237928=CARTESIAN_POINT('Ctrl Pts',(-45.1913516937128,33.4373475623424,
-44.3850850446023));
#237929=CARTESIAN_POINT('Ctrl Pts',(-45.6552987634885,33.2000269091421,
-44.3580214655319));
#237930=CARTESIAN_POINT('Ctrl Pts',(-45.8654097666201,33.0330879397658,
-44.3440960105084));
#237931=CARTESIAN_POINT('Ctrl Pts',(-46.2057253231842,32.6295959221004,
-44.3137864704197));
#237932=CARTESIAN_POINT('Ctrl Pts',(-46.3336705246337,32.3980205000053,
-44.2983559738024));
#237933=CARTESIAN_POINT('Ctrl Pts',(-46.4903121008032,31.9070661004001,
-44.2689851538715));
#237934=CARTESIAN_POINT('Ctrl Pts',(-46.520751545409,31.6533923832289,-44.2560288236222));
#237935=CARTESIAN_POINT('Ctrl Pts',(-46.4845522240017,31.1362381260368,
-44.2288473344909));
#237936=CARTESIAN_POINT('Ctrl Pts',(-46.4135981899322,30.8780272756441,
-44.2137335077321));
#237937=CARTESIAN_POINT('Ctrl Pts',(-46.1779317184528,30.4098513143393,
-44.1832085195513));
#237938=CARTESIAN_POINT('Ctrl Pts',(-46.0176196702392,30.2032850039629,
-44.1680974039245));
#237939=CARTESIAN_POINT('Ctrl Pts',(-45.6296444473373,29.8649864588488,
-44.1396912437655));
#237940=CARTESIAN_POINT('Ctrl Pts',(-45.4065243784234,29.7354739554711,
-44.1273666953388));
#237941=CARTESIAN_POINT('Ctrl Pts',(-44.9534608432788,29.5778783047637,
-44.1009379891221));
#237942=CARTESIAN_POINT('Ctrl Pts',(-44.7313283970238,29.5404524382925,
-44.0879802630906));
#237943=CARTESIAN_POINT('Ctrl Pts',(-44.5079524583208,29.5404524382925,
-44.0749499999997));
#237944=CARTESIAN_POINT('Ctrl Pts',(-44.5079524583208,29.5404524382925,
-43.9162000000005));
#237945=CARTESIAN_POINT('Ctrl Pts',(-44.6523156556797,29.5404524382925,
-43.9246211865131));
#237946=CARTESIAN_POINT('Ctrl Pts',(-44.7966026468966,29.5560832331624,
-43.9330379276674));
#237947=CARTESIAN_POINT('Ctrl Pts',(-45.1946723394097,29.6437828286242,
-43.9562586597307));
#237948=CARTESIAN_POINT('Ctrl Pts',(-45.4374028973042,29.7501928106054,
-43.9695350359824));
#237949=CARTESIAN_POINT('Ctrl Pts',(-45.8628387194137,30.0471402137679,
-43.9969448138196));
#237950=CARTESIAN_POINT('Ctrl Pts',(-46.042839741025,30.2328663342062,-44.0115773833593));
#237951=CARTESIAN_POINT('Ctrl Pts',(-46.3284304855397,30.6705111297737,
-44.042016118204));
#237952=CARTESIAN_POINT('Ctrl Pts',(-46.4279869739964,30.9204274153687,
-44.057545157159));
#237953=CARTESIAN_POINT('Ctrl Pts',(-46.5213614199234,31.4337420706773,
-44.0862002845104));
#237954=CARTESIAN_POINT('Ctrl Pts',(-46.5185326280804,31.6913556855195,
-44.0985147643764));
#237955=CARTESIAN_POINT('Ctrl Pts',(-46.4153325676931,32.1955284989266,
-44.1269946432222));
#237956=CARTESIAN_POINT('Ctrl Pts',(-46.3144431403658,32.4369980572508,
-44.1421358465379));
#237957=CARTESIAN_POINT('Ctrl Pts',(-46.0229009685275,32.8728250015037,
-44.1726563301967));
#237958=CARTESIAN_POINT('Ctrl Pts',(-45.8331176096775,33.0617240701592,
-44.1877345093751));
#237959=CARTESIAN_POINT('Ctrl Pts',(-45.4008481988035,33.3478966983426,
-44.2147992785349));
#237960=CARTESIAN_POINT('Ctrl Pts',(-45.1650614423334,33.4463305633755,
-44.227868642599));
#237961=CARTESIAN_POINT('Ctrl Pts',(-44.6603833204181,33.551808762868,-44.2573081997106));
#237962=CARTESIAN_POINT('Ctrl Pts',(-44.3955896792146,33.5544440813145,
-44.2727544954474));
#237963=CARTESIAN_POINT('Ctrl Pts',(-43.8773970976013,33.456865381138,-44.3029823960414));
#237964=CARTESIAN_POINT('Ctrl Pts',(-43.6293512739145,33.3565598115926,
-44.3167461524701));
#237965=CARTESIAN_POINT('Ctrl Pts',(-43.1945769409543,33.0702865657418,
-44.3438890648757));
#237966=CARTESIAN_POINT('Ctrl Pts',(-43.0100265915509,32.890091094939,-44.3583749249628));
#237967=CARTESIAN_POINT('Ctrl Pts',(-42.7130809076758,32.4618456208354,
-44.3886700092209));
#237968=CARTESIAN_POINT('Ctrl Pts',(-42.6067155290989,32.2156174147622,
-44.4042113258553));
#237969=CARTESIAN_POINT('Ctrl Pts',(-42.498271475132,31.7048127455013,-44.4331791835933));
#237970=CARTESIAN_POINT('Ctrl Pts',(-42.4937772998067,31.4459655722021,
-44.4455598594139));
#237971=CARTESIAN_POINT('Ctrl Pts',(-42.583197121164,30.9386415599925,-44.4737970073508));
#237972=CARTESIAN_POINT('Ctrl Pts',(-42.6770358458382,30.6951248891461,
-44.4888359815071));
#237973=CARTESIAN_POINT('Ctrl Pts',(-42.955689210157,30.2517373390094,-44.5193624894247));
#237974=CARTESIAN_POINT('Ctrl Pts',(-43.1400483434228,30.0574871098765,
-44.5345527927437));
#237975=CARTESIAN_POINT('Ctrl Pts',(-43.5641032727125,29.7590741737154,
-44.5619963305543));
#237976=CARTESIAN_POINT('Ctrl Pts',(-43.7970521365803,29.6539720334572,
-44.5747308145655));
#237977=CARTESIAN_POINT('Ctrl Pts',(-44.1959803359963,29.5587218245104,
-44.5980016261982));
#237978=CARTESIAN_POINT('Ctrl Pts',(-44.3518805815372,29.5404524382925,
-44.6070958071881));
#237979=CARTESIAN_POINT('Ctrl Pts',(-44.5079524583208,29.5404524382925,
-44.6162000000005));
#237980=CARTESIAN_POINT('Origin',(-44.5079524583208,31.5404524382925,235.35105));
#237981=CARTESIAN_POINT('',(-44.5079524583208,29.5404524382925,-43.2162000000004));
#237982=CARTESIAN_POINT('',(-44.5079524583208,29.5404524382925,-43.3749499999997));
#237983=CARTESIAN_POINT('',(-44.5079524583208,29.5404524382925,235.35105));
#237984=CARTESIAN_POINT('Ctrl Pts',(-44.5079524583208,29.5404524382925,
-44.0749499999997));
#237985=CARTESIAN_POINT('Ctrl Pts',(-44.4659149033209,29.5404524382925,
-44.0724978092913));
#237986=CARTESIAN_POINT('Ctrl Pts',(-44.4238333085281,29.5417777833755,
-44.070043049595));
#237987=CARTESIAN_POINT('Ctrl Pts',(-44.1262478307761,29.5605903219429,
-44.0526838967262));
#237988=CARTESIAN_POINT('Ctrl Pts',(-43.8761505507025,29.6256632463176,
-44.038094888722));
#237989=CARTESIAN_POINT('Ctrl Pts',(-43.4076485412583,29.8497097904113,
-44.0107656048379));
#237990=CARTESIAN_POINT('Ctrl Pts',(-43.1949244037257,30.009023590732,-43.997351631762));
#237991=CARTESIAN_POINT('Ctrl Pts',(-42.8436338287753,30.4006630372635,
-43.9673207569199));
#237992=CARTESIAN_POINT('Ctrl Pts',(-42.708417399813,30.6289986251821,-43.9518418532579));
#237993=CARTESIAN_POINT('Ctrl Pts',(-42.5371390233473,31.1160320104332,
-43.9222422090375));
#237994=CARTESIAN_POINT('Ctrl Pts',(-42.4992879688712,31.368867795911,-43.9088708527294));
#237995=CARTESIAN_POINT('Ctrl Pts',(-42.5204248231154,31.8869335563989,
-43.8820826380982));
#237996=CARTESIAN_POINT('Ctrl Pts',(-42.5838170893789,32.1470584640277,
-43.8670926682727));
#237997=CARTESIAN_POINT('Ctrl Pts',(-42.8060179358639,32.6225280247556,
-43.8365919683484));
#237998=CARTESIAN_POINT('Ctrl Pts',(-42.9607933466564,32.8342009250777,
-43.8213843625103));
#237999=CARTESIAN_POINT('Ctrl Pts',(-43.3388799803566,33.1830472982667,
-43.7927337627908));
#238000=CARTESIAN_POINT('Ctrl Pts',(-43.5572521065149,33.318375970392,-43.7804075205225));
#238001=CARTESIAN_POINT('Ctrl Pts',(-44.0445925985247,33.504264475221,-43.7519793251552));
#238002=CARTESIAN_POINT('Ctrl Pts',(-44.3105236922181,33.5484994715933,
-43.736466678023));
#238003=CARTESIAN_POINT('Ctrl Pts',(-44.8338347314534,33.5303552378897,
-43.7059402007342));
#238004=CARTESIAN_POINT('Ctrl Pts',(-45.0863523706445,33.4721359389528,
-43.6912100051146));
#238005=CARTESIAN_POINT('Ctrl Pts',(-45.5594039056671,33.2616584557708,
-43.6636153322382));
#238006=CARTESIAN_POINT('Ctrl Pts',(-45.7747585466089,33.1099506004804,
-43.6506229637377));
#238007=CARTESIAN_POINT('Ctrl Pts',(-46.1369220480862,32.7303908260498,
-43.6208852045413));
#238008=CARTESIAN_POINT('Ctrl Pts',(-46.2794099100104,32.5055569114119,
-43.6053711154687));
#238009=CARTESIAN_POINT('Ctrl Pts',(-46.4654971743976,32.0226338617521,
-43.5755471918944));
#238010=CARTESIAN_POINT('Ctrl Pts',(-46.5108100821409,31.7705479030538,
-43.5616573442314));
#238011=CARTESIAN_POINT('Ctrl Pts',(-46.5046812629471,31.251721794336,-43.5352684525709));
#238012=CARTESIAN_POINT('Ctrl Pts',(-46.4488675860034,30.9899180640861,
-43.5204147139232));
#238013=CARTESIAN_POINT('Ctrl Pts',(-46.2402959941818,30.5075754677912,
-43.4899643208948));
#238014=CARTESIAN_POINT('Ctrl Pts',(-46.0911896472629,30.2909636669984,
-43.4746725586453));
#238015=CARTESIAN_POINT('Ctrl Pts',(-45.7230171197802,29.9316987040934,
-43.4457847924941));
#238016=CARTESIAN_POINT('Ctrl Pts',(-45.5092312008947,29.7906239252334,
-43.4333579266496));
#238017=CARTESIAN_POINT('Ctrl Pts',(-45.0316282768101,29.5923624973419,
-43.405497756078));
#238018=CARTESIAN_POINT('Ctrl Pts',(-44.7710344880029,29.5404524382925,
-43.3902964517311));
#238019=CARTESIAN_POINT('Ctrl Pts',(-44.5079524583208,29.5404524382925,
-43.3749499999997));
#238020=CARTESIAN_POINT('Ctrl Pts',(-44.5079524583208,29.5404524382925,
-43.2162000000004));
#238021=CARTESIAN_POINT('Ctrl Pts',(-44.6923124819427,29.5404524382925,
-43.2269543347117));
#238022=CARTESIAN_POINT('Ctrl Pts',(-44.8761848820962,29.5659455735621,
-43.2376802247207));
#238023=CARTESIAN_POINT('Ctrl Pts',(-45.3029944073813,29.6871421391465,
-43.2625774470291));
#238024=CARTESIAN_POINT('Ctrl Pts',(-45.5356162731434,29.8053016743605,
-43.2751835905435));
#238025=CARTESIAN_POINT('Ctrl Pts',(-45.9423907698327,30.1231353045488,
-43.3031042132423));
#238026=CARTESIAN_POINT('Ctrl Pts',(-46.1128549381114,30.3195270278415,
-43.3179974310691));
#238027=CARTESIAN_POINT('Ctrl Pts',(-46.3749950428255,30.7749984950565,
-43.3486527593662));
#238028=CARTESIAN_POINT('Ctrl Pts',(-46.4606399108811,31.0317137236471,
-43.3641195127385));
#238029=CARTESIAN_POINT('Ctrl Pts',(-46.5239611741609,31.549537721084,-43.3921258925448));
#238030=CARTESIAN_POINT('Ctrl Pts',(-46.5065638074057,31.804915466823,-43.404600684881));
#238031=CARTESIAN_POINT('Ctrl Pts',(-46.3754196378857,32.3023837632647,
-43.4335569004592));
#238032=CARTESIAN_POINT('Ctrl Pts',(-46.2603040023265,32.5390640797171,
-43.4488710912159));
#238033=CARTESIAN_POINT('Ctrl Pts',(-45.9431660366353,32.9583356198413,
-43.4793017704969));
#238034=CARTESIAN_POINT('Ctrl Pts',(-45.7428384517924,33.1358646692272,
-43.4941130972777));
#238035=CARTESIAN_POINT('Ctrl Pts',(-45.2942118987344,33.3968653020267,
-43.5203833071489));
#238036=CARTESIAN_POINT('Ctrl Pts',(-45.0523152307769,33.4816508919774,
-43.5344455049398));
#238037=CARTESIAN_POINT('Ctrl Pts',(-44.5399322360448,33.5575267826389,
-43.5643345129657));
#238038=CARTESIAN_POINT('Ctrl Pts',(-44.2738433379105,33.5441523280242,
-43.5798563653568));
#238039=CARTESIAN_POINT('Ctrl Pts',(-43.7655792376963,33.4157336424454,
-43.6095051045359));
#238040=CARTESIAN_POINT('Ctrl Pts',(-43.5280652801099,33.303291173352,-43.6223913602693));
#238041=CARTESIAN_POINT('Ctrl Pts',(-43.1121019935912,32.9956692908682,
-43.6500641107506));
#238042=CARTESIAN_POINT('Ctrl Pts',(-42.936870233636,32.8044624020852,-43.6648344550947));
#238043=CARTESIAN_POINT('Ctrl Pts',(-42.6630627278422,32.3576054412223,
-43.6953948936784));
#238044=CARTESIAN_POINT('Ctrl Pts',(-42.570520521925,32.1041414138609,-43.7108985747384));
#238045=CARTESIAN_POINT('Ctrl Pts',(-42.4924111348435,31.5884547885678,
-43.7392282987389));
#238046=CARTESIAN_POINT('Ctrl Pts',(-42.5026411845677,31.3320188059258,
-43.7515747690521));
#238047=CARTESIAN_POINT('Ctrl Pts',(-42.619956356439,30.8311774693128,-43.7802980386102));
#238048=CARTESIAN_POINT('Ctrl Pts',(-42.7280476853849,30.5920206489724,
-43.7955324621489));
#238049=CARTESIAN_POINT('Ctrl Pts',(-43.0326172146599,30.164354510323,-43.8260206416101));
#238050=CARTESIAN_POINT('Ctrl Pts',(-43.227806385461,29.981114633024,-43.8409705984343));
#238051=CARTESIAN_POINT('Ctrl Pts',(-43.6683870931636,29.7075990362631,
-43.8676383706248));
#238052=CARTESIAN_POINT('Ctrl Pts',(-43.9071981376441,29.616033318842,-43.8811559979609));
#238053=CARTESIAN_POINT('Ctrl Pts',(-44.2729995134149,29.5507984087063,
-43.9024944115476));
#238054=CARTESIAN_POINT('Ctrl Pts',(-44.3905012068673,29.5404524382925,
-43.909348676999));
#238055=CARTESIAN_POINT('Ctrl Pts',(-44.5079524583208,29.5404524382925,
-43.9162000000005));
#238056=CARTESIAN_POINT('Origin',(-44.5079524583208,31.5404524382925,235.35105));
#238057=CARTESIAN_POINT('',(-44.5079524583208,29.5404524382925,-42.5162000000004));
#238058=CARTESIAN_POINT('',(-44.5079524583208,29.5404524382925,-42.6749499999997));
#238059=CARTESIAN_POINT('',(-44.5079524583208,29.5404524382925,235.35105));
#238060=CARTESIAN_POINT('Ctrl Pts',(-44.5079524583208,29.5404524382925,
-43.3749499999997));
#238061=CARTESIAN_POINT('Ctrl Pts',(-44.5034547997409,29.5404524382925,
-43.3746876365825));
#238062=CARTESIAN_POINT('Ctrl Pts',(-44.4989564139122,29.5404676099871,
-43.3744252307424));
#238063=CARTESIAN_POINT('Ctrl Pts',(-44.2370388629623,29.5422349497112,
-43.359146706937));
#238064=CARTESIAN_POINT('Ctrl Pts',(-43.9823295026895,29.593655263083,-43.3442886609212));
#238065=CARTESIAN_POINT('Ctrl Pts',(-43.5049324886095,29.7908658093173,
-43.3164405017666));
#238066=CARTESIAN_POINT('Ctrl Pts',(-43.2870296568381,29.9353163752196,
-43.3037615870405));
#238067=CARTESIAN_POINT('Ctrl Pts',(-42.9145603165496,30.3031142607244,
-43.2743174297311));
#238068=CARTESIAN_POINT('Ctrl Pts',(-42.7651297928638,30.5243514743431,
-43.2587825450337));
#238069=CARTESIAN_POINT('Ctrl Pts',(-42.564801016483,31.0029469157913,-43.228761866781));
#238070=CARTESIAN_POINT('Ctrl Pts',(-42.5122253282156,31.2543241065678,
-43.2145292989398));
#238071=CARTESIAN_POINT('Ctrl Pts',(-42.5040138827789,31.7738205426458,
-43.1880458003169));
#238072=CARTESIAN_POINT('Ctrl Pts',(-42.5525320299186,32.0371029262524,
-43.1735598993653));
#238073=CARTESIAN_POINT('Ctrl Pts',(-42.7480481725244,32.5258203225073,
-43.143168247181));
#238074=CARTESIAN_POINT('Ctrl Pts',(-42.891628989319,32.746984743603,-43.1278076562781));
#238075=CARTESIAN_POINT('Ctrl Pts',(-43.2503117884441,33.1160757216122,
-43.0987002817799));
#238076=CARTESIAN_POINT('Ctrl Pts',(-43.4598617949897,33.2625829045186,
-43.0860886220281));
#238077=CARTESIAN_POINT('Ctrl Pts',(-43.9333164345857,33.4743987861099,
-43.0584704347183));
#238078=CARTESIAN_POINT('Ctrl Pts',(-44.1945469816096,33.5334637551795,
-43.0432319861418));
#238079=CARTESIAN_POINT('Ctrl Pts',(-44.717759448349,33.5461054116061,-43.0127112589153));
#238080=CARTESIAN_POINT('Ctrl Pts',(-44.9746841494797,33.5023014180199,
-42.9977239846826));
#238081=CARTESIAN_POINT('Ctrl Pts',(-45.4567674143157,33.3197568490683,
-42.9696024609003));
#238082=CARTESIAN_POINT('Ctrl Pts',(-45.6774773406108,33.1831302570668,
-42.9571572330085));
#238083=CARTESIAN_POINT('Ctrl Pts',(-46.0609806578878,32.8282641030214,
-42.9280445385009));
#238084=CARTESIAN_POINT('Ctrl Pts',(-46.2178840852463,32.6111864822102,
-42.9125018290403));
#238085=CARTESIAN_POINT('Ctrl Pts',(-46.4337097693197,32.1376109875537,
-42.8822827560641));
#238086=CARTESIAN_POINT('Ctrl Pts',(-46.4941416980732,31.8872012781276,
-42.8678699232418));
#238087=CARTESIAN_POINT('Ctrl Pts',(-46.5180540212289,31.3662663370907,
-42.8408558117447));
#238088=CARTESIAN_POINT('Ctrl Pts',(-46.4770629652323,31.1005455540052,
-42.8268257751206));
#238089=CARTESIAN_POINT('Ctrl Pts',(-46.2948720769304,30.6047659797364,
-42.7964660080287));
#238090=CARTESIAN_POINT('Ctrl Pts',(-46.1571213548608,30.3790580324543,
-42.7810459310244));
#238091=CARTESIAN_POINT('Ctrl Pts',(-45.8082963202166,29.9999125950756,
-42.7517181419849));
#238092=CARTESIAN_POINT('Ctrl Pts',(-45.6029972554696,29.8478219583038,
-42.7388276131664));
#238093=CARTESIAN_POINT('Ctrl Pts',(-45.1357865257117,29.6231199988592,
-42.7115736539305));
#238094=CARTESIAN_POINT('Ctrl Pts',(-44.8763212518798,29.5568694496022,
-42.6964381796237));
#238095=CARTESIAN_POINT('Ctrl Pts',(-44.5770034733222,29.5413456320306,
-42.6789779758746));
#238096=CARTESIAN_POINT('Ctrl Pts',(-44.5424624403491,29.5404524382925,
-42.6769630822846));
#238097=CARTESIAN_POINT('Ctrl Pts',(-44.5079524583208,29.5404524382925,
-42.6749499999997));
#238098=CARTESIAN_POINT('Ctrl Pts',(-44.5079524583208,29.5404524382925,
-42.5162000000004));
#238099=CARTESIAN_POINT('Ctrl Pts',(-44.7332666959702,29.5404524382925,
-42.52934333053));
#238100=CARTESIAN_POINT('Ctrl Pts',(-44.957288796902,29.5785306087671,-42.5424112864178));
#238101=CARTESIAN_POINT('Ctrl Pts',(-45.4116046387501,29.7380281571039,
-42.568913043859));
#238102=CARTESIAN_POINT('Ctrl Pts',(-45.6342607733475,29.868103521915,-42.5812333548637));
#238103=CARTESIAN_POINT('Ctrl Pts',(-46.0212859603873,30.2074222321539,
-42.6096633424967));
#238104=CARTESIAN_POINT('Ctrl Pts',(-46.1810715288083,30.4144868042626,
-42.6247842737231));
#238105=CARTESIAN_POINT('Ctrl Pts',(-46.4154506575917,30.8833823440739,
-42.6553080661824));
#238106=CARTESIAN_POINT('Ctrl Pts',(-46.4856784980985,31.141787512218,-42.6704105288686));
#238107=CARTESIAN_POINT('Ctrl Pts',(-46.5204267239946,31.6590362307413,
-42.6975544663922));
#238108=CARTESIAN_POINT('Ctrl Pts',(-46.4892761910751,31.9126254579149,
-42.7105462163547));
#238109=CARTESIAN_POINT('Ctrl Pts',(-46.3312342187149,32.4032106010717,
-42.7399392270222));
#238110=CARTESIAN_POINT('Ctrl Pts',(-46.2025900374275,32.6344856994316,
-42.7553749387522));
#238111=CARTESIAN_POINT('Ctrl Pts',(-45.8612144213161,33.0368477454997,
-42.7856583131711));
#238112=CARTESIAN_POINT('Ctrl Pts',(-45.65085238483,33.2030525098178,-42.7995308376202));
#238113=CARTESIAN_POINT('Ctrl Pts',(-45.1864669965252,33.4391089222736,
-42.8266199852712));
#238114=CARTESIAN_POINT('Ctrl Pts',(-44.9386576993136,33.5101553199242,
-42.8410755276084));
#238115=CARTESIAN_POINT('Ctrl Pts',(-44.4198486332464,33.5560631483164,
-42.8713393897956));
#238116=CARTESIAN_POINT('Ctrl Pts',(-44.1534101472401,33.5265964113438,
-42.8868816348126));
#238117=CARTESIAN_POINT('Ctrl Pts',(-43.6557736215184,33.3679547677738,
-42.9159104321463));
#238118=CARTESIAN_POINT('Ctrl Pts',(-43.4284127082079,33.2435566432759,
-42.9283155714807));
#238119=CARTESIAN_POINT('Ctrl Pts',(-43.031883069797,32.9145002366682,-42.9565043396993));
#238120=CARTESIAN_POINT('Ctrl Pts',(-42.8668882421245,32.7124893320118,
-42.9715219057308));
#238121=CARTESIAN_POINT('Ctrl Pts',(-42.6197045856503,32.2509675743979,
-43.0020466537567));
#238122=CARTESIAN_POINT('Ctrl Pts',(-42.5422220334332,31.9946053198465,
-43.0172575079889));
#238123=CARTESIAN_POINT('Ctrl Pts',(-42.492926353371,31.4783695051474,-43.0447745762333));
#238124=CARTESIAN_POINT('Ctrl Pts',(-42.5169722905291,31.2238968880538,
-43.0574548787517));
#238125=CARTESIAN_POINT('Ctrl Pts',(-42.6610668231682,30.7296881573348,
-43.086624146029));
#238126=CARTESIAN_POINT('Ctrl Pts',(-42.7827215470223,30.4955141344456,
-43.102002446884));
#238127=CARTESIAN_POINT('Ctrl Pts',(-43.1115986924766,30.0842462329312,
-43.1323711899042));
#238128=CARTESIAN_POINT('Ctrl Pts',(-43.3167336698099,29.9121869880077,
-43.146712237337));
#238129=CARTESIAN_POINT('Ctrl Pts',(-43.7729361058758,29.6630475933886,
-43.1733240461077));
#238130=CARTESIAN_POINT('Ctrl Pts',(-44.0177595996246,29.5848033418876,
-43.1876054165764));
#238131=CARTESIAN_POINT('Ctrl Pts',(-44.3495422509698,29.5451520527569,
-43.2069594045716));
#238132=CARTESIAN_POINT('Ctrl Pts',(-44.4287923051265,29.5404524382925,
-43.2115823243974));
#238133=CARTESIAN_POINT('Ctrl Pts',(-44.5079524583208,29.5404524382925,
-43.2162000000004));
#238134=CARTESIAN_POINT('Origin',(-44.5079524583208,31.5404524382925,235.35105));
#238135=CARTESIAN_POINT('',(-44.5079524583208,29.5404524382925,-41.8162000000004));
#238136=CARTESIAN_POINT('',(-44.5079524583208,29.5404524382925,-41.9749499999997));
#238137=CARTESIAN_POINT('',(-44.5079524583208,29.5404524382925,235.35105));
#238138=CARTESIAN_POINT('Ctrl Pts',(-44.5079524583208,29.5404524382925,
-42.6749499999997));
#238139=CARTESIAN_POINT('Ctrl Pts',(-44.2841370889279,29.5404524382925,
-42.6618941034518));
#238140=CARTESIAN_POINT('Ctrl Pts',(-44.0616277856587,29.5780252361848,
-42.6489143940944));
#238141=CARTESIAN_POINT('Ctrl Pts',(-43.608121189646,29.7360690715554,-42.6224598426604));
#238142=CARTESIAN_POINT('Ctrl Pts',(-43.3848953730774,29.8658662543444,
-42.6101244952876));
#238143=CARTESIAN_POINT('Ctrl Pts',(-42.9918289387129,30.2092396644597,
-42.581313468677));
#238144=CARTESIAN_POINT('Ctrl Pts',(-42.8284287235735,30.4224474775894,
-42.5657767650923));
#238145=CARTESIAN_POINT('Ctrl Pts',(-42.5990408165836,30.8911903670437,
-42.5354062615487));
#238146=CARTESIAN_POINT('Ctrl Pts',(-42.5316937175442,31.1405451574942,
-42.5208450288135));
#238147=CARTESIAN_POINT('Ctrl Pts',(-42.4941235311099,31.6588290422461,
-42.4935664894262));
#238148=CARTESIAN_POINT('Ctrl Pts',(-42.5272417851303,31.9230050659609,
-42.4800615441608));
#238149=CARTESIAN_POINT('Ctrl Pts',(-42.6937873095637,32.4223833588244,
-42.4499762995813));
#238150=CARTESIAN_POINT('Ctrl Pts',(-42.8251719183327,32.6527680759523,
-42.4345056391277));
#238151=CARTESIAN_POINT('Ctrl Pts',(-43.1633820494583,33.0425645094426,
-42.404949382837));
#238152=CARTESIAN_POINT('Ctrl Pts',(-43.3642611890508,33.2006096207479,
-42.3916653240412));
#238153=CARTESIAN_POINT('Ctrl Pts',(-43.8247840964883,33.4387675987847,
-42.364801487774));
#238154=CARTESIAN_POINT('Ctrl Pts',(-44.082177298587,33.5125042425652,-42.3497868843181));
#238155=CARTESIAN_POINT('Ctrl Pts',(-44.6051606547095,33.5548870328411,
-42.3192795218776));
#238156=CARTESIAN_POINT('Ctrl Pts',(-44.8655627452052,33.5252772867362,
-42.3040893999319));
#238157=CARTESIAN_POINT('Ctrl Pts',(-45.3559248803719,33.3696272638332,
-42.2754849420471));
#238158=CARTESIAN_POINT('Ctrl Pts',(-45.5817988901373,33.2468485025364,
-42.2631667822709));
#238159=CARTESIAN_POINT('Ctrl Pts',(-45.9846177047329,32.9154576062036,
-42.234676645648));
#238160=CARTESIAN_POINT('Ctrl Pts',(-46.1546451592276,32.7064518049151,
-42.2191589254403));
#238161=CARTESIAN_POINT('Ctrl Pts',(-46.3979573784054,32.2431084125083,
-42.1886550687183));
#238162=CARTESIAN_POINT('Ctrl Pts',(-46.4724437982236,31.995044233128,-42.1739508050754));
#238163=CARTESIAN_POINT('Ctrl Pts',(-46.5240393417302,31.4795852093357,
-42.1464058995188));
#238164=CARTESIAN_POINT('Ctrl Pts',(-46.498851379292,31.2169451438094,-42.1333415623));
#238165=CARTESIAN_POINT('Ctrl Pts',(-46.3482309719834,30.7141407460003,
-42.1035477198246));
#238166=CARTESIAN_POINT('Ctrl Pts',(-46.2234947946519,30.4791681395843,
-42.088039200282));
#238167=CARTESIAN_POINT('Ctrl Pts',(-45.8962379917397,30.0785749281764,
-42.0582569828334));
#238168=CARTESIAN_POINT('Ctrl Pts',(-45.6997631742947,29.9144391357236,
-42.0444722917645));
#238169=CARTESIAN_POINT('Ctrl Pts',(-45.2460901769229,29.6628345948263,
-42.0180080335845));
#238170=CARTESIAN_POINT('Ctrl Pts',(-44.9910006366204,29.5816493308882,
-42.0031278104002));
#238171=CARTESIAN_POINT('Ctrl Pts',(-44.654499455299,29.5444745450108,-41.9834985748232));
#238172=CARTESIAN_POINT('Ctrl Pts',(-44.5811846202044,29.5404524382925,
-41.9792218761095));
#238173=CARTESIAN_POINT('Ctrl Pts',(-44.5079524583208,29.5404524382925,
-41.9749499999997));
#238174=CARTESIAN_POINT('Ctrl Pts',(-44.5079524583208,29.5404524382925,
-41.8162000000004));
#238175=CARTESIAN_POINT('Ctrl Pts',(-44.7729039134369,29.5404524382925,
-41.8316555015489));
#238176=CARTESIAN_POINT('Ctrl Pts',(-45.0352945948459,29.5931024916833,
-41.8469616246312));
#238177=CARTESIAN_POINT('Ctrl Pts',(-45.5139921448838,29.7933651489333,
-41.8748856483834));
#238178=CARTESIAN_POINT('Ctrl Pts',(-45.7273470393406,29.9349870020374,
-41.8873272005398));
#238179=CARTESIAN_POINT('Ctrl Pts',(-46.0945687985833,30.2952428951762,
-41.9162372959115));
#238180=CARTESIAN_POINT('Ctrl Pts',(-46.2431257236584,30.5123186077162,
-41.9315364693197));
#238181=CARTESIAN_POINT('Ctrl Pts',(-46.4503845331156,30.995297046345,-41.9619806944399));
#238182=CARTESIAN_POINT('Ctrl Pts',(-46.5054721111779,31.257249210245,-41.9768207537966));
#238183=CARTESIAN_POINT('Ctrl Pts',(-46.5101666263359,31.7761404805287,
-42.0031711034309));
#238184=CARTESIAN_POINT('Ctrl Pts',(-46.4641359997729,32.0281591361894,
-42.0171160194564));
#238185=CARTESIAN_POINT('Ctrl Pts',(-46.2766215298312,32.5106781500049,
-42.0469611587164));
#238186=CARTESIAN_POINT('Ctrl Pts',(-46.1334378488472,32.7351629111486,
-42.0624779039232));
#238187=CARTESIAN_POINT('Ctrl Pts',(-45.7702384727176,33.1135542276122,
-42.0921868477969));
#238188=CARTESIAN_POINT('Ctrl Pts',(-45.5546304034682,33.2645347610461,
-42.1051437865329));
#238189=CARTESIAN_POINT('Ctrl Pts',(-45.0811435304602,33.4736969370716,
-42.1327638541249));
#238190=CARTESIAN_POINT('Ctrl Pts',(-44.8284007905841,33.531246333344,-42.1475071806176));
#238191=CARTESIAN_POINT('Ctrl Pts',(-44.3048968527452,33.5479484634135,
-42.1780449103248));
#238192=CARTESIAN_POINT('Ctrl Pts',(-44.0390134197966,33.5029502399948,
-42.1935547772468));
#238193=CARTESIAN_POINT('Ctrl Pts',(-43.5522189874468,33.3156629807161,
-42.2219511191338));
#238194=CARTESIAN_POINT('Ctrl Pts',(-43.3343039869024,33.1797674883365,
-42.2342829191908));
#238195=CARTESIAN_POINT('Ctrl Pts',(-42.9571892165043,32.8298928830521,
-42.2629571172791));
#238196=CARTESIAN_POINT('Ctrl Pts',(-42.8029645057999,32.6177277261712,
-42.2781735289213));
#238197=CARTESIAN_POINT('Ctrl Pts',(-42.5820944686412,32.141564881733,-42.3086704369831));
#238198=CARTESIAN_POINT('Ctrl Pts',(-42.5194454807074,31.8812647971072,
-42.323647577475));
#238199=CARTESIAN_POINT('Ctrl Pts',(-42.4997839987105,31.3631178499939,
-42.3503968618138));
#238200=CARTESIAN_POINT('Ctrl Pts',(-42.5383649321693,31.1103595086761,
-42.3638145289975));
#238201=CARTESIAN_POINT('Ctrl Pts',(-42.7110890663376,30.6237209358429,
-42.3934363959587));
#238202=CARTESIAN_POINT('Ctrl Pts',(-42.8470193569132,30.3957173869416,
-42.4089193465882));
#238203=CARTESIAN_POINT('Ctrl Pts',(-43.1993815561311,30.0052535364079,
-42.4389220882051));
#238204=CARTESIAN_POINT('Ctrl Pts',(-43.412362825029,29.8466870834928,-42.4522906047249));
#238205=CARTESIAN_POINT('Ctrl Pts',(-43.8813116004633,29.6239590185105,
-42.4796459499587));
#238206=CARTESIAN_POINT('Ctrl Pts',(-44.1316518199665,29.559547318394,-42.4942491294297));
#238207=CARTESIAN_POINT('Ctrl Pts',(-44.4275126620251,29.5416644091701,
-42.5115076785499));
#238208=CARTESIAN_POINT('Ctrl Pts',(-44.4677531256547,29.5404524382925,
-42.5138550389283));
#238209=CARTESIAN_POINT('Ctrl Pts',(-44.5079524583208,29.5404524382925,
-42.5162000000005));
#238210=CARTESIAN_POINT('Origin',(-44.5079524583208,31.5404524382925,235.35105));
#238211=CARTESIAN_POINT('',(-44.5079524583208,29.5404524382925,-41.1162000000004));
#238212=CARTESIAN_POINT('',(-44.5079524583208,29.5404524382925,-41.2749499999996));
#238213=CARTESIAN_POINT('',(-44.5079524583208,29.5404524382925,235.35105));
#238214=CARTESIAN_POINT('Ctrl Pts',(-44.5079524583208,29.5404524382925,
-41.9749499999997));
#238215=CARTESIAN_POINT('Ctrl Pts',(-44.3218286908714,29.5404524382925,
-41.9640927802318));
#238216=CARTESIAN_POINT('Ctrl Pts',(-44.1362389523276,29.5664357012366,
-41.95326671215));
#238217=CARTESIAN_POINT('Ctrl Pts',(-43.7124429497979,29.6879690440001,
-41.9285452786692));
#238218=CARTESIAN_POINT('Ctrl Pts',(-43.4838809667533,29.8038473029044,
-41.9161446577051));
#238219=CARTESIAN_POINT('Ctrl Pts',(-43.0715512709672,30.123288631754,-41.8879807904063));
#238220=CARTESIAN_POINT('Ctrl Pts',(-42.8950699812305,30.3279432472202,
-41.8724946471893));
#238221=CARTESIAN_POINT('Ctrl Pts',(-42.6381064955435,30.7855503339349,
-41.8418824160708));
#238222=CARTESIAN_POINT('Ctrl Pts',(-42.5565808648473,31.0321393902305,
-41.8270473625978));
#238223=CARTESIAN_POINT('Ctrl Pts',(-42.4912079870856,31.5447228561652,
-41.7992458859848));
#238224=CARTESIAN_POINT('Ctrl Pts',(-42.5087479068552,31.805916250814,-41.7865160591014));
#238225=CARTESIAN_POINT('Ctrl Pts',(-42.6438718891428,32.3118355648619,
-41.7570168358879));
#238226=CARTESIAN_POINT('Ctrl Pts',(-42.7619824534228,32.5510986273815,
-41.7414848174939));
#238227=CARTESIAN_POINT('Ctrl Pts',(-43.078308585955,32.9620016550282,-41.7115005784364));
#238228=CARTESIAN_POINT('Ctrl Pts',(-43.2705076063607,33.1321374223604,
-41.6972998297061));
#238229=CARTESIAN_POINT('Ctrl Pts',(-43.7175229558531,33.3966417541728,
-41.6708996128849));
#238230=CARTESIAN_POINT('Ctrl Pts',(-43.9702286576964,33.484977612375,-41.6563172217035));
#238231=CARTESIAN_POINT('Ctrl Pts',(-44.4914644076179,33.5573495307964,
-41.6259118029579));
#238232=CARTESIAN_POINT('Ctrl Pts',(-44.7545856011578,33.5422834627067,
-41.610563066668));
#238233=CARTESIAN_POINT('Ctrl Pts',(-45.2528831641334,33.4137804886457,
-41.5814957088276));
#238234=CARTESIAN_POINT('Ctrl Pts',(-45.484057791781,33.304390870872,-41.568924498218));
#238235=CARTESIAN_POINT('Ctrl Pts',(-45.9027600729807,32.9981455705253,
-41.5412414027726));
#238236=CARTESIAN_POINT('Ctrl Pts',(-46.0835487375013,32.8005384566929,
-41.5259856545255));
#238237=CARTESIAN_POINT('Ctrl Pts',(-46.3538105203188,32.3524911214934,
-41.4954684973543));
#238238=CARTESIAN_POINT('Ctrl Pts',(-46.4430967263761,32.1077647451806,
-41.4805011929106));
#238239=CARTESIAN_POINT('Ctrl Pts',(-46.5236276705724,31.5984606951186,
-41.4524232760445));
#238240=CARTESIAN_POINT('Ctrl Pts',(-46.5143530940854,31.3387749910143,
-41.4399483139675));
#238241=CARTESIAN_POINT('Ctrl Pts',(-46.3961025789716,30.8296979833545,
-41.4107817127116));
#238242=CARTESIAN_POINT('Ctrl Pts',(-46.2853724928991,30.5859662992026,
-41.3952392117738));
#238243=CARTESIAN_POINT('Ctrl Pts',(-45.9811932080273,30.1639937114167,
-41.3650500420895));
#238244=CARTESIAN_POINT('Ctrl Pts',(-45.7937701872473,29.9874575277945,
-41.3506652561674));
#238245=CARTESIAN_POINT('Ctrl Pts',(-45.3529256117621,29.7082055742254,
-41.323699997708));
#238246=CARTESIAN_POINT('Ctrl Pts',(-45.1013335290938,29.6119614386068,
-41.3095638957945));
#238247=CARTESIAN_POINT('Ctrl Pts',(-44.7288150439468,29.5495931329844,
-41.2878336508276));
#238248=CARTESIAN_POINT('Ctrl Pts',(-44.6183508181325,29.5404524382925,
-41.281389904322));
#238249=CARTESIAN_POINT('Ctrl Pts',(-44.5079524583208,29.5404524382925,
-41.2749499999996));
#238250=CARTESIAN_POINT('Ctrl Pts',(-44.5079524583208,29.5404524382925,
-41.1162000000005));
#238251=CARTESIAN_POINT('Ctrl Pts',(-44.5442641855471,29.5404524382925,
-41.1183181840887));
#238252=CARTESIAN_POINT('Ctrl Pts',(-44.5806096277852,29.5414413320196,
-41.120438334886));
#238253=CARTESIAN_POINT('Ctrl Pts',(-44.8816866451562,29.5578738957329,
-41.1380011608993));
#238254=CARTESIAN_POINT('Ctrl Pts',(-45.1409681939803,29.6248249502642,
-41.1531259179141));
#238255=CARTESIAN_POINT('Ctrl Pts',(-45.6075611689831,29.8507843113607,
-41.1803438414559));
#238256=CARTESIAN_POINT('Ctrl Pts',(-45.8124464798734,30.0034257864677,
-41.1932666682341));
#238257=CARTESIAN_POINT('Ctrl Pts',(-46.1602937634056,30.3835599514533,
-41.222615888221));
#238258=CARTESIAN_POINT('Ctrl Pts',(-46.2974616923732,30.6097080927158,
-41.2380412048781));
#238259=CARTESIAN_POINT('Ctrl Pts',(-46.4782029531163,31.1058311080966,
-41.2683760411751));
#238260=CARTESIAN_POINT('Ctrl Pts',(-46.5184608384878,31.3714076229008,
-41.2823536744827));
#238261=CARTESIAN_POINT('Ctrl Pts',(-46.4932878027219,31.8921020041553,
-41.3093924041292));
#238262=CARTESIAN_POINT('Ctrl Pts',(-46.4322193782992,32.1424225938883,
-41.3238192992464));
#238263=CARTESIAN_POINT('Ctrl Pts',(-46.2151423082367,32.6155695235688,
-41.3540532206713));
#238264=CARTESIAN_POINT('Ctrl Pts',(-46.0576377189352,32.8322991372114,
-41.3695958833439));
#238265=CARTESIAN_POINT('Ctrl Pts',(-45.6732486620862,33.1861119639656,
-41.3986811997775));
#238266=CARTESIAN_POINT('Ctrl Pts',(-45.4523092165156,33.3221079656183,
-41.4111125224385));
#238267=CARTESIAN_POINT('Ctrl Pts',(-44.969848357842,33.5034537564664,-41.4392560725276));
#238268=CARTESIAN_POINT('Ctrl Pts',(-44.7127523988259,33.546630964103,-41.4542533368035));
#238269=CARTESIAN_POINT('Ctrl Pts',(-44.1895139304819,33.5326653521654,
-41.4847755807901));
#238270=CARTESIAN_POINT('Ctrl Pts',(-43.9284362195246,33.4729416759115,
-41.5000051139293));
#238271=CARTESIAN_POINT('Ctrl Pts',(-43.4555470252595,33.2599451113419,
-41.5275903169281));
#238272=CARTESIAN_POINT('Ctrl Pts',(-43.2463873872433,33.1129308446866,
-41.5402236168403));
#238273=CARTESIAN_POINT('Ctrl Pts',(-42.8885957004252,32.7429245610463,
-41.5693512401087));
#238274=CARTESIAN_POINT('Ctrl Pts',(-42.7455383109935,32.5213415806022,
-41.5847177092236));
#238275=CARTESIAN_POINT('Ctrl Pts',(-42.5512562589388,32.0320557203347,
-41.6151020848497));
#238276=CARTESIAN_POINT('Ctrl Pts',(-42.5034158782804,31.7686412814615,
-41.6295400052042));
#238277=CARTESIAN_POINT('Ctrl Pts',(-42.5129743893263,31.2490902760617,
-41.656065549982));
#238278=CARTESIAN_POINT('Ctrl Pts',(-42.5662271284927,30.9977868310396,
-41.6703141396422));
#238279=CARTESIAN_POINT('Ctrl Pts',(-42.7678951447684,30.5196043976839,
-41.7003530146546));
#238280=CARTESIAN_POINT('Ctrl Pts',(-42.9179735214712,30.2987157867033,
-41.7158891843053));
#238281=CARTESIAN_POINT('Ctrl Pts',(-43.2914015115809,29.9320275058476,
-41.7453052470623));
#238282=CARTESIAN_POINT('Ctrl Pts',(-43.5095446989283,29.7882544431415,
-41.757959547369));
#238283=CARTESIAN_POINT('Ctrl Pts',(-43.9873475189462,29.592298804994,-41.7858313785369));
#238284=CARTESIAN_POINT('Ctrl Pts',(-44.2422550479135,29.5415262495077,
-41.8007009843933));
#238285=CARTESIAN_POINT('Ctrl Pts',(-44.5024795660782,29.5404580538342,
-41.815880747953));
#238286=CARTESIAN_POINT('Ctrl Pts',(-44.5052161487644,29.5404524382925,
-41.816040381943));
#238287=CARTESIAN_POINT('Ctrl Pts',(-44.5079524583208,29.5404524382925,
-41.8162000000004));
#238288=CARTESIAN_POINT('Origin',(-44.5079524583208,31.5404524382925,235.35105));
#238289=CARTESIAN_POINT('',(-44.5079524583208,29.5404524382925,-40.4162000000004));
#238290=CARTESIAN_POINT('',(-44.5079524583208,29.5404524382925,-40.5749499999997));
#238291=CARTESIAN_POINT('',(-44.5079524583208,29.5404524382925,235.35105));
#238292=CARTESIAN_POINT('Ctrl Pts',(-44.5079524583208,29.5404524382925,
-41.2749499999996));
#238293=CARTESIAN_POINT('Ctrl Pts',(-44.3578015660496,29.5404524382925,
-41.2661911979505));
#238294=CARTESIAN_POINT('Ctrl Pts',(-44.2077725143422,29.557361800295,-41.2574395032674));
#238295=CARTESIAN_POINT('Ctrl Pts',(-43.8138468828723,29.6477343665768,
-41.2344605080985));
#238296=CARTESIAN_POINT('Ctrl Pts',(-43.5800166448313,29.7507411266094,
-41.2216314406855));
#238297=CARTESIAN_POINT('Ctrl Pts',(-43.1533656622638,30.0453145822135,
-41.1943061481038));
#238298=CARTESIAN_POINT('Ctrl Pts',(-42.9672845218358,30.2378997606675,
-41.1791497348536));
#238299=CARTESIAN_POINT('Ctrl Pts',(-42.684558257388,30.6789517759641,-41.1486224209118));
#238300=CARTESIAN_POINT('Ctrl Pts',(-42.5884992636513,30.9218467048739,
-41.1335500981595));
#238301=CARTESIAN_POINT('Ctrl Pts',(-42.4947427452761,31.4281892360414,
-41.1052360458316));
#238302=CARTESIAN_POINT('Ctrl Pts',(-42.4969211982232,31.6866403428544,
-41.092886602807));
#238303=CARTESIAN_POINT('Ctrl Pts',(-42.6006050062832,32.1982560191603,
-41.0640166150004));
#238304=CARTESIAN_POINT('Ctrl Pts',(-42.7048326024362,32.4456688198682,
-41.0484778068256));
#238305=CARTESIAN_POINT('Ctrl Pts',(-42.9982222886613,32.8769152557054,
-41.018134836135));
#238306=CARTESIAN_POINT('Ctrl Pts',(-43.1813530602796,33.0588701330176,
-41.0036014984407));
#238307=CARTESIAN_POINT('Ctrl Pts',(-43.6131789265666,33.348530028927,-40.9763734956889));
#238308=CARTESIAN_POINT('Ctrl Pts',(-43.8595281088582,33.4507810501543,
-40.962774753719));
#238309=CARTESIAN_POINT('Ctrl Pts',(-44.3761941666342,33.5533008432308,
-40.9326359003487));
#238310=CARTESIAN_POINT('Ctrl Pts',(-44.6412566326515,33.5531990720144,
-40.9171739231643));
#238311=CARTESIAN_POINT('Ctrl Pts',(-45.1471919732393,33.4524045635475,
-40.8876610282965));
#238312=CARTESIAN_POINT('Ctrl Pts',(-45.3839316726719,33.3561602304872,
-40.8744601355583));
#238313=CARTESIAN_POINT('Ctrl Pts',(-45.8188676392155,33.0740185112342,
-40.8475212259141));
#238314=CARTESIAN_POINT('Ctrl Pts',(-46.0103951893242,32.886908350919,-40.8324825468278));
#238315=CARTESIAN_POINT('Ctrl Pts',(-46.3061199456251,32.4536433767286,
-40.8019694971061));
#238316=CARTESIAN_POINT('Ctrl Pts',(-46.4093131594905,32.2128890246153,
-40.7867972309098));
#238317=CARTESIAN_POINT('Ctrl Pts',(-46.5170230053301,31.7097685641752,
-40.7582389795783));
#238318=CARTESIAN_POINT('Ctrl Pts',(-46.5222267679748,31.4525418257785,
-40.7459252526485));
#238319=CARTESIAN_POINT('Ctrl Pts',(-46.4337482063667,30.9384475986097,
-40.7173735393959));
#238320=CARTESIAN_POINT('Ctrl Pts',(-46.3364290625623,30.6873725516868,
-40.7018512178498));
#238321=CARTESIAN_POINT('Ctrl Pts',(-46.0545875790311,30.2467385831459,
-40.6713708289661));
#238322=CARTESIAN_POINT('Ctrl Pts',(-45.8760988962231,30.0592408825443,
-40.6566928723583));
#238323=CARTESIAN_POINT('Ctrl Pts',(-45.4536997868605,29.7588549154494,
-40.629197955426));
#238324=CARTESIAN_POINT('Ctrl Pts',(-45.2126607854844,29.6504945112309,
-40.6160579857508));
#238325=CARTESIAN_POINT('Ctrl Pts',(-44.8097429655949,29.5575438432581,
-40.5925544462573));
#238326=CARTESIAN_POINT('Ctrl Pts',(-44.6589093996137,29.5404524382925,
-40.583755821575));
#238327=CARTESIAN_POINT('Ctrl Pts',(-44.5079524583208,29.5404524382925,
-40.5749499999997));
#238328=CARTESIAN_POINT('Ctrl Pts',(-44.5079524583208,29.5404524382925,
-40.4162000000005));
#238329=CARTESIAN_POINT('Ctrl Pts',(-44.5829923762501,29.5404524382925,
-40.4205773285463));
#238330=CARTESIAN_POINT('Ctrl Pts',(-44.6581163348707,29.5446755687294,
-40.424959559466));
#238331=CARTESIAN_POINT('Ctrl Pts',(-44.9963174757759,29.5829688449569,
-40.4446879593522));
#238332=CARTESIAN_POINT('Ctrl Pts',(-45.2511810225848,29.6648445373245,
-40.4595549995827));
#238333=CARTESIAN_POINT('Ctrl Pts',(-45.7042087706374,29.9176993849155,
-40.4859816182191));
#238334=CARTESIAN_POINT('Ctrl Pts',(-45.900274393063,30.0824091221457,-40.4998184075873));
#238335=CARTESIAN_POINT('Ctrl Pts',(-46.2264944584649,30.4840139191428,
-40.5296214902895));
#238336=CARTESIAN_POINT('Ctrl Pts',(-46.3505978161064,30.7194081747423,
-40.5451328535272));
#238337=CARTESIAN_POINT('Ctrl Pts',(-46.4997227128501,31.2225224340371,
-40.5748987305729));
#238338=CARTESIAN_POINT('Ctrl Pts',(-46.5241698272145,31.4850206280497,
-40.5879266809833));
#238339=CARTESIAN_POINT('Ctrl Pts',(-46.47125040528,32.000207668004,-40.6154964595404));
#238340=CARTESIAN_POINT('Ctrl Pts',(-46.3960885197321,32.2481390631782,
-40.6302137162548));
#238341=CARTESIAN_POINT('Ctrl Pts',(-46.1514629950418,32.7109498599051,
-40.660728971973));
#238342=CARTESIAN_POINT('Ctrl Pts',(-45.9808127663973,32.9195471375113,
-40.6762442185664));
#238343=CARTESIAN_POINT('Ctrl Pts',(-45.5770770869542,33.2497974648976,
-40.704703477649));
#238344=CARTESIAN_POINT('Ctrl Pts',(-45.3509487745718,33.3719135158588,
-40.7170252148852));
#238345=CARTESIAN_POINT('Ctrl Pts',(-44.8601916059309,33.5262465147202,
-40.7456527163891));
#238346=CARTESIAN_POINT('Ctrl Pts',(-44.5996390813612,33.5551548713799,
-40.7608516136556));
#238347=CARTESIAN_POINT('Ctrl Pts',(-44.0767106440532,33.5113154004804,
-40.7913557724985));
#238348=CARTESIAN_POINT('Ctrl Pts',(-43.8195270625652,33.4368669124925,
-40.8063581480853));
#238349=CARTESIAN_POINT('Ctrl Pts',(-43.3596501657047,33.1974268160417,
-40.8331843004021));
#238350=CARTESIAN_POINT('Ctrl Pts',(-43.1591913872011,33.0388072324325,
-40.8465114211634));
#238351=CARTESIAN_POINT('Ctrl Pts',(-42.8220104306781,32.6479878959408,
-40.8760893350274));
#238352=CARTESIAN_POINT('Ctrl Pts',(-42.6912473505325,32.4171617775238,
-40.8915641663387));
#238353=CARTESIAN_POINT('Ctrl Pts',(-42.526207751472,31.9174494400805,-40.9216223634086));
#238354=CARTESIAN_POINT('Ctrl Pts',(-42.4938428204949,31.6534204444785,
-40.9350815343781));
#238355=CARTESIAN_POINT('Ctrl Pts',(-42.5327337940736,31.1353981648866,
-40.9623853809157));
#238356=CARTESIAN_POINT('Ctrl Pts',(-42.6007517442998,30.8861559029383,
-40.9769604954124));
#238357=CARTESIAN_POINT('Ctrl Pts',(-42.8314514208811,30.4179025768849,
-41.007344527066));
#238358=CARTESIAN_POINT('Ctrl Pts',(-42.9954778454,30.2050806326366,-41.0228800017097));
#238359=CARTESIAN_POINT('Ctrl Pts',(-43.3894653112581,29.8628281077271,
-41.0516612666937));
#238360=CARTESIAN_POINT('Ctrl Pts',(-43.6129381130091,29.7336912042102,
-41.0639908298572));
#238361=CARTESIAN_POINT('Ctrl Pts',(-44.0650998168327,29.5774371450193,
-41.090366929247));
#238362=CARTESIAN_POINT('Ctrl Pts',(-44.2858957213049,29.5404524382925,
-41.1032466903412));
#238363=CARTESIAN_POINT('Ctrl Pts',(-44.5079524583208,29.5404524382925,
-41.1162000000004));
#238364=CARTESIAN_POINT('Origin',(-44.5079524583208,31.5404524382925,235.35105));
#238365=CARTESIAN_POINT('',(-44.5079524583208,29.5404524382925,-39.7162000000004));
#238366=CARTESIAN_POINT('',(-44.5079524583208,29.5404524382925,-39.8749499999996));
#238367=CARTESIAN_POINT('',(-44.5079524583208,29.5404524382925,235.35105));
#238368=CARTESIAN_POINT('',(-43.0434008745115,32.9024688233232,-39.4567761906824));
#238369=CARTESIAN_POINT('Ctrl Pts',(-44.5079524583208,29.5404524382925,
-39.7162000000005));
#238370=CARTESIAN_POINT('Ctrl Pts',(-44.2727838454877,29.5404524382925,
-39.7024818309185));
#238371=CARTESIAN_POINT('Ctrl Pts',(-44.0391728207237,29.5819339445239,
-39.6888545211407));
#238372=CARTESIAN_POINT('Ctrl Pts',(-43.5769885436395,29.7518172548108,
-39.661893771644));
#238373=CARTESIAN_POINT('Ctrl Pts',(-43.3553604175783,29.8859300422344,
-39.6494994736688));
#238374=CARTESIAN_POINT('Ctrl Pts',(-42.9683294219119,30.2365875679526,
-39.6204965006525));
#238375=CARTESIAN_POINT('Ctrl Pts',(-42.8090308900948,30.4522665828854,
-39.6049545889581));
#238376=CARTESIAN_POINT('Ctrl Pts',(-42.5882152549613,30.9241122679227,
-39.5746773625219));
#238377=CARTESIAN_POINT('Ctrl Pts',(-42.5252433861803,31.1741567088814,
-39.5602089008022));
#238378=CARTESIAN_POINT('Ctrl Pts',(-42.4963483862349,31.6933438391783,
-39.5331377573946));
#238379=CARTESIAN_POINT('Ctrl Pts',(-42.5341552917939,31.9577132499568,
-39.5193565070205));
#238380=CARTESIAN_POINT('Ctrl Pts',(-42.6679048358913,32.3360106662249,
-39.4963445935783));
#238381=CARTESIAN_POINT('Ctrl Pts',(-42.7265667691374,32.4598822126121,
-39.4883758593432));
#238382=CARTESIAN_POINT('Ctrl Pts',(-42.8680765464176,32.6934533978673,
-39.4724489070045));
#238383=CARTESIAN_POINT('Ctrl Pts',(-42.9505054915165,32.802580106633,-39.4645318501545));
#238384=CARTESIAN_POINT('Ctrl Pts',(-43.0434008641317,32.9024688214384,
-39.4567762088531));
#238385=CARTESIAN_POINT('',(-43.3993761328101,33.2051021117905,-39.5898551227246));
#238386=CARTESIAN_POINT('Ctrl Pts',(-43.3993761338312,33.2051021109807,
-39.5898551212222));
#238387=CARTESIAN_POINT('Ctrl Pts',(-43.3343112356562,33.1617720296696,
-39.5680449019351));
#238388=CARTESIAN_POINT('Ctrl Pts',(-43.2718932132572,33.1146982543088,
-39.5459701333695));
#238389=CARTESIAN_POINT('Ctrl Pts',(-43.1529636864307,33.0135776982464,
-39.5015049864959));
#238390=CARTESIAN_POINT('Ctrl Pts',(-43.0965305096728,32.959598167928,-39.4791495394364));
#238391=CARTESIAN_POINT('Ctrl Pts',(-43.043400874595,32.9024688326895,-39.4567761622585));
#238392=CARTESIAN_POINT('Ctrl Pts',(-44.5079524583208,29.5404524382925,
-39.8749499999996));
#238393=CARTESIAN_POINT('Ctrl Pts',(-44.4373589931104,29.5404524382925,
-39.8708320478624));
#238394=CARTESIAN_POINT('Ctrl Pts',(-44.3666819864989,29.5441899135023,
-39.8667092224767));
#238395=CARTESIAN_POINT('Ctrl Pts',(-44.0426740209612,29.5786855502815,
-39.8478087578204));
#238396=CARTESIAN_POINT('Ctrl Pts',(-43.7965720231925,29.6539224734034,
-39.8334528079507));
#238397=CARTESIAN_POINT('Ctrl Pts',(-43.3351658396914,29.8985180124527,
-39.8065374472466));
#238398=CARTESIAN_POINT('Ctrl Pts',(-43.1265097586977,30.06971477229,-39.7922901984896));
#238399=CARTESIAN_POINT('Ctrl Pts',(-42.792355887439,30.4797122390129,-39.7618317309806));
#238400=CARTESIAN_POINT('Ctrl Pts',(-42.6684583528071,30.712981114929,-39.7464337411607));
#238401=CARTESIAN_POINT('Ctrl Pts',(-42.5199012825829,31.2060434353122,
-39.7171922310651));
#238402=CARTESIAN_POINT('Ctrl Pts',(-42.4935765041893,31.4602232063242,
-39.7044223309215));
#238403=CARTESIAN_POINT('Ctrl Pts',(-42.5381946201159,31.9768008141531,
-39.6770244248751));
#238404=CARTESIAN_POINT('Ctrl Pts',(-42.613350918841,32.2338428608599,-39.6618470778621));
#238405=CARTESIAN_POINT('Ctrl Pts',(-42.8150006258135,32.6186840080726,
-39.6365241658308));
#238406=CARTESIAN_POINT('Ctrl Pts',(-42.912317892686,32.7580827818824,-39.6266435775835));
#238407=CARTESIAN_POINT('Ctrl Pts',(-43.1367390871144,33.0056999129204,
-39.6075888004023));
#238408=CARTESIAN_POINT('Ctrl Pts',(-43.2621306492484,33.1137032434628,
-39.5984754182101));
#238409=CARTESIAN_POINT('Ctrl Pts',(-43.3993761335977,33.2051021108252,
-39.5898551233574));
#238410=CARTESIAN_POINT('Origin',(44.5079524583205,-57.4754524783491,-52.920575));
#238411=CARTESIAN_POINT('',(42.839207175268,-57.4754524783491,-40.04995));
#238412=CARTESIAN_POINT('',(42.839207175268,-57.4754524783491,-39.8912));
#238413=CARTESIAN_POINT('',(42.839207175268,-57.4754524783491,-52.920575));
#238414=CARTESIAN_POINT('',(43.0534153750531,-58.2933966653875,-39.8341885847849));
#238415=CARTESIAN_POINT('Ctrl Pts',(42.839207175268,-57.4754524783491,-39.8912));
#238416=CARTESIAN_POINT('Ctrl Pts',(42.839207175268,-57.9124736451316,-39.8647399998442));
#238417=CARTESIAN_POINT('Ctrl Pts',(43.0534153750531,-58.2933966653875,
-39.8341885847849));
#238418=CARTESIAN_POINT('',(43.3633213057583,-58.68975488891,-39.9581073773015));
#238419=CARTESIAN_POINT('Ctrl Pts',(43.3633213057583,-58.68975488891,-39.9581073773016));
#238420=CARTESIAN_POINT('Ctrl Pts',(43.3039463283678,-58.6337865829816,
-39.9376450972415));
#238421=CARTESIAN_POINT('Ctrl Pts',(43.2487306042849,-58.5735157107134,
-39.9172507770231));
#238422=CARTESIAN_POINT('Ctrl Pts',(43.1444016679814,-58.4413495448207,
-39.875725104448));
#238423=CARTESIAN_POINT('Ctrl Pts',(43.0960118137051,-58.3691452318743,
-39.8546807358163));
#238424=CARTESIAN_POINT('Ctrl Pts',(43.0534153750531,-58.2933966653875,
-39.8341885847849));
#238425=CARTESIAN_POINT('Ctrl Pts',(42.839207175268,-57.4754524783491,-40.04995));
#238426=CARTESIAN_POINT('Ctrl Pts',(42.839207175268,-58.1957120903124,-40.0063409693778));
#238427=CARTESIAN_POINT('Ctrl Pts',(43.3633213057583,-58.68975488891,-39.9581073773015));
#238428=CARTESIAN_POINT('Origin',(44.5079524583205,-57.4754524783491,-52.920575));
#238429=CARTESIAN_POINT('',(42.839207175268,-57.4754524783491,-40.74995));
#238430=CARTESIAN_POINT('',(42.839207175268,-57.4754524783491,-40.5912));
#238431=CARTESIAN_POINT('',(42.839207175268,-57.4754524783491,-52.920575));
#238432=CARTESIAN_POINT('',(45.3466064770396,-58.918147961324,-40.3575668307237));
#238433=CARTESIAN_POINT('Ctrl Pts',(42.839207175268,-57.4754524783491,-40.5912));
#238434=CARTESIAN_POINT('Ctrl Pts',(42.839207175268,-58.4389030167283,-40.5328666666667));
#238435=CARTESIAN_POINT('Ctrl Pts',(43.6735798167943,-58.920628285918,-40.4745333333334));
#238436=CARTESIAN_POINT('Ctrl Pts',(44.5079524583205,-59.4023535551075,
-40.4162));
#238437=CARTESIAN_POINT('Ctrl Pts',(45.3423250998467,-58.920628285918,-40.3578666666667));
#238438=CARTESIAN_POINT('Ctrl Pts',(45.3444676270302,-58.9193912972719,
-40.3577168765775));
#238439=CARTESIAN_POINT('Ctrl Pts',(45.3466064770396,-58.918147961324,-40.3575668307237));
#238440=CARTESIAN_POINT('',(46.1762417771239,-57.4364451908711,-40.2388223154955));
#238441=CARTESIAN_POINT('Ctrl Pts',(46.1762417771238,-57.4364451908711,
-40.2388223154955));
#238442=CARTESIAN_POINT('Ctrl Pts',(46.179661059212,-57.5826832954551,-40.2660212994017));
#238443=CARTESIAN_POINT('Ctrl Pts',(46.1638510938788,-57.7293501220844,
-40.2898469846044));
#238444=CARTESIAN_POINT('Ctrl Pts',(46.0933221577362,-58.0171833460811,
-40.3294337826712));
#238445=CARTESIAN_POINT('Ctrl Pts',(46.0386075282205,-58.15680126839,-40.3449195577534));
#238446=CARTESIAN_POINT('Ctrl Pts',(45.8931630193347,-58.417855944105,-40.36600443659));
#238447=CARTESIAN_POINT('Ctrl Pts',(45.8033935488223,-58.5379373447246,
-40.3715360596572));
#238448=CARTESIAN_POINT('Ctrl Pts',(45.6856994285344,-58.6578091204824,
-40.3719332463563));
#238449=CARTESIAN_POINT('Ctrl Pts',(45.6724768224328,-58.6708344909785,
-40.3718974824544));
#238450=CARTESIAN_POINT('Ctrl Pts',(45.5643373887037,-58.7738638224284,
-40.3709688119876));
#238451=CARTESIAN_POINT('Ctrl Pts',(45.4594840399648,-58.8525310498637,
-40.3661880411365));
#238452=CARTESIAN_POINT('Ctrl Pts',(45.3466064770396,-58.918147961324,-40.3575668307237));
#238453=CARTESIAN_POINT('Ctrl Pts',(46.1762417771239,-57.4364451908711,
-40.2388223154955));
#238454=CARTESIAN_POINT('Ctrl Pts',(46.1543247861016,-56.4990849082214,
-40.181302510566));
#238455=CARTESIAN_POINT('Ctrl Pts',(45.3423250998467,-56.0302766707802,
-40.1245333333334));
#238456=CARTESIAN_POINT('Ctrl Pts',(44.5079524583205,-55.5485514015906,
-40.0662));
#238457=CARTESIAN_POINT('Ctrl Pts',(43.6735798167943,-56.0302766707802,
-40.0078666666667));
#238458=CARTESIAN_POINT('Ctrl Pts',(42.839207175268,-56.5120019399698,-39.9495333333333));
#238459=CARTESIAN_POINT('Ctrl Pts',(42.839207175268,-57.4754524783491,-39.8912));
#238460=CARTESIAN_POINT('Ctrl Pts',(42.839207175268,-57.4754524783491,-40.74995));
#238461=CARTESIAN_POINT('Ctrl Pts',(42.839207175268,-58.4389030167283,-40.6916166666667));
#238462=CARTESIAN_POINT('Ctrl Pts',(43.6735798167943,-58.920628285918,-40.6332833333334));
#238463=CARTESIAN_POINT('Ctrl Pts',(44.5079524583205,-59.4023535551075,
-40.57495));
#238464=CARTESIAN_POINT('Ctrl Pts',(45.3423250998467,-58.920628285918,-40.5166166666667));
#238465=CARTESIAN_POINT('Ctrl Pts',(46.1766977413729,-58.4389030167283,
-40.4582833333333));
#238466=CARTESIAN_POINT('Ctrl Pts',(46.1766977413729,-57.4754524783491,
-40.39995));
#238467=CARTESIAN_POINT('Ctrl Pts',(46.1766977413729,-56.5120019399699,
-40.3416166666667));
#238468=CARTESIAN_POINT('Ctrl Pts',(45.3423250998467,-56.0302766707802,
-40.2832833333334));
#238469=CARTESIAN_POINT('Ctrl Pts',(44.5079524583205,-55.5485514015906,
-40.22495));
#238470=CARTESIAN_POINT('Ctrl Pts',(43.6735798167943,-56.0302766707802,
-40.1666166666667));
#238471=CARTESIAN_POINT('Ctrl Pts',(42.839207175268,-56.5120019399698,-40.1082833333334));
#238472=CARTESIAN_POINT('Ctrl Pts',(42.839207175268,-57.4754524783491,-40.04995));
#238473=CARTESIAN_POINT('Origin',(44.5079524583205,-57.4754524783491,-52.920575));
#238474=CARTESIAN_POINT('',(42.839207175268,-57.4754524783491,-41.44995));
#238475=CARTESIAN_POINT('',(42.839207175268,-57.4754524783491,-41.2912));
#238476=CARTESIAN_POINT('',(42.839207175268,-57.4754524783491,-52.920575));
#238477=CARTESIAN_POINT('Ctrl Pts',(42.839207175268,-57.4754524783491,-41.2912));
#238478=CARTESIAN_POINT('Ctrl Pts',(42.839207175268,-58.4389030167283,-41.2328666666667));
#238479=CARTESIAN_POINT('Ctrl Pts',(43.6735798167943,-58.920628285918,-41.1745333333334));
#238480=CARTESIAN_POINT('Ctrl Pts',(44.5079524583205,-59.4023535551075,
-41.1162));
#238481=CARTESIAN_POINT('Ctrl Pts',(45.3423250998467,-58.920628285918,-41.0578666666667));
#238482=CARTESIAN_POINT('Ctrl Pts',(46.1766977413729,-58.4389030167283,
-40.9995333333333));
#238483=CARTESIAN_POINT('Ctrl Pts',(46.1766977413729,-57.4754524783491,
-40.9412));
#238484=CARTESIAN_POINT('Ctrl Pts',(46.1766977413729,-56.5120019399699,
-40.8828666666667));
#238485=CARTESIAN_POINT('Ctrl Pts',(45.3423250998467,-56.0302766707802,
-40.8245333333333));
#238486=CARTESIAN_POINT('Ctrl Pts',(44.5079524583205,-55.5485514015906,
-40.7662));
#238487=CARTESIAN_POINT('Ctrl Pts',(43.6735798167943,-56.0302766707802,
-40.7078666666667));
#238488=CARTESIAN_POINT('Ctrl Pts',(42.839207175268,-56.5120019399698,-40.6495333333334));
#238489=CARTESIAN_POINT('Ctrl Pts',(42.839207175268,-57.4754524783491,-40.5912));
#238490=CARTESIAN_POINT('Ctrl Pts',(42.839207175268,-57.4754524783491,-41.44995));
#238491=CARTESIAN_POINT('Ctrl Pts',(42.839207175268,-58.4389030167283,-41.3916166666667));
#238492=CARTESIAN_POINT('Ctrl Pts',(43.6735798167943,-58.920628285918,-41.3332833333334));
#238493=CARTESIAN_POINT('Ctrl Pts',(44.5079524583205,-59.4023535551075,
-41.27495));
#238494=CARTESIAN_POINT('Ctrl Pts',(45.3423250998467,-58.920628285918,-41.2166166666667));
#238495=CARTESIAN_POINT('Ctrl Pts',(46.1766977413729,-58.4389030167283,
-41.1582833333333));
#238496=CARTESIAN_POINT('Ctrl Pts',(46.1766977413729,-57.4754524783491,
-41.09995));
#238497=CARTESIAN_POINT('Ctrl Pts',(46.1766977413729,-56.5120019399699,
-41.0416166666667));
#238498=CARTESIAN_POINT('Ctrl Pts',(45.3423250998467,-56.0302766707802,
-40.9832833333333));
#238499=CARTESIAN_POINT('Ctrl Pts',(44.5079524583205,-55.5485514015906,
-40.92495));
#238500=CARTESIAN_POINT('Ctrl Pts',(43.6735798167943,-56.0302766707802,
-40.8666166666667));
#238501=CARTESIAN_POINT('Ctrl Pts',(42.839207175268,-56.5120019399698,-40.8082833333334));
#238502=CARTESIAN_POINT('Ctrl Pts',(42.839207175268,-57.4754524783491,-40.74995));
#238503=CARTESIAN_POINT('Origin',(44.5079524583205,-57.4754524783491,-52.920575));
#238504=CARTESIAN_POINT('',(42.839207175268,-57.4754524783491,-42.14995));
#238505=CARTESIAN_POINT('',(42.839207175268,-57.4754524783491,-41.9912));
#238506=CARTESIAN_POINT('',(42.839207175268,-57.4754524783491,-52.920575));
#238507=CARTESIAN_POINT('Ctrl Pts',(42.839207175268,-57.4754524783491,-41.9912));
#238508=CARTESIAN_POINT('Ctrl Pts',(42.839207175268,-58.4389030167283,-41.9328666666667));
#238509=CARTESIAN_POINT('Ctrl Pts',(43.6735798167943,-58.920628285918,-41.8745333333334));
#238510=CARTESIAN_POINT('Ctrl Pts',(44.5079524583205,-59.4023535551075,
-41.8162));
#238511=CARTESIAN_POINT('Ctrl Pts',(45.3423250998467,-58.920628285918,-41.7578666666667));
#238512=CARTESIAN_POINT('Ctrl Pts',(46.1766977413729,-58.4389030167283,
-41.6995333333334));
#238513=CARTESIAN_POINT('Ctrl Pts',(46.1766977413729,-57.4754524783491,
-41.6412));
#238514=CARTESIAN_POINT('Ctrl Pts',(46.1766977413729,-56.5120019399699,
-41.5828666666667));
#238515=CARTESIAN_POINT('Ctrl Pts',(45.3423250998467,-56.0302766707802,
-41.5245333333334));
#238516=CARTESIAN_POINT('Ctrl Pts',(44.5079524583205,-55.5485514015906,
-41.4662));
#238517=CARTESIAN_POINT('Ctrl Pts',(43.6735798167943,-56.0302766707802,
-41.4078666666667));
#238518=CARTESIAN_POINT('Ctrl Pts',(42.839207175268,-56.5120019399698,-41.3495333333333));
#238519=CARTESIAN_POINT('Ctrl Pts',(42.839207175268,-57.4754524783491,-41.2912));
#238520=CARTESIAN_POINT('Ctrl Pts',(42.839207175268,-57.4754524783491,-42.14995));
#238521=CARTESIAN_POINT('Ctrl Pts',(42.839207175268,-58.4389030167283,-42.0916166666667));
#238522=CARTESIAN_POINT('Ctrl Pts',(43.6735798167943,-58.920628285918,-42.0332833333334));
#238523=CARTESIAN_POINT('Ctrl Pts',(44.5079524583205,-59.4023535551075,
-41.97495));
#238524=CARTESIAN_POINT('Ctrl Pts',(45.3423250998467,-58.920628285918,-41.9166166666667));
#238525=CARTESIAN_POINT('Ctrl Pts',(46.1766977413729,-58.4389030167283,
-41.8582833333333));
#238526=CARTESIAN_POINT('Ctrl Pts',(46.1766977413729,-57.4754524783491,
-41.79995));
#238527=CARTESIAN_POINT('Ctrl Pts',(46.1766977413729,-56.5120019399699,
-41.7416166666666));
#238528=CARTESIAN_POINT('Ctrl Pts',(45.3423250998467,-56.0302766707802,
-41.6832833333333));
#238529=CARTESIAN_POINT('Ctrl Pts',(44.5079524583205,-55.5485514015906,
-41.62495));
#238530=CARTESIAN_POINT('Ctrl Pts',(43.6735798167943,-56.0302766707802,
-41.5666166666667));
#238531=CARTESIAN_POINT('Ctrl Pts',(42.839207175268,-56.5120019399698,-41.5082833333334));
#238532=CARTESIAN_POINT('Ctrl Pts',(42.839207175268,-57.4754524783491,-41.44995));
#238533=CARTESIAN_POINT('Origin',(44.5079524583205,-57.4754524783491,-52.920575));
#238534=CARTESIAN_POINT('',(42.839207175268,-57.4754524783491,-42.84995));
#238535=CARTESIAN_POINT('',(42.839207175268,-57.4754524783491,-42.6912));
#238536=CARTESIAN_POINT('',(42.839207175268,-57.4754524783491,-52.920575));
#238537=CARTESIAN_POINT('Ctrl Pts',(42.839207175268,-57.4754524783491,-42.6912));
#238538=CARTESIAN_POINT('Ctrl Pts',(42.839207175268,-58.4389030167283,-42.6328666666667));
#238539=CARTESIAN_POINT('Ctrl Pts',(43.6735798167943,-58.920628285918,-42.5745333333333));
#238540=CARTESIAN_POINT('Ctrl Pts',(44.5079524583205,-59.4023535551075,
-42.5162));
#238541=CARTESIAN_POINT('Ctrl Pts',(45.3423250998467,-58.920628285918,-42.4578666666667));
#238542=CARTESIAN_POINT('Ctrl Pts',(46.1766977413729,-58.4389030167283,
-42.3995333333334));
#238543=CARTESIAN_POINT('Ctrl Pts',(46.1766977413729,-57.4754524783491,
-42.3412));
#238544=CARTESIAN_POINT('Ctrl Pts',(46.1766977413729,-56.5120019399699,
-42.2828666666667));
#238545=CARTESIAN_POINT('Ctrl Pts',(45.3423250998467,-56.0302766707802,
-42.2245333333333));
#238546=CARTESIAN_POINT('Ctrl Pts',(44.5079524583205,-55.5485514015906,
-42.1662));
#238547=CARTESIAN_POINT('Ctrl Pts',(43.6735798167943,-56.0302766707802,
-42.1078666666667));
#238548=CARTESIAN_POINT('Ctrl Pts',(42.839207175268,-56.5120019399698,-42.0495333333334));
#238549=CARTESIAN_POINT('Ctrl Pts',(42.839207175268,-57.4754524783491,-41.9912));
#238550=CARTESIAN_POINT('Ctrl Pts',(42.839207175268,-57.4754524783491,-42.84995));
#238551=CARTESIAN_POINT('Ctrl Pts',(42.839207175268,-58.4389030167283,-42.7916166666667));
#238552=CARTESIAN_POINT('Ctrl Pts',(43.6735798167943,-58.920628285918,-42.7332833333334));
#238553=CARTESIAN_POINT('Ctrl Pts',(44.5079524583205,-59.4023535551075,
-42.67495));
#238554=CARTESIAN_POINT('Ctrl Pts',(45.3423250998467,-58.920628285918,-42.6166166666667));
#238555=CARTESIAN_POINT('Ctrl Pts',(46.1766977413729,-58.4389030167283,
-42.5582833333333));
#238556=CARTESIAN_POINT('Ctrl Pts',(46.1766977413729,-57.4754524783491,
-42.49995));
#238557=CARTESIAN_POINT('Ctrl Pts',(46.1766977413729,-56.5120019399699,
-42.4416166666667));
#238558=CARTESIAN_POINT('Ctrl Pts',(45.3423250998467,-56.0302766707802,
-42.3832833333333));
#238559=CARTESIAN_POINT('Ctrl Pts',(44.5079524583205,-55.5485514015906,
-42.32495));
#238560=CARTESIAN_POINT('Ctrl Pts',(43.6735798167943,-56.0302766707802,
-42.2666166666667));
#238561=CARTESIAN_POINT('Ctrl Pts',(42.839207175268,-56.5120019399698,-42.2082833333333));
#238562=CARTESIAN_POINT('Ctrl Pts',(42.839207175268,-57.4754524783491,-42.14995));
#238563=CARTESIAN_POINT('Origin',(44.5079524583205,-57.4754524783491,-52.920575));
#238564=CARTESIAN_POINT('',(42.839207175268,-57.4754524783491,-43.54995));
#238565=CARTESIAN_POINT('',(42.839207175268,-57.4754524783491,-43.3912));
#238566=CARTESIAN_POINT('',(42.839207175268,-57.4754524783491,-52.920575));
#238567=CARTESIAN_POINT('Ctrl Pts',(42.839207175268,-57.4754524783491,-43.3912));
#238568=CARTESIAN_POINT('Ctrl Pts',(42.839207175268,-58.4389030167283,-43.3328666666667));
#238569=CARTESIAN_POINT('Ctrl Pts',(43.6735798167943,-58.920628285918,-43.2745333333334));
#238570=CARTESIAN_POINT('Ctrl Pts',(44.5079524583205,-59.4023535551075,
-43.2162));
#238571=CARTESIAN_POINT('Ctrl Pts',(45.3423250998467,-58.920628285918,-43.1578666666667));
#238572=CARTESIAN_POINT('Ctrl Pts',(46.1766977413729,-58.4389030167283,
-43.0995333333334));
#238573=CARTESIAN_POINT('Ctrl Pts',(46.1766977413729,-57.4754524783491,
-43.0412));
#238574=CARTESIAN_POINT('Ctrl Pts',(46.1766977413729,-56.5120019399699,
-42.9828666666667));
#238575=CARTESIAN_POINT('Ctrl Pts',(45.3423250998467,-56.0302766707802,
-42.9245333333334));
#238576=CARTESIAN_POINT('Ctrl Pts',(44.5079524583205,-55.5485514015906,
-42.8662));
#238577=CARTESIAN_POINT('Ctrl Pts',(43.6735798167943,-56.0302766707802,
-42.8078666666667));
#238578=CARTESIAN_POINT('Ctrl Pts',(42.839207175268,-56.5120019399698,-42.7495333333334));
#238579=CARTESIAN_POINT('Ctrl Pts',(42.839207175268,-57.4754524783491,-42.6912));
#238580=CARTESIAN_POINT('Ctrl Pts',(42.839207175268,-57.4754524783491,-43.54995));
#238581=CARTESIAN_POINT('Ctrl Pts',(42.839207175268,-58.4389030167283,-43.4916166666667));
#238582=CARTESIAN_POINT('Ctrl Pts',(43.6735798167943,-58.920628285918,-43.4332833333333));
#238583=CARTESIAN_POINT('Ctrl Pts',(44.5079524583205,-59.4023535551075,
-43.37495));
#238584=CARTESIAN_POINT('Ctrl Pts',(45.3423250998467,-58.920628285918,-43.3166166666667));
#238585=CARTESIAN_POINT('Ctrl Pts',(46.1766977413729,-58.4389030167283,
-43.2582833333333));
#238586=CARTESIAN_POINT('Ctrl Pts',(46.1766977413729,-57.4754524783491,
-43.19995));
#238587=CARTESIAN_POINT('Ctrl Pts',(46.1766977413729,-56.5120019399699,
-43.1416166666667));
#238588=CARTESIAN_POINT('Ctrl Pts',(45.3423250998467,-56.0302766707802,
-43.0832833333333));
#238589=CARTESIAN_POINT('Ctrl Pts',(44.5079524583205,-55.5485514015906,
-43.02495));
#238590=CARTESIAN_POINT('Ctrl Pts',(43.6735798167943,-56.0302766707802,
-42.9666166666667));
#238591=CARTESIAN_POINT('Ctrl Pts',(42.839207175268,-56.5120019399698,-42.9082833333333));
#238592=CARTESIAN_POINT('Ctrl Pts',(42.839207175268,-57.4754524783491,-42.84995));
#238593=CARTESIAN_POINT('Origin',(44.5079524583205,-57.4754524783491,-52.920575));
#238594=CARTESIAN_POINT('',(42.839207175268,-57.4754524783491,-44.24995));
#238595=CARTESIAN_POINT('',(42.839207175268,-57.4754524783491,-44.0912));
#238596=CARTESIAN_POINT('',(42.839207175268,-57.4754524783491,-52.920575));
#238597=CARTESIAN_POINT('Ctrl Pts',(42.839207175268,-57.4754524783491,-44.0912));
#238598=CARTESIAN_POINT('Ctrl Pts',(42.839207175268,-58.4389030167283,-44.0328666666667));
#238599=CARTESIAN_POINT('Ctrl Pts',(43.6735798167943,-58.920628285918,-43.9745333333333));
#238600=CARTESIAN_POINT('Ctrl Pts',(44.5079524583205,-59.4023535551075,
-43.9162));
#238601=CARTESIAN_POINT('Ctrl Pts',(45.3423250998467,-58.920628285918,-43.8578666666667));
#238602=CARTESIAN_POINT('Ctrl Pts',(46.1766977413729,-58.4389030167283,
-43.7995333333334));
#238603=CARTESIAN_POINT('Ctrl Pts',(46.1766977413729,-57.4754524783491,
-43.7412));
#238604=CARTESIAN_POINT('Ctrl Pts',(46.1766977413729,-56.5120019399699,
-43.6828666666667));
#238605=CARTESIAN_POINT('Ctrl Pts',(45.3423250998467,-56.0302766707802,
-43.6245333333333));
#238606=CARTESIAN_POINT('Ctrl Pts',(44.5079524583205,-55.5485514015906,
-43.5662));
#238607=CARTESIAN_POINT('Ctrl Pts',(43.6735798167943,-56.0302766707802,
-43.5078666666667));
#238608=CARTESIAN_POINT('Ctrl Pts',(42.839207175268,-56.5120019399698,-43.4495333333334));
#238609=CARTESIAN_POINT('Ctrl Pts',(42.839207175268,-57.4754524783491,-43.3912));
#238610=CARTESIAN_POINT('Ctrl Pts',(42.839207175268,-57.4754524783491,-44.24995));
#238611=CARTESIAN_POINT('Ctrl Pts',(42.839207175268,-58.4389030167283,-44.1916166666667));
#238612=CARTESIAN_POINT('Ctrl Pts',(43.6735798167943,-58.920628285918,-44.1332833333334));
#238613=CARTESIAN_POINT('Ctrl Pts',(44.5079524583205,-59.4023535551075,
-44.07495));
#238614=CARTESIAN_POINT('Ctrl Pts',(45.3423250998467,-58.920628285918,-44.0166166666667));
#238615=CARTESIAN_POINT('Ctrl Pts',(46.1766977413729,-58.4389030167283,
-43.9582833333334));
#238616=CARTESIAN_POINT('Ctrl Pts',(46.1766977413729,-57.4754524783491,
-43.89995));
#238617=CARTESIAN_POINT('Ctrl Pts',(46.1766977413729,-56.5120019399699,
-43.8416166666667));
#238618=CARTESIAN_POINT('Ctrl Pts',(45.3423250998467,-56.0302766707802,
-43.7832833333334));
#238619=CARTESIAN_POINT('Ctrl Pts',(44.5079524583205,-55.5485514015906,
-43.72495));
#238620=CARTESIAN_POINT('Ctrl Pts',(43.6735798167943,-56.0302766707802,
-43.6666166666667));
#238621=CARTESIAN_POINT('Ctrl Pts',(42.839207175268,-56.5120019399698,-43.6082833333334));
#238622=CARTESIAN_POINT('Ctrl Pts',(42.839207175268,-57.4754524783491,-43.54995));
#238623=CARTESIAN_POINT('Origin',(44.5079524583205,-57.4754524783491,-52.920575));
#238624=CARTESIAN_POINT('',(42.839207175268,-57.4754524783491,-44.94995));
#238625=CARTESIAN_POINT('',(42.839207175268,-57.4754524783491,-44.7912));
#238626=CARTESIAN_POINT('',(42.839207175268,-57.4754524783491,-52.920575));
#238627=CARTESIAN_POINT('Ctrl Pts',(42.839207175268,-57.4754524783491,-44.7912));
#238628=CARTESIAN_POINT('Ctrl Pts',(42.839207175268,-58.4389030167283,-44.7328666666667));
#238629=CARTESIAN_POINT('Ctrl Pts',(43.6735798167943,-58.920628285918,-44.6745333333334));
#238630=CARTESIAN_POINT('Ctrl Pts',(44.5079524583205,-59.4023535551075,
-44.6162));
#238631=CARTESIAN_POINT('Ctrl Pts',(45.3423250998467,-58.920628285918,-44.5578666666667));
#238632=CARTESIAN_POINT('Ctrl Pts',(46.1766977413729,-58.4389030167283,
-44.4995333333333));
#238633=CARTESIAN_POINT('Ctrl Pts',(46.1766977413729,-57.4754524783491,
-44.4412));
#238634=CARTESIAN_POINT('Ctrl Pts',(46.1766977413729,-56.5120019399699,
-44.3828666666667));
#238635=CARTESIAN_POINT('Ctrl Pts',(45.3423250998467,-56.0302766707802,
-44.3245333333334));
#238636=CARTESIAN_POINT('Ctrl Pts',(44.5079524583205,-55.5485514015906,
-44.2662));
#238637=CARTESIAN_POINT('Ctrl Pts',(43.6735798167943,-56.0302766707802,
-44.2078666666667));
#238638=CARTESIAN_POINT('Ctrl Pts',(42.839207175268,-56.5120019399698,-44.1495333333334));
#238639=CARTESIAN_POINT('Ctrl Pts',(42.839207175268,-57.4754524783491,-44.0912));
#238640=CARTESIAN_POINT('Ctrl Pts',(42.839207175268,-57.4754524783491,-44.94995));
#238641=CARTESIAN_POINT('Ctrl Pts',(42.839207175268,-58.4389030167283,-44.8916166666667));
#238642=CARTESIAN_POINT('Ctrl Pts',(43.6735798167943,-58.920628285918,-44.8332833333334));
#238643=CARTESIAN_POINT('Ctrl Pts',(44.5079524583205,-59.4023535551075,
-44.77495));
#238644=CARTESIAN_POINT('Ctrl Pts',(45.3423250998467,-58.920628285918,-44.7166166666667));
#238645=CARTESIAN_POINT('Ctrl Pts',(46.1766977413729,-58.4389030167283,
-44.6582833333334));
#238646=CARTESIAN_POINT('Ctrl Pts',(46.1766977413729,-57.4754524783491,
-44.59995));
#238647=CARTESIAN_POINT('Ctrl Pts',(46.1766977413729,-56.5120019399699,
-44.5416166666667));
#238648=CARTESIAN_POINT('Ctrl Pts',(45.3423250998467,-56.0302766707802,
-44.4832833333334));
#238649=CARTESIAN_POINT('Ctrl Pts',(44.5079524583205,-55.5485514015906,
-44.42495));
#238650=CARTESIAN_POINT('Ctrl Pts',(43.6735798167943,-56.0302766707802,
-44.3666166666667));
#238651=CARTESIAN_POINT('Ctrl Pts',(42.839207175268,-56.5120019399698,-44.3082833333334));
#238652=CARTESIAN_POINT('Ctrl Pts',(42.839207175268,-57.4754524783491,-44.24995));
#238653=CARTESIAN_POINT('Origin',(44.5079524583205,-57.4754524783491,-52.920575));
#238654=CARTESIAN_POINT('',(42.839207175268,-57.4754524783491,-45.64995));
#238655=CARTESIAN_POINT('',(42.839207175268,-57.4754524783491,-45.4912));
#238656=CARTESIAN_POINT('',(42.839207175268,-57.4754524783491,-52.920575));
#238657=CARTESIAN_POINT('Ctrl Pts',(42.839207175268,-57.4754524783491,-45.4912));
#238658=CARTESIAN_POINT('Ctrl Pts',(42.839207175268,-58.4389030167283,-45.4328666666666));
#238659=CARTESIAN_POINT('Ctrl Pts',(43.6735798167943,-58.920628285918,-45.3745333333334));
#238660=CARTESIAN_POINT('Ctrl Pts',(44.5079524583205,-59.4023535551075,
-45.3162));
#238661=CARTESIAN_POINT('Ctrl Pts',(45.3423250998467,-58.920628285918,-45.2578666666667));
#238662=CARTESIAN_POINT('Ctrl Pts',(46.1766977413729,-58.4389030167283,
-45.1995333333333));
#238663=CARTESIAN_POINT('Ctrl Pts',(46.1766977413729,-57.4754524783491,
-45.1412));
#238664=CARTESIAN_POINT('Ctrl Pts',(46.1766977413729,-56.5120019399699,
-45.0828666666667));
#238665=CARTESIAN_POINT('Ctrl Pts',(45.3423250998467,-56.0302766707802,
-45.0245333333334));
#238666=CARTESIAN_POINT('Ctrl Pts',(44.5079524583205,-55.5485514015906,
-44.9662));
#238667=CARTESIAN_POINT('Ctrl Pts',(43.6735798167943,-56.0302766707802,
-44.9078666666667));
#238668=CARTESIAN_POINT('Ctrl Pts',(42.839207175268,-56.5120019399698,-44.8495333333333));
#238669=CARTESIAN_POINT('Ctrl Pts',(42.839207175268,-57.4754524783491,-44.7912));
#238670=CARTESIAN_POINT('Ctrl Pts',(42.839207175268,-57.4754524783491,-45.64995));
#238671=CARTESIAN_POINT('Ctrl Pts',(42.839207175268,-58.4389030167283,-45.5916166666667));
#238672=CARTESIAN_POINT('Ctrl Pts',(43.6735798167943,-58.920628285918,-45.5332833333333));
#238673=CARTESIAN_POINT('Ctrl Pts',(44.5079524583205,-59.4023535551075,
-45.47495));
#238674=CARTESIAN_POINT('Ctrl Pts',(45.3423250998467,-58.920628285918,-45.4166166666667));
#238675=CARTESIAN_POINT('Ctrl Pts',(46.1766977413729,-58.4389030167283,
-45.3582833333334));
#238676=CARTESIAN_POINT('Ctrl Pts',(46.1766977413729,-57.4754524783491,
-45.29995));
#238677=CARTESIAN_POINT('Ctrl Pts',(46.1766977413729,-56.5120019399699,
-45.2416166666667));
#238678=CARTESIAN_POINT('Ctrl Pts',(45.3423250998467,-56.0302766707802,
-45.1832833333334));
#238679=CARTESIAN_POINT('Ctrl Pts',(44.5079524583205,-55.5485514015906,
-45.12495));
#238680=CARTESIAN_POINT('Ctrl Pts',(43.6735798167943,-56.0302766707802,
-45.0666166666667));
#238681=CARTESIAN_POINT('Ctrl Pts',(42.839207175268,-56.5120019399698,-45.0082833333334));
#238682=CARTESIAN_POINT('Ctrl Pts',(42.839207175268,-57.4754524783491,-44.94995));
#238683=CARTESIAN_POINT('Origin',(44.5079524583205,-57.4754524783491,-52.920575));
#238684=CARTESIAN_POINT('',(42.839207175268,-57.4754524783491,-46.34995));
#238685=CARTESIAN_POINT('',(42.839207175268,-57.4754524783491,-46.1912));
#238686=CARTESIAN_POINT('',(42.839207175268,-57.4754524783491,-52.920575));
#238687=CARTESIAN_POINT('Ctrl Pts',(42.839207175268,-57.4754524783491,-46.1912));
#238688=CARTESIAN_POINT('Ctrl Pts',(42.839207175268,-58.4389030167283,-46.1328666666667));
#238689=CARTESIAN_POINT('Ctrl Pts',(43.6735798167943,-58.920628285918,-46.0745333333334));
#238690=CARTESIAN_POINT('Ctrl Pts',(44.5079524583205,-59.4023535551075,
-46.0162));
#238691=CARTESIAN_POINT('Ctrl Pts',(45.3423250998467,-58.920628285918,-45.9578666666667));
#238692=CARTESIAN_POINT('Ctrl Pts',(46.1766977413729,-58.4389030167283,
-45.8995333333333));
#238693=CARTESIAN_POINT('Ctrl Pts',(46.1766977413729,-57.4754524783491,
-45.8412));
#238694=CARTESIAN_POINT('Ctrl Pts',(46.1766977413729,-56.5120019399699,
-45.7828666666667));
#238695=CARTESIAN_POINT('Ctrl Pts',(45.3423250998467,-56.0302766707802,
-45.7245333333333));
#238696=CARTESIAN_POINT('Ctrl Pts',(44.5079524583205,-55.5485514015906,
-45.6662));
#238697=CARTESIAN_POINT('Ctrl Pts',(43.6735798167943,-56.0302766707802,
-45.6078666666667));
#238698=CARTESIAN_POINT('Ctrl Pts',(42.839207175268,-56.5120019399698,-45.5495333333333));
#238699=CARTESIAN_POINT('Ctrl Pts',(42.839207175268,-57.4754524783491,-45.4912));
#238700=CARTESIAN_POINT('Ctrl Pts',(42.839207175268,-57.4754524783491,-46.34995));
#238701=CARTESIAN_POINT('Ctrl Pts',(42.839207175268,-58.4389030167283,-46.2916166666667));
#238702=CARTESIAN_POINT('Ctrl Pts',(43.6735798167943,-58.920628285918,-46.2332833333334));
#238703=CARTESIAN_POINT('Ctrl Pts',(44.5079524583205,-59.4023535551075,
-46.17495));
#238704=CARTESIAN_POINT('Ctrl Pts',(45.3423250998467,-58.920628285918,-46.1166166666667));
#238705=CARTESIAN_POINT('Ctrl Pts',(46.1766977413729,-58.4389030167283,
-46.0582833333333));
#238706=CARTESIAN_POINT('Ctrl Pts',(46.1766977413729,-57.4754524783491,
-45.99995));
#238707=CARTESIAN_POINT('Ctrl Pts',(46.1766977413729,-56.5120019399699,
-45.9416166666667));
#238708=CARTESIAN_POINT('Ctrl Pts',(45.3423250998467,-56.0302766707802,
-45.8832833333333));
#238709=CARTESIAN_POINT('Ctrl Pts',(44.5079524583205,-55.5485514015906,
-45.82495));
#238710=CARTESIAN_POINT('Ctrl Pts',(43.6735798167943,-56.0302766707802,
-45.7666166666667));
#238711=CARTESIAN_POINT('Ctrl Pts',(42.839207175268,-56.5120019399698,-45.7082833333333));
#238712=CARTESIAN_POINT('Ctrl Pts',(42.839207175268,-57.4754524783491,-45.64995));
#238713=CARTESIAN_POINT('Origin',(44.5079524583205,-57.4754524783491,-52.920575));
#238714=CARTESIAN_POINT('',(42.839207175268,-57.4754524783491,-47.04995));
#238715=CARTESIAN_POINT('',(42.839207175268,-57.4754524783491,-46.8912));
#238716=CARTESIAN_POINT('',(42.839207175268,-57.4754524783491,-52.920575));
#238717=CARTESIAN_POINT('Ctrl Pts',(42.839207175268,-57.4754524783491,-46.8912));
#238718=CARTESIAN_POINT('Ctrl Pts',(42.839207175268,-58.4389030167283,-46.8328666666667));
#238719=CARTESIAN_POINT('Ctrl Pts',(43.6735798167943,-58.920628285918,-46.7745333333334));
#238720=CARTESIAN_POINT('Ctrl Pts',(44.5079524583205,-59.4023535551075,
-46.7162));
#238721=CARTESIAN_POINT('Ctrl Pts',(45.3423250998467,-58.920628285918,-46.6578666666667));
#238722=CARTESIAN_POINT('Ctrl Pts',(46.1766977413729,-58.4389030167283,
-46.5995333333334));
#238723=CARTESIAN_POINT('Ctrl Pts',(46.1766977413729,-57.4754524783491,
-46.5412));
#238724=CARTESIAN_POINT('Ctrl Pts',(46.1766977413729,-56.5120019399699,
-46.4828666666667));
#238725=CARTESIAN_POINT('Ctrl Pts',(45.3423250998467,-56.0302766707802,
-46.4245333333334));
#238726=CARTESIAN_POINT('Ctrl Pts',(44.5079524583205,-55.5485514015906,
-46.3662));
#238727=CARTESIAN_POINT('Ctrl Pts',(43.6735798167943,-56.0302766707802,
-46.3078666666667));
#238728=CARTESIAN_POINT('Ctrl Pts',(42.839207175268,-56.5120019399698,-46.2495333333334));
#238729=CARTESIAN_POINT('Ctrl Pts',(42.839207175268,-57.4754524783491,-46.1912));
#238730=CARTESIAN_POINT('Ctrl Pts',(42.839207175268,-57.4754524783491,-47.04995));
#238731=CARTESIAN_POINT('Ctrl Pts',(42.839207175268,-58.4389030167283,-46.9916166666667));
#238732=CARTESIAN_POINT('Ctrl Pts',(43.6735798167943,-58.920628285918,-46.9332833333334));
#238733=CARTESIAN_POINT('Ctrl Pts',(44.5079524583205,-59.4023535551075,
-46.87495));
#238734=CARTESIAN_POINT('Ctrl Pts',(45.3423250998467,-58.920628285918,-46.8166166666667));
#238735=CARTESIAN_POINT('Ctrl Pts',(46.1766977413729,-58.4389030167283,
-46.7582833333333));
#238736=CARTESIAN_POINT('Ctrl Pts',(46.1766977413729,-57.4754524783491,
-46.69995));
#238737=CARTESIAN_POINT('Ctrl Pts',(46.1766977413729,-56.5120019399699,
-46.6416166666666));
#238738=CARTESIAN_POINT('Ctrl Pts',(45.3423250998467,-56.0302766707802,
-46.5832833333334));
#238739=CARTESIAN_POINT('Ctrl Pts',(44.5079524583205,-55.5485514015906,
-46.52495));
#238740=CARTESIAN_POINT('Ctrl Pts',(43.6735798167943,-56.0302766707802,
-46.4666166666667));
#238741=CARTESIAN_POINT('Ctrl Pts',(42.839207175268,-56.5120019399698,-46.4082833333333));
#238742=CARTESIAN_POINT('Ctrl Pts',(42.839207175268,-57.4754524783491,-46.34995));
#238743=CARTESIAN_POINT('Origin',(44.5079524583205,-57.4754524783491,-52.920575));
#238744=CARTESIAN_POINT('',(42.839207175268,-57.4754524783491,-47.74995));
#238745=CARTESIAN_POINT('',(42.839207175268,-57.4754524783491,-47.5912));
#238746=CARTESIAN_POINT('',(42.839207175268,-57.4754524783491,-52.920575));
#238747=CARTESIAN_POINT('Ctrl Pts',(42.839207175268,-57.4754524783491,-47.5912));
#238748=CARTESIAN_POINT('Ctrl Pts',(42.839207175268,-58.4389030167283,-47.5328666666667));
#238749=CARTESIAN_POINT('Ctrl Pts',(43.6735798167943,-58.920628285918,-47.4745333333334));
#238750=CARTESIAN_POINT('Ctrl Pts',(44.5079524583205,-59.4023535551075,
-47.4162));
#238751=CARTESIAN_POINT('Ctrl Pts',(45.3423250998467,-58.920628285918,-47.3578666666667));
#238752=CARTESIAN_POINT('Ctrl Pts',(46.1766977413729,-58.4389030167283,
-47.2995333333334));
#238753=CARTESIAN_POINT('Ctrl Pts',(46.1766977413729,-57.4754524783491,
-47.2412));
#238754=CARTESIAN_POINT('Ctrl Pts',(46.1766977413729,-56.5120019399699,
-47.1828666666667));
#238755=CARTESIAN_POINT('Ctrl Pts',(45.3423250998467,-56.0302766707802,
-47.1245333333333));
#238756=CARTESIAN_POINT('Ctrl Pts',(44.5079524583205,-55.5485514015906,
-47.0662));
#238757=CARTESIAN_POINT('Ctrl Pts',(43.6735798167943,-56.0302766707802,
-47.0078666666667));
#238758=CARTESIAN_POINT('Ctrl Pts',(42.839207175268,-56.5120019399698,-46.9495333333334));
#238759=CARTESIAN_POINT('Ctrl Pts',(42.839207175268,-57.4754524783491,-46.8912));
#238760=CARTESIAN_POINT('Ctrl Pts',(42.839207175268,-57.4754524783491,-47.74995));
#238761=CARTESIAN_POINT('Ctrl Pts',(42.839207175268,-58.4389030167283,-47.6916166666667));
#238762=CARTESIAN_POINT('Ctrl Pts',(43.6735798167943,-58.920628285918,-47.6332833333333));
#238763=CARTESIAN_POINT('Ctrl Pts',(44.5079524583205,-59.4023535551075,
-47.57495));
#238764=CARTESIAN_POINT('Ctrl Pts',(45.3423250998467,-58.920628285918,-47.5166166666667));
#238765=CARTESIAN_POINT('Ctrl Pts',(46.1766977413729,-58.4389030167283,
-47.4582833333333));
#238766=CARTESIAN_POINT('Ctrl Pts',(46.1766977413729,-57.4754524783491,
-47.39995));
#238767=CARTESIAN_POINT('Ctrl Pts',(46.1766977413729,-56.5120019399699,
-47.3416166666667));
#238768=CARTESIAN_POINT('Ctrl Pts',(45.3423250998467,-56.0302766707802,
-47.2832833333333));
#238769=CARTESIAN_POINT('Ctrl Pts',(44.5079524583205,-55.5485514015906,
-47.22495));
#238770=CARTESIAN_POINT('Ctrl Pts',(43.6735798167943,-56.0302766707802,
-47.1666166666667));
#238771=CARTESIAN_POINT('Ctrl Pts',(42.839207175268,-56.5120019399698,-47.1082833333333));
#238772=CARTESIAN_POINT('Ctrl Pts',(42.839207175268,-57.4754524783491,-47.04995));
#238773=CARTESIAN_POINT('Origin',(44.5079524583205,-57.4754524783491,-52.920575));
#238774=CARTESIAN_POINT('',(42.839207175268,-57.4754524783491,-48.44995));
#238775=CARTESIAN_POINT('',(42.839207175268,-57.4754524783491,-48.2912));
#238776=CARTESIAN_POINT('',(42.839207175268,-57.4754524783491,-52.920575));
#238777=CARTESIAN_POINT('Ctrl Pts',(42.839207175268,-57.4754524783491,-48.2912));
#238778=CARTESIAN_POINT('Ctrl Pts',(42.839207175268,-58.4389030167283,-48.2328666666667));
#238779=CARTESIAN_POINT('Ctrl Pts',(43.6735798167943,-58.920628285918,-48.1745333333334));
#238780=CARTESIAN_POINT('Ctrl Pts',(44.5079524583205,-59.4023535551075,
-48.1162));
#238781=CARTESIAN_POINT('Ctrl Pts',(45.3423250998467,-58.920628285918,-48.0578666666667));
#238782=CARTESIAN_POINT('Ctrl Pts',(46.1766977413729,-58.4389030167283,
-47.9995333333334));
#238783=CARTESIAN_POINT('Ctrl Pts',(46.1766977413729,-57.4754524783491,
-47.9412));
#238784=CARTESIAN_POINT('Ctrl Pts',(46.1766977413729,-56.5120019399699,
-47.8828666666667));
#238785=CARTESIAN_POINT('Ctrl Pts',(45.3423250998467,-56.0302766707802,
-47.8245333333333));
#238786=CARTESIAN_POINT('Ctrl Pts',(44.5079524583205,-55.5485514015906,
-47.7662));
#238787=CARTESIAN_POINT('Ctrl Pts',(43.6735798167943,-56.0302766707802,
-47.7078666666667));
#238788=CARTESIAN_POINT('Ctrl Pts',(42.839207175268,-56.5120019399698,-47.6495333333334));
#238789=CARTESIAN_POINT('Ctrl Pts',(42.839207175268,-57.4754524783491,-47.5912));
#238790=CARTESIAN_POINT('Ctrl Pts',(42.839207175268,-57.4754524783491,-48.44995));
#238791=CARTESIAN_POINT('Ctrl Pts',(42.839207175268,-58.4389030167283,-48.3916166666667));
#238792=CARTESIAN_POINT('Ctrl Pts',(43.6735798167943,-58.920628285918,-48.3332833333334));
#238793=CARTESIAN_POINT('Ctrl Pts',(44.5079524583205,-59.4023535551075,
-48.27495));
#238794=CARTESIAN_POINT('Ctrl Pts',(45.3423250998467,-58.920628285918,-48.2166166666667));
#238795=CARTESIAN_POINT('Ctrl Pts',(46.1766977413729,-58.4389030167283,
-48.1582833333334));
#238796=CARTESIAN_POINT('Ctrl Pts',(46.1766977413729,-57.4754524783491,
-48.09995));
#238797=CARTESIAN_POINT('Ctrl Pts',(46.1766977413729,-56.5120019399699,
-48.0416166666667));
#238798=CARTESIAN_POINT('Ctrl Pts',(45.3423250998467,-56.0302766707802,
-47.9832833333334));
#238799=CARTESIAN_POINT('Ctrl Pts',(44.5079524583205,-55.5485514015906,
-47.92495));
#238800=CARTESIAN_POINT('Ctrl Pts',(43.6735798167943,-56.0302766707802,
-47.8666166666667));
#238801=CARTESIAN_POINT('Ctrl Pts',(42.839207175268,-56.5120019399698,-47.8082833333333));
#238802=CARTESIAN_POINT('Ctrl Pts',(42.839207175268,-57.4754524783491,-47.74995));
#238803=CARTESIAN_POINT('Origin',(44.5079524583205,-57.4754524783491,-52.920575));
#238804=CARTESIAN_POINT('',(42.839207175268,-57.4754524783491,-49.14995));
#238805=CARTESIAN_POINT('',(42.839207175268,-57.4754524783491,-48.9912));
#238806=CARTESIAN_POINT('',(42.839207175268,-57.4754524783491,-52.920575));
#238807=CARTESIAN_POINT('Ctrl Pts',(42.839207175268,-57.4754524783491,-48.9912));
#238808=CARTESIAN_POINT('Ctrl Pts',(42.839207175268,-58.4389030167283,-48.9328666666667));
#238809=CARTESIAN_POINT('Ctrl Pts',(43.6735798167943,-58.920628285918,-48.8745333333334));
#238810=CARTESIAN_POINT('Ctrl Pts',(44.5079524583205,-59.4023535551075,
-48.8162));
#238811=CARTESIAN_POINT('Ctrl Pts',(45.3423250998467,-58.920628285918,-48.7578666666667));
#238812=CARTESIAN_POINT('Ctrl Pts',(46.1766977413729,-58.4389030167283,
-48.6995333333333));
#238813=CARTESIAN_POINT('Ctrl Pts',(46.1766977413729,-57.4754524783491,
-48.6412));
#238814=CARTESIAN_POINT('Ctrl Pts',(46.1766977413729,-56.5120019399699,
-48.5828666666667));
#238815=CARTESIAN_POINT('Ctrl Pts',(45.3423250998467,-56.0302766707802,
-48.5245333333334));
#238816=CARTESIAN_POINT('Ctrl Pts',(44.5079524583205,-55.5485514015906,
-48.4662));
#238817=CARTESIAN_POINT('Ctrl Pts',(43.6735798167943,-56.0302766707802,
-48.4078666666667));
#238818=CARTESIAN_POINT('Ctrl Pts',(42.839207175268,-56.5120019399698,-48.3495333333333));
#238819=CARTESIAN_POINT('Ctrl Pts',(42.839207175268,-57.4754524783491,-48.2912));
#238820=CARTESIAN_POINT('Ctrl Pts',(42.839207175268,-57.4754524783491,-49.14995));
#238821=CARTESIAN_POINT('Ctrl Pts',(42.839207175268,-58.4389030167283,-49.0916166666667));
#238822=CARTESIAN_POINT('Ctrl Pts',(43.6735798167943,-58.920628285918,-49.0332833333333));
#238823=CARTESIAN_POINT('Ctrl Pts',(44.5079524583205,-59.4023535551075,
-48.97495));
#238824=CARTESIAN_POINT('Ctrl Pts',(45.3423250998467,-58.920628285918,-48.9166166666667));
#238825=CARTESIAN_POINT('Ctrl Pts',(46.1766977413729,-58.4389030167283,
-48.8582833333333));
#238826=CARTESIAN_POINT('Ctrl Pts',(46.1766977413729,-57.4754524783491,
-48.79995));
#238827=CARTESIAN_POINT('Ctrl Pts',(46.1766977413729,-56.5120019399699,
-48.7416166666667));
#238828=CARTESIAN_POINT('Ctrl Pts',(45.3423250998467,-56.0302766707802,
-48.6832833333334));
#238829=CARTESIAN_POINT('Ctrl Pts',(44.5079524583205,-55.5485514015906,
-48.62495));
#238830=CARTESIAN_POINT('Ctrl Pts',(43.6735798167943,-56.0302766707802,
-48.5666166666667));
#238831=CARTESIAN_POINT('Ctrl Pts',(42.839207175268,-56.5120019399698,-48.5082833333334));
#238832=CARTESIAN_POINT('Ctrl Pts',(42.839207175268,-57.4754524783491,-48.44995));
#238833=CARTESIAN_POINT('Origin',(44.5079524583205,-57.4754524783491,-52.920575));
#238834=CARTESIAN_POINT('',(42.839207175268,-57.4754524783491,-49.84995));
#238835=CARTESIAN_POINT('',(42.839207175268,-57.4754524783491,-49.6912));
#238836=CARTESIAN_POINT('',(42.839207175268,-57.4754524783491,-52.920575));
#238837=CARTESIAN_POINT('Ctrl Pts',(42.839207175268,-57.4754524783491,-49.6912));
#238838=CARTESIAN_POINT('Ctrl Pts',(42.839207175268,-58.4389030167283,-49.6328666666667));
#238839=CARTESIAN_POINT('Ctrl Pts',(43.6735798167943,-58.920628285918,-49.5745333333334));
#238840=CARTESIAN_POINT('Ctrl Pts',(44.5079524583205,-59.4023535551075,
-49.5162));
#238841=CARTESIAN_POINT('Ctrl Pts',(45.3423250998467,-58.920628285918,-49.4578666666667));
#238842=CARTESIAN_POINT('Ctrl Pts',(46.1766977413729,-58.4389030167283,
-49.3995333333333));
#238843=CARTESIAN_POINT('Ctrl Pts',(46.1766977413729,-57.4754524783491,
-49.3412));
#238844=CARTESIAN_POINT('Ctrl Pts',(46.1766977413729,-56.5120019399699,
-49.2828666666667));
#238845=CARTESIAN_POINT('Ctrl Pts',(45.3423250998467,-56.0302766707802,
-49.2245333333334));
#238846=CARTESIAN_POINT('Ctrl Pts',(44.5079524583205,-55.5485514015906,
-49.1662));
#238847=CARTESIAN_POINT('Ctrl Pts',(43.6735798167943,-56.0302766707802,
-49.1078666666667));
#238848=CARTESIAN_POINT('Ctrl Pts',(42.839207175268,-56.5120019399698,-49.0495333333334));
#238849=CARTESIAN_POINT('Ctrl Pts',(42.839207175268,-57.4754524783491,-48.9912));
#238850=CARTESIAN_POINT('Ctrl Pts',(42.839207175268,-57.4754524783491,-49.84995));
#238851=CARTESIAN_POINT('Ctrl Pts',(42.839207175268,-58.4389030167283,-49.7916166666667));
#238852=CARTESIAN_POINT('Ctrl Pts',(43.6735798167943,-58.920628285918,-49.7332833333334));
#238853=CARTESIAN_POINT('Ctrl Pts',(44.5079524583205,-59.4023535551075,
-49.67495));
#238854=CARTESIAN_POINT('Ctrl Pts',(45.3423250998467,-58.920628285918,-49.6166166666667));
#238855=CARTESIAN_POINT('Ctrl Pts',(46.1766977413729,-58.4389030167283,
-49.5582833333334));
#238856=CARTESIAN_POINT('Ctrl Pts',(46.1766977413729,-57.4754524783491,
-49.49995));
#238857=CARTESIAN_POINT('Ctrl Pts',(46.1766977413729,-56.5120019399699,
-49.4416166666667));
#238858=CARTESIAN_POINT('Ctrl Pts',(45.3423250998467,-56.0302766707802,
-49.3832833333334));
#238859=CARTESIAN_POINT('Ctrl Pts',(44.5079524583205,-55.5485514015906,
-49.32495));
#238860=CARTESIAN_POINT('Ctrl Pts',(43.6735798167943,-56.0302766707802,
-49.2666166666667));
#238861=CARTESIAN_POINT('Ctrl Pts',(42.839207175268,-56.5120019399698,-49.2082833333334));
#238862=CARTESIAN_POINT('Ctrl Pts',(42.839207175268,-57.4754524783491,-49.14995));
#238863=CARTESIAN_POINT('Origin',(44.5079524583205,-57.4754524783491,-52.920575));
#238864=CARTESIAN_POINT('',(42.839207175268,-57.4754524783491,-50.54995));
#238865=CARTESIAN_POINT('',(42.839207175268,-57.4754524783491,-50.3912));
#238866=CARTESIAN_POINT('',(42.839207175268,-57.4754524783491,-52.920575));
#238867=CARTESIAN_POINT('Ctrl Pts',(42.839207175268,-57.4754524783491,-50.3912));
#238868=CARTESIAN_POINT('Ctrl Pts',(42.839207175268,-58.4389030167283,-50.3328666666667));
#238869=CARTESIAN_POINT('Ctrl Pts',(43.6735798167943,-58.920628285918,-50.2745333333334));
#238870=CARTESIAN_POINT('Ctrl Pts',(44.5079524583205,-59.4023535551075,
-50.2162));
#238871=CARTESIAN_POINT('Ctrl Pts',(45.3423250998467,-58.920628285918,-50.1578666666667));
#238872=CARTESIAN_POINT('Ctrl Pts',(46.1766977413729,-58.4389030167283,
-50.0995333333333));
#238873=CARTESIAN_POINT('Ctrl Pts',(46.1766977413729,-57.4754524783491,
-50.0412));
#238874=CARTESIAN_POINT('Ctrl Pts',(46.1766977413729,-56.5120019399699,
-49.9828666666667));
#238875=CARTESIAN_POINT('Ctrl Pts',(45.3423250998467,-56.0302766707802,
-49.9245333333334));
#238876=CARTESIAN_POINT('Ctrl Pts',(44.5079524583205,-55.5485514015906,
-49.8662));
#238877=CARTESIAN_POINT('Ctrl Pts',(43.6735798167943,-56.0302766707802,
-49.8078666666667));
#238878=CARTESIAN_POINT('Ctrl Pts',(42.839207175268,-56.5120019399698,-49.7495333333333));
#238879=CARTESIAN_POINT('Ctrl Pts',(42.839207175268,-57.4754524783491,-49.6912));
#238880=CARTESIAN_POINT('Ctrl Pts',(42.839207175268,-57.4754524783491,-50.54995));
#238881=CARTESIAN_POINT('Ctrl Pts',(42.839207175268,-58.4389030167283,-50.4916166666667));
#238882=CARTESIAN_POINT('Ctrl Pts',(43.6735798167943,-58.920628285918,-50.4332833333333));
#238883=CARTESIAN_POINT('Ctrl Pts',(44.5079524583205,-59.4023535551075,
-50.37495));
#238884=CARTESIAN_POINT('Ctrl Pts',(45.3423250998467,-58.920628285918,-50.3166166666667));
#238885=CARTESIAN_POINT('Ctrl Pts',(46.1766977413729,-58.4389030167283,
-50.2582833333334));
#238886=CARTESIAN_POINT('Ctrl Pts',(46.1766977413729,-57.4754524783491,
-50.19995));
#238887=CARTESIAN_POINT('Ctrl Pts',(46.1766977413729,-56.5120019399699,
-50.1416166666667));
#238888=CARTESIAN_POINT('Ctrl Pts',(45.3423250998467,-56.0302766707802,
-50.0832833333334));
#238889=CARTESIAN_POINT('Ctrl Pts',(44.5079524583205,-55.5485514015906,
-50.02495));
#238890=CARTESIAN_POINT('Ctrl Pts',(43.6735798167943,-56.0302766707802,
-49.9666166666667));
#238891=CARTESIAN_POINT('Ctrl Pts',(42.839207175268,-56.5120019399698,-49.9082833333334));
#238892=CARTESIAN_POINT('Ctrl Pts',(42.839207175268,-57.4754524783491,-49.84995));
#238893=CARTESIAN_POINT('Origin',(44.5079524583205,-57.4754524783491,-52.920575));
#238894=CARTESIAN_POINT('',(42.839207175268,-57.4754524783491,-51.24995));
#238895=CARTESIAN_POINT('',(42.839207175268,-57.4754524783491,-51.0912));
#238896=CARTESIAN_POINT('',(42.839207175268,-57.4754524783491,-52.920575));
#238897=CARTESIAN_POINT('Ctrl Pts',(42.839207175268,-57.4754524783491,-51.0912));
#238898=CARTESIAN_POINT('Ctrl Pts',(42.839207175268,-58.4389030167283,-51.0328666666667));
#238899=CARTESIAN_POINT('Ctrl Pts',(43.6735798167943,-58.920628285918,-50.9745333333333));
#238900=CARTESIAN_POINT('Ctrl Pts',(44.5079524583205,-59.4023535551075,
-50.9162));
#238901=CARTESIAN_POINT('Ctrl Pts',(45.3423250998467,-58.920628285918,-50.8578666666667));
#238902=CARTESIAN_POINT('Ctrl Pts',(46.1766977413729,-58.4389030167283,
-50.7995333333334));
#238903=CARTESIAN_POINT('Ctrl Pts',(46.1766977413729,-57.4754524783491,
-50.7412));
#238904=CARTESIAN_POINT('Ctrl Pts',(46.1766977413729,-56.5120019399699,
-50.6828666666667));
#238905=CARTESIAN_POINT('Ctrl Pts',(45.3423250998467,-56.0302766707802,
-50.6245333333333));
#238906=CARTESIAN_POINT('Ctrl Pts',(44.5079524583205,-55.5485514015906,
-50.5662));
#238907=CARTESIAN_POINT('Ctrl Pts',(43.6735798167943,-56.0302766707802,
-50.5078666666667));
#238908=CARTESIAN_POINT('Ctrl Pts',(42.839207175268,-56.5120019399698,-50.4495333333333));
#238909=CARTESIAN_POINT('Ctrl Pts',(42.839207175268,-57.4754524783491,-50.3912));
#238910=CARTESIAN_POINT('Ctrl Pts',(42.839207175268,-57.4754524783491,-51.24995));
#238911=CARTESIAN_POINT('Ctrl Pts',(42.839207175268,-58.4389030167283,-51.1916166666667));
#238912=CARTESIAN_POINT('Ctrl Pts',(43.6735798167943,-58.920628285918,-51.1332833333334));
#238913=CARTESIAN_POINT('Ctrl Pts',(44.5079524583205,-59.4023535551075,
-51.07495));
#238914=CARTESIAN_POINT('Ctrl Pts',(45.3423250998467,-58.920628285918,-51.0166166666667));
#238915=CARTESIAN_POINT('Ctrl Pts',(46.1766977413729,-58.4389030167283,
-50.9582833333334));
#238916=CARTESIAN_POINT('Ctrl Pts',(46.1766977413729,-57.4754524783491,
-50.89995));
#238917=CARTESIAN_POINT('Ctrl Pts',(46.1766977413729,-56.5120019399699,
-50.8416166666667));
#238918=CARTESIAN_POINT('Ctrl Pts',(45.3423250998467,-56.0302766707802,
-50.7832833333333));
#238919=CARTESIAN_POINT('Ctrl Pts',(44.5079524583205,-55.5485514015906,
-50.72495));
#238920=CARTESIAN_POINT('Ctrl Pts',(43.6735798167943,-56.0302766707802,
-50.6666166666667));
#238921=CARTESIAN_POINT('Ctrl Pts',(42.839207175268,-56.5120019399698,-50.6082833333334));
#238922=CARTESIAN_POINT('Ctrl Pts',(42.839207175268,-57.4754524783491,-50.54995));
#238923=CARTESIAN_POINT('Origin',(44.5079524583205,-57.4754524783491,-52.920575));
#238924=CARTESIAN_POINT('',(42.839207175268,-57.4754524783491,-51.94995));
#238925=CARTESIAN_POINT('',(42.839207175268,-57.4754524783491,-51.7912));
#238926=CARTESIAN_POINT('',(42.839207175268,-57.4754524783491,-52.920575));
#238927=CARTESIAN_POINT('Ctrl Pts',(42.839207175268,-57.4754524783491,-51.7912));
#238928=CARTESIAN_POINT('Ctrl Pts',(42.839207175268,-58.4389030167283,-51.7328666666667));
#238929=CARTESIAN_POINT('Ctrl Pts',(43.6735798167943,-58.920628285918,-51.6745333333334));
#238930=CARTESIAN_POINT('Ctrl Pts',(44.5079524583205,-59.4023535551075,
-51.6162));
#238931=CARTESIAN_POINT('Ctrl Pts',(45.3423250998467,-58.920628285918,-51.5578666666667));
#238932=CARTESIAN_POINT('Ctrl Pts',(46.1766977413729,-58.4389030167283,
-51.4995333333334));
#238933=CARTESIAN_POINT('Ctrl Pts',(46.1766977413729,-57.4754524783491,
-51.4412));
#238934=CARTESIAN_POINT('Ctrl Pts',(46.1766977413729,-56.5120019399699,
-51.3828666666667));
#238935=CARTESIAN_POINT('Ctrl Pts',(45.3423250998467,-56.0302766707802,
-51.3245333333334));
#238936=CARTESIAN_POINT('Ctrl Pts',(44.5079524583205,-55.5485514015906,
-51.2662));
#238937=CARTESIAN_POINT('Ctrl Pts',(43.6735798167943,-56.0302766707802,
-51.2078666666667));
#238938=CARTESIAN_POINT('Ctrl Pts',(42.839207175268,-56.5120019399698,-51.1495333333334));
#238939=CARTESIAN_POINT('Ctrl Pts',(42.839207175268,-57.4754524783491,-51.0912));
#238940=CARTESIAN_POINT('Ctrl Pts',(42.839207175268,-57.4754524783491,-51.94995));
#238941=CARTESIAN_POINT('Ctrl Pts',(42.839207175268,-58.4389030167283,-51.8916166666667));
#238942=CARTESIAN_POINT('Ctrl Pts',(43.6735798167943,-58.920628285918,-51.8332833333334));
#238943=CARTESIAN_POINT('Ctrl Pts',(44.5079524583205,-59.4023535551075,
-51.77495));
#238944=CARTESIAN_POINT('Ctrl Pts',(45.3423250998467,-58.920628285918,-51.7166166666667));
#238945=CARTESIAN_POINT('Ctrl Pts',(46.1766977413729,-58.4389030167283,
-51.6582833333333));
#238946=CARTESIAN_POINT('Ctrl Pts',(46.1766977413729,-57.4754524783491,
-51.59995));
#238947=CARTESIAN_POINT('Ctrl Pts',(46.1766977413729,-56.5120019399699,
-51.5416166666667));
#238948=CARTESIAN_POINT('Ctrl Pts',(45.3423250998467,-56.0302766707802,
-51.4832833333334));
#238949=CARTESIAN_POINT('Ctrl Pts',(44.5079524583205,-55.5485514015906,
-51.42495));
#238950=CARTESIAN_POINT('Ctrl Pts',(43.6735798167943,-56.0302766707802,
-51.3666166666667));
#238951=CARTESIAN_POINT('Ctrl Pts',(42.839207175268,-56.5120019399698,-51.3082833333333));
#238952=CARTESIAN_POINT('Ctrl Pts',(42.839207175268,-57.4754524783491,-51.24995));
#238953=CARTESIAN_POINT('Origin',(44.5079524583205,-57.4754524783491,-52.920575));
#238954=CARTESIAN_POINT('',(42.839207175268,-57.4754524783491,-52.64995));
#238955=CARTESIAN_POINT('',(42.839207175268,-57.4754524783491,-52.4912));
#238956=CARTESIAN_POINT('',(42.839207175268,-57.4754524783491,-52.920575));
#238957=CARTESIAN_POINT('',(44.2755200796093,-55.8229737314248,-52.64995));
#238958=CARTESIAN_POINT('Origin',(44.5079524583205,-57.4754524783491,-52.64995));
#238959=CARTESIAN_POINT('Ctrl Pts',(44.2755200796093,-55.8229737314248,
-52.64995));
#238960=CARTESIAN_POINT('Ctrl Pts',(43.9544082597716,-55.8681402936311,
-52.6275001713604));
#238961=CARTESIAN_POINT('Ctrl Pts',(43.6735798167943,-56.0302766707802,
-52.6078666666667));
#238962=CARTESIAN_POINT('Ctrl Pts',(42.839207175268,-56.5120019399698,-52.5495333333333));
#238963=CARTESIAN_POINT('Ctrl Pts',(42.839207175268,-57.4754524783491,-52.4912));
#238964=CARTESIAN_POINT('Origin',(44.5079524583206,-57.475452478349,235.35105));
#238965=CARTESIAN_POINT('',(44.5079524583206,-59.475452478349,-51.9662));
#238966=CARTESIAN_POINT('',(44.5079524583206,-59.475452478349,-52.1249500000001));
#238967=CARTESIAN_POINT('',(44.5079524583206,-59.475452478349,235.35105));
#238968=CARTESIAN_POINT('',(46.5079524583206,-57.4754524783491,-52.64995));
#238969=CARTESIAN_POINT('Ctrl Pts',(44.5079524583206,-59.475452478349,-52.1249500000001));
#238970=CARTESIAN_POINT('Ctrl Pts',(44.4513597608212,-59.475452478349,-52.1282512406875));
#238971=CARTESIAN_POINT('Ctrl Pts',(44.3947006314118,-59.4730504845328,
-52.1315563565699));
#238972=CARTESIAN_POINT('Ctrl Pts',(44.08355625845,-59.4465346697816,-52.1497064449927));
#238973=CARTESIAN_POINT('Ctrl Pts',(43.8354437380825,-59.3762551365555,
-52.1641796753474));
#238974=CARTESIAN_POINT('Ctrl Pts',(43.3705215162246,-59.1417508717089,
-52.1913001382892));
#238975=CARTESIAN_POINT('Ctrl Pts',(43.1598519544925,-58.9764452064066,
-52.2051088910806));
#238976=CARTESIAN_POINT('Ctrl Pts',(42.817179172053,-58.5754701885061,-52.2353600294226));
#238977=CARTESIAN_POINT('Ctrl Pts',(42.6876786575065,-58.3445662146524,
-52.2508019690164));
#238978=CARTESIAN_POINT('Ctrl Pts',(42.5279192111384,-57.8544356169778,
-52.2802221098797));
#238979=CARTESIAN_POINT('Ctrl Pts',(42.4958972035575,-57.6009487460923,
-52.2932585493062));
#238980=CARTESIAN_POINT('Ctrl Pts',(42.5288686707642,-57.0835863192722,
-52.3203564090341));
#238981=CARTESIAN_POINT('Ctrl Pts',(42.5982066316955,-56.8249460940721,
-52.3354447915466));
#238982=CARTESIAN_POINT('Ctrl Pts',(42.831006553102,-56.3551743566381,-52.3659667876725));
#238983=CARTESIAN_POINT('Ctrl Pts',(42.9901454516923,-56.1475015012174,
-52.3810995870422));
#238984=CARTESIAN_POINT('Ctrl Pts',(43.3760066384796,-55.8069348406429,
-52.4095586688083));
#238985=CARTESIAN_POINT('Ctrl Pts',(43.5980966363497,-55.6761710812624,
-52.4218750770519));
#238986=CARTESIAN_POINT('Ctrl Pts',(44.0897941185096,-55.5016056305671,
-52.4505574301779));
#238987=CARTESIAN_POINT('Ctrl Pts',(44.3560328624495,-55.4635321991934,
-52.4660880235743));
#238988=CARTESIAN_POINT('Ctrl Pts',(44.8776436126168,-55.493292462122,-52.4965153173341));
#238989=CARTESIAN_POINT('Ctrl Pts',(45.1282784417565,-55.5568947771729,
-52.5111356823672));
#238990=CARTESIAN_POINT('Ctrl Pts',(45.5977717555248,-55.7780117532505,
-52.538522792337));
#238991=CARTESIAN_POINT('Ctrl Pts',(45.8110667164859,-55.9356674403983,
-52.5518370765746));
#238992=CARTESIAN_POINT('Ctrl Pts',(46.1561721894381,-56.31527754973,-52.5810798527649));
#238993=CARTESIAN_POINT('Ctrl Pts',(46.288274338177,-56.530421203333,-52.5958014911562));
#238994=CARTESIAN_POINT('Ctrl Pts',(46.4636467216999,-56.9914153174137,
-52.6242050881466));
#238995=CARTESIAN_POINT('Ctrl Pts',(46.5079524583206,-57.2323982040817,
-52.6376713480658));
#238996=CARTESIAN_POINT('Ctrl Pts',(46.5079524583206,-57.4754524783491,
-52.6499499999999));
#238997=CARTESIAN_POINT('',(44.7865238868913,-59.4559569492311,-52.64995));
#238998=CARTESIAN_POINT('Origin',(44.5079524583206,-57.4754524783489,-52.64995));
#238999=CARTESIAN_POINT('Ctrl Pts',(44.7865238868906,-59.4559569492312,
-52.6499500000001));
#239000=CARTESIAN_POINT('Ctrl Pts',(44.9389460862256,-59.4345177298612,
-52.6410587050389));
#239001=CARTESIAN_POINT('Ctrl Pts',(45.0883897049096,-59.3955549779547,
-52.6323411606156));
#239002=CARTESIAN_POINT('Ctrl Pts',(45.3702837264581,-59.2860937769035,
-52.615897342692));
#239003=CARTESIAN_POINT('Ctrl Pts',(45.5021972948078,-59.217147964577,-52.6085217569117));
#239004=CARTESIAN_POINT('Ctrl Pts',(45.8375272388861,-58.9912737652174,
-52.5873305538517));
#239005=CARTESIAN_POINT('Ctrl Pts',(46.0203348377673,-58.8089227056349,
-52.572786627634));
#239006=CARTESIAN_POINT('Ctrl Pts',(46.3129166430222,-58.3770018942788,
-52.5424331519357));
#239007=CARTESIAN_POINT('Ctrl Pts',(46.4166592650751,-58.1293237884958,
-52.5268950861176));
#239008=CARTESIAN_POINT('Ctrl Pts',(46.5192669221118,-57.6175272330474,
-52.4980473483698));
#239009=CARTESIAN_POINT('Ctrl Pts',(46.5209222271569,-57.3591646298644,
-52.4857036381197));
#239010=CARTESIAN_POINT('Ctrl Pts',(46.4261832933532,-56.8530458580145,
-52.4573722359148));
#239011=CARTESIAN_POINT('Ctrl Pts',(46.3296214606361,-56.6102946503741,
-52.442292507558));
#239012=CARTESIAN_POINT('Ctrl Pts',(46.0459745854273,-56.1697773429461,
-52.4117653549204));
#239013=CARTESIAN_POINT('Ctrl Pts',(45.8595052204716,-55.9775718101498,
-52.3966167974505));
#239014=CARTESIAN_POINT('Ctrl Pts',(45.4322675281872,-55.6838697728091,
-52.3693184149391));
#239015=CARTESIAN_POINT('Ctrl Pts',(45.198236150389,-55.5813380716029,-52.3564665487041));
#239016=CARTESIAN_POINT('Ctrl Pts',(44.69592853734,-55.4671660403481,-52.3271652712762));
#239017=CARTESIAN_POINT('Ctrl Pts',(44.4316978233376,-55.4598310010966,
-52.3117518129594));
#239018=CARTESIAN_POINT('Ctrl Pts',(43.9107199000999,-55.5481767987879,
-52.2813614341039));
#239019=CARTESIAN_POINT('Ctrl Pts',(43.6594962686467,-55.6448427549355,
-52.2672657084199));
#239020=CARTESIAN_POINT('Ctrl Pts',(43.2192767418188,-55.9248207668429,
-52.2402820014233));
#239021=CARTESIAN_POINT('Ctrl Pts',(43.032146377683,-56.1017360044494,-52.2258866022144));
#239022=CARTESIAN_POINT('Ctrl Pts',(42.7287064066549,-56.5243603120291,
-52.1956860721732));
#239023=CARTESIAN_POINT('Ctrl Pts',(42.6184234279488,-56.7683526193353,
-52.1801434456677));
#239024=CARTESIAN_POINT('Ctrl Pts',(42.501183061899,-57.2776111785268,-52.1509971354455));
#239025=CARTESIAN_POINT('Ctrl Pts',(42.492401597098,-57.5372091531185,-52.1385337339152));
#239026=CARTESIAN_POINT('Ctrl Pts',(42.5738454144996,-58.0463118080004,
-52.1104393656924));
#239027=CARTESIAN_POINT('Ctrl Pts',(42.6635991909277,-58.2909179537301,
-52.095464497606));
#239028=CARTESIAN_POINT('Ctrl Pts',(42.9347253230964,-58.7384946609519,
-52.0649459054996));
#239029=CARTESIAN_POINT('Ctrl Pts',(43.1158831362097,-58.9357605337373,
-52.0496966292845));
#239030=CARTESIAN_POINT('Ctrl Pts',(43.5351370959696,-59.241203804816,-52.0220379602483));
#239031=CARTESIAN_POINT('Ctrl Pts',(43.7664919850463,-59.3501535032036,
-52.0094518609408));
#239032=CARTESIAN_POINT('Ctrl Pts',(44.1744699518852,-59.4545645545293,
-51.9856531462085));
#239033=CARTESIAN_POINT('Ctrl Pts',(44.3410712893685,-59.475452478349,-51.9759347348555));
#239034=CARTESIAN_POINT('Ctrl Pts',(44.5079524583206,-59.475452478349,-51.9662));
#239035=CARTESIAN_POINT('Origin',(44.5079524583206,-57.475452478349,235.35105));
#239036=CARTESIAN_POINT('',(44.5079524583206,-59.475452478349,-51.2662));
#239037=CARTESIAN_POINT('',(44.5079524583206,-59.475452478349,-51.4249500000001));
#239038=CARTESIAN_POINT('',(44.5079524583206,-59.475452478349,235.35105));
#239039=CARTESIAN_POINT('Ctrl Pts',(44.5079524583206,-59.475452478349,-51.4249500000001));
#239040=CARTESIAN_POINT('Ctrl Pts',(44.4125121220936,-59.475452478349,-51.4305173529467));
#239041=CARTESIAN_POINT('Ctrl Pts',(44.3169826779063,-59.4686210091442,
-51.4360899038576));
#239042=CARTESIAN_POINT('Ctrl Pts',(43.9706471848928,-59.4186073047783,
-51.4562928076168));
#239043=CARTESIAN_POINT('Ctrl Pts',(43.7283528405609,-59.3347051059968,
-51.4704266443695));
#239044=CARTESIAN_POINT('Ctrl Pts',(43.2787639257411,-59.0752295338068,
-51.4966526644006));
#239045=CARTESIAN_POINT('Ctrl Pts',(43.0777780687277,-58.8984478296677,
-51.5114429958136));
#239046=CARTESIAN_POINT('Ctrl Pts',(42.759033675885,-58.4800868047618,-51.541874531677));
#239047=CARTESIAN_POINT('Ctrl Pts',(42.6430709224838,-58.2437201427654,
-51.5571975847951));
#239048=CARTESIAN_POINT('Ctrl Pts',(42.5102536931264,-57.7466673953907,
-51.5861816051825));
#239049=CARTESIAN_POINT('Ctrl Pts',(42.4919941938421,-57.4914112410099,
-51.5986783434767));
#239050=CARTESIAN_POINT('Ctrl Pts',(42.5532078057466,-56.9761171215888,
-51.6264954453646));
#239051=CARTESIAN_POINT('Ctrl Pts',(42.6365867942621,-56.7215841050276,
-51.6417858692722));
#239052=CARTESIAN_POINT('Ctrl Pts',(42.8940849597355,-56.2663628040766,
-51.6722931697382));
#239053=CARTESIAN_POINT('Ctrl Pts',(43.0632307042696,-56.0685855867604,
-51.6872179261321));
#239054=CARTESIAN_POINT('Ctrl Pts',(43.4675083927591,-55.7480011186832,
-51.7152046924955));
#239055=CARTESIAN_POINT('Ctrl Pts',(43.6988294193687,-55.6283087693928,
-51.7277511560613));
#239056=CARTESIAN_POINT('Ctrl Pts',(44.2007382506901,-55.481523908706,-51.7570291712216));
#239057=CARTESIAN_POINT('Ctrl Pts',(44.4671516575844,-55.4584121001176,
-51.7725699532905));
#239058=CARTESIAN_POINT('Ctrl Pts',(44.9835717875786,-55.5161840363474,
-51.8026944608734));
#239059=CARTESIAN_POINT('Ctrl Pts',(45.2291480546249,-55.592670444065,-51.8170197431178));
#239060=CARTESIAN_POINT('Ctrl Pts',(45.6896505047163,-55.8398316248472,
-51.8438823860397));
#239061=CARTESIAN_POINT('Ctrl Pts',(45.8977889023861,-56.0125434124774,
-51.8582501054411));
#239062=CARTESIAN_POINT('Ctrl Pts',(46.2297443679366,-56.4248361486605,
-51.8887604055473));
#239063=CARTESIAN_POINT('Ctrl Pts',(46.3522042551334,-56.6586879284254,
-51.904145911207));
#239064=CARTESIAN_POINT('Ctrl Pts',(46.497899504113,-57.1524868272325,-51.9333411620947));
#239065=CARTESIAN_POINT('Ctrl Pts',(46.522763526501,-57.4068532858747,-51.9460525063153));
#239066=CARTESIAN_POINT('Ctrl Pts',(46.4751481959428,-57.9232136644451,
-51.973526857102));
#239067=CARTESIAN_POINT('Ctrl Pts',(46.3985005787866,-58.1798226132569,
-51.9887258215988));
#239068=CARTESIAN_POINT('Ctrl Pts',(46.1527842050746,-58.6422140890608,
-52.0192517104303));
#239069=CARTESIAN_POINT('Ctrl Pts',(45.9883831911795,-58.8448152691331,
-52.0342817765143));
#239070=CARTESIAN_POINT('Ctrl Pts',(45.5929487775531,-59.1750614020357,
-52.0624987034466));
#239071=CARTESIAN_POINT('Ctrl Pts',(45.3661383698148,-59.3001188717699,
-52.074889155163));
#239072=CARTESIAN_POINT('Ctrl Pts',(44.923153957511,-59.4429862119282,-52.1007299125474));
#239073=CARTESIAN_POINT('Ctrl Pts',(44.7160021186349,-59.475452478349,-52.1128137698151));
#239074=CARTESIAN_POINT('Ctrl Pts',(44.5079524583206,-59.475452478349,-52.1249500000001));
#239075=CARTESIAN_POINT('Ctrl Pts',(44.5079524583206,-59.475452478349,-51.9662));
#239076=CARTESIAN_POINT('Ctrl Pts',(44.6010399043629,-59.475452478349,-51.9607698989808));
#239077=CARTESIAN_POINT('Ctrl Pts',(44.6942144195173,-59.4689536852591,
-51.95533471893));
#239078=CARTESIAN_POINT('Ctrl Pts',(45.0493950081076,-59.4189460111751,
-51.9346158512622));
#239079=CARTESIAN_POINT('Ctrl Pts',(45.3019367943206,-59.3301253082591,
-51.9200700944071));
#239080=CARTESIAN_POINT('Ctrl Pts',(45.7484928539025,-59.064733753287,-51.8936384526703));
#239081=CARTESIAN_POINT('Ctrl Pts',(45.9403960211653,-58.8941892509691,
-51.8794256844553));
#239082=CARTESIAN_POINT('Ctrl Pts',(46.255965041182,-58.4825757154018,-51.8494276343015));
#239083=CARTESIAN_POINT('Ctrl Pts',(46.3736136173997,-58.2430235310882,
-51.8338944846615));
#239084=CARTESIAN_POINT('Ctrl Pts',(46.5076698892025,-57.7368972946749,
-51.804415949669));
#239085=CARTESIAN_POINT('Ctrl Pts',(46.5246850365527,-57.4758015300995,
-51.7917056669799));
#239086=CARTESIAN_POINT('Ctrl Pts',(46.4583579434643,-56.9634209222726,
-51.7638866071024));
#239087=CARTESIAN_POINT('Ctrl Pts',(46.3763441180367,-56.7169416968142,
-51.7490428630669));
#239088=CARTESIAN_POINT('Ctrl Pts',(46.118436752915,-56.2597477670313,-51.7184239740547));
#239089=CARTESIAN_POINT('Ctrl Pts',(45.9415108526329,-56.0554026569323,
-51.7029404986682));
#239090=CARTESIAN_POINT('Ctrl Pts',(45.5285249192671,-55.7367954676129,
-51.6747996302913));
#239091=CARTESIAN_POINT('Ctrl Pts',(45.2997732220664,-55.6213955602625,
-51.6623895445518));
#239092=CARTESIAN_POINT('Ctrl Pts',(44.8050242006444,-55.4805673939303,
-51.6335291849689));
#239093=CARTESIAN_POINT('Ctrl Pts',(44.5430377637212,-55.458877813189,-51.618246642815));
#239094=CARTESIAN_POINT('Ctrl Pts',(44.0209071528755,-55.5176399327209,
-51.5877890238489));
#239095=CARTESIAN_POINT('Ctrl Pts',(43.7659873176074,-55.5993442682777,
-51.572918700125));
#239096=CARTESIAN_POINT('Ctrl Pts',(43.3127992584962,-55.8518887331076,
-51.5464827300101));
#239097=CARTESIAN_POINT('Ctrl Pts',(43.1166320578916,-56.0164558665738,
-51.5326589625609));
#239098=CARTESIAN_POINT('Ctrl Pts',(42.7901543316252,-56.4178094217715,
-51.5028610570206));
#239099=CARTESIAN_POINT('Ctrl Pts',(42.6658936469586,-56.6530990885663,
-51.4873503887108));
#239100=CARTESIAN_POINT('Ctrl Pts',(42.5163972629145,-57.156136564909,-51.4575775555513));
#239101=CARTESIAN_POINT('Ctrl Pts',(42.491766179016,-57.4186699581944,-51.4445406476013));
#239102=CARTESIAN_POINT('Ctrl Pts',(42.5443566356938,-57.9339246682677,
-51.4169770452948));
#239103=CARTESIAN_POINT('Ctrl Pts',(42.6193506557171,-58.1818892358007,
-51.402263008852));
#239104=CARTESIAN_POINT('Ctrl Pts',(42.8636498665352,-58.6448327446183,
-51.3717505662526));
#239105=CARTESIAN_POINT('Ctrl Pts',(43.0341453932076,-58.8535317255553,
-51.3562346939359));
#239106=CARTESIAN_POINT('Ctrl Pts',(43.4376533039693,-59.1840656215097,
-51.3277677527474));
#239107=CARTESIAN_POINT('Ctrl Pts',(43.6637183498251,-59.3063463516232,
-51.3154469896621));
#239108=CARTESIAN_POINT('Ctrl Pts',(44.1015387374648,-59.4443516292416,
-51.2899074670498));
#239109=CARTESIAN_POINT('Ctrl Pts',(44.3043239750094,-59.475452478349,-51.2780783281931));
#239110=CARTESIAN_POINT('Ctrl Pts',(44.5079524583206,-59.475452478349,-51.2662));
#239111=CARTESIAN_POINT('Origin',(44.5079524583206,-57.475452478349,235.35105));
#239112=CARTESIAN_POINT('',(44.5079524583206,-59.475452478349,-50.5661999999999));
#239113=CARTESIAN_POINT('',(44.5079524583206,-59.475452478349,-50.7249500000001));
#239114=CARTESIAN_POINT('',(44.5079524583206,-59.475452478349,235.35105));
#239115=CARTESIAN_POINT('Ctrl Pts',(44.5079524583206,-59.475452478349,-50.7249500000001));
#239116=CARTESIAN_POINT('Ctrl Pts',(44.3732303097234,-59.475452478349,-50.7328087920016));
#239117=CARTESIAN_POINT('Ctrl Pts',(44.2385286748256,-59.4618398691135,
-50.7406663873707));
#239118=CARTESIAN_POINT('Ctrl Pts',(43.8577756421695,-59.3837085760508,
-50.7628769809423));
#239119=CARTESIAN_POINT('Ctrl Pts',(43.6216198460632,-59.2861254963707,
-50.775996186017));
#239120=CARTESIAN_POINT('Ctrl Pts',(43.1883124452698,-59.0015185944403,
-50.8030121322914));
#239121=CARTESIAN_POINT('Ctrl Pts',(42.9978490958847,-58.8133128673102,
-50.818075118197));
#239122=CARTESIAN_POINT('Ctrl Pts',(42.7046785832125,-58.37847689791,-50.8485930329154));
#239123=CARTESIAN_POINT('Ctrl Pts',(42.6028931943792,-58.1372827567734,
-50.8637464548754));
#239124=CARTESIAN_POINT('Ctrl Pts',(42.4979397582136,-57.6335177550656,
-50.8922568719562));
#239125=CARTESIAN_POINT('Ctrl Pts',(42.4941863971064,-57.3760557321509,
-50.9045698294716));
#239126=CARTESIAN_POINT('Ctrl Pts',(42.5856552766182,-56.8624355105712,
-50.9331848144449));
#239127=CARTESIAN_POINT('Ctrl Pts',(42.6843423686,-56.6120658856088,-50.9487113978683));
#239128=CARTESIAN_POINT('Ctrl Pts',(42.9684772538217,-56.173253814368,-50.9791666387562));
#239129=CARTESIAN_POINT('Ctrl Pts',(43.1478916112811,-55.9868366474121,
-50.9938170076487));
#239130=CARTESIAN_POINT('Ctrl Pts',(43.5721456417778,-55.6885491944948,
-51.0212600133965));
#239131=CARTESIAN_POINT('Ctrl Pts',(43.8142157450224,-55.581378245293,-51.0344820250577));
#239132=CARTESIAN_POINT('Ctrl Pts',(44.3269083595648,-55.4663537302885,
-51.0643890942393));
#239133=CARTESIAN_POINT('Ctrl Pts',(44.5925476488824,-55.4599886933024,
-51.0798847194495));
#239134=CARTESIAN_POINT('Ctrl Pts',(45.1016271919251,-55.5488304120265,
-51.109581026127));
#239135=CARTESIAN_POINT('Ctrl Pts',(45.3408222305017,-55.6395404222803,
-51.123161823708));
#239136=CARTESIAN_POINT('Ctrl Pts',(45.7824273092984,-55.911477008505,-51.1497797046997));
#239137=CARTESIAN_POINT('Ctrl Pts',(45.9782761977746,-56.0940024364279,
-51.1647128106296));
#239138=CARTESIAN_POINT('Ctrl Pts',(46.2844488827478,-56.520626893157,-51.1951951249564));
#239139=CARTESIAN_POINT('Ctrl Pts',(46.3934319368649,-56.7594815185977,
-51.210440290819));
#239140=CARTESIAN_POINT('Ctrl Pts',(46.5124987741093,-57.2599016385867,
-51.2391933715331));
#239141=CARTESIAN_POINT('Ctrl Pts',(46.523640990306,-57.5161983286478,-51.2515508227354));
#239142=CARTESIAN_POINT('Ctrl Pts',(46.4474139510621,-58.0321656305446,
-51.2798398241863));
#239143=CARTESIAN_POINT('Ctrl Pts',(46.3557443156348,-58.2860537421219,
-51.2953394792231));
#239144=CARTESIAN_POINT('Ctrl Pts',(46.0834084997015,-58.7340244154266,
-51.3259132562097));
#239145=CARTESIAN_POINT('Ctrl Pts',(45.9087756930046,-58.9258982429212,
-51.3406998235928));
#239146=CARTESIAN_POINT('Ctrl Pts',(45.4939813497915,-59.2348269490163,
-51.3684044982037));
#239147=CARTESIAN_POINT('Ctrl Pts',(45.2570989143405,-59.3480036986934,
-51.3812497900656));
#239148=CARTESIAN_POINT('Ctrl Pts',(44.8423276786983,-59.4544534084242,
-51.4054447788114));
#239149=CARTESIAN_POINT('Ctrl Pts',(44.6752770121716,-59.475452478349,-51.4151894010254));
#239150=CARTESIAN_POINT('Ctrl Pts',(44.5079524583206,-59.475452478349,-51.4249500000001));
#239151=CARTESIAN_POINT('Ctrl Pts',(44.5079524583206,-59.475452478349,-51.2662));
#239152=CARTESIAN_POINT('Ctrl Pts',(44.5631734525969,-59.475452478349,-51.2629787753339));
#239153=CARTESIAN_POINT('Ctrl Pts',(44.6184564602758,-59.4731655085845,
-51.2597539332191));
#239154=CARTESIAN_POINT('Ctrl Pts',(44.9378351352537,-59.446612498114,-51.2411235105121));
#239155=CARTESIAN_POINT('Ctrl Pts',(45.1950710343904,-59.3723409740258,
-51.2261180830625));
#239156=CARTESIAN_POINT('Ctrl Pts',(45.6551086957666,-59.1332196616792,
-51.1992825528155));
#239157=CARTESIAN_POINT('Ctrl Pts',(45.8556719818888,-58.9747430339204,
-51.1859662302413));
#239158=CARTESIAN_POINT('Ctrl Pts',(46.1931091254407,-58.5841781606304,
-51.1563936992655));
#239159=CARTESIAN_POINT('Ctrl Pts',(46.3240269851495,-58.3534617183551,
-51.1409198941859));
#239160=CARTESIAN_POINT('Ctrl Pts',(46.489441262139,-57.8538322926681,-51.1108549575582));
#239161=CARTESIAN_POINT('Ctrl Pts',(46.5219935519418,-57.5897667474203,
-51.097384477124));
#239162=CARTESIAN_POINT('Ctrl Pts',(46.4834312978279,-57.071679273164,-51.0700869247239));
#239163=CARTESIAN_POINT('Ctrl Pts',(46.4155803416157,-56.8224088306493,
-51.055515257256));
#239164=CARTESIAN_POINT('Ctrl Pts',(46.1852071369206,-56.3540332941882,
-51.0251345738557));
#239165=CARTESIAN_POINT('Ctrl Pts',(46.0213365265818,-56.1411151227246,
-51.0095987825716));
#239166=CARTESIAN_POINT('Ctrl Pts',(45.6275782266816,-55.7985834749711,
-50.9808101008255));
#239167=CARTESIAN_POINT('Ctrl Pts',(45.404166960123,-55.6692822412727,-50.9684791792718));
#239168=CARTESIAN_POINT('Ctrl Pts',(44.9177003933257,-55.5008196290297,
-50.9401019628753));
#239169=CARTESIAN_POINT('Ctrl Pts',(44.6588591761761,-55.4644147596997,
-50.9250028918749));
#239170=CARTESIAN_POINT('Ctrl Pts',(44.1355544264234,-55.4926223906537,
-50.8944767814726));
#239171=CARTESIAN_POINT('Ctrl Pts',(43.8762269335403,-55.5593990126897,
-50.8793493443878));
#239172=CARTESIAN_POINT('Ctrl Pts',(43.4094799788231,-55.7850452420739,
-50.8521224386959));
#239173=CARTESIAN_POINT('Ctrl Pts',(43.2044916462832,-55.9375494374975,
-50.839207740595));
#239174=CARTESIAN_POINT('Ctrl Pts',(42.8564006042176,-56.3174372521513,
-50.8098638561468));
#239175=CARTESIAN_POINT('Ctrl Pts',(42.7190873096172,-56.5434758284824,
-50.7944398346762));
#239176=CARTESIAN_POINT('Ctrl Pts',(42.537984808442,-57.0395134538714,-50.7640987759441));
#239177=CARTESIAN_POINT('Ctrl Pts',(42.4975442940095,-57.3051259012254,
-50.7501081547847));
#239178=CARTESIAN_POINT('Ctrl Pts',(42.5224030777523,-57.8258803250107,
-50.7230755575846));
#239179=CARTESIAN_POINT('Ctrl Pts',(42.5833128086047,-58.0762232854203,
-50.7086521609046));
#239180=CARTESIAN_POINT('Ctrl Pts',(42.8000779364503,-58.5494773740377,
-50.6784219243232));
#239181=CARTESIAN_POINT('Ctrl Pts',(42.9574327018484,-58.7662939090198,
-50.6628792404092));
#239182=CARTESIAN_POINT('Ctrl Pts',(43.3416010318863,-59.1203694379146,
-50.633787090615));
#239183=CARTESIAN_POINT('Ctrl Pts',(43.5624832180562,-59.2565226192977,
-50.6213523723485));
#239184=CARTESIAN_POINT('Ctrl Pts',(44.0285820716791,-59.4320414521156,
-50.5941632725539));
#239185=CARTESIAN_POINT('Ctrl Pts',(44.2673731131723,-59.475452478349,-50.5802337951336));
#239186=CARTESIAN_POINT('Ctrl Pts',(44.5079524583206,-59.475452478349,-50.5661999999999));
#239187=CARTESIAN_POINT('Origin',(44.5079524583206,-57.475452478349,235.35105));
#239188=CARTESIAN_POINT('',(44.5079524583206,-59.475452478349,-49.8662));
#239189=CARTESIAN_POINT('',(44.5079524583206,-59.475452478349,-50.02495));
#239190=CARTESIAN_POINT('',(44.5079524583206,-59.475452478349,235.35105));
#239191=CARTESIAN_POINT('Ctrl Pts',(44.5079524583206,-59.475452478349,-50.02495));
#239192=CARTESIAN_POINT('Ctrl Pts',(44.3365369173601,-59.475452478349,-50.0349492398894));
#239193=CARTESIAN_POINT('Ctrl Pts',(44.165453694393,-59.4534139082329,-50.0449290945625));
#239194=CARTESIAN_POINT('Ctrl Pts',(43.7537132796872,-59.3450617430205,
-50.0689472854204));
#239195=CARTESIAN_POINT('Ctrl Pts',(43.5230214878811,-59.2344889054372,
-50.0814805564355));
#239196=CARTESIAN_POINT('Ctrl Pts',(43.1058057632521,-58.9260884222208,
-50.1092291698292));
#239197=CARTESIAN_POINT('Ctrl Pts',(42.9260130342561,-58.7275672179406,
-50.1245020481139));
#239198=CARTESIAN_POINT('Ctrl Pts',(42.6580795457638,-58.2782626921982,
-50.1550148076391));
#239199=CARTESIAN_POINT('Ctrl Pts',(42.5700513130442,-58.0332173811712,
-50.169961533185));
#239200=CARTESIAN_POINT('Ctrl Pts',(42.4919764703888,-57.5233736810765,
-50.1979950758765));
#239201=CARTESIAN_POINT('Ctrl Pts',(42.5025803167883,-57.2634501512911,
-50.2105032775909));
#239202=CARTESIAN_POINT('Ctrl Pts',(42.623552088484,-56.7548663782633,-50.23972433153));
#239203=CARTESIAN_POINT('Ctrl Pts',(42.7354837407372,-56.5118407088338,
-50.2552662115914));
#239204=CARTESIAN_POINT('Ctrl Pts',(43.0416479502191,-56.0916300652184,
-50.2854242647528));
#239205=CARTESIAN_POINT('Ctrl Pts',(43.2298556124923,-55.9161173897087,
-50.2997802303169));
#239206=CARTESIAN_POINT('Ctrl Pts',(43.6723837433044,-55.6388246208237,
-50.3266956180905));
#239207=CARTESIAN_POINT('Ctrl Pts',(43.9249719861093,-55.5437209148654,
-50.3409428057877));
#239208=CARTESIAN_POINT('Ctrl Pts',(44.4471166845182,-55.45933233961,-50.3714012465282));
#239209=CARTESIAN_POINT('Ctrl Pts',(44.7110823320703,-55.4686675746012,
-50.3867992426354));
#239210=CARTESIAN_POINT('Ctrl Pts',(45.212365768875,-55.5865430738959,-50.416040776449));
#239211=CARTESIAN_POINT('Ctrl Pts',(45.4456545898622,-55.6908343352178,
-50.4288107077029));
#239212=CARTESIAN_POINT('Ctrl Pts',(45.8707157277807,-55.987762283461,-50.4562085744247));
#239213=CARTESIAN_POINT('Ctrl Pts',(46.055743094387,-56.1813700172138,-50.4713859102056));
#239214=CARTESIAN_POINT('Ctrl Pts',(46.3359749373623,-56.6238582150205,
-50.5019130234693));
#239215=CARTESIAN_POINT('Ctrl Pts',(46.4306733023535,-56.8671366434277,
-50.5169650349012));
#239216=CARTESIAN_POINT('Ctrl Pts',(46.5217720057947,-57.3740819004816,
-50.5452320162229));
#239217=CARTESIAN_POINT('Ctrl Pts',(46.5181755725226,-57.6327747083439,
-50.5575994536215));
#239218=CARTESIAN_POINT('Ctrl Pts',(46.4115762574803,-58.1438957866815,
-50.5865294908748));
#239219=CARTESIAN_POINT('Ctrl Pts',(46.3060378820656,-58.3905851910932,
-50.6020699854699));
#239220=CARTESIAN_POINT('Ctrl Pts',(46.010466834972,-58.8199970849343,-50.6323839015208));
#239221=CARTESIAN_POINT('Ctrl Pts',(45.8264646834458,-59.0008757128014,
-50.6468882843332));
#239222=CARTESIAN_POINT('Ctrl Pts',(45.3928328266298,-59.2884630472197,
-50.6740642598394));
#239223=CARTESIAN_POINT('Ctrl Pts',(45.1454464338896,-59.3895244960639,
-50.6877628514252));
#239224=CARTESIAN_POINT('Ctrl Pts',(44.7607754026071,-59.463469340792,-50.7102019949167));
#239225=CARTESIAN_POINT('Ctrl Pts',(44.6343549013126,-59.475452478349,-50.7175765241589));
#239226=CARTESIAN_POINT('Ctrl Pts',(44.5079524583206,-59.475452478349,-50.7249500000001));
#239227=CARTESIAN_POINT('Ctrl Pts',(44.5079524583206,-59.475452478349,-50.5661999999999));
#239228=CARTESIAN_POINT('Ctrl Pts',(44.525311884392,-59.475452478349,-50.5651873668124));
#239229=CARTESIAN_POINT('Ctrl Pts',(44.5426806214417,-59.475226466934,-50.5641741904845));
#239230=CARTESIAN_POINT('Ctrl Pts',(44.8251356375188,-59.4678657513322,
-50.54769764788));
#239231=CARTESIAN_POINT('Ctrl Pts',(45.0862516346071,-59.4083063571444,
-50.5324658813832));
#239232=CARTESIAN_POINT('Ctrl Pts',(45.5592819807103,-59.1956042615348,
-50.5048724445272));
#239233=CARTESIAN_POINT('Ctrl Pts',(45.7685389612303,-59.0487165462796,
-50.492244614897));
#239234=CARTESIAN_POINT('Ctrl Pts',(46.1265531213234,-58.678938656933,-50.4631220408816));
#239235=CARTESIAN_POINT('Ctrl Pts',(46.2697412585774,-58.4574600281666,
-50.4477570299421));
#239236=CARTESIAN_POINT('Ctrl Pts',(46.4643314628618,-57.9683157718007,
-50.4173708201097));
#239237=CARTESIAN_POINT('Ctrl Pts',(46.5123410384248,-57.7049341357576,
-50.4029209887124));
#239238=CARTESIAN_POINT('Ctrl Pts',(46.5031187675918,-57.1853964236243,
-50.3764059224922));
#239239=CARTESIAN_POINT('Ctrl Pts',(46.4500350089897,-56.9340744031033,
-50.362161323032));
#239240=CARTESIAN_POINT('Ctrl Pts',(46.2487011790163,-56.4557885441269,
-50.3321269702494));
#239241=CARTESIAN_POINT('Ctrl Pts',(46.098784427892,-56.2348127537926,-50.3165911105387));
#239242=CARTESIAN_POINT('Ctrl Pts',(45.7255955579612,-55.8678474518023,
-50.2871680275256));
#239243=CARTESIAN_POINT('Ctrl Pts',(45.5075123815212,-55.7239053571838,
-50.2745076621868));
#239244=CARTESIAN_POINT('Ctrl Pts',(45.0298108081354,-55.5276363640678,
-50.2466417370726));
#239245=CARTESIAN_POINT('Ctrl Pts',(44.774952613007,-55.47670198901,-50.2317750090234));
#239246=CARTESIAN_POINT('Ctrl Pts',(44.24976174175,-55.4741995360601,-50.2011388748668));
#239247=CARTESIAN_POINT('Ctrl Pts',(43.9844582170926,-55.5266928550564,
-50.1856628359284));
#239248=CARTESIAN_POINT('Ctrl Pts',(43.5031011930694,-55.727679343834,-50.1575836761937));
#239249=CARTESIAN_POINT('Ctrl Pts',(43.2896387143397,-55.8691645288258,
-50.1451458757219));
#239250=CARTESIAN_POINT('Ctrl Pts',(42.9221793307712,-56.2291728948758,
-50.1162413542509));
#239251=CARTESIAN_POINT('Ctrl Pts',(42.7734849989007,-56.4461328238379,
-50.1009440223164));
#239252=CARTESIAN_POINT('Ctrl Pts',(42.5658980022833,-56.9289527302484,
-50.0704982338248));
#239253=CARTESIAN_POINT('Ctrl Pts',(42.5106289671819,-57.1908680016921,
-50.0556547457096));
#239254=CARTESIAN_POINT('Ctrl Pts',(42.5055760603303,-57.7097431108916,
-50.0292947594122));
#239255=CARTESIAN_POINT('Ctrl Pts',(42.5514272695259,-57.9617785134588,
-50.0153636937856));
#239256=CARTESIAN_POINT('Ctrl Pts',(42.7385849251039,-58.4443986727495,
-49.9855238519291));
#239257=CARTESIAN_POINT('Ctrl Pts',(42.8815947303821,-58.6689709161487,
-49.9700077586553));
#239258=CARTESIAN_POINT('Ctrl Pts',(43.2445353236585,-59.0476544253552,
-49.9402916015783));
#239259=CARTESIAN_POINT('Ctrl Pts',(43.4600800296516,-59.1988167030237,
-49.9273258916723));
#239260=CARTESIAN_POINT('Ctrl Pts',(43.9334581156285,-59.4083078449751,
-49.8997121699903));
#239261=CARTESIAN_POINT('Ctrl Pts',(44.1861447161658,-59.4660248765132,
-49.8849721182923));
#239262=CARTESIAN_POINT('Ctrl Pts',(44.4645221691663,-59.4750990564982,
-49.8687334335339));
#239263=CARTESIAN_POINT('Ctrl Pts',(44.4862445813218,-59.475452478349,-49.8674662928249));
#239264=CARTESIAN_POINT('Ctrl Pts',(44.5079524583206,-59.475452478349,-49.8662));
#239265=CARTESIAN_POINT('Origin',(44.5079524583206,-57.475452478349,235.35105));
#239266=CARTESIAN_POINT('',(44.5079524583206,-59.475452478349,-49.1662));
#239267=CARTESIAN_POINT('',(44.5079524583206,-59.475452478349,-49.3249500000001));
#239268=CARTESIAN_POINT('',(44.5079524583206,-59.475452478349,235.35105));
#239269=CARTESIAN_POINT('Ctrl Pts',(44.5079524583206,-59.475452478349,-49.3249500000001));
#239270=CARTESIAN_POINT('Ctrl Pts',(44.2993850363199,-59.475452478349,-49.3371164329501));
#239271=CARTESIAN_POINT('Ctrl Pts',(44.0917630202625,-59.4428246129822,
-49.3492277172203));
#239272=CARTESIAN_POINT('Ctrl Pts',(43.6500545683669,-59.300019158842,-49.3749940435809));
#239273=CARTESIAN_POINT('Ctrl Pts',(43.4246875255532,-59.1759130933234,
-49.387307771915));
#239274=CARTESIAN_POINT('Ctrl Pts',(43.0237071573202,-58.8422425206466,
-49.4158594522137));
#239275=CARTESIAN_POINT('Ctrl Pts',(42.8549286887907,-58.6324245804788,
-49.4313817714165));
#239276=CARTESIAN_POINT('Ctrl Pts',(42.6142478061451,-58.1680262740998,
-49.4618621731236));
#239277=CARTESIAN_POINT('Ctrl Pts',(42.5411136494647,-57.9197018279802,
-49.4765401439522));
#239278=CARTESIAN_POINT('Ctrl Pts',(42.4921699010616,-57.4037007753935,
-49.5040350877759));
#239279=CARTESIAN_POINT('Ctrl Pts',(42.518845738177,-57.1407748289753,-49.5171750158715));
#239280=CARTESIAN_POINT('Ctrl Pts',(42.6724657743842,-56.6385980063255,
-49.547024643588));
#239281=CARTESIAN_POINT('Ctrl Pts',(42.7984669024605,-56.4044759374015,
-49.5625270899479));
#239282=CARTESIAN_POINT('Ctrl Pts',(43.1277988610394,-56.0059129337578,
-49.5922672704326));
#239283=CARTESIAN_POINT('Ctrl Pts',(43.3250966049773,-55.842927230864,-49.6059500752218));
#239284=CARTESIAN_POINT('Ctrl Pts',(43.7800628312528,-55.5938368428163,
-49.6324897717545));
#239285=CARTESIAN_POINT('Ctrl Pts',(44.0356007460214,-55.5140411370886,
-49.6473961501161));
#239286=CARTESIAN_POINT('Ctrl Pts',(44.5579835976218,-55.45921768084,-49.6778684831261));
#239287=CARTESIAN_POINT('Ctrl Pts',(44.8196105601658,-55.4828185316031,
-49.6931300559411));
#239288=CARTESIAN_POINT('Ctrl Pts',(45.3133155785361,-55.6272140610877,
-49.7219295153461));
#239289=CARTESIAN_POINT('Ctrl Pts',(45.5413713246016,-55.7443743383945,
-49.7343071876337));
#239290=CARTESIAN_POINT('Ctrl Pts',(45.9519402281426,-56.0660476571897,
-49.7625324544917));
#239291=CARTESIAN_POINT('Ctrl Pts',(46.1272280173218,-56.2715267988392,
-49.7780254408121));
#239292=CARTESIAN_POINT('Ctrl Pts',(46.3816599958988,-56.7302313335169,
-49.8086192773458));
#239293=CARTESIAN_POINT('Ctrl Pts',(46.4618772342432,-56.9771099115252,
-49.8234307954762));
#239294=CARTESIAN_POINT('Ctrl Pts',(46.5246920778563,-57.4902348273388,
-49.8511850158054));
#239295=CARTESIAN_POINT('Ctrl Pts',(46.5057422852615,-57.7516916526499,
-49.8639695550248));
#239296=CARTESIAN_POINT('Ctrl Pts',(46.3677524162161,-58.2570507134512,
-49.8935240636454));
#239297=CARTESIAN_POINT('Ctrl Pts',(46.2484052535005,-58.4955335504917,
-49.9090527339471));
#239298=CARTESIAN_POINT('Ctrl Pts',(45.9300547456721,-58.9045229115213,
-49.9389993423897));
#239299=CARTESIAN_POINT('Ctrl Pts',(45.7370659118431,-59.0735591688394,
-49.9531675821346));
#239300=CARTESIAN_POINT('Ctrl Pts',(45.2888264544129,-59.3356783731931,
-49.9794830098808));
#239301=CARTESIAN_POINT('Ctrl Pts',(45.0356851522591,-59.4227115455241,
-49.9941655928536));
#239302=CARTESIAN_POINT('Ctrl Pts',(44.6848476516991,-59.4695912588368,
-50.0146311137196));
#239303=CARTESIAN_POINT('Ctrl Pts',(44.5963558612004,-59.475452478349,-50.0197931348321));
#239304=CARTESIAN_POINT('Ctrl Pts',(44.5079524583206,-59.475452478349,-50.0249500000001));
#239305=CARTESIAN_POINT('Ctrl Pts',(44.5079524583206,-59.475452478349,-49.8662));
#239306=CARTESIAN_POINT('Ctrl Pts',(44.7527989264331,-59.475452478349,-49.8519172893601));
#239307=CARTESIAN_POINT('Ctrl Pts',(44.99579624215,-59.4304871657721,-49.8377424459432));
#239308=CARTESIAN_POINT('Ctrl Pts',(45.4624274771203,-59.2513430521657,
-49.81052229057));
#239309=CARTESIAN_POINT('Ctrl Pts',(45.6804567563558,-59.1155893798232,
-49.798191970945));
#239310=CARTESIAN_POINT('Ctrl Pts',(46.0578148199063,-58.765972037735,-49.7695236732668));
#239311=CARTESIAN_POINT('Ctrl Pts',(46.2121774971817,-58.5539299471189,
-49.7543094546795));
#239312=CARTESIAN_POINT('Ctrl Pts',(46.4333807998448,-58.0779402599982,
-49.723811573961));
#239313=CARTESIAN_POINT('Ctrl Pts',(46.4962158545024,-57.8176838117814,
-49.7088312109536));
#239314=CARTESIAN_POINT('Ctrl Pts',(46.516246592131,-57.2995570505814,-49.682072176414));
#239315=CARTESIAN_POINT('Ctrl Pts',(46.4778484030692,-57.0467794036011,
-49.668666194984));
#239316=CARTESIAN_POINT('Ctrl Pts',(46.3054863165889,-56.5600418323204,
-49.6390498865289));
#239317=CARTESIAN_POINT('Ctrl Pts',(46.1697347144584,-56.3319549329881,
-49.6235679369362));
#239318=CARTESIAN_POINT('Ctrl Pts',(45.8176406644073,-55.9411966105091,
-49.5935581401593));
#239319=CARTESIAN_POINT('Ctrl Pts',(45.604723775311,-55.7824431043697,-49.5801783268244));
#239320=CARTESIAN_POINT('Ctrl Pts',(45.1358868263273,-55.5593847398029,
-49.5528295048004));
#239321=CARTESIAN_POINT('Ctrl Pts',(44.8856073119475,-55.4948072943955,
-49.5382298664615));
#239322=CARTESIAN_POINT('Ctrl Pts',(44.3643334885523,-55.4629374060242,
-49.5078222267634));
#239323=CARTESIAN_POINT('Ctrl Pts',(44.0980535099889,-55.4998891566375,
-49.4922892280139));
#239324=CARTESIAN_POINT('Ctrl Pts',(43.6055726841607,-55.6723868202004,
-49.4635611798405));
#239325=CARTESIAN_POINT('Ctrl Pts',(43.3828003792474,-55.8023211373756,
-49.4512398953274));
#239326=CARTESIAN_POINT('Ctrl Pts',(42.9955369778988,-56.1413841849868,
-49.4228158753796));
#239327=CARTESIAN_POINT('Ctrl Pts',(42.8356192866904,-56.3483239727476,
-49.4076973944461));
#239328=CARTESIAN_POINT('Ctrl Pts',(42.6009172321237,-56.8170394584344,
-49.3771732793191));
#239329=CARTESIAN_POINT('Ctrl Pts',(42.5305072941766,-57.0753961113057,
-49.3620679563592));
#239330=CARTESIAN_POINT('Ctrl Pts',(42.4953952961135,-57.5926212844573,
-49.3349145982825));
#239331=CARTESIAN_POINT('Ctrl Pts',(42.5263675132484,-57.8462316166951,
-49.3219318186393));
#239332=CARTESIAN_POINT('Ctrl Pts',(42.6840582308023,-58.336909494207,-49.2925443681356));
#239333=CARTESIAN_POINT('Ctrl Pts',(42.8125271523483,-58.5682601143377,
-49.277109952928));
#239334=CARTESIAN_POINT('Ctrl Pts',(43.1536370793267,-58.9709056695457,
-49.2468200054185));
#239335=CARTESIAN_POINT('Ctrl Pts',(43.3639361748342,-59.1372944985489,
-49.2329342832032));
#239336=CARTESIAN_POINT('Ctrl Pts',(43.8282116719572,-59.3736681285028,
-49.205851545871));
#239337=CARTESIAN_POINT('Ctrl Pts',(44.075958726924,-59.4448710603739,-49.1913996343313));
#239338=CARTESIAN_POINT('Ctrl Pts',(44.3895030689671,-59.4728249807475,
-49.1731095477121));
#239339=CARTESIAN_POINT('Ctrl Pts',(44.4487628003175,-59.475452478349,-49.1696527300501));
#239340=CARTESIAN_POINT('Ctrl Pts',(44.5079524583206,-59.475452478349,-49.1662));
#239341=CARTESIAN_POINT('Origin',(44.5079524583206,-57.475452478349,235.35105));
#239342=CARTESIAN_POINT('',(44.5079524583206,-59.475452478349,-48.4662));
#239343=CARTESIAN_POINT('',(44.5079524583206,-59.475452478349,-48.6249500000001));
#239344=CARTESIAN_POINT('',(44.5079524583206,-59.475452478349,235.35105));
#239345=CARTESIAN_POINT('Ctrl Pts',(44.5079524583206,-59.475452478349,-48.6249500000001));
#239346=CARTESIAN_POINT('Ctrl Pts',(44.2628858061291,-59.475452478349,-48.6392455547112));
#239347=CARTESIAN_POINT('Ctrl Pts',(44.0197530000773,-59.4304074108024,
-48.653428301731));
#239348=CARTESIAN_POINT('Ctrl Pts',(43.5503561414569,-59.250085042783,-48.6808097851505));
#239349=CARTESIAN_POINT('Ctrl Pts',(43.3300987723401,-59.1122108366676,
-48.6932847306152));
#239350=CARTESIAN_POINT('Ctrl Pts',(42.9483494736007,-58.7552654889186,
-48.7224513032651));
#239351=CARTESIAN_POINT('Ctrl Pts',(42.7926360521606,-58.53750494125,-48.7379938044201));
#239352=CARTESIAN_POINT('Ctrl Pts',(42.5792853953837,-58.0630921017883,
-48.7681829902094));
#239353=CARTESIAN_POINT('Ctrl Pts',(42.5201114162669,-57.8125110023086,
-48.782567791142));
#239354=CARTESIAN_POINT('Ctrl Pts',(42.4986930893646,-57.2911026753661,
-48.8095330756611));
#239355=CARTESIAN_POINT('Ctrl Pts',(42.5411384880099,-57.025095625394,-48.8236691202661));
#239356=CARTESIAN_POINT('Ctrl Pts',(42.7262002695061,-56.5300023567024,
-48.8540779508556));
#239357=CARTESIAN_POINT('Ctrl Pts',(42.8651008634393,-56.3051702510185,
-48.8694873198933));
#239358=CARTESIAN_POINT('Ctrl Pts',(43.2158589037499,-55.9279840651222,
-48.8987725105074));
#239359=CARTESIAN_POINT('Ctrl Pts',(43.421980054436,-55.7769839375025,-48.9116016097736));
#239360=CARTESIAN_POINT('Ctrl Pts',(43.8904129903254,-55.5547787422683,
-48.938926864367));
#239361=CARTESIAN_POINT('Ctrl Pts',(44.1502370279982,-55.4899195933945,
-48.9540832665646));
#239362=CARTESIAN_POINT('Ctrl Pts',(44.673562407491,-55.4655959698017,-48.9846105803683));
#239363=CARTESIAN_POINT('Ctrl Pts',(44.9319452632814,-55.5038531889676,
-48.9996829136228));
#239364=CARTESIAN_POINT('Ctrl Pts',(45.4173294380215,-55.6758275679205,
-49.0279969904826));
#239365=CARTESIAN_POINT('Ctrl Pts',(45.6400656968707,-55.8069390138041,
-49.040346425058));
#239366=CARTESIAN_POINT('Ctrl Pts',(46.0312969479705,-56.15253847459,-49.0692163814486));
#239367=CARTESIAN_POINT('Ctrl Pts',(46.1934495883523,-56.3665082155528,
-49.0847551886198));
#239368=CARTESIAN_POINT('Ctrl Pts',(46.4202265107652,-56.836213844073,-49.1150981742418));
#239369=CARTESIAN_POINT('Ctrl Pts',(46.4862393844462,-57.0857870682806,
-49.1296315269398));
#239370=CARTESIAN_POINT('Ctrl Pts',(46.5211806859975,-57.6045889103354,
-49.1568595567621));
#239371=CARTESIAN_POINT('Ctrl Pts',(46.4865588826382,-57.8690589132808,
-49.1704582476425));
#239372=CARTESIAN_POINT('Ctrl Pts',(46.3170122058166,-58.367765103258,-49.20059707244));
#239373=CARTESIAN_POINT('Ctrl Pts',(46.1843934954698,-58.597265521946,-49.216059054403));
#239374=CARTESIAN_POINT('Ctrl Pts',(45.8441363149027,-58.9850222178621,
-49.2455719725367));
#239375=CARTESIAN_POINT('Ctrl Pts',(45.6424168786208,-59.1419232574092,
-49.258772908816));
#239376=CARTESIAN_POINT('Ctrl Pts',(45.1806076872912,-59.3775193679133,
-49.2857117783102));
#239377=CARTESIAN_POINT('Ctrl Pts',(44.9228019790787,-59.449832775337,-49.3007504446226));
#239378=CARTESIAN_POINT('Ctrl Pts',(44.6083029113298,-59.473566405843,-49.3190962235747));
#239379=CARTESIAN_POINT('Ctrl Pts',(44.5581003572643,-59.475452478349,-49.322024705895));
#239380=CARTESIAN_POINT('Ctrl Pts',(44.5079524583206,-59.475452478349,-49.3249500000001));
#239381=CARTESIAN_POINT('Ctrl Pts',(44.5079524583206,-59.475452478349,-49.1662));
#239382=CARTESIAN_POINT('Ctrl Pts',(44.7132715088587,-59.475452478349,-49.1542230553852));
#239383=CARTESIAN_POINT('Ctrl Pts',(44.9177473805613,-59.4438328899582,
-49.1422952962024));
#239384=CARTESIAN_POINT('Ctrl Pts',(45.358903240101,-59.3035316594213,-49.116561204396));
#239385=CARTESIAN_POINT('Ctrl Pts',(45.5863767543091,-59.1792682324807,
-49.1041529087429));
#239386=CARTESIAN_POINT('Ctrl Pts',(45.9831298528174,-58.8504548046765,
-49.0759698977774));
#239387=CARTESIAN_POINT('Ctrl Pts',(46.1482456265836,-58.6485645864941,
-49.0609549010088));
#239388=CARTESIAN_POINT('Ctrl Pts',(46.3957283829482,-58.1872209175729,
-49.0304304259471));
#239389=CARTESIAN_POINT('Ctrl Pts',(46.4733812498941,-57.9309093580201,
-49.0152171652196));
#239390=CARTESIAN_POINT('Ctrl Pts',(46.5230199061657,-57.4146992144779,
-48.9876913903617));
#239391=CARTESIAN_POINT('Ctrl Pts',(46.4991408743921,-57.1602047976489,
-48.9750172663038));
#239392=CARTESIAN_POINT('Ctrl Pts',(46.3553727362881,-56.6659126895361,
-48.9458533067957));
#239393=CARTESIAN_POINT('Ctrl Pts',(46.2338822787049,-56.4316732943863,
-48.9304764945548));
#239394=CARTESIAN_POINT('Ctrl Pts',(45.9052964648732,-56.0201967535934,
-48.9001057086371));
#239395=CARTESIAN_POINT('Ctrl Pts',(45.7002801752457,-55.8479994165806,
-48.885752450154));
#239396=CARTESIAN_POINT('Ctrl Pts',(45.2442659485269,-55.5985583229646,
-48.8591516202621));
#239397=CARTESIAN_POINT('Ctrl Pts',(44.9995138590369,-55.5201491841072,
-48.8448744150418));
#239398=CARTESIAN_POINT('Ctrl Pts',(44.484009019507,-55.4581707161369,-48.8148032994025));
#239399=CARTESIAN_POINT('Ctrl Pts',(44.217639991574,-55.4790228412861,-48.7992651061064));
#239400=CARTESIAN_POINT('Ctrl Pts',(43.7142356080425,-55.6215683034491,
-48.7698998504004));
#239401=CARTESIAN_POINT('Ctrl Pts',(43.4814911769751,-55.7395837163142,
-48.7572877552849));
#239402=CARTESIAN_POINT('Ctrl Pts',(43.0744826223804,-56.0571589538179,
-48.7293733594172));
#239403=CARTESIAN_POINT('Ctrl Pts',(42.9038953539184,-56.2534202770791,
-48.7144831387365));
#239404=CARTESIAN_POINT('Ctrl Pts',(42.6414553133673,-56.7086763374907,
-48.6838299442637));
#239405=CARTESIAN_POINT('Ctrl Pts',(42.5556337052545,-56.9653111080983,
-48.6683621005613));
#239406=CARTESIAN_POINT('Ctrl Pts',(42.4919360036821,-57.4830825969925,
-48.6403473939391));
#239407=CARTESIAN_POINT('Ctrl Pts',(42.5091508424181,-57.7384862452087,
-48.6278770682213));
#239408=CARTESIAN_POINT('Ctrl Pts',(42.6399410486995,-58.2360422490106,
-48.5989267457574));
#239409=CARTESIAN_POINT('Ctrl Pts',(42.7548773808458,-58.472788537187,-48.5836144519141));
#239410=CARTESIAN_POINT('Ctrl Pts',(43.0716962448171,-58.8922797794919,
-48.553181980819));
#239411=CARTESIAN_POINT('Ctrl Pts',(43.2718943390135,-59.0699569802348,
-48.5383669465165));
#239412=CARTESIAN_POINT('Ctrl Pts',(43.720316120413,-59.3312793356208,-48.5120864563225));
#239413=CARTESIAN_POINT('Ctrl Pts',(43.9621322449313,-59.4162392210301,
-48.4980395124476));
#239414=CARTESIAN_POINT('Ctrl Pts',(44.3111829714994,-59.4681993883674,
-48.4776782200645));
#239415=CARTESIAN_POINT('Ctrl Pts',(44.409611102366,-59.475452478349,-48.4719365790973));
#239416=CARTESIAN_POINT('Ctrl Pts',(44.5079524583206,-59.475452478349,-48.4662));
#239417=CARTESIAN_POINT('Origin',(44.5079524583206,-57.475452478349,235.35105));
#239418=CARTESIAN_POINT('',(44.5079524583206,-59.475452478349,-47.7662));
#239419=CARTESIAN_POINT('',(44.5079524583206,-59.475452478349,-47.9249500000001));
#239420=CARTESIAN_POINT('',(44.5079524583206,-59.475452478349,235.35105));
#239421=CARTESIAN_POINT('Ctrl Pts',(44.5079524583206,-59.475452478349,-47.9249500000001));
#239422=CARTESIAN_POINT('Ctrl Pts',(44.4812735172686,-59.475452478349,-47.9265062715615));
#239423=CARTESIAN_POINT('Ctrl Pts',(44.4545736600142,-59.4749186583905,
-47.9280637632347));
#239424=CARTESIAN_POINT('Ctrl Pts',(44.1714735144825,-59.4635736950934,
-47.9445779383907));
#239425=CARTESIAN_POINT('Ctrl Pts',(43.9194001871073,-59.4040494254147,
-47.9592822158209));
#239426=CARTESIAN_POINT('Ctrl Pts',(43.4472013548033,-59.1910043209327,
-47.9868271477054));
#239427=CARTESIAN_POINT('Ctrl Pts',(43.2323421053487,-59.0378716270781,
-47.9998914459693));
#239428=CARTESIAN_POINT('Ctrl Pts',(42.872209851426,-58.6560295349205,-48.0296852589112));
#239429=CARTESIAN_POINT('Ctrl Pts',(42.7310849722988,-58.4305188890606,
-48.0451937815271));
#239430=CARTESIAN_POINT('Ctrl Pts',(42.5477880010018,-57.946809992494,-48.0749760210836));
#239431=CARTESIAN_POINT('Ctrl Pts',(42.5038789014379,-57.6945899848913,
-48.0887607668151));
#239432=CARTESIAN_POINT('Ctrl Pts',(42.5128179882102,-57.1758953028072,
-48.115224985183));
#239433=CARTESIAN_POINT('Ctrl Pts',(42.57005350494,-56.914388489372,-48.13010519447));
#239434=CARTESIAN_POINT('Ctrl Pts',(42.7811922510803,-56.4333024154484,
-48.1605669856489));
#239435=CARTESIAN_POINT('Ctrl Pts',(42.9313712997834,-56.217603719075,-48.175843906689));
#239436=CARTESIAN_POINT('Ctrl Pts',(43.3014050122175,-55.8602827251107,
-48.2046877516896));
#239437=CARTESIAN_POINT('Ctrl Pts',(43.5160390694056,-55.7202808025766,
-48.2170883856467));
#239438=CARTESIAN_POINT('Ctrl Pts',(43.9988476680525,-55.5229120870323,
-48.2452522205677));
#239439=CARTESIAN_POINT('Ctrl Pts',(44.264324345215,-55.472401353952,-48.2607383600689));
#239440=CARTESIAN_POINT('Ctrl Pts',(44.7891056123032,-55.4786665482241,
-48.291350600649));
#239441=CARTESIAN_POINT('Ctrl Pts',(45.0434210252528,-55.5313571362534,
-48.3061856664044));
#239442=CARTESIAN_POINT('Ctrl Pts',(45.520018192311,-55.7310329889019,-48.3339871678161));
#239443=CARTESIAN_POINT('Ctrl Pts',(45.7374485981369,-55.8768189925122,
-48.3467169668236));
#239444=CARTESIAN_POINT('Ctrl Pts',(46.1080265911284,-56.2467982934191,
-48.3762161609043));
#239445=CARTESIAN_POINT('Ctrl Pts',(46.2561798782702,-56.4687162142566,
-48.3917481809377));
#239446=CARTESIAN_POINT('Ctrl Pts',(46.4538706739191,-56.9481137726077,
-48.4217324395466));
#239447=CARTESIAN_POINT('Ctrl Pts',(46.5051137679225,-57.1996308181294,
-48.4359332052579));
#239448=CARTESIAN_POINT('Ctrl Pts',(46.5106749708228,-57.719009698564,-48.4623334664469));
#239449=CARTESIAN_POINT('Ctrl Pts',(46.4608239245511,-57.9820273274215,
-48.4769158057141));
#239450=CARTESIAN_POINT('Ctrl Pts',(46.2628832553274,-58.4696172890998,
-48.5073212173507));
#239451=CARTESIAN_POINT('Ctrl Pts',(46.118275604911,-58.6899543335241,-48.5226699600301));
#239452=CARTESIAN_POINT('Ctrl Pts',(45.7578409129819,-59.057242152736,-48.5517373391578));
#239453=CARTESIAN_POINT('Ctrl Pts',(45.5475198216822,-59.2027509743537,
-48.5643085704707));
#239454=CARTESIAN_POINT('Ctrl Pts',(45.0729530614444,-59.4122363761628,
-48.5919916314846));
#239455=CARTESIAN_POINT('Ctrl Pts',(44.8114261044714,-59.4700010872062,
-48.6072473706413));
#239456=CARTESIAN_POINT('Ctrl Pts',(44.5335099733831,-59.4753300564951,
-48.6234591449548));
#239457=CARTESIAN_POINT('Ctrl Pts',(44.5207285878716,-59.475452478349,-48.6242047257763));
#239458=CARTESIAN_POINT('Ctrl Pts',(44.5079524583206,-59.475452478349,-48.6249500000001));
#239459=CARTESIAN_POINT('Ctrl Pts',(44.5079524583206,-59.475452478349,-48.4662));
#239460=CARTESIAN_POINT('Ctrl Pts',(44.6722461043367,-59.475452478349,-48.4566162039824));
#239461=CARTESIAN_POINT('Ctrl Pts',(44.8362975563793,-59.4552073494373,
-48.4470465359465));
#239462=CARTESIAN_POINT('Ctrl Pts',(45.2488941590956,-59.3513070975787,
-48.422978400788));
#239463=CARTESIAN_POINT('Ctrl Pts',(45.486541680707,-59.2390197994558,-48.4100833035931));
#239464=CARTESIAN_POINT('Ctrl Pts',(45.9027515590896,-58.9316738856167,
-48.3824173022742));
#239465=CARTESIAN_POINT('Ctrl Pts',(46.0781093830703,-58.7406079583137,
-48.3676504021756));
#239466=CARTESIAN_POINT('Ctrl Pts',(46.3522268646779,-58.2939865942306,
-48.3370928245439));
#239467=CARTESIAN_POINT('Ctrl Pts',(46.4449529529653,-58.0406124163855,
-48.3215883192794));
#239468=CARTESIAN_POINT('Ctrl Pts',(46.5234594666808,-57.5249853327108,
-48.2932500203511));
#239469=CARTESIAN_POINT('Ctrl Pts',(46.5134218647486,-57.2685197941095,
-48.2809056682711));
#239470=CARTESIAN_POINT('Ctrl Pts',(46.3964759327107,-56.767589888895,-48.2521886938865));
#239471=CARTESIAN_POINT('Ctrl Pts',(46.2885726388101,-56.5283697946779,
-48.2369565582243));
#239472=CARTESIAN_POINT('Ctrl Pts',(45.9843414414616,-56.1004848845509,
-48.2064671948478));
#239473=CARTESIAN_POINT('Ctrl Pts',(45.7892916557144,-55.9170947423855,
-48.1915137123182));
#239474=CARTESIAN_POINT('Ctrl Pts',(45.348927075157,-55.6432465319262,-48.164835440808));
#239475=CARTESIAN_POINT('Ctrl Pts',(45.1101967248856,-55.5515005415793,
-48.1513309155497));
#239476=CARTESIAN_POINT('Ctrl Pts',(44.6017017858425,-55.4604092580464,
-48.1216687107721));
#239477=CARTESIAN_POINT('Ctrl Pts',(44.336159119653,-55.4655573311246,-48.1061787219111));
#239478=CARTESIAN_POINT('Ctrl Pts',(43.8227104150117,-55.5782399321306,
-48.0762275474736));
#239479=CARTESIAN_POINT('Ctrl Pts',(43.5798406550112,-55.684489612824,-48.0629395338322));
#239480=CARTESIAN_POINT('Ctrl Pts',(43.154156374964,-55.9811549817676,-48.0355367571517));
#239481=CARTESIAN_POINT('Ctrl Pts',(42.9740323221626,-56.16673555949,-48.0209079517508));
#239482=CARTESIAN_POINT('Ctrl Pts',(42.6881360285851,-56.6041343058631,
-47.9904727350081));
#239483=CARTESIAN_POINT('Ctrl Pts',(42.5883969739102,-56.8539548963596,
-47.9749432055442));
#239484=CARTESIAN_POINT('Ctrl Pts',(42.4946218652844,-57.3672049541195,
-47.9462796555459));
#239485=CARTESIAN_POINT('Ctrl Pts',(42.4972562241896,-57.6248506055178,
-47.9339646567133));
#239486=CARTESIAN_POINT('Ctrl Pts',(42.6000879300122,-58.1291088776438,
-47.9054912043259));
#239487=CARTESIAN_POINT('Ctrl Pts',(42.7007890912238,-58.3706358676202,
-47.8903525907645));
#239488=CARTESIAN_POINT('Ctrl Pts',(42.9919888297182,-58.8066701715437,
-47.8598316193181));
#239489=CARTESIAN_POINT('Ctrl Pts',(43.1816290358722,-58.995714545876,-47.8447502748528));
#239490=CARTESIAN_POINT('Ctrl Pts',(43.6136801796984,-59.2822158687836,
-47.8176752667663));
#239491=CARTESIAN_POINT('Ctrl Pts',(43.8493896412147,-59.3808283931455,
-47.8046161643311));
#239492=CARTESIAN_POINT('Ctrl Pts',(44.2326665036937,-59.4612393661861,
-47.7822583473531));
#239493=CARTESIAN_POINT('Ctrl Pts',(44.3702910583955,-59.475452478349,-47.7742302483289));
#239494=CARTESIAN_POINT('Ctrl Pts',(44.5079524583206,-59.475452478349,-47.7662));
#239495=CARTESIAN_POINT('Origin',(44.5079524583206,-57.475452478349,235.35105));
#239496=CARTESIAN_POINT('',(44.5079524583206,-59.475452478349,-47.0662));
#239497=CARTESIAN_POINT('',(44.5079524583206,-59.475452478349,-47.2249500000001));
#239498=CARTESIAN_POINT('',(44.5079524583206,-59.475452478349,235.35105));
#239499=CARTESIAN_POINT('Ctrl Pts',(44.5079524583206,-59.475452478349,-47.2249500000001));
#239500=CARTESIAN_POINT('Ctrl Pts',(44.4440657053146,-59.475452478349,-47.2286767272588));
#239501=CARTESIAN_POINT('Ctrl Pts',(44.3801027710404,-59.4723914198285,
-47.2324078984249));
#239502=CARTESIAN_POINT('Ctrl Pts',(44.0622334462755,-59.4417876861605,
-47.2509502757029));
#239503=CARTESIAN_POINT('Ctrl Pts',(43.8151560576545,-59.3689190437521,
-47.2653631233725));
#239504=CARTESIAN_POINT('Ctrl Pts',(43.3520565585926,-59.1291615287946,
-47.2923772608178));
#239505=CARTESIAN_POINT('Ctrl Pts',(43.1424308834313,-58.9608025867536,
-47.3064072418367));
#239506=CARTESIAN_POINT('Ctrl Pts',(42.804167543703,-58.5551320031449,-47.3367669827188));
#239507=CARTESIAN_POINT('Ctrl Pts',(42.6775733797043,-58.3229827036197,
-47.3521870653023));
#239508=CARTESIAN_POINT('Ctrl Pts',(42.5236348995407,-57.8313190140775,
-47.3815148769473));
#239509=CARTESIAN_POINT('Ctrl Pts',(42.4945693561079,-57.577479578032,-47.3944054393407));
#239510=CARTESIAN_POINT('Ctrl Pts',(42.5335756423137,-57.0605121379261,
-47.4216593606253));
#239511=CARTESIAN_POINT('Ctrl Pts',(42.6059328844838,-56.8026831422405,
-47.4367948236942));
#239512=CARTESIAN_POINT('Ctrl Pts',(42.8440833337503,-56.3359092265583,
-47.4673214324781));
#239513=CARTESIAN_POINT('Ctrl Pts',(43.0054095238479,-56.1303104652254,
-47.4824132484568));
#239514=CARTESIAN_POINT('Ctrl Pts',(43.3952215439451,-55.7939871960042,
-47.5107731945863));
#239515=CARTESIAN_POINT('Ctrl Pts',(43.6192416365683,-55.6655659856764,
-47.523108535398));
#239516=CARTESIAN_POINT('Ctrl Pts',(44.1131444124268,-55.4968457401887,
-47.5519195306564));
#239517=CARTESIAN_POINT('Ctrl Pts',(44.3794878812615,-55.4619401339279,
-47.567456233005));
#239518=CARTESIAN_POINT('Ctrl Pts',(44.9001253313971,-55.4976543677708,
-47.5978267509296));
#239519=CARTESIAN_POINT('Ctrl Pts',(45.1497467158906,-55.5640067925415,
-47.6123879983584));
#239520=CARTESIAN_POINT('Ctrl Pts',(45.6173792779121,-55.7906106541898,
-47.6396665644763));
#239521=CARTESIAN_POINT('Ctrl Pts',(45.8296035617798,-55.9513791485695,
-47.6531714609698));
#239522=CARTESIAN_POINT('Ctrl Pts',(46.1788061885846,-56.3452997501013,
-47.6832566770517));
#239523=CARTESIAN_POINT('Ctrl Pts',(46.3126336338315,-56.5742741833758,
-47.6987273419733));
#239524=CARTESIAN_POINT('Ctrl Pts',(46.481103660285,-57.0620705652085,-47.7282836211598));
#239525=CARTESIAN_POINT('Ctrl Pts',(46.5175359190433,-57.3150594772912,
-47.7415677249412));
#239526=CARTESIAN_POINT('Ctrl Pts',(46.4935268385644,-57.8329630900862,
-47.7684315214364));
#239527=CARTESIAN_POINT('Ctrl Pts',(46.4286888059395,-58.092740649065,-47.7834461120366));
#239528=CARTESIAN_POINT('Ctrl Pts',(46.2039030615399,-58.566849637401,-47.8139534712186));
#239529=CARTESIAN_POINT('Ctrl Pts',(46.048059785429,-58.7775600987125,-47.8291436024916));
#239530=CARTESIAN_POINT('Ctrl Pts',(45.6680828398364,-59.1244022108298,
-47.8577480847495));
#239531=CARTESIAN_POINT('Ctrl Pts',(45.448816781282,-59.2586260436173,-47.8700662478273));
#239532=CARTESIAN_POINT('Ctrl Pts',(44.9854445467154,-59.4323969429685,
-47.8970962948437));
#239533=CARTESIAN_POINT('Ctrl Pts',(44.7475419366017,-59.475452478349,-47.9109739471004));
#239534=CARTESIAN_POINT('Ctrl Pts',(44.5079524583206,-59.475452478349,-47.9249500000001));
#239535=CARTESIAN_POINT('Ctrl Pts',(44.5079524583206,-59.475452478349,-47.7662));
#239536=CARTESIAN_POINT('Ctrl Pts',(44.6313030775092,-59.475452478349,-47.759004547214));
#239537=CARTESIAN_POINT('Ctrl Pts',(44.7546832795126,-59.4640410230751,
-47.7518073687637));
#239538=CARTESIAN_POINT('Ctrl Pts',(45.1370515644779,-59.3923532492405,
-47.7295025521408));
#239539=CARTESIAN_POINT('Ctrl Pts',(45.3852358868118,-59.2922063992075,
-47.7157249444625));
#239540=CARTESIAN_POINT('Ctrl Pts',(45.820249612569,-59.0062087994247,-47.688588974896));
#239541=CARTESIAN_POINT('Ctrl Pts',(46.0049145305874,-58.8261567023458,
-47.6741070161994));
#239542=CARTESIAN_POINT('Ctrl Pts',(46.3021477299,-58.3981562130439,-47.643815922253));
#239543=CARTESIAN_POINT('Ctrl Pts',(46.4086861793783,-58.1520249958447,
-47.6282744574157));
#239544=CARTESIAN_POINT('Ctrl Pts',(46.5175168144668,-57.6412869744509,
-47.5992986913219));
#239545=CARTESIAN_POINT('Ctrl Pts',(46.522199175265,-57.3824073136085,-47.5869150597897));
#239546=CARTESIAN_POINT('Ctrl Pts',(46.4331309042178,-56.8750041847558,
-47.5586841685773));
#239547=CARTESIAN_POINT('Ctrl Pts',(46.3394721976225,-56.6314380197376,
-47.5436479445944));
#239548=CARTESIAN_POINT('Ctrl Pts',(46.0611496297214,-56.1878629206276,
-47.5131216102789));
#239549=CARTESIAN_POINT('Ctrl Pts',(45.8769306728218,-55.993478493689,-47.4979286160126));
#239550=CARTESIAN_POINT('Ctrl Pts',(45.4530866298438,-55.6947548334533,
-47.470475531848));
#239551=CARTESIAN_POINT('Ctrl Pts',(45.2202087529216,-55.5894829466028,
-47.4577482838518));
#239552=CARTESIAN_POINT('Ctrl Pts',(44.719497596083,-55.469551318773,-47.4285401330362));
#239553=CARTESIAN_POINT('Ctrl Pts',(44.4556856297394,-55.4591062061042,
-47.4131511016661));
#239554=CARTESIAN_POINT('Ctrl Pts',(43.9353429727177,-55.5409072719665,
-47.3827977800065));
#239555=CARTESIAN_POINT('Ctrl Pts',(43.6842138557186,-55.6337907462551,
-47.3685449650591));
#239556=CARTESIAN_POINT('Ctrl Pts',(43.2415863401375,-55.906606008996,-47.3418528738837));
#239557=CARTESIAN_POINT('Ctrl Pts',(43.0522030195489,-56.0805650309788,
-47.327541105985));
#239558=CARTESIAN_POINT('Ctrl Pts',(42.7430570731635,-56.4980950413809,
-47.2974315061241));
#239559=CARTESIAN_POINT('Ctrl Pts',(42.629317206933,-56.7400426823803,-47.2818913464887));
#239560=CARTESIAN_POINT('Ctrl Pts',(42.5042318600095,-57.2478692796583,
-47.2525885643891));
#239561=CARTESIAN_POINT('Ctrl Pts',(42.4916160868242,-57.5081563403832,
-47.2400243389413));
#239562=CARTESIAN_POINT('Ctrl Pts',(42.5659866783359,-58.018807860116,-47.2120580273557));
#239563=CARTESIAN_POINT('Ctrl Pts',(42.6521178711617,-58.2643216483869,
-47.1971429655331));
#239564=CARTESIAN_POINT('Ctrl Pts',(42.9126065722437,-58.7087982931983,
-47.1670912412467));
#239565=CARTESIAN_POINT('Ctrl Pts',(43.0844502985395,-58.9037183457706,
-47.1522321323951));
#239566=CARTESIAN_POINT('Ctrl Pts',(43.4938571975499,-59.2186407206989,
-47.124381802521));
#239567=CARTESIAN_POINT('Ctrl Pts',(43.7278636795627,-59.335174960608,-47.1117051787608));
#239568=CARTESIAN_POINT('Ctrl Pts',(44.1507753466232,-59.4514755926062,
-47.0870353315156));
#239569=CARTESIAN_POINT('Ctrl Pts',(44.3291584670778,-59.475452478349,-47.0766296494891));
#239570=CARTESIAN_POINT('Ctrl Pts',(44.5079524583206,-59.475452478349,-47.0662));
#239571=CARTESIAN_POINT('Origin',(44.5079524583206,-57.475452478349,235.35105));
#239572=CARTESIAN_POINT('',(44.5079524583206,-59.475452478349,-46.3662));
#239573=CARTESIAN_POINT('',(44.5079524583206,-59.475452478349,-46.5249500000001));
#239574=CARTESIAN_POINT('',(44.5079524583206,-59.475452478349,235.35105));
#239575=CARTESIAN_POINT('Ctrl Pts',(44.5079524583206,-59.475452478349,-46.5249500000001));
#239576=CARTESIAN_POINT('Ctrl Pts',(44.4042739832461,-59.475452478349,-46.5309979110461));
#239577=CARTESIAN_POINT('Ctrl Pts',(44.3005150510559,-59.4673907344713,
-46.537050515424));
#239578=CARTESIAN_POINT('Ctrl Pts',(43.9467671950224,-59.4118283130573,
-46.5576858070259));
#239579=CARTESIAN_POINT('Ctrl Pts',(43.7057975820276,-59.3250281505324,
-46.5715757119894));
#239580=CARTESIAN_POINT('Ctrl Pts',(43.2595445886996,-59.0603086524142,
-46.5979645632259));
#239581=CARTESIAN_POINT('Ctrl Pts',(43.0607222290518,-58.8810713066766,
-46.612818287574));
#239582=CARTESIAN_POINT('Ctrl Pts',(42.74728581496,-58.4592725694533,-46.643268674252));
#239583=CARTESIAN_POINT('Ctrl Pts',(42.634246955762,-58.2218370397722,-46.6585604443391));
#239584=CARTESIAN_POINT('Ctrl Pts',(42.5071992348591,-57.7233581402891,
-46.6874482339606));
#239585=CARTESIAN_POINT('Ctrl Pts',(42.4919171279419,-57.4676768193125,
-46.6998751147625));
#239586=CARTESIAN_POINT('Ctrl Pts',(42.5596016163837,-56.9504674630264,
-46.7279777047698));
#239587=CARTESIAN_POINT('Ctrl Pts',(42.6472914041524,-56.6946922299341,
-46.7434566148015));
#239588=CARTESIAN_POINT('Ctrl Pts',(42.9128987581068,-56.2417300473847,
-46.7740863067859));
#239589=CARTESIAN_POINT('Ctrl Pts',(43.0847842513759,-56.0468549063726,
-46.7889443649961));
#239590=CARTESIAN_POINT('Ctrl Pts',(43.4942711729337,-55.7320212087172,
-46.8167925490495));
#239591=CARTESIAN_POINT('Ctrl Pts',(43.7283199576162,-55.6155365287536,
-46.8294714374591));
#239592=CARTESIAN_POINT('Ctrl Pts',(44.2330764345255,-55.4768661041142,
-46.8589155652787));
#239593=CARTESIAN_POINT('Ctrl Pts',(44.4993887678175,-55.4580733083678,
-46.8744504513874));
#239594=CARTESIAN_POINT('Ctrl Pts',(45.0140292962556,-55.5238797838391,
-46.9044711488796));
#239595=CARTESIAN_POINT('Ctrl Pts',(45.2580164631152,-55.6040358428384,
-46.9187037336131));
#239596=CARTESIAN_POINT('Ctrl Pts',(45.7120200559247,-55.8566715438271,
-46.9451872765269));
#239597=CARTESIAN_POINT('Ctrl Pts',(45.9157706920935,-56.0303301365342,
-46.9596731266758));
#239598=CARTESIAN_POINT('Ctrl Pts',(46.2412554684407,-56.4440099576876,
-46.9900647713114));
#239599=CARTESIAN_POINT('Ctrl Pts',(46.3609997236072,-56.6789365473775,
-47.0054253684444));
#239600=CARTESIAN_POINT('Ctrl Pts',(46.5013017891596,-57.1741101225957,
-47.0345327642559));
#239601=CARTESIAN_POINT('Ctrl Pts',(46.5234063952971,-57.4288392538153,
-47.04714444637));
#239602=CARTESIAN_POINT('Ctrl Pts',(46.470118383048,-57.9447710465749,-47.074762599011));
#239603=CARTESIAN_POINT('Ctrl Pts',(46.3906555534907,-58.2005360292035,
-47.0900010382605));
#239604=CARTESIAN_POINT('Ctrl Pts',(46.1399985072978,-58.6599728667733,
-47.120521767186));
#239605=CARTESIAN_POINT('Ctrl Pts',(45.97360126581,-58.8605746742798,-47.1355090519746));
#239606=CARTESIAN_POINT('Ctrl Pts',(45.5744722927262,-59.1867997188816,
-47.1636305989549));
#239607=CARTESIAN_POINT('Ctrl Pts',(45.3457956844884,-59.3096273670682,
-47.1760758118071));
#239608=CARTESIAN_POINT('Ctrl Pts',(44.9079694493998,-59.445334969169,-47.2016156755206));
#239609=CARTESIAN_POINT('Ctrl Pts',(44.7083356845824,-59.475452478349,-47.2132609784681));
#239610=CARTESIAN_POINT('Ctrl Pts',(44.5079524583206,-59.475452478349,-47.2249500000001));
#239611=CARTESIAN_POINT('Ctrl Pts',(44.5079524583206,-59.475452478349,-47.0662));
#239612=CARTESIAN_POINT('Ctrl Pts',(44.5924271409675,-59.475452478349,-47.0612723101789));
#239613=CARTESIAN_POINT('Ctrl Pts',(44.6769935411895,-59.4701006492632,
-47.0563392701659));
#239614=CARTESIAN_POINT('Ctrl Pts',(45.0135599292962,-59.4271476052498,
-47.0367062308597));
#239615=CARTESIAN_POINT('Ctrl Pts',(45.2575720473973,-59.3470479781173,
-47.0224721906372));
#239616=CARTESIAN_POINT('Ctrl Pts',(45.711641066771,-59.0945154240205,-46.9959848311737));
#239617=CARTESIAN_POINT('Ctrl Pts',(45.9154328226276,-58.9209039851203,
-46.9815033566545));
#239618=CARTESIAN_POINT('Ctrl Pts',(46.2410181893005,-58.5072951339138,
-46.9511123634047));
#239619=CARTESIAN_POINT('Ctrl Pts',(46.3608190217601,-58.2723905884207,
-46.9357512297327));
#239620=CARTESIAN_POINT('Ctrl Pts',(46.5012332875956,-57.7772454347755,
-46.9066419972182));
#239621=CARTESIAN_POINT('Ctrl Pts',(46.5233953924273,-57.5225239937747,
-46.8940283847204));
#239622=CARTESIAN_POINT('Ctrl Pts',(46.4702257197404,-57.0065830249847,
-46.8664132200939));
#239623=CARTESIAN_POINT('Ctrl Pts',(46.3908215178601,-56.75080011293,-46.851175585057));
#239624=CARTESIAN_POINT('Ctrl Pts',(46.140267168965,-56.2913011007345,-46.8206547105223));
#239625=CARTESIAN_POINT('Ctrl Pts',(45.9739113259972,-56.0906573913506,
-46.8056665163854));
#239626=CARTESIAN_POINT('Ctrl Pts',(45.5748593452836,-55.7643483249545,
-46.7775429703905));
#239627=CARTESIAN_POINT('Ctrl Pts',(45.3462218937679,-55.6414740431258,
-46.7650990504012));
#239628=CARTESIAN_POINT('Ctrl Pts',(44.8471901486515,-55.4866647470764,
-46.7359888652694));
#239629=CARTESIAN_POINT('Ctrl Pts',(44.5807437012705,-55.459257464827,-46.7204461558388));
#239630=CARTESIAN_POINT('Ctrl Pts',(44.0626789576252,-55.5090156063934,
-46.6902257124594));
#239631=CARTESIAN_POINT('Ctrl Pts',(43.8155796410498,-55.5818302308093,
-46.6758115856592));
#239632=CARTESIAN_POINT('Ctrl Pts',(43.352441813358,-55.8214777672794,-46.6487952123772));
#239633=CARTESIAN_POINT('Ctrl Pts',(43.1427941923756,-55.9897724887097,
-46.6347700196637));
#239634=CARTESIAN_POINT('Ctrl Pts',(42.8044379796576,-56.3953447375082,
-46.6044125376785));
#239635=CARTESIAN_POINT('Ctrl Pts',(42.677782736474,-56.6274682800165,-46.5889919748156));
#239636=CARTESIAN_POINT('Ctrl Pts',(42.523722154733,-57.1191000281729,-46.5596622154942));
#239637=CARTESIAN_POINT('Ctrl Pts',(42.4945945119314,-57.3729319034361,
-46.5467687564028));
#239638=CARTESIAN_POINT('Ctrl Pts',(42.5334738337986,-57.8899079106368,
-46.519518105451));
#239639=CARTESIAN_POINT('Ctrl Pts',(42.6057676504509,-58.1477543480952,
-46.504383611167));
#239640=CARTESIAN_POINT('Ctrl Pts',(42.8438059234446,-58.6145919678895,
-46.4738570559773));
#239641=CARTESIAN_POINT('Ctrl Pts',(43.0050863640377,-58.8202345987045,
-46.4587643581541));
#239642=CARTESIAN_POINT('Ctrl Pts',(43.3948153248215,-59.1566472643482,
-46.4304023184461));
#239643=CARTESIAN_POINT('Ctrl Pts',(43.6187946416987,-59.2851179128159,
-46.4180675393028));
#239644=CARTESIAN_POINT('Ctrl Pts',(44.0695283912006,-59.4392184739542,
-46.3917747372486));
#239645=CARTESIAN_POINT('Ctrl Pts',(44.2881621760599,-59.475452478349,-46.3790210997985));
#239646=CARTESIAN_POINT('Ctrl Pts',(44.5079524583206,-59.475452478349,-46.3662));
#239647=CARTESIAN_POINT('Origin',(44.5079524583206,-57.475452478349,235.35105));
#239648=CARTESIAN_POINT('',(44.5079524583206,-59.475452478349,-45.6662));
#239649=CARTESIAN_POINT('',(44.5079524583206,-59.475452478349,-45.8249500000001));
#239650=CARTESIAN_POINT('',(44.5079524583206,-59.475452478349,235.35105));
#239651=CARTESIAN_POINT('Ctrl Pts',(44.5079524583206,-59.475452478349,-45.8249500000001));
#239652=CARTESIAN_POINT('Ctrl Pts',(44.3649863637798,-59.475452478349,-45.8332896888483));
#239653=CARTESIAN_POINT('Ctrl Pts',(44.2220900392258,-59.4601227788311,
-45.8416253077807));
#239654=CARTESIAN_POINT('Ctrl Pts',(43.8342749498873,-59.375535093521,-45.8642478546587));
#239655=CARTESIAN_POINT('Ctrl Pts',(43.5993670496297,-59.275060254976,-45.8772042214215));
#239656=CARTESIAN_POINT('Ctrl Pts',(43.1695971414633,-58.9851348581437,
-45.9043856713432));
#239657=CARTESIAN_POINT('Ctrl Pts',(42.9814564463317,-58.7945819919116,
-45.9194994862883));
#239658=CARTESIAN_POINT('Ctrl Pts',(42.6938360810368,-58.3564016474037,
-45.9500244733467));
#239659=CARTESIAN_POINT('Ctrl Pts',(42.5950997064634,-58.1142844010626,
-45.9651355992899));
#239660=CARTESIAN_POINT('Ctrl Pts',(42.4961107636773,-57.6091390557547,
-45.9935417843835));
#239661=CARTESIAN_POINT('Ctrl Pts',(42.4955089275564,-57.3511552825602,
-46.0058663278879));
#239662=CARTESIAN_POINT('Ctrl Pts',(42.5934707759449,-56.8385875537474,
-46.0346175211341));
#239663=CARTESIAN_POINT('Ctrl Pts',(42.6951126763407,-56.5897747239274,
-46.0501516400613));
#239664=CARTESIAN_POINT('Ctrl Pts',(42.9841901064911,-56.1549598604126,
-46.0805491069759));
#239665=CARTESIAN_POINT('Ctrl Pts',(43.1655930810649,-55.9709051582107,
-46.0951381298556));
#239666=CARTESIAN_POINT('Ctrl Pts',(43.593873124054,-55.6771926934943,-46.1224674410341));
#239667=CARTESIAN_POINT('Ctrl Pts',(43.8382044477795,-55.5726244620485,
-46.1358813660518));
#239668=CARTESIAN_POINT('Ctrl Pts',(44.3530189412511,-55.4642160359475,
-46.1659122115043));
#239669=CARTESIAN_POINT('Ctrl Pts',(44.6183716492554,-55.4612821467786,
-46.1813911194712));
#239670=CARTESIAN_POINT('Ctrl Pts',(45.1257945209625,-55.5564658975393,
-46.2109907869875));
#239671=CARTESIAN_POINT('Ctrl Pts',(45.3636825728427,-55.6501031130295,
-46.2243621912732));
#239672=CARTESIAN_POINT('Ctrl Pts',(45.8017731021026,-55.9274397505774,
-46.2511503651651));
#239673=CARTESIAN_POINT('Ctrl Pts',(45.995352296195,-56.1124009356582,-46.2661403216174));
#239674=CARTESIAN_POINT('Ctrl Pts',(46.2960219183106,-56.5425664516416,
-46.2966410177018));
#239675=CARTESIAN_POINT('Ctrl Pts',(46.4019490570959,-56.782442098733,-46.311848632824));
#239676=CARTESIAN_POINT('Ctrl Pts',(46.5150170033861,-57.2842975723613,
-46.3404992572935));
#239677=CARTESIAN_POINT('Ctrl Pts',(46.5230297623749,-57.541077598839,-46.3528255048842));
#239678=CARTESIAN_POINT('Ctrl Pts',(46.4403452397433,-58.0560713358598,
-46.3812536669056));
#239679=CARTESIAN_POINT('Ctrl Pts',(46.3456890407522,-58.3084922745376,
-46.3967663111878));
#239680=CARTESIAN_POINT('Ctrl Pts',(46.0683213604673,-58.7526217442415,
-46.4272928003906));
#239681=CARTESIAN_POINT('Ctrl Pts',(45.8916436383633,-58.9421993412834,
-46.4420230098285));
#239682=CARTESIAN_POINT('Ctrl Pts',(45.472839989253,-59.2466363315248,-46.4696177093593));
#239683=CARTESIAN_POINT('Ctrl Pts',(45.2337803403992,-59.3572856056787,
-46.4826100402123));
#239684=CARTESIAN_POINT('Ctrl Pts',(44.8252063906043,-59.4565575163686,
-46.506443520617));
#239685=CARTESIAN_POINT('Ctrl Pts',(44.6666737061617,-59.475452478349,-46.5156912605427));
#239686=CARTESIAN_POINT('Ctrl Pts',(44.5079524583206,-59.475452478349,-46.5249500000001));
#239687=CARTESIAN_POINT('Ctrl Pts',(44.5079524583206,-59.475452478349,-46.3662));
#239688=CARTESIAN_POINT('Ctrl Pts',(44.5533920533117,-59.475452478349,-46.3635493569588));
#239689=CARTESIAN_POINT('Ctrl Pts',(44.5988810789836,-59.4739039391127,
-46.3608958304612));
#239690=CARTESIAN_POINT('Ctrl Pts',(44.899651414889,-59.453345274133,-46.3433508942001));
#239691=CARTESIAN_POINT('Ctrl Pts',(45.1492944950089,-59.3870507353323,
-46.3287883811931));
#239692=CARTESIAN_POINT('Ctrl Pts',(45.616966533528,-59.16056274243,-46.3015075122795));
#239693=CARTESIAN_POINT('Ctrl Pts',(45.8292134984025,-58.9998603054208,
-46.2880068140626));
#239694=CARTESIAN_POINT('Ctrl Pts',(46.1785109975564,-58.6060430867782,
-46.2579240535827));
#239695=CARTESIAN_POINT('Ctrl Pts',(46.3124015001476,-58.3770974501211,
-46.2424530042404));
#239696=CARTESIAN_POINT('Ctrl Pts',(46.4809988880742,-57.8893355595287,
-46.2128947527779));
#239697=CARTESIAN_POINT('Ctrl Pts',(46.5174955209621,-57.6363536693044,
-46.1996067695942));
#239698=CARTESIAN_POINT('Ctrl Pts',(46.4936168806862,-57.1184425749291,
-46.1727463996494));
#239699=CARTESIAN_POINT('Ctrl Pts',(46.4288444702513,-56.8586490605961,
-46.1577329169946));
#239700=CARTESIAN_POINT('Ctrl Pts',(46.2041759466876,-56.3844779714447,
-46.1272258395355));
#239701=CARTESIAN_POINT('Ctrl Pts',(46.0483810452414,-56.173723684135,-46.112034905182));
#239702=CARTESIAN_POINT('Ctrl Pts',(45.6684898985691,-55.8267904777021,
-46.0834283234764));
#239703=CARTESIAN_POINT('Ctrl Pts',(45.4492645527083,-55.6925164292725,
-46.0711098721726));
#239704=CARTESIAN_POINT('Ctrl Pts',(44.9609109157122,-55.5092348402656,
-46.0426225766812));
#239705=CARTESIAN_POINT('Ctrl Pts',(44.6948966776886,-55.466421146957,-46.0271050794631));
#239706=CARTESIAN_POINT('Ctrl Pts',(44.1719552637017,-55.4872490067109,
-45.9966001636472));
#239707=CARTESIAN_POINT('Ctrl Pts',(43.9198615833972,-55.5467139895591,
-45.9818946989627));
#239708=CARTESIAN_POINT('Ctrl Pts',(43.4476238767116,-55.7596422861188,
-45.9543474994061));
#239709=CARTESIAN_POINT('Ctrl Pts',(43.2327420701107,-55.9127100154752,
-45.9412865529017));
#239710=CARTESIAN_POINT('Ctrl Pts',(42.8725171468024,-56.2944482407933,
-45.9114952842631));
#239711=CARTESIAN_POINT('Ctrl Pts',(42.7313301285655,-56.5199282406862,
-45.8959864974339));
#239712=CARTESIAN_POINT('Ctrl Pts',(42.5479060980174,-57.0036014693219,
-45.8662023538604));
#239713=CARTESIAN_POINT('Ctrl Pts',(42.5039330557245,-57.2558153013869,
-45.8524128961093));
#239714=CARTESIAN_POINT('Ctrl Pts',(42.5127439979152,-57.7745160849174,
-45.8259521070579));
#239715=CARTESIAN_POINT('Ctrl Pts',(42.5699147052662,-58.0360366126589,
-45.8110730952231));
#239716=CARTESIAN_POINT('Ctrl Pts',(42.7809365385862,-58.5171802899984,
-45.7806118039836));
#239717=CARTESIAN_POINT('Ctrl Pts',(42.931066783459,-58.7329207418088,-45.7653341969811));
#239718=CARTESIAN_POINT('Ctrl Pts',(43.3010156764702,-59.0903304477651,
-45.7364883443148));
#239719=CARTESIAN_POINT('Ctrl Pts',(43.5156109547163,-59.2303813196796,
-45.7240865877101));
#239720=CARTESIAN_POINT('Ctrl Pts',(43.9911480609499,-59.4249145608405,
-45.6963469231798));
#239721=CARTESIAN_POINT('Ctrl Pts',(44.2483722690796,-59.475452478349,-45.6813421777057));
#239722=CARTESIAN_POINT('Ctrl Pts',(44.5079524583206,-59.475452478349,-45.6662));
#239723=CARTESIAN_POINT('Origin',(44.5079524583206,-57.475452478349,235.35105));
#239724=CARTESIAN_POINT('',(44.5079524583206,-59.475452478349,-44.9662));
#239725=CARTESIAN_POINT('',(44.5079524583206,-59.475452478349,-45.1249500000001));
#239726=CARTESIAN_POINT('',(44.5079524583206,-59.475452478349,235.35105));
#239727=CARTESIAN_POINT('Ctrl Pts',(44.5079524583206,-59.475452478349,-45.1249500000001));
#239728=CARTESIAN_POINT('Ctrl Pts',(44.3289485674432,-59.475452478349,-45.1353918936346));
#239729=CARTESIAN_POINT('Ctrl Pts',(44.1503748551903,-59.4514192683433,
-45.1458086935161));
#239730=CARTESIAN_POINT('Ctrl Pts',(43.732385405699,-59.3363422420862,-45.1701914114031));
#239731=CARTESIAN_POINT('Ctrl Pts',(43.5027963386504,-59.2230401662548,
-45.1826488257283));
#239732=CARTESIAN_POINT('Ctrl Pts',(43.0869374091872,-58.9080994510816,
-45.2106882663391));
#239733=CARTESIAN_POINT('Ctrl Pts',(42.9080664507182,-58.7051234786716,
-45.2261593062883));
#239734=CARTESIAN_POINT('Ctrl Pts',(42.6460245302134,-58.249764899943,-45.2568060679619));
#239735=CARTESIAN_POINT('Ctrl Pts',(42.5618699260756,-58.0037788926928,
-45.2716873349057));
#239736=CARTESIAN_POINT('Ctrl Pts',(42.4913598877592,-57.4922932120912,
-45.2995831872859));
#239737=CARTESIAN_POINT('Ctrl Pts',(42.5060818538212,-57.2316212385311,
-45.3122133434975));
#239738=CARTESIAN_POINT('Ctrl Pts',(42.6354663213177,-56.7246010300115,
-45.3416007793467));
#239739=CARTESIAN_POINT('Ctrl Pts',(42.7510853474001,-56.4837937980965,
-45.3571381364555));
#239740=CARTESIAN_POINT('Ctrl Pts',(43.0633231251013,-56.0690871789363,
-45.3871952822316));
#239741=CARTESIAN_POINT('Ctrl Pts',(43.2539216026626,-55.8967600573789,
-45.4014600516205));
#239742=CARTESIAN_POINT('Ctrl Pts',(43.6984473177722,-55.627495460869,-45.4280281338647));
#239743=CARTESIAN_POINT('Ctrl Pts',(43.9502613805181,-55.5365564921131,
-45.4424180204615));
#239744=CARTESIAN_POINT('Ctrl Pts',(44.4710062930961,-55.4587926522892,
-45.4727948070285));
#239745=CARTESIAN_POINT('Ctrl Pts',(44.7345321573533,-55.4712190921781,
-45.4881671491102));
#239746=CARTESIAN_POINT('Ctrl Pts',(45.2342145752133,-55.5948235845074,
-45.517315290152));
#239747=CARTESIAN_POINT('Ctrl Pts',(45.4663606805312,-55.7018539653741,
-45.5299713266606));
#239748=CARTESIAN_POINT('Ctrl Pts',(45.8880149955959,-56.0037936314747,
-45.5575230104231));
#239749=CARTESIAN_POINT('Ctrl Pts',(46.0707759682939,-56.1995620811647,
-45.5727433984171));
#239750=CARTESIAN_POINT('Ctrl Pts',(46.3456644749568,-56.6450653435323,
-45.6032669798511));
#239751=CARTESIAN_POINT('Ctrl Pts',(46.4374570994028,-56.8891365027887,
-45.6182742878118));
#239752=CARTESIAN_POINT('Ctrl Pts',(46.5228815768366,-57.3973557454645,
-45.6464401302699));
#239753=CARTESIAN_POINT('Ctrl Pts',(46.5162444921619,-57.6565754485845,
-45.6588581461298));
#239754=CARTESIAN_POINT('Ctrl Pts',(46.4034008475248,-58.166614580002,-45.6879156517078));
#239755=CARTESIAN_POINT('Ctrl Pts',(46.295070642816,-58.4117320342241,-45.7034581626441));
#239756=CARTESIAN_POINT('Ctrl Pts',(45.9948641831446,-58.8371781813898,
-45.7337069360488));
#239757=CARTESIAN_POINT('Ctrl Pts',(45.8090163519768,-59.0157376485121,
-45.748147991477));
#239758=CARTESIAN_POINT('Ctrl Pts',(45.3715180164748,-59.29886832691,-45.7752115972674));
#239759=CARTESIAN_POINT('Ctrl Pts',(45.1218896599051,-59.3973609193807,
-45.7891369965743));
#239760=CARTESIAN_POINT('Ctrl Pts',(44.7436924583087,-59.4650367847731,
-45.8111985000008));
#239761=CARTESIAN_POINT('Ctrl Pts',(44.6257987552545,-59.475452478349,-45.8180756326789));
#239762=CARTESIAN_POINT('Ctrl Pts',(44.5079524583206,-59.475452478349,-45.8249500000001));
#239763=CARTESIAN_POINT('Ctrl Pts',(44.5079524583206,-59.475452478349,-45.6662));
#239764=CARTESIAN_POINT('Ctrl Pts',(44.5157509961426,-59.475452478349,-45.6657450852937));
#239765=CARTESIAN_POINT('Ctrl Pts',(44.5235516604141,-59.4754068654962,
-45.6652900465444));
#239766=CARTESIAN_POINT('Ctrl Pts',(44.7886381494436,-59.472304928927,-45.6498266680177));
#239767=CARTESIAN_POINT('Ctrl Pts',(45.0429716896782,-59.4196722948256,
-45.6349905448373));
#239768=CARTESIAN_POINT('Ctrl Pts',(45.5196054658849,-59.2201090456352,
-45.6071869078919));
#239769=CARTESIAN_POINT('Ctrl Pts',(45.7370574577538,-59.0743841677975,
-45.5944595061318));
#239770=CARTESIAN_POINT('Ctrl Pts',(46.1077220718494,-58.7045045479164,
-45.5649628213031));
#239771=CARTESIAN_POINT('Ctrl Pts',(46.2559338267876,-58.4826175982597,
-45.5494306605658));
#239772=CARTESIAN_POINT('Ctrl Pts',(46.4537453137754,-58.0032564081277,
-45.5194447190478));
#239773=CARTESIAN_POINT('Ctrl Pts',(46.5050493459787,-57.7517456048985,
-45.5052424913214));
#239774=CARTESIAN_POINT('Ctrl Pts',(46.5107317100971,-57.2323610559215,
-45.4788384098993));
#239775=CARTESIAN_POINT('Ctrl Pts',(46.4609415843893,-56.9693311808515,
-45.4642605386169));
#239776=CARTESIAN_POINT('Ctrl Pts',(46.2631116586593,-56.4816894154821,
-45.4338557399724));
#239777=CARTESIAN_POINT('Ctrl Pts',(46.1185508664246,-56.2613144328984,
-45.4185064474244));
#239778=CARTESIAN_POINT('Ctrl Pts',(45.75819622982,-55.8939441087259,-45.3894372352459));
#239779=CARTESIAN_POINT('Ctrl Pts',(45.5479104800947,-55.7483896228915,
-45.3768642179368));
#239780=CARTESIAN_POINT('Ctrl Pts',(45.0733945528864,-55.5387974566262,
-45.349184122183));
#239781=CARTESIAN_POINT('Ctrl Pts',(44.8118810224575,-55.4809731764661,
-45.3339291662413));
#239782=CARTESIAN_POINT('Ctrl Pts',(44.2887266335646,-55.4708223858735,
-45.3034118268891));
#239783=CARTESIAN_POINT('Ctrl Pts',(44.0321282941721,-55.5158043248852,
-45.2884435904246));
#239784=CARTESIAN_POINT('Ctrl Pts',(43.5507578965307,-55.7006049862007,
-45.2603636505621));
#239785=CARTESIAN_POINT('Ctrl Pts',(43.3304798078508,-55.8384219509829,
-45.2478901323969));
#239786=CARTESIAN_POINT('Ctrl Pts',(42.9486499874786,-56.1952720441168,
-45.2187260232862));
#239787=CARTESIAN_POINT('Ctrl Pts',(42.7928819508842,-56.4130014215983,
-45.2031835038493));
#239788=CARTESIAN_POINT('Ctrl Pts',(42.5794177640479,-56.8873761501774,
-45.1729929320579));
#239789=CARTESIAN_POINT('Ctrl Pts',(42.5201861094759,-57.1379495293302,
-45.1586068389411));
#239790=CARTESIAN_POINT('Ctrl Pts',(42.4986533657732,-57.6593362115786,
-45.1316393107151));
#239791=CARTESIAN_POINT('Ctrl Pts',(42.5410319282442,-57.9253301041547,
-45.1175081973955));
#239792=CARTESIAN_POINT('Ctrl Pts',(42.7259619103225,-58.4204550598936,
-45.0871016101847));
#239793=CARTESIAN_POINT('Ctrl Pts',(42.8648098408148,-58.6453274923437,
-45.0716917399305));
#239794=CARTESIAN_POINT('Ctrl Pts',(43.2154792362735,-59.0226036586122,
-45.0424045891495));
#239795=CARTESIAN_POINT('Ctrl Pts',(43.4215625673015,-59.1736538398396,
-45.0295727436427));
#239796=CARTESIAN_POINT('Ctrl Pts',(43.8899394289875,-59.395973850698,-45.0022507600444));
#239797=CARTESIAN_POINT('Ctrl Pts',(44.1497471451407,-59.4608969960235,
-44.9870953099354));
#239798=CARTESIAN_POINT('Ctrl Pts',(44.4457278897632,-59.4747271146837,
-44.9698297664991));
#239799=CARTESIAN_POINT('Ctrl Pts',(44.4768532435007,-59.475452478349,-44.9680141208644));
#239800=CARTESIAN_POINT('Ctrl Pts',(44.5079524583206,-59.475452478349,-44.9662));
#239801=CARTESIAN_POINT('Origin',(44.5079524583206,-57.475452478349,235.35105));
#239802=CARTESIAN_POINT('',(44.5079524583206,-59.475452478349,-44.2662));
#239803=CARTESIAN_POINT('',(44.5079524583206,-59.475452478349,-44.4249500000001));
#239804=CARTESIAN_POINT('',(44.5079524583206,-59.475452478349,235.35105));
#239805=CARTESIAN_POINT('Ctrl Pts',(44.5079524583206,-59.475452478349,-44.4249500000001));
#239806=CARTESIAN_POINT('Ctrl Pts',(44.283285075366,-59.475452478349,-44.4380555973391));
#239807=CARTESIAN_POINT('Ctrl Pts',(44.059893467904,-59.4375926222143,-44.4510867744411));
#239808=CARTESIAN_POINT('Ctrl Pts',(43.6059949604271,-59.2787307478272,
-44.4775641873773));
#239809=CARTESIAN_POINT('Ctrl Pts',(43.383184097842,-59.1488432296001,-44.4898858079534));
#239810=CARTESIAN_POINT('Ctrl Pts',(42.995841679397,-58.8098650069049,-44.5183078473687));
#239811=CARTESIAN_POINT('Ctrl Pts',(42.8358801787966,-58.6029666331937,
-44.533425513915));
#239812=CARTESIAN_POINT('Ctrl Pts',(42.601071027619,-58.1343109279424,-44.5639497326963));
#239813=CARTESIAN_POINT('Ctrl Pts',(42.5306006882951,-57.8759703986851,
-44.5790560028278));
#239814=CARTESIAN_POINT('Ctrl Pts',(42.4953680131583,-57.3587530563562,
-44.6062124850538));
#239815=CARTESIAN_POINT('Ctrl Pts',(42.5262810842606,-57.1051357115976,
-44.6191923023582));
#239816=CARTESIAN_POINT('Ctrl Pts',(42.6838553056735,-56.6144270951757,
-44.6485779079306));
#239817=CARTESIAN_POINT('Ctrl Pts',(42.8122660918713,-56.3830514562381,
-44.6640118914276));
#239818=CARTESIAN_POINT('Ctrl Pts',(43.1532878715183,-55.9803118855556,
-44.694304017461));
#239819=CARTESIAN_POINT('Ctrl Pts',(43.3635660886199,-55.8138619965146,
-44.7081941284342));
#239820=CARTESIAN_POINT('Ctrl Pts',(43.827805132134,-55.577383175988,-44.7352747393058));
#239821=CARTESIAN_POINT('Ctrl Pts',(44.0755315270225,-55.5061283512199,
-44.7497254456743));
#239822=CARTESIAN_POINT('Ctrl Pts',(44.594254452503,-55.4597669706736,-44.779984282994));
#239823=CARTESIAN_POINT('Ctrl Pts',(44.8606946758697,-55.4889912576162,
-44.795526629357));
#239824=CARTESIAN_POINT('Ctrl Pts',(45.3584959850637,-55.6471822161361,
-44.82456503906));
#239825=CARTESIAN_POINT('Ctrl Pts',(45.5860068450698,-55.7714009808656,
-44.8369743929198));
#239826=CARTESIAN_POINT('Ctrl Pts',(45.9828340158242,-56.1001338486245,
-44.8651554945815));
#239827=CARTESIAN_POINT('Ctrl Pts',(46.147989864832,-56.3019840430269,-44.880169638284));
#239828=CARTESIAN_POINT('Ctrl Pts',(46.3955717459517,-56.7632686316113,
-44.9106940198552));
#239829=CARTESIAN_POINT('Ctrl Pts',(46.4732810656571,-57.01956335981,-44.9259080768327));
#239830=CARTESIAN_POINT('Ctrl Pts',(46.5230334210941,-57.5357649746953,
-44.9534367370643));
#239831=CARTESIAN_POINT('Ctrl Pts',(46.4992097142434,-57.7902666281475,
-44.9661088246886));
#239832=CARTESIAN_POINT('Ctrl Pts',(46.3555497542076,-58.2845863549509,
-44.9952710242482));
#239833=CARTESIAN_POINT('Ctrl Pts',(46.2341137483518,-58.5188473904699,
-45.0106473413109));
#239834=CARTESIAN_POINT('Ctrl Pts',(45.9125846210923,-58.9216731144069,
-45.0403752844146));
#239835=CARTESIAN_POINT('Ctrl Pts',(45.717770169913,-59.0881462927263,-45.0543773001572));
#239836=CARTESIAN_POINT('Ctrl Pts',(45.266724227889,-59.3448244804227,-45.0806883134419));
#239837=CARTESIAN_POINT('Ctrl Pts',(45.0125641481616,-59.4288087849436,
-45.0955143180927));
#239838=CARTESIAN_POINT('Ctrl Pts',(44.6691833888416,-59.4705837361307,
-45.1155448623864));
#239839=CARTESIAN_POINT('Ctrl Pts',(44.5885243462159,-59.475452478349,-45.1202499732062));
#239840=CARTESIAN_POINT('Ctrl Pts',(44.5079524583206,-59.475452478349,-45.1249500000001));
#239841=CARTESIAN_POINT('Ctrl Pts',(44.5079524583206,-59.475452478349,-44.9662));
#239842=CARTESIAN_POINT('Ctrl Pts',(44.7350982804284,-59.475452478349,-44.9529498270437));
#239843=CARTESIAN_POINT('Ctrl Pts',(44.9608496675886,-59.436753282891,-44.939780996126));
#239844=CARTESIAN_POINT('Ctrl Pts',(45.4168910322583,-59.2752972816714,
-44.913178583187));
#239845=CARTESIAN_POINT('Ctrl Pts',(45.6396497792772,-59.1442463664141,
-44.9008298723489));
#239846=CARTESIAN_POINT('Ctrl Pts',(46.0309656080461,-58.7987492821338,
-44.8719626209811));
#239847=CARTESIAN_POINT('Ctrl Pts',(46.1931757392732,-58.5848144534829,
-44.856423900699));
#239848=CARTESIAN_POINT('Ctrl Pts',(46.4200729111258,-58.1151528227274,
-44.8260796304873));
#239849=CARTESIAN_POINT('Ctrl Pts',(46.4861472020093,-57.8655894967344,
-44.8115449864937));
#239850=CARTESIAN_POINT('Ctrl Pts',(46.5212095777296,-57.346811429197,-44.7843146263861));
#239851=CARTESIAN_POINT('Ctrl Pts',(46.4866571426256,-57.0823550036448,
-44.7707203300023));
#239852=CARTESIAN_POINT('Ctrl Pts',(46.317248794841,-56.5836176484322,-44.7405839653918));
#239853=CARTESIAN_POINT('Ctrl Pts',(46.184686832037,-56.3540763338423,-44.7251215725803));
#239854=CARTESIAN_POINT('Ctrl Pts',(45.8445238885936,-55.966225588339,-44.6956066518184));
#239855=CARTESIAN_POINT('Ctrl Pts',(45.6428432591009,-55.8092718386522,
-44.6824019633789));
#239856=CARTESIAN_POINT('Ctrl Pts',(45.1810933209143,-55.5735574485446,
-44.655466550318));
#239857=CARTESIAN_POINT('Ctrl Pts',(44.9233064714477,-55.5011783070721,
-44.6404289840991));
#239858=CARTESIAN_POINT('Ctrl Pts',(44.4002298059176,-55.4615698607251,
-44.6099161786099));
#239859=CARTESIAN_POINT('Ctrl Pts',(44.1401193669863,-55.4925138456731,
-44.5947430696722));
#239860=CARTESIAN_POINT('Ctrl Pts',(43.6505122983323,-55.6506718760281,
-44.566182657334));
#239861=CARTESIAN_POINT('Ctrl Pts',(43.4251218828497,-55.774716568916,-44.5538688042061));
#239862=CARTESIAN_POINT('Ctrl Pts',(43.024056446069,-56.1082818723179,-44.5253199607502));
#239863=CARTESIAN_POINT('Ctrl Pts',(42.855220178695,-56.3180624394509,-44.5097978437643));
#239864=CARTESIAN_POINT('Ctrl Pts',(42.614417600695,-56.78241231548,-44.4793163392209));
#239865=CARTESIAN_POINT('Ctrl Pts',(42.5412209361295,-57.030724894256,-44.464637144762));
#239866=CARTESIAN_POINT('Ctrl Pts',(42.4921545656837,-57.5467009642602,
-44.4371398865358));
#239867=CARTESIAN_POINT('Ctrl Pts',(42.5187614856851,-57.8096136419463,
-44.4240035333981));
#239868=CARTESIAN_POINT('Ctrl Pts',(42.6722426971373,-58.3118196887116,
-44.3941564783888));
#239869=CARTESIAN_POINT('Ctrl Pts',(42.7981854105964,-58.5459812622667,
-44.3786537400878));
#239870=CARTESIAN_POINT('Ctrl Pts',(43.1274214550792,-58.9446382608674,
-44.3489116086462));
#239871=CARTESIAN_POINT('Ctrl Pts',(43.3246810481936,-59.1076771589167,
-44.3352241655906));
#239872=CARTESIAN_POINT('Ctrl Pts',(43.7795874523815,-59.3568840913519,
-44.3086879586797));
#239873=CARTESIAN_POINT('Ctrl Pts',(44.0351047616619,-59.4367442456094,
-44.293782782305));
#239874=CARTESIAN_POINT('Ctrl Pts',(44.3683379691323,-59.4718019510095,
-44.2743441785359));
#239875=CARTESIAN_POINT('Ctrl Pts',(44.4381850249233,-59.475452478349,-44.2702697669481));
#239876=CARTESIAN_POINT('Ctrl Pts',(44.5079524583206,-59.475452478349,-44.2662));
#239877=CARTESIAN_POINT('Origin',(44.5079524583206,-57.475452478349,235.35105));
#239878=CARTESIAN_POINT('',(44.5079524583206,-59.475452478349,-43.5662));
#239879=CARTESIAN_POINT('',(44.5079524583206,-59.475452478349,-43.7249500000001));
#239880=CARTESIAN_POINT('',(44.5079524583206,-59.475452478349,235.35105));
#239881=CARTESIAN_POINT('Ctrl Pts',(44.5079524583206,-59.475452478349,-43.7249500000001));
#239882=CARTESIAN_POINT('Ctrl Pts',(44.2436230538572,-59.475452478349,-43.7403692152604));
#239883=CARTESIAN_POINT('Ctrl Pts',(43.9818301375788,-59.4230492364018,
-43.7556404687101));
#239884=CARTESIAN_POINT('Ctrl Pts',(43.5034961874671,-59.2234533329351,
-43.7835432824667));
#239885=CARTESIAN_POINT('Ctrl Pts',(43.2899979499798,-59.0820135561926,
-43.7959798486351));
#239886=CARTESIAN_POINT('Ctrl Pts',(42.9224596309662,-58.7220874350348,
-43.8248825175301));
#239887=CARTESIAN_POINT('Ctrl Pts',(42.7737196678051,-58.5051659915419,
-43.8401792361626));
#239888=CARTESIAN_POINT('Ctrl Pts',(42.5660236645173,-58.0223988037884,
-43.8706255407665));
#239889=CARTESIAN_POINT('Ctrl Pts',(42.5106943495575,-57.7604958177748,
-43.885470166407));
#239890=CARTESIAN_POINT('Ctrl Pts',(42.5055223779315,-57.2416260954196,
-43.9118333532936));
#239891=CARTESIAN_POINT('Ctrl Pts',(42.5513139929662,-56.9895851188607,
-43.9257598308716));
#239892=CARTESIAN_POINT('Ctrl Pts',(42.7383531367516,-56.5069313848787,
-43.9555979122654));
#239893=CARTESIAN_POINT('Ctrl Pts',(42.8813051785868,-56.2823301133647,
-43.9711137872188));
#239894=CARTESIAN_POINT('Ctrl Pts',(43.2441597913404,-55.9035495656452,
-44.0008323387365));
#239895=CARTESIAN_POINT('Ctrl Pts',(43.459683452574,-55.7523269100348,-44.0138009746649));
#239896=CARTESIAN_POINT('Ctrl Pts',(43.9330253986036,-55.5427265246074,
-44.0414125881832));
#239897=CARTESIAN_POINT('Ctrl Pts',(44.1856933327387,-55.484953837572,-44.0561515510078));
#239898=CARTESIAN_POINT('Ctrl Pts',(44.7091334295394,-55.4677711128755,
-44.0866855566545));
#239899=CARTESIAN_POINT('Ctrl Pts',(44.9750329771393,-55.5125150255964,
-44.1021963635978));
#239900=CARTESIAN_POINT('Ctrl Pts',(45.4620095151533,-55.69933629957,-44.1306033283153));
#239901=CARTESIAN_POINT('Ctrl Pts',(45.6800767517487,-55.8350428842699,
-44.1429331696617));
#239902=CARTESIAN_POINT('Ctrl Pts',(46.0575155752788,-56.1845748082541,
-44.1715995076749));
#239903=CARTESIAN_POINT('Ctrl Pts',(46.2119240342626,-56.3965760234397,
-44.186812996611));
#239904=CARTESIAN_POINT('Ctrl Pts',(46.4332379459014,-56.8725081731857,
-44.217311196743));
#239905=CARTESIAN_POINT('Ctrl Pts',(46.4961347650193,-57.1327501044986,
-44.2322926278467));
#239906=CARTESIAN_POINT('Ctrl Pts',(46.5162880877179,-57.650870144721,-44.2590548982529));
#239907=CARTESIAN_POINT('Ctrl Pts',(46.4779505554758,-57.903654212139,-44.2724570142984));
#239908=CARTESIAN_POINT('Ctrl Pts',(46.3057086310559,-58.3904246214665,
-44.3020714769441));
#239909=CARTESIAN_POINT('Ctrl Pts',(46.1700163462968,-58.6185391547815,
-44.3175530924643));
#239910=CARTESIAN_POINT('Ctrl Pts',(45.818011324453,-59.0093951996859,-44.3475652293412));
#239911=CARTESIAN_POINT('Ctrl Pts',(45.6051158043426,-59.1682108024561,
-44.3609488048155));
#239912=CARTESIAN_POINT('Ctrl Pts',(45.1363159779013,-59.3913787735358,
-44.3882954613579));
#239913=CARTESIAN_POINT('Ctrl Pts',(44.886056630806,-59.4560112053162,-44.4028939232718));
#239914=CARTESIAN_POINT('Ctrl Pts',(44.5896200096801,-59.4742032392965,
-44.4201860595041));
#239915=CARTESIAN_POINT('Ctrl Pts',(44.5487651838402,-59.475452478349,-44.4225692576781));
#239916=CARTESIAN_POINT('Ctrl Pts',(44.5079524583206,-59.475452478349,-44.4249500000001));
#239917=CARTESIAN_POINT('Ctrl Pts',(44.5079524583206,-59.475452478349,-44.2662));
#239918=CARTESIAN_POINT('Ctrl Pts',(44.6974398807997,-59.475452478349,-44.255146567022));
#239919=CARTESIAN_POINT('Ctrl Pts',(44.8863399620151,-59.4485215007381,
-44.2441273956178));
#239920=CARTESIAN_POINT('Ctrl Pts',(45.3128592425604,-59.3238888304483,
-44.2192471042526));
#239921=CARTESIAN_POINT('Ctrl Pts',(45.5409384166266,-59.2067880626703,
-44.2068684444618));
#239922=CARTESIAN_POINT('Ctrl Pts',(45.9515891183784,-58.8852182334852,
-44.1786460199261));
#239923=CARTESIAN_POINT('Ctrl Pts',(46.1269323684712,-58.6797772042736,
-44.1631533413656));
#239924=CARTESIAN_POINT('Ctrl Pts',(46.3814819126568,-58.2211232935122,
-44.1325586332614));
#239925=CARTESIAN_POINT('Ctrl Pts',(46.4617598831783,-57.9742579987788,
-44.1177460148224));
#239926=CARTESIAN_POINT('Ctrl Pts',(46.5246934873947,-57.4611581443313,
-44.089989596696));
#239927=CARTESIAN_POINT('Ctrl Pts',(46.5058092502291,-57.1997136035875,
-44.0772076723267));
#239928=CARTESIAN_POINT('Ctrl Pts',(46.3679525499589,-56.6943283526042,
-44.047655724716));
#239929=CARTESIAN_POINT('Ctrl Pts',(46.2486627364475,-56.4558091263641,
-44.0321268887843));
#239930=CARTESIAN_POINT('Ctrl Pts',(45.9304060416829,-56.046730632363,-44.0021785137235));
#239931=CARTESIAN_POINT('Ctrl Pts',(45.7374537689556,-55.8776432070875,
-43.9880087554335));
#239932=CARTESIAN_POINT('Ctrl Pts',(45.2892709116404,-55.6154130555524,
-43.9616893736779));
#239933=CARTESIAN_POINT('Ctrl Pts',(45.0361497099667,-55.5283193103871,
-43.947011506346));
#239934=CARTESIAN_POINT('Ctrl Pts',(44.514698625747,-55.4585153078826,-43.9165935264332));
#239935=CARTESIAN_POINT('Ctrl Pts',(44.2517792160158,-55.4748358885902,
-43.9012565608655));
#239936=CARTESIAN_POINT('Ctrl Pts',(43.7541456155875,-55.6056693303521,
-43.8722279341739));
#239937=CARTESIAN_POINT('Ctrl Pts',(43.5234314201282,-55.7161871084399,
-43.8596929656892));
#239938=CARTESIAN_POINT('Ctrl Pts',(43.1061464323116,-56.0244873685016,
-43.8319473952074));
#239939=CARTESIAN_POINT('Ctrl Pts',(42.9263072608162,-56.2229661580715,
-43.8166753050625));
#239940=CARTESIAN_POINT('Ctrl Pts',(42.6582653170492,-56.6722124621946,
-43.7861623235068));
#239941=CARTESIAN_POINT('Ctrl Pts',(42.5701785351436,-56.9172430758713,
-43.7712146327592));
#239942=CARTESIAN_POINT('Ctrl Pts',(42.49198937607,-57.4270617299001,-43.7431790211196));
#239943=CARTESIAN_POINT('Ctrl Pts',(42.5025312701276,-57.6869741329687,
-43.7306724356183));
#239944=CARTESIAN_POINT('Ctrl Pts',(42.6233762732508,-58.1955810180198,
-43.7014539115192));
#239945=CARTESIAN_POINT('Ctrl Pts',(42.7352520455834,-58.4386397034046,
-43.6859119933839));
#239946=CARTESIAN_POINT('Ctrl Pts',(43.0413240068088,-58.8589326285793,
-43.6557524740846));
#239947=CARTESIAN_POINT('Ctrl Pts',(43.2294952386905,-59.0344930600324,
-43.6413951585317));
#239948=CARTESIAN_POINT('Ctrl Pts',(43.6719449506611,-59.3118772021662,
-43.614477441967));
#239949=CARTESIAN_POINT('Ctrl Pts',(43.9244866719363,-59.4070341679364,
-43.6002355042056));
#239950=CARTESIAN_POINT('Ctrl Pts',(44.2942567973847,-59.4668961143992,
-43.5786655802211));
#239951=CARTESIAN_POINT('Ctrl Pts',(44.4011409321713,-59.475452478349,-43.5724306723587));
#239952=CARTESIAN_POINT('Ctrl Pts',(44.5079524583206,-59.475452478349,-43.5662));
#239953=CARTESIAN_POINT('Origin',(44.5079524583206,-57.475452478349,235.35105));
#239954=CARTESIAN_POINT('',(44.5079524583206,-59.475452478349,-42.8662));
#239955=CARTESIAN_POINT('',(44.5079524583206,-59.475452478349,-43.0249500000001));
#239956=CARTESIAN_POINT('',(44.5079524583206,-59.475452478349,235.35105));
#239957=CARTESIAN_POINT('Ctrl Pts',(44.5079524583206,-59.475452478349,-43.0249500000001));
#239958=CARTESIAN_POINT('Ctrl Pts',(44.4722388018602,-59.475452478349,-43.0270332966269));
#239959=CARTESIAN_POINT('Ctrl Pts',(44.4364923191056,-59.4744958911332,
-43.0291185081211));
#239960=CARTESIAN_POINT('Ctrl Pts',(44.1359989856678,-59.4583660521796,
-43.046647285905));
#239961=CARTESIAN_POINT('Ctrl Pts',(43.8766562345333,-59.3916474688325,
-43.0617756130545));
#239962=CARTESIAN_POINT('Ctrl Pts',(43.4098580688571,-59.1661054233476,
-43.0890055060523));
#239963=CARTESIAN_POINT('Ctrl Pts',(43.2048354570692,-59.0136468877318,
-43.1019175121918));
#239964=CARTESIAN_POINT('Ctrl Pts',(42.8566633521768,-58.6338410191185,
-43.1312596212102));
#239965=CARTESIAN_POINT('Ctrl Pts',(42.7193017262729,-58.4078389051919,
-43.1466832103306));
#239966=CARTESIAN_POINT('Ctrl Pts',(42.5380790697365,-57.9118297106231,
-43.1770263373216));
#239967=CARTESIAN_POINT('Ctrl Pts',(42.4975777986357,-57.6462053086828,
-43.1910212889106));
#239968=CARTESIAN_POINT('Ctrl Pts',(42.5223320692649,-57.1254309277759,
-43.2180518460084));
#239969=CARTESIAN_POINT('Ctrl Pts',(42.5831890276793,-56.8750805503825,
-43.2324740781846));
#239970=CARTESIAN_POINT('Ctrl Pts',(42.7998504127542,-56.4017908720666,
-43.2627030868609));
#239971=CARTESIAN_POINT('Ctrl Pts',(42.9571553464097,-56.1849454547931,
-43.2782457764289));
#239972=CARTESIAN_POINT('Ctrl Pts',(43.341250259259,-55.8307825783057,-43.3073401975271));
#239973=CARTESIAN_POINT('Ctrl Pts',(43.5621134093721,-55.6945771218292,
-43.3197760554782));
#239974=CARTESIAN_POINT('Ctrl Pts',(44.0444488513265,-55.5128328693985,
-43.3479122895921));
#239975=CARTESIAN_POINT('Ctrl Pts',(44.3014880521876,-55.4694472573116,
-43.3629062429757));
#239976=CARTESIAN_POINT('Ctrl Pts',(44.8247182520767,-55.4829727685835,
-43.3934280046359));
#239977=CARTESIAN_POINT('Ctrl Pts',(45.0858469543679,-55.5424775393722,
-43.4086605122695));
#239978=CARTESIAN_POINT('Ctrl Pts',(45.5589242140665,-55.7550817256449,
-43.4362566857519));
#239979=CARTESIAN_POINT('Ctrl Pts',(45.7682135630241,-55.9019273753259,
-43.4488827073125));
#239980=CARTESIAN_POINT('Ctrl Pts',(46.1263016611398,-56.2716293412843,
-43.4780036023445));
#239981=CARTESIAN_POINT('Ctrl Pts',(46.2695332415759,-56.4930732678543,
-43.4933681272861));
#239982=CARTESIAN_POINT('Ctrl Pts',(46.4642258513371,-56.9821704159436,
-43.523754944122));
#239983=CARTESIAN_POINT('Ctrl Pts',(46.5122916603142,-57.2455411256538,
-43.5382087440721));
#239984=CARTESIAN_POINT('Ctrl Pts',(46.5031811471748,-57.7650743711394,
-43.5647203250463));
#239985=CARTESIAN_POINT('Ctrl Pts',(46.4501535560201,-58.0164025409574,
-43.5789635969404));
#239986=CARTESIAN_POINT('Ctrl Pts',(46.2489308158815,-58.4947227266461,
-43.6089964437248));
#239987=CARTESIAN_POINT('Ctrl Pts',(46.0990677974513,-58.7157274688955,
-43.6245321988292));
#239988=CARTESIAN_POINT('Ctrl Pts',(45.7259584296462,-59.0827848377704,
-43.6539576140789));
#239989=CARTESIAN_POINT('Ctrl Pts',(45.5078951969149,-59.2267831259288,
-43.6666200069155));
#239990=CARTESIAN_POINT('Ctrl Pts',(45.0302272821456,-59.4231562527943,
-43.6944839686103));
#239991=CARTESIAN_POINT('Ctrl Pts',(44.7753855036338,-59.4741443929355,
-43.7093497390236));
#239992=CARTESIAN_POINT('Ctrl Pts',(44.5145975316104,-59.4754441999115,
-43.7245623707249));
#239993=CARTESIAN_POINT('Ctrl Pts',(44.511274794611,-59.475452478349,-43.7247561970498));
#239994=CARTESIAN_POINT('Ctrl Pts',(44.5079524583206,-59.475452478349,-43.7249500000001));
#239995=CARTESIAN_POINT('Ctrl Pts',(44.5079524583206,-59.475452478349,-43.5662));
#239996=CARTESIAN_POINT('Ctrl Pts',(44.6615663204189,-59.475452478349,-43.5572391913776));
#239997=CARTESIAN_POINT('Ctrl Pts',(44.815030002254,-59.4577540742531,-43.5482871432704));
#239998=CARTESIAN_POINT('Ctrl Pts',(45.2118852073288,-59.3645408368662,
-43.5251372563077));
#239999=CARTESIAN_POINT('Ctrl Pts',(45.4451992360649,-59.2603095681955,
-43.512364644595));
#240000=CARTESIAN_POINT('Ctrl Pts',(45.8703347392719,-58.9634915289442,
-43.4849701612844));
#240001=CARTESIAN_POINT('Ctrl Pts',(46.0554114531177,-58.7699314236281,
-43.4697937923094));
#240002=CARTESIAN_POINT('Ctrl Pts',(46.335759964064,-58.3275099888803,-43.4392666489761));
#240003=CARTESIAN_POINT('Ctrl Pts',(46.4305219085137,-58.0842493054552,
-43.424213679587));
#240004=CARTESIAN_POINT('Ctrl Pts',(46.5217447918344,-57.5773321239347,
-43.3959444946762));
#240005=CARTESIAN_POINT('Ctrl Pts',(46.51821469771,-57.3186506821524,-43.3835779788817));
#240006=CARTESIAN_POINT('Ctrl Pts',(46.4117517357226,-56.8075063233078,
-43.3546507425044));
#240007=CARTESIAN_POINT('Ctrl Pts',(46.3062745611358,-56.5607829365096,
-43.3391103162062));
#240008=CARTESIAN_POINT('Ctrl Pts',(46.0108052920072,-56.1312850003737,
-43.3087950219819));
#240009=CARTESIAN_POINT('Ctrl Pts',(45.8268437575018,-55.9503559439615,
-43.2942892762759));
#240010=CARTESIAN_POINT('Ctrl Pts',(45.393296353515,-55.6626715628225,-43.2671108613565));
#240011=CARTESIAN_POINT('Ctrl Pts',(45.1459586054206,-55.5615543425804,
-43.2534170252475));
#240012=CARTESIAN_POINT('Ctrl Pts',(44.6283997479283,-55.4619145925842,
-43.2232260918937));
#240013=CARTESIAN_POINT('Ctrl Pts',(44.3634911982133,-55.463494642993,-43.2077730931604));
#240014=CARTESIAN_POINT('Ctrl Pts',(43.8582876714391,-55.567021828036,-43.1783028874318));
#240015=CARTESIAN_POINT('Ctrl Pts',(43.6221045851968,-55.664542137411,-43.1651799413221));
#240016=CARTESIAN_POINT('Ctrl Pts',(43.1887206949131,-55.9490334918029,
-43.138167601352));
#240017=CARTESIAN_POINT('Ctrl Pts',(42.9982072889421,-56.1371879745595,
-43.1231057442334));
#240018=CARTESIAN_POINT('Ctrl Pts',(42.7049167935935,-56.5719506013494,
-43.0925880351531));
#240019=CARTESIAN_POINT('Ctrl Pts',(42.6030653396854,-56.8131242966944,
-43.0774337191787));
#240020=CARTESIAN_POINT('Ctrl Pts',(42.4979825906407,-57.3168591547252,
-43.048921053275));
#240021=CARTESIAN_POINT('Ctrl Pts',(42.4941611025798,-57.5743100567886,
-43.0366081460423));
#240022=CARTESIAN_POINT('Ctrl Pts',(42.5854895496084,-58.0879526889787,
-43.0079961248739));
#240023=CARTESIAN_POINT('Ctrl Pts',(42.6841124987043,-58.3383556059968,
-42.9924697304316));
#240024=CARTESIAN_POINT('Ctrl Pts',(42.9681399198854,-58.7772535078167,
-42.9620132879096));
#240025=CARTESIAN_POINT('Ctrl Pts',(43.1475109432184,-58.9637215259788,
-42.9473616140203));
#240026=CARTESIAN_POINT('Ctrl Pts',(43.5716778728517,-59.26210764927,-42.9199161640698));
#240027=CARTESIAN_POINT('Ctrl Pts',(43.8136994076378,-59.3693345857257,
-42.9066980946229));
#240028=CARTESIAN_POINT('Ctrl Pts',(44.213802706673,-59.4592184173348,-42.8833587355126));
#240029=CARTESIAN_POINT('Ctrl Pts',(44.3608300508606,-59.475452478349,-42.8747821404351));
#240030=CARTESIAN_POINT('Ctrl Pts',(44.5079524583206,-59.475452478349,-42.8662));
#240031=CARTESIAN_POINT('Origin',(44.5079524583206,-57.475452478349,235.35105));
#240032=CARTESIAN_POINT('',(44.5079524583206,-59.475452478349,-42.1661999999999));
#240033=CARTESIAN_POINT('',(44.5079524583206,-59.475452478349,-42.3249500000001));
#240034=CARTESIAN_POINT('',(44.5079524583206,-59.475452478349,235.35105));
#240035=CARTESIAN_POINT('Ctrl Pts',(44.5079524583206,-59.475452478349,-42.3249500000001));
#240036=CARTESIAN_POINT('Ctrl Pts',(44.4335108999353,-59.475452478349,-42.3292924242392));
#240037=CARTESIAN_POINT('Ctrl Pts',(44.3589857355706,-59.4712964286506,
-42.3336397254938));
#240038=CARTESIAN_POINT('Ctrl Pts',(44.0213468793765,-59.433374420538,-42.3533353254385));
#240039=CARTESIAN_POINT('Ctrl Pts',(43.7664083172945,-59.3517271833582,
-42.3682067415599));
#240040=CARTESIAN_POINT('Ctrl Pts',(43.3131668649557,-59.0992861318309,
-42.3946458262797));
#240041=CARTESIAN_POINT('Ctrl Pts',(43.1169658201907,-58.9347664927564,
-42.408465268112));
#240042=CARTESIAN_POINT('Ctrl Pts',(42.7904022899136,-58.533496628627,-42.4382614483514));
#240043=CARTESIAN_POINT('Ctrl Pts',(42.6660892211492,-58.2982418210313,
-42.4537718835088));
#240044=CARTESIAN_POINT('Ctrl Pts',(42.5164690992943,-57.7952299475756,
-42.4835470322772));
#240045=CARTESIAN_POINT('Ctrl Pts',(42.4917767288961,-57.5326848236753,
-42.4965869357688));
#240046=CARTESIAN_POINT('Ctrl Pts',(42.5442576277417,-57.0174075895169,
-42.5241484805135));
#240047=CARTESIAN_POINT('Ctrl Pts',(42.6191957453779,-56.7694320003765,
-42.5388614432612));
#240048=CARTESIAN_POINT('Ctrl Pts',(42.8633862777626,-56.3064443476726,
-42.5693729461404));
#240049=CARTESIAN_POINT('Ctrl Pts',(43.033830275666,-56.0977115237113,-42.5848890252216));
#240050=CARTESIAN_POINT('Ctrl Pts',(43.4372623221583,-55.7670832112067,
-42.6133585234516));
#240051=CARTESIAN_POINT('Ctrl Pts',(43.6633063090487,-55.6447476374709,
-42.625678974626));
#240052=CARTESIAN_POINT('Ctrl Pts',(44.1539326420176,-55.4899780632874,
-42.6542988440492));
#240053=CARTESIAN_POINT('Ctrl Pts',(44.4144355075536,-55.4608371500119,
-42.6694948445387));
#240054=CARTESIAN_POINT('Ctrl Pts',(44.9373826012068,-55.5041937692303,
-42.7000000916685));
#240055=CARTESIAN_POINT('Ctrl Pts',(45.1946358903184,-55.5784063694658,
-42.7150065335333));
#240056=CARTESIAN_POINT('Ctrl Pts',(45.654727057096,-55.8174215434278,-42.7418451849287));
#240057=CARTESIAN_POINT('Ctrl Pts',(45.8553251402743,-55.9758505920282,
-42.7551579256919));
#240058=CARTESIAN_POINT('Ctrl Pts',(46.1928475373647,-56.366330761512,-42.7847286641498));
#240059=CARTESIAN_POINT('Ctrl Pts',(46.3238168947725,-56.5970106765827,
-42.8002021259589));
#240060=CARTESIAN_POINT('Ctrl Pts',(46.4893558836183,-57.0966124757606,
-42.8302693043756));
#240061=CARTESIAN_POINT('Ctrl Pts',(46.5219705461844,-57.3606901912239,
-42.8437435608347));
#240062=CARTESIAN_POINT('Ctrl Pts',(46.4835176912486,-57.8787993498951,
-42.871039017882));
#240063=CARTESIAN_POINT('Ctrl Pts',(46.4157223067143,-58.1280791453904,
-42.8856095370046));
#240064=CARTESIAN_POINT('Ctrl Pts',(46.1854577537387,-58.5964953000075,
-42.9159891033505));
#240065=CARTESIAN_POINT('Ctrl Pts',(46.0216390045741,-58.8094454681241,
-42.9315249984287));
#240066=CARTESIAN_POINT('Ctrl Pts',(45.627956981107,-59.1520699862854,-42.9603161470866));
#240067=CARTESIAN_POINT('Ctrl Pts',(45.4045661840963,-59.2814259098854,
-42.9726475326633));
#240068=CARTESIAN_POINT('Ctrl Pts',(44.9519576094212,-59.4382730917703,
-42.9990496995194));
#240069=CARTESIAN_POINT('Ctrl Pts',(44.7305929026539,-59.475452478349,-43.0119626407473));
#240070=CARTESIAN_POINT('Ctrl Pts',(44.5079524583206,-59.475452478349,-43.0249500000001));
#240071=CARTESIAN_POINT('Ctrl Pts',(44.5079524583206,-59.475452478349,-42.8662));
#240072=CARTESIAN_POINT('Ctrl Pts',(44.6227546351814,-59.475452478349,-42.8595032063498));
#240073=CARTESIAN_POINT('Ctrl Pts',(44.737614695619,-59.4655679660078,-42.8528030361574));
#240074=CARTESIAN_POINT('Ctrl Pts',(45.1011058928316,-59.4022356541609,
-42.8315993829867));
#240075=CARTESIAN_POINT('Ctrl Pts',(45.3403292438796,-59.3115885970665,
-42.8180138742986));
#240076=CARTESIAN_POINT('Ctrl Pts',(45.7820095842752,-59.0397681873013,
-42.7913996671966));
#240077=CARTESIAN_POINT('Ctrl Pts',(45.9779068823429,-58.8572953967276,
-42.7764678084617));
#240078=CARTESIAN_POINT('Ctrl Pts',(46.2841973240556,-58.4307477847042,
-42.7459859416155));
#240079=CARTESIAN_POINT('Ctrl Pts',(46.393245926337,-58.1919155116682,-42.7307399931335));
#240080=CARTESIAN_POINT('Ctrl Pts',(46.5124415638417,-57.6915264323124,
-42.7019847238606));
#240081=CARTESIAN_POINT('Ctrl Pts',(46.5236508000073,-57.4352399244353,
-42.6896264045268));
#240082=CARTESIAN_POINT('Ctrl Pts',(46.4475620650062,-56.9192521004401,
-42.6613404002113));
#240083=CARTESIAN_POINT('Ctrl Pts',(46.3559566047958,-56.6653329466362,
-42.6458410487559));
#240084=CARTESIAN_POINT('Ctrl Pts',(46.0837290779512,-56.2172806396749,
-42.6152663062198));
#240085=CARTESIAN_POINT('Ctrl Pts',(45.9091403711885,-56.0253578881873,
-42.6004785535353));
#240086=CARTESIAN_POINT('Ctrl Pts',(45.4944319230012,-55.7163332450967,
-42.5727715376367));
#240087=CARTESIAN_POINT('Ctrl Pts',(45.2575957865996,-55.6031026233215,
-42.5599291941495));
#240088=CARTESIAN_POINT('Ctrl Pts',(44.750008238189,-55.4726832794671,-42.5303199204922));
#240089=CARTESIAN_POINT('Ctrl Pts',(44.4838674301552,-55.4582549240482,
-42.5147950400236));
#240090=CARTESIAN_POINT('Ctrl Pts',(43.9711540783505,-55.5321567162246,
-42.4848867611683));
#240091=CARTESIAN_POINT('Ctrl Pts',(43.7288317395534,-55.6159982417038,
-42.4707512914051));
#240092=CARTESIAN_POINT('Ctrl Pts',(43.2791701979494,-55.8753631474548,
-42.4445210348116));
#240093=CARTESIAN_POINT('Ctrl Pts',(43.078139009641,-56.0520943766476,-42.4297358571075));
#240094=CARTESIAN_POINT('Ctrl Pts',(42.7592844524011,-56.4703800500612,
-42.3993049147337));
#240095=CARTESIAN_POINT('Ctrl Pts',(42.6432600435373,-56.7067237562461,
-42.3839812230163));
#240096=CARTESIAN_POINT('Ctrl Pts',(42.5103209946102,-57.2037461827188,
-42.354995181314));
#240097=CARTESIAN_POINT('Ctrl Pts',(42.491998760499,-57.4589935379043,-42.3424967913847));
#240098=CARTESIAN_POINT('Ctrl Pts',(42.5530828863182,-57.9742984445225,
-42.3146829212251));
#240099=CARTESIAN_POINT('Ctrl Pts',(42.6363980620258,-58.2288520804956,
-42.2993933168699));
#240100=CARTESIAN_POINT('Ctrl Pts',(42.8937850504995,-58.6841430634323,
-42.2688857388614));
#240101=CARTESIAN_POINT('Ctrl Pts',(43.06288627497,-58.8819667140344,-42.2539599352457));
#240102=CARTESIAN_POINT('Ctrl Pts',(43.4670799663806,-59.2026435486667,
-42.2259709526097));
#240103=CARTESIAN_POINT('Ctrl Pts',(43.698357440717,-59.3223873201503,-42.2134263760266));
#240104=CARTESIAN_POINT('Ctrl Pts',(44.1289367369284,-59.4484346369407,
-42.1883092504143));
#240105=CARTESIAN_POINT('Ctrl Pts',(44.3181598941138,-59.475452478349,-42.177271232912));
#240106=CARTESIAN_POINT('Ctrl Pts',(44.5079524583206,-59.475452478349,-42.1662));
#240107=CARTESIAN_POINT('Origin',(44.5079524583206,-57.475452478349,235.35105));
#240108=CARTESIAN_POINT('',(44.5079524583206,-59.475452478349,-41.4662));
#240109=CARTESIAN_POINT('',(44.5079524583206,-59.475452478349,-41.6249500000001));
#240110=CARTESIAN_POINT('',(44.5079524583206,-59.475452478349,235.35105));
#240111=CARTESIAN_POINT('Ctrl Pts',(44.5079524583206,-59.475452478349,-41.6249500000001));
#240112=CARTESIAN_POINT('Ctrl Pts',(44.3963129281412,-59.475452478349,-41.6314623059272));
#240113=CARTESIAN_POINT('Ctrl Pts',(44.284610180426,-59.4661050893039,-41.637978299544));
#240114=CARTESIAN_POINT('Ctrl Pts',(43.911142678792,-59.4028619686822,-41.659763903806));
#240115=CARTESIAN_POINT('Ctrl Pts',(43.6598786140261,-59.3062423031846,
-41.6738640414497));
#240116=CARTESIAN_POINT('Ctrl Pts',(43.2195904327178,-59.0263440056424,
-41.7008457238465));
#240117=CARTESIAN_POINT('Ctrl Pts',(43.0324278880756,-58.8494703777636,
-41.715239959607));
#240118=CARTESIAN_POINT('Ctrl Pts',(42.728906649178,-58.4269175895807,-41.7454392469336));
#240119=CARTESIAN_POINT('Ctrl Pts',(42.6185745343544,-58.1829538690468,
-41.760981862425));
#240120=CARTESIAN_POINT('Ctrl Pts',(42.5012232192591,-57.6737152098165,
-41.7901304033518));
#240121=CARTESIAN_POINT('Ctrl Pts',(42.4923876021727,-57.4141076143141,
-41.8025950539835));
#240122=CARTESIAN_POINT('Ctrl Pts',(42.5737311241404,-56.9049828108047,
-41.8306876158305));
#240123=CARTESIAN_POINT('Ctrl Pts',(42.6634335294862,-56.6603634107947,
-41.8456616551753));
#240124=CARTESIAN_POINT('Ctrl Pts',(42.9344647249112,-56.2127349077193,
-41.8761800949239));
#240125=CARTESIAN_POINT('Ctrl Pts',(43.1155820075873,-56.0154315039811,
-41.8914300849956));
#240126=CARTESIAN_POINT('Ctrl Pts',(43.5347753777698,-55.709900089237,-41.9190914396905));
#240127=CARTESIAN_POINT('Ctrl Pts',(43.7661104404675,-55.6009020538235,
-41.9316758822919));
#240128=CARTESIAN_POINT('Ctrl Pts',(44.2646382087956,-55.4732097928478,
-41.9607566687777));
#240129=CARTESIAN_POINT('Ctrl Pts',(44.5278281986985,-55.4585803441233,
-41.9761094181887));
#240130=CARTESIAN_POINT('Ctrl Pts',(45.0489862984194,-55.5318451887435,
-42.0065103073391));
#240131=CARTESIAN_POINT('Ctrl Pts',(45.3015461474302,-55.6206126054169,
-42.0210600730208));
#240132=CARTESIAN_POINT('Ctrl Pts',(45.7481527830709,-55.885906664465,-42.0474882645792));
#240133=CARTESIAN_POINT('Ctrl Pts',(45.9400885160742,-56.0564062583027,
-42.061699713935));
#240134=CARTESIAN_POINT('Ctrl Pts',(46.2557408430406,-56.4679417525677,
-42.0916962513727));
#240135=CARTESIAN_POINT('Ctrl Pts',(46.3734402397765,-56.7074621950644,
-42.10722927974));
#240136=CARTESIAN_POINT('Ctrl Pts',(46.5076138855837,-57.2135657321372,
-42.1367100914123));
#240137=CARTESIAN_POINT('Ctrl Pts',(46.5246867087515,-57.4746722153939,
-42.1494225002558));
#240138=CARTESIAN_POINT('Ctrl Pts',(46.4584645450735,-57.9870751538133,
-42.1772396277924));
#240139=CARTESIAN_POINT('Ctrl Pts',(46.3765044067399,-58.2335665054474,
-42.1920824185463));
#240140=CARTESIAN_POINT('Ctrl Pts',(46.1187008222665,-58.6908059681195,
-42.2227005808602));
#240141=CARTESIAN_POINT('Ctrl Pts',(45.9418237970571,-58.8951851640859,
-42.2381843526787));
#240142=CARTESIAN_POINT('Ctrl Pts',(45.5289100107533,-59.2138841198949,
-42.2663277526395));
#240143=CARTESIAN_POINT('Ctrl Pts',(45.3001791987696,-59.3293366322367,
-42.2787367734739));
#240144=CARTESIAN_POINT('Ctrl Pts',(44.8773365012054,-59.4497959150024,
-42.3034025974984));
#240145=CARTESIAN_POINT('Ctrl Pts',(44.6929025187842,-59.475452478349,-42.314161246473));
#240146=CARTESIAN_POINT('Ctrl Pts',(44.5079524583206,-59.475452478349,-42.3249500000001));
#240147=CARTESIAN_POINT('Ctrl Pts',(44.5079524583206,-59.475452478349,-42.1661999999999));
#240148=CARTESIAN_POINT('Ctrl Pts',(44.5819299860625,-59.475452478349,-42.161884644215));
#240149=CARTESIAN_POINT('Ctrl Pts',(44.6559940233556,-59.4713480872461,
-42.1575642420394));
#240150=CARTESIAN_POINT('Ctrl Pts',(44.9830823256217,-59.4348404808826,
-42.1384840910739));
#240151=CARTESIAN_POINT('Ctrl Pts',(45.2286836340998,-59.3584131739,-42.1241573480794));
#240152=CARTESIAN_POINT('Ctrl Pts',(45.6892289950069,-59.1113735572966,
-42.0972922020265));
#240153=CARTESIAN_POINT('Ctrl Pts',(45.8973919788335,-58.9387337125747,
-42.0829302727521));
#240154=CARTESIAN_POINT('Ctrl Pts',(46.2294519095304,-58.5265497382248,
-42.0524224201923));
#240155=CARTESIAN_POINT('Ctrl Pts',(46.3519800320567,-58.2927254065234,
-42.0370363109609));
#240156=CARTESIAN_POINT('Ctrl Pts',(46.497811004372,-57.7989613281489,-42.0078388605397));
#240157=CARTESIAN_POINT('Ctrl Pts',(46.5227443568654,-57.5446038131605,
-41.995124827779));
#240158=CARTESIAN_POINT('Ctrl Pts',(46.4752713728182,-57.0282329744125,
-41.9676541003368));
#240159=CARTESIAN_POINT('Ctrl Pts',(46.3986945235629,-56.7716032555838,
-41.952456150641));
#240160=CARTESIAN_POINT('Ctrl Pts',(46.1531025911945,-56.3091383174921,
-41.92193018017));
#240161=CARTESIAN_POINT('Ctrl Pts',(45.9887519767006,-56.1064872107599,
-41.9068990618661));
#240162=CARTESIAN_POINT('Ctrl Pts',(45.5934103745848,-55.7761403469175,
-41.8786797531957));
#240163=CARTESIAN_POINT('Ctrl Pts',(45.3666465129243,-55.6510270662813,
-41.8662904865186));
#240164=CARTESIAN_POINT('Ctrl Pts',(44.8696684889806,-55.4905895017291,
-41.8373001017886));
#240165=CARTESIAN_POINT('Ctrl Pts',(44.6032390529754,-55.4601559654108,
-41.8217583846883));
#240166=CARTESIAN_POINT('Ctrl Pts',(44.0840904291311,-55.5042544757982,
-41.791474714964));
#240167=CARTESIAN_POINT('Ctrl Pts',(43.8359523532419,-55.5744690499767,
-41.7769999938704));
#240168=CARTESIAN_POINT('Ctrl Pts',(43.3709847734867,-55.8088419811641,
-41.7498768850514));
#240169=CARTESIAN_POINT('Ctrl Pts',(43.1602892241647,-55.9740716865162,
-41.7360734668819));
#240170=CARTESIAN_POINT('Ctrl Pts',(42.817506900039,-56.3749293567097,-41.705825061763));
#240171=CARTESIAN_POINT('Ctrl Pts',(42.6879340204009,-56.6058018069247,
-41.6903826040365));
#240172=CARTESIAN_POINT('Ctrl Pts',(42.5280293442433,-57.0958938829126,
-41.6609601733486));
#240173=CARTESIAN_POINT('Ctrl Pts',(42.495933675203,-57.3493721621776,-41.647919891983));
#240174=CARTESIAN_POINT('Ctrl Pts',(42.5287550455231,-57.8667440966951,
-41.6208259297696));
#240175=CARTESIAN_POINT('Ctrl Pts',(42.5980177961076,-58.1254040341162,
-41.6057387450673));
#240176=CARTESIAN_POINT('Ctrl Pts',(42.830684161527,-58.5952495445704,-41.5752169174479));
#240177=CARTESIAN_POINT('Ctrl Pts',(42.9897683285869,-58.8029736952618,
-41.5600831230724));
#240178=CARTESIAN_POINT('Ctrl Pts',(43.3755311450215,-59.1436457213512,
-41.5316215875709));
#240179=CARTESIAN_POINT('Ctrl Pts',(43.597573413174,-59.2744675958978,-41.5193054443001));
#240180=CARTESIAN_POINT('Ctrl Pts',(44.0535417110567,-59.4365006200257,
-41.4927072935903));
#240181=CARTESIAN_POINT('Ctrl Pts',(44.2800678724856,-59.475452478349,-41.479493267507));
#240182=CARTESIAN_POINT('Ctrl Pts',(44.5079524583206,-59.475452478349,-41.4662));
#240183=CARTESIAN_POINT('Origin',(44.5079524583206,-57.475452478349,235.35105));
#240184=CARTESIAN_POINT('',(44.5079524583206,-59.475452478349,-40.7662));
#240185=CARTESIAN_POINT('',(44.5079524583206,-59.475452478349,-40.9249500000001));
#240186=CARTESIAN_POINT('',(44.5079524583206,-59.475452478349,235.35105));
#240187=CARTESIAN_POINT('Ctrl Pts',(44.5079524583206,-59.475452478349,-40.9249500000001));
#240188=CARTESIAN_POINT('Ctrl Pts',(44.3556832620905,-59.475452478349,-40.9338323697802));
#240189=CARTESIAN_POINT('Ctrl Pts',(44.2035477074772,-59.4580626051099,
-40.9427069437994));
#240190=CARTESIAN_POINT('Ctrl Pts',(43.7996698653827,-59.364054039355,-40.9662664845882));
#240191=CARTESIAN_POINT('Ctrl Pts',(43.5589663513918,-59.2553062210328,
-40.9793805123415));
#240192=CARTESIAN_POINT('Ctrl Pts',(43.1371734125507,-58.9542357473873,
-41.0068923293039));
#240193=CARTESIAN_POINT('Ctrl Pts',(42.9589885091226,-58.7663860387722,
-41.0215792084729));
#240194=CARTESIAN_POINT('Ctrl Pts',(42.6778986677055,-58.3251594171462,
-41.0520676141982));
#240195=CARTESIAN_POINT('Ctrl Pts',(42.5810274339302,-58.0738554741762,
-41.0675884351065));
#240196=CARTESIAN_POINT('Ctrl Pts',(42.4935259126035,-57.5596078215576,
-41.0961194021204));
#240197=CARTESIAN_POINT('Ctrl Pts',(42.4992034595432,-57.3024572643112,
-41.1084342187911));
#240198=CARTESIAN_POINT('Ctrl Pts',(42.607815229616,-56.7995486188924,-41.1370080757433));
#240199=CARTESIAN_POINT('Ctrl Pts',(42.7114689037048,-56.5589399783078,
-41.1521864109526));
#240200=CARTESIAN_POINT('Ctrl Pts',(43.0080279189641,-56.1261925223017,
-41.1826976491666));
#240201=CARTESIAN_POINT('Ctrl Pts',(43.1999024039458,-55.9394423174307,
-41.1977282629041));
#240202=CARTESIAN_POINT('Ctrl Pts',(43.6353704033976,-55.6581082265016,
-41.224641890287));
#240203=CARTESIAN_POINT('Ctrl Pts',(43.8723021658698,-55.5623022940588,
-41.2378703996071));
#240204=CARTESIAN_POINT('Ctrl Pts',(44.3784883874681,-55.4624487207122,
-41.2673979292003));
#240205=CARTESIAN_POINT('Ctrl Pts',(44.6436019396349,-55.462856007272,-41.2828628864101));
#240206=CARTESIAN_POINT('Ctrl Pts',(45.1599592078587,-55.5663656558035,
-41.3129837270564));
#240207=CARTESIAN_POINT('Ctrl Pts',(45.4059688703599,-55.6690062719493,
-41.326550494208));
#240208=CARTESIAN_POINT('Ctrl Pts',(45.837201140743,-55.9593461274327,-41.3537955340446));
#240209=CARTESIAN_POINT('Ctrl Pts',(46.0200442270936,-56.1416537602683,
-41.3683383014746));
#240210=CARTESIAN_POINT('Ctrl Pts',(46.3127147158099,-56.5735006762076,
-41.3986906307142));
#240211=CARTESIAN_POINT('Ctrl Pts',(46.4165105622606,-56.8211497271544,
-41.414228781114));
#240212=CARTESIAN_POINT('Ctrl Pts',(46.5192362568492,-57.3329264870405,
-41.4430789615887));
#240213=CARTESIAN_POINT('Ctrl Pts',(46.5209489371288,-57.591298778833,-41.455423276652));
#240214=CARTESIAN_POINT('Ctrl Pts',(46.4263177960313,-58.0974421277088,
-41.4837527764889));
#240215=CARTESIAN_POINT('Ctrl Pts',(46.3298111331428,-58.3402091566098,
-41.4988316949865));
#240216=CARTESIAN_POINT('Ctrl Pts',(46.0462652316372,-58.7807852345967,
-41.5293588715376));
#240217=CARTESIAN_POINT('Ctrl Pts',(45.8598384293943,-58.9730324669386,
-41.5445082941789));
#240218=CARTESIAN_POINT('Ctrl Pts',(45.4326650871948,-59.2668301475951,
-41.571809631536));
#240219=CARTESIAN_POINT('Ctrl Pts',(45.1986558057962,-59.3694139804964,
-41.5846589713973));
#240220=CARTESIAN_POINT('Ctrl Pts',(44.8057459523781,-59.4588118646948,
-41.6075787128467));
#240221=CARTESIAN_POINT('Ctrl Pts',(44.6569054744755,-59.475452478349,-41.6162610740577));
#240222=CARTESIAN_POINT('Ctrl Pts',(44.5079524583206,-59.475452478349,-41.6249500000001));
#240223=CARTESIAN_POINT('Ctrl Pts',(44.5079524583206,-59.475452478349,-41.4662));
#240224=CARTESIAN_POINT('Ctrl Pts',(44.5457150412834,-59.475452478349,-41.4639971826605));
#240225=CARTESIAN_POINT('Ctrl Pts',(44.5835149259749,-59.474382984109,-41.4617921893868));
#240226=CARTESIAN_POINT('Ctrl Pts',(44.8770856294728,-59.4577173897901,
-41.4446672316827));
#240227=CARTESIAN_POINT('Ctrl Pts',(45.1277452030424,-59.394183437444,-41.4300454232245));
#240228=CARTESIAN_POINT('Ctrl Pts',(45.5972843930366,-59.1732023971889,
-41.4026556371415));
#240229=CARTESIAN_POINT('Ctrl Pts',(45.8106057972645,-59.015623433461,-41.3893458627232));
#240230=CARTESIAN_POINT('Ctrl Pts',(46.1643828643518,-58.6267167277128,
-41.3593805181985));
#240231=CARTESIAN_POINT('Ctrl Pts',(46.3012566561433,-58.3991559118811,
-41.3438924148386));
#240232=CARTESIAN_POINT('Ctrl Pts',(46.475894211567,-57.9130419854652,-41.3142412439232));
#240233=CARTESIAN_POINT('Ctrl Pts',(46.515440600153,-57.6603847032348,-41.300760837746));
#240234=CARTESIAN_POINT('Ctrl Pts',(46.4977283275787,-57.1421326714575,
-41.2740630966662));
#240235=CARTESIAN_POINT('Ctrl Pts',(46.4360619646601,-56.8816045311775,
-41.2591030951212));
#240236=CARTESIAN_POINT('Ctrl Pts',(46.2169532500797,-56.4045315959542,
-41.2286115828665));
#240237=CARTESIAN_POINT('Ctrl Pts',(46.0634583460397,-56.1917183083876,
-41.2133837148898));
#240238=CARTESIAN_POINT('Ctrl Pts',(45.6876284766909,-55.840486585305,-41.1846784340035));
#240239=CARTESIAN_POINT('Ctrl Pts',(45.470315286488,-55.7038429311988,-41.1723378316431));
#240240=CARTESIAN_POINT('Ctrl Pts',(44.9842432072125,-55.5147120063731,
-41.1439836270187));
#240241=CARTESIAN_POINT('Ctrl Pts',(44.7184258538704,-55.4687071560742,
-41.1284776147404));
#240242=CARTESIAN_POINT('Ctrl Pts',(44.1946734695817,-55.4835061931311,
-41.0979253923236));
#240243=CARTESIAN_POINT('Ctrl Pts',(43.9416365793137,-55.5401710005153,
-41.0831649070579));
#240244=CARTESIAN_POINT('Ctrl Pts',(43.4675773117692,-55.7475991719258,
-41.0555114497845));
#240245=CARTESIAN_POINT('Ctrl Pts',(43.251635465688,-55.8976235119033,-41.0425997525014));
#240246=CARTESIAN_POINT('Ctrl Pts',(42.8870752719029,-56.2744751676231,
-41.0129288989228));
#240247=CARTESIAN_POINT('Ctrl Pts',(42.742976768466,-56.4984970825621,-40.9974088535276));
#240248=CARTESIAN_POINT('Ctrl Pts',(42.5535830260601,-56.9804819149329,
-40.9675358880115));
#240249=CARTESIAN_POINT('Ctrl Pts',(42.5066076402285,-57.232413236575,-40.9535171163813));
#240250=CARTESIAN_POINT('Ctrl Pts',(42.5094167419912,-57.751388203542,-40.9272175297695));
#240251=CARTESIAN_POINT('Ctrl Pts',(42.5635494460456,-58.0135322888619,
-40.9123956253898));
#240252=CARTESIAN_POINT('Ctrl Pts',(42.7690799993602,-58.4973409176244,
-40.8819598680719));
#240253=CARTESIAN_POINT('Ctrl Pts',(42.9169127288896,-58.7150242563767,
-40.8666511208824));
#240254=CARTESIAN_POINT('Ctrl Pts',(43.2828838041862,-59.076581472659,-40.8377117633567));
#240255=CARTESIAN_POINT('Ctrl Pts',(43.4956739950599,-59.2189219816486,
-40.8252495770234));
#240256=CARTESIAN_POINT('Ctrl Pts',(43.9757997011733,-59.421823142488,-40.7972422441668));
#240257=CARTESIAN_POINT('Ctrl Pts',(44.2405470537739,-59.475452478349,-40.7817986485985));
#240258=CARTESIAN_POINT('Ctrl Pts',(44.5079524583207,-59.475452478349,-40.7661999999999));
#240259=CARTESIAN_POINT('Origin',(44.5079524583206,-57.475452478349,235.35105));
#240260=CARTESIAN_POINT('',(44.5079524583206,-59.475452478349,-40.0662));
#240261=CARTESIAN_POINT('',(44.5079524583206,-59.475452478349,-40.22495));
#240262=CARTESIAN_POINT('',(44.5079524583206,-59.475452478349,235.35105));
#240263=CARTESIAN_POINT('',(45.4139072126472,-59.2584969021125,-40.0133531362322));
#240264=CARTESIAN_POINT('Ctrl Pts',(44.5079524583206,-59.475452478349,-40.0662));
#240265=CARTESIAN_POINT('Ctrl Pts',(44.6477540810448,-59.475452478349,-40.058044905341));
#240266=CARTESIAN_POINT('Ctrl Pts',(44.7872831379324,-59.4607938517436,
-40.0499057103559));
#240267=CARTESIAN_POINT('Ctrl Pts',(45.0942698010449,-59.3954660374654,
-40.0319981550077));
#240268=CARTESIAN_POINT('Ctrl Pts',(45.2588837491004,-59.3372630397163,
-40.0223956747045));
#240269=CARTESIAN_POINT('Ctrl Pts',(45.4139070277165,-59.2584965939532,
-40.0133526501186));
#240270=CARTESIAN_POINT('',(46.5057019923328,-57.5702877145999,-39.8960552477251));
#240271=CARTESIAN_POINT('Ctrl Pts',(45.4139070626845,-59.2584965761862,
-40.0133533627948));
#240272=CARTESIAN_POINT('Ctrl Pts',(45.5708274797814,-59.178766201284,-40.0284745705566));
#240273=CARTESIAN_POINT('Ctrl Pts',(45.7167913486008,-59.0785403908483,
-40.0374253375929));
#240274=CARTESIAN_POINT('Ctrl Pts',(45.9789089800695,-58.8419935930646,
-40.0424294628079));
#240275=CARTESIAN_POINT('Ctrl Pts',(46.0936204899094,-58.7070030684609,
-40.0384624535326));
#240276=CARTESIAN_POINT('Ctrl Pts',(46.2846200996576,-58.4106275181728,
-40.0178326575726));
#240277=CARTESIAN_POINT('Ctrl Pts',(46.3598125890322,-58.2509288938826,
-40.0012757421132));
#240278=CARTESIAN_POINT('Ctrl Pts',(46.4665664629444,-57.9166464805059,
-39.9566009687345));
#240279=CARTESIAN_POINT('Ctrl Pts',(46.4974588687898,-57.7439490347554,
-39.9287059824097));
#240280=CARTESIAN_POINT('Ctrl Pts',(46.5057027546467,-57.5702878806477,
-39.8960539311642));
#240281=CARTESIAN_POINT('',(43.0434015151427,-58.8374706322701,-39.4567770164569));
#240282=CARTESIAN_POINT('Ctrl Pts',(43.0434024600225,-58.8374705775258,
-39.456776075616));
#240283=CARTESIAN_POINT('Ctrl Pts',(42.9505070828511,-58.7375820925191,
-39.4645317054413));
#240284=CARTESIAN_POINT('Ctrl Pts',(42.8680780966169,-58.6284556232212,
-39.4724487513936));
#240285=CARTESIAN_POINT('Ctrl Pts',(42.7265681044559,-58.3948848309218,
-39.4883756901483));
#240286=CARTESIAN_POINT('Ctrl Pts',(42.6679060158213,-58.2710134250182,
-39.4963444218185));
#240287=CARTESIAN_POINT('Ctrl Pts',(42.5341559488002,-57.8927163453032,
-39.5193563335106));
#240288=CARTESIAN_POINT('Ctrl Pts',(42.4963486406859,-57.6283470788705,
-39.5331376031768));
#240289=CARTESIAN_POINT('Ctrl Pts',(42.5252427856916,-57.1091600280751,
-39.5602087176322));
#240290=CARTESIAN_POINT('Ctrl Pts',(42.5882142281025,-56.8591155236405,
-39.5746771701227));
#240291=CARTESIAN_POINT('Ctrl Pts',(42.8090290264238,-56.3872695438299,
-39.6049543870431));
#240292=CARTESIAN_POINT('Ctrl Pts',(42.9683271570434,-56.1715902919037,
-39.6204962990084));
#240293=CARTESIAN_POINT('Ctrl Pts',(43.3553575620516,-55.8209320584954,
-39.6494992905482));
#240294=CARTESIAN_POINT('Ctrl Pts',(43.5769855334451,-55.6868188496488,
-39.661893596049));
#240295=CARTESIAN_POINT('Ctrl Pts',(44.0682014711997,-55.506263568743,-39.6905478590847));
#240296=CARTESIAN_POINT('Ctrl Pts',(44.3343106141816,-55.4652516279505,
-39.7060708924254));
#240297=CARTESIAN_POINT('Ctrl Pts',(44.8567640004058,-55.4894779008722,
-39.7365473399551));
#240298=CARTESIAN_POINT('Ctrl Pts',(45.1083113153773,-55.5505185872555,
-39.7512209333284));
#240299=CARTESIAN_POINT('Ctrl Pts',(45.5795114174102,-55.7665565411676,
-39.778707605947));
#240300=CARTESIAN_POINT('Ctrl Pts',(45.7937919860029,-55.9213584811786,
-39.7918603681415));
#240301=CARTESIAN_POINT('Ctrl Pts',(46.1515412850048,-56.3058630393379,
-39.8217191810845));
#240302=CARTESIAN_POINT('Ctrl Pts',(46.2910697333296,-56.5321542872952,
-39.8372205757081));
#240303=CARTESIAN_POINT('Ctrl Pts',(46.4304078182913,-56.9072207565103,
-39.8602322667956));
#240304=CARTESIAN_POINT('Ctrl Pts',(46.4647739918623,-57.0400469563788,
-39.8679447472216));
#240305=CARTESIAN_POINT('Ctrl Pts',(46.5051437473397,-57.3060403765032,
-39.8825596935352));
#240306=CARTESIAN_POINT('Ctrl Pts',(46.5119682426376,-57.4383022409662,
-39.8892061117466));
#240307=CARTESIAN_POINT('Ctrl Pts',(46.5057027656803,-57.5702876482191,
-39.8960565132351));
#240308=CARTESIAN_POINT('',(43.3993759211742,-59.1401020382204,-39.589855096412));
#240309=CARTESIAN_POINT('Origin',(44.6251460650309,-57.3664988654425,-39.4575809488933));
#240310=CARTESIAN_POINT('Ctrl Pts',(43.3993759361741,-59.1401020194073,
-39.589855135757));
#240311=CARTESIAN_POINT('Ctrl Pts',(43.2536892830903,-59.0430817162051,
-39.5990056158952));
#240312=CARTESIAN_POINT('Ctrl Pts',(43.1213873644818,-58.9273679902937,
-39.60871006505));
#240313=CARTESIAN_POINT('Ctrl Pts',(42.8872222066712,-58.6609972317884,
-39.6289964397015));
#240314=CARTESIAN_POINT('Ctrl Pts',(42.7873202434622,-58.5106839058266,
-39.6395037978923));
#240315=CARTESIAN_POINT('Ctrl Pts',(42.5930417605153,-58.1105886447152,
-39.6653823254816));
#240316=CARTESIAN_POINT('Ctrl Pts',(42.5257866956149,-57.8514113611987,
-39.6804370880517));
#240317=CARTESIAN_POINT('Ctrl Pts',(42.4969681427887,-57.3337914820228,
-39.7074268271265));
#240318=CARTESIAN_POINT('Ctrl Pts',(42.5310306699669,-57.0805391543703,
-39.7205734044732));
#240319=CARTESIAN_POINT('Ctrl Pts',(42.6948165101306,-56.5914815004161,
-39.7500567786919));
#240320=CARTESIAN_POINT('Ctrl Pts',(42.8263205480509,-56.3614596380144,
-39.7655125917468));
#240321=CARTESIAN_POINT('Ctrl Pts',(43.1720218424975,-55.9637414363319,
-39.7956875333634));
#240322=CARTESIAN_POINT('Ctrl Pts',(43.3834109997795,-55.8005377803727,
-39.8093517482518));
#240323=CARTESIAN_POINT('Ctrl Pts',(43.8495886138448,-55.5696795120759,
-39.8365454424056));
#240324=CARTESIAN_POINT('Ctrl Pts',(44.0984046783535,-55.5012074295454,
-39.8510597128353));
#240325=CARTESIAN_POINT('Ctrl Pts',(44.6182428099406,-55.4608949849634,
-39.8813836038445));
#240326=CARTESIAN_POINT('Ctrl Pts',(44.8846423726718,-55.4933495918306,
-39.8969235783371));
#240327=CARTESIAN_POINT('Ctrl Pts',(45.380236549904,-55.657535245913,-39.9258332386757));
#240328=CARTESIAN_POINT('Ctrl Pts',(45.6057567875752,-55.7841433844684,
-39.9381941555478));
#240329=CARTESIAN_POINT('Ctrl Pts',(45.9986064673138,-56.1171896181519,
-39.9664771503155));
#240330=CARTESIAN_POINT('Ctrl Pts',(46.1615993591797,-56.3211756711888,
-39.9815361073918));
#240331=CARTESIAN_POINT('Ctrl Pts',(46.4038443510521,-56.7855990008045,
-40.0120633930789));
#240332=CARTESIAN_POINT('Ctrl Pts',(46.4785203864252,-57.0427784721124,
-40.0272336748473));
#240333=CARTESIAN_POINT('Ctrl Pts',(46.5221743812755,-57.5594246147262,
-40.0546069229462));
#240334=CARTESIAN_POINT('Ctrl Pts',(46.4953792794438,-57.8135450608098,
-40.0673965290231));
#240335=CARTESIAN_POINT('Ctrl Pts',(46.3458998218777,-58.306368914152,-40.0966528951696));
#240336=CARTESIAN_POINT('Ctrl Pts',(46.2215394421076,-58.5394480650177,
-40.1120548000812));
#240337=CARTESIAN_POINT('Ctrl Pts',(45.8866789349324,-58.948704885331,-40.1424964617192));
#240338=CARTESIAN_POINT('Ctrl Pts',(45.6778563177999,-59.1194142087351,
-40.1567056081972));
#240339=CARTESIAN_POINT('Ctrl Pts',(45.2161593327308,-59.3631817568321,
-40.1836379323262));
#240340=CARTESIAN_POINT('Ctrl Pts',(44.9698889176337,-59.4380144849026,
-40.1980037065402));
#240341=CARTESIAN_POINT('Ctrl Pts',(44.6469276953965,-59.4718354739981,
-40.2168431111707));
#240342=CARTESIAN_POINT('Ctrl Pts',(44.5773988698809,-59.475452478349,-40.2208989593257));
#240343=CARTESIAN_POINT('Ctrl Pts',(44.5079524583206,-59.475452478349,-40.2249500000001));
#240344=CARTESIAN_POINT('Origin',(-44.5079524583207,-57.4754524783487,-52.920575));
#240345=CARTESIAN_POINT('',(-44.5079524583207,-55.8067071952963,-40.04995));
#240346=CARTESIAN_POINT('',(-44.5079524583207,-55.8067071952963,-39.8912));
#240347=CARTESIAN_POINT('',(-44.5079524583207,-55.8067071952962,-52.920575));
#240348=CARTESIAN_POINT('',(-45.3258935545055,-56.0209136569754,-39.8341888326825));
#240349=CARTESIAN_POINT('Ctrl Pts',(-44.5079524583208,-55.8067071952963,
-39.8912));
#240350=CARTESIAN_POINT('Ctrl Pts',(-44.9449717304834,-55.8067071952963,
-39.8647401145564));
#240351=CARTESIAN_POINT('Ctrl Pts',(-45.3258935545055,-56.0209136569754,
-39.8341888326825));
#240352=CARTESIAN_POINT('',(-45.7222549758842,-56.3308214393021,-39.9581073668549));
#240353=CARTESIAN_POINT('Ctrl Pts',(-45.7222549758842,-56.3308214393021,
-39.9581073668549));
#240354=CARTESIAN_POINT('Ctrl Pts',(-45.7045762341998,-56.3120666267883,
-39.9516436713479));
#240355=CARTESIAN_POINT('Ctrl Pts',(-45.686660871375,-56.2939315400474,
-39.9452586862569));
#240356=CARTESIAN_POINT('Ctrl Pts',(-45.6685147272012,-56.2763687588793,
-39.9389426841664));
#240357=CARTESIAN_POINT('Ctrl Pts',(-45.648505858845,-56.2570031364642,
-39.9319783366359));
#240358=CARTESIAN_POINT('Ctrl Pts',(-45.6282239848617,-56.238342887266,
-39.9251019846523));
#240359=CARTESIAN_POINT('Ctrl Pts',(-45.6076972509794,-56.2203564794336,
-39.9183131959778));
#240360=CARTESIAN_POINT('Ctrl Pts',(-45.5657790231701,-56.1836259237927,
-39.9044496172986));
#240361=CARTESIAN_POINT('Ctrl Pts',(-45.5228400189614,-56.1497051629388,
-39.8909512030947));
#240362=CARTESIAN_POINT('Ctrl Pts',(-45.4790691672601,-56.118382182885,
-39.8778157637598));
#240363=CARTESIAN_POINT('Ctrl Pts',(-45.4340050705677,-56.086133740212,
-39.864292227313));
#240364=CARTESIAN_POINT('Ctrl Pts',(-45.3880438891079,-56.0566341670122,
-39.8511484168624));
#240365=CARTESIAN_POINT('Ctrl Pts',(-45.3413791392512,-56.0297312061481,
-39.8383987109864));
#240366=CARTESIAN_POINT('Ctrl Pts',(-45.3362271142298,-56.0267609828437,
-39.8369910788038));
#240367=CARTESIAN_POINT('Ctrl Pts',(-45.3310650292783,-56.0238217689367,
-39.8355877210878));
#240368=CARTESIAN_POINT('Ctrl Pts',(-45.3258935545055,-56.0209136569754,
-39.8341888326825));
#240369=CARTESIAN_POINT('Ctrl Pts',(-44.5079524583208,-55.8067071952963,
-40.04995));
#240370=CARTESIAN_POINT('Ctrl Pts',(-45.2282121628138,-55.8067071952963,
-40.0063409637755));
#240371=CARTESIAN_POINT('Ctrl Pts',(-45.7222549758842,-56.3308214393021,
-39.9581073668549));
#240372=CARTESIAN_POINT('Origin',(-44.5079524583207,-57.4754524783487,-52.920575));
#240373=CARTESIAN_POINT('',(-44.5079524583207,-55.8067071952963,-40.74995));
#240374=CARTESIAN_POINT('',(-44.5079524583207,-55.8067071952963,-40.5912));
#240375=CARTESIAN_POINT('',(-44.5079524583207,-55.8067071952962,-52.920575));
#240376=CARTESIAN_POINT('',(-45.9506478428458,-58.3141066664263,-40.3575668188428));
#240377=CARTESIAN_POINT('Ctrl Pts',(-44.5079524583208,-55.8067071952963,
-40.5912));
#240378=CARTESIAN_POINT('Ctrl Pts',(-45.4714029967,-55.8067071952963,-40.5328666666667));
#240379=CARTESIAN_POINT('Ctrl Pts',(-45.9531282658897,-56.6410798368225,
-40.4745333333334));
#240380=CARTESIAN_POINT('Ctrl Pts',(-46.4348535350793,-57.4754524783487,
-40.4162));
#240381=CARTESIAN_POINT('Ctrl Pts',(-45.9531282658897,-58.309825119875,
-40.3578666666667));
#240382=CARTESIAN_POINT('Ctrl Pts',(-45.9518912282699,-58.3119677318833,
-40.3577168706472));
#240383=CARTESIAN_POINT('Ctrl Pts',(-45.9506478428458,-58.3141066664263,
-40.3575668188428));
#240384=CARTESIAN_POINT('',(-44.4689492302737,-59.1437418920632,-40.2388225645966));
#240385=CARTESIAN_POINT('Ctrl Pts',(-44.4689492302736,-59.1437418920632,
-40.2388225645967));
#240386=CARTESIAN_POINT('Ctrl Pts',(-44.6151980966235,-59.1471610697185,
-40.266024559964));
#240387=CARTESIAN_POINT('Ctrl Pts',(-44.7618474420247,-59.1313541404608,
-40.2898435667392));
#240388=CARTESIAN_POINT('Ctrl Pts',(-45.0497620148851,-59.0608004987189,
-40.3294471928174));
#240389=CARTESIAN_POINT('Ctrl Pts',(-45.1893227978148,-59.0060957201154,
-40.3449203569677));
#240390=CARTESIAN_POINT('Ctrl Pts',(-45.4502212571483,-58.8607378909715,
-40.365994271027));
#240391=CARTESIAN_POINT('Ctrl Pts',(-45.5702107742475,-58.771067079493,
-40.3715288199669));
#240392=CARTESIAN_POINT('Ctrl Pts',(-45.6900411584965,-58.6534685340575,
-40.3719332763248));
#240393=CARTESIAN_POINT('Ctrl Pts',(-45.7030763481267,-58.6402419523344,
-40.3718986213114));
#240394=CARTESIAN_POINT('Ctrl Pts',(-45.8062133726342,-58.5320358540091,
-40.3709726646665));
#240395=CARTESIAN_POINT('Ctrl Pts',(-45.8849732379958,-58.4270834459435,
-40.3661946462488));
#240396=CARTESIAN_POINT('Ctrl Pts',(-45.9506478428458,-58.3141066664263,
-40.3575668188428));
#240397=CARTESIAN_POINT('Ctrl Pts',(-44.4689492302737,-59.1437418920632,
-40.2388225645966));
#240398=CARTESIAN_POINT('Ctrl Pts',(-43.5315862238041,-59.121827119476,
-40.1813026722985));
#240399=CARTESIAN_POINT('Ctrl Pts',(-43.0627766507519,-58.309825119875,
-40.1245333333334));
#240400=CARTESIAN_POINT('Ctrl Pts',(-42.5810513815623,-57.4754524783487,
-40.0662));
#240401=CARTESIAN_POINT('Ctrl Pts',(-43.0627766507519,-56.6410798368225,
-40.0078666666667));
#240402=CARTESIAN_POINT('Ctrl Pts',(-43.5445019199415,-55.8067071952963,
-39.9495333333333));
#240403=CARTESIAN_POINT('Ctrl Pts',(-44.5079524583208,-55.8067071952963,
-39.8912));
#240404=CARTESIAN_POINT('Ctrl Pts',(-44.5079524583208,-55.8067071952963,
-40.74995));
#240405=CARTESIAN_POINT('Ctrl Pts',(-45.4714029967,-55.8067071952963,-40.6916166666667));
#240406=CARTESIAN_POINT('Ctrl Pts',(-45.9531282658897,-56.6410798368225,
-40.6332833333334));
#240407=CARTESIAN_POINT('Ctrl Pts',(-46.4348535350793,-57.4754524783487,
-40.57495));
#240408=CARTESIAN_POINT('Ctrl Pts',(-45.9531282658897,-58.309825119875,
-40.5166166666667));
#240409=CARTESIAN_POINT('Ctrl Pts',(-45.4714029967,-59.1441977614012,-40.4582833333333));
#240410=CARTESIAN_POINT('Ctrl Pts',(-44.5079524583208,-59.1441977614012,
-40.39995));
#240411=CARTESIAN_POINT('Ctrl Pts',(-43.5445019199415,-59.1441977614012,
-40.3416166666667));
#240412=CARTESIAN_POINT('Ctrl Pts',(-43.0627766507519,-58.309825119875,
-40.2832833333334));
#240413=CARTESIAN_POINT('Ctrl Pts',(-42.5810513815623,-57.4754524783487,
-40.22495));
#240414=CARTESIAN_POINT('Ctrl Pts',(-43.0627766507519,-56.6410798368225,
-40.1666166666667));
#240415=CARTESIAN_POINT('Ctrl Pts',(-43.5445019199415,-55.8067071952963,
-40.1082833333334));
#240416=CARTESIAN_POINT('Ctrl Pts',(-44.5079524583208,-55.8067071952963,
-40.04995));
#240417=CARTESIAN_POINT('Origin',(-44.5079524583207,-57.4754524783487,-52.920575));
#240418=CARTESIAN_POINT('',(-44.5079524583207,-55.8067071952963,-41.44995));
#240419=CARTESIAN_POINT('',(-44.5079524583207,-55.8067071952963,-41.2912));
#240420=CARTESIAN_POINT('',(-44.5079524583207,-55.8067071952962,-52.920575));
#240421=CARTESIAN_POINT('Ctrl Pts',(-44.5079524583208,-55.8067071952963,
-41.2912));
#240422=CARTESIAN_POINT('Ctrl Pts',(-45.4714029967,-55.8067071952963,-41.2328666666667));
#240423=CARTESIAN_POINT('Ctrl Pts',(-45.9531282658897,-56.6410798368225,
-41.1745333333334));
#240424=CARTESIAN_POINT('Ctrl Pts',(-46.4348535350793,-57.4754524783487,
-41.1162));
#240425=CARTESIAN_POINT('Ctrl Pts',(-45.9531282658897,-58.309825119875,
-41.0578666666667));
#240426=CARTESIAN_POINT('Ctrl Pts',(-45.4714029967,-59.1441977614012,-40.9995333333333));
#240427=CARTESIAN_POINT('Ctrl Pts',(-44.5079524583208,-59.1441977614012,
-40.9412));
#240428=CARTESIAN_POINT('Ctrl Pts',(-43.5445019199415,-59.1441977614012,
-40.8828666666667));
#240429=CARTESIAN_POINT('Ctrl Pts',(-43.0627766507519,-58.309825119875,
-40.8245333333333));
#240430=CARTESIAN_POINT('Ctrl Pts',(-42.5810513815623,-57.4754524783487,
-40.7662));
#240431=CARTESIAN_POINT('Ctrl Pts',(-43.0627766507519,-56.6410798368225,
-40.7078666666667));
#240432=CARTESIAN_POINT('Ctrl Pts',(-43.5445019199415,-55.8067071952963,
-40.6495333333334));
#240433=CARTESIAN_POINT('Ctrl Pts',(-44.5079524583208,-55.8067071952963,
-40.5912));
#240434=CARTESIAN_POINT('Ctrl Pts',(-44.5079524583208,-55.8067071952963,
-41.44995));
#240435=CARTESIAN_POINT('Ctrl Pts',(-45.4714029967,-55.8067071952963,-41.3916166666667));
#240436=CARTESIAN_POINT('Ctrl Pts',(-45.9531282658897,-56.6410798368225,
-41.3332833333334));
#240437=CARTESIAN_POINT('Ctrl Pts',(-46.4348535350793,-57.4754524783487,
-41.27495));
#240438=CARTESIAN_POINT('Ctrl Pts',(-45.9531282658897,-58.309825119875,
-41.2166166666667));
#240439=CARTESIAN_POINT('Ctrl Pts',(-45.4714029967,-59.1441977614012,-41.1582833333333));
#240440=CARTESIAN_POINT('Ctrl Pts',(-44.5079524583208,-59.1441977614012,
-41.09995));
#240441=CARTESIAN_POINT('Ctrl Pts',(-43.5445019199415,-59.1441977614012,
-41.0416166666667));
#240442=CARTESIAN_POINT('Ctrl Pts',(-43.0627766507519,-58.309825119875,
-40.9832833333333));
#240443=CARTESIAN_POINT('Ctrl Pts',(-42.5810513815623,-57.4754524783487,
-40.92495));
#240444=CARTESIAN_POINT('Ctrl Pts',(-43.0627766507519,-56.6410798368225,
-40.8666166666667));
#240445=CARTESIAN_POINT('Ctrl Pts',(-43.5445019199415,-55.8067071952963,
-40.8082833333334));
#240446=CARTESIAN_POINT('Ctrl Pts',(-44.5079524583208,-55.8067071952963,
-40.74995));
#240447=CARTESIAN_POINT('Origin',(-44.5079524583207,-57.4754524783487,-52.920575));
#240448=CARTESIAN_POINT('',(-44.5079524583207,-55.8067071952963,-42.14995));
#240449=CARTESIAN_POINT('',(-44.5079524583207,-55.8067071952963,-41.9912));
#240450=CARTESIAN_POINT('',(-44.5079524583207,-55.8067071952962,-52.920575));
#240451=CARTESIAN_POINT('Ctrl Pts',(-44.5079524583208,-55.8067071952963,
-41.9912));
#240452=CARTESIAN_POINT('Ctrl Pts',(-45.4714029967,-55.8067071952963,-41.9328666666667));
#240453=CARTESIAN_POINT('Ctrl Pts',(-45.9531282658897,-56.6410798368225,
-41.8745333333334));
#240454=CARTESIAN_POINT('Ctrl Pts',(-46.4348535350793,-57.4754524783487,
-41.8162));
#240455=CARTESIAN_POINT('Ctrl Pts',(-45.9531282658897,-58.309825119875,
-41.7578666666667));
#240456=CARTESIAN_POINT('Ctrl Pts',(-45.4714029967,-59.1441977614012,-41.6995333333334));
#240457=CARTESIAN_POINT('Ctrl Pts',(-44.5079524583208,-59.1441977614012,
-41.6412));
#240458=CARTESIAN_POINT('Ctrl Pts',(-43.5445019199415,-59.1441977614012,
-41.5828666666667));
#240459=CARTESIAN_POINT('Ctrl Pts',(-43.0627766507519,-58.309825119875,
-41.5245333333334));
#240460=CARTESIAN_POINT('Ctrl Pts',(-42.5810513815623,-57.4754524783487,
-41.4662));
#240461=CARTESIAN_POINT('Ctrl Pts',(-43.0627766507519,-56.6410798368225,
-41.4078666666667));
#240462=CARTESIAN_POINT('Ctrl Pts',(-43.5445019199415,-55.8067071952963,
-41.3495333333333));
#240463=CARTESIAN_POINT('Ctrl Pts',(-44.5079524583208,-55.8067071952963,
-41.2912));
#240464=CARTESIAN_POINT('Ctrl Pts',(-44.5079524583208,-55.8067071952963,
-42.14995));
#240465=CARTESIAN_POINT('Ctrl Pts',(-45.4714029967,-55.8067071952963,-42.0916166666667));
#240466=CARTESIAN_POINT('Ctrl Pts',(-45.9531282658897,-56.6410798368225,
-42.0332833333334));
#240467=CARTESIAN_POINT('Ctrl Pts',(-46.4348535350793,-57.4754524783487,
-41.97495));
#240468=CARTESIAN_POINT('Ctrl Pts',(-45.9531282658897,-58.309825119875,
-41.9166166666667));
#240469=CARTESIAN_POINT('Ctrl Pts',(-45.4714029967,-59.1441977614012,-41.8582833333333));
#240470=CARTESIAN_POINT('Ctrl Pts',(-44.5079524583208,-59.1441977614012,
-41.79995));
#240471=CARTESIAN_POINT('Ctrl Pts',(-43.5445019199415,-59.1441977614012,
-41.7416166666666));
#240472=CARTESIAN_POINT('Ctrl Pts',(-43.0627766507519,-58.309825119875,
-41.6832833333333));
#240473=CARTESIAN_POINT('Ctrl Pts',(-42.5810513815623,-57.4754524783487,
-41.62495));
#240474=CARTESIAN_POINT('Ctrl Pts',(-43.0627766507519,-56.6410798368225,
-41.5666166666667));
#240475=CARTESIAN_POINT('Ctrl Pts',(-43.5445019199415,-55.8067071952963,
-41.5082833333334));
#240476=CARTESIAN_POINT('Ctrl Pts',(-44.5079524583208,-55.8067071952963,
-41.44995));
#240477=CARTESIAN_POINT('Origin',(-44.5079524583207,-57.4754524783487,-52.920575));
#240478=CARTESIAN_POINT('',(-44.5079524583207,-55.8067071952963,-42.84995));
#240479=CARTESIAN_POINT('',(-44.5079524583207,-55.8067071952963,-42.6912));
#240480=CARTESIAN_POINT('',(-44.5079524583207,-55.8067071952962,-52.920575));
#240481=CARTESIAN_POINT('Ctrl Pts',(-44.5079524583208,-55.8067071952963,
-42.6912));
#240482=CARTESIAN_POINT('Ctrl Pts',(-45.4714029967,-55.8067071952963,-42.6328666666667));
#240483=CARTESIAN_POINT('Ctrl Pts',(-45.9531282658897,-56.6410798368225,
-42.5745333333333));
#240484=CARTESIAN_POINT('Ctrl Pts',(-46.4348535350793,-57.4754524783487,
-42.5162));
#240485=CARTESIAN_POINT('Ctrl Pts',(-45.9531282658897,-58.309825119875,
-42.4578666666667));
#240486=CARTESIAN_POINT('Ctrl Pts',(-45.4714029967,-59.1441977614012,-42.3995333333334));
#240487=CARTESIAN_POINT('Ctrl Pts',(-44.5079524583208,-59.1441977614012,
-42.3412));
#240488=CARTESIAN_POINT('Ctrl Pts',(-43.5445019199415,-59.1441977614012,
-42.2828666666667));
#240489=CARTESIAN_POINT('Ctrl Pts',(-43.0627766507519,-58.309825119875,
-42.2245333333333));
#240490=CARTESIAN_POINT('Ctrl Pts',(-42.5810513815623,-57.4754524783487,
-42.1662));
#240491=CARTESIAN_POINT('Ctrl Pts',(-43.0627766507519,-56.6410798368225,
-42.1078666666667));
#240492=CARTESIAN_POINT('Ctrl Pts',(-43.5445019199415,-55.8067071952963,
-42.0495333333334));
#240493=CARTESIAN_POINT('Ctrl Pts',(-44.5079524583208,-55.8067071952963,
-41.9912));
#240494=CARTESIAN_POINT('Ctrl Pts',(-44.5079524583208,-55.8067071952963,
-42.84995));
#240495=CARTESIAN_POINT('Ctrl Pts',(-45.4714029967,-55.8067071952963,-42.7916166666667));
#240496=CARTESIAN_POINT('Ctrl Pts',(-45.9531282658897,-56.6410798368225,
-42.7332833333334));
#240497=CARTESIAN_POINT('Ctrl Pts',(-46.4348535350793,-57.4754524783487,
-42.67495));
#240498=CARTESIAN_POINT('Ctrl Pts',(-45.9531282658897,-58.309825119875,
-42.6166166666667));
#240499=CARTESIAN_POINT('Ctrl Pts',(-45.4714029967,-59.1441977614012,-42.5582833333333));
#240500=CARTESIAN_POINT('Ctrl Pts',(-44.5079524583208,-59.1441977614012,
-42.49995));
#240501=CARTESIAN_POINT('Ctrl Pts',(-43.5445019199415,-59.1441977614012,
-42.4416166666667));
#240502=CARTESIAN_POINT('Ctrl Pts',(-43.0627766507519,-58.309825119875,
-42.3832833333333));
#240503=CARTESIAN_POINT('Ctrl Pts',(-42.5810513815623,-57.4754524783487,
-42.32495));
#240504=CARTESIAN_POINT('Ctrl Pts',(-43.0627766507519,-56.6410798368225,
-42.2666166666667));
#240505=CARTESIAN_POINT('Ctrl Pts',(-43.5445019199415,-55.8067071952963,
-42.2082833333333));
#240506=CARTESIAN_POINT('Ctrl Pts',(-44.5079524583208,-55.8067071952963,
-42.14995));
#240507=CARTESIAN_POINT('Origin',(-44.5079524583207,-57.4754524783487,-52.920575));
#240508=CARTESIAN_POINT('',(-44.5079524583207,-55.8067071952963,-43.54995));
#240509=CARTESIAN_POINT('',(-44.5079524583207,-55.8067071952963,-43.3912));
#240510=CARTESIAN_POINT('',(-44.5079524583207,-55.8067071952962,-52.920575));
#240511=CARTESIAN_POINT('Ctrl Pts',(-44.5079524583208,-55.8067071952963,
-43.3912));
#240512=CARTESIAN_POINT('Ctrl Pts',(-45.4714029967,-55.8067071952963,-43.3328666666667));
#240513=CARTESIAN_POINT('Ctrl Pts',(-45.9531282658897,-56.6410798368225,
-43.2745333333334));
#240514=CARTESIAN_POINT('Ctrl Pts',(-46.4348535350793,-57.4754524783487,
-43.2162));
#240515=CARTESIAN_POINT('Ctrl Pts',(-45.9531282658897,-58.309825119875,
-43.1578666666667));
#240516=CARTESIAN_POINT('Ctrl Pts',(-45.4714029967,-59.1441977614012,-43.0995333333334));
#240517=CARTESIAN_POINT('Ctrl Pts',(-44.5079524583208,-59.1441977614012,
-43.0412));
#240518=CARTESIAN_POINT('Ctrl Pts',(-43.5445019199415,-59.1441977614012,
-42.9828666666667));
#240519=CARTESIAN_POINT('Ctrl Pts',(-43.0627766507519,-58.309825119875,
-42.9245333333334));
#240520=CARTESIAN_POINT('Ctrl Pts',(-42.5810513815623,-57.4754524783487,
-42.8662));
#240521=CARTESIAN_POINT('Ctrl Pts',(-43.0627766507519,-56.6410798368225,
-42.8078666666667));
#240522=CARTESIAN_POINT('Ctrl Pts',(-43.5445019199415,-55.8067071952963,
-42.7495333333334));
#240523=CARTESIAN_POINT('Ctrl Pts',(-44.5079524583208,-55.8067071952963,
-42.6912));
#240524=CARTESIAN_POINT('Ctrl Pts',(-44.5079524583208,-55.8067071952963,
-43.54995));
#240525=CARTESIAN_POINT('Ctrl Pts',(-45.4714029967,-55.8067071952963,-43.4916166666667));
#240526=CARTESIAN_POINT('Ctrl Pts',(-45.9531282658897,-56.6410798368225,
-43.4332833333333));
#240527=CARTESIAN_POINT('Ctrl Pts',(-46.4348535350793,-57.4754524783487,
-43.37495));
#240528=CARTESIAN_POINT('Ctrl Pts',(-45.9531282658897,-58.309825119875,
-43.3166166666667));
#240529=CARTESIAN_POINT('Ctrl Pts',(-45.4714029967,-59.1441977614012,-43.2582833333333));
#240530=CARTESIAN_POINT('Ctrl Pts',(-44.5079524583208,-59.1441977614012,
-43.19995));
#240531=CARTESIAN_POINT('Ctrl Pts',(-43.5445019199415,-59.1441977614012,
-43.1416166666667));
#240532=CARTESIAN_POINT('Ctrl Pts',(-43.0627766507519,-58.309825119875,
-43.0832833333333));
#240533=CARTESIAN_POINT('Ctrl Pts',(-42.5810513815623,-57.4754524783487,
-43.02495));
#240534=CARTESIAN_POINT('Ctrl Pts',(-43.0627766507519,-56.6410798368225,
-42.9666166666667));
#240535=CARTESIAN_POINT('Ctrl Pts',(-43.5445019199415,-55.8067071952963,
-42.9082833333333));
#240536=CARTESIAN_POINT('Ctrl Pts',(-44.5079524583208,-55.8067071952963,
-42.84995));
#240537=CARTESIAN_POINT('Origin',(-44.5079524583207,-57.4754524783487,-52.920575));
#240538=CARTESIAN_POINT('',(-44.5079524583207,-55.8067071952963,-44.24995));
#240539=CARTESIAN_POINT('',(-44.5079524583207,-55.8067071952963,-44.0912));
#240540=CARTESIAN_POINT('',(-44.5079524583207,-55.8067071952962,-52.920575));
#240541=CARTESIAN_POINT('Ctrl Pts',(-44.5079524583208,-55.8067071952963,
-44.0912));
#240542=CARTESIAN_POINT('Ctrl Pts',(-45.4714029967,-55.8067071952963,-44.0328666666667));
#240543=CARTESIAN_POINT('Ctrl Pts',(-45.9531282658897,-56.6410798368225,
-43.9745333333333));
#240544=CARTESIAN_POINT('Ctrl Pts',(-46.4348535350793,-57.4754524783487,
-43.9162));
#240545=CARTESIAN_POINT('Ctrl Pts',(-45.9531282658897,-58.309825119875,
-43.8578666666667));
#240546=CARTESIAN_POINT('Ctrl Pts',(-45.4714029967,-59.1441977614012,-43.7995333333334));
#240547=CARTESIAN_POINT('Ctrl Pts',(-44.5079524583208,-59.1441977614012,
-43.7412));
#240548=CARTESIAN_POINT('Ctrl Pts',(-43.5445019199415,-59.1441977614012,
-43.6828666666667));
#240549=CARTESIAN_POINT('Ctrl Pts',(-43.0627766507519,-58.309825119875,
-43.6245333333333));
#240550=CARTESIAN_POINT('Ctrl Pts',(-42.5810513815623,-57.4754524783487,
-43.5662));
#240551=CARTESIAN_POINT('Ctrl Pts',(-43.0627766507519,-56.6410798368225,
-43.5078666666667));
#240552=CARTESIAN_POINT('Ctrl Pts',(-43.5445019199415,-55.8067071952963,
-43.4495333333334));
#240553=CARTESIAN_POINT('Ctrl Pts',(-44.5079524583208,-55.8067071952963,
-43.3912));
#240554=CARTESIAN_POINT('Ctrl Pts',(-44.5079524583208,-55.8067071952963,
-44.24995));
#240555=CARTESIAN_POINT('Ctrl Pts',(-45.4714029967,-55.8067071952963,-44.1916166666667));
#240556=CARTESIAN_POINT('Ctrl Pts',(-45.9531282658897,-56.6410798368225,
-44.1332833333334));
#240557=CARTESIAN_POINT('Ctrl Pts',(-46.4348535350793,-57.4754524783487,
-44.07495));
#240558=CARTESIAN_POINT('Ctrl Pts',(-45.9531282658897,-58.309825119875,
-44.0166166666667));
#240559=CARTESIAN_POINT('Ctrl Pts',(-45.4714029967,-59.1441977614012,-43.9582833333334));
#240560=CARTESIAN_POINT('Ctrl Pts',(-44.5079524583208,-59.1441977614012,
-43.89995));
#240561=CARTESIAN_POINT('Ctrl Pts',(-43.5445019199415,-59.1441977614012,
-43.8416166666667));
#240562=CARTESIAN_POINT('Ctrl Pts',(-43.0627766507519,-58.309825119875,
-43.7832833333334));
#240563=CARTESIAN_POINT('Ctrl Pts',(-42.5810513815623,-57.4754524783487,
-43.72495));
#240564=CARTESIAN_POINT('Ctrl Pts',(-43.0627766507519,-56.6410798368225,
-43.6666166666667));
#240565=CARTESIAN_POINT('Ctrl Pts',(-43.5445019199415,-55.8067071952963,
-43.6082833333334));
#240566=CARTESIAN_POINT('Ctrl Pts',(-44.5079524583208,-55.8067071952963,
-43.54995));
#240567=CARTESIAN_POINT('Origin',(-44.5079524583207,-57.4754524783487,-52.920575));
#240568=CARTESIAN_POINT('',(-44.5079524583207,-55.8067071952963,-44.94995));
#240569=CARTESIAN_POINT('',(-44.5079524583207,-55.8067071952963,-44.7912));
#240570=CARTESIAN_POINT('',(-44.5079524583207,-55.8067071952962,-52.920575));
#240571=CARTESIAN_POINT('Ctrl Pts',(-44.5079524583208,-55.8067071952963,
-44.7912));
#240572=CARTESIAN_POINT('Ctrl Pts',(-45.4714029967,-55.8067071952963,-44.7328666666667));
#240573=CARTESIAN_POINT('Ctrl Pts',(-45.9531282658897,-56.6410798368225,
-44.6745333333334));
#240574=CARTESIAN_POINT('Ctrl Pts',(-46.4348535350793,-57.4754524783487,
-44.6162));
#240575=CARTESIAN_POINT('Ctrl Pts',(-45.9531282658897,-58.309825119875,
-44.5578666666667));
#240576=CARTESIAN_POINT('Ctrl Pts',(-45.4714029967,-59.1441977614012,-44.4995333333333));
#240577=CARTESIAN_POINT('Ctrl Pts',(-44.5079524583208,-59.1441977614012,
-44.4412));
#240578=CARTESIAN_POINT('Ctrl Pts',(-43.5445019199415,-59.1441977614012,
-44.3828666666667));
#240579=CARTESIAN_POINT('Ctrl Pts',(-43.0627766507519,-58.309825119875,
-44.3245333333334));
#240580=CARTESIAN_POINT('Ctrl Pts',(-42.5810513815623,-57.4754524783487,
-44.2662));
#240581=CARTESIAN_POINT('Ctrl Pts',(-43.0627766507519,-56.6410798368225,
-44.2078666666667));
#240582=CARTESIAN_POINT('Ctrl Pts',(-43.5445019199415,-55.8067071952963,
-44.1495333333334));
#240583=CARTESIAN_POINT('Ctrl Pts',(-44.5079524583208,-55.8067071952963,
-44.0912));
#240584=CARTESIAN_POINT('Ctrl Pts',(-44.5079524583208,-55.8067071952963,
-44.94995));
#240585=CARTESIAN_POINT('Ctrl Pts',(-45.4714029967,-55.8067071952963,-44.8916166666667));
#240586=CARTESIAN_POINT('Ctrl Pts',(-45.9531282658897,-56.6410798368225,
-44.8332833333334));
#240587=CARTESIAN_POINT('Ctrl Pts',(-46.4348535350793,-57.4754524783487,
-44.77495));
#240588=CARTESIAN_POINT('Ctrl Pts',(-45.9531282658897,-58.309825119875,
-44.7166166666667));
#240589=CARTESIAN_POINT('Ctrl Pts',(-45.4714029967,-59.1441977614012,-44.6582833333334));
#240590=CARTESIAN_POINT('Ctrl Pts',(-44.5079524583208,-59.1441977614012,
-44.59995));
#240591=CARTESIAN_POINT('Ctrl Pts',(-43.5445019199415,-59.1441977614012,
-44.5416166666667));
#240592=CARTESIAN_POINT('Ctrl Pts',(-43.0627766507519,-58.309825119875,
-44.4832833333334));
#240593=CARTESIAN_POINT('Ctrl Pts',(-42.5810513815623,-57.4754524783487,
-44.42495));
#240594=CARTESIAN_POINT('Ctrl Pts',(-43.0627766507519,-56.6410798368225,
-44.3666166666667));
#240595=CARTESIAN_POINT('Ctrl Pts',(-43.5445019199415,-55.8067071952963,
-44.3082833333334));
#240596=CARTESIAN_POINT('Ctrl Pts',(-44.5079524583208,-55.8067071952963,
-44.24995));
#240597=CARTESIAN_POINT('Origin',(-44.5079524583207,-57.4754524783487,-52.920575));
#240598=CARTESIAN_POINT('',(-44.5079524583207,-55.8067071952963,-45.64995));
#240599=CARTESIAN_POINT('',(-44.5079524583207,-55.8067071952963,-45.4912));
#240600=CARTESIAN_POINT('',(-44.5079524583207,-55.8067071952962,-52.920575));
#240601=CARTESIAN_POINT('Ctrl Pts',(-44.5079524583208,-55.8067071952963,
-45.4912));
#240602=CARTESIAN_POINT('Ctrl Pts',(-45.4714029967,-55.8067071952963,-45.4328666666666));
#240603=CARTESIAN_POINT('Ctrl Pts',(-45.9531282658897,-56.6410798368225,
-45.3745333333334));
#240604=CARTESIAN_POINT('Ctrl Pts',(-46.4348535350793,-57.4754524783487,
-45.3162));
#240605=CARTESIAN_POINT('Ctrl Pts',(-45.9531282658897,-58.309825119875,
-45.2578666666667));
#240606=CARTESIAN_POINT('Ctrl Pts',(-45.4714029967,-59.1441977614012,-45.1995333333333));
#240607=CARTESIAN_POINT('Ctrl Pts',(-44.5079524583208,-59.1441977614012,
-45.1412));
#240608=CARTESIAN_POINT('Ctrl Pts',(-43.5445019199415,-59.1441977614012,
-45.0828666666667));
#240609=CARTESIAN_POINT('Ctrl Pts',(-43.0627766507519,-58.309825119875,
-45.0245333333334));
#240610=CARTESIAN_POINT('Ctrl Pts',(-42.5810513815623,-57.4754524783487,
-44.9662));
#240611=CARTESIAN_POINT('Ctrl Pts',(-43.0627766507519,-56.6410798368225,
-44.9078666666667));
#240612=CARTESIAN_POINT('Ctrl Pts',(-43.5445019199415,-55.8067071952963,
-44.8495333333333));
#240613=CARTESIAN_POINT('Ctrl Pts',(-44.5079524583208,-55.8067071952963,
-44.7912));
#240614=CARTESIAN_POINT('Ctrl Pts',(-44.5079524583208,-55.8067071952963,
-45.64995));
#240615=CARTESIAN_POINT('Ctrl Pts',(-45.4714029967,-55.8067071952963,-45.5916166666667));
#240616=CARTESIAN_POINT('Ctrl Pts',(-45.9531282658897,-56.6410798368225,
-45.5332833333333));
#240617=CARTESIAN_POINT('Ctrl Pts',(-46.4348535350793,-57.4754524783487,
-45.47495));
#240618=CARTESIAN_POINT('Ctrl Pts',(-45.9531282658897,-58.309825119875,
-45.4166166666667));
#240619=CARTESIAN_POINT('Ctrl Pts',(-45.4714029967,-59.1441977614012,-45.3582833333334));
#240620=CARTESIAN_POINT('Ctrl Pts',(-44.5079524583208,-59.1441977614012,
-45.29995));
#240621=CARTESIAN_POINT('Ctrl Pts',(-43.5445019199415,-59.1441977614012,
-45.2416166666667));
#240622=CARTESIAN_POINT('Ctrl Pts',(-43.0627766507519,-58.309825119875,
-45.1832833333334));
#240623=CARTESIAN_POINT('Ctrl Pts',(-42.5810513815623,-57.4754524783487,
-45.12495));
#240624=CARTESIAN_POINT('Ctrl Pts',(-43.0627766507519,-56.6410798368225,
-45.0666166666667));
#240625=CARTESIAN_POINT('Ctrl Pts',(-43.5445019199415,-55.8067071952963,
-45.0082833333334));
#240626=CARTESIAN_POINT('Ctrl Pts',(-44.5079524583208,-55.8067071952963,
-44.94995));
#240627=CARTESIAN_POINT('Origin',(-44.5079524583207,-57.4754524783487,-52.920575));
#240628=CARTESIAN_POINT('',(-44.5079524583207,-55.8067071952963,-46.34995));
#240629=CARTESIAN_POINT('',(-44.5079524583207,-55.8067071952963,-46.1912));
#240630=CARTESIAN_POINT('',(-44.5079524583207,-55.8067071952962,-52.920575));
#240631=CARTESIAN_POINT('Ctrl Pts',(-44.5079524583208,-55.8067071952963,
-46.1912));
#240632=CARTESIAN_POINT('Ctrl Pts',(-45.4714029967,-55.8067071952963,-46.1328666666667));
#240633=CARTESIAN_POINT('Ctrl Pts',(-45.9531282658897,-56.6410798368225,
-46.0745333333334));
#240634=CARTESIAN_POINT('Ctrl Pts',(-46.4348535350793,-57.4754524783487,
-46.0162));
#240635=CARTESIAN_POINT('Ctrl Pts',(-45.9531282658897,-58.309825119875,
-45.9578666666667));
#240636=CARTESIAN_POINT('Ctrl Pts',(-45.4714029967,-59.1441977614012,-45.8995333333333));
#240637=CARTESIAN_POINT('Ctrl Pts',(-44.5079524583208,-59.1441977614012,
-45.8412));
#240638=CARTESIAN_POINT('Ctrl Pts',(-43.5445019199415,-59.1441977614012,
-45.7828666666667));
#240639=CARTESIAN_POINT('Ctrl Pts',(-43.0627766507519,-58.309825119875,
-45.7245333333333));
#240640=CARTESIAN_POINT('Ctrl Pts',(-42.5810513815623,-57.4754524783487,
-45.6662));
#240641=CARTESIAN_POINT('Ctrl Pts',(-43.0627766507519,-56.6410798368225,
-45.6078666666667));
#240642=CARTESIAN_POINT('Ctrl Pts',(-43.5445019199415,-55.8067071952963,
-45.5495333333333));
#240643=CARTESIAN_POINT('Ctrl Pts',(-44.5079524583208,-55.8067071952963,
-45.4912));
#240644=CARTESIAN_POINT('Ctrl Pts',(-44.5079524583208,-55.8067071952963,
-46.34995));
#240645=CARTESIAN_POINT('Ctrl Pts',(-45.4714029967,-55.8067071952963,-46.2916166666667));
#240646=CARTESIAN_POINT('Ctrl Pts',(-45.9531282658897,-56.6410798368225,
-46.2332833333334));
#240647=CARTESIAN_POINT('Ctrl Pts',(-46.4348535350793,-57.4754524783487,
-46.17495));
#240648=CARTESIAN_POINT('Ctrl Pts',(-45.9531282658897,-58.309825119875,
-46.1166166666667));
#240649=CARTESIAN_POINT('Ctrl Pts',(-45.4714029967,-59.1441977614012,-46.0582833333333));
#240650=CARTESIAN_POINT('Ctrl Pts',(-44.5079524583208,-59.1441977614012,
-45.99995));
#240651=CARTESIAN_POINT('Ctrl Pts',(-43.5445019199415,-59.1441977614012,
-45.9416166666667));
#240652=CARTESIAN_POINT('Ctrl Pts',(-43.0627766507519,-58.309825119875,
-45.8832833333333));
#240653=CARTESIAN_POINT('Ctrl Pts',(-42.5810513815623,-57.4754524783487,
-45.82495));
#240654=CARTESIAN_POINT('Ctrl Pts',(-43.0627766507519,-56.6410798368225,
-45.7666166666667));
#240655=CARTESIAN_POINT('Ctrl Pts',(-43.5445019199415,-55.8067071952963,
-45.7082833333333));
#240656=CARTESIAN_POINT('Ctrl Pts',(-44.5079524583208,-55.8067071952963,
-45.64995));
#240657=CARTESIAN_POINT('Origin',(-44.5079524583207,-57.4754524783487,-52.920575));
#240658=CARTESIAN_POINT('',(-44.5079524583207,-55.8067071952963,-47.04995));
#240659=CARTESIAN_POINT('',(-44.5079524583207,-55.8067071952963,-46.8912));
#240660=CARTESIAN_POINT('',(-44.5079524583207,-55.8067071952962,-52.920575));
#240661=CARTESIAN_POINT('Ctrl Pts',(-44.5079524583208,-55.8067071952963,
-46.8912));
#240662=CARTESIAN_POINT('Ctrl Pts',(-45.4714029967,-55.8067071952963,-46.8328666666667));
#240663=CARTESIAN_POINT('Ctrl Pts',(-45.9531282658897,-56.6410798368225,
-46.7745333333334));
#240664=CARTESIAN_POINT('Ctrl Pts',(-46.4348535350793,-57.4754524783487,
-46.7162));
#240665=CARTESIAN_POINT('Ctrl Pts',(-45.9531282658897,-58.309825119875,
-46.6578666666667));
#240666=CARTESIAN_POINT('Ctrl Pts',(-45.4714029967,-59.1441977614012,-46.5995333333334));
#240667=CARTESIAN_POINT('Ctrl Pts',(-44.5079524583208,-59.1441977614012,
-46.5412));
#240668=CARTESIAN_POINT('Ctrl Pts',(-43.5445019199415,-59.1441977614012,
-46.4828666666667));
#240669=CARTESIAN_POINT('Ctrl Pts',(-43.0627766507519,-58.309825119875,
-46.4245333333334));
#240670=CARTESIAN_POINT('Ctrl Pts',(-42.5810513815623,-57.4754524783487,
-46.3662));
#240671=CARTESIAN_POINT('Ctrl Pts',(-43.0627766507519,-56.6410798368225,
-46.3078666666667));
#240672=CARTESIAN_POINT('Ctrl Pts',(-43.5445019199415,-55.8067071952963,
-46.2495333333334));
#240673=CARTESIAN_POINT('Ctrl Pts',(-44.5079524583208,-55.8067071952963,
-46.1912));
#240674=CARTESIAN_POINT('Ctrl Pts',(-44.5079524583208,-55.8067071952963,
-47.04995));
#240675=CARTESIAN_POINT('Ctrl Pts',(-45.4714029967,-55.8067071952963,-46.9916166666667));
#240676=CARTESIAN_POINT('Ctrl Pts',(-45.9531282658897,-56.6410798368225,
-46.9332833333334));
#240677=CARTESIAN_POINT('Ctrl Pts',(-46.4348535350793,-57.4754524783487,
-46.87495));
#240678=CARTESIAN_POINT('Ctrl Pts',(-45.9531282658897,-58.309825119875,
-46.8166166666667));
#240679=CARTESIAN_POINT('Ctrl Pts',(-45.4714029967,-59.1441977614012,-46.7582833333333));
#240680=CARTESIAN_POINT('Ctrl Pts',(-44.5079524583208,-59.1441977614012,
-46.69995));
#240681=CARTESIAN_POINT('Ctrl Pts',(-43.5445019199415,-59.1441977614012,
-46.6416166666666));
#240682=CARTESIAN_POINT('Ctrl Pts',(-43.0627766507519,-58.309825119875,
-46.5832833333334));
#240683=CARTESIAN_POINT('Ctrl Pts',(-42.5810513815623,-57.4754524783487,
-46.52495));
#240684=CARTESIAN_POINT('Ctrl Pts',(-43.0627766507519,-56.6410798368225,
-46.4666166666667));
#240685=CARTESIAN_POINT('Ctrl Pts',(-43.5445019199415,-55.8067071952963,
-46.4082833333333));
#240686=CARTESIAN_POINT('Ctrl Pts',(-44.5079524583208,-55.8067071952963,
-46.34995));
#240687=CARTESIAN_POINT('Origin',(-44.5079524583207,-57.4754524783487,-52.920575));
#240688=CARTESIAN_POINT('',(-44.5079524583207,-55.8067071952963,-47.74995));
#240689=CARTESIAN_POINT('',(-44.5079524583207,-55.8067071952963,-47.5912));
#240690=CARTESIAN_POINT('',(-44.5079524583207,-55.8067071952962,-52.920575));
#240691=CARTESIAN_POINT('Ctrl Pts',(-44.5079524583208,-55.8067071952963,
-47.5912));
#240692=CARTESIAN_POINT('Ctrl Pts',(-45.4714029967,-55.8067071952963,-47.5328666666667));
#240693=CARTESIAN_POINT('Ctrl Pts',(-45.9531282658897,-56.6410798368225,
-47.4745333333334));
#240694=CARTESIAN_POINT('Ctrl Pts',(-46.4348535350793,-57.4754524783487,
-47.4162));
#240695=CARTESIAN_POINT('Ctrl Pts',(-45.9531282658897,-58.309825119875,
-47.3578666666667));
#240696=CARTESIAN_POINT('Ctrl Pts',(-45.4714029967,-59.1441977614012,-47.2995333333334));
#240697=CARTESIAN_POINT('Ctrl Pts',(-44.5079524583208,-59.1441977614012,
-47.2412));
#240698=CARTESIAN_POINT('Ctrl Pts',(-43.5445019199415,-59.1441977614012,
-47.1828666666667));
#240699=CARTESIAN_POINT('Ctrl Pts',(-43.0627766507519,-58.309825119875,
-47.1245333333333));
#240700=CARTESIAN_POINT('Ctrl Pts',(-42.5810513815623,-57.4754524783487,
-47.0662));
#240701=CARTESIAN_POINT('Ctrl Pts',(-43.0627766507519,-56.6410798368225,
-47.0078666666667));
#240702=CARTESIAN_POINT('Ctrl Pts',(-43.5445019199415,-55.8067071952963,
-46.9495333333334));
#240703=CARTESIAN_POINT('Ctrl Pts',(-44.5079524583208,-55.8067071952963,
-46.8912));
#240704=CARTESIAN_POINT('Ctrl Pts',(-44.5079524583208,-55.8067071952963,
-47.74995));
#240705=CARTESIAN_POINT('Ctrl Pts',(-45.4714029967,-55.8067071952963,-47.6916166666667));
#240706=CARTESIAN_POINT('Ctrl Pts',(-45.9531282658897,-56.6410798368225,
-47.6332833333333));
#240707=CARTESIAN_POINT('Ctrl Pts',(-46.4348535350793,-57.4754524783487,
-47.57495));
#240708=CARTESIAN_POINT('Ctrl Pts',(-45.9531282658897,-58.309825119875,
-47.5166166666667));
#240709=CARTESIAN_POINT('Ctrl Pts',(-45.4714029967,-59.1441977614012,-47.4582833333333));
#240710=CARTESIAN_POINT('Ctrl Pts',(-44.5079524583208,-59.1441977614012,
-47.39995));
#240711=CARTESIAN_POINT('Ctrl Pts',(-43.5445019199415,-59.1441977614012,
-47.3416166666667));
#240712=CARTESIAN_POINT('Ctrl Pts',(-43.0627766507519,-58.309825119875,
-47.2832833333333));
#240713=CARTESIAN_POINT('Ctrl Pts',(-42.5810513815623,-57.4754524783487,
-47.22495));
#240714=CARTESIAN_POINT('Ctrl Pts',(-43.0627766507519,-56.6410798368225,
-47.1666166666667));
#240715=CARTESIAN_POINT('Ctrl Pts',(-43.5445019199415,-55.8067071952963,
-47.1082833333333));
#240716=CARTESIAN_POINT('Ctrl Pts',(-44.5079524583208,-55.8067071952963,
-47.04995));
#240717=CARTESIAN_POINT('Origin',(-44.5079524583207,-57.4754524783487,-52.920575));
#240718=CARTESIAN_POINT('',(-44.5079524583207,-55.8067071952963,-48.44995));
#240719=CARTESIAN_POINT('',(-44.5079524583207,-55.8067071952963,-48.2912));
#240720=CARTESIAN_POINT('',(-44.5079524583207,-55.8067071952962,-52.920575));
#240721=CARTESIAN_POINT('Ctrl Pts',(-44.5079524583208,-55.8067071952963,
-48.2912));
#240722=CARTESIAN_POINT('Ctrl Pts',(-45.4714029967,-55.8067071952963,-48.2328666666667));
#240723=CARTESIAN_POINT('Ctrl Pts',(-45.9531282658897,-56.6410798368225,
-48.1745333333334));
#240724=CARTESIAN_POINT('Ctrl Pts',(-46.4348535350793,-57.4754524783487,
-48.1162));
#240725=CARTESIAN_POINT('Ctrl Pts',(-45.9531282658897,-58.309825119875,
-48.0578666666667));
#240726=CARTESIAN_POINT('Ctrl Pts',(-45.4714029967,-59.1441977614012,-47.9995333333334));
#240727=CARTESIAN_POINT('Ctrl Pts',(-44.5079524583208,-59.1441977614012,
-47.9412));
#240728=CARTESIAN_POINT('Ctrl Pts',(-43.5445019199415,-59.1441977614012,
-47.8828666666667));
#240729=CARTESIAN_POINT('Ctrl Pts',(-43.0627766507519,-58.309825119875,
-47.8245333333333));
#240730=CARTESIAN_POINT('Ctrl Pts',(-42.5810513815623,-57.4754524783487,
-47.7662));
#240731=CARTESIAN_POINT('Ctrl Pts',(-43.0627766507519,-56.6410798368225,
-47.7078666666667));
#240732=CARTESIAN_POINT('Ctrl Pts',(-43.5445019199415,-55.8067071952963,
-47.6495333333334));
#240733=CARTESIAN_POINT('Ctrl Pts',(-44.5079524583208,-55.8067071952963,
-47.5912));
#240734=CARTESIAN_POINT('Ctrl Pts',(-44.5079524583208,-55.8067071952963,
-48.44995));
#240735=CARTESIAN_POINT('Ctrl Pts',(-45.4714029967,-55.8067071952963,-48.3916166666667));
#240736=CARTESIAN_POINT('Ctrl Pts',(-45.9531282658897,-56.6410798368225,
-48.3332833333334));
#240737=CARTESIAN_POINT('Ctrl Pts',(-46.4348535350793,-57.4754524783487,
-48.27495));
#240738=CARTESIAN_POINT('Ctrl Pts',(-45.9531282658897,-58.309825119875,
-48.2166166666667));
#240739=CARTESIAN_POINT('Ctrl Pts',(-45.4714029967,-59.1441977614012,-48.1582833333334));
#240740=CARTESIAN_POINT('Ctrl Pts',(-44.5079524583208,-59.1441977614012,
-48.09995));
#240741=CARTESIAN_POINT('Ctrl Pts',(-43.5445019199415,-59.1441977614012,
-48.0416166666667));
#240742=CARTESIAN_POINT('Ctrl Pts',(-43.0627766507519,-58.309825119875,
-47.9832833333334));
#240743=CARTESIAN_POINT('Ctrl Pts',(-42.5810513815623,-57.4754524783487,
-47.92495));
#240744=CARTESIAN_POINT('Ctrl Pts',(-43.0627766507519,-56.6410798368225,
-47.8666166666667));
#240745=CARTESIAN_POINT('Ctrl Pts',(-43.5445019199415,-55.8067071952963,
-47.8082833333333));
#240746=CARTESIAN_POINT('Ctrl Pts',(-44.5079524583208,-55.8067071952963,
-47.74995));
#240747=CARTESIAN_POINT('Origin',(-44.5079524583207,-57.4754524783487,-52.920575));
#240748=CARTESIAN_POINT('',(-44.5079524583207,-55.8067071952963,-49.14995));
#240749=CARTESIAN_POINT('',(-44.5079524583207,-55.8067071952963,-48.9912));
#240750=CARTESIAN_POINT('',(-44.5079524583207,-55.8067071952962,-52.920575));
#240751=CARTESIAN_POINT('Ctrl Pts',(-44.5079524583208,-55.8067071952963,
-48.9912));
#240752=CARTESIAN_POINT('Ctrl Pts',(-45.4714029967,-55.8067071952963,-48.9328666666667));
#240753=CARTESIAN_POINT('Ctrl Pts',(-45.9531282658897,-56.6410798368225,
-48.8745333333334));
#240754=CARTESIAN_POINT('Ctrl Pts',(-46.4348535350793,-57.4754524783487,
-48.8162));
#240755=CARTESIAN_POINT('Ctrl Pts',(-45.9531282658897,-58.309825119875,
-48.7578666666667));
#240756=CARTESIAN_POINT('Ctrl Pts',(-45.4714029967,-59.1441977614012,-48.6995333333333));
#240757=CARTESIAN_POINT('Ctrl Pts',(-44.5079524583208,-59.1441977614012,
-48.6412));
#240758=CARTESIAN_POINT('Ctrl Pts',(-43.5445019199415,-59.1441977614012,
-48.5828666666667));
#240759=CARTESIAN_POINT('Ctrl Pts',(-43.0627766507519,-58.309825119875,
-48.5245333333334));
#240760=CARTESIAN_POINT('Ctrl Pts',(-42.5810513815623,-57.4754524783487,
-48.4662));
#240761=CARTESIAN_POINT('Ctrl Pts',(-43.0627766507519,-56.6410798368225,
-48.4078666666667));
#240762=CARTESIAN_POINT('Ctrl Pts',(-43.5445019199415,-55.8067071952963,
-48.3495333333333));
#240763=CARTESIAN_POINT('Ctrl Pts',(-44.5079524583208,-55.8067071952963,
-48.2912));
#240764=CARTESIAN_POINT('Ctrl Pts',(-44.5079524583208,-55.8067071952963,
-49.14995));
#240765=CARTESIAN_POINT('Ctrl Pts',(-45.4714029967,-55.8067071952963,-49.0916166666667));
#240766=CARTESIAN_POINT('Ctrl Pts',(-45.9531282658897,-56.6410798368225,
-49.0332833333333));
#240767=CARTESIAN_POINT('Ctrl Pts',(-46.4348535350793,-57.4754524783487,
-48.97495));
#240768=CARTESIAN_POINT('Ctrl Pts',(-45.9531282658897,-58.309825119875,
-48.9166166666667));
#240769=CARTESIAN_POINT('Ctrl Pts',(-45.4714029967,-59.1441977614012,-48.8582833333333));
#240770=CARTESIAN_POINT('Ctrl Pts',(-44.5079524583208,-59.1441977614012,
-48.79995));
#240771=CARTESIAN_POINT('Ctrl Pts',(-43.5445019199415,-59.1441977614012,
-48.7416166666667));
#240772=CARTESIAN_POINT('Ctrl Pts',(-43.0627766507519,-58.309825119875,
-48.6832833333334));
#240773=CARTESIAN_POINT('Ctrl Pts',(-42.5810513815623,-57.4754524783487,
-48.62495));
#240774=CARTESIAN_POINT('Ctrl Pts',(-43.0627766507519,-56.6410798368225,
-48.5666166666667));
#240775=CARTESIAN_POINT('Ctrl Pts',(-43.5445019199415,-55.8067071952963,
-48.5082833333334));
#240776=CARTESIAN_POINT('Ctrl Pts',(-44.5079524583208,-55.8067071952963,
-48.44995));
#240777=CARTESIAN_POINT('Origin',(-44.5079524583207,-57.4754524783487,-52.920575));
#240778=CARTESIAN_POINT('',(-44.5079524583207,-55.8067071952963,-49.84995));
#240779=CARTESIAN_POINT('',(-44.5079524583207,-55.8067071952963,-49.6912));
#240780=CARTESIAN_POINT('',(-44.5079524583207,-55.8067071952962,-52.920575));
#240781=CARTESIAN_POINT('Ctrl Pts',(-44.5079524583208,-55.8067071952963,
-49.6912));
#240782=CARTESIAN_POINT('Ctrl Pts',(-45.4714029967,-55.8067071952963,-49.6328666666667));
#240783=CARTESIAN_POINT('Ctrl Pts',(-45.9531282658897,-56.6410798368225,
-49.5745333333334));
#240784=CARTESIAN_POINT('Ctrl Pts',(-46.4348535350793,-57.4754524783487,
-49.5162));
#240785=CARTESIAN_POINT('Ctrl Pts',(-45.9531282658897,-58.309825119875,
-49.4578666666667));
#240786=CARTESIAN_POINT('Ctrl Pts',(-45.4714029967,-59.1441977614012,-49.3995333333333));
#240787=CARTESIAN_POINT('Ctrl Pts',(-44.5079524583208,-59.1441977614012,
-49.3412));
#240788=CARTESIAN_POINT('Ctrl Pts',(-43.5445019199415,-59.1441977614012,
-49.2828666666667));
#240789=CARTESIAN_POINT('Ctrl Pts',(-43.0627766507519,-58.309825119875,
-49.2245333333334));
#240790=CARTESIAN_POINT('Ctrl Pts',(-42.5810513815623,-57.4754524783487,
-49.1662));
#240791=CARTESIAN_POINT('Ctrl Pts',(-43.0627766507519,-56.6410798368225,
-49.1078666666667));
#240792=CARTESIAN_POINT('Ctrl Pts',(-43.5445019199415,-55.8067071952963,
-49.0495333333334));
#240793=CARTESIAN_POINT('Ctrl Pts',(-44.5079524583208,-55.8067071952963,
-48.9912));
#240794=CARTESIAN_POINT('Ctrl Pts',(-44.5079524583208,-55.8067071952963,
-49.84995));
#240795=CARTESIAN_POINT('Ctrl Pts',(-45.4714029967,-55.8067071952963,-49.7916166666667));
#240796=CARTESIAN_POINT('Ctrl Pts',(-45.9531282658897,-56.6410798368225,
-49.7332833333334));
#240797=CARTESIAN_POINT('Ctrl Pts',(-46.4348535350793,-57.4754524783487,
-49.67495));
#240798=CARTESIAN_POINT('Ctrl Pts',(-45.9531282658897,-58.309825119875,
-49.6166166666667));
#240799=CARTESIAN_POINT('Ctrl Pts',(-45.4714029967,-59.1441977614012,-49.5582833333334));
#240800=CARTESIAN_POINT('Ctrl Pts',(-44.5079524583208,-59.1441977614012,
-49.49995));
#240801=CARTESIAN_POINT('Ctrl Pts',(-43.5445019199415,-59.1441977614012,
-49.4416166666667));
#240802=CARTESIAN_POINT('Ctrl Pts',(-43.0627766507519,-58.309825119875,
-49.3832833333334));
#240803=CARTESIAN_POINT('Ctrl Pts',(-42.5810513815623,-57.4754524783487,
-49.32495));
#240804=CARTESIAN_POINT('Ctrl Pts',(-43.0627766507519,-56.6410798368225,
-49.2666166666667));
#240805=CARTESIAN_POINT('Ctrl Pts',(-43.5445019199415,-55.8067071952963,
-49.2082833333334));
#240806=CARTESIAN_POINT('Ctrl Pts',(-44.5079524583208,-55.8067071952963,
-49.14995));
#240807=CARTESIAN_POINT('Origin',(-44.5079524583207,-57.4754524783487,-52.920575));
#240808=CARTESIAN_POINT('',(-44.5079524583207,-55.8067071952963,-50.54995));
#240809=CARTESIAN_POINT('',(-44.5079524583207,-55.8067071952963,-50.3912));
#240810=CARTESIAN_POINT('',(-44.5079524583207,-55.8067071952962,-52.920575));
#240811=CARTESIAN_POINT('Ctrl Pts',(-44.5079524583208,-55.8067071952963,
-50.3912));
#240812=CARTESIAN_POINT('Ctrl Pts',(-45.4714029967,-55.8067071952963,-50.3328666666667));
#240813=CARTESIAN_POINT('Ctrl Pts',(-45.9531282658897,-56.6410798368225,
-50.2745333333334));
#240814=CARTESIAN_POINT('Ctrl Pts',(-46.4348535350793,-57.4754524783487,
-50.2162));
#240815=CARTESIAN_POINT('Ctrl Pts',(-45.9531282658897,-58.309825119875,
-50.1578666666667));
#240816=CARTESIAN_POINT('Ctrl Pts',(-45.4714029967,-59.1441977614012,-50.0995333333333));
#240817=CARTESIAN_POINT('Ctrl Pts',(-44.5079524583208,-59.1441977614012,
-50.0412));
#240818=CARTESIAN_POINT('Ctrl Pts',(-43.5445019199415,-59.1441977614012,
-49.9828666666667));
#240819=CARTESIAN_POINT('Ctrl Pts',(-43.0627766507519,-58.309825119875,
-49.9245333333334));
#240820=CARTESIAN_POINT('Ctrl Pts',(-42.5810513815623,-57.4754524783487,
-49.8662));
#240821=CARTESIAN_POINT('Ctrl Pts',(-43.0627766507519,-56.6410798368225,
-49.8078666666667));
#240822=CARTESIAN_POINT('Ctrl Pts',(-43.5445019199415,-55.8067071952963,
-49.7495333333333));
#240823=CARTESIAN_POINT('Ctrl Pts',(-44.5079524583208,-55.8067071952963,
-49.6912));
#240824=CARTESIAN_POINT('Ctrl Pts',(-44.5079524583208,-55.8067071952963,
-50.54995));
#240825=CARTESIAN_POINT('Ctrl Pts',(-45.4714029967,-55.8067071952963,-50.4916166666667));
#240826=CARTESIAN_POINT('Ctrl Pts',(-45.9531282658897,-56.6410798368225,
-50.4332833333333));
#240827=CARTESIAN_POINT('Ctrl Pts',(-46.4348535350793,-57.4754524783487,
-50.37495));
#240828=CARTESIAN_POINT('Ctrl Pts',(-45.9531282658897,-58.309825119875,
-50.3166166666667));
#240829=CARTESIAN_POINT('Ctrl Pts',(-45.4714029967,-59.1441977614012,-50.2582833333334));
#240830=CARTESIAN_POINT('Ctrl Pts',(-44.5079524583208,-59.1441977614012,
-50.19995));
#240831=CARTESIAN_POINT('Ctrl Pts',(-43.5445019199415,-59.1441977614012,
-50.1416166666667));
#240832=CARTESIAN_POINT('Ctrl Pts',(-43.0627766507519,-58.309825119875,
-50.0832833333334));
#240833=CARTESIAN_POINT('Ctrl Pts',(-42.5810513815623,-57.4754524783487,
-50.02495));
#240834=CARTESIAN_POINT('Ctrl Pts',(-43.0627766507519,-56.6410798368225,
-49.9666166666667));
#240835=CARTESIAN_POINT('Ctrl Pts',(-43.5445019199415,-55.8067071952963,
-49.9082833333334));
#240836=CARTESIAN_POINT('Ctrl Pts',(-44.5079524583208,-55.8067071952963,
-49.84995));
#240837=CARTESIAN_POINT('Origin',(-44.5079524583207,-57.4754524783487,-52.920575));
#240838=CARTESIAN_POINT('',(-44.5079524583207,-55.8067071952963,-51.24995));
#240839=CARTESIAN_POINT('',(-44.5079524583207,-55.8067071952963,-51.0912));
#240840=CARTESIAN_POINT('',(-44.5079524583207,-55.8067071952962,-52.920575));
#240841=CARTESIAN_POINT('Ctrl Pts',(-44.5079524583208,-55.8067071952963,
-51.0912));
#240842=CARTESIAN_POINT('Ctrl Pts',(-45.4714029967,-55.8067071952963,-51.0328666666667));
#240843=CARTESIAN_POINT('Ctrl Pts',(-45.9531282658897,-56.6410798368225,
-50.9745333333333));
#240844=CARTESIAN_POINT('Ctrl Pts',(-46.4348535350793,-57.4754524783487,
-50.9162));
#240845=CARTESIAN_POINT('Ctrl Pts',(-45.9531282658897,-58.309825119875,
-50.8578666666667));
#240846=CARTESIAN_POINT('Ctrl Pts',(-45.4714029967,-59.1441977614012,-50.7995333333334));
#240847=CARTESIAN_POINT('Ctrl Pts',(-44.5079524583208,-59.1441977614012,
-50.7412));
#240848=CARTESIAN_POINT('Ctrl Pts',(-43.5445019199415,-59.1441977614012,
-50.6828666666667));
#240849=CARTESIAN_POINT('Ctrl Pts',(-43.0627766507519,-58.309825119875,
-50.6245333333333));
#240850=CARTESIAN_POINT('Ctrl Pts',(-42.5810513815623,-57.4754524783487,
-50.5662));
#240851=CARTESIAN_POINT('Ctrl Pts',(-43.0627766507519,-56.6410798368225,
-50.5078666666667));
#240852=CARTESIAN_POINT('Ctrl Pts',(-43.5445019199415,-55.8067071952963,
-50.4495333333333));
#240853=CARTESIAN_POINT('Ctrl Pts',(-44.5079524583208,-55.8067071952963,
-50.3912));
#240854=CARTESIAN_POINT('Ctrl Pts',(-44.5079524583208,-55.8067071952963,
-51.24995));
#240855=CARTESIAN_POINT('Ctrl Pts',(-45.4714029967,-55.8067071952963,-51.1916166666667));
#240856=CARTESIAN_POINT('Ctrl Pts',(-45.9531282658897,-56.6410798368225,
-51.1332833333334));
#240857=CARTESIAN_POINT('Ctrl Pts',(-46.4348535350793,-57.4754524783487,
-51.07495));
#240858=CARTESIAN_POINT('Ctrl Pts',(-45.9531282658897,-58.309825119875,
-51.0166166666667));
#240859=CARTESIAN_POINT('Ctrl Pts',(-45.4714029967,-59.1441977614012,-50.9582833333334));
#240860=CARTESIAN_POINT('Ctrl Pts',(-44.5079524583208,-59.1441977614012,
-50.89995));
#240861=CARTESIAN_POINT('Ctrl Pts',(-43.5445019199415,-59.1441977614012,
-50.8416166666667));
#240862=CARTESIAN_POINT('Ctrl Pts',(-43.0627766507519,-58.309825119875,
-50.7832833333333));
#240863=CARTESIAN_POINT('Ctrl Pts',(-42.5810513815623,-57.4754524783487,
-50.72495));
#240864=CARTESIAN_POINT('Ctrl Pts',(-43.0627766507519,-56.6410798368225,
-50.6666166666667));
#240865=CARTESIAN_POINT('Ctrl Pts',(-43.5445019199415,-55.8067071952963,
-50.6082833333334));
#240866=CARTESIAN_POINT('Ctrl Pts',(-44.5079524583208,-55.8067071952963,
-50.54995));
#240867=CARTESIAN_POINT('Origin',(-44.5079524583207,-57.4754524783487,-52.920575));
#240868=CARTESIAN_POINT('',(-44.5079524583207,-55.8067071952963,-51.94995));
#240869=CARTESIAN_POINT('',(-44.5079524583207,-55.8067071952963,-51.7912));
#240870=CARTESIAN_POINT('',(-44.5079524583207,-55.8067071952962,-52.920575));
#240871=CARTESIAN_POINT('Ctrl Pts',(-44.5079524583208,-55.8067071952963,
-51.7912));
#240872=CARTESIAN_POINT('Ctrl Pts',(-45.4714029967,-55.8067071952963,-51.7328666666667));
#240873=CARTESIAN_POINT('Ctrl Pts',(-45.9531282658897,-56.6410798368225,
-51.6745333333334));
#240874=CARTESIAN_POINT('Ctrl Pts',(-46.4348535350793,-57.4754524783487,
-51.6162));
#240875=CARTESIAN_POINT('Ctrl Pts',(-45.9531282658897,-58.309825119875,
-51.5578666666667));
#240876=CARTESIAN_POINT('Ctrl Pts',(-45.4714029967,-59.1441977614012,-51.4995333333334));
#240877=CARTESIAN_POINT('Ctrl Pts',(-44.5079524583208,-59.1441977614012,
-51.4412));
#240878=CARTESIAN_POINT('Ctrl Pts',(-43.5445019199415,-59.1441977614012,
-51.3828666666667));
#240879=CARTESIAN_POINT('Ctrl Pts',(-43.0627766507519,-58.309825119875,
-51.3245333333334));
#240880=CARTESIAN_POINT('Ctrl Pts',(-42.5810513815623,-57.4754524783487,
-51.2662));
#240881=CARTESIAN_POINT('Ctrl Pts',(-43.0627766507519,-56.6410798368225,
-51.2078666666667));
#240882=CARTESIAN_POINT('Ctrl Pts',(-43.5445019199415,-55.8067071952963,
-51.1495333333334));
#240883=CARTESIAN_POINT('Ctrl Pts',(-44.5079524583208,-55.8067071952963,
-51.0912));
#240884=CARTESIAN_POINT('Ctrl Pts',(-44.5079524583208,-55.8067071952963,
-51.94995));
#240885=CARTESIAN_POINT('Ctrl Pts',(-45.4714029967,-55.8067071952963,-51.8916166666667));
#240886=CARTESIAN_POINT('Ctrl Pts',(-45.9531282658897,-56.6410798368225,
-51.8332833333334));
#240887=CARTESIAN_POINT('Ctrl Pts',(-46.4348535350793,-57.4754524783487,
-51.77495));
#240888=CARTESIAN_POINT('Ctrl Pts',(-45.9531282658897,-58.309825119875,
-51.7166166666667));
#240889=CARTESIAN_POINT('Ctrl Pts',(-45.4714029967,-59.1441977614012,-51.6582833333333));
#240890=CARTESIAN_POINT('Ctrl Pts',(-44.5079524583208,-59.1441977614012,
-51.59995));
#240891=CARTESIAN_POINT('Ctrl Pts',(-43.5445019199415,-59.1441977614012,
-51.5416166666667));
#240892=CARTESIAN_POINT('Ctrl Pts',(-43.0627766507519,-58.309825119875,
-51.4832833333334));
#240893=CARTESIAN_POINT('Ctrl Pts',(-42.5810513815623,-57.4754524783487,
-51.42495));
#240894=CARTESIAN_POINT('Ctrl Pts',(-43.0627766507519,-56.6410798368225,
-51.3666166666667));
#240895=CARTESIAN_POINT('Ctrl Pts',(-43.5445019199415,-55.8067071952963,
-51.3082833333333));
#240896=CARTESIAN_POINT('Ctrl Pts',(-44.5079524583208,-55.8067071952963,
-51.24995));
#240897=CARTESIAN_POINT('Origin',(-44.5079524583207,-57.4754524783487,-52.920575));
#240898=CARTESIAN_POINT('',(-44.5079524583208,-55.8067071952963,-52.64995));
#240899=CARTESIAN_POINT('',(-44.5079524583207,-55.8067071952963,-52.4912));
#240900=CARTESIAN_POINT('',(-44.5079524583207,-55.8067071952962,-52.920575));
#240901=CARTESIAN_POINT('',(-42.8554737113965,-57.2430200996376,-52.64995));
#240902=CARTESIAN_POINT('Origin',(-44.5079524583207,-57.4754524783487,-52.64995));
#240903=CARTESIAN_POINT('Ctrl Pts',(-42.8554737113965,-57.2430200996376,
-52.64995));
#240904=CARTESIAN_POINT('Ctrl Pts',(-42.9006402736028,-56.9219082798,-52.6275001713604));
#240905=CARTESIAN_POINT('Ctrl Pts',(-43.0627766507519,-56.6410798368225,
-52.6078666666667));
#240906=CARTESIAN_POINT('Ctrl Pts',(-43.5445019199415,-55.8067071952963,
-52.5495333333333));
#240907=CARTESIAN_POINT('Ctrl Pts',(-44.5079524583208,-55.8067071952963,
-52.4912));
#240908=CARTESIAN_POINT('Origin',(-44.5079524583206,-57.475452478349,235.35105));
#240909=CARTESIAN_POINT('',(-44.5079524583206,-59.475452478349,-52.4912000000001));
#240910=CARTESIAN_POINT('',(-44.5079524583208,-59.4754524783489,-52.64995));
#240911=CARTESIAN_POINT('',(-44.5079524583206,-59.475452478349,235.35105));
#240912=CARTESIAN_POINT('',(-46.4884569292071,-57.7540239068883,-52.64995));
#240913=CARTESIAN_POINT('Origin',(-44.5079524583206,-57.4754524783489,-52.64995));
#240914=CARTESIAN_POINT('Ctrl Pts',(-46.4884569292073,-57.7540239068874,
-52.6499500000019));
#240915=CARTESIAN_POINT('Ctrl Pts',(-46.4571755210013,-57.9764191795565,
-52.6369769424295));
#240916=CARTESIAN_POINT('Ctrl Pts',(-46.3886551524865,-58.1919907826354,
-52.62440193225));
#240917=CARTESIAN_POINT('Ctrl Pts',(-46.1844788607781,-58.5881583563758,
-52.6012921571151));
#240918=CARTESIAN_POINT('Ctrl Pts',(-46.0513419995026,-58.7665170353615,
-52.5898464658721));
#240919=CARTESIAN_POINT('Ctrl Pts',(-45.7029579949069,-59.1003460934955,
-52.5625100701119));
#240920=CARTESIAN_POINT('Ctrl Pts',(-45.4806104593203,-59.2424403948135,
-52.5471330671567));
#240921=CARTESIAN_POINT('Ctrl Pts',(-45.0046748918109,-59.4288214762729,
-52.5176535685792));
#240922=CARTESIAN_POINT('Ctrl Pts',(-44.757311248525,-59.475452478349,-52.5037971444069));
#240923=CARTESIAN_POINT('Ctrl Pts',(-44.5079524583206,-59.475452478349,
-52.4912000000001));
#240924=CARTESIAN_POINT('Origin',(-44.5079524583206,-57.475452478349,235.35105));
#240925=CARTESIAN_POINT('',(-44.5079524583206,-59.475452478349,-51.7912000000001));
#240926=CARTESIAN_POINT('',(-44.5079524583207,-59.475452478349,-51.9499499999999));
#240927=CARTESIAN_POINT('',(-44.5079524583206,-59.475452478349,235.35105));
#240928=CARTESIAN_POINT('Ctrl Pts',(-44.5079524583208,-59.475452478349,
-51.9499499999999));
#240929=CARTESIAN_POINT('Ctrl Pts',(-44.5462530077334,-59.475452478349,
-51.9518848728448));
#240930=CARTESIAN_POINT('Ctrl Pts',(-44.5845870500328,-59.4743523002202,
-51.9538535262171));
#240931=CARTESIAN_POINT('Ctrl Pts',(-44.8876628879482,-59.4569033381397,
-51.9696732844808));
#240932=CARTESIAN_POINT('Ctrl Pts',(-45.1467151397867,-59.389156943588,
-51.9847360611302));
#240933=CARTESIAN_POINT('Ctrl Pts',(-45.618038707975,-59.159186107665,-52.0152539378795));
#240934=CARTESIAN_POINT('Ctrl Pts',(-45.8267932266755,-59.0012079574294,
-52.0304075257151));
#240935=CARTESIAN_POINT('Ctrl Pts',(-46.1695860436834,-58.6174282183136,
-52.0589183598922));
#240936=CARTESIAN_POINT('Ctrl Pts',(-46.3015774721523,-58.3963443508154,
-52.0712313074395));
#240937=CARTESIAN_POINT('Ctrl Pts',(-46.47919784431,-57.9058111734347,-52.0998457427868));
#240938=CARTESIAN_POINT('Ctrl Pts',(-46.5189305178084,-57.6396417713126,
-52.1153722912439));
#240939=CARTESIAN_POINT('Ctrl Pts',(-46.4922937440839,-57.1175481044096,
-52.1458277551466));
#240940=CARTESIAN_POINT('Ctrl Pts',(-46.4301366114906,-56.8663947730836,
-52.1604783661406));
#240941=CARTESIAN_POINT('Ctrl Pts',(-46.2118887101475,-56.3959354740626,
-52.1879218252502));
#240942=CARTESIAN_POINT('Ctrl Pts',(-46.0558483200505,-56.1820831689376,
-52.2011431051022));
#240943=CARTESIAN_POINT('Ctrl Pts',(-45.669376355768,-55.8261041251902,
-52.2310496753152));
#240944=CARTESIAN_POINT('Ctrl Pts',(-45.4425144507322,-55.687759774618,
-52.2465453622934));
#240945=CARTESIAN_POINT('Ctrl Pts',(-44.9572247708576,-55.5101339142034,
-52.2762420526951));
#240946=CARTESIAN_POINT('Ctrl Pts',(-44.7047220768785,-55.4690808303961,
-52.289823723447));
#240947=CARTESIAN_POINT('Ctrl Pts',(-44.1863112510203,-55.4837566408039,
-52.3164409230299));
#240948=CARTESIAN_POINT('Ctrl Pts',(-43.9254355283081,-55.5438909091359,
-52.3313737977038));
#240949=CARTESIAN_POINT('Ctrl Pts',(-43.446958185133,-55.7602489202191,
-52.3618560291959));
#240950=CARTESIAN_POINT('Ctrl Pts',(-43.2331403216415,-55.9126018978207,
-52.3771013403007));
#240951=CARTESIAN_POINT('Ctrl Pts',(-42.8797975441431,-56.2864280845043,
-52.4058548270031));
#240952=CARTESIAN_POINT('Ctrl Pts',(-42.7419899350815,-56.5028085687393,
-52.4182124386061));
#240953=CARTESIAN_POINT('Ctrl Pts',(-42.5499967148387,-56.9877533495184,
-52.4465008841515));
#240954=CARTESIAN_POINT('Ctrl Pts',(-42.5024277035354,-57.2534607575844,
-52.4620004829554));
#240955=CARTESIAN_POINT('Ctrl Pts',(-42.5142671348049,-57.7775857217385,
-52.4925744391976));
#240956=CARTESIAN_POINT('Ctrl Pts',(-42.5695550463785,-58.0310735043884,
-52.5073612265188));
#240957=CARTESIAN_POINT('Ctrl Pts',(-42.7742904349951,-58.5060182293466,
-52.5350663354747));
#240958=CARTESIAN_POINT('Ctrl Pts',(-42.922835831421,-58.7224777476931,
-52.5479110797891));
#240959=CARTESIAN_POINT('Ctrl Pts',(-43.2963567570324,-59.0882185387781,
-52.5774481051372));
#240960=CARTESIAN_POINT('Ctrl Pts',(-43.5183762271097,-59.23320900112,-52.5928930061934));
#240961=CARTESIAN_POINT('Ctrl Pts',(-43.9991306930556,-59.4264496379907,
-52.6228160169642));
#240962=CARTESIAN_POINT('Ctrl Pts',(-44.2523385936067,-59.475452478349,
-52.6370368608098));
#240963=CARTESIAN_POINT('Ctrl Pts',(-44.5079524583208,-59.475452478349,
-52.6499499999999));
#240964=CARTESIAN_POINT('Ctrl Pts',(-44.5079524583206,-59.475452478349,
-52.4912000000001));
#240965=CARTESIAN_POINT('Ctrl Pts',(-44.4925286932249,-59.475452478349,
-52.4904208199437));
#240966=CARTESIAN_POINT('Ctrl Pts',(-44.477097811945,-59.4752740593648,
-52.4896360765039));
#240967=CARTESIAN_POINT('Ctrl Pts',(-44.2069952709762,-59.4690209166747,
-52.475808612886));
#240968=CARTESIAN_POINT('Ctrl Pts',(-43.9558318021867,-59.4145263539375,
-52.4615308747119));
#240969=CARTESIAN_POINT('Ctrl Pts',(-43.4784164929003,-59.2104037693686,
-52.4314591618121));
#240970=CARTESIAN_POINT('Ctrl Pts',(-43.2581721074967,-59.0591390019468,
-52.4159209341823));
#240971=CARTESIAN_POINT('Ctrl Pts',(-42.8935213295786,-58.6839566192263,
-52.3865566325171));
#240972=CARTESIAN_POINT('Ctrl Pts',(-42.7509892352242,-58.4653719356495,
-52.3739453016761));
#240973=CARTESIAN_POINT('Ctrl Pts',(-42.5573395383357,-57.9868257843532,
-52.3460301095172));
#240974=CARTESIAN_POINT('Ctrl Pts',(-42.5077592542388,-57.7315582833632,
-52.3311395052927));
#240975=CARTESIAN_POINT('Ctrl Pts',(-42.5081545171318,-57.2060702590284,
-52.3004860372065));
#240976=CARTESIAN_POINT('Ctrl Pts',(-42.5621729208094,-56.9409096061898,
-52.2850183324575));
#240977=CARTESIAN_POINT('Ctrl Pts',(-42.7659398738441,-56.4606757368225,
-52.2570046900777));
#240978=CARTESIAN_POINT('Ctrl Pts',(-42.9085687365412,-56.248111646219,
-52.2445337968481));
#240979=CARTESIAN_POINT('Ctrl Pts',(-43.2706479599599,-55.8826429388458,
-52.215582720886));
#240980=CARTESIAN_POINT('Ctrl Pts',(-43.4885745251695,-55.7351015622851,
-52.2002701841412));
#240981=CARTESIAN_POINT('Ctrl Pts',(-43.9727146276586,-55.5302656294541,
-52.1698379411483));
#240982=CARTESIAN_POINT('Ctrl Pts',(-44.2349347373735,-55.4765163817129,
-52.1550233802994));
#240983=CARTESIAN_POINT('Ctrl Pts',(-44.7539426804031,-55.4744641746777,
-52.1287442038941));
#240984=CARTESIAN_POINT('Ctrl Pts',(-45.005839303614,-55.5218192558505,
-52.1146953140424));
#240985=CARTESIAN_POINT('Ctrl Pts',(-45.4876087021152,-55.7119684484848,
-52.0848111978816));
#240986=CARTESIAN_POINT('Ctrl Pts',(-45.7114435671204,-55.8564342500284,
-52.0692898890414));
#240987=CARTESIAN_POINT('Ctrl Pts',(-46.0876759464907,-56.2215404682432,
-52.0396343944449));
#240988=CARTESIAN_POINT('Ctrl Pts',(-46.2373163864829,-56.4376165206826,
-52.0267404308638));
#240989=CARTESIAN_POINT('Ctrl Pts',(-46.4440468364767,-56.9119056175668,
-51.9990735668789));
#240990=CARTESIAN_POINT('Ctrl Pts',(-46.50035524974,-57.1650600281304,-51.9843062262627));
#240991=CARTESIAN_POINT('Ctrl Pts',(-46.5143879192962,-57.688910498562,
-51.9537482821542));
#240992=CARTESIAN_POINT('Ctrl Pts',(-46.4679778896413,-57.9547002203644,
-51.9382438817157));
#240993=CARTESIAN_POINT('Ctrl Pts',(-46.2781052302168,-58.440480852866,
-51.9099066781532));
#240994=CARTESIAN_POINT('Ctrl Pts',(-46.1411602364249,-58.6575521547172,
-51.8975620592599));
#240995=CARTESIAN_POINT('Ctrl Pts',(-45.7893819371086,-59.0328638289246,
-51.8688442803793));
#240996=CARTESIAN_POINT('Ctrl Pts',(-45.5763081280395,-59.1860638545062,
-51.8536118519604));
#240997=CARTESIAN_POINT('Ctrl Pts',(-45.0988702536503,-59.404461648935,
-51.8231226388258));
#240998=CARTESIAN_POINT('Ctrl Pts',(-44.8382512812852,-59.4657317505508,
-51.8081696062334));
#240999=CARTESIAN_POINT('Ctrl Pts',(-44.5514667254131,-59.4750976575076,
-51.7934086091506));
#241000=CARTESIAN_POINT('Ctrl Pts',(-44.5297032459204,-59.475452478349,
-51.7922988095192));
#241001=CARTESIAN_POINT('Ctrl Pts',(-44.5079524583207,-59.475452478349,
-51.7912000000001));
#241002=CARTESIAN_POINT('Origin',(-44.5079524583206,-57.475452478349,235.35105));
#241003=CARTESIAN_POINT('',(-44.5079524583208,-59.475452478349,-51.0912000000001));
#241004=CARTESIAN_POINT('',(-44.5079524583208,-59.475452478349,-51.2499499999999));
#241005=CARTESIAN_POINT('',(-44.5079524583206,-59.475452478349,235.35105));
#241006=CARTESIAN_POINT('Ctrl Pts',(-44.5079524583209,-59.475452478349,
-51.2499499999999));
#241007=CARTESIAN_POINT('Ctrl Pts',(-44.5831034040224,-59.475452478349,
-51.2537464866388));
#241008=CARTESIAN_POINT('Ctrl Pts',(-44.6583291409112,-59.4712171014566,
-51.2576702834159));
#241009=CARTESIAN_POINT('Ctrl Pts',(-44.9968439360842,-59.432834683858,
-51.2758909113062));
#241010=CARTESIAN_POINT('Ctrl Pts',(-45.2518131349861,-59.3508177570532,
-51.2911636435384));
#241011=CARTESIAN_POINT('Ctrl Pts',(-45.7085146235329,-59.0956947682382,
-51.3216764443555));
#241012=CARTESIAN_POINT('Ctrl Pts',(-45.9072800035909,-58.9275012065103,
-51.3366233489031));
#241013=CARTESIAN_POINT('Ctrl Pts',(-46.2298326839446,-58.5250156496126,
-51.364657275202));
#241014=CARTESIAN_POINT('Ctrl Pts',(-46.3506201644387,-58.2946208767058,
-51.3771651767626));
#241015=CARTESIAN_POINT('Ctrl Pts',(-46.5001699212596,-57.7936965633861,
-51.4063857617063));
#241016=CARTESIAN_POINT('Ctrl Pts',(-46.5247591345641,-57.5272642115913,
-51.4219276488944));
#241017=CARTESIAN_POINT('Ctrl Pts',(-46.469740912205,-57.0102643525022,
-51.4520859740079));
#241018=CARTESIAN_POINT('Ctrl Pts',(-46.3945149093217,-56.7641577939788,
-51.4664421899218));
#241019=CARTESIAN_POINT('Ctrl Pts',(-46.1499417528502,-56.3027437439466,
-51.493358009507));
#241020=CARTESIAN_POINT('Ctrl Pts',(-45.9787581791892,-56.0940831577275,
-51.5076042232839));
#241021=CARTESIAN_POINT('Ctrl Pts',(-45.5687807345382,-55.7599101662309,
-51.5380622369886));
#241022=CARTESIAN_POINT('Ctrl Pts',(-45.3355169770568,-55.6360001125875,
-51.5534603333726));
#241023=CARTESIAN_POINT('Ctrl Pts',(-44.8424610981469,-55.4874181004114,
-51.5827022455307));
#241024=CARTESIAN_POINT('Ctrl Pts',(-44.5882829367332,-55.4610806010797,
-51.5954726732046));
#241025=CARTESIAN_POINT('Ctrl Pts',(-44.071703466241,-55.5056726343423,
-51.6228699126051));
#241026=CARTESIAN_POINT('Ctrl Pts',(-43.8146576896166,-55.5808159438177,
-51.6380470691935));
#241027=CARTESIAN_POINT('Ctrl Pts',(-43.3507131484704,-55.8238845064,-51.6685741881859));
#241028=CARTESIAN_POINT('Ctrl Pts',(-43.1470541791173,-55.9872118799288,
-51.6836263773153));
#241029=CARTESIAN_POINT('Ctrl Pts',(-42.8146704204402,-56.3806739780254,
-51.7118937672742));
#241030=CARTESIAN_POINT('Ctrl Pts',(-42.688429019529,-56.6064987614925,
-51.7242610331834));
#241031=CARTESIAN_POINT('Ctrl Pts',(-42.5251621390899,-57.1024333545853,
-51.7531905511137));
#241032=CARTESIAN_POINT('Ctrl Pts',(-42.4932033721177,-57.3688416175935,
-51.7687310331225));
#241033=CARTESIAN_POINT('Ctrl Pts',(-42.5344451390283,-57.8885131333919,
-51.7990452048774));
#241034=CARTESIAN_POINT('Ctrl Pts',(-42.6033451648736,-58.1371640294665,
-51.8135498404817));
#241035=CARTESIAN_POINT('Ctrl Pts',(-42.8350651409272,-58.6030456506682,
-51.8407262683851));
#241036=CARTESIAN_POINT('Ctrl Pts',(-42.9987643329247,-58.814265075649,
-51.8544239775063));
#241037=CARTESIAN_POINT('Ctrl Pts',(-43.3972520846828,-59.1592529371033,
-51.8846169869057));
#241038=CARTESIAN_POINT('Ctrl Pts',(-43.6274837288687,-59.2902844759237,
-51.9000696165241));
#241039=CARTESIAN_POINT('Ctrl Pts',(-44.0803611280474,-59.4409948871493,
-51.92734386458));
#241040=CARTESIAN_POINT('Ctrl Pts',(-44.293581933249,-59.475452478349,-51.9391203979687));
#241041=CARTESIAN_POINT('Ctrl Pts',(-44.5079524583208,-59.475452478349,
-51.9499499999999));
#241042=CARTESIAN_POINT('Ctrl Pts',(-44.5079524583207,-59.475452478349,
-51.7912000000001));
#241043=CARTESIAN_POINT('Ctrl Pts',(-44.2766221791823,-59.475452478349,
-51.7795136225936));
#241044=CARTESIAN_POINT('Ctrl Pts',(-44.0468438420911,-59.4353231275902,
-51.7667352070288));
#241045=CARTESIAN_POINT('Ctrl Pts',(-43.5814391635927,-59.2673125783722,
-51.7383235166572));
#241046=CARTESIAN_POINT('Ctrl Pts',(-43.3540581067742,-59.1300583783617,
-51.7228333991501));
#241047=CARTESIAN_POINT('Ctrl Pts',(-42.9657803176365,-58.7757113218568,
-51.6928832016369));
#241048=CARTESIAN_POINT('Ctrl Pts',(-42.8085994167965,-58.5622526766641,
-51.6795966782353));
#241049=CARTESIAN_POINT('Ctrl Pts',(-42.5883241925499,-58.0924754578454,
-51.6521930071375));
#241050=CARTESIAN_POINT('Ctrl Pts',(-42.5251453740978,-57.841687688488,
-51.6375637205917));
#241051=CARTESIAN_POINT('Ctrl Pts',(-42.4963007968343,-57.319933397626,
-51.6071280536247));
#241052=CARTESIAN_POINT('Ctrl Pts',(-42.5348608396013,-57.053713957869,
-51.5915985863055));
#241053=CARTESIAN_POINT('Ctrl Pts',(-42.7103226845749,-56.5623572492977,
-51.5629361116388));
#241054=CARTESIAN_POINT('Ctrl Pts',(-42.8414463899597,-56.340562711555,
-51.5506211829297));
#241055=CARTESIAN_POINT('Ctrl Pts',(-43.1826656768646,-55.955311056523,
-51.5221469096991));
#241056=CARTESIAN_POINT('Ctrl Pts',(-43.3906560935106,-55.7965114929554,
-51.5070079649958));
#241057=CARTESIAN_POINT('Ctrl Pts',(-43.8608842598543,-55.5645393626881,
-51.4764870548346));
#241058=CARTESIAN_POINT('Ctrl Pts',(-44.1196462450192,-55.4956674411495,
-51.4614061140497));
#241059=CARTESIAN_POINT('Ctrl Pts',(-44.6370673296782,-55.4636258727586,
-51.4343324130851));
#241060=CARTESIAN_POINT('Ctrl Pts',(-44.8905011111168,-55.4961043414681,
-51.4212720043211));
#241061=CARTESIAN_POINT('Ctrl Pts',(-45.3803927456486,-55.6567638879207,
-51.3918376825142));
#241062=CARTESIAN_POINT('Ctrl Pts',(-45.6111009889157,-55.7867127862103,
-51.3763925530081));
#241063=CARTESIAN_POINT('Ctrl Pts',(-46.0113485626539,-56.1300641139995,
-51.3461583728924));
#241064=CARTESIAN_POINT('Ctrl Pts',(-46.1761836167742,-56.3408947000873,
-51.3323825370652));
#241065=CARTESIAN_POINT('Ctrl Pts',(-46.4098736954516,-56.8060979471342,
-51.3052456809875));
#241066=CARTESIAN_POINT('Ctrl Pts',(-46.4797503444935,-57.0543686399577,
-51.2907632239061));
#241067=CARTESIAN_POINT('Ctrl Pts',(-46.5231141856447,-57.5736532824897,
-51.2604716197584));
#241068=CARTESIAN_POINT('Ctrl Pts',(-46.4922882589103,-57.8400780776405,
-51.2449301733746));
#241069=CARTESIAN_POINT('Ctrl Pts',(-46.3311223508435,-58.3367881966841,
-51.2159554164305));
#241070=CARTESIAN_POINT('Ctrl Pts',(-46.2057188345087,-58.5633101349482,
-51.203572165685));
#241071=CARTESIAN_POINT('Ctrl Pts',(-45.8748480738052,-58.9581688225288,
-51.1753404757225));
#241072=CARTESIAN_POINT('Ctrl Pts',(-45.6719374286852,-59.1222570032394,
-51.1603039003384));
#241073=CARTESIAN_POINT('Ctrl Pts',(-45.2090908576926,-59.3672011933224,
-51.1297775429632));
#241074=CARTESIAN_POINT('Ctrl Pts',(-44.9523534101276,-59.4434097910955,
-51.1145848916794));
#241075=CARTESIAN_POINT('Ctrl Pts',(-44.6281752479175,-59.4727453981219,
-51.0973523892512));
#241076=CARTESIAN_POINT('Ctrl Pts',(-44.5680326999524,-59.475452478349,
-51.094235142572));
#241077=CARTESIAN_POINT('Ctrl Pts',(-44.507952458321,-59.475452478349,-51.0912000000001));
#241078=CARTESIAN_POINT('Origin',(-44.5079524583206,-57.475452478349,235.35105));
#241079=CARTESIAN_POINT('',(-44.5079524583207,-59.475452478349,-50.3912000000001));
#241080=CARTESIAN_POINT('',(-44.5079524583206,-59.475452478349,-50.5499499999999));
#241081=CARTESIAN_POINT('',(-44.5079524583206,-59.475452478349,235.35105));
#241082=CARTESIAN_POINT('Ctrl Pts',(-44.5079524583206,-59.475452478349,
-50.5499499999999));
#241083=CARTESIAN_POINT('Ctrl Pts',(-44.6213616955837,-59.475452478349,
-50.5556792246953));
#241084=CARTESIAN_POINT('Ctrl Pts',(-44.7348059108359,-59.4658080199635,
-50.5616915131168));
#241085=CARTESIAN_POINT('Ctrl Pts',(-45.1098602422553,-59.4012787529964,
-50.5825206671672));
#241086=CARTESIAN_POINT('Ctrl Pts',(-45.3609414688666,-59.3039716755222,
-50.5980429489653));
#241087=CARTESIAN_POINT('Ctrl Pts',(-45.8015914280971,-59.0221504360446,
-50.6285235552176));
#241088=CARTESIAN_POINT('Ctrl Pts',(-45.9890986230645,-58.8436699323974,
-50.6432017529043));
#241089=CARTESIAN_POINT('Ctrl Pts',(-46.2895030469822,-58.4212871603916,
-50.670697125735));
#241090=CARTESIAN_POINT('Ctrl Pts',(-46.3978739009398,-58.1802572104635,
-50.6838363906266));
#241091=CARTESIAN_POINT('Ctrl Pts',(-46.5159484522013,-57.6685574805219,
-50.7136855415399));
#241092=CARTESIAN_POINT('Ctrl Pts',(-46.5239023467295,-57.4028003281862,
-50.7291880420928));
#241093=CARTESIAN_POINT('Ctrl Pts',(-46.4379981133226,-56.8929624627827,
-50.7589285842414));
#241094=CARTESIAN_POINT('Ctrl Pts',(-46.3486371608918,-56.6531588287568,
-50.7726122482007));
#241095=CARTESIAN_POINT('Ctrl Pts',(-46.0791904496544,-56.209943946477,
-50.7991512979196));
#241096=CARTESIAN_POINT('Ctrl Pts',(-45.8977952569553,-56.0130614435529,
-50.8140574535467));
#241097=CARTESIAN_POINT('Ctrl Pts',(-45.4728237624427,-55.7043709288116,
-50.8445296999843));
#241098=CARTESIAN_POINT('Ctrl Pts',(-45.2344517260874,-55.593984902286,
-50.8597914063684));
#241099=CARTESIAN_POINT('Ctrl Pts',(-44.734698350124,-55.4721600076459,
-50.8885912477494));
#241100=CARTESIAN_POINT('Ctrl Pts',(-44.4786178970573,-55.4595841859626,
-50.9009691025291));
#241101=CARTESIAN_POINT('Ctrl Pts',(-43.9622145966234,-55.5328528041225,
-50.9291938425372));
#241102=CARTESIAN_POINT('Ctrl Pts',(-43.7076659751875,-55.6231478076247,
-50.9446867718779));
#241103=CARTESIAN_POINT('Ctrl Pts',(-43.2579549673169,-55.8931625756044,
-50.9752807701127));
#241104=CARTESIAN_POINT('Ctrl Pts',(-43.0650369926213,-56.0668493158641,
-50.9900924922746));
#241105=CARTESIAN_POINT('Ctrl Pts',(-42.7540585407624,-56.4798060755593,
-51.0178471200605));
#241106=CARTESIAN_POINT('Ctrl Pts',(-42.6397317435719,-56.7157011752985,
-51.0306311739886));
#241107=CARTESIAN_POINT('Ctrl Pts',(-42.5065311368032,-57.2223417564747,
-51.0601852078905));
#241108=CARTESIAN_POINT('Ctrl Pts',(-42.4906348128566,-57.4885480607252,
-51.0757139089717));
#241109=CARTESIAN_POINT('Ctrl Pts',(-42.5618164365921,-58.0019241078571,
-51.1056608450544));
#241110=CARTESIAN_POINT('Ctrl Pts',(-42.644420928482,-58.244813044795,-51.1198293663758));
#241111=CARTESIAN_POINT('Ctrl Pts',(-42.9015287135843,-58.6959472311451,
-51.1461455272462));
#241112=CARTESIAN_POINT('Ctrl Pts',(-43.0772300847524,-58.8978986829694,
-51.1608272355602));
#241113=CARTESIAN_POINT('Ctrl Pts',(-43.4939761355689,-59.218992128493,
-51.1912456999591));
#241114=CARTESIAN_POINT('Ctrl Pts',(-43.7298491568058,-59.3362706282669,
-51.2065821911959));
#241115=CARTESIAN_POINT('Ctrl Pts',(-44.1534726225493,-59.4518347281563,
-51.2313534839495));
#241116=CARTESIAN_POINT('Ctrl Pts',(-44.3304689495412,-59.475452478349,
-51.2409838617374));
#241117=CARTESIAN_POINT('Ctrl Pts',(-44.5079524583209,-59.475452478349,
-51.2499499999999));
#241118=CARTESIAN_POINT('Ctrl Pts',(-44.507952458321,-59.475452478349,-51.0912000000001));
#241119=CARTESIAN_POINT('Ctrl Pts',(-44.3155292379269,-59.475452478349,
-51.081479135167));
#241120=CARTESIAN_POINT('Ctrl Pts',(-44.1238270035994,-59.4476910747681,
-51.0709849856108));
#241121=CARTESIAN_POINT('Ctrl Pts',(-43.6880346010131,-59.3183107915699,
-51.0451959686849));
#241122=CARTESIAN_POINT('Ctrl Pts',(-43.4543534409762,-59.19542761922,-51.029806736601));
#241123=CARTESIAN_POINT('Ctrl Pts',(-43.0427356756326,-58.8628243208416,
-50.9993116396479));
#241124=CARTESIAN_POINT('Ctrl Pts',(-42.8704701156885,-58.6545334333459,
-50.9849797223751));
#241125=CARTESIAN_POINT('Ctrl Pts',(-42.6240633703296,-58.1937648214756,
-50.9581015533493));
#241126=CARTESIAN_POINT('Ctrl Pts',(-42.5479439098418,-57.9480333564835,
-50.9437672178914));
#241127=CARTESIAN_POINT('Ctrl Pts',(-42.4909739825197,-57.4314427985909,
-50.913632768681));
#241128=CARTESIAN_POINT('Ctrl Pts',(-42.5145162301838,-57.1650230507651,
-50.8980916167245));
#241129=CARTESIAN_POINT('Ctrl Pts',(-42.6621071878323,-56.6634005101717,
-50.8688303018565));
#241130=CARTESIAN_POINT('Ctrl Pts',(-42.78211869464,-56.4323497013107,-50.8562954287898));
#241131=CARTESIAN_POINT('Ctrl Pts',(-43.1032765292122,-56.0285935944511,
-50.8282949098101));
#241132=CARTESIAN_POINT('Ctrl Pts',(-43.3013418874345,-55.8597244716109,
-50.8133636652038));
#241133=CARTESIAN_POINT('Ctrl Pts',(-43.7569953943809,-55.6029168978137,
-50.7828546727482));
#241134=CARTESIAN_POINT('Ctrl Pts',(-44.0116561683845,-55.5199341998579,
-50.7675693532458));
#241135=CARTESIAN_POINT('Ctrl Pts',(-44.5270170631809,-55.45952453514,-50.7397723264492));
#241136=CARTESIAN_POINT('Ctrl Pts',(-44.7822186864924,-55.4781735824444,
-50.7272652124056));
#241137=CARTESIAN_POINT('Ctrl Pts',(-45.2790829766877,-55.6117474079419,
-50.6982686451386));
#241138=CARTESIAN_POINT('Ctrl Pts',(-45.5153068061894,-55.7280930343386,
-50.6829416405246));
#241139=CARTESIAN_POINT('Ctrl Pts',(-45.9331993908207,-56.0475213946705,
-50.6525138203448));
#241140=CARTESIAN_POINT('Ctrl Pts',(-46.1096674151591,-56.2487886211153,
-50.6377553916718));
#241141=CARTESIAN_POINT('Ctrl Pts',(-46.3684553054871,-56.6988281977221,
-50.6115030830364));
#241142=CARTESIAN_POINT('Ctrl Pts',(-46.4519805126622,-56.9412961747351,
-50.5973591177107));
#241143=CARTESIAN_POINT('Ctrl Pts',(-46.5251864516007,-57.4541805161915,
-50.5674408644591));
#241144=CARTESIAN_POINT('Ctrl Pts',(-46.5103824320334,-57.7203388394583,
-50.5519149622686));
#241145=CARTESIAN_POINT('Ctrl Pts',(-46.3792507450676,-58.2276845613751,
-50.5223197951568));
#241146=CARTESIAN_POINT('Ctrl Pts',(-46.2657394275693,-58.4642795373728,
-50.5094926873508));
#241147=CARTESIAN_POINT('Ctrl Pts',(-45.9562147847162,-58.8785401443913,
-50.481773474424));
#241148=CARTESIAN_POINT('Ctrl Pts',(-45.7640371376476,-59.0528987269253,
-50.4669795568434));
#241149=CARTESIAN_POINT('Ctrl Pts',(-45.3155596585774,-59.3245613274818,
-50.4363998124163));
#241150=CARTESIAN_POINT('Ctrl Pts',(-45.0614789223731,-59.4158320621292,
-50.4209020609462));
#241151=CARTESIAN_POINT('Ctrl Pts',(-44.7010492059048,-59.4684672724759,
-50.4011586253512));
#241152=CARTESIAN_POINT('Ctrl Pts',(-44.6044663788676,-59.475452478349,
-50.3960757045758));
#241153=CARTESIAN_POINT('Ctrl Pts',(-44.5079524583207,-59.475452478349,
-50.3912000000001));
#241154=CARTESIAN_POINT('Origin',(-44.5079524583206,-57.475452478349,235.35105));
#241155=CARTESIAN_POINT('',(-44.5079524583206,-59.475452478349,-49.6912000000001));
#241156=CARTESIAN_POINT('',(-44.5079524583206,-59.475452478349,-49.8499499999999));
#241157=CARTESIAN_POINT('',(-44.5079524583206,-59.475452478349,235.35105));
#241158=CARTESIAN_POINT('Ctrl Pts',(-44.5079524583205,-59.475452478349,
-49.8499499999999));
#241159=CARTESIAN_POINT('Ctrl Pts',(-44.6599129559212,-59.475452478349,
-49.857626762992));
#241160=CARTESIAN_POINT('Ctrl Pts',(-44.8116920785691,-59.4581383328145,
-49.8657993591687));
#241161=CARTESIAN_POINT('Ctrl Pts',(-45.21861949929,-59.363635675348,-49.8891129065688));
#241162=CARTESIAN_POINT('Ctrl Pts',(-45.4623574287261,-59.2529162806659,
-49.9046554111746));
#241163=CARTESIAN_POINT('Ctrl Pts',(-45.8843456253122,-58.9487546700144,
-49.9348448538885));
#241164=CARTESIAN_POINT('Ctrl Pts',(-46.0608908843471,-58.7613386430007,
-49.9492298942989));
#241165=CARTESIAN_POINT('Ctrl Pts',(-46.3401602182985,-58.3205090227498,
-49.9761955945888));
#241166=CARTESIAN_POINT('Ctrl Pts',(-46.4364144565539,-58.0689257646349,
-49.9903307249666));
#241167=CARTESIAN_POINT('Ctrl Pts',(-46.5237169735492,-57.5476386510155,
-50.0207391399278));
#241168=CARTESIAN_POINT('Ctrl Pts',(-46.515853770386,-57.2834764456064,
-50.03614860191));
#241169=CARTESIAN_POINT('Ctrl Pts',(-46.40070405108,-56.7814383793904,-50.0654341557726));
#241170=CARTESIAN_POINT('Ctrl Pts',(-46.2977086690653,-56.547603329606,
-50.078263763375));
#241171=CARTESIAN_POINT('Ctrl Pts',(-46.0031560806814,-56.1209382868014,
-50.1055884118738));
#241172=CARTESIAN_POINT('Ctrl Pts',(-45.810579985855,-55.9348478385497,
-50.1207446377143));
#241173=CARTESIAN_POINT('Ctrl Pts',(-45.3695407548981,-55.6520995124664,
-50.1512719492794));
#241174=CARTESIAN_POINT('Ctrl Pts',(-45.1266492563282,-55.5560284728997,
-50.166344450074));
#241175=CARTESIAN_POINT('Ctrl Pts',(-44.6203120790311,-55.4622484213822,
-50.1946589183177));
#241176=CARTESIAN_POINT('Ctrl Pts',(-44.3618630975721,-55.4644143364923,
-50.2070082182243));
#241177=CARTESIAN_POINT('Ctrl Pts',(-43.8502430762259,-55.568072356457,
-50.2358776733816));
#241178=CARTESIAN_POINT('Ctrl Pts',(-43.6028239071385,-55.6722883382533,
-50.251416464523));
#241179=CARTESIAN_POINT('Ctrl Pts',(-43.1715612934929,-55.9656586820565,
-50.2817596883325));
#241180=CARTESIAN_POINT('Ctrl Pts',(-42.9895969155478,-56.1487817190571,
-50.2962932803883));
#241181=CARTESIAN_POINT('Ctrl Pts',(-42.6999187108287,-56.580591609061,
-50.3235217420922));
#241182=CARTESIAN_POINT('Ctrl Pts',(-42.5976571949136,-56.826931644352,
-50.3371196180167));
#241183=CARTESIAN_POINT('Ctrl Pts',(-42.4951107390491,-57.3435893973861,
-50.3672579869436));
#241184=CARTESIAN_POINT('Ctrl Pts',(-42.4951988047948,-57.608653251943,
-50.3827200451261));
#241185=CARTESIAN_POINT('Ctrl Pts',(-42.5959679797622,-58.1145953544506,
-50.412233334439));
#241186=CARTESIAN_POINT('Ctrl Pts',(-42.6922005031069,-58.3513402222056,
-50.425434965518));
#241187=CARTESIAN_POINT('Ctrl Pts',(-42.9743204684951,-58.7862905290305,
-50.4523731944552));
#241188=CARTESIAN_POINT('Ctrl Pts',(-43.1614209398734,-58.9778274350877,
-50.4674116569562));
#241189=CARTESIAN_POINT('Ctrl Pts',(-43.5946719927533,-59.2735746790815,
-50.49792465929));
#241190=CARTESIAN_POINT('Ctrl Pts',(-43.8354224305791,-59.3767803006319,
-50.5130970896344));
#241191=CARTESIAN_POINT('Ctrl Pts',(-44.227140195886,-59.4606605256588,
-50.5353324524567));
#241192=CARTESIAN_POINT('Ctrl Pts',(-44.3674974673574,-59.475452478349,
-50.5428544739012));
#241193=CARTESIAN_POINT('Ctrl Pts',(-44.5079524583206,-59.475452478349,
-50.5499499999999));
#241194=CARTESIAN_POINT('Ctrl Pts',(-44.5079524583207,-59.475452478349,
-50.3912000000001));
#241195=CARTESIAN_POINT('Ctrl Pts',(-44.3513025812242,-59.475452478349,
-50.383286338238));
#241196=CARTESIAN_POINT('Ctrl Pts',(-44.1948889936747,-59.4570535088991,
-50.3748479767774));
#241197=CARTESIAN_POINT('Ctrl Pts',(-43.788923747471,-59.3597737085898,
-50.3515020366529));
#241198=CARTESIAN_POINT('Ctrl Pts',(-43.5502083419417,-59.250383299058,
-50.3362520227229));
#241199=CARTESIAN_POINT('Ctrl Pts',(-43.1240620521067,-58.9434789960096,
-50.3057725256417));
#241200=CARTESIAN_POINT('Ctrl Pts',(-42.9418640111444,-58.7473294489174,
-50.2908471894852));
#241201=CARTESIAN_POINT('Ctrl Pts',(-42.6706496560568,-58.3052567302801,
-50.264252154778));
#241202=CARTESIAN_POINT('Ctrl Pts',(-42.5803309933147,-58.0658855487501,
-50.250641929107));
#241203=CARTESIAN_POINT('Ctrl Pts',(-42.4923404721843,-57.5565856752963,
-50.2209327698221));
#241204=CARTESIAN_POINT('Ctrl Pts',(-42.4991659477739,-57.2909112651402,
-50.2054350958963));
#241205=CARTESIAN_POINT('Ctrl Pts',(-42.6150752109583,-56.7785057137568,
-50.1755447720656));
#241206=CARTESIAN_POINT('Ctrl Pts',(-42.7225942132042,-56.5367374890622,
-50.162347139195));
#241207=CARTESIAN_POINT('Ctrl Pts',(-43.0214952362546,-56.1130252706333,
-50.134888939872));
#241208=CARTESIAN_POINT('Ctrl Pts',(-43.2082285435438,-55.9338806860874,
-50.1202304685317));
#241209=CARTESIAN_POINT('Ctrl Pts',(-43.6475740771907,-55.6504146457762,
-50.0897677860873));
#241210=CARTESIAN_POINT('Ctrl Pts',(-43.8981505276236,-55.5521267023332,
-50.0742423960563));
#241211=CARTESIAN_POINT('Ctrl Pts',(-44.4119099094751,-55.4615313574422,
-50.0456458590569));
#241212=CARTESIAN_POINT('Ctrl Pts',(-44.6693028709624,-55.4657084686857,
-50.0333330761666));
#241213=CARTESIAN_POINT('Ctrl Pts',(-45.172880169066,-55.5714664870943,
-50.0048086745423));
#241214=CARTESIAN_POINT('Ctrl Pts',(-45.4139467989259,-55.6736629018997,
-49.9896497059584));
#241215=CARTESIAN_POINT('Ctrl Pts',(-45.84832585836,-55.967579699605,-49.9591331068387));
#241216=CARTESIAN_POINT('Ctrl Pts',(-46.036212499502,-56.1583542910206,
-49.9440771626739));
#241217=CARTESIAN_POINT('Ctrl Pts',(-46.320100302134,-56.5921374674081,
-49.9170836671766));
#241218=CARTESIAN_POINT('Ctrl Pts',(-46.417292771059,-56.8284632261593,
-49.903941039711));
#241219=CARTESIAN_POINT('Ctrl Pts',(-46.5201186902985,-57.3338550090348,
-49.8744598523766));
#241220=CARTESIAN_POINT('Ctrl Pts',(-46.521319403242,-57.5988038392898,
-49.859004503945));
#241221=CARTESIAN_POINT('Ctrl Pts',(-46.4209398179983,-58.1161341573481,
-49.8288269020583));
#241222=CARTESIAN_POINT('Ctrl Pts',(-46.3195313044318,-58.363217860143,
-49.8151577856296));
#241223=CARTESIAN_POINT('Ctrl Pts',(-46.0313398527511,-58.7963238182018,
-49.7879666299516));
#241224=CARTESIAN_POINT('Ctrl Pts',(-45.850147359489,-58.9800728327082,
-49.7734537744037));
#241225=CARTESIAN_POINT('Ctrl Pts',(-45.4202000744181,-59.2750097298543,
-49.7431313074193));
#241226=CARTESIAN_POINT('Ctrl Pts',(-45.1732993036512,-59.3801668480655,
-49.7275912549891));
#241227=CARTESIAN_POINT('Ctrl Pts',(-44.7794705425607,-59.4616264148727,
-49.7053198510996));
#241228=CARTESIAN_POINT('Ctrl Pts',(-44.6437432571755,-59.475452478349,
-49.6980598997489));
#241229=CARTESIAN_POINT('Ctrl Pts',(-44.5079524583206,-59.475452478349,
-49.6912000000001));
#241230=CARTESIAN_POINT('Origin',(-44.5079524583206,-57.475452478349,235.35105));
#241231=CARTESIAN_POINT('',(-44.5079524583205,-59.475452478349,-48.9912000000001));
#241232=CARTESIAN_POINT('',(-44.5079524583204,-59.475452478349,-49.1499499999999));
#241233=CARTESIAN_POINT('',(-44.5079524583206,-59.475452478349,235.35105));
#241234=CARTESIAN_POINT('Ctrl Pts',(-44.5079524583202,-59.475452478349,
-49.1499499999999));
#241235=CARTESIAN_POINT('Ctrl Pts',(-44.7019516755273,-59.475452478349,
-49.1597504812741));
#241236=CARTESIAN_POINT('Ctrl Pts',(-44.8952411044441,-59.4472344414536,
-49.1703381314341));
#241237=CARTESIAN_POINT('Ctrl Pts',(-45.3341697230981,-59.3157735812064,
-49.1963462676865));
#241238=CARTESIAN_POINT('Ctrl Pts',(-45.5691499075924,-59.1910487434321,
-49.2118548393225));
#241239=CARTESIAN_POINT('Ctrl Pts',(-45.9697612694271,-58.8638105260088,
-49.2416374316203));
#241240=CARTESIAN_POINT('Ctrl Pts',(-46.1339073546182,-58.667343055432,
-49.2554230496701));
#241241=CARTESIAN_POINT('Ctrl Pts',(-46.3855343432818,-58.213681630364,
-49.2818866327991));
#241242=CARTESIAN_POINT('Ctrl Pts',(-46.4667320066789,-57.9585961298683,
-49.296766620328));
#241243=CARTESIAN_POINT('Ctrl Pts',(-46.5244476178428,-57.4363955805834,
-49.3272283190364));
#241244=CARTESIAN_POINT('Ctrl Pts',(-46.5022497916875,-57.1745033260573,
-49.3425053672171));
#241245=CARTESIAN_POINT('Ctrl Pts',(-46.3604735179476,-56.6800310354043,
-49.3713495841718));
#241246=CARTESIAN_POINT('Ctrl Pts',(-46.2446066891854,-56.4514645244218,
-49.3837504255677));
#241247=CARTESIAN_POINT('Ctrl Pts',(-45.925185283618,-56.0391191431053,
-49.4119137438739));
#241248=CARTESIAN_POINT('Ctrl Pts',(-45.7205380520192,-55.8626272248705,
-49.4273998240695));
#241249=CARTESIAN_POINT('Ctrl Pts',(-45.2629408143957,-55.6056411808176,
-49.4580122155826));
#241250=CARTESIAN_POINT('Ctrl Pts',(-45.0163543710696,-55.5241038847157,
-49.4728474772943));
#241251=CARTESIAN_POINT('Ctrl Pts',(-44.503775747153,-55.4587082044725,
-49.50064937437));
#241252=CARTESIAN_POINT('Ctrl Pts',(-44.2425846895981,-55.4762355767426,
-49.5133787287316));
#241253=CARTESIAN_POINT('Ctrl Pts',(-43.7366604177638,-55.6113340358778,
-49.542877457978));
#241254=CARTESIAN_POINT('Ctrl Pts',(-43.4973904340246,-55.7294335646316,
-49.5584095041497));
#241255=CARTESIAN_POINT('Ctrl Pts',(-43.086470406459,-56.0457416171329,
-49.5883940746774));
#241256=CARTESIAN_POINT('Ctrl Pts',(-42.916324862786,-56.2379335754247,
-49.602595111312));
#241257=CARTESIAN_POINT('Ctrl Pts',(-42.6517993134929,-56.6849379663124,
-49.628996080375));
#241258=CARTESIAN_POINT('Ctrl Pts',(-42.5634518622002,-56.937639760177,
-49.6435775914398));
#241259=CARTESIAN_POINT('Ctrl Pts',(-42.4910559618037,-57.4588734433419,
-49.6739828896244));
#241260=CARTESIAN_POINT('Ctrl Pts',(-42.5061103059526,-57.7219964938289,
-49.6893317342361));
#241261=CARTESIAN_POINT('Ctrl Pts',(-42.6345915085431,-58.2203002441122,
-49.7183994530026));
#241262=CARTESIAN_POINT('Ctrl Pts',(-42.7439706046001,-58.4514791784199,
-49.7309710147522));
#241263=CARTESIAN_POINT('Ctrl Pts',(-43.0501967270924,-58.8701946608091,
-49.7586535264024));
#241264=CARTESIAN_POINT('Ctrl Pts',(-43.2477956880408,-59.0509921616579,
-49.7739091205071));
#241265=CARTESIAN_POINT('Ctrl Pts',(-43.6958317872822,-59.3212746258446,
-49.804426313265));
#241266=CARTESIAN_POINT('Ctrl Pts',(-43.9405552984306,-59.4105720159264,
-49.8193937991665));
#241267=CARTESIAN_POINT('Ctrl Pts',(-44.2990888000906,-59.4672790910993,
-49.8391602042242));
#241268=CARTESIAN_POINT('Ctrl Pts',(-44.4035512640085,-59.475452478349,
-49.8446758449564));
#241269=CARTESIAN_POINT('Ctrl Pts',(-44.5079524583205,-59.475452478349,
-49.8499499999999));
#241270=CARTESIAN_POINT('Ctrl Pts',(-44.5079524583206,-59.475452478349,
-49.6912000000001));
#241271=CARTESIAN_POINT('Ctrl Pts',(-44.3885780724371,-59.475452478349,
-49.6851694270405));
#241272=CARTESIAN_POINT('Ctrl Pts',(-44.269186440873,-59.4647669035076,
-49.6788263202615));
#241273=CARTESIAN_POINT('Ctrl Pts',(-43.8966411141707,-59.397228324263,
-49.6580361448761));
#241274=CARTESIAN_POINT('Ctrl Pts',(-43.6534734865964,-59.3021339659884,
-49.6429781810931));
#241275=CARTESIAN_POINT('Ctrl Pts',(-43.2114016638356,-59.0211756506772,
-49.6124509135494));
#241276=CARTESIAN_POINT('Ctrl Pts',(-43.0180908202016,-58.8358411034676,
-49.5972796166733));
#241277=CARTESIAN_POINT('Ctrl Pts',(-42.7218475977894,-58.4103169154255,
-49.5699028354042));
#241278=CARTESIAN_POINT('Ctrl Pts',(-42.6179300357161,-58.1768709471206,
-49.5571160773453));
#241279=CARTESIAN_POINT('Ctrl Pts',(-42.5008395774885,-57.6753697000545,
-49.527861837933));
#241280=CARTESIAN_POINT('Ctrl Pts',(-42.4919282202469,-57.4113466039644,
-49.5124604906611));
#241281=CARTESIAN_POINT('Ctrl Pts',(-42.5771568260949,-56.889448221801,
-49.4820164183682));
#241282=CARTESIAN_POINT('Ctrl Pts',(-42.6725922982354,-56.6371497732339,
-49.467801834985));
#241283=CARTESIAN_POINT('Ctrl Pts',(-42.9504544477179,-56.1951104579857,
-49.4408719402785));
#241284=CARTESIAN_POINT('Ctrl Pts',(-43.1262646751023,-56.0071300685192,
-49.4265075717347));
#241285=CARTESIAN_POINT('Ctrl Pts',(-43.5469878758011,-55.7015412112566,
-49.3963404062447));
#241286=CARTESIAN_POINT('Ctrl Pts',(-43.7902191393219,-55.5899580215752,
-49.3807983034421));
#241287=CARTESIAN_POINT('Ctrl Pts',(-44.2989467591262,-55.4697764255278,
-49.3515930294198));
#241288=CARTESIAN_POINT('Ctrl Pts',(-44.5588010092762,-55.4595586946896,
-49.339094794039));
#241289=CARTESIAN_POINT('Ctrl Pts',(-45.0684884434839,-55.5383462550722,
-49.3110483580103));
#241290=CARTESIAN_POINT('Ctrl Pts',(-45.3134418880181,-55.6267395221787,
-49.2960956265532));
#241291=CARTESIAN_POINT('Ctrl Pts',(-45.7623829581058,-55.895349048267,
-49.2655815103716));
#241292=CARTESIAN_POINT('Ctrl Pts',(-45.9606395150753,-56.0754311885403,
-49.2503135604168));
#241293=CARTESIAN_POINT('Ctrl Pts',(-46.2684150070898,-56.4930786251726,
-49.2225839288215));
#241294=CARTESIAN_POINT('Ctrl Pts',(-46.3786445516313,-56.7239102050038,
-49.210039965945));
#241295=CARTESIAN_POINT('Ctrl Pts',(-46.5088833214484,-57.2217135426928,
-49.1810014379132));
#241296=CARTESIAN_POINT('Ctrl Pts',(-46.5248838699055,-57.484685009209,
-49.1656614356997));
#241297=CARTESIAN_POINT('Ctrl Pts',(-46.4544244517634,-58.0060822547599,
-49.135246596376));
#241298=CARTESIAN_POINT('Ctrl Pts',(-46.3670135365742,-58.259097962154,
-49.1205933304447));
#241299=CARTESIAN_POINT('Ctrl Pts',(-46.1042025134809,-58.706983944617,
-49.0942532629833));
#241300=CARTESIAN_POINT('Ctrl Pts',(-45.9348472313648,-58.8997445162226,
-49.0800755643444));
#241301=CARTESIAN_POINT('Ctrl Pts',(-45.5253022608469,-59.2175094848837,
-49.050117965765));
#241302=CARTESIAN_POINT('Ctrl Pts',(-45.2865926692342,-59.3364987682916,
-49.0345882783886));
#241303=CARTESIAN_POINT('Ctrl Pts',(-44.8605785192526,-59.452085760637,
-49.0096955449969));
#241304=CARTESIAN_POINT('Ctrl Pts',(-44.6844897702049,-59.475452478349,
-49.0001183381472));
#241305=CARTESIAN_POINT('Ctrl Pts',(-44.5079524583203,-59.475452478349,
-48.9912000000001));
#241306=CARTESIAN_POINT('Origin',(-44.5079524583206,-57.475452478349,235.35105));
#241307=CARTESIAN_POINT('',(-44.5079524583205,-59.475452478349,-48.2912000000001));
#241308=CARTESIAN_POINT('',(-44.5079524583205,-59.475452478349,-48.4499499999999));
#241309=CARTESIAN_POINT('',(-44.5079524583206,-59.475452478349,235.35105));
#241310=CARTESIAN_POINT('Ctrl Pts',(-44.5079524583205,-59.475452478349,
-48.4499499999999));
#241311=CARTESIAN_POINT('Ctrl Pts',(-44.7430370280651,-59.475452478349,
-48.461826037217));
#241312=CARTESIAN_POINT('Ctrl Pts',(-44.9765380902944,-59.434011449719,
-48.4748307752346));
#241313=CARTESIAN_POINT('Ctrl Pts',(-45.4435506997623,-59.262418474562,
-48.5034281827251));
#241314=CARTESIAN_POINT('Ctrl Pts',(-45.6692665229574,-59.1246781509403,
-48.518848354318));
#241315=CARTESIAN_POINT('Ctrl Pts',(-46.0484296267242,-58.7758705731551,
-48.5481765266724));
#241316=CARTESIAN_POINT('Ctrl Pts',(-46.2005301026568,-58.5705789077536,
-48.5610676249514));
#241317=CARTESIAN_POINT('Ctrl Pts',(-46.4252545442384,-58.1033792102185,
-48.588320940641));
#241318=CARTESIAN_POINT('Ctrl Pts',(-46.4915176197873,-57.8439172034373,
-48.6034562243699));
#241319=CARTESIAN_POINT('Ctrl Pts',(-46.5186841281559,-57.3206040777301,
-48.6339828233695));
#241320=CARTESIAN_POINT('Ctrl Pts',(-46.4817823289692,-57.0618844316932,
-48.6490748027217));
#241321=CARTESIAN_POINT('Ctrl Pts',(-46.3123784502638,-56.5757072795242,
-48.6774351365982));
#241322=CARTESIAN_POINT('Ctrl Pts',(-46.1825930825342,-56.3524770495347,
-48.6897703728452));
#241323=CARTESIAN_POINT('Ctrl Pts',(-45.83923971478,-55.9593941285552,-48.7185808678125));
#241324=CARTESIAN_POINT('Ctrl Pts',(-45.6260387883208,-55.7959827045881,
-48.7341175504196));
#241325=CARTESIAN_POINT('Ctrl Pts',(-45.1573046245358,-55.5665713247126,
-48.7644882977844));
#241326=CARTESIAN_POINT('Ctrl Pts',(-44.9079518312746,-55.4992122245449,
-48.7790497796583));
#241327=CARTESIAN_POINT('Ctrl Pts',(-44.3896726195646,-55.4616184041298,
-48.8063287722967));
#241328=CARTESIAN_POINT('Ctrl Pts',(-44.1254992307615,-55.4947231661162,
-48.8198328906914));
#241329=CARTESIAN_POINT('Ctrl Pts',(-43.6261149392988,-55.6612417325591,
-48.8499176520344));
#241330=CARTESIAN_POINT('Ctrl Pts',(-43.3957223068424,-55.7926152285137,
-48.8653883882319));
#241331=CARTESIAN_POINT('Ctrl Pts',(-43.0059075585446,-56.1308069479149,
-48.8949450327441));
#241332=CARTESIAN_POINT('Ctrl Pts',(-42.8478521658473,-56.3316785550261,
-48.9082298544728));
#241333=CARTESIAN_POINT('Ctrl Pts',(-42.6096712164602,-56.7921899013986,
-48.9350930163445));
#241334=CARTESIAN_POINT('Ctrl Pts',(-42.5359218161572,-57.0495793664238,
-48.9501074018042));
#241335=CARTESIAN_POINT('Ctrl Pts',(-42.4935129329832,-57.5725617747053,
-48.9806147089539));
#241336=CARTESIAN_POINT('Ctrl Pts',(-42.5231101205008,-57.8329665762101,
-48.9958049890417));
#241337=CARTESIAN_POINT('Ctrl Pts',(-42.6787365533554,-58.3233357959971,
-49.0244098601959));
#241338=CARTESIAN_POINT('Ctrl Pts',(-42.8015034319804,-58.5492143585533,
-49.0367280760931));
#241339=CARTESIAN_POINT('Ctrl Pts',(-43.1328738911161,-58.9520496191419,
-49.0652176599413));
#241340=CARTESIAN_POINT('Ctrl Pts',(-43.3418723851366,-59.1220882452236,
-49.0807353368372));
#241341=CARTESIAN_POINT('Ctrl Pts',(-43.8052062623671,-59.365424015634,
-49.1112393997809));
#241342=CARTESIAN_POINT('Ctrl Pts',(-44.0532680775006,-59.4399225452165,
-49.1259438971879));
#241343=CARTESIAN_POINT('Ctrl Pts',(-44.3750039639929,-59.4721422398772,
-49.1431371395912));
#241344=CARTESIAN_POINT('Ctrl Pts',(-44.4415149442898,-59.475452478349,
-49.1465936997965));
#241345=CARTESIAN_POINT('Ctrl Pts',(-44.5079524583202,-59.475452478349,
-49.1499499999999));
#241346=CARTESIAN_POINT('Ctrl Pts',(-44.5079524583203,-59.475452478349,
-48.9912000000001));
#241347=CARTESIAN_POINT('Ctrl Pts',(-44.4259098953645,-59.475452478349,
-48.987055361617));
#241348=CARTESIAN_POINT('Ctrl Pts',(-44.3437854394165,-59.4704047613634,
-48.9827593610728));
#241349=CARTESIAN_POINT('Ctrl Pts',(-44.0067217856789,-59.4286432605234,
-48.9645134855666));
#241350=CARTESIAN_POINT('Ctrl Pts',(-43.7599263287128,-59.3480471172143,
-48.9496951151626));
#241351=CARTESIAN_POINT('Ctrl Pts',(-43.3015381377503,-59.09288174759,-48.9190958691554));
#241352=CARTESIAN_POINT('Ctrl Pts',(-43.0962970319428,-58.9172480387275,
-48.903604818641));
#241353=CARTESIAN_POINT('Ctrl Pts',(-42.7752695593589,-58.5061689076375,
-48.875397297101));
#241354=CARTESIAN_POINT('Ctrl Pts',(-42.6584805553404,-58.277966884615,
-48.8630133403658));
#241355=CARTESIAN_POINT('Ctrl Pts',(-42.5148357827412,-57.7840415274964,
-48.8342010278671));
#241356=CARTESIAN_POINT('Ctrl Pts',(-42.491636918027,-57.5223377588128,
-48.8189349746939));
#241357=CARTESIAN_POINT('Ctrl Pts',(-42.5472895037159,-57.0000055215278,
-48.7884655941856));
#241358=CARTESIAN_POINT('Ctrl Pts',(-42.6274873819553,-56.7445964917713,
-48.7735667341164));
#241359=CARTESIAN_POINT('Ctrl Pts',(-42.8773051311541,-56.2900038195635,
-48.7470488282376));
#241360=CARTESIAN_POINT('Ctrl Pts',(-43.0406230148019,-56.0929441708537,
-48.7333369411703));
#241361=CARTESIAN_POINT('Ctrl Pts',(-43.4397728318041,-55.7642112632147,
-48.7035845882801));
#241362=CARTESIAN_POINT('Ctrl Pts',(-43.6741413291616,-55.6385750584568,
-48.6880803364087));
#241363=CARTESIAN_POINT('Ctrl Pts',(-44.1765003305804,-55.4858217928749,
-48.658246786168));
#241364=CARTESIAN_POINT('Ctrl Pts',(-44.4393434915333,-55.4595761570491,
-48.6451290573474));
#241365=CARTESIAN_POINT('Ctrl Pts',(-44.9551883989394,-55.5092856781278,
-48.6176196666527));
#241366=CARTESIAN_POINT('Ctrl Pts',(-45.203438467538,-55.5828102316503,
-48.6029340666643));
#241367=CARTESIAN_POINT('Ctrl Pts',(-45.6675337712541,-55.824251070524,
-48.5724468067007));
#241368=CARTESIAN_POINT('Ctrl Pts',(-45.8771180295607,-55.9933904222787,
-48.5569257669122));
#241369=CARTESIAN_POINT('Ctrl Pts',(-46.2101309659608,-56.3949019520463,
-48.5283918169692));
#241370=CARTESIAN_POINT('Ctrl Pts',(-46.3338537554103,-56.6204150673259,
-48.5160771823096));
#241371=CARTESIAN_POINT('Ctrl Pts',(-46.4913750186542,-57.1102141906313,
-48.4875055667834));
#241372=CARTESIAN_POINT('Ctrl Pts',(-46.5219804278959,-57.3703993207582,
-48.4723281008594));
#241373=CARTESIAN_POINT('Ctrl Pts',(-46.4816675517556,-57.8934536961542,
-48.441816595628));
#241374=CARTESIAN_POINT('Ctrl Pts',(-46.40894351168,-58.1511412894893,-48.4267848193501));
#241375=CARTESIAN_POINT('Ctrl Pts',(-46.1726084551324,-58.6125800873386,
-48.3998675561423));
#241376=CARTESIAN_POINT('Ctrl Pts',(-46.0153779364691,-58.8140570978205,
-48.3866430428381));
#241377=CARTESIAN_POINT('Ctrl Pts',(-45.6270334709081,-59.1537251060519,
-48.3571176158634));
#241378=CARTESIAN_POINT('Ctrl Pts',(-45.3972776717518,-59.2859889199384,
-48.3416530836987));
#241379=CARTESIAN_POINT('Ctrl Pts',(-44.9418533362197,-59.4399713428427,
-48.3141547354598));
#241380=CARTESIAN_POINT('Ctrl Pts',(-44.7254848228503,-59.475452478349,
-48.3021893323067));
#241381=CARTESIAN_POINT('Ctrl Pts',(-44.5079524583203,-59.475452478349,
-48.2912000000001));
#241382=CARTESIAN_POINT('Origin',(-44.5079524583206,-57.475452478349,235.35105));
#241383=CARTESIAN_POINT('',(-44.5079524583206,-59.475452478349,-47.5912000000001));
#241384=CARTESIAN_POINT('',(-44.5079524583206,-59.475452478349,-47.7499499999999));
#241385=CARTESIAN_POINT('',(-44.5079524583206,-59.475452478349,235.35105));
#241386=CARTESIAN_POINT('Ctrl Pts',(-44.5079524583206,-59.475452478349,
-47.7499499999999));
#241387=CARTESIAN_POINT('Ctrl Pts',(-44.5157926193897,-59.475452478349,
-47.7503460704215));
#241388=CARTESIAN_POINT('Ctrl Pts',(-44.5236346243393,-59.475406377275,
-47.7507435786071));
#241389=CARTESIAN_POINT('Ctrl Pts',(-44.7965847178638,-59.4721954961175,
-47.7646261626801));
#241390=CARTESIAN_POINT('Ctrl Pts',(-45.0583911087667,-59.4163947421566,
-47.7794796588187));
#241391=CARTESIAN_POINT('Ctrl Pts',(-45.5407450561074,-59.2078465043819,
-47.8099299441212));
#241392=CARTESIAN_POINT('Ctrl Pts',(-45.7573651276197,-59.0587499264138,
-47.8252218392644));
#241393=CARTESIAN_POINT('Ctrl Pts',(-46.1166477375133,-58.6905943186293,
-47.8541100034177));
#241394=CARTESIAN_POINT('Ctrl Pts',(-46.2577322577609,-58.4768160833543,
-47.8665371230414));
#241395=CARTESIAN_POINT('Ctrl Pts',(-46.4577427899821,-57.9950663769071,
-47.8946391892509));
#241396=CARTESIAN_POINT('Ctrl Pts',(-46.5097010685008,-57.7297147229521,
-47.9101180357316));
#241397=CARTESIAN_POINT('Ctrl Pts',(-46.506182691861,-57.2046317958789,
-47.9407478731442));
#241398=CARTESIAN_POINT('Ctrl Pts',(-46.4547739127248,-56.9499188909053,
-47.9556061259344));
#241399=CARTESIAN_POINT('Ctrl Pts',(-46.2575857249768,-56.4725146387524,
-47.98345470731));
#241400=CARTESIAN_POINT('Ctrl Pts',(-46.1131472434065,-56.2546075239529,
-47.9961331758922));
#241401=CARTESIAN_POINT('Ctrl Pts',(-45.7453691322896,-55.8821210794356,
-48.0255768331097));
#241402=CARTESIAN_POINT('Ctrl Pts',(-45.5241381173083,-55.7326789994757,
-48.0411117417214));
#241403=CARTESIAN_POINT('Ctrl Pts',(-45.0455500066651,-55.5323263409505,
-48.0711327461981));
#241404=CARTESIAN_POINT('Ctrl Pts',(-44.7941741147582,-55.4797385821954,
-48.0853656004787));
#241405=CARTESIAN_POINT('Ctrl Pts',(-44.2746766753311,-55.4715031245149,
-48.1118498501461));
#241406=CARTESIAN_POINT('Ctrl Pts',(-44.0113919228789,-55.5200091917417,
-48.1263348897029));
#241407=CARTESIAN_POINT('Ctrl Pts',(-43.5226643663141,-55.7155033463606,
-48.156726413851));
#241408=CARTESIAN_POINT('Ctrl Pts',(-43.3014924724896,-55.859074841667,
-48.1720871103856));
#241409=CARTESIAN_POINT('Ctrl Pts',(-42.9323851716076,-56.2177417601912,
-48.2011948463009));
#241410=CARTESIAN_POINT('Ctrl Pts',(-42.7858689475892,-56.427284799075,
-48.2138068853757));
#241411=CARTESIAN_POINT('Ctrl Pts',(-42.5740319970683,-56.90072936033,-48.2414244847822));
#241412=CARTESIAN_POINT('Ctrl Pts',(-42.5149552732893,-57.1619571957634,
-48.2566627751824));
#241413=CARTESIAN_POINT('Ctrl Pts',(-42.5022899998702,-57.6851701559193,
-48.2871835311915));
#241414=CARTESIAN_POINT('Ctrl Pts',(-42.5460828168514,-57.9420979254273,
-48.3021709844128));
#241415=CARTESIAN_POINT('Ctrl Pts',(-42.7286059994751,-58.4241879338099,
-48.3302929015684));
#241416=CARTESIAN_POINT('Ctrl Pts',(-42.8652213300627,-58.6449019543281,
-48.3427378745441));
#241417=CARTESIAN_POINT('Ctrl Pts',(-43.2200686874805,-59.028421094374,
-48.3718500809782));
#241418=CARTESIAN_POINT('Ctrl Pts',(-43.4371401100596,-59.1853352594998,
-48.3873927905004));
#241419=CARTESIAN_POINT('Ctrl Pts',(-43.9107079826349,-59.4011832891677,
-48.4176121301696));
#241420=CARTESIAN_POINT('Ctrl Pts',(-44.1611161152121,-59.4616265808456,
-48.4320252147509));
#241421=CARTESIAN_POINT('Ctrl Pts',(-44.4467642018672,-59.4747510539149,
-48.4468384243579));
#241422=CARTESIAN_POINT('Ctrl Pts',(-44.4773707112758,-59.475452478349,
-48.4484050667596));
#241423=CARTESIAN_POINT('Ctrl Pts',(-44.5079524583205,-59.475452478349,
-48.4499499999999));
#241424=CARTESIAN_POINT('Ctrl Pts',(-44.5079524583203,-59.475452478349,
-48.2912000000001));
#241425=CARTESIAN_POINT('Ctrl Pts',(-44.4621954116032,-59.475452478349,
-48.2888884387167));
#241426=CARTESIAN_POINT('Ctrl Pts',(-44.4163914604066,-59.4738822430967,
-48.2865287093776));
#241427=CARTESIAN_POINT('Ctrl Pts',(-44.1153387113921,-59.4531611952842,
-48.2707157179857));
#241428=CARTESIAN_POINT('Ctrl Pts',(-43.8658276208728,-59.3867643302114,
-48.2561743044177));
#241429=CARTESIAN_POINT('Ctrl Pts',(-43.3963975797605,-59.1592356822322,
-48.2258233156324));
#241430=CARTESIAN_POINT('Ctrl Pts',(-43.1826463715709,-58.9967236975126,
-48.2102850674558));
#241431=CARTESIAN_POINT('Ctrl Pts',(-42.8376871341619,-58.604963811654,
-48.1814320354511));
#241432=CARTESIAN_POINT('Ctrl Pts',(-42.7069540844508,-58.3820868789375,
-48.1690870067012));
#241433=CARTESIAN_POINT('Ctrl Pts',(-42.5357120482107,-57.8964763928939,
-48.1407597283487));
#241434=CARTESIAN_POINT('Ctrl Pts',(-42.4978407438657,-57.6379968708878,
-48.1256817562316));
#241435=CARTESIAN_POINT('Ctrl Pts',(-42.5229742600458,-57.1146733989098,
-48.0951545536995));
#241436=CARTESIAN_POINT('Ctrl Pts',(-42.5882336096158,-56.8549517116878,
-48.0800041219449));
#241437=CARTESIAN_POINT('Ctrl Pts',(-42.8111568346108,-56.3868696565536,
-48.0526993353954));
#241438=CARTESIAN_POINT('Ctrl Pts',(-42.9624701342427,-56.1809849963628,
-48.039852937411));
#241439=CARTESIAN_POINT('Ctrl Pts',(-43.3402192219354,-55.8307817084993,
-48.01055549032));
#241440=CARTESIAN_POINT('Ctrl Pts',(-43.5653034425167,-55.6922107984702,
-47.9951430006849));
#241441=CARTESIAN_POINT('Ctrl Pts',(-44.0605946738937,-55.5079736091455,
-47.964748219992));
#241442=CARTESIAN_POINT('Ctrl Pts',(-44.3265194290946,-55.4659462558285,
-47.9506429255464));
#241443=CARTESIAN_POINT('Ctrl Pts',(-44.8477921988355,-55.4880805475756,
-47.9236636068181));
#241444=CARTESIAN_POINT('Ctrl Pts',(-45.0983247630082,-55.547615488173,
-47.9092707297562));
#241445=CARTESIAN_POINT('Ctrl Pts',(-45.5724986425265,-55.7616765882054,
-47.8790728945193));
#241446=CARTESIAN_POINT('Ctrl Pts',(-45.7900638885917,-55.9177317315564,
-47.8635302927506));
#241447=CARTESIAN_POINT('Ctrl Pts',(-46.1464129696538,-56.2999848121768,
-47.8343791487517));
#241448=CARTESIAN_POINT('Ctrl Pts',(-46.2839289948305,-56.520371900573,
-47.8219130337035));
#241449=CARTESIAN_POINT('Ctrl Pts',(-46.4681601359308,-57.0019225276565,
-47.7938225804569));
#241450=CARTESIAN_POINT('Ctrl Pts',(-46.5128449253758,-57.2586037516272,
-47.7788495090587));
#241451=CARTESIAN_POINT('Ctrl Pts',(-46.502065453837,-57.7817739277742,
-47.7483312487834));
#241452=CARTESIAN_POINT('Ctrl Pts',(-46.4439278569422,-58.0432165967563,
-47.7330804264262));
#241453=CARTESIAN_POINT('Ctrl Pts',(-46.2337741368597,-58.5174649721109,
-47.7054159378638));
#241454=CARTESIAN_POINT('Ctrl Pts',(-46.087979354215,-58.7275648603756,
-47.6928334223038));
#241455=CARTESIAN_POINT('Ctrl Pts',(-45.7201749141811,-59.0874981065514,
-47.6637545699499));
#241456=CARTESIAN_POINT('Ctrl Pts',(-45.4996004399675,-59.2318121470762,
-47.6484023963791));
#241457=CARTESIAN_POINT('Ctrl Pts',(-45.0192141980181,-59.4260158553972,
-47.6184698980189));
#241458=CARTESIAN_POINT('Ctrl Pts',(-44.7646955321978,-59.475452478349,
-47.6041701847465));
#241459=CARTESIAN_POINT('Ctrl Pts',(-44.5079524583206,-59.475452478349,
-47.5912000000001));
#241460=CARTESIAN_POINT('Origin',(-44.5079524583206,-57.475452478349,235.35105));
#241461=CARTESIAN_POINT('',(-44.5079524583207,-59.475452478349,-46.8912000000001));
#241462=CARTESIAN_POINT('',(-44.5079524583207,-59.475452478349,-47.0499499999999));
#241463=CARTESIAN_POINT('',(-44.5079524583206,-59.475452478349,235.35105));
#241464=CARTESIAN_POINT('Ctrl Pts',(-44.5079524583209,-59.475452478349,
-47.0499499999999));
#241465=CARTESIAN_POINT('Ctrl Pts',(-44.554453134705,-59.475452478349,-47.0522991280773));
#241466=CARTESIAN_POINT('Ctrl Pts',(-44.6009987273649,-59.4738307924441,
-47.0546978244141));
#241467=CARTESIAN_POINT('Ctrl Pts',(-44.912068432154,-59.4520723435267,
-47.0710471113981));
#241468=CARTESIAN_POINT('Ctrl Pts',(-45.1702827452092,-59.3811311768095,
-47.0861607377864));
#241469=CARTESIAN_POINT('Ctrl Pts',(-45.6384714922981,-59.1454875048052,
-47.1166857068967));
#241470=CARTESIAN_POINT('Ctrl Pts',(-45.845046645952,-58.985184775525,-47.1317969974673));
#241471=CARTESIAN_POINT('Ctrl Pts',(-46.1833632812087,-58.5972263874509,
-47.160203580491));
#241472=CARTESIAN_POINT('Ctrl Pts',(-46.3128857665671,-58.3741145541745,
-47.1725280455769));
#241473=CARTESIAN_POINT('Ctrl Pts',(-46.4843556329206,-57.8812457960168,
-47.2012787231362));
#241474=CARTESIAN_POINT('Ctrl Pts',(-46.5207502878101,-57.6149470298648,
-47.2168128178284));
#241475=CARTESIAN_POINT('Ctrl Pts',(-46.4878332043256,-57.0938436840021,
-47.2472105130038));
#241476=CARTESIAN_POINT('Ctrl Pts',(-46.4227720017422,-56.8437420795107,
-47.2617997732658));
#241477=CARTESIAN_POINT('Ctrl Pts',(-46.1987488490944,-56.3752321350285,
-47.2891295200273));
#241478=CARTESIAN_POINT('Ctrl Pts',(-46.0394483233293,-56.1625034323286,
-47.302542678224));
#241479=CARTESIAN_POINT('Ctrl Pts',(-45.6478297363726,-55.8111938166951,
-47.3325730546324));
#241480=CARTESIAN_POINT('Ctrl Pts',(-45.4195000234809,-55.6759647095067,
-47.3480520312806));
#241481=CARTESIAN_POINT('Ctrl Pts',(-44.9324736341766,-55.5046606707868,
-47.3776520705612));
#241482=CARTESIAN_POINT('Ctrl Pts',(-44.6796392315179,-55.4667966578895,
-47.3910242406569));
#241483=CARTESIAN_POINT('Ctrl Pts',(-44.1615720164789,-55.487907304876,
-47.417811764391));
#241484=CARTESIAN_POINT('Ctrl Pts',(-43.901443977928,-55.5512863718557,
-47.4328015074059));
#241485=CARTESIAN_POINT('Ctrl Pts',(-43.4259620690812,-55.7734635967845,
-47.4633021421722));
#241486=CARTESIAN_POINT('Ctrl Pts',(-43.2142804121466,-55.9282292382173,
-47.4785099054385));
#241487=CARTESIAN_POINT('Ctrl Pts',(-42.8654157666587,-56.3062986137255,
-47.5071609248768));
#241488=CARTESIAN_POINT('Ctrl Pts',(-42.730077021945,-56.5246626077399,
-47.5194872575478));
#241489=CARTESIAN_POINT('Ctrl Pts',(-42.5441636461992,-57.011993405316,
-47.5479148874064));
#241490=CARTESIAN_POINT('Ctrl Pts',(-42.4999150827817,-57.2779236701761,
-47.5634274861899));
#241491=CARTESIAN_POINT('Ctrl Pts',(-42.5180336880231,-57.8012381724356,
-47.5939541654883));
#241492=CARTESIAN_POINT('Ctrl Pts',(-42.5762410848256,-58.0537598286179,
-47.6086845954322));
#241493=CARTESIAN_POINT('Ctrl Pts',(-42.7866951827343,-58.5268191123656,
-47.6362797203175));
#241494=CARTESIAN_POINT('Ctrl Pts',(-42.9383900915285,-58.7421782610436,
-47.6492714505179));
#241495=CARTESIAN_POINT('Ctrl Pts',(-43.3179290873681,-59.1043602072032,
-47.6790086979881));
#241496=CARTESIAN_POINT('Ctrl Pts',(-43.542756808932,-59.2468604545175,
-47.6945228354385));
#241497=CARTESIAN_POINT('Ctrl Pts',(-44.018347888704,-59.4301501778751,
-47.723894766522));
#241498=CARTESIAN_POINT('Ctrl Pts',(-44.2621782516623,-59.475452478349,
-47.7375339421171));
#241499=CARTESIAN_POINT('Ctrl Pts',(-44.5079524583206,-59.475452478349,
-47.7499499999999));
#241500=CARTESIAN_POINT('Ctrl Pts',(-44.5079524583206,-59.475452478349,
-47.5912000000001));
#241501=CARTESIAN_POINT('Ctrl Pts',(-44.4998432267422,-59.475452478349,
-47.5907903366346));
#241502=CARTESIAN_POINT('Ctrl Pts',(-44.4917319195567,-59.475403158648,
-47.5903791299219));
#241503=CARTESIAN_POINT('Ctrl Pts',(-44.2291784192164,-59.4722085024506,
-47.577022235716));
#241504=CARTESIAN_POINT('Ctrl Pts',(-43.9777007086603,-59.4205837749565,
-47.5628123261575));
#241505=CARTESIAN_POINT('Ctrl Pts',(-43.4985314033797,-59.2221372272902,
-47.5328175557038));
#241506=CARTESIAN_POINT('Ctrl Pts',(-43.2768076913432,-59.0736178742876,
-47.5172846698186));
#241507=CARTESIAN_POINT('Ctrl Pts',(-42.907452770555,-58.7024976143473,
-47.4878012021461));
#241508=CARTESIAN_POINT('Ctrl Pts',(-42.7620494834633,-58.4849319964058,
-47.4750863052201));
#241509=CARTESIAN_POINT('Ctrl Pts',(-42.5630790326398,-58.0081056120536,
-47.4472714327996));
#241510=CARTESIAN_POINT('Ctrl Pts',(-42.5107516006776,-57.7536768518206,
-47.4324297551193));
#241511=CARTESIAN_POINT('Ctrl Pts',(-42.5052648978142,-57.2288086346005,
-47.4018124424481));
#241512=CARTESIAN_POINT('Ctrl Pts',(-42.5561860249955,-56.9633666331564,
-47.3863283256972));
#241513=CARTESIAN_POINT('Ctrl Pts',(-42.7543039331701,-56.4808577221684,
-47.3581819725562));
#241514=CARTESIAN_POINT('Ctrl Pts',(-42.8946125818443,-56.2664665314353,
-47.3457741867631));
#241515=CARTESIAN_POINT('Ctrl Pts',(-43.2524894351964,-55.8969644685894,
-47.3169177672217));
#241516=CARTESIAN_POINT('Ctrl Pts',(-43.4684496307538,-55.7470914534659,
-47.301636561692));
#241517=CARTESIAN_POINT('Ctrl Pts',(-43.9405559987394,-55.540767590807,
-47.2717688427325));
#241518=CARTESIAN_POINT('Ctrl Pts',(-44.1914799958216,-55.4842633210659,
-47.2574445857863));
#241519=CARTESIAN_POINT('Ctrl Pts',(-44.7138839733911,-55.468148873538,
-47.2305836993226));
#241520=CARTESIAN_POINT('Ctrl Pts',(-44.980503307442,-55.5137048163344,
-47.2162119128134));
#241521=CARTESIAN_POINT('Ctrl Pts',(-45.4741062072976,-55.7048858038013,
-47.1856998960573));
#241522=CARTESIAN_POINT('Ctrl Pts',(-45.6970536289956,-55.8462180502047,
-47.1703148145681));
#241523=CARTESIAN_POINT('Ctrl Pts',(-46.070058607397,-56.2010815829189,
-47.141121107287));
#241524=CARTESIAN_POINT('Ctrl Pts',(-46.2187357219036,-56.4089671497174,
-47.1284116441701));
#241525=CARTESIAN_POINT('Ctrl Pts',(-46.4355896459721,-56.8799995998964,
-47.100934751243));
#241526=CARTESIAN_POINT('Ctrl Pts',(-46.4974650403638,-57.1405654723828,
-47.085735075348));
#241527=CARTESIAN_POINT('Ctrl Pts',(-46.5157627592656,-57.6638654177115,
-47.0552092452038));
#241528=CARTESIAN_POINT('Ctrl Pts',(-46.4746397536553,-57.9215110250732,
-47.0401799181078));
#241529=CARTESIAN_POINT('Ctrl Pts',(-46.2972148278118,-58.4052011155574,
-47.0119646628295));
#241530=CARTESIAN_POINT('Ctrl Pts',(-46.1632721103581,-58.6268916802298,
-46.9995733740313));
#241531=CARTESIAN_POINT('Ctrl Pts',(-45.812900239099,-59.0141610223658,
-46.9705778799776));
#241532=CARTESIAN_POINT('Ctrl Pts',(-45.597316934554,-59.1736214523215,
-46.9550360813658));
#241533=CARTESIAN_POINT('Ctrl Pts',(-45.1255903396062,-59.3947747987772,
-46.924755021227));
#241534=CARTESIAN_POINT('Ctrl Pts',(-44.875571576505,-59.4579187488746,
-46.9102828376669));
#241535=CARTESIAN_POINT('Ctrl Pts',(-44.5829155271721,-59.4743998206703,
-46.8950176979641));
#241536=CARTESIAN_POINT('Ctrl Pts',(-44.5454166966125,-59.475452478349,
-46.8930926239556));
#241537=CARTESIAN_POINT('Ctrl Pts',(-44.5079524583208,-59.475452478349,
-46.8912000000001));
#241538=CARTESIAN_POINT('Origin',(-44.5079524583206,-57.475452478349,235.35105));
#241539=CARTESIAN_POINT('',(-44.5079524583208,-59.475452478349,-46.1912000000001));
#241540=CARTESIAN_POINT('',(-44.5079524583207,-59.475452478349,-46.3499499999999));
#241541=CARTESIAN_POINT('',(-44.5079524583206,-59.475452478349,235.35105));
#241542=CARTESIAN_POINT('Ctrl Pts',(-44.5079524583208,-59.475452478349,
-46.3499499999999));
#241543=CARTESIAN_POINT('Ctrl Pts',(-44.5908361851837,-59.475452478349,
-46.3541371324263));
#241544=CARTESIAN_POINT('Ctrl Pts',(-44.6737964586255,-59.4703007458636,
-46.3584783907082));
#241545=CARTESIAN_POINT('Ctrl Pts',(-45.0221714091031,-59.4266932865337,
-46.3773495324395));
#241546=CARTESIAN_POINT('Ctrl Pts',(-45.2785715363833,-59.340358089104,
-46.3928205020837));
#241547=CARTESIAN_POINT('Ctrl Pts',(-45.7332000740234,-59.0770467485376,
-46.4234674081851));
#241548=CARTESIAN_POINT('Ctrl Pts',(-45.9290817432164,-58.906102037805,
-46.4383488748448));
#241549=CARTESIAN_POINT('Ctrl Pts',(-46.2459051699612,-58.4984129368513,
-46.4662451398937));
#241550=CARTESIAN_POINT('Ctrl Pts',(-46.3635011048669,-58.2653115293938,
-46.4788748886891));
#241551=CARTESIAN_POINT('Ctrl Pts',(-46.5049851294361,-57.761535363337,
-46.5082618317092));
#241552=CARTESIAN_POINT('Ctrl Pts',(-46.5252725773139,-57.4951803379431,
-46.5237992081905));
#241553=CARTESIAN_POINT('Ctrl Pts',(-46.4622439250661,-56.9799096304069,
-46.5538566661302));
#241554=CARTESIAN_POINT('Ctrl Pts',(-46.3833552663526,-56.735365973496,
-46.5681217127833));
#241555=CARTESIAN_POINT('Ctrl Pts',(-46.133036947415,-56.279900627202,-46.5946905246505));
#241556=CARTESIAN_POINT('Ctrl Pts',(-45.9604381818125,-56.075230259504,
-46.6090795918312));
#241557=CARTESIAN_POINT('Ctrl Pts',(-45.5483555492046,-55.7474930231164,
-46.6394562462098));
#241558=CARTESIAN_POINT('Ctrl Pts',(-45.313926539347,-55.6264808190422,
-46.654828688374));
#241559=CARTESIAN_POINT('Ctrl Pts',(-44.8193921321944,-55.4836626264803,
-46.683977181636));
#241560=CARTESIAN_POINT('Ctrl Pts',(-44.5648339726336,-55.4602695427118,
-46.6966336155873));
#241561=CARTESIAN_POINT('Ctrl Pts',(-44.0486990700218,-55.5109070677797,
-46.7241847230859));
#241562=CARTESIAN_POINT('Ctrl Pts',(-43.792535812555,-55.5890557487495,
-46.739404953109));
#241563=CARTESIAN_POINT('Ctrl Pts',(-43.3317119004113,-55.837408838538,
-46.7699285557454));
#241564=CARTESIAN_POINT('Ctrl Pts',(-43.1301735590373,-56.0028763520636,
-46.7849360354254));
#241565=CARTESIAN_POINT('Ctrl Pts',(-42.8020680499677,-56.4002800798801,
-46.8131022603353));
#241566=CARTESIAN_POINT('Ctrl Pts',(-42.6781971428059,-56.6280819866651,
-46.8255200546518));
#241567=CARTESIAN_POINT('Ctrl Pts',(-42.5208805642364,-57.1262024590094,
-46.8545770822051));
#241568=CARTESIAN_POINT('Ctrl Pts',(-42.492126463739,-57.3926454432649,
-46.87011958962));
#241569=CARTESIAN_POINT('Ctrl Pts',(-42.5393672164669,-57.9112001860202,
-46.9003686162807));
#241570=CARTESIAN_POINT('Ctrl Pts',(-42.6110260474126,-58.1587652900053,
-46.9148099140131));
#241571=CARTESIAN_POINT('Ctrl Pts',(-42.8483243182583,-58.6227201281582,
-46.9418739462387));
#241572=CARTESIAN_POINT('Ctrl Pts',(-43.0152502744431,-58.8328355800266,
-46.9557984564599));
#241573=CARTESIAN_POINT('Ctrl Pts',(-43.4187222852275,-59.1731699315095,
-46.9861075340231));
#241574=CARTESIAN_POINT('Ctrl Pts',(-43.6502924057069,-59.301127519383,
-47.0015381240831));
#241575=CARTESIAN_POINT('Ctrl Pts',(-44.0968123151278,-59.4436164931208,
-47.0282514116003));
#241576=CARTESIAN_POINT('Ctrl Pts',(-44.3018947694972,-59.475452478349,
-47.0395403470652));
#241577=CARTESIAN_POINT('Ctrl Pts',(-44.5079524583209,-59.475452478349,
-47.0499499999999));
#241578=CARTESIAN_POINT('Ctrl Pts',(-44.5079524583208,-59.475452478349,
-46.8912000000001));
#241579=CARTESIAN_POINT('Ctrl Pts',(-44.2808580754121,-59.475452478349,
-46.8797276122286));
#241580=CARTESIAN_POINT('Ctrl Pts',(-44.0551473047433,-59.4367820789147,
-46.8671972353355));
#241581=CARTESIAN_POINT('Ctrl Pts',(-43.5933321620571,-59.2732901054593,
-46.8390986734603));
#241582=CARTESIAN_POINT('Ctrl Pts',(-43.3657623743608,-59.1380271069426,
-46.823657098329));
#241583=CARTESIAN_POINT('Ctrl Pts',(-42.9824160998001,-58.793366905255,
-46.7942385650673));
#241584=CARTESIAN_POINT('Ctrl Pts',(-42.8279825519172,-58.5898207593303,
-46.7812048163908));
#241585=CARTESIAN_POINT('Ctrl Pts',(-42.59795005691,-58.1252391266868,-46.7541042211533));
#241586=CARTESIAN_POINT('Ctrl Pts',(-42.5287310253326,-57.8665667397225,
-46.7390149985803));
#241587=CARTESIAN_POINT('Ctrl Pts',(-42.4955628885015,-57.343330519362,
-46.7084928857259));
#241588=CARTESIAN_POINT('Ctrl Pts',(-42.5295960628064,-57.0839230875256,
-46.6933607855354));
#241589=CARTESIAN_POINT('Ctrl Pts',(-42.6935751068041,-56.5960826489329,
-46.6649034266175));
#241590=CARTESIAN_POINT('Ctrl Pts',(-42.8205782309082,-56.3718114885146,
-46.65258682635));
#241591=CARTESIAN_POINT('Ctrl Pts',(-43.1592022603968,-55.9748533589649,
-46.6239022218791));
#241592=CARTESIAN_POINT('Ctrl Pts',(-43.3707644901368,-55.8088081333853,
-46.6083715039825));
#241593=CARTESIAN_POINT('Ctrl Pts',(-43.8374104957225,-55.5738739682217,
-46.5779451652662));
#241594=CARTESIAN_POINT('Ctrl Pts',(-44.0862767230464,-55.5036880267608,
-46.5633258142649));
#241595=CARTESIAN_POINT('Ctrl Pts',(-44.6034481677545,-55.4605330491705,
-46.5359405835467));
#241596=CARTESIAN_POINT('Ctrl Pts',(-44.8670057249247,-55.4904753426572,
-46.5226231268631));
#241597=CARTESIAN_POINT('Ctrl Pts',(-45.3677801070811,-55.6506619888066,
-46.4926528217206));
#241598=CARTESIAN_POINT('Ctrl Pts',(-45.6000180238917,-55.7794118764381,
-46.4771653870833));
#241599=CARTESIAN_POINT('Ctrl Pts',(-45.9941310039061,-56.1132670012756,
-46.4475180878708));
#241600=CARTESIAN_POINT('Ctrl Pts',(-46.1546038227961,-56.3123768136984,
-46.4340460804379));
#241601=CARTESIAN_POINT('Ctrl Pts',(-46.3981604390762,-56.7701693522984,
-46.4073415156862));
#241602=CARTESIAN_POINT('Ctrl Pts',(-46.4748923274485,-57.0266655892397,
-46.392379235198));
#241603=CARTESIAN_POINT('Ctrl Pts',(-46.5234131951804,-57.5493898930644,
-46.3618869841416));
#241604=CARTESIAN_POINT('Ctrl Pts',(-46.4967628570803,-57.8104132845754,
-46.3466606196368));
#241605=CARTESIAN_POINT('Ctrl Pts',(-46.346663598018,-58.3024334517028,
-46.3179594432211));
#241606=CARTESIAN_POINT('Ctrl Pts',(-46.2266684269433,-58.5293809990701,
-46.3056201001042));
#241607=CARTESIAN_POINT('Ctrl Pts',(-45.9000785678642,-58.9360461067693,
-46.2772603194458));
#241608=CARTESIAN_POINT('Ctrl Pts',(-45.6928021629035,-59.1086854318011,
-46.2617537855815));
#241609=CARTESIAN_POINT('Ctrl Pts',(-45.2317220985817,-59.3575112238338,
-46.2312034554625));
#241610=CARTESIAN_POINT('Ctrl Pts',(-44.9842283485895,-59.4348358761522,
-46.2164452270749));
#241611=CARTESIAN_POINT('Ctrl Pts',(-44.6553612302489,-59.471382934638,
-46.1987655132635));
#241612=CARTESIAN_POINT('Ctrl Pts',(-44.5816172779389,-59.475452478349,
-46.1949214103008));
#241613=CARTESIAN_POINT('Ctrl Pts',(-44.507952458321,-59.475452478349,-46.1912000000001));
#241614=CARTESIAN_POINT('Origin',(-44.5079524583206,-57.475452478349,235.35105));
#241615=CARTESIAN_POINT('',(-44.5079524583206,-59.475452478349,-45.4912000000001));
#241616=CARTESIAN_POINT('',(-44.5079524583206,-59.475452478349,-45.6499499999999));
#241617=CARTESIAN_POINT('',(-44.5079524583206,-59.475452478349,235.35105));
#241618=CARTESIAN_POINT('Ctrl Pts',(-44.5079524583206,-59.475452478349,
-45.6499499999999));
#241619=CARTESIAN_POINT('Ctrl Pts',(-44.6297441139361,-59.475452478349,
-45.6561026889509));
#241620=CARTESIAN_POINT('Ctrl Pts',(-44.7515417358596,-59.4643298262064,
-45.6625800899963));
#241621=CARTESIAN_POINT('Ctrl Pts',(-45.1337106204023,-59.3936149337826,
-45.6839490721741));
#241622=CARTESIAN_POINT('Ctrl Pts',(-45.3832534767605,-59.2933478816507,
-45.6994799709494));
#241623=CARTESIAN_POINT('Ctrl Pts',(-45.8199388022307,-59.0065682461395,
-45.7299049111287));
#241624=CARTESIAN_POINT('Ctrl Pts',(-46.005097617392,-58.8260886971062,
-45.7445227785059));
#241625=CARTESIAN_POINT('Ctrl Pts',(-46.3009460682604,-58.3996852797117,
-45.7719052608371));
#241626=CARTESIAN_POINT('Ctrl Pts',(-46.406731146095,-58.1564119291741,
-45.7852273653686));
#241627=CARTESIAN_POINT('Ctrl Pts',(-46.5182327027892,-57.6425839989162,
-45.8152006613004));
#241628=CARTESIAN_POINT('Ctrl Pts',(-46.5227680569918,-57.3770920683106,
-45.8306876905857));
#241629=CARTESIAN_POINT('Ctrl Pts',(-46.4305442437757,-56.8688927081907,
-45.8603326532594));
#241630=CARTESIAN_POINT('Ctrl Pts',(-46.3382757391706,-56.6303958485609,
-45.8737996082983));
#241631=CARTESIAN_POINT('Ctrl Pts',(-46.0634635452641,-56.1906583335379,
-45.9005082890561));
#241632=CARTESIAN_POINT('Ctrl Pts',(-45.8796383631409,-55.9960133343155,
-45.9154719427252));
#241633=CARTESIAN_POINT('Ctrl Pts',(-45.4511207021371,-55.6927639318498,
-45.9459646358205));
#241634=CARTESIAN_POINT('Ctrl Pts',(-45.2117179810681,-55.5854059851322,
-45.9611900914936));
#241635=CARTESIAN_POINT('Ctrl Pts',(-44.7105316985395,-55.4695306937223,
-45.9898887905671));
#241636=CARTESIAN_POINT('Ctrl Pts',(-44.4539800785212,-55.4600514463944,
-46.0022273879353));
#241637=CARTESIAN_POINT('Ctrl Pts',(-43.9385263862013,-55.5397101292635,
-46.0305905323871));
#241638=CARTESIAN_POINT('Ctrl Pts',(-43.6854136309263,-55.6329692967654,
-46.0460973792111));
#241639=CARTESIAN_POINT('Ctrl Pts',(-43.2394770383604,-55.9079850838125,
-46.0766465640289));
#241640=CARTESIAN_POINT('Ctrl Pts',(-43.0488205774223,-56.0837080598058,
-46.0914034289118));
#241641=CARTESIAN_POINT('Ctrl Pts',(-42.7422758405384,-56.5006333173148,
-46.1190498214788));
#241642=CARTESIAN_POINT('Ctrl Pts',(-42.6304392461764,-56.7386689927291,
-46.1319709633388));
#241643=CARTESIAN_POINT('Ctrl Pts',(-42.5035589820785,-57.2474506857119,
-46.1616498954294));
#241644=CARTESIAN_POINT('Ctrl Pts',(-42.4909937423021,-57.5134969494907,
-46.1771692608165));
#241645=CARTESIAN_POINT('Ctrl Pts',(-42.5683675957886,-58.025504112438,
-46.2070363453217));
#241646=CARTESIAN_POINT('Ctrl Pts',(-42.6538337684111,-58.2670866382577,
-46.2210393529167));
#241647=CARTESIAN_POINT('Ctrl Pts',(-42.9160906849344,-58.7149129781829,
-46.2473496883661));
#241648=CARTESIAN_POINT('Ctrl Pts',(-43.0941978562435,-58.9147341367152,
-46.2621754500287));
#241649=CARTESIAN_POINT('Ctrl Pts',(-43.5143261571294,-59.2306248434691,
-46.2926130328917));
#241650=CARTESIAN_POINT('Ctrl Pts',(-43.7512634012235,-59.3450399339582,
-46.3079197705927));
#241651=CARTESIAN_POINT('Ctrl Pts',(-44.1685463803989,-59.4538108059516,
-46.3321726178903));
#241652=CARTESIAN_POINT('Ctrl Pts',(-44.3380564620073,-59.475452478349,
-46.3413671688194));
#241653=CARTESIAN_POINT('Ctrl Pts',(-44.5079524583208,-59.475452478349,
-46.3499499999999));
#241654=CARTESIAN_POINT('Ctrl Pts',(-44.507952458321,-59.475452478349,-46.1912000000001));
#241655=CARTESIAN_POINT('Ctrl Pts',(-44.3220721510077,-59.475452478349,
-46.181809671022));
#241656=CARTESIAN_POINT('Ctrl Pts',(-44.1367724407075,-59.4495470295496,
-46.1716930971401));
#241657=CARTESIAN_POINT('Ctrl Pts',(-43.7037790848822,-59.3255571982284,
-46.1462027043874));
#241658=CARTESIAN_POINT('Ctrl Pts',(-43.4670490297897,-59.203484337701,
-46.130683081865));
#241659=CARTESIAN_POINT('Ctrl Pts',(-43.0622163648016,-58.8805848381541,
-46.1008137830855));
#241660=CARTESIAN_POINT('Ctrl Pts',(-42.8956711117532,-58.6858213338311,
-46.0868048499034));
#241661=CARTESIAN_POINT('Ctrl Pts',(-42.6388372387598,-58.2348563683312,
-46.0604985602492));
#241662=CARTESIAN_POINT('Ctrl Pts',(-42.5547671602554,-57.9807253290289,
-46.0456742496232));
#241663=CARTESIAN_POINT('Ctrl Pts',(-42.4911096915645,-57.4589499384175,
-46.0152373518375));
#241664=CARTESIAN_POINT('Ctrl Pts',(-42.5104177753976,-57.1965357354181,
-45.9999298566625));
#241665=CARTESIAN_POINT('Ctrl Pts',(-42.6468081439976,-56.7004985387426,
-45.9709943535231));
#241666=CARTESIAN_POINT('Ctrl Pts',(-42.7600313966352,-56.4708778366039,
-45.9585349754709));
#241667=CARTESIAN_POINT('Ctrl Pts',(-43.0748340898635,-56.0549111182015,
-45.9304993636291));
#241668=CARTESIAN_POINT('Ctrl Pts',(-43.2777582471938,-55.8759672341481,
-45.9150288142856));
#241669=CARTESIAN_POINT('Ctrl Pts',(-43.733047124395,-55.6137701281319,
-45.8843810475599));
#241670=CARTESIAN_POINT('Ctrl Pts',(-43.979014233557,-55.5295350993375,
-45.8694983895933));
#241671=CARTESIAN_POINT('Ctrl Pts',(-44.4904661217093,-55.4588679546952,
-45.8415996620773));
#241672=CARTESIAN_POINT('Ctrl Pts',(-44.7511223131829,-55.4735040185731,
-45.8289723392249));
#241673=CARTESIAN_POINT('Ctrl Pts',(-45.2581756857081,-55.6027132949404,
-45.7995883377328));
#241674=CARTESIAN_POINT('Ctrl Pts',(-45.4990296628474,-55.7182559587453,
-45.7840508463748));
#241675=CARTESIAN_POINT('Ctrl Pts',(-45.9138517687926,-56.0303682340407,
-45.7539915269071));
#241676=CARTESIAN_POINT('Ctrl Pts',(-46.0862455518917,-56.2209174650915,
-45.739724826257));
#241677=CARTESIAN_POINT('Ctrl Pts',(-46.3556550946895,-56.6653663866578,
-45.7131516614064));
#241678=CARTESIAN_POINT('Ctrl Pts',(-46.4466733942451,-56.9171528251501,
-45.6987674797699));
#241679=CARTESIAN_POINT('Ctrl Pts',(-46.5246017804916,-57.4378819276168,
-45.6683916154593));
#241680=CARTESIAN_POINT('Ctrl Pts',(-46.5122560120561,-57.7014197356871,
-45.6530185766552));
#241681=CARTESIAN_POINT('Ctrl Pts',(-46.3888011260386,-58.2011442186326,
-45.6238679818168));
#241682=CARTESIAN_POINT('Ctrl Pts',(-46.2818425465019,-58.4333200741879,
-45.6112091714481));
#241683=CARTESIAN_POINT('Ctrl Pts',(-45.9800340851223,-58.8550639774218,
-45.583661502917));
#241684=CARTESIAN_POINT('Ctrl Pts',(-45.7843219229271,-59.0378846869053,
-45.5684422161401));
#241685=CARTESIAN_POINT('Ctrl Pts',(-45.3388968597982,-59.3129136606705,
-45.5379184882298));
#241686=CARTESIAN_POINT('Ctrl Pts',(-45.0948460428784,-59.4047825186084,
-45.5229099844494));
#241687=CARTESIAN_POINT('Ctrl Pts',(-44.7300666440941,-59.4662076315768,
-45.5026904387972));
#241688=CARTESIAN_POINT('Ctrl Pts',(-44.6189869517897,-59.475452478349,
-45.4968092570358));
#241689=CARTESIAN_POINT('Ctrl Pts',(-44.5079524583207,-59.475452478349,
-45.4912000000001));
#241690=CARTESIAN_POINT('Origin',(-44.5079524583206,-57.475452478349,235.35105));
#241691=CARTESIAN_POINT('',(-44.5079524583206,-59.475452478349,-44.7912000000002));
#241692=CARTESIAN_POINT('',(-44.5079524583205,-59.475452478349,-44.9499499999999));
#241693=CARTESIAN_POINT('',(-44.5079524583206,-59.475452478349,235.35105));
#241694=CARTESIAN_POINT('Ctrl Pts',(-44.5079524583205,-59.475452478349,
-44.9499499999999));
#241695=CARTESIAN_POINT('Ctrl Pts',(-44.6703684237631,-59.475452478349,
-44.9581549538697));
#241696=CARTESIAN_POINT('Ctrl Pts',(-44.8325030142928,-59.4556741995973,
-44.9669225596634));
#241697=CARTESIAN_POINT('Ctrl Pts',(-45.247675743369,-59.3523848442981,
-44.9909089234627));
#241698=CARTESIAN_POINT('Ctrl Pts',(-45.4893066193448,-59.2381195950336,
-45.0064484043874));
#241699=CARTESIAN_POINT('Ctrl Pts',(-45.9060511378812,-58.9281085094198,
-45.0365435558811));
#241700=CARTESIAN_POINT('Ctrl Pts',(-46.0795556928749,-58.7383847653617,
-45.0508422939668));
#241701=CARTESIAN_POINT('Ctrl Pts',(-46.3513816465344,-58.2952247764233,
-45.0774999375521));
#241702=CARTESIAN_POINT('Ctrl Pts',(-46.4437230807142,-58.0439030757439,
-45.0917903818188));
#241703=CARTESIAN_POINT('Ctrl Pts',(-46.5243979108967,-57.5234451878826,
-45.1221504252774));
#241704=CARTESIAN_POINT('Ctrl Pts',(-46.513399658897,-57.2597115764675,
-45.1375348859433));
#241705=CARTESIAN_POINT('Ctrl Pts',(-46.3924429660938,-56.759286698404,
-45.1667263371637));
#241706=CARTESIAN_POINT('Ctrl Pts',(-46.2866811829253,-56.5266133472947,
-45.1794330593757));
#241707=CARTESIAN_POINT('Ctrl Pts',(-45.9870610340795,-56.1033784147385,
-45.2069136667644));
#241708=CARTESIAN_POINT('Ctrl Pts',(-45.7922898933191,-55.9195645725112,
-45.2221143812524));
#241709=CARTESIAN_POINT('Ctrl Pts',(-45.348174920298,-55.642197391229,-45.2526401235552));
#241710=CARTESIAN_POINT('Ctrl Pts',(-45.1044666494907,-55.5490583428045,
-45.2676683697628));
#241711=CARTESIAN_POINT('Ctrl Pts',(-44.5968355188062,-55.461004847915,
-45.2958811815676));
#241712=CARTESIAN_POINT('Ctrl Pts',(-44.3378617632765,-55.4662308166362,
-45.3082737018668));
#241713=CARTESIAN_POINT('Ctrl Pts',(-43.8273168932962,-55.5761779309857,
-45.3372722742871));
#241714=CARTESIAN_POINT('Ctrl Pts',(-43.5814664495911,-55.683215764723,
-45.3528141203417));
#241715=CARTESIAN_POINT('Ctrl Pts',(-43.154174566203,-55.9812782558104,
-45.383093604506));
#241716=CARTESIAN_POINT('Ctrl Pts',(-42.9745369553145,-56.1662734510742,
-45.3975642572139));
#241717=CARTESIAN_POINT('Ctrl Pts',(-42.6893359665779,-56.601978518829,
-45.4246801476068));
#241718=CARTESIAN_POINT('Ctrl Pts',(-42.5896481370744,-56.8505634377133,
-45.4384981392962));
#241719=CARTESIAN_POINT('Ctrl Pts',(-42.4936376452033,-57.3692352948812,
-45.468753997631));
#241720=CARTESIAN_POINT('Ctrl Pts',(-42.4970744065062,-57.6339388582957,
-45.4841950388301));
#241721=CARTESIAN_POINT('Ctrl Pts',(-42.6040345512156,-58.1382162765997,
-45.5136112215644));
#241722=CARTESIAN_POINT('Ctrl Pts',(-42.7031637847086,-58.3737025820734,
-45.5266410457028));
#241723=CARTESIAN_POINT('Ctrl Pts',(-42.9906155422345,-58.8051218901766,
-45.5537456394447));
#241724=CARTESIAN_POINT('Ctrl Pts',(-43.1800795861886,-58.994347381544,
-45.5688360889943));
#241725=CARTESIAN_POINT('Ctrl Pts',(-43.6167121529827,-59.2845558038791,
-45.5993583701853));
#241726=CARTESIAN_POINT('Ctrl Pts',(-43.8584044517106,-59.3847122446367,
-45.6144894471589));
#241727=CARTESIAN_POINT('Ctrl Pts',(-44.2429768168709,-59.4622861285099,
-45.6361799026449));
#241728=CARTESIAN_POINT('Ctrl Pts',(-44.3754414902991,-59.475452478349,
-45.6432557912323));
#241729=CARTESIAN_POINT('Ctrl Pts',(-44.5079524583206,-59.475452478349,
-45.6499499999999));
#241730=CARTESIAN_POINT('Ctrl Pts',(-44.5079524583207,-59.475452478349,
-45.4912000000001));
#241731=CARTESIAN_POINT('Ctrl Pts',(-44.3631837356181,-59.475452478349,
-45.4838865521606));
#241732=CARTESIAN_POINT('Ctrl Pts',(-44.2185386657933,-59.4597381216607,
-45.4761210156323));
#241733=CARTESIAN_POINT('Ctrl Pts',(-43.8173863312277,-59.3711192579799,
-45.4532708255445));
#241734=CARTESIAN_POINT('Ctrl Pts',(-43.5722271629013,-59.2628621673636,
-45.4377283397833));
#241735=CARTESIAN_POINT('Ctrl Pts',(-43.1466761350244,-58.9627769154267,
-45.4074778032249));
#241736=CARTESIAN_POINT('Ctrl Pts',(-42.9680554613902,-58.7769772398011,
-45.3930350602937));
#241737=CARTESIAN_POINT('Ctrl Pts',(-42.6848073184084,-58.3395805164596,
-45.3659684840981));
#241738=CARTESIAN_POINT('Ctrl Pts',(-42.5862468213381,-58.0900114512799,
-45.3520492734212));
#241739=CARTESIAN_POINT('Ctrl Pts',(-42.4930970950562,-57.5704717910895,
-45.3217427932434));
#241740=CARTESIAN_POINT('Ctrl Pts',(-42.497992524066,-57.3059384089094,
-45.3063116792829));
#241741=CARTESIAN_POINT('Ctrl Pts',(-42.6076504567339,-56.8023940160349,
-45.2769382563651));
#241742=CARTESIAN_POINT('Ctrl Pts',(-42.7080488419627,-56.5674533582485,
-45.2639778239381));
#241743=CARTESIAN_POINT('Ctrl Pts',(-42.9978337533079,-56.1375895827023,
-45.2368007332845));
#241744=CARTESIAN_POINT('Ctrl Pts',(-43.1883249155673,-55.949387068423,
-45.2216882324514));
#241745=CARTESIAN_POINT('Ctrl Pts',(-43.6264177179127,-55.6616194103928,
-45.1911633718228));
#241746=CARTESIAN_POINT('Ctrl Pts',(-43.8685110354901,-55.5628022955403,
-45.1760510997916));
#241747=CARTESIAN_POINT('Ctrl Pts',(-44.3736200988442,-55.4636554886945,
-45.1476421432267));
#241748=CARTESIAN_POINT('Ctrl Pts',(-44.6315898416643,-55.4629700035312,
-45.1353181404835));
#241749=CARTESIAN_POINT('Ctrl Pts',(-45.144185906275,-55.5607596082545,
-45.1065705395388));
#241750=CARTESIAN_POINT('Ctrl Pts',(-45.3930404753725,-55.66232340238,-45.0910365901201));
#241751=CARTESIAN_POINT('Ctrl Pts',(-45.8279620987918,-55.9512703836321,
-45.0606375346524));
#241752=CARTESIAN_POINT('Ctrl Pts',(-46.0120797555593,-56.132620985077,
-45.0460468589742));
#241753=CARTESIAN_POINT('Ctrl Pts',(-46.3059139123148,-56.5607942558644,
-45.0187145143283));
#241754=CARTESIAN_POINT('Ctrl Pts',(-46.4105515514957,-56.8050651998506,
-45.005305924579));
#241755=CARTESIAN_POINT('Ctrl Pts',(-46.5191363970842,-57.319823682072,
-44.9752783464494));
#241756=CARTESIAN_POINT('Ctrl Pts',(-46.5221615004682,-57.585184577012,
-44.9597989609113));
#241757=CARTESIAN_POINT('Ctrl Pts',(-46.4271463345645,-58.0926518279142,
-44.9301967046087));
#241758=CARTESIAN_POINT('Ctrl Pts',(-46.333587196176,-58.3305744990687,
-44.9168199612882));
#241759=CARTESIAN_POINT('Ctrl Pts',(-46.0563945341639,-58.768759149932,
-44.8900363155604));
#241760=CARTESIAN_POINT('Ctrl Pts',(-45.8714980102073,-58.96239935367,-44.8750478462204));
#241761=CARTESIAN_POINT('Ctrl Pts',(-45.4414261170752,-59.2632164444138,
-44.8445475786209));
#241762=CARTESIAN_POINT('Ctrl Pts',(-45.2015772341122,-59.3692252891307,
-44.8293389324833));
#241763=CARTESIAN_POINT('Ctrl Pts',(-44.8033600491983,-59.459077523037,
-44.8066010474234));
#241764=CARTESIAN_POINT('Ctrl Pts',(-44.6557335545469,-59.475452478349,
-44.7986656273728));
#241765=CARTESIAN_POINT('Ctrl Pts',(-44.5079524583206,-59.475452478349,
-44.7912000000001));
#241766=CARTESIAN_POINT('Origin',(-44.5079524583206,-57.475452478349,235.35105));
#241767=CARTESIAN_POINT('',(-44.5079524583204,-59.475452478349,-44.0912000000001));
#241768=CARTESIAN_POINT('',(-44.5079524583204,-59.475452478349,-44.2499499999999));
#241769=CARTESIAN_POINT('',(-44.5079524583206,-59.475452478349,235.35105));
#241770=CARTESIAN_POINT('Ctrl Pts',(-44.5079524583202,-59.475452478349,
-44.2499499999999));
#241771=CARTESIAN_POINT('Ctrl Pts',(-44.7020823833798,-59.475452478349,
-44.2597570843928));
#241772=CARTESIAN_POINT('Ctrl Pts',(-44.895461652298,-59.4471963517014,
-44.2703503840545));
#241773=CARTESIAN_POINT('Ctrl Pts',(-45.3326169478005,-59.3162010396124,
-44.2962553568166));
#241774=CARTESIAN_POINT('Ctrl Pts',(-45.5660396176025,-59.1926805068228,
-44.3116501201319));
#241775=CARTESIAN_POINT('Ctrl Pts',(-45.9766397528035,-58.8591026172973,
-44.3421222338695));
#241776=CARTESIAN_POINT('Ctrl Pts',(-46.148233658917,-58.6505822291728,
-44.3564007645353));
#241777=CARTESIAN_POINT('Ctrl Pts',(-46.3935029008547,-58.1894129661638,
-44.3833023048775));
#241778=CARTESIAN_POINT('Ctrl Pts',(-46.4690683573656,-57.9434484530477,
-44.3976502348093));
#241779=CARTESIAN_POINT('Ctrl Pts',(-46.5248279196195,-57.4266031567635,
-44.4277995437592));
#241780=CARTESIAN_POINT('Ctrl Pts',(-46.500636301891,-57.1601751210114,
-44.4433411791781));
#241781=CARTESIAN_POINT('Ctrl Pts',(-46.3518301060207,-56.6589853359418,
-44.4725772499739));
#241782=CARTESIAN_POINT('Ctrl Pts',(-46.2313372582583,-56.4283416300066,
-44.4850951904043));
#241783=CARTESIAN_POINT('Ctrl Pts',(-45.9093143253537,-56.0253732506028,
-44.5131164371659));
#241784=CARTESIAN_POINT('Ctrl Pts',(-45.710814646849,-55.8569226816391,
-44.5280574150073));
#241785=CARTESIAN_POINT('Ctrl Pts',(-45.2545105909144,-55.6011591450698,
-44.5585688209075));
#241786=CARTESIAN_POINT('Ctrl Pts',(-44.9996581311869,-55.5187751452991,
-44.5738463619873));
#241787=CARTESIAN_POINT('Ctrl Pts',(-44.4841973251914,-55.4595792055189,
-44.601613035802));
#241788=CARTESIAN_POINT('Ctrl Pts',(-44.2290775712395,-55.4788165537459,
-44.6141363618394));
#241789=CARTESIAN_POINT('Ctrl Pts',(-43.7324987118838,-55.6135337419647,
-44.6431518577482));
#241790=CARTESIAN_POINT('Ctrl Pts',(-43.4964918993264,-55.7304577057381,
-44.6584847672415));
#241791=CARTESIAN_POINT('Ctrl Pts',(-43.0793092444697,-56.0509185764088,
-44.6889068379682));
#241792=CARTESIAN_POINT('Ctrl Pts',(-42.9033161117682,-56.2526102145332,
-44.7036175346107));
#241793=CARTESIAN_POINT('Ctrl Pts',(-42.6455690443934,-56.703328973278,
-44.7299094622041));
#241794=CARTESIAN_POINT('Ctrl Pts',(-42.5626142744282,-56.9460582767092,
-44.7440686715709));
#241795=CARTESIAN_POINT('Ctrl Pts',(-42.4906627140526,-57.4592483089433,
-44.7740047567846));
#241796=CARTESIAN_POINT('Ctrl Pts',(-42.5061436817519,-57.7254368847256,
-44.7895324237052));
#241797=CARTESIAN_POINT('Ctrl Pts',(-42.6385579739842,-58.2323459492272,
-44.8191021191344));
#241798=CARTESIAN_POINT('Ctrl Pts',(-42.7525747976378,-58.4685069477834,
-44.8319023259275));
#241799=CARTESIAN_POINT('Ctrl Pts',(-43.0630004304665,-58.8819598003333,
-44.8596434956944));
#241800=CARTESIAN_POINT('Ctrl Pts',(-43.2556370349585,-59.0559024907331,
-44.8744484687671));
#241801=CARTESIAN_POINT('Ctrl Pts',(-43.7048794642206,-59.3265447748553,
-44.9050370978322));
#241802=CARTESIAN_POINT('Ctrl Pts',(-43.9592505100791,-59.4172112392399,
-44.920531890674));
#241803=CARTESIAN_POINT('Ctrl Pts',(-44.3182135068885,-59.468708630863,
-44.9401680439288));
#241804=CARTESIAN_POINT('Ctrl Pts',(-44.4131209121855,-59.475452478349,
-44.9451592858646));
#241805=CARTESIAN_POINT('Ctrl Pts',(-44.5079524583205,-59.475452478349,
-44.9499499999999));
#241806=CARTESIAN_POINT('Ctrl Pts',(-44.5079524583205,-59.475452478349,
-44.7912000000001));
#241807=CARTESIAN_POINT('Ctrl Pts',(-44.4022180531919,-59.475452478349,
-44.7858584936146));
#241808=CARTESIAN_POINT('Ctrl Pts',(-44.2964294722225,-59.467069050198,
-44.7802697337115));
#241809=CARTESIAN_POINT('Ctrl Pts',(-43.9279727565971,-59.4080384353609,
-44.7599342563497));
#241810=CARTESIAN_POINT('Ctrl Pts',(-43.6755120802264,-59.3134619513892,
-44.7444219296143));
#241811=CARTESIAN_POINT('Ctrl Pts',(-43.2312790046323,-59.0362283816049,
-44.7138941179901));
#241812=CARTESIAN_POINT('Ctrl Pts',(-43.0416396211848,-58.8596050514797,
-44.69916237365));
#241813=CARTESIAN_POINT('Ctrl Pts',(-42.7370820431139,-58.4409087264589,
-44.6715647125313));
#241814=CARTESIAN_POINT('Ctrl Pts',(-42.626364776298,-58.2019077703289,
-44.6585765586991));
#241815=CARTESIAN_POINT('Ctrl Pts',(-42.5023275829223,-57.6921756209946,
-44.6288421833212));
#241816=CARTESIAN_POINT('Ctrl Pts',(-42.4912550434187,-57.4262143382321,
-44.61332777516));
#241817=CARTESIAN_POINT('Ctrl Pts',(-42.5713911869543,-56.9149042401955,
-44.5835013527745));
#241818=CARTESIAN_POINT('Ctrl Pts',(-42.6581149484718,-56.6738996256653,
-44.569605074587));
#241819=CARTESIAN_POINT('Ctrl Pts',(-42.9226934049082,-56.2275563495412,
-44.5432207152669));
#241820=CARTESIAN_POINT('Ctrl Pts',(-43.1018661319024,-56.0286765671277,
-44.5283685805073));
#241821=CARTESIAN_POINT('Ctrl Pts',(-43.5235695202026,-55.7150992511455,
-44.4979189010419));
#241822=CARTESIAN_POINT('Ctrl Pts',(-43.7609767029779,-55.6019814627906,
-44.4826262608876));
#241823=CARTESIAN_POINT('Ctrl Pts',(-44.2594174029405,-55.4747781833009,
-44.4537358639097));
#241824=CARTESIAN_POINT('Ctrl Pts',(-44.5150870437871,-55.4594156358102,
-44.4413073151922));
#241825=CARTESIAN_POINT('Ctrl Pts',(-45.0323200202224,-55.5269341683579,
-44.4132083723189));
#241826=CARTESIAN_POINT('Ctrl Pts',(-45.2881313028365,-55.6145463245205,
-44.3977299053872));
#241827=CARTESIAN_POINT('Ctrl Pts',(-45.7411894271921,-55.8800221740483,
-44.3670992021461));
#241828=CARTESIAN_POINT('Ctrl Pts',(-45.9361224564827,-56.0518538285405,
-44.352239789825));
#241829=CARTESIAN_POINT('Ctrl Pts',(-46.2510704556164,-56.4612376024201,
-44.3243888399465));
#241830=CARTESIAN_POINT('Ctrl Pts',(-46.3676190157825,-56.6952318620315,
-44.3117128692851));
#241831=CARTESIAN_POINT('Ctrl Pts',(-46.5064512434471,-57.1999321684089,
-44.2822720180798));
#241832=CARTESIAN_POINT('Ctrl Pts',(-46.5253299068317,-57.46624717571,-44.2667369759872));
#241833=CARTESIAN_POINT('Ctrl Pts',(-46.4596829413825,-57.9809243189306,
-44.2367141426327));
#241834=CARTESIAN_POINT('Ctrl Pts',(-46.3795996217551,-58.2249436443509,
-44.2224796819832));
#241835=CARTESIAN_POINT('Ctrl Pts',(-46.1270968753499,-58.6790315645635,
-44.1959912199709));
#241836=CARTESIAN_POINT('Ctrl Pts',(-45.9534990634237,-58.8828352001413,
-44.1815110087529));
#241837=CARTESIAN_POINT('Ctrl Pts',(-45.5399107234176,-59.2084496299062,
-44.1511202040175));
#241838=CARTESIAN_POINT('Ctrl Pts',(-45.3050125501161,-59.328266809786,
-44.1357589154571));
#241839=CARTESIAN_POINT('Ctrl Pts',(-44.8758366402836,-59.4500035041743,
-44.110527089502));
#241840=CARTESIAN_POINT('Ctrl Pts',(-44.6921881144964,-59.475452478349,
-44.1005072442478));
#241841=CARTESIAN_POINT('Ctrl Pts',(-44.5079524583202,-59.475452478349,
-44.0912000000001));
#241842=CARTESIAN_POINT('Origin',(-44.5079524583206,-57.475452478349,235.35105));
#241843=CARTESIAN_POINT('',(-44.5079524583205,-59.475452478349,-43.3912000000001));
#241844=CARTESIAN_POINT('',(-44.5079524583206,-59.475452478349,-43.5499499999999));
#241845=CARTESIAN_POINT('',(-44.5079524583206,-59.475452478349,235.35105));
#241846=CARTESIAN_POINT('Ctrl Pts',(-44.5079524583206,-59.475452478349,
-43.5499499999999));
#241847=CARTESIAN_POINT('Ctrl Pts',(-44.7411427905853,-59.475452478349,
-43.5617303438466));
#241848=CARTESIAN_POINT('Ctrl Pts',(-44.9727332695675,-59.4346746567168,
-43.5746192191985));
#241849=CARTESIAN_POINT('Ctrl Pts',(-45.4394749499459,-59.2647243400995,
-43.6031550289789));
#241850=CARTESIAN_POINT('Ctrl Pts',(-45.6665336475973,-59.1267917585162,
-43.6186486476269));
#241851=CARTESIAN_POINT('Ctrl Pts',(-46.0536883181991,-58.7714288945144,
-43.6485717349899));
#241852=CARTESIAN_POINT('Ctrl Pts',(-46.2101594603455,-58.5577253477594,
-43.6618174159511));
#241853=CARTESIAN_POINT('Ctrl Pts',(-46.4291739303611,-58.087523674963,
-43.6892458468642));
#241854=CARTESIAN_POINT('Ctrl Pts',(-46.4917176646714,-57.8365081053396,
-43.7038884217589));
#241855=CARTESIAN_POINT('Ctrl Pts',(-46.5191896482408,-57.3145417089397,
-43.734336461549));
#241856=CARTESIAN_POINT('Ctrl Pts',(-46.4799004743569,-57.0483527973918,
-43.7498641480559));
#241857=CARTESIAN_POINT('Ctrl Pts',(-46.3030962153959,-56.5575077643044,
-43.7784967749861));
#241858=CARTESIAN_POINT('Ctrl Pts',(-46.171433025635,-56.3361553339704,
-43.7908102082948));
#241859=CARTESIAN_POINT('Ctrl Pts',(-45.8292354738008,-55.9518183888728,
-43.8193072226185));
#241860=CARTESIAN_POINT('Ctrl Pts',(-45.6207697531512,-55.7935289585522,
-43.8344552999138));
#241861=CARTESIAN_POINT('Ctrl Pts',(-45.1498597268732,-55.5628001339988,
-43.864974393293));
#241862=CARTESIAN_POINT('Ctrl Pts',(-44.8909167319963,-55.4946276437662,
-43.8800440782737));
#241863=CARTESIAN_POINT('Ctrl Pts',(-44.3734087572596,-55.4639808994358,
-43.9070814863956));
#241864=CARTESIAN_POINT('Ctrl Pts',(-44.1200539898213,-55.4971445208707,
-43.9201785970292));
#241865=CARTESIAN_POINT('Ctrl Pts',(-43.6305221796573,-55.6591557814902,
-43.9496341661717));
#241866=CARTESIAN_POINT('Ctrl Pts',(-43.400109458794,-55.7897775013242,
-43.9650839903949));
#241867=CARTESIAN_POINT('Ctrl Pts',(-43.0009549861012,-56.1341461785003,
-43.99529262176));
#241868=CARTESIAN_POINT('Ctrl Pts',(-42.8368259016293,-56.3452184044869,
-44.0090196790247));
#241869=CARTESIAN_POINT('Ctrl Pts',(-42.6043594635739,-56.810843263918,
-44.0361811291582));
#241870=CARTESIAN_POINT('Ctrl Pts',(-42.5350891087905,-57.0593505250132,
-44.0506773860554));
#241871=CARTESIAN_POINT('Ctrl Pts',(-42.4930428685444,-57.578876428523,
-44.0809830637601));
#241872=CARTESIAN_POINT('Ctrl Pts',(-42.5245722780062,-57.8452915051078,
-44.0965239432275));
#241873=CARTESIAN_POINT('Ctrl Pts',(-42.687043176314,-58.341520393353,-44.1254706283751));
#241874=CARTESIAN_POINT('Ctrl Pts',(-42.812967013659,-58.5676091816501,
-44.137843710689));
#241875=CARTESIAN_POINT('Ctrl Pts',(-43.1447772426943,-58.9616010236369,
-44.1660975778558));
#241876=CARTESIAN_POINT('Ctrl Pts',(-43.3481527596839,-59.1252173029631,
-44.1811438739157));
#241877=CARTESIAN_POINT('Ctrl Pts',(-43.8116818273377,-59.3689977237109,
-44.2116707664864));
#241878=CARTESIAN_POINT('Ctrl Pts',(-44.0686112146914,-59.4445451620155,
-44.2268538303952));
#241879=CARTESIAN_POINT('Ctrl Pts',(-44.3911492849965,-59.4728971911007,
-44.2439747907269));
#241880=CARTESIAN_POINT('Ctrl Pts',(-44.4495810412991,-59.475452478349,
-44.2470011840835));
#241881=CARTESIAN_POINT('Ctrl Pts',(-44.5079524583202,-59.475452478349,
-44.2499499999999));
#241882=CARTESIAN_POINT('Ctrl Pts',(-44.5079524583202,-59.475452478349,
-44.0912000000001));
#241883=CARTESIAN_POINT('Ctrl Pts',(-44.4396380533254,-59.475452478349,
-44.0877488827402));
#241884=CARTESIAN_POINT('Ctrl Pts',(-44.3712532747759,-59.4719525857611,
-44.0841921301382));
#241885=CARTESIAN_POINT('Ctrl Pts',(-44.0392127721053,-59.4377567333654,
-44.0664206796701));
#241886=CARTESIAN_POINT('Ctrl Pts',(-43.78342468228,-59.3583694715361,-44.0511832771466));
#241887=CARTESIAN_POINT('Ctrl Pts',(-43.3239077102798,-59.1078447978339,
-44.0206623608423));
#241888=CARTESIAN_POINT('Ctrl Pts',(-43.1232518957464,-58.941500918052,
-44.0056739041018));
#241889=CARTESIAN_POINT('Ctrl Pts',(-42.7969185541133,-58.5424711832971,
-43.9775497806073));
#241890=CARTESIAN_POINT('Ctrl Pts',(-42.6740307994288,-58.3138450434982,
-43.9651062329672));
#241891=CARTESIAN_POINT('Ctrl Pts',(-42.5191875880454,-57.8148255859975,
-43.935996764613));
#241892=CARTESIAN_POINT('Ctrl Pts',(-42.4917621021746,-57.5483791414746,
-43.9204540553491));
#241893=CARTESIAN_POINT('Ctrl Pts',(-42.5414862336479,-57.0303076934156,
-43.890233220879));
#241894=CARTESIAN_POINT('Ctrl Pts',(-42.6142852507321,-56.7832020438742,
-43.8758187246558));
#241895=CARTESIAN_POINT('Ctrl Pts',(-42.8539010143348,-56.3200531443656,
-43.8488017055177));
#241896=CARTESIAN_POINT('Ctrl Pts',(-43.0221771847699,-56.110399183978,
-43.8347778949015));
#241897=CARTESIAN_POINT('Ctrl Pts',(-43.4277210247951,-55.7720161446635,
-43.8044210656325));
#241898=CARTESIAN_POINT('Ctrl Pts',(-43.6598371235613,-55.6453432575024,
-43.7890003641977));
#241899=CARTESIAN_POINT('Ctrl Pts',(-44.1514596426019,-55.4912474024193,
-43.7596700423083));
#241900=CARTESIAN_POINT('Ctrl Pts',(-44.4052893349927,-55.4621018207231,
-43.746775745096));
#241901=CARTESIAN_POINT('Ctrl Pts',(-44.9222678148284,-55.5009444674812,
-43.7195260389219));
#241902=CARTESIAN_POINT('Ctrl Pts',(-45.1801192875519,-55.5732199621532,
-43.7043918246567));
#241903=CARTESIAN_POINT('Ctrl Pts',(-45.6469753039607,-55.8112258285714,
-43.6738652852958));
#241904=CARTESIAN_POINT('Ctrl Pts',(-45.8526306051278,-55.9724930517351,
-43.6587723328983));
#241905=CARTESIAN_POINT('Ctrl Pts',(-46.1890690927262,-56.3621980191077,
-43.6304096885208));
#241906=CARTESIAN_POINT('Ctrl Pts',(-46.3175540210956,-56.5861655594622,
-43.6180750702683));
#241907=CARTESIAN_POINT('Ctrl Pts',(-46.4864333897417,-57.0800086426784,
-43.5892675570807));
#241908=CARTESIAN_POINT('Ctrl Pts',(-46.5214251156315,-57.3463497448326,
-43.5737309927884));
#241909=CARTESIAN_POINT('Ctrl Pts',(-46.4858725815761,-57.8670145459856,
-43.5433588793878));
#241910=CARTESIAN_POINT('Ctrl Pts',(-46.4195947636065,-58.1166638901354,
-43.5287960009791));
#241911=CARTESIAN_POINT('Ctrl Pts',(-46.193140237254,-58.5843473292451,
-43.5015144670311));
#241912=CARTESIAN_POINT('Ctrl Pts',(-46.0324568770958,-58.7966008445079,
-43.4880149800194));
#241913=CARTESIAN_POINT('Ctrl Pts',(-45.6386695182338,-59.1459257410061,
-43.4579329289112));
#241914=CARTESIAN_POINT('Ctrl Pts',(-45.4097322015845,-59.2798344543604,
-43.442461768733));
#241915=CARTESIAN_POINT('Ctrl Pts',(-44.9510044081974,-59.4384338924148,
-43.4146618729776));
#241916=CARTESIAN_POINT('Ctrl Pts',(-44.7301421454,-59.475452478349,-43.4024246116192));
#241917=CARTESIAN_POINT('Ctrl Pts',(-44.5079524583205,-59.475452478349,
-43.3912000000001));
#241918=CARTESIAN_POINT('Origin',(-44.5079524583206,-57.475452478349,235.35105));
#241919=CARTESIAN_POINT('',(-44.5079524583206,-59.475452478349,-42.6912000000002));
#241920=CARTESIAN_POINT('',(-44.5079524583206,-59.475452478349,-42.8499499999999));
#241921=CARTESIAN_POINT('',(-44.5079524583206,-59.475452478349,235.35105));
#241922=CARTESIAN_POINT('Ctrl Pts',(-44.5079524583206,-59.475452478349,
-42.8499499999999));
#241923=CARTESIAN_POINT('Ctrl Pts',(-44.5276346988284,-59.475452478349,
-42.8509443103497));
#241924=CARTESIAN_POINT('Ctrl Pts',(-44.5473281463706,-59.4751619365887,
-42.8519476609929));
#241925=CARTESIAN_POINT('Ctrl Pts',(-44.8218121533896,-59.4670509640143,
-42.8660506548686));
#241926=CARTESIAN_POINT('Ctrl Pts',(-45.0727776159488,-59.410885272387,
-42.8803671313939));
#241927=CARTESIAN_POINT('Ctrl Pts',(-45.5491409754711,-59.2034632813881,
-42.9104819344268));
#241928=CARTESIAN_POINT('Ctrl Pts',(-45.7685085447205,-59.0506058229546,
-42.9260223204158));
#241929=CARTESIAN_POINT('Ctrl Pts',(-46.1304126464785,-58.6730704055913,
-42.9553164952639));
#241930=CARTESIAN_POINT('Ctrl Pts',(-46.2712780829291,-58.4538901331987,
-42.9678744701338));
#241931=CARTESIAN_POINT('Ctrl Pts',(-46.4618157928791,-57.9743456480368,
-42.9958478984349));
#241932=CARTESIAN_POINT('Ctrl Pts',(-46.5097830405982,-57.7186009486152,
-43.0107663392346));
#241933=CARTESIAN_POINT('Ctrl Pts',(-46.5059607988654,-57.1956479648935,
-43.0412719299517));
#241934=CARTESIAN_POINT('Ctrl Pts',(-46.4512970185361,-56.9334422805496,
-43.0565672615384));
#241935=CARTESIAN_POINT('Ctrl Pts',(-46.2473694361858,-56.4562447360175,
-43.0844037849695));
#241936=CARTESIAN_POINT('Ctrl Pts',(-46.1042283225714,-56.244081623675,
-43.0968907486846));
#241937=CARTESIAN_POINT('Ctrl Pts',(-45.7412219755972,-55.8795061147239,
-43.1258626095916));
#241938=CARTESIAN_POINT('Ctrl Pts',(-45.5228641533644,-55.7324834035986,
-43.1411818049009));
#241939=CARTESIAN_POINT('Ctrl Pts',(-45.038137520016,-55.5288830734955,
-43.1716076399338));
#241940=CARTESIAN_POINT('Ctrl Pts',(-44.7757837472277,-55.4758154631358,
-43.1864090721034));
#241941=CARTESIAN_POINT('Ctrl Pts',(-44.256718078785,-55.4751083907211,
-43.2126519315965));
#241942=CARTESIAN_POINT('Ctrl Pts',(-44.0048826118991,-55.5231388650409,
-43.2267550101799));
#241943=CARTESIAN_POINT('Ctrl Pts',(-43.5234974835783,-55.7146320702014,
-43.256658914088));
#241944=CARTESIAN_POINT('Ctrl Pts',(-43.2999967969317,-55.859750680214,
-43.2721823811033));
#241945=CARTESIAN_POINT('Ctrl Pts',(-42.9248666517407,-56.2258268948668,
-43.3018104844325));
#241946=CARTESIAN_POINT('Ctrl Pts',(-42.7759085245037,-56.4421417661968,
-43.3146735417911));
#241947=CARTESIAN_POINT('Ctrl Pts',(-42.5704203330931,-56.9168393697716,
-43.342364235333));
#241948=CARTESIAN_POINT('Ctrl Pts',(-42.514747104781,-57.1702018246777,
-43.3571437118691));
#241949=CARTESIAN_POINT('Ctrl Pts',(-42.5020797657798,-57.694224253965,
-43.3877116869108));
#241950=CARTESIAN_POINT('Ctrl Pts',(-42.5492113844385,-57.9599632971108,
-43.4032131310943));
#241951=CARTESIAN_POINT('Ctrl Pts',(-42.7404045078387,-58.4452239052171,
-43.4315199999005));
#241952=CARTESIAN_POINT('Ctrl Pts',(-42.8778864535938,-58.6618649124905,
-43.4438724460826));
#241953=CARTESIAN_POINT('Ctrl Pts',(-43.2306386228494,-59.0362522793755,
-43.4726124641059));
#241954=CARTESIAN_POINT('Ctrl Pts',(-43.4441758847969,-59.1889255509586,
-43.487852941648));
#241955=CARTESIAN_POINT('Ctrl Pts',(-43.9222617083629,-59.406054454791,
-43.5183378786663));
#241956=CARTESIAN_POINT('Ctrl Pts',(-44.1830410702355,-59.4666177912531,
-43.533278399856));
#241957=CARTESIAN_POINT('Ctrl Pts',(-44.4680414873419,-59.4751539757667,
-43.5479250653137));
#241958=CARTESIAN_POINT('Ctrl Pts',(-44.4880023952141,-59.475452478349,
-43.5489421597482));
#241959=CARTESIAN_POINT('Ctrl Pts',(-44.5079524583206,-59.475452478349,
-43.5499499999999));
#241960=CARTESIAN_POINT('Ctrl Pts',(-44.5079524583205,-59.475452478349,
-43.3912000000001));
#241961=CARTESIAN_POINT('Ctrl Pts',(-44.4773116517654,-59.475452478349,
-43.3896520831827));
#241962=CARTESIAN_POINT('Ctrl Pts',(-44.4466476465931,-59.4747483419293,
-43.388082457102));
#241963=CARTESIAN_POINT('Ctrl Pts',(-44.1510871580738,-59.4611428803614,
-43.3727544624739));
#241964=CARTESIAN_POINT('Ctrl Pts',(-43.8912890391863,-59.3963894216387,
-43.3577412999638));
#241965=CARTESIAN_POINT('Ctrl Pts',(-43.4171000214185,-59.171754753365,
-43.3272343042302));
#241966=CARTESIAN_POINT('Ctrl Pts',(-43.206333079655,-59.0159738242197,
-43.3120431381224));
#241967=CARTESIAN_POINT('Ctrl Pts',(-42.8593735673371,-58.636107456305,
-43.2834359502061));
#241968=CARTESIAN_POINT('Ctrl Pts',(-42.7250850178345,-58.4168938658302,
-43.2711174142699));
#241969=CARTESIAN_POINT('Ctrl Pts',(-42.541767545564,-57.9285541339348,
-43.2426309299094));
#241970=CARTESIAN_POINT('Ctrl Pts',(-42.4989342989933,-57.6625409902181,
-43.2271134965259));
#241971=CARTESIAN_POINT('Ctrl Pts',(-42.5197252561373,-57.1395943993428,
-43.1966082787248));
#241972=CARTESIAN_POINT('Ctrl Pts',(-42.5791731179057,-56.8874948444075,
-43.1819024713535));
#241973=CARTESIAN_POINT('Ctrl Pts',(-42.7920676850265,-56.4152459138284,
-43.1543546170697));
#241974=CARTESIAN_POINT('Ctrl Pts',(-42.9451166578166,-56.2003575940057,
-43.1412946370089));
#241975=CARTESIAN_POINT('Ctrl Pts',(-43.3268248912264,-55.8401059161665,
-43.1115041031655));
#241976=CARTESIAN_POINT('Ctrl Pts',(-43.5522960392943,-55.6989009570075,
-43.0959952402373));
#241977=CARTESIAN_POINT('Ctrl Pts',(-44.0359589670054,-55.5154402389995,
-43.0662105469964));
#241978=CARTESIAN_POINT('Ctrl Pts',(-44.2881710172024,-55.4714487340392,
-43.0524197273675));
#241979=CARTESIAN_POINT('Ctrl Pts',(-44.8068735603992,-55.4802226785142,
-43.025959928521));
#241980=CARTESIAN_POINT('Ctrl Pts',(-45.0683980446005,-55.5373746737467,
-43.0110812625833));
#241981=CARTESIAN_POINT('Ctrl Pts',(-45.5495583476536,-55.7483627495522,
-42.9806201160377));
#241982=CARTESIAN_POINT('Ctrl Pts',(-45.7653108529225,-55.8984789018917,
-42.965342311149));
#241983=CARTESIAN_POINT('Ctrl Pts',(-46.12274617044,-56.2684033051083,-42.9364958789197));
#241984=CARTESIAN_POINT('Ctrl Pts',(-46.2628111744314,-56.4829873890269,
-42.924093796877));
#241985=CARTESIAN_POINT('Ctrl Pts',(-46.4603340143122,-56.9657343748614,
-42.8959335560367));
#241986=CARTESIAN_POINT('Ctrl Pts',(-46.5109291662741,-57.2312039689145,
-42.880447829717));
#241987=CARTESIAN_POINT('Ctrl Pts',(-46.5048240924326,-57.7560032140316,
-42.8498345404185));
#241988=CARTESIAN_POINT('Ctrl Pts',(-46.4522081901623,-58.0103419850332,
-42.8349981121101));
#241989=CARTESIAN_POINT('Ctrl Pts',(-46.2526774483189,-58.4869863285353,
-42.8071938587392));
#241990=CARTESIAN_POINT('Ctrl Pts',(-46.1069702144933,-58.7044445518999,
-42.7944671477351));
#241991=CARTESIAN_POINT('Ctrl Pts',(-45.7371193706181,-59.0751341683654,
-42.7649711873811));
#241992=CARTESIAN_POINT('Ctrl Pts',(-45.5152413641435,-59.2233627999929,
-42.7494389862001));
#241993=CARTESIAN_POINT('Ctrl Pts',(-45.0358906779062,-59.4212091256449,
-42.7194525591918));
#241994=CARTESIAN_POINT('Ctrl Pts',(-44.7843816793554,-59.4725307487516,
-42.7052499095664));
#241995=CARTESIAN_POINT('Ctrl Pts',(-44.5226272522411,-59.4754121097202,
-42.6919425208378));
#241996=CARTESIAN_POINT('Ctrl Pts',(-44.5152890012201,-59.475452478349,
-42.6915706285642));
#241997=CARTESIAN_POINT('Ctrl Pts',(-44.5079524583206,-59.475452478349,
-42.6912000000002));
#241998=CARTESIAN_POINT('Origin',(-44.5079524583206,-57.475452478349,235.35105));
#241999=CARTESIAN_POINT('',(-44.5079524583208,-59.475452478349,-41.9912000000002));
#242000=CARTESIAN_POINT('',(-44.5079524583208,-59.475452478349,-42.1499499999999));
#242001=CARTESIAN_POINT('',(-44.5079524583206,-59.475452478349,235.35105));
#242002=CARTESIAN_POINT('Ctrl Pts',(-44.507952458321,-59.475452478349,-42.1499499999999));
#242003=CARTESIAN_POINT('Ctrl Pts',(-44.5650747796958,-59.475452478349,
-42.1528357139169));
#242004=CARTESIAN_POINT('Ctrl Pts',(-44.6222599632747,-59.4730053748643,
-42.1557959773676));
#242005=CARTESIAN_POINT('Ctrl Pts',(-44.9347278022592,-59.4461278479024,
-42.1723652019455));
#242006=CARTESIAN_POINT('Ctrl Pts',(-45.1834747757773,-59.3752762646862,
-42.1869979430166));
#242007=CARTESIAN_POINT('Ctrl Pts',(-45.649619547893,-59.1390434386582,
-42.2174368379546));
#242008=CARTESIAN_POINT('Ctrl Pts',(-45.8607911058115,-58.9723798878383,
-42.2329658543202));
#242009=CARTESIAN_POINT('Ctrl Pts',(-46.1982987190847,-58.5745118910737,
-42.2616205973047));
#242010=CARTESIAN_POINT('Ctrl Pts',(-46.3246473098617,-58.3499943901759,
-42.2739350551434));
#242011=CARTESIAN_POINT('Ctrl Pts',(-46.4873433377963,-57.8617628708698,
-42.302415227103));
#242012=CARTESIAN_POINT('Ctrl Pts',(-46.5206965595169,-57.6021973631596,
-42.3175565483861));
#242013=CARTESIAN_POINT('Ctrl Pts',(-46.4861088430538,-57.0789894607449,
-42.3480770093603));
#242014=CARTESIAN_POINT('Ctrl Pts',(-46.4161921970786,-56.820508868563,
-42.3631550439043));
#242015=CARTESIAN_POINT('Ctrl Pts',(-46.1849060981301,-56.3565494080106,
-42.3902193457699));
#242016=CARTESIAN_POINT('Ctrl Pts',(-46.0299185779906,-56.1534150975443,
-42.4032891797458));
#242017=CARTESIAN_POINT('Ctrl Pts',(-45.6455808442644,-55.8097419487664,
-42.4327290106458));
#242018=CARTESIAN_POINT('Ctrl Pts',(-45.4175748781868,-55.675070498779,
-42.4481753672027));
#242019=CARTESIAN_POINT('Ctrl Pts',(-44.9200132742906,-55.500498582363,
-42.4784029391186));
#242020=CARTESIAN_POINT('Ctrl Pts',(-44.6550483564574,-55.4633522733737,
-42.4921660649213));
#242021=CARTESIAN_POINT('Ctrl Pts',(-44.1353892897578,-55.4939013682113,
-42.5193092941163));
#242022=CARTESIAN_POINT('Ctrl Pts',(-43.8854675233247,-55.5576883309377,
-42.5337953321194));
#242023=CARTESIAN_POINT('Ctrl Pts',(-43.4141880609877,-55.7801031930307,
-42.5640905981526));
#242024=CARTESIAN_POINT('Ctrl Pts',(-43.1989634690461,-55.9401681677463,
-42.5796319078233));
#242025=CARTESIAN_POINT('Ctrl Pts',(-42.8496595906262,-56.328327415621,
-42.6085994044402));
#242026=CARTESIAN_POINT('Ctrl Pts',(-42.7163521133916,-56.5502515671372,
-42.620979946846));
#242027=CARTESIAN_POINT('Ctrl Pts',(-42.5401456495728,-57.0343218554623,
-42.6492173803316));
#242028=CARTESIAN_POINT('Ctrl Pts',(-42.4996622819459,-57.2921349904168,
-42.6642564798706));
#242029=CARTESIAN_POINT('Ctrl Pts',(-42.5193067596286,-57.8154466839436,
-42.6947829953263));
#242030=CARTESIAN_POINT('Ctrl Pts',(-42.5818499425991,-58.0758497743081,
-42.7099731755975));
#242031=CARTESIAN_POINT('Ctrl Pts',(-42.7999012454534,-58.5463029491167,
-42.7374162774613));
#242032=CARTESIAN_POINT('Ctrl Pts',(-42.9490964919264,-58.7537934143169,
-42.7501510933475));
#242033=CARTESIAN_POINT('Ctrl Pts',(-43.3230349053399,-59.107742718469,
-42.7793652910375));
#242034=CARTESIAN_POINT('Ctrl Pts',(-43.5464048897313,-59.2485347493895,
-42.7947559633267));
#242035=CARTESIAN_POINT('Ctrl Pts',(-44.019696696047,-59.4304161605894,
-42.8239706636009));
#242036=CARTESIAN_POINT('Ctrl Pts',(-44.2628906747684,-59.475452478349,
-42.8375699324134));
#242037=CARTESIAN_POINT('Ctrl Pts',(-44.5079524583206,-59.475452478349,
-42.8499499999999));
#242038=CARTESIAN_POINT('Ctrl Pts',(-44.5079524583206,-59.475452478349,
-42.6912000000002));
#242039=CARTESIAN_POINT('Ctrl Pts',(-44.2504290540854,-59.475452478349,
-42.6781903944089));
#242040=CARTESIAN_POINT('Ctrl Pts',(-43.9951550570802,-59.4257145549608,
-42.663843735274));
#242041=CARTESIAN_POINT('Ctrl Pts',(-43.514305376544,-59.2306775940827,
-42.6338635216549));
#242042=CARTESIAN_POINT('Ctrl Pts',(-43.2939194442701,-59.0861303300434,
-42.6185140705213));
#242043=CARTESIAN_POINT('Ctrl Pts',(-42.9265253044388,-58.7257988038404,
-42.5894443292731));
#242044=CARTESIAN_POINT('Ctrl Pts',(-42.7809576370071,-58.5155232546435,
-42.576870795284));
#242045=CARTESIAN_POINT('Ctrl Pts',(-42.5713346547531,-58.0410220017098,
-42.5491915555295));
#242046=CARTESIAN_POINT('Ctrl Pts',(-42.5134931808606,-57.7795123493802,
-42.5339368258103));
#242047=CARTESIAN_POINT('Ctrl Pts',(-42.5033078965441,-57.2563570745263,
-42.5034194347771));
#242048=CARTESIAN_POINT('Ctrl Pts',(-42.5482735346596,-56.9997541785442,
-42.4884509325115));
#242049=CARTESIAN_POINT('Ctrl Pts',(-42.7330429464916,-56.5183738869157,
-42.4603704154998));
#242050=CARTESIAN_POINT('Ctrl Pts',(-42.8708433909339,-56.298089817614,
-42.4478973081275));
#242051=CARTESIAN_POINT('Ctrl Pts',(-43.2276659902567,-55.9162367588301,
-42.4187339101662));
#242052=CARTESIAN_POINT('Ctrl Pts',(-43.4453863688403,-55.7604529601252,
-42.4031913856087));
#242053=CARTESIAN_POINT('Ctrl Pts',(-43.9197500928027,-55.5469560070576,
-42.3730004140684));
#242054=CARTESIAN_POINT('Ctrl Pts',(-44.1703212412459,-55.4877077061276,
-42.3586139481242));
#242055=CARTESIAN_POINT('Ctrl Pts',(-44.6917016753155,-55.4661419405827,
-42.3316457724076));
#242056=CARTESIAN_POINT('Ctrl Pts',(-44.9576917709601,-55.5085012155312,
-42.3175160810923));
#242057=CARTESIAN_POINT('Ctrl Pts',(-45.4528258682846,-55.6933931606017,
-42.2871101414782));
#242058=CARTESIAN_POINT('Ctrl Pts',(-45.677709936842,-55.8322258902904,
-42.2717001267461));
#242059=CARTESIAN_POINT('Ctrl Pts',(-46.0550120706384,-56.1828697013188,
-42.2424124103462));
#242060=CARTESIAN_POINT('Ctrl Pts',(-46.2060766973967,-56.3889421190976,
-42.2295797709562));
#242061=CARTESIAN_POINT('Ctrl Pts',(-46.4284298403303,-56.8573027972508,
-42.2022587313973));
#242062=CARTESIAN_POINT('Ctrl Pts',(-46.4933714527608,-57.1171058003779,
-42.1871035562149));
#242063=CARTESIAN_POINT('Ctrl Pts',(-46.5178619269603,-57.6404308900813,
-42.1565762593156));
#242064=CARTESIAN_POINT('Ctrl Pts',(-46.4796841978071,-57.8988337075529,
-42.1415027616298));
#242065=CARTESIAN_POINT('Ctrl Pts',(-46.3078606964485,-58.3842645324407,
-42.1131859635114));
#242066=CARTESIAN_POINT('Ctrl Pts',(-46.1768272466949,-58.6070297692475,
-42.1008374601594));
#242067=CARTESIAN_POINT('Ctrl Pts',(-45.8313597047937,-58.9983700010671,
-42.0719709894624));
#242068=CARTESIAN_POINT('Ctrl Pts',(-45.617434952966,-59.1605967201461,
-42.0564322944304));
#242069=CARTESIAN_POINT('Ctrl Pts',(-45.1477860234778,-59.3875285888647,
-42.0260876538713));
#242070=CARTESIAN_POINT('Ctrl Pts',(-44.8982255564231,-59.4536206016677,
-42.0115526374167));
#242071=CARTESIAN_POINT('Ctrl Pts',(-44.5979575875366,-59.4739351411411,
-41.9957911481571));
#242072=CARTESIAN_POINT('Ctrl Pts',(-44.5529321463451,-59.475452478349,
-41.9934722905617));
#242073=CARTESIAN_POINT('Ctrl Pts',(-44.5079524583209,-59.475452478349,
-41.9912000000002));
#242074=CARTESIAN_POINT('Origin',(-44.5079524583206,-57.475452478349,235.35105));
#242075=CARTESIAN_POINT('',(-44.5079524583208,-59.475452478349,-41.2912000000002));
#242076=CARTESIAN_POINT('',(-44.5079524583207,-59.475452478349,-41.4499499999999));
#242077=CARTESIAN_POINT('',(-44.5079524583206,-59.475452478349,235.35105));
#242078=CARTESIAN_POINT('Ctrl Pts',(-44.5079524583208,-59.475452478349,
-41.4499499999999));
#242079=CARTESIAN_POINT('Ctrl Pts',(-44.6009259794205,-59.475452478349,
-41.4546468501504));
#242080=CARTESIAN_POINT('Ctrl Pts',(-44.6939771241189,-59.4689702732022,
-41.4595366860181));
#242081=CARTESIAN_POINT('Ctrl Pts',(-45.0416143584034,-59.4200877927684,
-41.4785244144753));
#242082=CARTESIAN_POINT('Ctrl Pts',(-45.2874346307486,-59.3352317064797,
-41.4934177686947));
#242083=CARTESIAN_POINT('Ctrl Pts',(-45.7421834212317,-59.0718365676755,
-41.5240731938623));
#242084=CARTESIAN_POINT('Ctrl Pts',(-45.9447065234524,-58.8923298930035,
-41.5395398973705));
#242085=CARTESIAN_POINT('Ctrl Pts',(-46.2584426863796,-58.4755311426912,
-41.5675458976735));
#242086=CARTESIAN_POINT('Ctrl Pts',(-46.3710572059469,-58.2456657066199,
-41.5800208950175));
#242087=CARTESIAN_POINT('Ctrl Pts',(-46.5062012038549,-57.749268837484,
-41.6089773790505));
#242088=CARTESIAN_POINT('Ctrl Pts',(-46.5248397171714,-57.4867383743764,
-41.6242916560651));
#242089=CARTESIAN_POINT('Ctrl Pts',(-46.4598083536196,-56.9650709933012,
-41.6547222532945));
#242090=CARTESIAN_POINT('Ctrl Pts',(-46.37507561606,-56.7111654338419,-41.6695334109297));
#242091=CARTESIAN_POINT('Ctrl Pts',(-46.1170385297601,-56.2608270119092,
-41.6958031522091));
#242092=CARTESIAN_POINT('Ctrl Pts',(-45.9499355131943,-56.0664572462705,
-41.7098660467572));
#242093=CARTESIAN_POINT('Ctrl Pts',(-45.5441242268398,-55.7445682618479,
-41.7397553103185));
#242094=CARTESIAN_POINT('Ctrl Pts',(-45.3069921100196,-55.6231143727148,
-41.7552771909227));
#242095=CARTESIAN_POINT('Ctrl Pts',(-44.8026094104671,-55.4802147431357,
-41.7849255769294));
#242096=CARTESIAN_POINT('Ctrl Pts',(-44.5406967898439,-55.4588449667596,
-41.7978114312412));
#242097=CARTESIAN_POINT('Ctrl Pts',(-44.0266545219183,-55.5172882033606,
-41.8254844892962));
#242098=CARTESIAN_POINT('Ctrl Pts',(-43.779297689101,-55.5952707848365,
-41.8402549904821));
#242099=CARTESIAN_POINT('Ctrl Pts',(-43.3187518271973,-55.8453728770303,
-41.8708155591053));
#242100=CARTESIAN_POINT('Ctrl Pts',(-43.1118811272099,-56.0186157977966,
-41.8863192023811));
#242101=CARTESIAN_POINT('Ctrl Pts',(-42.7864074243799,-56.4261702229759,
-41.9146485353188));
#242102=CARTESIAN_POINT('Ctrl Pts',(-42.6670571871209,-56.6533685443121,
-41.9269951038478));
#242103=CARTESIAN_POINT('Ctrl Pts',(-42.5182510384644,-57.1457723700787,
-41.9557186603508));
#242104=CARTESIAN_POINT('Ctrl Pts',(-42.4922913340079,-57.406935701447,
-41.970953188014));
#242105=CARTESIAN_POINT('Ctrl Pts',(-42.5422415623305,-57.9295892736244,
-42.0014413130576));
#242106=CARTESIAN_POINT('Ctrl Pts',(-42.6196693330092,-58.1858714881189,
-42.0163911089031));
#242107=CARTESIAN_POINT('Ctrl Pts',(-42.864481736838,-58.6430250877798,
-42.0430584022166));
#242108=CARTESIAN_POINT('Ctrl Pts',(-43.0255226079038,-58.8417235688324,
-42.0565766287346));
#242109=CARTESIAN_POINT('Ctrl Pts',(-43.4206431894206,-59.1745575448617,
-42.0862450466026));
#242110=CARTESIAN_POINT('Ctrl Pts',(-43.6533100929671,-59.3026879263632,
-42.1017360839267));
#242111=CARTESIAN_POINT('Ctrl Pts',(-44.0997626031168,-59.4440829473174,
-42.1284140596013));
#242112=CARTESIAN_POINT('Ctrl Pts',(-44.3034083695787,-59.4754524783491,
-42.1396168113389));
#242113=CARTESIAN_POINT('Ctrl Pts',(-44.507952458321,-59.475452478349,-42.1499499999999));
#242114=CARTESIAN_POINT('Ctrl Pts',(-44.5079524583209,-59.475452478349,
-41.9912000000002));
#242115=CARTESIAN_POINT('Ctrl Pts',(-44.2895268033131,-59.4754524783491,
-41.9801655403125));
#242116=CARTESIAN_POINT('Ctrl Pts',(-44.072284646167,-59.4396792295317,
-41.9681474823218));
#242117=CARTESIAN_POINT('Ctrl Pts',(-43.6162554978214,-59.2848170542454,
-41.9405929206148));
#242118=CARTESIAN_POINT('Ctrl Pts',(-43.3867023861031,-59.1522714670058,
-41.9251304094548));
#242119=CARTESIAN_POINT('Ctrl Pts',(-42.9988245054448,-58.8121357155321,
-41.8956149109742));
#242120=CARTESIAN_POINT('Ctrl Pts',(-42.8418555471031,-58.6104662814462,
-41.8824091385142));
#242121=CARTESIAN_POINT('Ctrl Pts',(-42.6061070337851,-58.1487334399722,
-41.8554747227616));
#242122=CARTESIAN_POINT('Ctrl Pts',(-42.5337089287158,-57.8909520345353,
-41.8404374741111));
#242123=CARTESIAN_POINT('Ctrl Pts',(-42.494061758467,-57.3678765695541,
-41.8099247386538));
#242124=CARTESIAN_POINT('Ctrl Pts',(-42.5249871347537,-57.1077620134154,
-41.7947513895457));
#242125=CARTESIAN_POINT('Ctrl Pts',(-42.6831101613391,-56.6181443811625,
-41.7661903609976));
#242126=CARTESIAN_POINT('Ctrl Pts',(-42.8071371501217,-56.3927472221573,
-41.7538764704305));
#242127=CARTESIAN_POINT('Ctrl Pts',(-43.1406720840627,-55.991657246832,
-41.725328445476));
#242128=CARTESIAN_POINT('Ctrl Pts',(-43.3504418669979,-55.8228043071185,
-41.7098063870112));
#242129=CARTESIAN_POINT('Ctrl Pts',(-43.8147777661047,-55.5819666242096,
-41.6793245646629));
#242130=CARTESIAN_POINT('Ctrl Pts',(-44.0630869185102,-55.5087519276968,
-41.664645017366));
#242131=CARTESIAN_POINT('Ctrl Pts',(-44.5790557803663,-55.4596501846947,
-41.6371470915826));
#242132=CARTESIAN_POINT('Ctrl Pts',(-44.8419646313228,-55.4862372264034,
-41.6240117682738));
#242133=CARTESIAN_POINT('Ctrl Pts',(-45.3441791046204,-55.6396783934614,
-41.5941654555332));
#242134=CARTESIAN_POINT('Ctrl Pts',(-45.5783520708578,-55.7656042547414,
-41.5786626332168));
#242135=CARTESIAN_POINT('Ctrl Pts',(-45.9770361819292,-56.0948126302783,
-41.5489199391143));
#242136=CARTESIAN_POINT('Ctrl Pts',(-46.1400904248351,-56.2920612198681,
-41.5352311567446));
#242137=CARTESIAN_POINT('Ctrl Pts',(-46.3893309714318,-56.7469503676705,
-41.5086959564562));
#242138=CARTESIAN_POINT('Ctrl Pts',(-46.4692097135499,-57.0024617306042,
-41.4937911269517));
#242139=CARTESIAN_POINT('Ctrl Pts',(-46.5242043250541,-57.5248342425204,
-41.46331939709));
#242140=CARTESIAN_POINT('Ctrl Pts',(-46.5006864397953,-57.7864771094481,
-41.4480568965192));
#242141=CARTESIAN_POINT('Ctrl Pts',(-46.3564458786342,-58.2802276366138,
-41.4192547824346));
#242142=CARTESIAN_POINT('Ctrl Pts',(-46.2393622733395,-58.5083135685649,
-41.4068758364452));
#242143=CARTESIAN_POINT('Ctrl Pts',(-45.9178222925651,-58.9189878596702,
-41.3786542317732));
#242144=CARTESIAN_POINT('Ctrl Pts',(-45.7123922578584,-59.0943471035571,
-41.3631616421491));
#242145=CARTESIAN_POINT('Ctrl Pts',(-45.2537529527428,-59.3489305525486,
-41.332566683005));
#242146=CARTESIAN_POINT('Ctrl Pts',(-45.0068914917131,-59.4292260382104,
-41.3177537473793));
#242147=CARTESIAN_POINT('Ctrl Pts',(-44.6705784160196,-59.4704991177613,
-41.2995600353072));
#242148=CARTESIAN_POINT('Ctrl Pts',(-44.5892245188092,-59.475452478349,
-41.2953057140252));
#242149=CARTESIAN_POINT('Ctrl Pts',(-44.5079524583209,-59.475452478349,
-41.2912000000002));
#242150=CARTESIAN_POINT('Origin',(-44.5079524583206,-57.475452478349,235.35105));
#242151=CARTESIAN_POINT('',(-44.5079524583206,-59.475452478349,-40.5912000000001));
#242152=CARTESIAN_POINT('',(-44.5079524583206,-59.475452478349,-40.7499499999999));
#242153=CARTESIAN_POINT('',(-44.5079524583206,-59.475452478349,235.35105));
#242154=CARTESIAN_POINT('Ctrl Pts',(-44.5079524583206,-59.475452478349,
-40.7499499999999));
#242155=CARTESIAN_POINT('Ctrl Pts',(-44.6385960929674,-59.475452478349,
-40.7565498745426));
#242156=CARTESIAN_POINT('Ctrl Pts',(-44.769204040552,-59.4626545153701,
-40.7635212201612));
#242157=CARTESIAN_POINT('Ctrl Pts',(-45.1520824190208,-59.3865372026326,
-40.785083615251));
#242158=CARTESIAN_POINT('Ctrl Pts',(-45.3939906952831,-59.2870988818203,
-40.8002046578447));
#242159=CARTESIAN_POINT('Ctrl Pts',(-45.8314081075506,-58.9981985528729,
-40.8307284352522));
#242160=CARTESIAN_POINT('Ctrl Pts',(-46.0214237092286,-58.8095209785697,
-40.8458307675625));
#242161=CARTESIAN_POINT('Ctrl Pts',(-46.3101271098484,-58.37893535582,-40.8729742761734));
#242162=CARTESIAN_POINT('Ctrl Pts',(-46.4099370609394,-58.1437421486912,
-40.8859664358967));
#242163=CARTESIAN_POINT('Ctrl Pts',(-46.5183453086989,-57.6398576279405,
-40.9153596996072));
#242164=CARTESIAN_POINT('Ctrl Pts',(-46.5225650990151,-57.3752444181325,
-40.9307954701794));
#242165=CARTESIAN_POINT('Ctrl Pts',(-46.4280892393463,-56.8561059894309,
-40.961078545187));
#242166=CARTESIAN_POINT('Ctrl Pts',(-46.3290060834648,-56.6069932463964,
-40.9749504700387));
#242167=CARTESIAN_POINT('Ctrl Pts',(-46.044853192413,-56.1703797098378,
-41.0020399094839));
#242168=CARTESIAN_POINT('Ctrl Pts',(-45.8657612276326,-55.9849518339394,
-41.0164956170126));
#242169=CARTESIAN_POINT('Ctrl Pts',(-45.4394030099877,-55.6858019193976,
-41.0467596506296));
#242170=CARTESIAN_POINT('Ctrl Pts',(-45.1939230531916,-55.5781088311712,
-41.0623018919607));
#242171=CARTESIAN_POINT('Ctrl Pts',(-44.6836335356126,-55.4666944261493,
-41.0913303604284));
#242172=CARTESIAN_POINT('Ctrl Pts',(-44.4245355192991,-55.4607537804227,
-41.1037353572947));
#242173=CARTESIAN_POINT('Ctrl Pts',(-43.9166058575354,-55.547474839854,
-41.1319243876361));
#242174=CARTESIAN_POINT('Ctrl Pts',(-43.6727127176413,-55.6399315150409,
-41.1469420705348));
#242175=CARTESIAN_POINT('Ctrl Pts',(-43.2278922594853,-55.9160430858539,
-41.1774668306685));
#242176=CARTESIAN_POINT('Ctrl Pts',(-43.0326148387811,-56.099323910573,
-41.1926775751379));
#242177=CARTESIAN_POINT('Ctrl Pts',(-42.7318185640421,-56.5217582212481,
-41.2201942467576));
#242178=CARTESIAN_POINT('Ctrl Pts',(-42.6254137272816,-56.7541638828771,
-41.2328748319307));
#242179=CARTESIAN_POINT('Ctrl Pts',(-42.5031136631561,-57.2542126081442,
-41.2620443409046));
#242180=CARTESIAN_POINT('Ctrl Pts',(-42.4913907026965,-57.5178417825212,
-41.2774227094099));
#242181=CARTESIAN_POINT('Ctrl Pts',(-42.5705889589166,-58.0384472049299,
-41.3077913590504));
#242182=CARTESIAN_POINT('Ctrl Pts',(-42.6622192643798,-58.2900196235696,
-41.322131851386));
#242183=CARTESIAN_POINT('Ctrl Pts',(-42.9327467595647,-58.7338742660884,
-41.3487441599825));
#242184=CARTESIAN_POINT('Ctrl Pts',(-43.105654569544,-58.9240426415747,
-41.3630257200316));
#242185=CARTESIAN_POINT('Ctrl Pts',(-43.5213667545882,-59.2351848995639,
-41.3931017124761));
#242186=CARTESIAN_POINT('Ctrl Pts',(-43.7625807260854,-59.350137595176,
-41.4086401826768));
#242187=CARTESIAN_POINT('Ctrl Pts',(-44.1793416823659,-59.4551740438799,
-41.432757737665));
#242188=CARTESIAN_POINT('Ctrl Pts',(-44.3434954665592,-59.475452478349,
-41.4416419372593));
#242189=CARTESIAN_POINT('Ctrl Pts',(-44.5079524583208,-59.475452478349,
-41.4499499999999));
#242190=CARTESIAN_POINT('Ctrl Pts',(-44.5079524583209,-59.475452478349,
-41.2912000000002));
#242191=CARTESIAN_POINT('Ctrl Pts',(-44.3305589288781,-59.475452478349,
-41.2822384073272));
#242192=CARTESIAN_POINT('Ctrl Pts',(-44.1536253369592,-59.4518585597956,
-41.2726118938888));
#242193=CARTESIAN_POINT('Ctrl Pts',(-43.7269650664756,-59.3355102624255,
-41.2476643149557));
#242194=CARTESIAN_POINT('Ctrl Pts',(-43.4884353487384,-59.2162369893224,
-41.2321354314417));
#242195=CARTESIAN_POINT('Ctrl Pts',(-43.0793311543506,-58.8980073529936,
-41.2021865472492));
#242196=CARTESIAN_POINT('Ctrl Pts',(-42.9102289746349,-58.7050656262889,
-41.1880163511847));
#242197=CARTESIAN_POINT('Ctrl Pts',(-42.6479668302325,-58.2568990964046,
-41.1616958294253));
#242198=CARTESIAN_POINT('Ctrl Pts',(-42.560855617791,-58.003783693849,-41.1470193209044));
#242199=CARTESIAN_POINT('Ctrl Pts',(-42.4910155252582,-57.4823355542716,
-41.1166015127624));
#242200=CARTESIAN_POINT('Ctrl Pts',(-42.5073184864561,-57.2194132681746,
-41.1012643794067));
#242201=CARTESIAN_POINT('Ctrl Pts',(-42.6381191854166,-56.7217703164105,
-41.0722352072204));
#242202=CARTESIAN_POINT('Ctrl Pts',(-42.7486210868745,-56.4910496596015,
-41.059699748032));
#242203=CARTESIAN_POINT('Ctrl Pts',(-43.0568924459804,-56.0737447010577,
-41.0319550550934));
#242204=CARTESIAN_POINT('Ctrl Pts',(-43.255359002887,-55.8938921394422,
-41.0166831923748));
#242205=CARTESIAN_POINT('Ctrl Pts',(-43.7045885134784,-55.6258189241425,
-40.9861701471109));
#242206=CARTESIAN_POINT('Ctrl Pts',(-43.9496148865039,-55.5377152595265,
-40.9712221781807));
#242207=CARTESIAN_POINT('Ctrl Pts',(-44.4594263172017,-55.4594931372893,
-40.9431859700249));
#242208=CARTESIAN_POINT('Ctrl Pts',(-44.7193355129139,-55.4700171688899,
-40.9306798493055));
#242209=CARTESIAN_POINT('Ctrl Pts',(-45.2279490595016,-55.5908256202746,
-40.9014620547703));
#242210=CARTESIAN_POINT('Ctrl Pts',(-45.4710172622289,-55.7026852787828,
-40.8859201258229));
#242211=CARTESIAN_POINT('Ctrl Pts',(-45.891333908348,-56.0087306376859,
-40.8557601840865));
#242212=CARTESIAN_POINT('Ctrl Pts',(-46.0669081081037,-56.1968913632185,
-40.8414024794196));
#242213=CARTESIAN_POINT('Ctrl Pts',(-46.344318594368,-56.6393184641795,
-40.8144840914861));
#242214=CARTESIAN_POINT('Ctrl Pts',(-46.4394909143367,-56.8918467737974,
-40.8002436660988));
#242215=CARTESIAN_POINT('Ctrl Pts',(-46.5240532042183,-57.4139405955126,
-40.7697881931655));
#242216=CARTESIAN_POINT('Ctrl Pts',(-46.5148055933205,-57.6779181751886,
-40.7543895010177));
#242217=CARTESIAN_POINT('Ctrl Pts',(-46.3970923876378,-58.1792466717677,
-40.7251453387173));
#242218=CARTESIAN_POINT('Ctrl Pts',(-46.292878414085,-58.4125679690147,
-40.7123719527804));
#242219=CARTESIAN_POINT('Ctrl Pts',(-45.9960920612698,-58.8377249087666,
-40.6849784449773));
#242220=CARTESIAN_POINT('Ctrl Pts',(-45.8025456890086,-59.022815846432,
-40.6698023549094));
#242221=CARTESIAN_POINT('Ctrl Pts',(-45.3601435069346,-59.30319798829,-40.6392752032839));
#242222=CARTESIAN_POINT('Ctrl Pts',(-45.1168879421948,-59.397978261341,
-40.6242219578971));
#242223=CARTESIAN_POINT('Ctrl Pts',(-44.7450953866053,-59.4649119571554,
-40.603487453548));
#242224=CARTESIAN_POINT('Ctrl Pts',(-44.6265137360848,-59.475452478349,
-40.597189496243));
#242225=CARTESIAN_POINT('Ctrl Pts',(-44.5079524583206,-59.475452478349,
-40.5912000000001));
#242226=CARTESIAN_POINT('Origin',(-44.5079524583206,-57.475452478349,235.35105));
#242227=CARTESIAN_POINT('',(-44.5079524583206,-59.475452478349,-39.8912000000002));
#242228=CARTESIAN_POINT('',(-44.5079524583205,-59.475452478349,-40.0499499999999));
#242229=CARTESIAN_POINT('',(-44.5079524583206,-59.475452478349,235.35105));
#242230=CARTESIAN_POINT('',(-45.8699702267784,-56.010901219983,-39.4567770046169));
#242231=CARTESIAN_POINT('Ctrl Pts',(-44.5079524583206,-59.475452478349,
-39.8912000000001));
#242232=CARTESIAN_POINT('Ctrl Pts',(-44.4030527700808,-59.475452478349,
-39.8859006619664));
#242233=CARTESIAN_POINT('Ctrl Pts',(-44.2982740085944,-59.4672023132265,
-39.8803668031122));
#242234=CARTESIAN_POINT('Ctrl Pts',(-44.0546664311063,-59.428549470864,
-39.8669328247549));
#242235=CARTESIAN_POINT('Ctrl Pts',(-43.917561197412,-59.3915650040988,
-39.8589278085776));
#242236=CARTESIAN_POINT('Ctrl Pts',(-43.539674380705,-59.2451842460787,
-39.835568227459));
#242237=CARTESIAN_POINT('Ctrl Pts',(-43.3150565229897,-59.1022652247094,
-39.8200524776984));
#242238=CARTESIAN_POINT('Ctrl Pts',(-42.9362205101898,-58.7394597649563,
-39.7903325578167));
#242239=CARTESIAN_POINT('Ctrl Pts',(-42.7849633394211,-58.5239481327958,
-39.7773622465096));
#242240=CARTESIAN_POINT('Ctrl Pts',(-42.5753005145157,-58.0506268460953,
-39.7497518381187));
#242241=CARTESIAN_POINT('Ctrl Pts',(-42.5174960198121,-57.7979695862523,
-39.7350134979612));
#242242=CARTESIAN_POINT('Ctrl Pts',(-42.5002448277343,-57.2745386206229,
-39.7044800249661));
#242243=CARTESIAN_POINT('Ctrl Pts',(-42.5449525069551,-57.0086367960749,
-39.6889690852008));
#242244=CARTESIAN_POINT('Ctrl Pts',(-42.7317073816525,-56.5216343248397,
-39.660560607712));
#242245=CARTESIAN_POINT('Ctrl Pts',(-42.8673870546418,-56.3035453915529,
-39.6482310367443));
#242246=CARTESIAN_POINT('Ctrl Pts',(-43.2168701600232,-55.9260604160653,
-39.6195658188577));
#242247=CARTESIAN_POINT('Ctrl Pts',(-43.4288480106903,-55.7716257976807,
-39.6043527472713));
#242248=CARTESIAN_POINT('Ctrl Pts',(-43.9047472663919,-55.5502486800498,
-39.5738543653773));
#242249=CARTESIAN_POINT('Ctrl Pts',(-44.1649808945557,-55.4873165642459,
-39.5588723242467));
#242250=CARTESIAN_POINT('Ctrl Pts',(-44.6830970893764,-55.4670931849909,
-39.5321082047868));
#242251=CARTESIAN_POINT('Ctrl Pts',(-44.935884828577,-55.5053960545974,
-39.5187082946409));
#242252=CARTESIAN_POINT('Ctrl Pts',(-45.3036945482771,-55.6354872771797,
-39.4963329012561));
#242253=CARTESIAN_POINT('Ctrl Pts',(-45.4275250240718,-55.6941435067538,
-39.4883664081885));
#242254=CARTESIAN_POINT('Ctrl Pts',(-45.661019427692,-55.8356263389039,
-39.4724441206155));
#242255=CARTESIAN_POINT('Ctrl Pts',(-45.7701110912147,-55.9180341425543,
-39.4645294508118));
#242256=CARTESIAN_POINT('Ctrl Pts',(-45.8699701444046,-56.0109020958785,
-39.4567761076897));
#242257=CARTESIAN_POINT('',(-46.1726021450474,-56.3668761778516,-39.5898551203275));
#242258=CARTESIAN_POINT('Ctrl Pts',(-46.1726021471674,-56.3668761781232,
-39.5898551143304));
#242259=CARTESIAN_POINT('Ctrl Pts',(-46.1292686891332,-56.3018062073701,
-39.5680429301834));
#242260=CARTESIAN_POINT('Ctrl Pts',(-46.0821985274757,-56.239393519002,
-39.5459682234167));
#242261=CARTESIAN_POINT('Ctrl Pts',(-45.9810865903201,-56.1204740032778,
-39.5015108791791));
#242262=CARTESIAN_POINT('Ctrl Pts',(-45.927110977529,-56.0640425168199,
-39.4791550503913));
#242263=CARTESIAN_POINT('Ctrl Pts',(-45.8699701303408,-56.0109020827993,
-39.456778435228));
#242264=CARTESIAN_POINT('Ctrl Pts',(-46.1726021464359,-56.3668761770248,
-39.5898551218874));
#242265=CARTESIAN_POINT('Ctrl Pts',(-46.0838141022853,-56.2335511277457,
-39.5982291767623));
#242266=CARTESIAN_POINT('Ctrl Pts',(-45.9793476562866,-56.111398861529,
-39.6070694026315));
#242267=CARTESIAN_POINT('Ctrl Pts',(-45.7403294976802,-55.8916874465253,
-39.6255524070794));
#242268=CARTESIAN_POINT('Ctrl Pts',(-45.605941082968,-55.7957258336973,
-39.6351403413518));
#242269=CARTESIAN_POINT('Ctrl Pts',(-45.2282291009047,-55.5909056020896,
-39.6601955747942));
#242270=CARTESIAN_POINT('Ctrl Pts',(-44.9722651093681,-55.5120963029165,
-39.6754250063023));
#242271=CARTESIAN_POINT('Ctrl Pts',(-44.4562316377863,-55.4601269365062,
-39.7030098350655));
#242272=CARTESIAN_POINT('Ctrl Pts',(-44.2015878989259,-55.4828723992968,
-39.7156433846842));
#242273=CARTESIAN_POINT('Ctrl Pts',(-43.7067316346864,-55.6244254417704,
-39.7447712373595));
#242274=CARTESIAN_POINT('Ctrl Pts',(-43.4720515882353,-55.744800314759,
-39.7601377726042));
#242275=CARTESIAN_POINT('Ctrl Pts',(-43.0591643804455,-56.0714058466317,
-39.790522064583));
#242276=CARTESIAN_POINT('Ctrl Pts',(-42.8860320916942,-56.2756143860978,
-39.8049594446186));
#242277=CARTESIAN_POINT('Ctrl Pts',(-42.6345474374558,-56.7303461705793,
-39.83148546538));
#242278=CARTESIAN_POINT('Ctrl Pts',(-42.5550210142441,-56.9746108140771,
-39.8457342362507));
#242279=CARTESIAN_POINT('Ctrl Pts',(-42.4905949281106,-57.4895664751933,
-39.8757733164824));
#242280=CARTESIAN_POINT('Ctrl Pts',(-42.5101306523353,-57.7559010506206,
-39.891309500049));
#242281=CARTESIAN_POINT('Ctrl Pts',(-42.6502003430826,-58.2601709403834,
-39.9207252436185));
#242282=CARTESIAN_POINT('Ctrl Pts',(-42.7672375565043,-58.4937483705101,
-39.9333792695209));
#242283=CARTESIAN_POINT('Ctrl Pts',(-43.0830602239057,-58.9023423061901,
-39.9612513690734));
#242284=CARTESIAN_POINT('Ctrl Pts',(-43.2784359602378,-59.0737611424876,
-39.976121105604));
#242285=CARTESIAN_POINT('Ctrl Pts',(-43.7322273873726,-59.3382290998623,
-40.0067594570893));
#242286=CARTESIAN_POINT('Ctrl Pts',(-43.9883139194582,-59.4252464536864,
-40.0222344807131));
#242287=CARTESIAN_POINT('Ctrl Pts',(-44.338359511837,-59.4700651055624,
-40.0412253466293));
#242288=CARTESIAN_POINT('Ctrl Pts',(-44.4231941692624,-59.475452478349,
-40.045668168162));
#242289=CARTESIAN_POINT('Ctrl Pts',(-44.5079524583204,-59.475452478349,
-40.0499499999999));
#242290=CARTESIAN_POINT('Origin',(-44.5079524583202,31.5404524382932,-52.920575));
#242291=CARTESIAN_POINT('',(-42.8392071752677,31.5404524382931,-40.04995));
#242292=CARTESIAN_POINT('',(-42.8392071752677,31.5404524382931,-39.8912));
#242293=CARTESIAN_POINT('',(-42.8392071752678,31.5404524382932,-52.920575));
#242294=CARTESIAN_POINT('',(-43.0534148594279,32.3583957084033,-39.8341886583259));
#242295=CARTESIAN_POINT('Ctrl Pts',(-42.8392071752677,31.5404524382931,
-39.8912));
#242296=CARTESIAN_POINT('Ctrl Pts',(-42.8392071752677,31.97747304302,-39.8647400338745));
#242297=CARTESIAN_POINT('Ctrl Pts',(-43.0534148594279,32.3583957084033,
-39.8341886583259));
#242298=CARTESIAN_POINT('',(-43.3633208282253,32.7547543987198,-39.9581074212484));
#242299=CARTESIAN_POINT('Ctrl Pts',(-43.3633208282253,32.7547543987198,
-39.9581074212484));
#242300=CARTESIAN_POINT('Ctrl Pts',(-43.3034586305286,32.6983267825555,
-39.9374768681555));
#242301=CARTESIAN_POINT('Ctrl Pts',(-43.247828429449,32.6375299746023,-39.916915604885));
#242302=CARTESIAN_POINT('Ctrl Pts',(-43.1436618117789,32.5052440677468,
-39.8754008689186));
#242303=CARTESIAN_POINT('Ctrl Pts',(-43.0956858178016,32.4335655894238,
-39.8545232151814));
#242304=CARTESIAN_POINT('Ctrl Pts',(-43.0534148594279,32.3583957084032,
-39.834188658326));
#242305=CARTESIAN_POINT('Ctrl Pts',(-42.8392071752677,31.5404524382931,
-40.04995));
#242306=CARTESIAN_POINT('Ctrl Pts',(-42.8392071752677,32.2607116610065,
-40.0063409929454));
#242307=CARTESIAN_POINT('Ctrl Pts',(-43.3633208282253,32.7547543987198,
-39.9581074212484));
#242308=CARTESIAN_POINT('Origin',(-44.5079524583202,31.5404524382932,-52.920575));
#242309=CARTESIAN_POINT('',(-42.8392071752677,31.5404524382931,-40.74995));
#242310=CARTESIAN_POINT('',(-42.8392071752677,31.5404524382931,-40.5912));
#242311=CARTESIAN_POINT('',(-42.8392071752678,31.5404524382932,-52.920575));
#242312=CARTESIAN_POINT('',(-45.3466072487201,32.9831474726816,-40.3575667765883));
#242313=CARTESIAN_POINT('Ctrl Pts',(-42.8392071752677,31.5404524382931,
-40.5912));
#242314=CARTESIAN_POINT('Ctrl Pts',(-42.8392071752677,32.5039029766724,
-40.5328666666667));
#242315=CARTESIAN_POINT('Ctrl Pts',(-43.6735798167939,32.985628245862,-40.4745333333334));
#242316=CARTESIAN_POINT('Ctrl Pts',(-44.5079524583201,33.4673535150516,
-40.4162));
#242317=CARTESIAN_POINT('Ctrl Pts',(-45.3423250998464,32.985628245862,-40.3578666666667));
#242318=CARTESIAN_POINT('Ctrl Pts',(-45.3444680135345,32.9843910340674,
-40.3577168495559));
#242319=CARTESIAN_POINT('Ctrl Pts',(-45.3466072487201,32.9831474726816,
-40.3575667765883));
#242320=CARTESIAN_POINT('',(-46.1762418209585,31.5014470256211,-40.2388224305403));
#242321=CARTESIAN_POINT('Ctrl Pts',(-46.1762415911269,31.5014371968004,
-40.2388206025736));
#242322=CARTESIAN_POINT('Ctrl Pts',(-46.1796538231586,31.6473807982463,
-40.2659631539464));
#242323=CARTESIAN_POINT('Ctrl Pts',(-46.1639045822899,31.7938643599,-40.2897732731299));
#242324=CARTESIAN_POINT('Ctrl Pts',(-46.0934988211157,32.0817317952749,
-40.3293811885115));
#242325=CARTESIAN_POINT('Ctrl Pts',(-46.0387181149382,32.221603202291,-40.3449011256526));
#242326=CARTESIAN_POINT('Ctrl Pts',(-45.8931721207653,32.482839107779,-40.3660091204542));
#242327=CARTESIAN_POINT('Ctrl Pts',(-45.8033957445043,32.6029396495541,
-40.371534813758));
#242328=CARTESIAN_POINT('Ctrl Pts',(-45.6856456418945,32.7228632916643,
-40.3719334317363));
#242329=CARTESIAN_POINT('Ctrl Pts',(-45.6723922330737,32.7359175307787,
-40.3718982162907));
#242330=CARTESIAN_POINT('Ctrl Pts',(-45.5642589075492,32.8389209808004,
-40.3709686031484));
#242331=CARTESIAN_POINT('Ctrl Pts',(-45.4594610512511,32.9175442926251,
-40.3661892700017));
#242332=CARTESIAN_POINT('Ctrl Pts',(-45.3466072487201,32.9831474726816,
-40.3575667765883));
#242333=CARTESIAN_POINT('Ctrl Pts',(-46.1762418209585,31.501447025621,-40.2388224305402));
#242334=CARTESIAN_POINT('Ctrl Pts',(-46.1543258544958,30.5640854850033,
-40.1813025852605));
#242335=CARTESIAN_POINT('Ctrl Pts',(-45.3423250998464,30.0952766307242,
-40.1245333333334));
#242336=CARTESIAN_POINT('Ctrl Pts',(-44.5079524583202,29.6135513615346,
-40.0662));
#242337=CARTESIAN_POINT('Ctrl Pts',(-43.6735798167939,30.0952766307242,
-40.0078666666667));
#242338=CARTESIAN_POINT('Ctrl Pts',(-42.8392071752677,30.5770018999139,
-39.9495333333333));
#242339=CARTESIAN_POINT('Ctrl Pts',(-42.8392071752677,31.5404524382931,
-39.8912));
#242340=CARTESIAN_POINT('Ctrl Pts',(-42.8392071752677,31.5404524382931,
-40.74995));
#242341=CARTESIAN_POINT('Ctrl Pts',(-42.8392071752677,32.5039029766724,
-40.6916166666667));
#242342=CARTESIAN_POINT('Ctrl Pts',(-43.6735798167939,32.985628245862,-40.6332833333334));
#242343=CARTESIAN_POINT('Ctrl Pts',(-44.5079524583201,33.4673535150516,
-40.57495));
#242344=CARTESIAN_POINT('Ctrl Pts',(-45.3423250998464,32.985628245862,-40.5166166666666));
#242345=CARTESIAN_POINT('Ctrl Pts',(-46.1766977413726,32.5039029766724,
-40.4582833333333));
#242346=CARTESIAN_POINT('Ctrl Pts',(-46.1766977413726,31.5404524382932,
-40.39995));
#242347=CARTESIAN_POINT('Ctrl Pts',(-46.1766977413726,30.5770018999139,
-40.3416166666667));
#242348=CARTESIAN_POINT('Ctrl Pts',(-45.3423250998464,30.0952766307242,
-40.2832833333334));
#242349=CARTESIAN_POINT('Ctrl Pts',(-44.5079524583202,29.6135513615346,
-40.22495));
#242350=CARTESIAN_POINT('Ctrl Pts',(-43.6735798167939,30.0952766307242,
-40.1666166666667));
#242351=CARTESIAN_POINT('Ctrl Pts',(-42.8392071752677,30.5770018999139,
-40.1082833333334));
#242352=CARTESIAN_POINT('Ctrl Pts',(-42.8392071752677,31.5404524382931,
-40.04995));
#242353=CARTESIAN_POINT('Origin',(-44.5079524583202,31.5404524382932,-52.920575));
#242354=CARTESIAN_POINT('',(-42.8392071752677,31.5404524382931,-41.44995));
#242355=CARTESIAN_POINT('',(-42.8392071752677,31.5404524382931,-41.2912));
#242356=CARTESIAN_POINT('',(-42.8392071752678,31.5404524382932,-52.920575));
#242357=CARTESIAN_POINT('Ctrl Pts',(-42.8392071752677,31.5404524382931,
-41.2912));
#242358=CARTESIAN_POINT('Ctrl Pts',(-42.8392071752677,32.5039029766724,
-41.2328666666667));
#242359=CARTESIAN_POINT('Ctrl Pts',(-43.6735798167939,32.985628245862,-41.1745333333334));
#242360=CARTESIAN_POINT('Ctrl Pts',(-44.5079524583201,33.4673535150516,
-41.1162));
#242361=CARTESIAN_POINT('Ctrl Pts',(-45.3423250998464,32.985628245862,-41.0578666666667));
#242362=CARTESIAN_POINT('Ctrl Pts',(-46.1766977413726,32.5039029766724,
-40.9995333333333));
#242363=CARTESIAN_POINT('Ctrl Pts',(-46.1766977413726,31.5404524382932,
-40.9412));
#242364=CARTESIAN_POINT('Ctrl Pts',(-46.1766977413726,30.5770018999139,
-40.8828666666667));
#242365=CARTESIAN_POINT('Ctrl Pts',(-45.3423250998464,30.0952766307242,
-40.8245333333333));
#242366=CARTESIAN_POINT('Ctrl Pts',(-44.5079524583202,29.6135513615346,
-40.7662));
#242367=CARTESIAN_POINT('Ctrl Pts',(-43.6735798167939,30.0952766307242,
-40.7078666666667));
#242368=CARTESIAN_POINT('Ctrl Pts',(-42.8392071752677,30.5770018999139,
-40.6495333333333));
#242369=CARTESIAN_POINT('Ctrl Pts',(-42.8392071752677,31.5404524382931,
-40.5912));
#242370=CARTESIAN_POINT('Ctrl Pts',(-42.8392071752677,31.5404524382931,
-41.44995));
#242371=CARTESIAN_POINT('Ctrl Pts',(-42.8392071752677,32.5039029766724,
-41.3916166666667));
#242372=CARTESIAN_POINT('Ctrl Pts',(-43.6735798167939,32.985628245862,-41.3332833333334));
#242373=CARTESIAN_POINT('Ctrl Pts',(-44.5079524583201,33.4673535150516,
-41.27495));
#242374=CARTESIAN_POINT('Ctrl Pts',(-45.3423250998464,32.985628245862,-41.2166166666667));
#242375=CARTESIAN_POINT('Ctrl Pts',(-46.1766977413726,32.5039029766724,
-41.1582833333333));
#242376=CARTESIAN_POINT('Ctrl Pts',(-46.1766977413726,31.5404524382932,
-41.09995));
#242377=CARTESIAN_POINT('Ctrl Pts',(-46.1766977413726,30.5770018999139,
-41.0416166666667));
#242378=CARTESIAN_POINT('Ctrl Pts',(-45.3423250998464,30.0952766307242,
-40.9832833333333));
#242379=CARTESIAN_POINT('Ctrl Pts',(-44.5079524583202,29.6135513615346,
-40.92495));
#242380=CARTESIAN_POINT('Ctrl Pts',(-43.6735798167939,30.0952766307242,
-40.8666166666667));
#242381=CARTESIAN_POINT('Ctrl Pts',(-42.8392071752677,30.5770018999139,
-40.8082833333334));
#242382=CARTESIAN_POINT('Ctrl Pts',(-42.8392071752677,31.5404524382931,
-40.74995));
#242383=CARTESIAN_POINT('Origin',(-44.5079524583202,31.5404524382932,-52.920575));
#242384=CARTESIAN_POINT('',(-42.8392071752677,31.5404524382931,-42.14995));
#242385=CARTESIAN_POINT('',(-42.8392071752677,31.5404524382931,-41.9912));
#242386=CARTESIAN_POINT('',(-42.8392071752678,31.5404524382932,-52.920575));
#242387=CARTESIAN_POINT('Ctrl Pts',(-42.8392071752677,31.5404524382931,
-41.9912));
#242388=CARTESIAN_POINT('Ctrl Pts',(-42.8392071752677,32.5039029766724,
-41.9328666666667));
#242389=CARTESIAN_POINT('Ctrl Pts',(-43.6735798167939,32.985628245862,-41.8745333333334));
#242390=CARTESIAN_POINT('Ctrl Pts',(-44.5079524583201,33.4673535150516,
-41.8162));
#242391=CARTESIAN_POINT('Ctrl Pts',(-45.3423250998464,32.985628245862,-41.7578666666667));
#242392=CARTESIAN_POINT('Ctrl Pts',(-46.1766977413726,32.5039029766724,
-41.6995333333334));
#242393=CARTESIAN_POINT('Ctrl Pts',(-46.1766977413726,31.5404524382932,
-41.6412));
#242394=CARTESIAN_POINT('Ctrl Pts',(-46.1766977413726,30.5770018999139,
-41.5828666666667));
#242395=CARTESIAN_POINT('Ctrl Pts',(-45.3423250998464,30.0952766307242,
-41.5245333333334));
#242396=CARTESIAN_POINT('Ctrl Pts',(-44.5079524583202,29.6135513615346,
-41.4662));
#242397=CARTESIAN_POINT('Ctrl Pts',(-43.6735798167939,30.0952766307242,
-41.4078666666667));
#242398=CARTESIAN_POINT('Ctrl Pts',(-42.8392071752677,30.5770018999139,
-41.3495333333333));
#242399=CARTESIAN_POINT('Ctrl Pts',(-42.8392071752677,31.5404524382931,
-41.2912));
#242400=CARTESIAN_POINT('Ctrl Pts',(-42.8392071752677,31.5404524382931,
-42.14995));
#242401=CARTESIAN_POINT('Ctrl Pts',(-42.8392071752677,32.5039029766724,
-42.0916166666667));
#242402=CARTESIAN_POINT('Ctrl Pts',(-43.6735798167939,32.985628245862,-42.0332833333334));
#242403=CARTESIAN_POINT('Ctrl Pts',(-44.5079524583201,33.4673535150516,
-41.97495));
#242404=CARTESIAN_POINT('Ctrl Pts',(-45.3423250998464,32.985628245862,-41.9166166666666));
#242405=CARTESIAN_POINT('Ctrl Pts',(-46.1766977413726,32.5039029766724,
-41.8582833333333));
#242406=CARTESIAN_POINT('Ctrl Pts',(-46.1766977413726,31.5404524382932,
-41.79995));
#242407=CARTESIAN_POINT('Ctrl Pts',(-46.1766977413726,30.5770018999139,
-41.7416166666666));
#242408=CARTESIAN_POINT('Ctrl Pts',(-45.3423250998464,30.0952766307242,
-41.6832833333333));
#242409=CARTESIAN_POINT('Ctrl Pts',(-44.5079524583202,29.6135513615346,
-41.62495));
#242410=CARTESIAN_POINT('Ctrl Pts',(-43.6735798167939,30.0952766307242,
-41.5666166666667));
#242411=CARTESIAN_POINT('Ctrl Pts',(-42.8392071752677,30.5770018999139,
-41.5082833333334));
#242412=CARTESIAN_POINT('Ctrl Pts',(-42.8392071752677,31.5404524382931,
-41.44995));
#242413=CARTESIAN_POINT('Origin',(-44.5079524583202,31.5404524382932,-52.920575));
#242414=CARTESIAN_POINT('',(-42.8392071752677,31.5404524382931,-42.84995));
#242415=CARTESIAN_POINT('',(-42.8392071752677,31.5404524382931,-42.6912));
#242416=CARTESIAN_POINT('',(-42.8392071752678,31.5404524382932,-52.920575));
#242417=CARTESIAN_POINT('Ctrl Pts',(-42.8392071752677,31.5404524382931,
-42.6912));
#242418=CARTESIAN_POINT('Ctrl Pts',(-42.8392071752677,32.5039029766724,
-42.6328666666667));
#242419=CARTESIAN_POINT('Ctrl Pts',(-43.6735798167939,32.985628245862,-42.5745333333333));
#242420=CARTESIAN_POINT('Ctrl Pts',(-44.5079524583201,33.4673535150516,
-42.5162));
#242421=CARTESIAN_POINT('Ctrl Pts',(-45.3423250998464,32.985628245862,-42.4578666666667));
#242422=CARTESIAN_POINT('Ctrl Pts',(-46.1766977413726,32.5039029766724,
-42.3995333333334));
#242423=CARTESIAN_POINT('Ctrl Pts',(-46.1766977413726,31.5404524382932,
-42.3412));
#242424=CARTESIAN_POINT('Ctrl Pts',(-46.1766977413726,30.5770018999139,
-42.2828666666667));
#242425=CARTESIAN_POINT('Ctrl Pts',(-45.3423250998464,30.0952766307242,
-42.2245333333333));
#242426=CARTESIAN_POINT('Ctrl Pts',(-44.5079524583202,29.6135513615346,
-42.1662));
#242427=CARTESIAN_POINT('Ctrl Pts',(-43.6735798167939,30.0952766307242,
-42.1078666666667));
#242428=CARTESIAN_POINT('Ctrl Pts',(-42.8392071752677,30.5770018999139,
-42.0495333333334));
#242429=CARTESIAN_POINT('Ctrl Pts',(-42.8392071752677,31.5404524382931,
-41.9912));
#242430=CARTESIAN_POINT('Ctrl Pts',(-42.8392071752677,31.5404524382931,
-42.84995));
#242431=CARTESIAN_POINT('Ctrl Pts',(-42.8392071752677,32.5039029766724,
-42.7916166666667));
#242432=CARTESIAN_POINT('Ctrl Pts',(-43.6735798167939,32.985628245862,-42.7332833333334));
#242433=CARTESIAN_POINT('Ctrl Pts',(-44.5079524583201,33.4673535150516,
-42.67495));
#242434=CARTESIAN_POINT('Ctrl Pts',(-45.3423250998464,32.985628245862,-42.6166166666667));
#242435=CARTESIAN_POINT('Ctrl Pts',(-46.1766977413726,32.5039029766724,
-42.5582833333333));
#242436=CARTESIAN_POINT('Ctrl Pts',(-46.1766977413726,31.5404524382932,
-42.49995));
#242437=CARTESIAN_POINT('Ctrl Pts',(-46.1766977413726,30.5770018999139,
-42.4416166666666));
#242438=CARTESIAN_POINT('Ctrl Pts',(-45.3423250998464,30.0952766307242,
-42.3832833333333));
#242439=CARTESIAN_POINT('Ctrl Pts',(-44.5079524583202,29.6135513615346,
-42.32495));
#242440=CARTESIAN_POINT('Ctrl Pts',(-43.6735798167939,30.0952766307242,
-42.2666166666667));
#242441=CARTESIAN_POINT('Ctrl Pts',(-42.8392071752677,30.5770018999139,
-42.2082833333333));
#242442=CARTESIAN_POINT('Ctrl Pts',(-42.8392071752677,31.5404524382931,
-42.14995));
#242443=CARTESIAN_POINT('Origin',(-44.5079524583202,31.5404524382932,-52.920575));
#242444=CARTESIAN_POINT('',(-42.8392071752677,31.5404524382931,-43.54995));
#242445=CARTESIAN_POINT('',(-42.8392071752677,31.5404524382931,-43.3912));
#242446=CARTESIAN_POINT('',(-42.8392071752678,31.5404524382932,-52.920575));
#242447=CARTESIAN_POINT('Ctrl Pts',(-42.8392071752677,31.5404524382931,
-43.3912));
#242448=CARTESIAN_POINT('Ctrl Pts',(-42.8392071752677,32.5039029766724,
-43.3328666666667));
#242449=CARTESIAN_POINT('Ctrl Pts',(-43.6735798167939,32.985628245862,-43.2745333333334));
#242450=CARTESIAN_POINT('Ctrl Pts',(-44.5079524583201,33.4673535150516,
-43.2162));
#242451=CARTESIAN_POINT('Ctrl Pts',(-45.3423250998464,32.985628245862,-43.1578666666667));
#242452=CARTESIAN_POINT('Ctrl Pts',(-46.1766977413726,32.5039029766724,
-43.0995333333334));
#242453=CARTESIAN_POINT('Ctrl Pts',(-46.1766977413726,31.5404524382932,
-43.0412));
#242454=CARTESIAN_POINT('Ctrl Pts',(-46.1766977413726,30.5770018999139,
-42.9828666666667));
#242455=CARTESIAN_POINT('Ctrl Pts',(-45.3423250998464,30.0952766307242,
-42.9245333333334));
#242456=CARTESIAN_POINT('Ctrl Pts',(-44.5079524583202,29.6135513615346,
-42.8662));
#242457=CARTESIAN_POINT('Ctrl Pts',(-43.6735798167939,30.0952766307242,
-42.8078666666667));
#242458=CARTESIAN_POINT('Ctrl Pts',(-42.8392071752677,30.5770018999139,
-42.7495333333334));
#242459=CARTESIAN_POINT('Ctrl Pts',(-42.8392071752677,31.5404524382931,
-42.6912));
#242460=CARTESIAN_POINT('Ctrl Pts',(-42.8392071752677,31.5404524382931,
-43.54995));
#242461=CARTESIAN_POINT('Ctrl Pts',(-42.8392071752677,32.5039029766724,
-43.4916166666667));
#242462=CARTESIAN_POINT('Ctrl Pts',(-43.6735798167939,32.985628245862,-43.4332833333333));
#242463=CARTESIAN_POINT('Ctrl Pts',(-44.5079524583201,33.4673535150516,
-43.37495));
#242464=CARTESIAN_POINT('Ctrl Pts',(-45.3423250998464,32.985628245862,-43.3166166666667));
#242465=CARTESIAN_POINT('Ctrl Pts',(-46.1766977413726,32.5039029766724,
-43.2582833333333));
#242466=CARTESIAN_POINT('Ctrl Pts',(-46.1766977413726,31.5404524382932,
-43.19995));
#242467=CARTESIAN_POINT('Ctrl Pts',(-46.1766977413726,30.5770018999139,
-43.1416166666666));
#242468=CARTESIAN_POINT('Ctrl Pts',(-45.3423250998464,30.0952766307242,
-43.0832833333333));
#242469=CARTESIAN_POINT('Ctrl Pts',(-44.5079524583202,29.6135513615346,
-43.02495));
#242470=CARTESIAN_POINT('Ctrl Pts',(-43.6735798167939,30.0952766307242,
-42.9666166666667));
#242471=CARTESIAN_POINT('Ctrl Pts',(-42.8392071752677,30.5770018999139,
-42.9082833333333));
#242472=CARTESIAN_POINT('Ctrl Pts',(-42.8392071752677,31.5404524382931,
-42.84995));
#242473=CARTESIAN_POINT('Origin',(-44.5079524583202,31.5404524382932,-52.920575));
#242474=CARTESIAN_POINT('',(-42.8392071752677,31.5404524382931,-44.24995));
#242475=CARTESIAN_POINT('',(-42.8392071752677,31.5404524382931,-44.0912));
#242476=CARTESIAN_POINT('',(-42.8392071752678,31.5404524382932,-52.920575));
#242477=CARTESIAN_POINT('Ctrl Pts',(-42.8392071752677,31.5404524382931,
-44.0912));
#242478=CARTESIAN_POINT('Ctrl Pts',(-42.8392071752677,32.5039029766724,
-44.0328666666667));
#242479=CARTESIAN_POINT('Ctrl Pts',(-43.6735798167939,32.985628245862,-43.9745333333333));
#242480=CARTESIAN_POINT('Ctrl Pts',(-44.5079524583201,33.4673535150516,
-43.9162));
#242481=CARTESIAN_POINT('Ctrl Pts',(-45.3423250998464,32.985628245862,-43.8578666666667));
#242482=CARTESIAN_POINT('Ctrl Pts',(-46.1766977413726,32.5039029766724,
-43.7995333333334));
#242483=CARTESIAN_POINT('Ctrl Pts',(-46.1766977413726,31.5404524382932,
-43.7412));
#242484=CARTESIAN_POINT('Ctrl Pts',(-46.1766977413726,30.5770018999139,
-43.6828666666667));
#242485=CARTESIAN_POINT('Ctrl Pts',(-45.3423250998464,30.0952766307242,
-43.6245333333333));
#242486=CARTESIAN_POINT('Ctrl Pts',(-44.5079524583202,29.6135513615346,
-43.5662));
#242487=CARTESIAN_POINT('Ctrl Pts',(-43.6735798167939,30.0952766307242,
-43.5078666666667));
#242488=CARTESIAN_POINT('Ctrl Pts',(-42.8392071752677,30.5770018999139,
-43.4495333333334));
#242489=CARTESIAN_POINT('Ctrl Pts',(-42.8392071752677,31.5404524382931,
-43.3912));
#242490=CARTESIAN_POINT('Ctrl Pts',(-42.8392071752677,31.5404524382931,
-44.24995));
#242491=CARTESIAN_POINT('Ctrl Pts',(-42.8392071752677,32.5039029766724,
-44.1916166666667));
#242492=CARTESIAN_POINT('Ctrl Pts',(-43.6735798167939,32.985628245862,-44.1332833333334));
#242493=CARTESIAN_POINT('Ctrl Pts',(-44.5079524583201,33.4673535150516,
-44.07495));
#242494=CARTESIAN_POINT('Ctrl Pts',(-45.3423250998464,32.985628245862,-44.0166166666667));
#242495=CARTESIAN_POINT('Ctrl Pts',(-46.1766977413726,32.5039029766724,
-43.9582833333334));
#242496=CARTESIAN_POINT('Ctrl Pts',(-46.1766977413726,31.5404524382932,
-43.89995));
#242497=CARTESIAN_POINT('Ctrl Pts',(-46.1766977413726,30.5770018999139,
-43.8416166666667));
#242498=CARTESIAN_POINT('Ctrl Pts',(-45.3423250998464,30.0952766307242,
-43.7832833333334));
#242499=CARTESIAN_POINT('Ctrl Pts',(-44.5079524583202,29.6135513615346,
-43.72495));
#242500=CARTESIAN_POINT('Ctrl Pts',(-43.6735798167939,30.0952766307242,
-43.6666166666667));
#242501=CARTESIAN_POINT('Ctrl Pts',(-42.8392071752677,30.5770018999139,
-43.6082833333333));
#242502=CARTESIAN_POINT('Ctrl Pts',(-42.8392071752677,31.5404524382931,
-43.54995));
#242503=CARTESIAN_POINT('Origin',(-44.5079524583202,31.5404524382932,-52.920575));
#242504=CARTESIAN_POINT('',(-42.8392071752677,31.5404524382931,-44.94995));
#242505=CARTESIAN_POINT('',(-42.8392071752677,31.5404524382931,-44.7912));
#242506=CARTESIAN_POINT('',(-42.8392071752678,31.5404524382932,-52.920575));
#242507=CARTESIAN_POINT('Ctrl Pts',(-42.8392071752677,31.5404524382931,
-44.7912));
#242508=CARTESIAN_POINT('Ctrl Pts',(-42.8392071752677,32.5039029766724,
-44.7328666666667));
#242509=CARTESIAN_POINT('Ctrl Pts',(-43.6735798167939,32.985628245862,-44.6745333333334));
#242510=CARTESIAN_POINT('Ctrl Pts',(-44.5079524583201,33.4673535150516,
-44.6162));
#242511=CARTESIAN_POINT('Ctrl Pts',(-45.3423250998464,32.985628245862,-44.5578666666667));
#242512=CARTESIAN_POINT('Ctrl Pts',(-46.1766977413726,32.5039029766724,
-44.4995333333333));
#242513=CARTESIAN_POINT('Ctrl Pts',(-46.1766977413726,31.5404524382932,
-44.4412));
#242514=CARTESIAN_POINT('Ctrl Pts',(-46.1766977413726,30.5770018999139,
-44.3828666666667));
#242515=CARTESIAN_POINT('Ctrl Pts',(-45.3423250998464,30.0952766307242,
-44.3245333333334));
#242516=CARTESIAN_POINT('Ctrl Pts',(-44.5079524583202,29.6135513615346,
-44.2662));
#242517=CARTESIAN_POINT('Ctrl Pts',(-43.6735798167939,30.0952766307242,
-44.2078666666667));
#242518=CARTESIAN_POINT('Ctrl Pts',(-42.8392071752677,30.5770018999139,
-44.1495333333334));
#242519=CARTESIAN_POINT('Ctrl Pts',(-42.8392071752677,31.5404524382931,
-44.0912));
#242520=CARTESIAN_POINT('Ctrl Pts',(-42.8392071752677,31.5404524382931,
-44.94995));
#242521=CARTESIAN_POINT('Ctrl Pts',(-42.8392071752677,32.5039029766724,
-44.8916166666667));
#242522=CARTESIAN_POINT('Ctrl Pts',(-43.6735798167939,32.985628245862,-44.8332833333334));
#242523=CARTESIAN_POINT('Ctrl Pts',(-44.5079524583201,33.4673535150516,
-44.77495));
#242524=CARTESIAN_POINT('Ctrl Pts',(-45.3423250998464,32.985628245862,-44.7166166666667));
#242525=CARTESIAN_POINT('Ctrl Pts',(-46.1766977413726,32.5039029766724,
-44.6582833333333));
#242526=CARTESIAN_POINT('Ctrl Pts',(-46.1766977413726,31.5404524382932,
-44.59995));
#242527=CARTESIAN_POINT('Ctrl Pts',(-46.1766977413726,30.5770018999139,
-44.5416166666667));
#242528=CARTESIAN_POINT('Ctrl Pts',(-45.3423250998464,30.0952766307242,
-44.4832833333334));
#242529=CARTESIAN_POINT('Ctrl Pts',(-44.5079524583202,29.6135513615346,
-44.42495));
#242530=CARTESIAN_POINT('Ctrl Pts',(-43.6735798167939,30.0952766307242,
-44.3666166666667));
#242531=CARTESIAN_POINT('Ctrl Pts',(-42.8392071752677,30.5770018999139,
-44.3082833333334));
#242532=CARTESIAN_POINT('Ctrl Pts',(-42.8392071752677,31.5404524382931,
-44.24995));
#242533=CARTESIAN_POINT('Origin',(-44.5079524583202,31.5404524382932,-52.920575));
#242534=CARTESIAN_POINT('',(-42.8392071752677,31.5404524382931,-45.64995));
#242535=CARTESIAN_POINT('',(-42.8392071752677,31.5404524382931,-45.4912));
#242536=CARTESIAN_POINT('',(-42.8392071752678,31.5404524382932,-52.920575));
#242537=CARTESIAN_POINT('Ctrl Pts',(-42.8392071752677,31.5404524382931,
-45.4912));
#242538=CARTESIAN_POINT('Ctrl Pts',(-42.8392071752677,32.5039029766724,
-45.4328666666666));
#242539=CARTESIAN_POINT('Ctrl Pts',(-43.6735798167939,32.985628245862,-45.3745333333333));
#242540=CARTESIAN_POINT('Ctrl Pts',(-44.5079524583201,33.4673535150516,
-45.3162));
#242541=CARTESIAN_POINT('Ctrl Pts',(-45.3423250998464,32.985628245862,-45.2578666666667));
#242542=CARTESIAN_POINT('Ctrl Pts',(-46.1766977413726,32.5039029766724,
-45.1995333333333));
#242543=CARTESIAN_POINT('Ctrl Pts',(-46.1766977413726,31.5404524382932,
-45.1412));
#242544=CARTESIAN_POINT('Ctrl Pts',(-46.1766977413726,30.5770018999139,
-45.0828666666667));
#242545=CARTESIAN_POINT('Ctrl Pts',(-45.3423250998464,30.0952766307242,
-45.0245333333333));
#242546=CARTESIAN_POINT('Ctrl Pts',(-44.5079524583202,29.6135513615346,
-44.9662));
#242547=CARTESIAN_POINT('Ctrl Pts',(-43.6735798167939,30.0952766307242,
-44.9078666666666));
#242548=CARTESIAN_POINT('Ctrl Pts',(-42.8392071752677,30.5770018999139,
-44.8495333333333));
#242549=CARTESIAN_POINT('Ctrl Pts',(-42.8392071752677,31.5404524382931,
-44.7912));
#242550=CARTESIAN_POINT('Ctrl Pts',(-42.8392071752677,31.5404524382931,
-45.64995));
#242551=CARTESIAN_POINT('Ctrl Pts',(-42.8392071752677,32.5039029766724,
-45.5916166666667));
#242552=CARTESIAN_POINT('Ctrl Pts',(-43.6735798167939,32.985628245862,-45.5332833333333));
#242553=CARTESIAN_POINT('Ctrl Pts',(-44.5079524583201,33.4673535150516,
-45.47495));
#242554=CARTESIAN_POINT('Ctrl Pts',(-45.3423250998464,32.985628245862,-45.4166166666667));
#242555=CARTESIAN_POINT('Ctrl Pts',(-46.1766977413726,32.5039029766724,
-45.3582833333334));
#242556=CARTESIAN_POINT('Ctrl Pts',(-46.1766977413726,31.5404524382932,
-45.29995));
#242557=CARTESIAN_POINT('Ctrl Pts',(-46.1766977413726,30.5770018999139,
-45.2416166666667));
#242558=CARTESIAN_POINT('Ctrl Pts',(-45.3423250998464,30.0952766307242,
-45.1832833333333));
#242559=CARTESIAN_POINT('Ctrl Pts',(-44.5079524583202,29.6135513615346,
-45.12495));
#242560=CARTESIAN_POINT('Ctrl Pts',(-43.6735798167939,30.0952766307242,
-45.0666166666667));
#242561=CARTESIAN_POINT('Ctrl Pts',(-42.8392071752677,30.5770018999139,
-45.0082833333334));
#242562=CARTESIAN_POINT('Ctrl Pts',(-42.8392071752677,31.5404524382931,
-44.94995));
#242563=CARTESIAN_POINT('Origin',(-44.5079524583202,31.5404524382932,-52.920575));
#242564=CARTESIAN_POINT('',(-42.8392071752677,31.5404524382931,-46.34995));
#242565=CARTESIAN_POINT('',(-42.8392071752677,31.5404524382931,-46.1912));
#242566=CARTESIAN_POINT('',(-42.8392071752678,31.5404524382932,-52.920575));
#242567=CARTESIAN_POINT('Ctrl Pts',(-42.8392071752677,31.5404524382931,
-46.1912));
#242568=CARTESIAN_POINT('Ctrl Pts',(-42.8392071752677,32.5039029766724,
-46.1328666666667));
#242569=CARTESIAN_POINT('Ctrl Pts',(-43.6735798167939,32.985628245862,-46.0745333333334));
#242570=CARTESIAN_POINT('Ctrl Pts',(-44.5079524583201,33.4673535150516,
-46.0162));
#242571=CARTESIAN_POINT('Ctrl Pts',(-45.3423250998464,32.985628245862,-45.9578666666667));
#242572=CARTESIAN_POINT('Ctrl Pts',(-46.1766977413726,32.5039029766724,
-45.8995333333333));
#242573=CARTESIAN_POINT('Ctrl Pts',(-46.1766977413726,31.5404524382932,
-45.8412));
#242574=CARTESIAN_POINT('Ctrl Pts',(-46.1766977413726,30.5770018999139,
-45.7828666666667));
#242575=CARTESIAN_POINT('Ctrl Pts',(-45.3423250998464,30.0952766307242,
-45.7245333333333));
#242576=CARTESIAN_POINT('Ctrl Pts',(-44.5079524583202,29.6135513615346,
-45.6662));
#242577=CARTESIAN_POINT('Ctrl Pts',(-43.6735798167939,30.0952766307242,
-45.6078666666667));
#242578=CARTESIAN_POINT('Ctrl Pts',(-42.8392071752677,30.5770018999139,
-45.5495333333333));
#242579=CARTESIAN_POINT('Ctrl Pts',(-42.8392071752677,31.5404524382931,
-45.4912));
#242580=CARTESIAN_POINT('Ctrl Pts',(-42.8392071752677,31.5404524382931,
-46.34995));
#242581=CARTESIAN_POINT('Ctrl Pts',(-42.8392071752677,32.5039029766724,
-46.2916166666667));
#242582=CARTESIAN_POINT('Ctrl Pts',(-43.6735798167939,32.985628245862,-46.2332833333334));
#242583=CARTESIAN_POINT('Ctrl Pts',(-44.5079524583201,33.4673535150516,
-46.17495));
#242584=CARTESIAN_POINT('Ctrl Pts',(-45.3423250998464,32.985628245862,-46.1166166666667));
#242585=CARTESIAN_POINT('Ctrl Pts',(-46.1766977413726,32.5039029766724,
-46.0582833333333));
#242586=CARTESIAN_POINT('Ctrl Pts',(-46.1766977413726,31.5404524382932,
-45.99995));
#242587=CARTESIAN_POINT('Ctrl Pts',(-46.1766977413726,30.5770018999139,
-45.9416166666667));
#242588=CARTESIAN_POINT('Ctrl Pts',(-45.3423250998464,30.0952766307242,
-45.8832833333333));
#242589=CARTESIAN_POINT('Ctrl Pts',(-44.5079524583202,29.6135513615346,
-45.82495));
#242590=CARTESIAN_POINT('Ctrl Pts',(-43.6735798167939,30.0952766307242,
-45.7666166666667));
#242591=CARTESIAN_POINT('Ctrl Pts',(-42.8392071752677,30.5770018999139,
-45.7082833333333));
#242592=CARTESIAN_POINT('Ctrl Pts',(-42.8392071752677,31.5404524382931,
-45.64995));
#242593=CARTESIAN_POINT('Origin',(-44.5079524583202,31.5404524382932,-52.920575));
#242594=CARTESIAN_POINT('',(-42.8392071752677,31.5404524382931,-47.04995));
#242595=CARTESIAN_POINT('',(-42.8392071752677,31.5404524382931,-46.8912));
#242596=CARTESIAN_POINT('',(-42.8392071752678,31.5404524382932,-52.920575));
#242597=CARTESIAN_POINT('Ctrl Pts',(-42.8392071752677,31.5404524382931,
-46.8912));
#242598=CARTESIAN_POINT('Ctrl Pts',(-42.8392071752677,32.5039029766724,
-46.8328666666667));
#242599=CARTESIAN_POINT('Ctrl Pts',(-43.6735798167939,32.985628245862,-46.7745333333333));
#242600=CARTESIAN_POINT('Ctrl Pts',(-44.5079524583201,33.4673535150516,
-46.7162));
#242601=CARTESIAN_POINT('Ctrl Pts',(-45.3423250998464,32.985628245862,-46.6578666666667));
#242602=CARTESIAN_POINT('Ctrl Pts',(-46.1766977413726,32.5039029766724,
-46.5995333333333));
#242603=CARTESIAN_POINT('Ctrl Pts',(-46.1766977413726,31.5404524382932,
-46.5412));
#242604=CARTESIAN_POINT('Ctrl Pts',(-46.1766977413726,30.5770018999139,
-46.4828666666667));
#242605=CARTESIAN_POINT('Ctrl Pts',(-45.3423250998464,30.0952766307242,
-46.4245333333333));
#242606=CARTESIAN_POINT('Ctrl Pts',(-44.5079524583202,29.6135513615346,
-46.3662));
#242607=CARTESIAN_POINT('Ctrl Pts',(-43.6735798167939,30.0952766307242,
-46.3078666666667));
#242608=CARTESIAN_POINT('Ctrl Pts',(-42.8392071752677,30.5770018999139,
-46.2495333333334));
#242609=CARTESIAN_POINT('Ctrl Pts',(-42.8392071752677,31.5404524382931,
-46.1912));
#242610=CARTESIAN_POINT('Ctrl Pts',(-42.8392071752677,31.5404524382931,
-47.04995));
#242611=CARTESIAN_POINT('Ctrl Pts',(-42.8392071752677,32.5039029766724,
-46.9916166666667));
#242612=CARTESIAN_POINT('Ctrl Pts',(-43.6735798167939,32.985628245862,-46.9332833333333));
#242613=CARTESIAN_POINT('Ctrl Pts',(-44.5079524583201,33.4673535150516,
-46.87495));
#242614=CARTESIAN_POINT('Ctrl Pts',(-45.3423250998464,32.985628245862,-46.8166166666667));
#242615=CARTESIAN_POINT('Ctrl Pts',(-46.1766977413726,32.5039029766724,
-46.7582833333333));
#242616=CARTESIAN_POINT('Ctrl Pts',(-46.1766977413726,31.5404524382932,
-46.69995));
#242617=CARTESIAN_POINT('Ctrl Pts',(-46.1766977413726,30.5770018999139,
-46.6416166666666));
#242618=CARTESIAN_POINT('Ctrl Pts',(-45.3423250998464,30.0952766307242,
-46.5832833333334));
#242619=CARTESIAN_POINT('Ctrl Pts',(-44.5079524583202,29.6135513615346,
-46.52495));
#242620=CARTESIAN_POINT('Ctrl Pts',(-43.6735798167939,30.0952766307242,
-46.4666166666667));
#242621=CARTESIAN_POINT('Ctrl Pts',(-42.8392071752677,30.5770018999139,
-46.4082833333333));
#242622=CARTESIAN_POINT('Ctrl Pts',(-42.8392071752677,31.5404524382931,
-46.34995));
#242623=CARTESIAN_POINT('Origin',(-44.5079524583202,31.5404524382932,-52.920575));
#242624=CARTESIAN_POINT('',(-42.8392071752677,31.5404524382931,-47.74995));
#242625=CARTESIAN_POINT('',(-42.8392071752677,31.5404524382931,-47.5912));
#242626=CARTESIAN_POINT('',(-42.8392071752678,31.5404524382932,-52.920575));
#242627=CARTESIAN_POINT('Ctrl Pts',(-42.8392071752677,31.5404524382931,
-47.5912));
#242628=CARTESIAN_POINT('Ctrl Pts',(-42.8392071752677,32.5039029766724,
-47.5328666666667));
#242629=CARTESIAN_POINT('Ctrl Pts',(-43.6735798167939,32.985628245862,-47.4745333333334));
#242630=CARTESIAN_POINT('Ctrl Pts',(-44.5079524583201,33.4673535150516,
-47.4162));
#242631=CARTESIAN_POINT('Ctrl Pts',(-45.3423250998464,32.985628245862,-47.3578666666667));
#242632=CARTESIAN_POINT('Ctrl Pts',(-46.1766977413726,32.5039029766724,
-47.2995333333334));
#242633=CARTESIAN_POINT('Ctrl Pts',(-46.1766977413726,31.5404524382932,
-47.2412));
#242634=CARTESIAN_POINT('Ctrl Pts',(-46.1766977413726,30.5770018999139,
-47.1828666666667));
#242635=CARTESIAN_POINT('Ctrl Pts',(-45.3423250998464,30.0952766307242,
-47.1245333333333));
#242636=CARTESIAN_POINT('Ctrl Pts',(-44.5079524583202,29.6135513615346,
-47.0662));
#242637=CARTESIAN_POINT('Ctrl Pts',(-43.6735798167939,30.0952766307242,
-47.0078666666667));
#242638=CARTESIAN_POINT('Ctrl Pts',(-42.8392071752677,30.5770018999139,
-46.9495333333334));
#242639=CARTESIAN_POINT('Ctrl Pts',(-42.8392071752677,31.5404524382931,
-46.8912));
#242640=CARTESIAN_POINT('Ctrl Pts',(-42.8392071752677,31.5404524382931,
-47.74995));
#242641=CARTESIAN_POINT('Ctrl Pts',(-42.8392071752677,32.5039029766724,
-47.6916166666667));
#242642=CARTESIAN_POINT('Ctrl Pts',(-43.6735798167939,32.985628245862,-47.6332833333333));
#242643=CARTESIAN_POINT('Ctrl Pts',(-44.5079524583201,33.4673535150516,
-47.57495));
#242644=CARTESIAN_POINT('Ctrl Pts',(-45.3423250998464,32.985628245862,-47.5166166666667));
#242645=CARTESIAN_POINT('Ctrl Pts',(-46.1766977413726,32.5039029766724,
-47.4582833333333));
#242646=CARTESIAN_POINT('Ctrl Pts',(-46.1766977413726,31.5404524382932,
-47.39995));
#242647=CARTESIAN_POINT('Ctrl Pts',(-46.1766977413726,30.5770018999139,
-47.3416166666666));
#242648=CARTESIAN_POINT('Ctrl Pts',(-45.3423250998464,30.0952766307242,
-47.2832833333333));
#242649=CARTESIAN_POINT('Ctrl Pts',(-44.5079524583202,29.6135513615346,
-47.22495));
#242650=CARTESIAN_POINT('Ctrl Pts',(-43.6735798167939,30.0952766307242,
-47.1666166666667));
#242651=CARTESIAN_POINT('Ctrl Pts',(-42.8392071752677,30.5770018999139,
-47.1082833333333));
#242652=CARTESIAN_POINT('Ctrl Pts',(-42.8392071752677,31.5404524382931,
-47.04995));
#242653=CARTESIAN_POINT('Origin',(-44.5079524583202,31.5404524382932,-52.920575));
#242654=CARTESIAN_POINT('',(-42.8392071752677,31.5404524382931,-48.44995));
#242655=CARTESIAN_POINT('',(-42.8392071752677,31.5404524382931,-48.2912));
#242656=CARTESIAN_POINT('',(-42.8392071752678,31.5404524382932,-52.920575));
#242657=CARTESIAN_POINT('Ctrl Pts',(-42.8392071752677,31.5404524382931,
-48.2912));
#242658=CARTESIAN_POINT('Ctrl Pts',(-42.8392071752677,32.5039029766724,
-48.2328666666667));
#242659=CARTESIAN_POINT('Ctrl Pts',(-43.6735798167939,32.985628245862,-48.1745333333334));
#242660=CARTESIAN_POINT('Ctrl Pts',(-44.5079524583201,33.4673535150516,
-48.1162));
#242661=CARTESIAN_POINT('Ctrl Pts',(-45.3423250998464,32.985628245862,-48.0578666666667));
#242662=CARTESIAN_POINT('Ctrl Pts',(-46.1766977413726,32.5039029766724,
-47.9995333333334));
#242663=CARTESIAN_POINT('Ctrl Pts',(-46.1766977413726,31.5404524382932,
-47.9412));
#242664=CARTESIAN_POINT('Ctrl Pts',(-46.1766977413726,30.5770018999139,
-47.8828666666667));
#242665=CARTESIAN_POINT('Ctrl Pts',(-45.3423250998464,30.0952766307242,
-47.8245333333333));
#242666=CARTESIAN_POINT('Ctrl Pts',(-44.5079524583202,29.6135513615346,
-47.7662));
#242667=CARTESIAN_POINT('Ctrl Pts',(-43.6735798167939,30.0952766307242,
-47.7078666666667));
#242668=CARTESIAN_POINT('Ctrl Pts',(-42.8392071752677,30.5770018999139,
-47.6495333333334));
#242669=CARTESIAN_POINT('Ctrl Pts',(-42.8392071752677,31.5404524382931,
-47.5912));
#242670=CARTESIAN_POINT('Ctrl Pts',(-42.8392071752677,31.5404524382931,
-48.44995));
#242671=CARTESIAN_POINT('Ctrl Pts',(-42.8392071752677,32.5039029766724,
-48.3916166666667));
#242672=CARTESIAN_POINT('Ctrl Pts',(-43.6735798167939,32.985628245862,-48.3332833333333));
#242673=CARTESIAN_POINT('Ctrl Pts',(-44.5079524583201,33.4673535150516,
-48.27495));
#242674=CARTESIAN_POINT('Ctrl Pts',(-45.3423250998464,32.985628245862,-48.2166166666667));
#242675=CARTESIAN_POINT('Ctrl Pts',(-46.1766977413726,32.5039029766724,
-48.1582833333333));
#242676=CARTESIAN_POINT('Ctrl Pts',(-46.1766977413726,31.5404524382932,
-48.09995));
#242677=CARTESIAN_POINT('Ctrl Pts',(-46.1766977413726,30.5770018999139,
-48.0416166666667));
#242678=CARTESIAN_POINT('Ctrl Pts',(-45.3423250998464,30.0952766307242,
-47.9832833333334));
#242679=CARTESIAN_POINT('Ctrl Pts',(-44.5079524583202,29.6135513615346,
-47.92495));
#242680=CARTESIAN_POINT('Ctrl Pts',(-43.6735798167939,30.0952766307242,
-47.8666166666667));
#242681=CARTESIAN_POINT('Ctrl Pts',(-42.8392071752677,30.5770018999139,
-47.8082833333333));
#242682=CARTESIAN_POINT('Ctrl Pts',(-42.8392071752677,31.5404524382931,
-47.74995));
#242683=CARTESIAN_POINT('Origin',(-44.5079524583202,31.5404524382932,-52.920575));
#242684=CARTESIAN_POINT('',(-42.8392071752677,31.5404524382931,-49.14995));
#242685=CARTESIAN_POINT('',(-42.8392071752677,31.5404524382931,-48.9912));
#242686=CARTESIAN_POINT('',(-42.8392071752678,31.5404524382932,-52.920575));
#242687=CARTESIAN_POINT('Ctrl Pts',(-42.8392071752677,31.5404524382931,
-48.9912));
#242688=CARTESIAN_POINT('Ctrl Pts',(-42.8392071752677,32.5039029766724,
-48.9328666666667));
#242689=CARTESIAN_POINT('Ctrl Pts',(-43.6735798167939,32.985628245862,-48.8745333333333));
#242690=CARTESIAN_POINT('Ctrl Pts',(-44.5079524583201,33.4673535150516,
-48.8162));
#242691=CARTESIAN_POINT('Ctrl Pts',(-45.3423250998464,32.985628245862,-48.7578666666667));
#242692=CARTESIAN_POINT('Ctrl Pts',(-46.1766977413726,32.5039029766724,
-48.6995333333333));
#242693=CARTESIAN_POINT('Ctrl Pts',(-46.1766977413726,31.5404524382932,
-48.6412));
#242694=CARTESIAN_POINT('Ctrl Pts',(-46.1766977413726,30.5770018999139,
-48.5828666666667));
#242695=CARTESIAN_POINT('Ctrl Pts',(-45.3423250998464,30.0952766307242,
-48.5245333333333));
#242696=CARTESIAN_POINT('Ctrl Pts',(-44.5079524583202,29.6135513615346,
-48.4662));
#242697=CARTESIAN_POINT('Ctrl Pts',(-43.6735798167939,30.0952766307242,
-48.4078666666667));
#242698=CARTESIAN_POINT('Ctrl Pts',(-42.8392071752677,30.5770018999139,
-48.3495333333333));
#242699=CARTESIAN_POINT('Ctrl Pts',(-42.8392071752677,31.5404524382931,
-48.2912));
#242700=CARTESIAN_POINT('Ctrl Pts',(-42.8392071752677,31.5404524382931,
-49.14995));
#242701=CARTESIAN_POINT('Ctrl Pts',(-42.8392071752677,32.5039029766724,
-49.0916166666667));
#242702=CARTESIAN_POINT('Ctrl Pts',(-43.6735798167939,32.985628245862,-49.0332833333333));
#242703=CARTESIAN_POINT('Ctrl Pts',(-44.5079524583201,33.4673535150516,
-48.97495));
#242704=CARTESIAN_POINT('Ctrl Pts',(-45.3423250998464,32.985628245862,-48.9166166666667));
#242705=CARTESIAN_POINT('Ctrl Pts',(-46.1766977413726,32.5039029766724,
-48.8582833333333));
#242706=CARTESIAN_POINT('Ctrl Pts',(-46.1766977413726,31.5404524382932,
-48.79995));
#242707=CARTESIAN_POINT('Ctrl Pts',(-46.1766977413726,30.5770018999139,
-48.7416166666667));
#242708=CARTESIAN_POINT('Ctrl Pts',(-45.3423250998464,30.0952766307242,
-48.6832833333333));
#242709=CARTESIAN_POINT('Ctrl Pts',(-44.5079524583202,29.6135513615346,
-48.62495));
#242710=CARTESIAN_POINT('Ctrl Pts',(-43.6735798167939,30.0952766307242,
-48.5666166666667));
#242711=CARTESIAN_POINT('Ctrl Pts',(-42.8392071752677,30.5770018999139,
-48.5082833333334));
#242712=CARTESIAN_POINT('Ctrl Pts',(-42.8392071752677,31.5404524382931,
-48.44995));
#242713=CARTESIAN_POINT('Origin',(-44.5079524583202,31.5404524382932,-52.920575));
#242714=CARTESIAN_POINT('',(-42.8392071752677,31.5404524382931,-49.84995));
#242715=CARTESIAN_POINT('',(-42.8392071752677,31.5404524382931,-49.6912));
#242716=CARTESIAN_POINT('',(-42.8392071752678,31.5404524382932,-52.920575));
#242717=CARTESIAN_POINT('Ctrl Pts',(-42.8392071752677,31.5404524382931,
-49.6912));
#242718=CARTESIAN_POINT('Ctrl Pts',(-42.8392071752677,32.5039029766724,
-49.6328666666667));
#242719=CARTESIAN_POINT('Ctrl Pts',(-43.6735798167939,32.985628245862,-49.5745333333333));
#242720=CARTESIAN_POINT('Ctrl Pts',(-44.5079524583201,33.4673535150516,
-49.5162));
#242721=CARTESIAN_POINT('Ctrl Pts',(-45.3423250998464,32.985628245862,-49.4578666666667));
#242722=CARTESIAN_POINT('Ctrl Pts',(-46.1766977413726,32.5039029766724,
-49.3995333333333));
#242723=CARTESIAN_POINT('Ctrl Pts',(-46.1766977413726,31.5404524382932,
-49.3412));
#242724=CARTESIAN_POINT('Ctrl Pts',(-46.1766977413726,30.5770018999139,
-49.2828666666667));
#242725=CARTESIAN_POINT('Ctrl Pts',(-45.3423250998464,30.0952766307242,
-49.2245333333333));
#242726=CARTESIAN_POINT('Ctrl Pts',(-44.5079524583202,29.6135513615346,
-49.1662));
#242727=CARTESIAN_POINT('Ctrl Pts',(-43.6735798167939,30.0952766307242,
-49.1078666666667));
#242728=CARTESIAN_POINT('Ctrl Pts',(-42.8392071752677,30.5770018999139,
-49.0495333333334));
#242729=CARTESIAN_POINT('Ctrl Pts',(-42.8392071752677,31.5404524382931,
-48.9912));
#242730=CARTESIAN_POINT('Ctrl Pts',(-42.8392071752677,31.5404524382931,
-49.84995));
#242731=CARTESIAN_POINT('Ctrl Pts',(-42.8392071752677,32.5039029766724,
-49.7916166666667));
#242732=CARTESIAN_POINT('Ctrl Pts',(-43.6735798167939,32.985628245862,-49.7332833333333));
#242733=CARTESIAN_POINT('Ctrl Pts',(-44.5079524583201,33.4673535150516,
-49.67495));
#242734=CARTESIAN_POINT('Ctrl Pts',(-45.3423250998464,32.985628245862,-49.6166166666667));
#242735=CARTESIAN_POINT('Ctrl Pts',(-46.1766977413726,32.5039029766724,
-49.5582833333334));
#242736=CARTESIAN_POINT('Ctrl Pts',(-46.1766977413726,31.5404524382932,
-49.49995));
#242737=CARTESIAN_POINT('Ctrl Pts',(-46.1766977413726,30.5770018999139,
-49.4416166666667));
#242738=CARTESIAN_POINT('Ctrl Pts',(-45.3423250998464,30.0952766307242,
-49.3832833333334));
#242739=CARTESIAN_POINT('Ctrl Pts',(-44.5079524583202,29.6135513615346,
-49.32495));
#242740=CARTESIAN_POINT('Ctrl Pts',(-43.6735798167939,30.0952766307242,
-49.2666166666667));
#242741=CARTESIAN_POINT('Ctrl Pts',(-42.8392071752677,30.5770018999139,
-49.2082833333334));
#242742=CARTESIAN_POINT('Ctrl Pts',(-42.8392071752677,31.5404524382931,
-49.14995));
#242743=CARTESIAN_POINT('Origin',(-44.5079524583202,31.5404524382932,-52.920575));
#242744=CARTESIAN_POINT('',(-42.8392071752677,31.5404524382931,-50.54995));
#242745=CARTESIAN_POINT('',(-42.8392071752677,31.5404524382931,-50.3912));
#242746=CARTESIAN_POINT('',(-42.8392071752678,31.5404524382932,-52.920575));
#242747=CARTESIAN_POINT('Ctrl Pts',(-42.8392071752677,31.5404524382931,
-50.3912));
#242748=CARTESIAN_POINT('Ctrl Pts',(-42.8392071752677,32.5039029766724,
-50.3328666666666));
#242749=CARTESIAN_POINT('Ctrl Pts',(-43.6735798167939,32.985628245862,-50.2745333333333));
#242750=CARTESIAN_POINT('Ctrl Pts',(-44.5079524583201,33.4673535150516,
-50.2162));
#242751=CARTESIAN_POINT('Ctrl Pts',(-45.3423250998464,32.985628245862,-50.1578666666667));
#242752=CARTESIAN_POINT('Ctrl Pts',(-46.1766977413726,32.5039029766724,
-50.0995333333333));
#242753=CARTESIAN_POINT('Ctrl Pts',(-46.1766977413726,31.5404524382932,
-50.0412));
#242754=CARTESIAN_POINT('Ctrl Pts',(-46.1766977413726,30.5770018999139,
-49.9828666666667));
#242755=CARTESIAN_POINT('Ctrl Pts',(-45.3423250998464,30.0952766307242,
-49.9245333333334));
#242756=CARTESIAN_POINT('Ctrl Pts',(-44.5079524583202,29.6135513615346,
-49.8662));
#242757=CARTESIAN_POINT('Ctrl Pts',(-43.6735798167939,30.0952766307242,
-49.8078666666667));
#242758=CARTESIAN_POINT('Ctrl Pts',(-42.8392071752677,30.5770018999139,
-49.7495333333333));
#242759=CARTESIAN_POINT('Ctrl Pts',(-42.8392071752677,31.5404524382931,
-49.6912));
#242760=CARTESIAN_POINT('Ctrl Pts',(-42.8392071752677,31.5404524382931,
-50.54995));
#242761=CARTESIAN_POINT('Ctrl Pts',(-42.8392071752677,32.5039029766724,
-50.4916166666667));
#242762=CARTESIAN_POINT('Ctrl Pts',(-43.6735798167939,32.985628245862,-50.4332833333333));
#242763=CARTESIAN_POINT('Ctrl Pts',(-44.5079524583201,33.4673535150516,
-50.37495));
#242764=CARTESIAN_POINT('Ctrl Pts',(-45.3423250998464,32.985628245862,-50.3166166666667));
#242765=CARTESIAN_POINT('Ctrl Pts',(-46.1766977413726,32.5039029766724,
-50.2582833333334));
#242766=CARTESIAN_POINT('Ctrl Pts',(-46.1766977413726,31.5404524382932,
-50.19995));
#242767=CARTESIAN_POINT('Ctrl Pts',(-46.1766977413726,30.5770018999139,
-50.1416166666667));
#242768=CARTESIAN_POINT('Ctrl Pts',(-45.3423250998464,30.0952766307242,
-50.0832833333333));
#242769=CARTESIAN_POINT('Ctrl Pts',(-44.5079524583202,29.6135513615346,
-50.02495));
#242770=CARTESIAN_POINT('Ctrl Pts',(-43.6735798167939,30.0952766307242,
-49.9666166666667));
#242771=CARTESIAN_POINT('Ctrl Pts',(-42.8392071752677,30.5770018999139,
-49.9082833333334));
#242772=CARTESIAN_POINT('Ctrl Pts',(-42.8392071752677,31.5404524382931,
-49.84995));
#242773=CARTESIAN_POINT('Origin',(-44.5079524583202,31.5404524382932,-52.920575));
#242774=CARTESIAN_POINT('',(-42.8392071752677,31.5404524382931,-51.24995));
#242775=CARTESIAN_POINT('',(-42.8392071752677,31.5404524382931,-51.0912));
#242776=CARTESIAN_POINT('',(-42.8392071752678,31.5404524382932,-52.920575));
#242777=CARTESIAN_POINT('Ctrl Pts',(-42.8392071752677,31.5404524382931,
-51.0912));
#242778=CARTESIAN_POINT('Ctrl Pts',(-42.8392071752677,32.5039029766724,
-51.0328666666667));
#242779=CARTESIAN_POINT('Ctrl Pts',(-43.6735798167939,32.985628245862,-50.9745333333333));
#242780=CARTESIAN_POINT('Ctrl Pts',(-44.5079524583201,33.4673535150516,
-50.9162));
#242781=CARTESIAN_POINT('Ctrl Pts',(-45.3423250998464,32.985628245862,-50.8578666666667));
#242782=CARTESIAN_POINT('Ctrl Pts',(-46.1766977413726,32.5039029766724,
-50.7995333333333));
#242783=CARTESIAN_POINT('Ctrl Pts',(-46.1766977413726,31.5404524382932,
-50.7412));
#242784=CARTESIAN_POINT('Ctrl Pts',(-46.1766977413726,30.5770018999139,
-50.6828666666667));
#242785=CARTESIAN_POINT('Ctrl Pts',(-45.3423250998464,30.0952766307242,
-50.6245333333333));
#242786=CARTESIAN_POINT('Ctrl Pts',(-44.5079524583202,29.6135513615346,
-50.5662));
#242787=CARTESIAN_POINT('Ctrl Pts',(-43.6735798167939,30.0952766307242,
-50.5078666666667));
#242788=CARTESIAN_POINT('Ctrl Pts',(-42.8392071752677,30.5770018999139,
-50.4495333333333));
#242789=CARTESIAN_POINT('Ctrl Pts',(-42.8392071752677,31.5404524382931,
-50.3912));
#242790=CARTESIAN_POINT('Ctrl Pts',(-42.8392071752677,31.5404524382931,
-51.24995));
#242791=CARTESIAN_POINT('Ctrl Pts',(-42.8392071752677,32.5039029766724,
-51.1916166666667));
#242792=CARTESIAN_POINT('Ctrl Pts',(-43.6735798167939,32.985628245862,-51.1332833333333));
#242793=CARTESIAN_POINT('Ctrl Pts',(-44.5079524583201,33.4673535150516,
-51.07495));
#242794=CARTESIAN_POINT('Ctrl Pts',(-45.3423250998464,32.985628245862,-51.0166166666667));
#242795=CARTESIAN_POINT('Ctrl Pts',(-46.1766977413726,32.5039029766724,
-50.9582833333334));
#242796=CARTESIAN_POINT('Ctrl Pts',(-46.1766977413726,31.5404524382932,
-50.89995));
#242797=CARTESIAN_POINT('Ctrl Pts',(-46.1766977413726,30.5770018999139,
-50.8416166666667));
#242798=CARTESIAN_POINT('Ctrl Pts',(-45.3423250998464,30.0952766307242,
-50.7832833333333));
#242799=CARTESIAN_POINT('Ctrl Pts',(-44.5079524583202,29.6135513615346,
-50.72495));
#242800=CARTESIAN_POINT('Ctrl Pts',(-43.6735798167939,30.0952766307242,
-50.6666166666667));
#242801=CARTESIAN_POINT('Ctrl Pts',(-42.8392071752677,30.5770018999139,
-50.6082833333334));
#242802=CARTESIAN_POINT('Ctrl Pts',(-42.8392071752677,31.5404524382931,
-50.54995));
#242803=CARTESIAN_POINT('Origin',(-44.5079524583202,31.5404524382932,-52.920575));
#242804=CARTESIAN_POINT('',(-42.8392071752677,31.5404524382931,-51.94995));
#242805=CARTESIAN_POINT('',(-42.8392071752677,31.5404524382931,-51.7912));
#242806=CARTESIAN_POINT('',(-42.8392071752678,31.5404524382932,-52.920575));
#242807=CARTESIAN_POINT('Ctrl Pts',(-42.8392071752677,31.5404524382931,
-51.7912));
#242808=CARTESIAN_POINT('Ctrl Pts',(-42.8392071752677,32.5039029766724,
-51.7328666666667));
#242809=CARTESIAN_POINT('Ctrl Pts',(-43.6735798167939,32.985628245862,-51.6745333333333));
#242810=CARTESIAN_POINT('Ctrl Pts',(-44.5079524583201,33.4673535150516,
-51.6162));
#242811=CARTESIAN_POINT('Ctrl Pts',(-45.3423250998464,32.985628245862,-51.5578666666667));
#242812=CARTESIAN_POINT('Ctrl Pts',(-46.1766977413726,32.5039029766724,
-51.4995333333333));
#242813=CARTESIAN_POINT('Ctrl Pts',(-46.1766977413726,31.5404524382932,
-51.4412));
#242814=CARTESIAN_POINT('Ctrl Pts',(-46.1766977413726,30.5770018999139,
-51.3828666666667));
#242815=CARTESIAN_POINT('Ctrl Pts',(-45.3423250998464,30.0952766307242,
-51.3245333333334));
#242816=CARTESIAN_POINT('Ctrl Pts',(-44.5079524583202,29.6135513615346,
-51.2662));
#242817=CARTESIAN_POINT('Ctrl Pts',(-43.6735798167939,30.0952766307242,
-51.2078666666667));
#242818=CARTESIAN_POINT('Ctrl Pts',(-42.8392071752677,30.5770018999139,
-51.1495333333333));
#242819=CARTESIAN_POINT('Ctrl Pts',(-42.8392071752677,31.5404524382931,
-51.0912));
#242820=CARTESIAN_POINT('Ctrl Pts',(-42.8392071752677,31.5404524382931,
-51.94995));
#242821=CARTESIAN_POINT('Ctrl Pts',(-42.8392071752677,32.5039029766724,
-51.8916166666666));
#242822=CARTESIAN_POINT('Ctrl Pts',(-43.6735798167939,32.985628245862,-51.8332833333333));
#242823=CARTESIAN_POINT('Ctrl Pts',(-44.5079524583201,33.4673535150516,
-51.77495));
#242824=CARTESIAN_POINT('Ctrl Pts',(-45.3423250998464,32.985628245862,-51.7166166666667));
#242825=CARTESIAN_POINT('Ctrl Pts',(-46.1766977413726,32.5039029766724,
-51.6582833333333));
#242826=CARTESIAN_POINT('Ctrl Pts',(-46.1766977413726,31.5404524382932,
-51.59995));
#242827=CARTESIAN_POINT('Ctrl Pts',(-46.1766977413726,30.5770018999139,
-51.5416166666667));
#242828=CARTESIAN_POINT('Ctrl Pts',(-45.3423250998464,30.0952766307242,
-51.4832833333333));
#242829=CARTESIAN_POINT('Ctrl Pts',(-44.5079524583202,29.6135513615346,
-51.42495));
#242830=CARTESIAN_POINT('Ctrl Pts',(-43.6735798167939,30.0952766307242,
-51.3666166666667));
#242831=CARTESIAN_POINT('Ctrl Pts',(-42.8392071752677,30.5770018999139,
-51.3082833333333));
#242832=CARTESIAN_POINT('Ctrl Pts',(-42.8392071752677,31.5404524382931,
-51.24995));
#242833=CARTESIAN_POINT('Origin',(-44.5079524583202,31.5404524382932,-52.920575));
#242834=CARTESIAN_POINT('',(-42.8392071752677,31.5404524382931,-52.64995));
#242835=CARTESIAN_POINT('',(-42.8392071752677,31.5404524382931,-52.4912));
#242836=CARTESIAN_POINT('',(-42.8392071752678,31.5404524382932,-52.920575));
#242837=CARTESIAN_POINT('',(-44.2755200796091,29.8879736913688,-52.64995));
#242838=CARTESIAN_POINT('Origin',(-44.5079524583202,31.5404524382932,-52.64995));
#242839=CARTESIAN_POINT('Ctrl Pts',(-44.2755200796091,29.8879736913688,
-52.64995));
#242840=CARTESIAN_POINT('Ctrl Pts',(-43.9544082597714,29.9331402535751,
-52.6275001713604));
#242841=CARTESIAN_POINT('Ctrl Pts',(-43.6735798167939,30.0952766307242,
-52.6078666666667));
#242842=CARTESIAN_POINT('Ctrl Pts',(-42.8392071752677,30.5770018999139,
-52.5495333333333));
#242843=CARTESIAN_POINT('Ctrl Pts',(-42.8392071752677,31.5404524382931,
-52.4912));
#242844=CARTESIAN_POINT('Origin',(44.5079524583208,31.5404524382925,-52.920575));
#242845=CARTESIAN_POINT('',(44.5079524583208,29.87170715524,-40.04995));
#242846=CARTESIAN_POINT('',(44.5079524583208,29.87170715524,-39.8912));
#242847=CARTESIAN_POINT('',(44.5079524583209,29.8717071552401,-52.920575));
#242848=CARTESIAN_POINT('',(45.3258959266108,30.0859149508445,-39.8341886424312));
#242849=CARTESIAN_POINT('Ctrl Pts',(44.5079524583208,29.87170715524,-39.8912));
#242850=CARTESIAN_POINT('Ctrl Pts',(44.9449731845273,29.87170715524,-39.8647400265194));
#242851=CARTESIAN_POINT('Ctrl Pts',(45.3258959266108,30.0859149508445,-39.8341886424312));
#242852=CARTESIAN_POINT('',(45.7222548898542,30.3958213079794,-39.958107375254));
#242853=CARTESIAN_POINT('Ctrl Pts',(45.7222548898542,30.3958213079794,-39.9581073752541));
#242854=CARTESIAN_POINT('Ctrl Pts',(45.6645243102482,30.3345767888213,-39.937000346169));
#242855=CARTESIAN_POINT('Ctrl Pts',(45.6022203991058,30.2777619587592,-39.9159679625448));
#242856=CARTESIAN_POINT('Ctrl Pts',(45.4695708655712,30.1740414353458,-39.8744792788644));
#242857=CARTESIAN_POINT('Ctrl Pts',(45.3994027590463,30.1272507252637,-39.8540736326231));
#242858=CARTESIAN_POINT('Ctrl Pts',(45.3258959266108,30.0859149508445,-39.8341886424312));
#242859=CARTESIAN_POINT('Ctrl Pts',(44.5079524583208,29.87170715524,-40.04995));
#242860=CARTESIAN_POINT('Ctrl Pts',(45.22821208842,29.87170715524,-40.0063409682797));
#242861=CARTESIAN_POINT('Ctrl Pts',(45.7222548898542,30.3958213079794,-39.958107375254));
#242862=CARTESIAN_POINT('Origin',(44.5079524583208,31.5404524382925,-52.920575));
#242863=CARTESIAN_POINT('',(44.5079524583208,29.87170715524,-40.74995));
#242864=CARTESIAN_POINT('',(44.5079524583208,29.87170715524,-40.5912));
#242865=CARTESIAN_POINT('',(44.5079524583209,29.8717071552401,-52.920575));
#242866=CARTESIAN_POINT('',(45.9506566843147,32.3790914166432,-40.3575678858381));
#242867=CARTESIAN_POINT('Ctrl Pts',(44.5079524583208,29.87170715524,-40.5912));
#242868=CARTESIAN_POINT('Ctrl Pts',(45.4714029967,29.87170715524,-40.5328666666667));
#242869=CARTESIAN_POINT('Ctrl Pts',(45.9531282658897,30.7060797967663,-40.4745333333334));
#242870=CARTESIAN_POINT('Ctrl Pts',(46.4348535350793,31.5404524382925,-40.4162));
#242871=CARTESIAN_POINT('Ctrl Pts',(45.9531282658897,32.3748250798187,-40.3578666666667));
#242872=CARTESIAN_POINT('Ctrl Pts',(45.9518956264848,32.3769600738953,-40.3577174032382));
#242873=CARTESIAN_POINT('Ctrl Pts',(45.9506566843147,32.3790914166432,-40.3575678858381));
#242874=CARTESIAN_POINT('',(44.4689444465313,33.2087417401602,-40.2388222710491));
#242875=CARTESIAN_POINT('Ctrl Pts',(44.4689444465313,33.2087417401601,-40.2388222710491));
#242876=CARTESIAN_POINT('Ctrl Pts',(44.6155079330583,33.2121686938689,-40.2660845126688));
#242877=CARTESIAN_POINT('Ctrl Pts',(44.762424616678,33.1962849161559,-40.2899383159198));
#242878=CARTESIAN_POINT('Ctrl Pts',(45.0501580461342,33.1256303733612,-40.3294880310719));
#242879=CARTESIAN_POINT('Ctrl Pts',(45.1895314514539,33.0709802808554,-40.3449374316991));
#242880=CARTESIAN_POINT('Ctrl Pts',(45.450238361729,32.9257274737428,-40.3659945174197));
#242881=CARTESIAN_POINT('Ctrl Pts',(45.5702035368922,32.8360707980695,-40.3715333771918));
#242882=CARTESIAN_POINT('Ctrl Pts',(45.6900480373997,32.7184621594941,-40.3719335667203));
#242883=CARTESIAN_POINT('Ctrl Pts',(45.703109839145,32.7052081033347,-40.3718982256622));
#242884=CARTESIAN_POINT('Ctrl Pts',(45.8062679295088,32.596969205699,-40.3709718752492));
#242885=CARTESIAN_POINT('Ctrl Pts',(45.8850264885628,32.4919945408818,-40.3661895545283));
#242886=CARTESIAN_POINT('Ctrl Pts',(45.9506566843147,32.3790914166432,-40.357567885838));
#242887=CARTESIAN_POINT('Ctrl Pts',(44.4689444465313,33.2087417401602,-40.2388222710491));
#242888=CARTESIAN_POINT('Ctrl Pts',(43.5315846498844,33.1868243533108,-40.1813024817086));
#242889=CARTESIAN_POINT('Ctrl Pts',(43.0627766507519,32.3748250798187,-40.1245333333334));
#242890=CARTESIAN_POINT('Ctrl Pts',(42.5810513815623,31.5404524382925,-40.0662));
#242891=CARTESIAN_POINT('Ctrl Pts',(43.0627766507519,30.7060797967663,-40.0078666666667));
#242892=CARTESIAN_POINT('Ctrl Pts',(43.5445019199415,29.87170715524,-39.9495333333333));
#242893=CARTESIAN_POINT('Ctrl Pts',(44.5079524583208,29.87170715524,-39.8912));
#242894=CARTESIAN_POINT('Ctrl Pts',(44.5079524583208,29.87170715524,-40.74995));
#242895=CARTESIAN_POINT('Ctrl Pts',(45.4714029967,29.87170715524,-40.6916166666667));
#242896=CARTESIAN_POINT('Ctrl Pts',(45.9531282658897,30.7060797967663,-40.6332833333334));
#242897=CARTESIAN_POINT('Ctrl Pts',(46.4348535350793,31.5404524382925,-40.57495));
#242898=CARTESIAN_POINT('Ctrl Pts',(45.9531282658897,32.3748250798187,-40.5166166666666));
#242899=CARTESIAN_POINT('Ctrl Pts',(45.4714029967,33.2091977213449,-40.4582833333333));
#242900=CARTESIAN_POINT('Ctrl Pts',(44.5079524583208,33.2091977213449,-40.39995));
#242901=CARTESIAN_POINT('Ctrl Pts',(43.5445019199415,33.2091977213449,-40.3416166666667));
#242902=CARTESIAN_POINT('Ctrl Pts',(43.0627766507519,32.3748250798187,-40.2832833333334));
#242903=CARTESIAN_POINT('Ctrl Pts',(42.5810513815623,31.5404524382925,-40.22495));
#242904=CARTESIAN_POINT('Ctrl Pts',(43.0627766507519,30.7060797967663,-40.1666166666667));
#242905=CARTESIAN_POINT('Ctrl Pts',(43.5445019199415,29.87170715524,-40.1082833333334));
#242906=CARTESIAN_POINT('Ctrl Pts',(44.5079524583208,29.87170715524,-40.04995));
#242907=CARTESIAN_POINT('Origin',(44.5079524583208,31.5404524382925,-52.920575));
#242908=CARTESIAN_POINT('',(44.5079524583208,29.87170715524,-41.44995));
#242909=CARTESIAN_POINT('',(44.5079524583208,29.87170715524,-41.2912));
#242910=CARTESIAN_POINT('',(44.5079524583209,29.8717071552401,-52.920575));
#242911=CARTESIAN_POINT('Ctrl Pts',(44.5079524583208,29.87170715524,-41.2912));
#242912=CARTESIAN_POINT('Ctrl Pts',(45.4714029967,29.87170715524,-41.2328666666667));
#242913=CARTESIAN_POINT('Ctrl Pts',(45.9531282658897,30.7060797967663,-41.1745333333334));
#242914=CARTESIAN_POINT('Ctrl Pts',(46.4348535350793,31.5404524382925,-41.1162));
#242915=CARTESIAN_POINT('Ctrl Pts',(45.9531282658897,32.3748250798187,-41.0578666666667));
#242916=CARTESIAN_POINT('Ctrl Pts',(45.4714029967,33.2091977213449,-40.9995333333333));
#242917=CARTESIAN_POINT('Ctrl Pts',(44.5079524583208,33.2091977213449,-40.9412));
#242918=CARTESIAN_POINT('Ctrl Pts',(43.5445019199415,33.2091977213449,-40.8828666666667));
#242919=CARTESIAN_POINT('Ctrl Pts',(43.0627766507519,32.3748250798187,-40.8245333333333));
#242920=CARTESIAN_POINT('Ctrl Pts',(42.5810513815623,31.5404524382925,-40.7662));
#242921=CARTESIAN_POINT('Ctrl Pts',(43.0627766507519,30.7060797967663,-40.7078666666667));
#242922=CARTESIAN_POINT('Ctrl Pts',(43.5445019199415,29.87170715524,-40.6495333333333));
#242923=CARTESIAN_POINT('Ctrl Pts',(44.5079524583208,29.87170715524,-40.5912));
#242924=CARTESIAN_POINT('Ctrl Pts',(44.5079524583208,29.87170715524,-41.44995));
#242925=CARTESIAN_POINT('Ctrl Pts',(45.4714029967,29.87170715524,-41.3916166666667));
#242926=CARTESIAN_POINT('Ctrl Pts',(45.9531282658897,30.7060797967663,-41.3332833333334));
#242927=CARTESIAN_POINT('Ctrl Pts',(46.4348535350793,31.5404524382925,-41.27495));
#242928=CARTESIAN_POINT('Ctrl Pts',(45.9531282658897,32.3748250798187,-41.2166166666667));
#242929=CARTESIAN_POINT('Ctrl Pts',(45.4714029967,33.2091977213449,-41.1582833333333));
#242930=CARTESIAN_POINT('Ctrl Pts',(44.5079524583208,33.2091977213449,-41.09995));
#242931=CARTESIAN_POINT('Ctrl Pts',(43.5445019199415,33.2091977213449,-41.0416166666667));
#242932=CARTESIAN_POINT('Ctrl Pts',(43.0627766507519,32.3748250798187,-40.9832833333333));
#242933=CARTESIAN_POINT('Ctrl Pts',(42.5810513815623,31.5404524382925,-40.92495));
#242934=CARTESIAN_POINT('Ctrl Pts',(43.0627766507519,30.7060797967663,-40.8666166666667));
#242935=CARTESIAN_POINT('Ctrl Pts',(43.5445019199415,29.87170715524,-40.8082833333334));
#242936=CARTESIAN_POINT('Ctrl Pts',(44.5079524583208,29.87170715524,-40.74995));
#242937=CARTESIAN_POINT('Origin',(44.5079524583208,31.5404524382925,-52.920575));
#242938=CARTESIAN_POINT('',(44.5079524583208,29.87170715524,-42.14995));
#242939=CARTESIAN_POINT('',(44.5079524583208,29.87170715524,-41.9912));
#242940=CARTESIAN_POINT('',(44.5079524583209,29.8717071552401,-52.920575));
#242941=CARTESIAN_POINT('Ctrl Pts',(44.5079524583208,29.87170715524,-41.9912));
#242942=CARTESIAN_POINT('Ctrl Pts',(45.4714029967,29.87170715524,-41.9328666666667));
#242943=CARTESIAN_POINT('Ctrl Pts',(45.9531282658897,30.7060797967663,-41.8745333333334));
#242944=CARTESIAN_POINT('Ctrl Pts',(46.4348535350793,31.5404524382925,-41.8162));
#242945=CARTESIAN_POINT('Ctrl Pts',(45.9531282658897,32.3748250798187,-41.7578666666667));
#242946=CARTESIAN_POINT('Ctrl Pts',(45.4714029967,33.2091977213449,-41.6995333333334));
#242947=CARTESIAN_POINT('Ctrl Pts',(44.5079524583208,33.2091977213449,-41.6412));
#242948=CARTESIAN_POINT('Ctrl Pts',(43.5445019199415,33.2091977213449,-41.5828666666667));
#242949=CARTESIAN_POINT('Ctrl Pts',(43.0627766507519,32.3748250798187,-41.5245333333334));
#242950=CARTESIAN_POINT('Ctrl Pts',(42.5810513815623,31.5404524382925,-41.4662));
#242951=CARTESIAN_POINT('Ctrl Pts',(43.0627766507519,30.7060797967663,-41.4078666666667));
#242952=CARTESIAN_POINT('Ctrl Pts',(43.5445019199415,29.87170715524,-41.3495333333333));
#242953=CARTESIAN_POINT('Ctrl Pts',(44.5079524583208,29.87170715524,-41.2912));
#242954=CARTESIAN_POINT('Ctrl Pts',(44.5079524583208,29.87170715524,-42.14995));
#242955=CARTESIAN_POINT('Ctrl Pts',(45.4714029967,29.87170715524,-42.0916166666667));
#242956=CARTESIAN_POINT('Ctrl Pts',(45.9531282658897,30.7060797967663,-42.0332833333334));
#242957=CARTESIAN_POINT('Ctrl Pts',(46.4348535350793,31.5404524382925,-41.97495));
#242958=CARTESIAN_POINT('Ctrl Pts',(45.9531282658897,32.3748250798187,-41.9166166666666));
#242959=CARTESIAN_POINT('Ctrl Pts',(45.4714029967,33.2091977213449,-41.8582833333333));
#242960=CARTESIAN_POINT('Ctrl Pts',(44.5079524583208,33.2091977213449,-41.79995));
#242961=CARTESIAN_POINT('Ctrl Pts',(43.5445019199415,33.2091977213449,-41.7416166666666));
#242962=CARTESIAN_POINT('Ctrl Pts',(43.0627766507519,32.3748250798187,-41.6832833333333));
#242963=CARTESIAN_POINT('Ctrl Pts',(42.5810513815623,31.5404524382925,-41.62495));
#242964=CARTESIAN_POINT('Ctrl Pts',(43.0627766507519,30.7060797967663,-41.5666166666667));
#242965=CARTESIAN_POINT('Ctrl Pts',(43.5445019199415,29.87170715524,-41.5082833333334));
#242966=CARTESIAN_POINT('Ctrl Pts',(44.5079524583208,29.87170715524,-41.44995));
#242967=CARTESIAN_POINT('Origin',(44.5079524583208,31.5404524382925,-52.920575));
#242968=CARTESIAN_POINT('',(44.5079524583208,29.87170715524,-42.84995));
#242969=CARTESIAN_POINT('',(44.5079524583208,29.87170715524,-42.6912));
#242970=CARTESIAN_POINT('',(44.5079524583209,29.8717071552401,-52.920575));
#242971=CARTESIAN_POINT('Ctrl Pts',(44.5079524583208,29.87170715524,-42.6912));
#242972=CARTESIAN_POINT('Ctrl Pts',(45.4714029967,29.87170715524,-42.6328666666667));
#242973=CARTESIAN_POINT('Ctrl Pts',(45.9531282658897,30.7060797967663,-42.5745333333333));
#242974=CARTESIAN_POINT('Ctrl Pts',(46.4348535350793,31.5404524382925,-42.5162));
#242975=CARTESIAN_POINT('Ctrl Pts',(45.9531282658897,32.3748250798187,-42.4578666666667));
#242976=CARTESIAN_POINT('Ctrl Pts',(45.4714029967,33.2091977213449,-42.3995333333334));
#242977=CARTESIAN_POINT('Ctrl Pts',(44.5079524583208,33.2091977213449,-42.3412));
#242978=CARTESIAN_POINT('Ctrl Pts',(43.5445019199415,33.2091977213449,-42.2828666666667));
#242979=CARTESIAN_POINT('Ctrl Pts',(43.0627766507519,32.3748250798187,-42.2245333333333));
#242980=CARTESIAN_POINT('Ctrl Pts',(42.5810513815623,31.5404524382925,-42.1662));
#242981=CARTESIAN_POINT('Ctrl Pts',(43.0627766507519,30.7060797967663,-42.1078666666667));
#242982=CARTESIAN_POINT('Ctrl Pts',(43.5445019199415,29.87170715524,-42.0495333333334));
#242983=CARTESIAN_POINT('Ctrl Pts',(44.5079524583208,29.87170715524,-41.9912));
#242984=CARTESIAN_POINT('Ctrl Pts',(44.5079524583208,29.87170715524,-42.84995));
#242985=CARTESIAN_POINT('Ctrl Pts',(45.4714029967,29.87170715524,-42.7916166666667));
#242986=CARTESIAN_POINT('Ctrl Pts',(45.9531282658897,30.7060797967663,-42.7332833333334));
#242987=CARTESIAN_POINT('Ctrl Pts',(46.4348535350793,31.5404524382925,-42.67495));
#242988=CARTESIAN_POINT('Ctrl Pts',(45.9531282658897,32.3748250798187,-42.6166166666667));
#242989=CARTESIAN_POINT('Ctrl Pts',(45.4714029967,33.2091977213449,-42.5582833333333));
#242990=CARTESIAN_POINT('Ctrl Pts',(44.5079524583208,33.2091977213449,-42.49995));
#242991=CARTESIAN_POINT('Ctrl Pts',(43.5445019199415,33.2091977213449,-42.4416166666666));
#242992=CARTESIAN_POINT('Ctrl Pts',(43.0627766507519,32.3748250798187,-42.3832833333333));
#242993=CARTESIAN_POINT('Ctrl Pts',(42.5810513815623,31.5404524382925,-42.32495));
#242994=CARTESIAN_POINT('Ctrl Pts',(43.0627766507519,30.7060797967663,-42.2666166666667));
#242995=CARTESIAN_POINT('Ctrl Pts',(43.5445019199415,29.87170715524,-42.2082833333333));
#242996=CARTESIAN_POINT('Ctrl Pts',(44.5079524583208,29.87170715524,-42.14995));
#242997=CARTESIAN_POINT('Origin',(44.5079524583208,31.5404524382925,-52.920575));
#242998=CARTESIAN_POINT('',(44.5079524583208,29.87170715524,-43.54995));
#242999=CARTESIAN_POINT('',(44.5079524583208,29.87170715524,-43.3912));
#243000=CARTESIAN_POINT('',(44.5079524583209,29.8717071552401,-52.920575));
#243001=CARTESIAN_POINT('Ctrl Pts',(44.5079524583208,29.87170715524,-43.3912));
#243002=CARTESIAN_POINT('Ctrl Pts',(45.4714029967,29.87170715524,-43.3328666666667));
#243003=CARTESIAN_POINT('Ctrl Pts',(45.9531282658897,30.7060797967663,-43.2745333333334));
#243004=CARTESIAN_POINT('Ctrl Pts',(46.4348535350793,31.5404524382925,-43.2162));
#243005=CARTESIAN_POINT('Ctrl Pts',(45.9531282658897,32.3748250798187,-43.1578666666667));
#243006=CARTESIAN_POINT('Ctrl Pts',(45.4714029967,33.2091977213449,-43.0995333333334));
#243007=CARTESIAN_POINT('Ctrl Pts',(44.5079524583208,33.2091977213449,-43.0412));
#243008=CARTESIAN_POINT('Ctrl Pts',(43.5445019199415,33.2091977213449,-42.9828666666667));
#243009=CARTESIAN_POINT('Ctrl Pts',(43.0627766507519,32.3748250798187,-42.9245333333334));
#243010=CARTESIAN_POINT('Ctrl Pts',(42.5810513815623,31.5404524382925,-42.8662));
#243011=CARTESIAN_POINT('Ctrl Pts',(43.0627766507519,30.7060797967663,-42.8078666666667));
#243012=CARTESIAN_POINT('Ctrl Pts',(43.5445019199415,29.87170715524,-42.7495333333334));
#243013=CARTESIAN_POINT('Ctrl Pts',(44.5079524583208,29.87170715524,-42.6912));
#243014=CARTESIAN_POINT('Ctrl Pts',(44.5079524583208,29.87170715524,-43.54995));
#243015=CARTESIAN_POINT('Ctrl Pts',(45.4714029967,29.87170715524,-43.4916166666667));
#243016=CARTESIAN_POINT('Ctrl Pts',(45.9531282658897,30.7060797967663,-43.4332833333333));
#243017=CARTESIAN_POINT('Ctrl Pts',(46.4348535350793,31.5404524382925,-43.37495));
#243018=CARTESIAN_POINT('Ctrl Pts',(45.9531282658897,32.3748250798187,-43.3166166666667));
#243019=CARTESIAN_POINT('Ctrl Pts',(45.4714029967,33.2091977213449,-43.2582833333333));
#243020=CARTESIAN_POINT('Ctrl Pts',(44.5079524583208,33.2091977213449,-43.19995));
#243021=CARTESIAN_POINT('Ctrl Pts',(43.5445019199415,33.2091977213449,-43.1416166666666));
#243022=CARTESIAN_POINT('Ctrl Pts',(43.0627766507519,32.3748250798187,-43.0832833333333));
#243023=CARTESIAN_POINT('Ctrl Pts',(42.5810513815623,31.5404524382925,-43.02495));
#243024=CARTESIAN_POINT('Ctrl Pts',(43.0627766507519,30.7060797967663,-42.9666166666667));
#243025=CARTESIAN_POINT('Ctrl Pts',(43.5445019199415,29.87170715524,-42.9082833333333));
#243026=CARTESIAN_POINT('Ctrl Pts',(44.5079524583208,29.87170715524,-42.84995));
#243027=CARTESIAN_POINT('Origin',(44.5079524583208,31.5404524382925,-52.920575));
#243028=CARTESIAN_POINT('',(44.5079524583208,29.87170715524,-44.24995));
#243029=CARTESIAN_POINT('',(44.5079524583208,29.87170715524,-44.0912));
#243030=CARTESIAN_POINT('',(44.5079524583209,29.8717071552401,-52.920575));
#243031=CARTESIAN_POINT('Ctrl Pts',(44.5079524583208,29.87170715524,-44.0912));
#243032=CARTESIAN_POINT('Ctrl Pts',(45.4714029967,29.87170715524,-44.0328666666667));
#243033=CARTESIAN_POINT('Ctrl Pts',(45.9531282658897,30.7060797967663,-43.9745333333333));
#243034=CARTESIAN_POINT('Ctrl Pts',(46.4348535350793,31.5404524382925,-43.9162));
#243035=CARTESIAN_POINT('Ctrl Pts',(45.9531282658897,32.3748250798187,-43.8578666666667));
#243036=CARTESIAN_POINT('Ctrl Pts',(45.4714029967,33.2091977213449,-43.7995333333334));
#243037=CARTESIAN_POINT('Ctrl Pts',(44.5079524583208,33.2091977213449,-43.7412));
#243038=CARTESIAN_POINT('Ctrl Pts',(43.5445019199415,33.2091977213449,-43.6828666666667));
#243039=CARTESIAN_POINT('Ctrl Pts',(43.0627766507519,32.3748250798187,-43.6245333333333));
#243040=CARTESIAN_POINT('Ctrl Pts',(42.5810513815623,31.5404524382925,-43.5662));
#243041=CARTESIAN_POINT('Ctrl Pts',(43.0627766507519,30.7060797967663,-43.5078666666667));
#243042=CARTESIAN_POINT('Ctrl Pts',(43.5445019199415,29.87170715524,-43.4495333333334));
#243043=CARTESIAN_POINT('Ctrl Pts',(44.5079524583208,29.87170715524,-43.3912));
#243044=CARTESIAN_POINT('Ctrl Pts',(44.5079524583208,29.87170715524,-44.24995));
#243045=CARTESIAN_POINT('Ctrl Pts',(45.4714029967,29.87170715524,-44.1916166666667));
#243046=CARTESIAN_POINT('Ctrl Pts',(45.9531282658897,30.7060797967663,-44.1332833333334));
#243047=CARTESIAN_POINT('Ctrl Pts',(46.4348535350793,31.5404524382925,-44.07495));
#243048=CARTESIAN_POINT('Ctrl Pts',(45.9531282658897,32.3748250798187,-44.0166166666667));
#243049=CARTESIAN_POINT('Ctrl Pts',(45.4714029967,33.2091977213449,-43.9582833333334));
#243050=CARTESIAN_POINT('Ctrl Pts',(44.5079524583208,33.2091977213449,-43.89995));
#243051=CARTESIAN_POINT('Ctrl Pts',(43.5445019199415,33.2091977213449,-43.8416166666667));
#243052=CARTESIAN_POINT('Ctrl Pts',(43.0627766507519,32.3748250798187,-43.7832833333334));
#243053=CARTESIAN_POINT('Ctrl Pts',(42.5810513815623,31.5404524382925,-43.72495));
#243054=CARTESIAN_POINT('Ctrl Pts',(43.0627766507519,30.7060797967663,-43.6666166666667));
#243055=CARTESIAN_POINT('Ctrl Pts',(43.5445019199415,29.87170715524,-43.6082833333333));
#243056=CARTESIAN_POINT('Ctrl Pts',(44.5079524583208,29.87170715524,-43.54995));
#243057=CARTESIAN_POINT('Origin',(44.5079524583208,31.5404524382925,-52.920575));
#243058=CARTESIAN_POINT('',(44.5079524583208,29.87170715524,-44.94995));
#243059=CARTESIAN_POINT('',(44.5079524583208,29.87170715524,-44.7912));
#243060=CARTESIAN_POINT('',(44.5079524583209,29.8717071552401,-52.920575));
#243061=CARTESIAN_POINT('Ctrl Pts',(44.5079524583208,29.87170715524,-44.7912));
#243062=CARTESIAN_POINT('Ctrl Pts',(45.4714029967,29.87170715524,-44.7328666666667));
#243063=CARTESIAN_POINT('Ctrl Pts',(45.9531282658897,30.7060797967663,-44.6745333333334));
#243064=CARTESIAN_POINT('Ctrl Pts',(46.4348535350793,31.5404524382925,-44.6162));
#243065=CARTESIAN_POINT('Ctrl Pts',(45.9531282658897,32.3748250798187,-44.5578666666667));
#243066=CARTESIAN_POINT('Ctrl Pts',(45.4714029967,33.2091977213449,-44.4995333333333));
#243067=CARTESIAN_POINT('Ctrl Pts',(44.5079524583208,33.2091977213449,-44.4412));
#243068=CARTESIAN_POINT('Ctrl Pts',(43.5445019199415,33.2091977213449,-44.3828666666667));
#243069=CARTESIAN_POINT('Ctrl Pts',(43.0627766507519,32.3748250798187,-44.3245333333334));
#243070=CARTESIAN_POINT('Ctrl Pts',(42.5810513815623,31.5404524382925,-44.2662));
#243071=CARTESIAN_POINT('Ctrl Pts',(43.0627766507519,30.7060797967663,-44.2078666666667));
#243072=CARTESIAN_POINT('Ctrl Pts',(43.5445019199415,29.87170715524,-44.1495333333334));
#243073=CARTESIAN_POINT('Ctrl Pts',(44.5079524583208,29.87170715524,-44.0912));
#243074=CARTESIAN_POINT('Ctrl Pts',(44.5079524583208,29.87170715524,-44.94995));
#243075=CARTESIAN_POINT('Ctrl Pts',(45.4714029967,29.87170715524,-44.8916166666667));
#243076=CARTESIAN_POINT('Ctrl Pts',(45.9531282658897,30.7060797967663,-44.8332833333334));
#243077=CARTESIAN_POINT('Ctrl Pts',(46.4348535350793,31.5404524382925,-44.77495));
#243078=CARTESIAN_POINT('Ctrl Pts',(45.9531282658897,32.3748250798187,-44.7166166666667));
#243079=CARTESIAN_POINT('Ctrl Pts',(45.4714029967,33.2091977213449,-44.6582833333333));
#243080=CARTESIAN_POINT('Ctrl Pts',(44.5079524583208,33.2091977213449,-44.59995));
#243081=CARTESIAN_POINT('Ctrl Pts',(43.5445019199415,33.2091977213449,-44.5416166666667));
#243082=CARTESIAN_POINT('Ctrl Pts',(43.0627766507519,32.3748250798187,-44.4832833333334));
#243083=CARTESIAN_POINT('Ctrl Pts',(42.5810513815623,31.5404524382925,-44.42495));
#243084=CARTESIAN_POINT('Ctrl Pts',(43.0627766507519,30.7060797967663,-44.3666166666667));
#243085=CARTESIAN_POINT('Ctrl Pts',(43.5445019199415,29.87170715524,-44.3082833333334));
#243086=CARTESIAN_POINT('Ctrl Pts',(44.5079524583208,29.87170715524,-44.24995));
#243087=CARTESIAN_POINT('Origin',(44.5079524583208,31.5404524382925,-52.920575));
#243088=CARTESIAN_POINT('',(44.5079524583208,29.87170715524,-45.64995));
#243089=CARTESIAN_POINT('',(44.5079524583208,29.87170715524,-45.4912));
#243090=CARTESIAN_POINT('',(44.5079524583209,29.8717071552401,-52.920575));
#243091=CARTESIAN_POINT('Ctrl Pts',(44.5079524583208,29.87170715524,-45.4912));
#243092=CARTESIAN_POINT('Ctrl Pts',(45.4714029967,29.87170715524,-45.4328666666666));
#243093=CARTESIAN_POINT('Ctrl Pts',(45.9531282658897,30.7060797967663,-45.3745333333333));
#243094=CARTESIAN_POINT('Ctrl Pts',(46.4348535350793,31.5404524382925,-45.3162));
#243095=CARTESIAN_POINT('Ctrl Pts',(45.9531282658897,32.3748250798187,-45.2578666666667));
#243096=CARTESIAN_POINT('Ctrl Pts',(45.4714029967,33.2091977213449,-45.1995333333333));
#243097=CARTESIAN_POINT('Ctrl Pts',(44.5079524583208,33.2091977213449,-45.1412));
#243098=CARTESIAN_POINT('Ctrl Pts',(43.5445019199415,33.2091977213449,-45.0828666666667));
#243099=CARTESIAN_POINT('Ctrl Pts',(43.0627766507519,32.3748250798187,-45.0245333333333));
#243100=CARTESIAN_POINT('Ctrl Pts',(42.5810513815623,31.5404524382925,-44.9662));
#243101=CARTESIAN_POINT('Ctrl Pts',(43.0627766507519,30.7060797967663,-44.9078666666666));
#243102=CARTESIAN_POINT('Ctrl Pts',(43.5445019199415,29.87170715524,-44.8495333333333));
#243103=CARTESIAN_POINT('Ctrl Pts',(44.5079524583208,29.87170715524,-44.7912));
#243104=CARTESIAN_POINT('Ctrl Pts',(44.5079524583208,29.87170715524,-45.64995));
#243105=CARTESIAN_POINT('Ctrl Pts',(45.4714029967,29.87170715524,-45.5916166666667));
#243106=CARTESIAN_POINT('Ctrl Pts',(45.9531282658897,30.7060797967663,-45.5332833333333));
#243107=CARTESIAN_POINT('Ctrl Pts',(46.4348535350793,31.5404524382925,-45.47495));
#243108=CARTESIAN_POINT('Ctrl Pts',(45.9531282658897,32.3748250798187,-45.4166166666667));
#243109=CARTESIAN_POINT('Ctrl Pts',(45.4714029967,33.2091977213449,-45.3582833333334));
#243110=CARTESIAN_POINT('Ctrl Pts',(44.5079524583208,33.2091977213449,-45.29995));
#243111=CARTESIAN_POINT('Ctrl Pts',(43.5445019199415,33.2091977213449,-45.2416166666667));
#243112=CARTESIAN_POINT('Ctrl Pts',(43.0627766507519,32.3748250798187,-45.1832833333333));
#243113=CARTESIAN_POINT('Ctrl Pts',(42.5810513815623,31.5404524382925,-45.12495));
#243114=CARTESIAN_POINT('Ctrl Pts',(43.0627766507519,30.7060797967663,-45.0666166666667));
#243115=CARTESIAN_POINT('Ctrl Pts',(43.5445019199415,29.87170715524,-45.0082833333334));
#243116=CARTESIAN_POINT('Ctrl Pts',(44.5079524583208,29.87170715524,-44.94995));
#243117=CARTESIAN_POINT('Origin',(44.5079524583208,31.5404524382925,-52.920575));
#243118=CARTESIAN_POINT('',(44.5079524583208,29.87170715524,-46.34995));
#243119=CARTESIAN_POINT('',(44.5079524583208,29.87170715524,-46.1912));
#243120=CARTESIAN_POINT('',(44.5079524583209,29.8717071552401,-52.920575));
#243121=CARTESIAN_POINT('Ctrl Pts',(44.5079524583208,29.87170715524,-46.1912));
#243122=CARTESIAN_POINT('Ctrl Pts',(45.4714029967,29.87170715524,-46.1328666666667));
#243123=CARTESIAN_POINT('Ctrl Pts',(45.9531282658897,30.7060797967663,-46.0745333333334));
#243124=CARTESIAN_POINT('Ctrl Pts',(46.4348535350793,31.5404524382925,-46.0162));
#243125=CARTESIAN_POINT('Ctrl Pts',(45.9531282658897,32.3748250798187,-45.9578666666667));
#243126=CARTESIAN_POINT('Ctrl Pts',(45.4714029967,33.2091977213449,-45.8995333333333));
#243127=CARTESIAN_POINT('Ctrl Pts',(44.5079524583208,33.2091977213449,-45.8412));
#243128=CARTESIAN_POINT('Ctrl Pts',(43.5445019199415,33.2091977213449,-45.7828666666667));
#243129=CARTESIAN_POINT('Ctrl Pts',(43.0627766507519,32.3748250798187,-45.7245333333333));
#243130=CARTESIAN_POINT('Ctrl Pts',(42.5810513815623,31.5404524382925,-45.6662));
#243131=CARTESIAN_POINT('Ctrl Pts',(43.0627766507519,30.7060797967663,-45.6078666666667));
#243132=CARTESIAN_POINT('Ctrl Pts',(43.5445019199415,29.87170715524,-45.5495333333333));
#243133=CARTESIAN_POINT('Ctrl Pts',(44.5079524583208,29.87170715524,-45.4912));
#243134=CARTESIAN_POINT('Ctrl Pts',(44.5079524583208,29.87170715524,-46.34995));
#243135=CARTESIAN_POINT('Ctrl Pts',(45.4714029967,29.87170715524,-46.2916166666667));
#243136=CARTESIAN_POINT('Ctrl Pts',(45.9531282658897,30.7060797967663,-46.2332833333334));
#243137=CARTESIAN_POINT('Ctrl Pts',(46.4348535350793,31.5404524382925,-46.17495));
#243138=CARTESIAN_POINT('Ctrl Pts',(45.9531282658897,32.3748250798187,-46.1166166666667));
#243139=CARTESIAN_POINT('Ctrl Pts',(45.4714029967,33.2091977213449,-46.0582833333333));
#243140=CARTESIAN_POINT('Ctrl Pts',(44.5079524583208,33.2091977213449,-45.99995));
#243141=CARTESIAN_POINT('Ctrl Pts',(43.5445019199415,33.2091977213449,-45.9416166666667));
#243142=CARTESIAN_POINT('Ctrl Pts',(43.0627766507519,32.3748250798187,-45.8832833333333));
#243143=CARTESIAN_POINT('Ctrl Pts',(42.5810513815623,31.5404524382925,-45.82495));
#243144=CARTESIAN_POINT('Ctrl Pts',(43.0627766507519,30.7060797967663,-45.7666166666667));
#243145=CARTESIAN_POINT('Ctrl Pts',(43.5445019199415,29.87170715524,-45.7082833333333));
#243146=CARTESIAN_POINT('Ctrl Pts',(44.5079524583208,29.87170715524,-45.64995));
#243147=CARTESIAN_POINT('Origin',(44.5079524583208,31.5404524382925,-52.920575));
#243148=CARTESIAN_POINT('',(44.5079524583208,29.87170715524,-47.04995));
#243149=CARTESIAN_POINT('',(44.5079524583208,29.87170715524,-46.8912));
#243150=CARTESIAN_POINT('',(44.5079524583209,29.8717071552401,-52.920575));
#243151=CARTESIAN_POINT('Ctrl Pts',(44.5079524583208,29.87170715524,-46.8912));
#243152=CARTESIAN_POINT('Ctrl Pts',(45.4714029967,29.87170715524,-46.8328666666667));
#243153=CARTESIAN_POINT('Ctrl Pts',(45.9531282658897,30.7060797967663,-46.7745333333333));
#243154=CARTESIAN_POINT('Ctrl Pts',(46.4348535350793,31.5404524382925,-46.7162));
#243155=CARTESIAN_POINT('Ctrl Pts',(45.9531282658897,32.3748250798187,-46.6578666666667));
#243156=CARTESIAN_POINT('Ctrl Pts',(45.4714029967,33.2091977213449,-46.5995333333333));
#243157=CARTESIAN_POINT('Ctrl Pts',(44.5079524583208,33.2091977213449,-46.5412));
#243158=CARTESIAN_POINT('Ctrl Pts',(43.5445019199415,33.2091977213449,-46.4828666666667));
#243159=CARTESIAN_POINT('Ctrl Pts',(43.0627766507519,32.3748250798187,-46.4245333333333));
#243160=CARTESIAN_POINT('Ctrl Pts',(42.5810513815623,31.5404524382925,-46.3662));
#243161=CARTESIAN_POINT('Ctrl Pts',(43.0627766507519,30.7060797967663,-46.3078666666667));
#243162=CARTESIAN_POINT('Ctrl Pts',(43.5445019199415,29.87170715524,-46.2495333333334));
#243163=CARTESIAN_POINT('Ctrl Pts',(44.5079524583208,29.87170715524,-46.1912));
#243164=CARTESIAN_POINT('Ctrl Pts',(44.5079524583208,29.87170715524,-47.04995));
#243165=CARTESIAN_POINT('Ctrl Pts',(45.4714029967,29.87170715524,-46.9916166666667));
#243166=CARTESIAN_POINT('Ctrl Pts',(45.9531282658897,30.7060797967663,-46.9332833333333));
#243167=CARTESIAN_POINT('Ctrl Pts',(46.4348535350793,31.5404524382925,-46.87495));
#243168=CARTESIAN_POINT('Ctrl Pts',(45.9531282658897,32.3748250798187,-46.8166166666667));
#243169=CARTESIAN_POINT('Ctrl Pts',(45.4714029967,33.2091977213449,-46.7582833333333));
#243170=CARTESIAN_POINT('Ctrl Pts',(44.5079524583208,33.2091977213449,-46.69995));
#243171=CARTESIAN_POINT('Ctrl Pts',(43.5445019199415,33.2091977213449,-46.6416166666666));
#243172=CARTESIAN_POINT('Ctrl Pts',(43.0627766507519,32.3748250798187,-46.5832833333334));
#243173=CARTESIAN_POINT('Ctrl Pts',(42.5810513815623,31.5404524382925,-46.52495));
#243174=CARTESIAN_POINT('Ctrl Pts',(43.0627766507519,30.7060797967663,-46.4666166666667));
#243175=CARTESIAN_POINT('Ctrl Pts',(43.5445019199415,29.87170715524,-46.4082833333333));
#243176=CARTESIAN_POINT('Ctrl Pts',(44.5079524583208,29.87170715524,-46.34995));
#243177=CARTESIAN_POINT('Origin',(44.5079524583208,31.5404524382925,-52.920575));
#243178=CARTESIAN_POINT('',(44.5079524583208,29.87170715524,-47.74995));
#243179=CARTESIAN_POINT('',(44.5079524583208,29.87170715524,-47.5912));
#243180=CARTESIAN_POINT('',(44.5079524583209,29.8717071552401,-52.920575));
#243181=CARTESIAN_POINT('Ctrl Pts',(44.5079524583208,29.87170715524,-47.5912));
#243182=CARTESIAN_POINT('Ctrl Pts',(45.4714029967,29.87170715524,-47.5328666666667));
#243183=CARTESIAN_POINT('Ctrl Pts',(45.9531282658897,30.7060797967663,-47.4745333333334));
#243184=CARTESIAN_POINT('Ctrl Pts',(46.4348535350793,31.5404524382925,-47.4162));
#243185=CARTESIAN_POINT('Ctrl Pts',(45.9531282658897,32.3748250798187,-47.3578666666667));
#243186=CARTESIAN_POINT('Ctrl Pts',(45.4714029967,33.2091977213449,-47.2995333333334));
#243187=CARTESIAN_POINT('Ctrl Pts',(44.5079524583208,33.2091977213449,-47.2412));
#243188=CARTESIAN_POINT('Ctrl Pts',(43.5445019199415,33.2091977213449,-47.1828666666667));
#243189=CARTESIAN_POINT('Ctrl Pts',(43.0627766507519,32.3748250798187,-47.1245333333333));
#243190=CARTESIAN_POINT('Ctrl Pts',(42.5810513815623,31.5404524382925,-47.0662));
#243191=CARTESIAN_POINT('Ctrl Pts',(43.0627766507519,30.7060797967663,-47.0078666666667));
#243192=CARTESIAN_POINT('Ctrl Pts',(43.5445019199415,29.87170715524,-46.9495333333334));
#243193=CARTESIAN_POINT('Ctrl Pts',(44.5079524583208,29.87170715524,-46.8912));
#243194=CARTESIAN_POINT('Ctrl Pts',(44.5079524583208,29.87170715524,-47.74995));
#243195=CARTESIAN_POINT('Ctrl Pts',(45.4714029967,29.87170715524,-47.6916166666667));
#243196=CARTESIAN_POINT('Ctrl Pts',(45.9531282658897,30.7060797967663,-47.6332833333333));
#243197=CARTESIAN_POINT('Ctrl Pts',(46.4348535350793,31.5404524382925,-47.57495));
#243198=CARTESIAN_POINT('Ctrl Pts',(45.9531282658897,32.3748250798187,-47.5166166666667));
#243199=CARTESIAN_POINT('Ctrl Pts',(45.4714029967,33.2091977213449,-47.4582833333333));
#243200=CARTESIAN_POINT('Ctrl Pts',(44.5079524583208,33.2091977213449,-47.39995));
#243201=CARTESIAN_POINT('Ctrl Pts',(43.5445019199415,33.2091977213449,-47.3416166666666));
#243202=CARTESIAN_POINT('Ctrl Pts',(43.0627766507519,32.3748250798187,-47.2832833333333));
#243203=CARTESIAN_POINT('Ctrl Pts',(42.5810513815623,31.5404524382925,-47.22495));
#243204=CARTESIAN_POINT('Ctrl Pts',(43.0627766507519,30.7060797967663,-47.1666166666667));
#243205=CARTESIAN_POINT('Ctrl Pts',(43.5445019199415,29.87170715524,-47.1082833333333));
#243206=CARTESIAN_POINT('Ctrl Pts',(44.5079524583208,29.87170715524,-47.04995));
#243207=CARTESIAN_POINT('Origin',(44.5079524583208,31.5404524382925,-52.920575));
#243208=CARTESIAN_POINT('',(44.5079524583208,29.87170715524,-48.44995));
#243209=CARTESIAN_POINT('',(44.5079524583208,29.87170715524,-48.2912));
#243210=CARTESIAN_POINT('',(44.5079524583209,29.8717071552401,-52.920575));
#243211=CARTESIAN_POINT('Ctrl Pts',(44.5079524583208,29.87170715524,-48.2912));
#243212=CARTESIAN_POINT('Ctrl Pts',(45.4714029967,29.87170715524,-48.2328666666667));
#243213=CARTESIAN_POINT('Ctrl Pts',(45.9531282658897,30.7060797967663,-48.1745333333334));
#243214=CARTESIAN_POINT('Ctrl Pts',(46.4348535350793,31.5404524382925,-48.1162));
#243215=CARTESIAN_POINT('Ctrl Pts',(45.9531282658897,32.3748250798187,-48.0578666666667));
#243216=CARTESIAN_POINT('Ctrl Pts',(45.4714029967,33.2091977213449,-47.9995333333334));
#243217=CARTESIAN_POINT('Ctrl Pts',(44.5079524583208,33.2091977213449,-47.9412));
#243218=CARTESIAN_POINT('Ctrl Pts',(43.5445019199415,33.2091977213449,-47.8828666666667));
#243219=CARTESIAN_POINT('Ctrl Pts',(43.0627766507519,32.3748250798187,-47.8245333333333));
#243220=CARTESIAN_POINT('Ctrl Pts',(42.5810513815623,31.5404524382925,-47.7662));
#243221=CARTESIAN_POINT('Ctrl Pts',(43.0627766507519,30.7060797967663,-47.7078666666667));
#243222=CARTESIAN_POINT('Ctrl Pts',(43.5445019199415,29.87170715524,-47.6495333333334));
#243223=CARTESIAN_POINT('Ctrl Pts',(44.5079524583208,29.87170715524,-47.5912));
#243224=CARTESIAN_POINT('Ctrl Pts',(44.5079524583208,29.87170715524,-48.44995));
#243225=CARTESIAN_POINT('Ctrl Pts',(45.4714029967,29.87170715524,-48.3916166666667));
#243226=CARTESIAN_POINT('Ctrl Pts',(45.9531282658897,30.7060797967663,-48.3332833333333));
#243227=CARTESIAN_POINT('Ctrl Pts',(46.4348535350793,31.5404524382925,-48.27495));
#243228=CARTESIAN_POINT('Ctrl Pts',(45.9531282658897,32.3748250798187,-48.2166166666667));
#243229=CARTESIAN_POINT('Ctrl Pts',(45.4714029967,33.2091977213449,-48.1582833333333));
#243230=CARTESIAN_POINT('Ctrl Pts',(44.5079524583208,33.2091977213449,-48.09995));
#243231=CARTESIAN_POINT('Ctrl Pts',(43.5445019199415,33.2091977213449,-48.0416166666667));
#243232=CARTESIAN_POINT('Ctrl Pts',(43.0627766507519,32.3748250798187,-47.9832833333334));
#243233=CARTESIAN_POINT('Ctrl Pts',(42.5810513815623,31.5404524382925,-47.92495));
#243234=CARTESIAN_POINT('Ctrl Pts',(43.0627766507519,30.7060797967663,-47.8666166666667));
#243235=CARTESIAN_POINT('Ctrl Pts',(43.5445019199415,29.87170715524,-47.8082833333333));
#243236=CARTESIAN_POINT('Ctrl Pts',(44.5079524583208,29.87170715524,-47.74995));
#243237=CARTESIAN_POINT('Origin',(44.5079524583208,31.5404524382925,-52.920575));
#243238=CARTESIAN_POINT('',(44.5079524583208,29.87170715524,-49.14995));
#243239=CARTESIAN_POINT('',(44.5079524583208,29.87170715524,-48.9912));
#243240=CARTESIAN_POINT('',(44.5079524583209,29.8717071552401,-52.920575));
#243241=CARTESIAN_POINT('Ctrl Pts',(44.5079524583208,29.87170715524,-48.9912));
#243242=CARTESIAN_POINT('Ctrl Pts',(45.4714029967,29.87170715524,-48.9328666666667));
#243243=CARTESIAN_POINT('Ctrl Pts',(45.9531282658897,30.7060797967663,-48.8745333333333));
#243244=CARTESIAN_POINT('Ctrl Pts',(46.4348535350793,31.5404524382925,-48.8162));
#243245=CARTESIAN_POINT('Ctrl Pts',(45.9531282658897,32.3748250798187,-48.7578666666667));
#243246=CARTESIAN_POINT('Ctrl Pts',(45.4714029967,33.2091977213449,-48.6995333333333));
#243247=CARTESIAN_POINT('Ctrl Pts',(44.5079524583208,33.2091977213449,-48.6412));
#243248=CARTESIAN_POINT('Ctrl Pts',(43.5445019199415,33.2091977213449,-48.5828666666667));
#243249=CARTESIAN_POINT('Ctrl Pts',(43.0627766507519,32.3748250798187,-48.5245333333333));
#243250=CARTESIAN_POINT('Ctrl Pts',(42.5810513815623,31.5404524382925,-48.4662));
#243251=CARTESIAN_POINT('Ctrl Pts',(43.0627766507519,30.7060797967663,-48.4078666666667));
#243252=CARTESIAN_POINT('Ctrl Pts',(43.5445019199415,29.87170715524,-48.3495333333333));
#243253=CARTESIAN_POINT('Ctrl Pts',(44.5079524583208,29.87170715524,-48.2912));
#243254=CARTESIAN_POINT('Ctrl Pts',(44.5079524583208,29.87170715524,-49.14995));
#243255=CARTESIAN_POINT('Ctrl Pts',(45.4714029967,29.87170715524,-49.0916166666667));
#243256=CARTESIAN_POINT('Ctrl Pts',(45.9531282658897,30.7060797967663,-49.0332833333333));
#243257=CARTESIAN_POINT('Ctrl Pts',(46.4348535350793,31.5404524382925,-48.97495));
#243258=CARTESIAN_POINT('Ctrl Pts',(45.9531282658897,32.3748250798187,-48.9166166666667));
#243259=CARTESIAN_POINT('Ctrl Pts',(45.4714029967,33.2091977213449,-48.8582833333333));
#243260=CARTESIAN_POINT('Ctrl Pts',(44.5079524583208,33.2091977213449,-48.79995));
#243261=CARTESIAN_POINT('Ctrl Pts',(43.5445019199415,33.2091977213449,-48.7416166666667));
#243262=CARTESIAN_POINT('Ctrl Pts',(43.0627766507519,32.3748250798187,-48.6832833333333));
#243263=CARTESIAN_POINT('Ctrl Pts',(42.5810513815623,31.5404524382925,-48.62495));
#243264=CARTESIAN_POINT('Ctrl Pts',(43.0627766507519,30.7060797967663,-48.5666166666667));
#243265=CARTESIAN_POINT('Ctrl Pts',(43.5445019199415,29.87170715524,-48.5082833333334));
#243266=CARTESIAN_POINT('Ctrl Pts',(44.5079524583208,29.87170715524,-48.44995));
#243267=CARTESIAN_POINT('Origin',(44.5079524583208,31.5404524382925,-52.920575));
#243268=CARTESIAN_POINT('',(44.5079524583208,29.87170715524,-49.84995));
#243269=CARTESIAN_POINT('',(44.5079524583208,29.87170715524,-49.6912));
#243270=CARTESIAN_POINT('',(44.5079524583209,29.8717071552401,-52.920575));
#243271=CARTESIAN_POINT('Ctrl Pts',(44.5079524583208,29.87170715524,-49.6912));
#243272=CARTESIAN_POINT('Ctrl Pts',(45.4714029967,29.87170715524,-49.6328666666667));
#243273=CARTESIAN_POINT('Ctrl Pts',(45.9531282658897,30.7060797967663,-49.5745333333333));
#243274=CARTESIAN_POINT('Ctrl Pts',(46.4348535350793,31.5404524382925,-49.5162));
#243275=CARTESIAN_POINT('Ctrl Pts',(45.9531282658897,32.3748250798187,-49.4578666666667));
#243276=CARTESIAN_POINT('Ctrl Pts',(45.4714029967,33.2091977213449,-49.3995333333333));
#243277=CARTESIAN_POINT('Ctrl Pts',(44.5079524583208,33.2091977213449,-49.3412));
#243278=CARTESIAN_POINT('Ctrl Pts',(43.5445019199415,33.2091977213449,-49.2828666666667));
#243279=CARTESIAN_POINT('Ctrl Pts',(43.0627766507519,32.3748250798187,-49.2245333333333));
#243280=CARTESIAN_POINT('Ctrl Pts',(42.5810513815623,31.5404524382925,-49.1662));
#243281=CARTESIAN_POINT('Ctrl Pts',(43.0627766507519,30.7060797967663,-49.1078666666667));
#243282=CARTESIAN_POINT('Ctrl Pts',(43.5445019199415,29.87170715524,-49.0495333333334));
#243283=CARTESIAN_POINT('Ctrl Pts',(44.5079524583208,29.87170715524,-48.9912));
#243284=CARTESIAN_POINT('Ctrl Pts',(44.5079524583208,29.87170715524,-49.84995));
#243285=CARTESIAN_POINT('Ctrl Pts',(45.4714029967,29.87170715524,-49.7916166666667));
#243286=CARTESIAN_POINT('Ctrl Pts',(45.9531282658897,30.7060797967663,-49.7332833333333));
#243287=CARTESIAN_POINT('Ctrl Pts',(46.4348535350793,31.5404524382925,-49.67495));
#243288=CARTESIAN_POINT('Ctrl Pts',(45.9531282658897,32.3748250798187,-49.6166166666667));
#243289=CARTESIAN_POINT('Ctrl Pts',(45.4714029967,33.2091977213449,-49.5582833333334));
#243290=CARTESIAN_POINT('Ctrl Pts',(44.5079524583208,33.2091977213449,-49.49995));
#243291=CARTESIAN_POINT('Ctrl Pts',(43.5445019199415,33.2091977213449,-49.4416166666667));
#243292=CARTESIAN_POINT('Ctrl Pts',(43.0627766507519,32.3748250798187,-49.3832833333334));
#243293=CARTESIAN_POINT('Ctrl Pts',(42.5810513815623,31.5404524382925,-49.32495));
#243294=CARTESIAN_POINT('Ctrl Pts',(43.0627766507519,30.7060797967663,-49.2666166666667));
#243295=CARTESIAN_POINT('Ctrl Pts',(43.5445019199415,29.87170715524,-49.2082833333334));
#243296=CARTESIAN_POINT('Ctrl Pts',(44.5079524583208,29.87170715524,-49.14995));
#243297=CARTESIAN_POINT('Origin',(44.5079524583208,31.5404524382925,-52.920575));
#243298=CARTESIAN_POINT('',(44.5079524583208,29.87170715524,-50.54995));
#243299=CARTESIAN_POINT('',(44.5079524583208,29.87170715524,-50.3912));
#243300=CARTESIAN_POINT('',(44.5079524583209,29.8717071552401,-52.920575));
#243301=CARTESIAN_POINT('Ctrl Pts',(44.5079524583208,29.87170715524,-50.3912));
#243302=CARTESIAN_POINT('Ctrl Pts',(45.4714029967,29.87170715524,-50.3328666666666));
#243303=CARTESIAN_POINT('Ctrl Pts',(45.9531282658897,30.7060797967663,-50.2745333333333));
#243304=CARTESIAN_POINT('Ctrl Pts',(46.4348535350793,31.5404524382925,-50.2162));
#243305=CARTESIAN_POINT('Ctrl Pts',(45.9531282658897,32.3748250798187,-50.1578666666667));
#243306=CARTESIAN_POINT('Ctrl Pts',(45.4714029967,33.2091977213449,-50.0995333333333));
#243307=CARTESIAN_POINT('Ctrl Pts',(44.5079524583208,33.2091977213449,-50.0412));
#243308=CARTESIAN_POINT('Ctrl Pts',(43.5445019199415,33.2091977213449,-49.9828666666667));
#243309=CARTESIAN_POINT('Ctrl Pts',(43.0627766507519,32.3748250798187,-49.9245333333334));
#243310=CARTESIAN_POINT('Ctrl Pts',(42.5810513815623,31.5404524382925,-49.8662));
#243311=CARTESIAN_POINT('Ctrl Pts',(43.0627766507519,30.7060797967663,-49.8078666666667));
#243312=CARTESIAN_POINT('Ctrl Pts',(43.5445019199415,29.87170715524,-49.7495333333333));
#243313=CARTESIAN_POINT('Ctrl Pts',(44.5079524583208,29.87170715524,-49.6912));
#243314=CARTESIAN_POINT('Ctrl Pts',(44.5079524583208,29.87170715524,-50.54995));
#243315=CARTESIAN_POINT('Ctrl Pts',(45.4714029967,29.87170715524,-50.4916166666667));
#243316=CARTESIAN_POINT('Ctrl Pts',(45.9531282658897,30.7060797967663,-50.4332833333333));
#243317=CARTESIAN_POINT('Ctrl Pts',(46.4348535350793,31.5404524382925,-50.37495));
#243318=CARTESIAN_POINT('Ctrl Pts',(45.9531282658897,32.3748250798187,-50.3166166666667));
#243319=CARTESIAN_POINT('Ctrl Pts',(45.4714029967,33.2091977213449,-50.2582833333334));
#243320=CARTESIAN_POINT('Ctrl Pts',(44.5079524583208,33.2091977213449,-50.19995));
#243321=CARTESIAN_POINT('Ctrl Pts',(43.5445019199415,33.2091977213449,-50.1416166666667));
#243322=CARTESIAN_POINT('Ctrl Pts',(43.0627766507519,32.3748250798187,-50.0832833333333));
#243323=CARTESIAN_POINT('Ctrl Pts',(42.5810513815623,31.5404524382925,-50.02495));
#243324=CARTESIAN_POINT('Ctrl Pts',(43.0627766507519,30.7060797967663,-49.9666166666667));
#243325=CARTESIAN_POINT('Ctrl Pts',(43.5445019199415,29.87170715524,-49.9082833333334));
#243326=CARTESIAN_POINT('Ctrl Pts',(44.5079524583208,29.87170715524,-49.84995));
#243327=CARTESIAN_POINT('Origin',(44.5079524583208,31.5404524382925,-52.920575));
#243328=CARTESIAN_POINT('',(44.5079524583208,29.87170715524,-51.24995));
#243329=CARTESIAN_POINT('',(44.5079524583208,29.87170715524,-51.0912));
#243330=CARTESIAN_POINT('',(44.5079524583209,29.8717071552401,-52.920575));
#243331=CARTESIAN_POINT('Ctrl Pts',(44.5079524583208,29.87170715524,-51.0912));
#243332=CARTESIAN_POINT('Ctrl Pts',(45.4714029967,29.87170715524,-51.0328666666667));
#243333=CARTESIAN_POINT('Ctrl Pts',(45.9531282658897,30.7060797967663,-50.9745333333333));
#243334=CARTESIAN_POINT('Ctrl Pts',(46.4348535350793,31.5404524382925,-50.9162));
#243335=CARTESIAN_POINT('Ctrl Pts',(45.9531282658897,32.3748250798187,-50.8578666666667));
#243336=CARTESIAN_POINT('Ctrl Pts',(45.4714029967,33.2091977213449,-50.7995333333333));
#243337=CARTESIAN_POINT('Ctrl Pts',(44.5079524583208,33.2091977213449,-50.7412));
#243338=CARTESIAN_POINT('Ctrl Pts',(43.5445019199415,33.2091977213449,-50.6828666666667));
#243339=CARTESIAN_POINT('Ctrl Pts',(43.0627766507519,32.3748250798187,-50.6245333333333));
#243340=CARTESIAN_POINT('Ctrl Pts',(42.5810513815623,31.5404524382925,-50.5662));
#243341=CARTESIAN_POINT('Ctrl Pts',(43.0627766507519,30.7060797967663,-50.5078666666667));
#243342=CARTESIAN_POINT('Ctrl Pts',(43.5445019199415,29.87170715524,-50.4495333333333));
#243343=CARTESIAN_POINT('Ctrl Pts',(44.5079524583208,29.87170715524,-50.3912));
#243344=CARTESIAN_POINT('Ctrl Pts',(44.5079524583208,29.87170715524,-51.24995));
#243345=CARTESIAN_POINT('Ctrl Pts',(45.4714029967,29.87170715524,-51.1916166666667));
#243346=CARTESIAN_POINT('Ctrl Pts',(45.9531282658897,30.7060797967663,-51.1332833333333));
#243347=CARTESIAN_POINT('Ctrl Pts',(46.4348535350793,31.5404524382925,-51.07495));
#243348=CARTESIAN_POINT('Ctrl Pts',(45.9531282658897,32.3748250798187,-51.0166166666667));
#243349=CARTESIAN_POINT('Ctrl Pts',(45.4714029967,33.2091977213449,-50.9582833333334));
#243350=CARTESIAN_POINT('Ctrl Pts',(44.5079524583208,33.2091977213449,-50.89995));
#243351=CARTESIAN_POINT('Ctrl Pts',(43.5445019199415,33.2091977213449,-50.8416166666667));
#243352=CARTESIAN_POINT('Ctrl Pts',(43.0627766507519,32.3748250798187,-50.7832833333333));
#243353=CARTESIAN_POINT('Ctrl Pts',(42.5810513815623,31.5404524382925,-50.72495));
#243354=CARTESIAN_POINT('Ctrl Pts',(43.0627766507519,30.7060797967663,-50.6666166666667));
#243355=CARTESIAN_POINT('Ctrl Pts',(43.5445019199415,29.87170715524,-50.6082833333334));
#243356=CARTESIAN_POINT('Ctrl Pts',(44.5079524583208,29.87170715524,-50.54995));
#243357=CARTESIAN_POINT('Origin',(44.5079524583208,31.5404524382925,-52.920575));
#243358=CARTESIAN_POINT('',(44.5079524583208,29.87170715524,-51.94995));
#243359=CARTESIAN_POINT('',(44.5079524583208,29.87170715524,-51.7912));
#243360=CARTESIAN_POINT('',(44.5079524583209,29.8717071552401,-52.920575));
#243361=CARTESIAN_POINT('Ctrl Pts',(44.5079524583208,29.87170715524,-51.7912));
#243362=CARTESIAN_POINT('Ctrl Pts',(45.4714029967,29.87170715524,-51.7328666666667));
#243363=CARTESIAN_POINT('Ctrl Pts',(45.9531282658897,30.7060797967663,-51.6745333333333));
#243364=CARTESIAN_POINT('Ctrl Pts',(46.4348535350793,31.5404524382925,-51.6162));
#243365=CARTESIAN_POINT('Ctrl Pts',(45.9531282658897,32.3748250798187,-51.5578666666667));
#243366=CARTESIAN_POINT('Ctrl Pts',(45.4714029967,33.2091977213449,-51.4995333333333));
#243367=CARTESIAN_POINT('Ctrl Pts',(44.5079524583208,33.2091977213449,-51.4412));
#243368=CARTESIAN_POINT('Ctrl Pts',(43.5445019199415,33.2091977213449,-51.3828666666667));
#243369=CARTESIAN_POINT('Ctrl Pts',(43.0627766507519,32.3748250798187,-51.3245333333334));
#243370=CARTESIAN_POINT('Ctrl Pts',(42.5810513815623,31.5404524382925,-51.2662));
#243371=CARTESIAN_POINT('Ctrl Pts',(43.0627766507519,30.7060797967663,-51.2078666666667));
#243372=CARTESIAN_POINT('Ctrl Pts',(43.5445019199415,29.87170715524,-51.1495333333333));
#243373=CARTESIAN_POINT('Ctrl Pts',(44.5079524583208,29.87170715524,-51.0912));
#243374=CARTESIAN_POINT('Ctrl Pts',(44.5079524583208,29.87170715524,-51.94995));
#243375=CARTESIAN_POINT('Ctrl Pts',(45.4714029967,29.87170715524,-51.8916166666666));
#243376=CARTESIAN_POINT('Ctrl Pts',(45.9531282658897,30.7060797967663,-51.8332833333333));
#243377=CARTESIAN_POINT('Ctrl Pts',(46.4348535350793,31.5404524382925,-51.77495));
#243378=CARTESIAN_POINT('Ctrl Pts',(45.9531282658897,32.3748250798187,-51.7166166666667));
#243379=CARTESIAN_POINT('Ctrl Pts',(45.4714029967,33.2091977213449,-51.6582833333333));
#243380=CARTESIAN_POINT('Ctrl Pts',(44.5079524583208,33.2091977213449,-51.59995));
#243381=CARTESIAN_POINT('Ctrl Pts',(43.5445019199415,33.2091977213449,-51.5416166666667));
#243382=CARTESIAN_POINT('Ctrl Pts',(43.0627766507519,32.3748250798187,-51.4832833333333));
#243383=CARTESIAN_POINT('Ctrl Pts',(42.5810513815623,31.5404524382925,-51.42495));
#243384=CARTESIAN_POINT('Ctrl Pts',(43.0627766507519,30.7060797967663,-51.3666166666667));
#243385=CARTESIAN_POINT('Ctrl Pts',(43.5445019199415,29.87170715524,-51.3082833333333));
#243386=CARTESIAN_POINT('Ctrl Pts',(44.5079524583208,29.87170715524,-51.24995));
#243387=CARTESIAN_POINT('Origin',(44.5079524583208,31.5404524382925,-52.920575));
#243388=CARTESIAN_POINT('',(44.5079524583208,29.87170715524,-52.64995));
#243389=CARTESIAN_POINT('',(44.5079524583208,29.87170715524,-52.4912));
#243390=CARTESIAN_POINT('',(44.5079524583209,29.8717071552401,-52.920575));
#243391=CARTESIAN_POINT('',(42.8554737113965,31.3080200595814,-52.64995));
#243392=CARTESIAN_POINT('Origin',(44.5079524583208,31.5404524382925,-52.64995));
#243393=CARTESIAN_POINT('Ctrl Pts',(42.8554737113965,31.3080200595814,-52.64995));
#243394=CARTESIAN_POINT('Ctrl Pts',(42.9006402736027,30.9869082397437,-52.6275001713604));
#243395=CARTESIAN_POINT('Ctrl Pts',(43.0627766507519,30.7060797967663,-52.6078666666667));
#243396=CARTESIAN_POINT('Ctrl Pts',(43.5445019199415,29.87170715524,-52.5495333333333));
#243397=CARTESIAN_POINT('Ctrl Pts',(44.5079524583208,29.87170715524,-52.4912));
#243398=CARTESIAN_POINT('Origin',(-73.0894692252869,64.3905251417593,178.93805));
#243399=CARTESIAN_POINT('',(73.0894692252869,64.3905251417593,-27.14995));
#243400=CARTESIAN_POINT('',(-63.0894692252869,64.3905251417593,-27.14995));
#243401=CARTESIAN_POINT('',(-73.0894692252869,64.3905251417593,-27.14995));
#243402=CARTESIAN_POINT('',(-63.0894692252869,64.3905251417593,153.53805));
#243403=CARTESIAN_POINT('',(-63.0894692252869,64.3905251417593,178.93805));
#243404=CARTESIAN_POINT('',(-52.7694692252869,64.3905251417593,153.53805));
#243405=CARTESIAN_POINT('',(-52.7694692252869,64.3905251417593,153.53805));
#243406=CARTESIAN_POINT('',(-52.7694692252869,64.3905251417593,10.95005));
#243407=CARTESIAN_POINT('',(-52.7694692252869,64.3905251417593,10.95005));
#243408=CARTESIAN_POINT('',(52.7165405689488,64.3905251417593,10.95005));
#243409=CARTESIAN_POINT('',(-52.7694692252869,64.3905251417593,10.95005));
#243410=CARTESIAN_POINT('',(52.7165405689488,64.3905251417593,153.53805));
#243411=CARTESIAN_POINT('',(52.7165405689488,64.3905251417593,10.95005));
#243412=CARTESIAN_POINT('',(73.0894692252869,64.3905251417593,153.53805));
#243413=CARTESIAN_POINT('',(73.0894692252869,64.3905251417593,153.53805));
#243414=CARTESIAN_POINT('',(73.0894692252869,64.3905251417593,178.93805));
#243415=CARTESIAN_POINT('Origin',(73.0894692252869,-92.5030998968147,178.93805));
#243416=CARTESIAN_POINT('',(73.0894692252869,-92.5030998968147,143.53805));
#243417=CARTESIAN_POINT('',(73.0894692252869,-92.5030998968147,-17.1499499999999));
#243418=CARTESIAN_POINT('',(73.0894692252869,-92.5030998968147,178.93805));
#243419=CARTESIAN_POINT('',(73.0894692252869,-82.5030998968147,-27.14995));
#243420=CARTESIAN_POINT('Origin',(73.0894692252869,-82.5030998968147,-17.14995));
#243421=CARTESIAN_POINT('',(73.0894692252869,-92.5030998968147,-27.14995));
#243422=CARTESIAN_POINT('',(73.0894692252869,-82.5030998968147,153.53805));
#243423=CARTESIAN_POINT('',(73.0894692252869,-92.5030998968147,153.53805));
#243424=CARTESIAN_POINT('Origin',(73.0894692252869,-82.5030998968147,143.53805));
#243425=CARTESIAN_POINT('Origin',(-73.0894692252869,-92.5030998968147,178.93805));
#243426=CARTESIAN_POINT('',(1.41042477341199E-15,-92.5030998968147,-17.7284445206843));
#243427=CARTESIAN_POINT('',(5.38401031719611,-92.5030998968147,-17.14995));
#243428=CARTESIAN_POINT('Ctrl Pts',(2.91433543964104E-16,-92.5030998968147,
-17.7284445206843));
#243429=CARTESIAN_POINT('Ctrl Pts',(0.147229163500497,-92.5030998968147,
-17.7284445207334));
#243430=CARTESIAN_POINT('Ctrl Pts',(0.293871405581726,-92.5030998968147,
-17.7239593344788));
#243431=CARTESIAN_POINT('Ctrl Pts',(0.44004554522873,-92.5030998968147,
-17.7155634484342));
#243432=CARTESIAN_POINT('Ctrl Pts',(0.517553206202418,-92.5030998968147,
-17.7111115974386));
#243433=CARTESIAN_POINT('Ctrl Pts',(0.594929276459816,-92.5030998968147,
-17.7055592859653));
#243434=CARTESIAN_POINT('Ctrl Pts',(0.672191588762477,-92.5030998968147,
-17.6989863163936));
#243435=CARTESIAN_POINT('Ctrl Pts',(0.817842223176104,-92.5030998968147,
-17.686595317994));
#243436=CARTESIAN_POINT('Ctrl Pts',(0.963088078591146,-92.5030998968147,
-17.6706470841864));
#243437=CARTESIAN_POINT('Ctrl Pts',(1.10803994708469,-92.5030998968147,
-17.6522190746586));
#243438=CARTESIAN_POINT('Ctrl Pts',(1.1872147971738,-92.5030998968147,-17.6421534238535));
#243439=CARTESIAN_POINT('Ctrl Pts',(1.26630195606147,-92.5030998968147,
-17.6313468742016));
#243440=CARTESIAN_POINT('Ctrl Pts',(1.34531959863512,-92.5030998968147,
-17.6199686692659));
#243441=CARTESIAN_POINT('Ctrl Pts',(1.52436111987836,-92.5030998968147,
-17.5941874506121));
#243442=CARTESIAN_POINT('Ctrl Pts',(1.70304430645085,-92.5030998968147,
-17.5655472846095));
#243443=CARTESIAN_POINT('Ctrl Pts',(1.88158201618799,-92.5030998968147,
-17.5359412079341));
#243444=CARTESIAN_POINT('Ctrl Pts',(1.92738834388522,-92.5030998968147,
-17.5283453580041));
#243445=CARTESIAN_POINT('Ctrl Pts',(1.97318510093253,-92.5030998968147,
-17.5206856425068));
#243446=CARTESIAN_POINT('Ctrl Pts',(2.0189758909695,-92.5030998968147,-17.5129935633713));
#243447=CARTESIAN_POINT('Ctrl Pts',(2.2426386144668,-92.5030998968147,-17.475422004387));
#243448=CARTESIAN_POINT('Ctrl Pts',(2.46615860930815,-92.5030998968147,
-17.4370978585973));
#243449=CARTESIAN_POINT('Ctrl Pts',(2.68997472098224,-92.5030998968146,
-17.4006914213871));
#243450=CARTESIAN_POINT('Ctrl Pts',(2.69089693821404,-92.5030998968146,
-17.400541411437));
#243451=CARTESIAN_POINT('Ctrl Pts',(2.6918191587813,-92.5030998968146,-17.4003914343617));
#243452=CARTESIAN_POINT('Ctrl Pts',(2.69274138269184,-92.5030998968146,
-17.4002414903531));
#243453=CARTESIAN_POINT('Ctrl Pts',(2.91701904908716,-92.5030998968146,
-17.3637762762437));
#243454=CARTESIAN_POINT('Ctrl Pts',(3.14149484510243,-92.5030998968146,
-17.3292456165492));
#243455=CARTESIAN_POINT('Ctrl Pts',(3.36629960048568,-92.5030998968147,
-17.2984515031681));
#243456=CARTESIAN_POINT('Ctrl Pts',(3.58776424796595,-92.5030998968147,
-17.2681149230864));
#243457=CARTESIAN_POINT('Ctrl Pts',(3.8095485406857,-92.5030998968147,-17.2413843839963));
#243458=CARTESIAN_POINT('Ctrl Pts',(4.03178888983265,-92.5030998968147,
-17.2193800201178));
#243459=CARTESIAN_POINT('Ctrl Pts',(4.0343401623378,-92.5030998968147,-17.2191274146447));
#243460=CARTESIAN_POINT('Ctrl Pts',(4.03689149329264,-92.5030998968147,
-17.218875432595));
#243461=CARTESIAN_POINT('Ctrl Pts',(4.03944288277982,-92.5030998968147,
-17.2186240757152));
#243462=CARTESIAN_POINT('Ctrl Pts',(4.28517101203901,-92.5030998968146,
-17.1944155194854));
#243463=CARTESIAN_POINT('Ctrl Pts',(4.53144181435921,-92.5030998968146,
-17.176053999827));
#243464=CARTESIAN_POINT('Ctrl Pts',(4.77834069452045,-92.5030998968147,
-17.1644308424862));
#243465=CARTESIAN_POINT('Ctrl Pts',(4.97979715780893,-92.5030998968147,
-17.1549469591708));
#243466=CARTESIAN_POINT('Ctrl Pts',(5.18167176193193,-92.5030998968147,
-17.14995000057));
#243467=CARTESIAN_POINT('Ctrl Pts',(5.38401031719608,-92.5030998968147,
-17.14995));
#243468=CARTESIAN_POINT('',(73.0894692252869,-92.5030998968147,-17.14995));
#243469=CARTESIAN_POINT('',(-63.0894692252869,-92.5030998968147,143.53805));
#243470=CARTESIAN_POINT('',(-73.0894692252869,-92.5030998968147,143.53805));
#243471=CARTESIAN_POINT('',(-63.0894692252869,-92.5030998968147,-17.14995));
#243472=CARTESIAN_POINT('',(-63.0894692252869,-92.5030998968147,178.93805));
#243473=CARTESIAN_POINT('',(-5.38401031719611,-92.5030998968147,-17.14995));
#243474=CARTESIAN_POINT('',(73.0894692252869,-92.5030998968147,-17.14995));
#243475=CARTESIAN_POINT('Ctrl Pts',(-5.38401031719611,-92.5030998968147,
-17.14995));
#243476=CARTESIAN_POINT('Ctrl Pts',(-5.17485934008524,-92.5030998968147,
-17.1499500004992));
#243477=CARTESIAN_POINT('Ctrl Pts',(-4.96574937219036,-92.5030998968147,
-17.1553183575515));
#243478=CARTESIAN_POINT('Ctrl Pts',(-4.75693472932383,-92.5030998968147,
-17.165480868006));
#243479=CARTESIAN_POINT('Ctrl Pts',(-4.53691595770484,-92.5030998968146,
-17.1761886566749));
#243480=CARTESIAN_POINT('Ctrl Pts',(-4.31722468835889,-92.5030998968146,
-17.1922190450184));
#243481=CARTESIAN_POINT('Ctrl Pts',(-4.09814106884925,-92.5030998968147,
-17.2129547281307));
#243482=CARTESIAN_POINT('Ctrl Pts',(-4.0782215499176,-92.5030998968147,
-17.2148400577288));
#243483=CARTESIAN_POINT('Ctrl Pts',(-4.05830704542795,-92.5030998968147,
-17.2167643191585));
#243484=CARTESIAN_POINT('Ctrl Pts',(-4.0383977610556,-92.5030998968147,
-17.2187270683337));
#243485=CARTESIAN_POINT('Ctrl Pts',(-4.03578258234885,-92.5030998968146,
-17.218984884725));
#243486=CARTESIAN_POINT('Ctrl Pts',(-4.03316747486925,-92.5030998968147,
-17.2192433566002));
#243487=CARTESIAN_POINT('Ctrl Pts',(-4.03055243826174,-92.5030998968147,
-17.2195024821027));
#243488=CARTESIAN_POINT('Ctrl Pts',(-3.80825137721949,-92.5030998968147,
-17.2415304238898));
#243489=CARTESIAN_POINT('Ctrl Pts',(-3.58653411126924,-92.5030998968147,
-17.2682720627626));
#243490=CARTESIAN_POINT('Ctrl Pts',(-3.36523550080909,-92.5030998968146,
-17.2985975766844));
#243491=CARTESIAN_POINT('Ctrl Pts',(-3.14061523848556,-92.5030998968146,
-17.3293782710504));
#243492=CARTESIAN_POINT('Ctrl Pts',(-2.91642667300228,-92.5030998968146,
-17.3638716676672));
#243493=CARTESIAN_POINT('Ctrl Pts',(-2.69248545255446,-92.5030998968146,
-17.4002835179756));
#243494=CARTESIAN_POINT('Ctrl Pts',(-2.69114305863619,-92.5030998968146,
-17.4005017852795));
#243495=CARTESIAN_POINT('Ctrl Pts',(-2.68980067362,-92.5030998968146,-17.4007201222748));
#243496=CARTESIAN_POINT('Ctrl Pts',(-2.68845829746235,-92.5030998968146,
-17.4009385283737));
#243497=CARTESIAN_POINT('Ctrl Pts',(-2.46547921905367,-92.5030998968146,
-17.4372174732668));
#243498=CARTESIAN_POINT('Ctrl Pts',(-2.2427730556341,-92.5030998968147,
-17.4753971680139));
#243499=CARTESIAN_POINT('Ctrl Pts',(-2.01994046127722,-92.5030998968147,
-17.512831695184));
#243500=CARTESIAN_POINT('Ctrl Pts',(-1.82567729605443,-92.5030998968147,
-17.5454667311745));
#243501=CARTESIAN_POINT('Ctrl Pts',(-1.63131786476234,-92.5030998968147,
-17.5775261019158));
#243502=CARTESIAN_POINT('Ctrl Pts',(-1.43658485311307,-92.5030998968147,
-17.606583833856));
#243503=CARTESIAN_POINT('Ctrl Pts',(-1.40682826463025,-92.5030998968147,
-17.6110240618598));
#243504=CARTESIAN_POINT('Ctrl Pts',(-1.37706295113733,-92.5030998968147,
-17.6153941011427));
#243505=CARTESIAN_POINT('Ctrl Pts',(-1.34728792074641,-92.5030998968147,
-17.6196851681245));
#243506=CARTESIAN_POINT('Ctrl Pts',(-1.19021355623138,-92.5030998968147,
-17.6423221431472));
#243507=CARTESIAN_POINT('Ctrl Pts',(-1.03286783750708,-92.5030998968147,
-17.6627117449257));
#243508=CARTESIAN_POINT('Ctrl Pts',(-0.875104001456876,-92.5030998968147,
-17.6795039821736));
#243509=CARTESIAN_POINT('Ctrl Pts',(-0.80818557225273,-92.5030998968147,
-17.686626718078));
#243510=CARTESIAN_POINT('Ctrl Pts',(-0.741191904926731,-92.5030998968147,
-17.6931016412339));
#243511=CARTESIAN_POINT('Ctrl Pts',(-0.674111743118813,-92.5030998968147,
-17.6988227621603));
#243512=CARTESIAN_POINT('Ctrl Pts',(-0.516701310019878,-92.5030998968147,
-17.7122479552213));
#243513=CARTESIAN_POINT('Ctrl Pts',(-0.358814095941945,-92.5030998968147,
-17.7214461823106));
#243514=CARTESIAN_POINT('Ctrl Pts',(-0.200315373111298,-92.5030998968147,
-17.7257206232356));
#243515=CARTESIAN_POINT('Ctrl Pts',(-0.133655118857088,-92.5030998968147,
-17.7275183368939));
#243516=CARTESIAN_POINT('Ctrl Pts',(-0.0668866878046401,-92.5030998968147,
-17.7284445206844));
#243517=CARTESIAN_POINT('Ctrl Pts',(-2.77555756156289E-14,-92.5030998968147,
-17.7284445206844));
#243518=CARTESIAN_POINT('Origin',(-73.0894692252869,-64.3905251417593,178.93805));
#243519=CARTESIAN_POINT('',(-73.0894692252869,-82.5030998968147,143.53805));
#243520=CARTESIAN_POINT('',(-73.0894692252869,54.3905251417593,143.53805));
#243521=CARTESIAN_POINT('',(-73.0894692252869,64.3905251417593,143.53805));
#243522=CARTESIAN_POINT('',(-73.0894692252869,54.3905251417593,-17.14995));
#243523=CARTESIAN_POINT('',(-73.0894692252869,54.3905251417593,178.93805));
#243524=CARTESIAN_POINT('',(-73.0894692252869,-82.5030998968147,-17.14995));
#243525=CARTESIAN_POINT('',(-73.0894692252869,-92.5030998968147,-17.14995));
#243526=CARTESIAN_POINT('',(-73.0894692252869,-82.5030998968147,178.93805));
#243527=CARTESIAN_POINT('Origin',(-52.7694692252869,296.281453912738,10.95005));
#243528=CARTESIAN_POINT('',(-52.7694692252869,97.9199999800001,153.53805));
#243529=CARTESIAN_POINT('',(-52.7694692252869,97.9199999800001,153.53805));
#243530=CARTESIAN_POINT('',(-52.7694692252869,97.9199999800001,10.95005));
#243531=CARTESIAN_POINT('',(-52.7694692252869,97.9199999800001,10.95005));
#243532=CARTESIAN_POINT('',(-52.7694692252869,296.281453912738,10.95005));
#243533=CARTESIAN_POINT('Origin',(52.7165405689488,296.281453912738,10.95005));
#243534=CARTESIAN_POINT('',(52.7165405689488,97.9199999800001,153.53805));
#243535=CARTESIAN_POINT('',(52.7165405689488,64.3905251417593,153.53805));
#243536=CARTESIAN_POINT('',(52.7165405689488,97.9199999800001,10.95005));
#243537=CARTESIAN_POINT('',(52.7165405689488,296.281453912738,10.95005));
#243538=CARTESIAN_POINT('',(52.7165405689488,97.9199999800001,10.95005));
#243539=CARTESIAN_POINT('Origin',(45.,97.9199999800001,-179.84995));
#243540=CARTESIAN_POINT('',(52.7165405689488,97.9199999800001,153.53805));
#243541=CARTESIAN_POINT('',(-52.7694692252869,97.9199999800001,10.95005));
#243542=CARTESIAN_POINT('Origin',(0.,0.,-27.14995));
#243543=CARTESIAN_POINT('',(5.38401031719611,-82.5030998968147,-27.14995));
#243544=CARTESIAN_POINT('',(-73.0894692252869,-82.5030998968147,-27.14995));
#243545=CARTESIAN_POINT('',(-5.38401031719611,-82.5030998968147,-27.14995));
#243546=CARTESIAN_POINT('Origin',(1.73472347597681E-15,-79.8550000300563,
-27.14995));
#243547=CARTESIAN_POINT('',(-63.0894692252869,-82.5030998968147,-27.14995));
#243548=CARTESIAN_POINT('',(-73.0894692252869,-82.5030998968147,-27.14995));
#243549=CARTESIAN_POINT('',(-63.0894692252869,-17.612385611532,-27.14995));
#243550=CARTESIAN_POINT('',(-63.0894692252869,64.3905251417593,-27.14995));
#243551=CARTESIAN_POINT('',(-63.0894692252869,-8.3226144285248,-27.14995));
#243552=CARTESIAN_POINT('Origin',(-66.8875000100282,-12.9675000200284,-27.14995));
#243553=CARTESIAN_POINT('',(-63.0894692252869,64.3905251417593,-27.14995));
#243554=CARTESIAN_POINT('',(72.8875000100282,-12.9675000200274,-27.14995));
#243555=CARTESIAN_POINT('Origin',(66.8875000100282,-12.9675000200274,-27.14995));
#243556=CARTESIAN_POINT('',(-2.46951155546522E-15,59.91999999,-27.14995));
#243557=CARTESIAN_POINT('Origin',(-1.73472347597681E-15,53.91999999,-27.14995));
#243558=CARTESIAN_POINT('',(-55.8761336488114,-39.4730326646711,-27.14995));
#243559=CARTESIAN_POINT('',(-55.7820023947001,-39.0050779822088,-27.14995));
#243560=CARTESIAN_POINT('Ctrl Pts',(-55.8761336488114,-39.4730326646711,
-27.14995));
#243561=CARTESIAN_POINT('Ctrl Pts',(-55.857436348509,-39.4770567377031,
-27.14995));
#243562=CARTESIAN_POINT('Ctrl Pts',(-55.8345450449543,-39.478704339892,
-27.14995));
#243563=CARTESIAN_POINT('Ctrl Pts',(-55.8010467908434,-39.4734293400209,
-27.14995));
#243564=CARTESIAN_POINT('Ctrl Pts',(-55.7843587662846,-39.4674032100666,
-27.14995));
#243565=CARTESIAN_POINT('Ctrl Pts',(-55.7594408254806,-39.4513001221049,
-27.14995));
#243566=CARTESIAN_POINT('Ctrl Pts',(-55.74702264916,-39.4384648268173,-27.14995));
#243567=CARTESIAN_POINT('Ctrl Pts',(-55.7281173639228,-39.4097003595277,
-27.14995));
#243568=CARTESIAN_POINT('Ctrl Pts',(-55.7199815038304,-39.3877113716395,
-27.14995));
#243569=CARTESIAN_POINT('Ctrl Pts',(-55.7068870219065,-39.3286173033286,
-27.14995));
#243570=CARTESIAN_POINT('Ctrl Pts',(-55.7084166181688,-39.2794539793635,
-27.14995));
#243571=CARTESIAN_POINT('Ctrl Pts',(-55.7242400077265,-39.1630314139732,
-27.14995));
#243572=CARTESIAN_POINT('Ctrl Pts',(-55.7527257002045,-39.0757581751218,
-27.14995));
#243573=CARTESIAN_POINT('Ctrl Pts',(-55.7820023947002,-39.0050779822088,
-27.14995));
#243574=CARTESIAN_POINT('',(-53.5626016629799,-44.3631853290296,-27.149950000041));
#243575=CARTESIAN_POINT('',(-60.2627421407299,-28.1876153178796,-27.14995));
#243576=CARTESIAN_POINT('',(-53.5586640602543,-44.3727771923847,-27.14995));
#243577=CARTESIAN_POINT('Ctrl Pts',(-53.5586640602543,-44.3727771923846,
-27.14995));
#243578=CARTESIAN_POINT('Ctrl Pts',(-53.5593152758377,-44.3711764813904,
-27.14995));
#243579=CARTESIAN_POINT('Ctrl Pts',(-53.5599690168506,-44.3695767986133,
-27.1499500000007));
#243580=CARTESIAN_POINT('Ctrl Pts',(-53.5612815516416,-44.3663795033483,
-27.1499500000007));
#243581=CARTESIAN_POINT('Ctrl Pts',(-53.5619403445691,-44.3647818929451,
-27.14995));
#243582=CARTESIAN_POINT('Ctrl Pts',(-53.5626016635193,-44.3631853277664,
-27.14995));
#243583=CARTESIAN_POINT('',(-53.2522037718306,-45.0092559826887,-27.1499499611498));
#243584=CARTESIAN_POINT('Ctrl Pts',(-53.2522036547411,-45.0092557774118,
-27.14995));
#243585=CARTESIAN_POINT('Ctrl Pts',(-53.3294790538135,-44.9004089637583,
-27.14995));
#243586=CARTESIAN_POINT('Ctrl Pts',(-53.3831793339603,-44.793525414087,
-27.14995));
#243587=CARTESIAN_POINT('Ctrl Pts',(-53.4750626849387,-44.5886297190003,
-27.14995));
#243588=CARTESIAN_POINT('Ctrl Pts',(-53.513383785808,-44.4840786455929,
-27.14995));
#243589=CARTESIAN_POINT('Ctrl Pts',(-53.5586640602543,-44.3727771923846,
-27.14995));
#243590=CARTESIAN_POINT('',(-52.345151028036,-45.4735034267004,-27.1499501536531));
#243591=CARTESIAN_POINT('Ctrl Pts',(-52.3451484065213,-45.4735122149407,
-27.1499499998352));
#243592=CARTESIAN_POINT('Ctrl Pts',(-52.3459275035447,-45.4737446180718,
-27.1499500014364));
#243593=CARTESIAN_POINT('Ctrl Pts',(-52.346637838916,-45.4739531739643,
-27.1499500089096));
#243594=CARTESIAN_POINT('Ctrl Pts',(-52.3473191716821,-45.4741281319922,
-27.1499500260981));
#243595=CARTESIAN_POINT('Ctrl Pts',(-52.3482254969746,-45.4743608653843,
-27.1499500489628));
#243596=CARTESIAN_POINT('Ctrl Pts',(-52.3490793422263,-45.47453678322,-27.1499500935485));
#243597=CARTESIAN_POINT('Ctrl Pts',(-52.3499379336497,-45.4747048986454,
-27.1499501664179));
#243598=CARTESIAN_POINT('Ctrl Pts',(-52.3508910661715,-45.474891525573,
-27.149950247311));
#243599=CARTESIAN_POINT('Ctrl Pts',(-52.3518546868251,-45.4750614608143,
-27.1499503632212));
#243600=CARTESIAN_POINT('Ctrl Pts',(-52.3529246660297,-45.4752419002879,
-27.1499505368206));
#243601=CARTESIAN_POINT('Ctrl Pts',(-52.3535486204709,-45.4753471229038,
-27.1499506380545));
#243602=CARTESIAN_POINT('Ctrl Pts',(-52.3543069993715,-45.475480515556,
-27.1499507672218));
#243603=CARTESIAN_POINT('Ctrl Pts',(-52.3551332277138,-45.4756238142328,
-27.1499509263529));
#243604=CARTESIAN_POINT('Ctrl Pts',(-52.3567068551066,-45.4758967396599,
-27.1499512294326));
#243605=CARTESIAN_POINT('Ctrl Pts',(-52.3585273930797,-45.4762015051856,
-27.1499516548711));
#243606=CARTESIAN_POINT('Ctrl Pts',(-52.3601264666894,-45.4764605215105,
-27.1499520866353));
#243607=CARTESIAN_POINT('Ctrl Pts',(-52.3614001841934,-45.4766668369827,
-27.1499524305505));
#243608=CARTESIAN_POINT('Ctrl Pts',(-52.3625330431393,-45.4768463573693,
-27.1499527703999));
#243609=CARTESIAN_POINT('Ctrl Pts',(-52.3632870358042,-45.4769745988415,
-27.149952977261));
#243610=CARTESIAN_POINT('Ctrl Pts',(-52.3639857420081,-45.4770934370165,
-27.1499531689539));
#243611=CARTESIAN_POINT('Ctrl Pts',(-52.3647126753518,-45.4772172193922,
-27.1499533707677));
#243612=CARTESIAN_POINT('Ctrl Pts',(-52.3654678294564,-45.4773457555014,
-27.1499535811654));
#243613=CARTESIAN_POINT('Ctrl Pts',(-52.367087805466,-45.4776214944691,
-27.1499540325159));
#243614=CARTESIAN_POINT('Ctrl Pts',(-52.3688375340627,-45.4779190999074,
-27.14995452436));
#243615=CARTESIAN_POINT('Ctrl Pts',(-52.3707158918108,-45.4782384677742,
-27.1499550323686));
#243616=CARTESIAN_POINT('Ctrl Pts',(-52.3725442373027,-45.4785493323048,
-27.1499555268512));
#243617=CARTESIAN_POINT('Ctrl Pts',(-52.3750453259033,-45.4789803305049,
-27.1499561520407));
#243618=CARTESIAN_POINT('Ctrl Pts',(-52.3771208085955,-45.4793308918207,
-27.149956637901));
#243619=CARTESIAN_POINT('Ctrl Pts',(-52.3781715347264,-45.4795083656856,
-27.1499568838708));
#243620=CARTESIAN_POINT('Ctrl Pts',(-52.3791131815617,-45.4796663726659,
-27.1499570932415));
#243621=CARTESIAN_POINT('Ctrl Pts',(-52.37980339475,-45.4797837664548,-27.1499572335388));
#243622=CARTESIAN_POINT('Ctrl Pts',(-52.3816853956202,-45.4801038635155,
-27.1499576160867));
#243623=CARTESIAN_POINT('Ctrl Pts',(-52.3837163183772,-45.4804481688642,
-27.1499579779973));
#243624=CARTESIAN_POINT('Ctrl Pts',(-52.3858957243288,-45.4808133331965,
-27.1499582713809));
#243625=CARTESIAN_POINT('Ctrl Pts',(-52.3884725173317,-45.4812450806164,
-27.1499586182592));
#243626=CARTESIAN_POINT('Ctrl Pts',(-52.3912547089599,-45.4817150874301,
-27.1499588202072));
#243627=CARTESIAN_POINT('Ctrl Pts',(-52.3942399854462,-45.4822229778649,
-27.1499587218464));
#243628=CARTESIAN_POINT('Ctrl Pts',(-52.3982047554552,-45.4828975112869,
-27.1499585912127));
#243629=CARTESIAN_POINT('Ctrl Pts',(-52.4032077802452,-45.4837599356511,
-27.1499577375115));
#243630=CARTESIAN_POINT('Ctrl Pts',(-52.4077765937205,-45.4845400810146,
-27.1499560472647));
#243631=CARTESIAN_POINT('Ctrl Pts',(-52.4095574402195,-45.4848441685303,
-27.1499553884349));
#243632=CARTESIAN_POINT('Ctrl Pts',(-52.411272670905,-45.4851361374688,
-27.149954621023));
#243633=CARTESIAN_POINT('Ctrl Pts',(-52.4128361264391,-45.4854020484429,
-27.1499538159014));
#243634=CARTESIAN_POINT('Ctrl Pts',(-52.4173474081285,-45.48616932278,-27.1499514927587));
#243635=CARTESIAN_POINT('Ctrl Pts',(-52.4217963551763,-45.4866586938774,
-27.1499500079827));
#243636=CARTESIAN_POINT('Ctrl Pts',(-52.4262642309366,-45.4869505480063,
-27.1499494127242));
#243637=CARTESIAN_POINT('Ctrl Pts',(-52.4312521526722,-45.4872763729915,
-27.1499487481797));
#243638=CARTESIAN_POINT('Ctrl Pts',(-52.4362563424152,-45.4873670236692,
-27.1499492753577));
#243639=CARTESIAN_POINT('Ctrl Pts',(-52.4413789434443,-45.4874163648212,
-27.1499497332176));
#243640=CARTESIAN_POINT('Ctrl Pts',(-52.4430077900509,-45.487432053954,
-27.1499498788045));
#243641=CARTESIAN_POINT('Ctrl Pts',(-52.4446486005821,-45.487443961417,
-27.14995));
#243642=CARTESIAN_POINT('Ctrl Pts',(-52.4463046574406,-45.4874594061206,
-27.14995));
#243643=CARTESIAN_POINT('Ctrl Pts',(-52.4511323504925,-45.4875044301112,
-27.14995));
#243644=CARTESIAN_POINT('Ctrl Pts',(-52.4562630265793,-45.4874833394179,
-27.149949981182));
#243645=CARTESIAN_POINT('Ctrl Pts',(-52.4612401260371,-45.487394572175,
-27.1499499742965));
#243646=CARTESIAN_POINT('Ctrl Pts',(-52.4667587388206,-45.4872961469686,
-27.1499499666618));
#243647=CARTESIAN_POINT('Ctrl Pts',(-52.4720883220187,-45.4871148353533,
-27.1499499814094));
#243648=CARTESIAN_POINT('Ctrl Pts',(-52.4766216320627,-45.4869142695831,
-27.1499499942742));
#243649=CARTESIAN_POINT('Ctrl Pts',(-52.4777638653127,-45.4868637341268,
-27.1499499975157));
#243650=CARTESIAN_POINT('Ctrl Pts',(-52.4788556174783,-45.4868122411815,
-27.14995));
#243651=CARTESIAN_POINT('Ctrl Pts',(-52.4798872980886,-45.486761251452,
-27.14995));
#243652=CARTESIAN_POINT('Ctrl Pts',(-52.4856274379354,-45.4864775510753,
-27.14995));
#243653=CARTESIAN_POINT('Ctrl Pts',(-52.4924152853978,-45.4860650982164,
-27.1499498564486));
#243654=CARTESIAN_POINT('Ctrl Pts',(-52.4997470974223,-45.4854718698351,
-27.1499498264905));
#243655=CARTESIAN_POINT('Ctrl Pts',(-52.5020014705864,-45.4852894649755,
-27.149949817279));
#243656=CARTESIAN_POINT('Ctrl Pts',(-52.5043073701312,-45.4850903128208,
-27.1499498205136));
#243657=CARTESIAN_POINT('Ctrl Pts',(-52.5066504691328,-45.4848739122105,
-27.1499498482367));
#243658=CARTESIAN_POINT('Ctrl Pts',(-52.5138001026149,-45.4842135965139,
-27.1499499328297));
#243659=CARTESIAN_POINT('Ctrl Pts',(-52.5212928305955,-45.4834010173043,
-27.1499499622158));
#243660=CARTESIAN_POINT('Ctrl Pts',(-52.5287234875121,-45.4824712805355,
-27.1499499765901));
#243661=CARTESIAN_POINT('Ctrl Pts',(-52.5352735769052,-45.4816517219129,
-27.1499499892609));
#243662=CARTESIAN_POINT('Ctrl Pts',(-52.5417754929017,-45.4807422838156,
-27.1499499937208));
#243663=CARTESIAN_POINT('Ctrl Pts',(-52.5479631027218,-45.4797987114518,
-27.1499499898166));
#243664=CARTESIAN_POINT('Ctrl Pts',(-52.5566877067233,-45.4784682631107,
-27.1499499843116));
#243665=CARTESIAN_POINT('Ctrl Pts',(-52.5649219427036,-45.4770557430141,
-27.1499500428287));
#243666=CARTESIAN_POINT('Ctrl Pts',(-52.572986092149,-45.4755497840266,
-27.1499500764828));
#243667=CARTESIAN_POINT('Ctrl Pts',(-52.5813327839574,-45.4739910609858,
-27.1499501113161));
#243668=CARTESIAN_POINT('Ctrl Pts',(-52.5894975461691,-45.4723317537798,
-27.1499501069544));
#243669=CARTESIAN_POINT('Ctrl Pts',(-52.5978166954089,-45.4705078966956,
-27.1499500626457));
#243670=CARTESIAN_POINT('Ctrl Pts',(-52.6026387135951,-45.4694507366693,
-27.1499500369632));
#243671=CARTESIAN_POINT('Ctrl Pts',(-52.6075122389011,-45.4683374225039,
-27.14995));
#243672=CARTESIAN_POINT('Ctrl Pts',(-52.6124993356304,-45.4671482695449,
-27.14995));
#243673=CARTESIAN_POINT('Ctrl Pts',(-52.627793731053,-45.4635013830774,
-27.14995));
#243674=CARTESIAN_POINT('Ctrl Pts',(-52.6429619515309,-45.4594379777908,
-27.1499496611238));
#243675=CARTESIAN_POINT('Ctrl Pts',(-52.6579886217047,-45.4549557198868,
-27.1499498084471));
#243676=CARTESIAN_POINT('Ctrl Pts',(-52.6860026011899,-45.4465995185783,
-27.1499500830997));
#243677=CARTESIAN_POINT('Ctrl Pts',(-52.7135780856693,-45.4368490997121,
-27.1499486186568));
#243678=CARTESIAN_POINT('Ctrl Pts',(-52.7405840158337,-45.4259326684973,
-27.1499479502485));
#243679=CARTESIAN_POINT('Ctrl Pts',(-52.7613299576862,-45.4175466715759,
-27.1499474367776));
#243680=CARTESIAN_POINT('Ctrl Pts',(-52.7817402072434,-45.408472118313,
-27.1499474429761));
#243681=CARTESIAN_POINT('Ctrl Pts',(-52.8017665864966,-45.3987978865569,
-27.1499480642926));
#243682=CARTESIAN_POINT('Ctrl Pts',(-52.8108546681608,-45.3944076666811,
-27.1499483462494));
#243683=CARTESIAN_POINT('Ctrl Pts',(-52.8196245960772,-45.3900100214443,
-27.1499490848697));
#243684=CARTESIAN_POINT('Ctrl Pts',(-52.8284043464921,-45.385459859022,
-27.1499495201295));
#243685=CARTESIAN_POINT('Ctrl Pts',(-52.837148245319,-45.3809282769169,
-27.1499499536118));
#243686=CARTESIAN_POINT('Ctrl Pts',(-52.8459020777059,-45.3762451854422,
-27.149950050525));
#243687=CARTESIAN_POINT('Ctrl Pts',(-52.8549538192956,-45.3712314506474,
-27.1499500157449));
#243688=CARTESIAN_POINT('Ctrl Pts',(-52.8568413065408,-45.3701859766486,
-27.1499500084925));
#243689=CARTESIAN_POINT('Ctrl Pts',(-52.8587416139914,-45.3691260055679,
-27.14995));
#243690=CARTESIAN_POINT('Ctrl Pts',(-52.860657134334,-45.3680497216908,
-27.14995));
#243691=CARTESIAN_POINT('Ctrl Pts',(-52.8790418427447,-45.3577198051622,
-27.14995));
#243692=CARTESIAN_POINT('Ctrl Pts',(-52.8969351392667,-45.346949593182,
-27.1499512477437));
#243693=CARTESIAN_POINT('Ctrl Pts',(-52.9143346753781,-45.3357995458469,
-27.1499502874174));
#243694=CARTESIAN_POINT('Ctrl Pts',(-52.9354078751652,-45.3222953251814,
-27.149949124332));
#243695=CARTESIAN_POINT('Ctrl Pts',(-52.9557647883118,-45.3082165069823,
-27.1499463866147));
#243696=CARTESIAN_POINT('Ctrl Pts',(-52.9754070241005,-45.293686770453,
-27.1499452341524));
#243697=CARTESIAN_POINT('Ctrl Pts',(-52.9895115081847,-45.2832534145036,
-27.1499444066047));
#243698=CARTESIAN_POINT('Ctrl Pts',(-53.0030953312206,-45.2726984482425,
-27.1499455008849));
#243699=CARTESIAN_POINT('Ctrl Pts',(-53.016353957345,-45.2619395866555,
-27.1499467204705));
#243700=CARTESIAN_POINT('Ctrl Pts',(-53.0300370747147,-45.2508362668637,
-27.1499479791026));
#243701=CARTESIAN_POINT('Ctrl Pts',(-53.0433739841894,-45.2395153060101,
-27.1499492614315));
#243702=CARTESIAN_POINT('Ctrl Pts',(-53.0565343570519,-45.2278539896112,
-27.1499497201218));
#243703=CARTESIAN_POINT('Ctrl Pts',(-53.0630437485743,-45.2220860622963,
-27.1499499469995));
#243704=CARTESIAN_POINT('Ctrl Pts',(-53.069509252334,-45.216234425568,-27.14995));
#243705=CARTESIAN_POINT('Ctrl Pts',(-53.0759473313773,-45.2102819476699,
-27.14995));
#243706=CARTESIAN_POINT('Ctrl Pts',(-53.0919806669554,-45.1954579489247,
-27.14995));
#243707=CARTESIAN_POINT('Ctrl Pts',(-53.1078101056455,-45.1800393974224,
-27.1499491809342));
#243708=CARTESIAN_POINT('Ctrl Pts',(-53.1233647837272,-45.1640567641704,
-27.1499491278329));
#243709=CARTESIAN_POINT('Ctrl Pts',(-53.1297654807438,-45.1574799650599,
-27.1499491059819));
#243710=CARTESIAN_POINT('Ctrl Pts',(-53.136356763247,-45.1505658263301,
-27.1499477144818));
#243711=CARTESIAN_POINT('Ctrl Pts',(-53.1428321977,-45.143611524022,-27.149947486813));
#243712=CARTESIAN_POINT('Ctrl Pts',(-53.1495450082546,-45.1364022913024,
-27.1499472507983));
#243713=CARTESIAN_POINT('Ctrl Pts',(-53.1561332556085,-45.1291501133495,
-27.1499483370776));
#243714=CARTESIAN_POINT('Ctrl Pts',(-53.1623094714303,-45.1222061453175,
-27.1499493180657));
#243715=CARTESIAN_POINT('Ctrl Pts',(-53.1646538467079,-45.1195703457515,
-27.1499496904302));
#243716=CARTESIAN_POINT('Ctrl Pts',(-53.1669393916557,-45.1169791342172,
-27.14995));
#243717=CARTESIAN_POINT('Ctrl Pts',(-53.1691521892031,-45.1144522908955,
-27.14995));
#243718=CARTESIAN_POINT('Ctrl Pts',(-53.1832815234621,-45.0983176861041,
-27.14995));
#243719=CARTESIAN_POINT('Ctrl Pts',(-53.1976035909501,-45.0811624281401,
-27.1499475469042));
#243720=CARTESIAN_POINT('Ctrl Pts',(-53.2119604318319,-45.0629713614228,
-27.1499474781223));
#243721=CARTESIAN_POINT('Ctrl Pts',(-53.22537529149,-45.0459738472028,-27.1499474138532));
#243722=CARTESIAN_POINT('Ctrl Pts',(-53.2388193211434,-45.0280729758151,
-27.14995));
#243723=CARTESIAN_POINT('Ctrl Pts',(-53.2522038624528,-45.0092562151227,
-27.14995));
#243724=CARTESIAN_POINT('',(-46.5036191527319,-43.0538517754469,-27.14995));
#243725=CARTESIAN_POINT('',(3.82683432365091,-22.2062953451411,-27.14995));
#243726=CARTESIAN_POINT('',(-54.1572878000337,-24.5762611252214,-27.14995));
#243727=CARTESIAN_POINT('Origin',(0.,-12.9675000200281,-27.14995));
#243728=CARTESIAN_POINT('',(-59.9987583592935,-26.9958774300648,-27.1499499915518));
#243729=CARTESIAN_POINT('',(-60.645425573095,-27.2637357853684,-27.14995));
#243730=CARTESIAN_POINT('',(-60.3119373224971,-27.9655514979169,-27.1499499611521));
#243731=CARTESIAN_POINT('Ctrl Pts',(-60.3119375509452,-27.9655513976194,
-27.14995));
#243732=CARTESIAN_POINT('Ctrl Pts',(-60.315915240292,-27.9419723101595,
-27.14995));
#243733=CARTESIAN_POINT('Ctrl Pts',(-60.319153179389,-27.9190421520094,
-27.14995));
#243734=CARTESIAN_POINT('Ctrl Pts',(-60.3217313771192,-27.8968214356441,
-27.14995));
#243735=CARTESIAN_POINT('Ctrl Pts',(-60.3243095748493,-27.8746007192789,
-27.14995));
#243736=CARTESIAN_POINT('Ctrl Pts',(-60.3261016152477,-27.855008293032,
-27.14995));
#243737=CARTESIAN_POINT('Ctrl Pts',(-60.3275996320819,-27.8323854269183,
-27.14995));
#243738=CARTESIAN_POINT('Ctrl Pts',(-60.3305956657503,-27.7871396946909,
-27.14995));
#243739=CARTESIAN_POINT('Ctrl Pts',(-60.3311172816358,-27.7413426078692,
-27.14995));
#243740=CARTESIAN_POINT('Ctrl Pts',(-60.3294555661254,-27.6988630851455,
-27.14995));
#243741=CARTESIAN_POINT('Ctrl Pts',(-60.3277938506151,-27.6563835624219,
-27.14995));
#243742=CARTESIAN_POINT('Ctrl Pts',(-60.3239443539489,-27.6128971630214,
-27.14995));
#243743=CARTESIAN_POINT('Ctrl Pts',(-60.3173464366114,-27.5687770367428,
-27.14995));
#243744=CARTESIAN_POINT('Ctrl Pts',(-60.3140474779426,-27.5467169736035,
-27.14995));
#243745=CARTESIAN_POINT('Ctrl Pts',(-60.3100616489501,-27.5245016407786,
-27.14995));
#243746=CARTESIAN_POINT('Ctrl Pts',(-60.30532142818,-27.5021961390353,-27.14995));
#243747=CARTESIAN_POINT('Ctrl Pts',(-60.3005812074099,-27.4798906372921,
-27.14995));
#243748=CARTESIAN_POINT('Ctrl Pts',(-60.2947466238143,-27.4562643586996,
-27.14995));
#243749=CARTESIAN_POINT('Ctrl Pts',(-60.2887929107262,-27.435035580692,
-27.14995));
#243750=CARTESIAN_POINT('Ctrl Pts',(-60.27688548455,-27.3925780246767,-27.14995));
#243751=CARTESIAN_POINT('Ctrl Pts',(-60.2623025201996,-27.3504009664825,
-27.14995));
#243752=CARTESIAN_POINT('Ctrl Pts',(-60.2448262721408,-27.3092030144389,
-27.14995));
#243753=CARTESIAN_POINT('Ctrl Pts',(-60.2360881481114,-27.2886040384171,
-27.14995));
#243754=CARTESIAN_POINT('Ctrl Pts',(-60.226625880273,-27.268254849865,-27.14995));
#243755=CARTESIAN_POINT('Ctrl Pts',(-60.2164086170247,-27.24826843343,-27.14995));
#243756=CARTESIAN_POINT('Ctrl Pts',(-60.2061913537764,-27.2282820169949,
-27.14995));
#243757=CARTESIAN_POINT('Ctrl Pts',(-60.1944578757994,-27.2074570444496,
-27.14995));
#243758=CARTESIAN_POINT('Ctrl Pts',(-60.1834132478005,-27.1894928213111,
-27.14995));
#243759=CARTESIAN_POINT('Ctrl Pts',(-60.177890933801,-27.1805107097419,
-27.14995));
#243760=CARTESIAN_POINT('Ctrl Pts',(-60.1720349812705,-27.1713636479865,
-27.14995));
#243761=CARTESIAN_POINT('Ctrl Pts',(-60.1658052523223,-27.1620782693979,
-27.14995));
#243762=CARTESIAN_POINT('Ctrl Pts',(-60.1595755233741,-27.1527928908093,
-27.14995));
#243763=CARTESIAN_POINT('Ctrl Pts',(-60.1541727712369,-27.1449958026448,
-27.14995));
#243764=CARTESIAN_POINT('Ctrl Pts',(-60.14594718448,-27.1338491692113,-27.14995));
#243765=CARTESIAN_POINT('Ctrl Pts',(-60.1377215977232,-27.1227025357779,
-27.14995));
#243766=CARTESIAN_POINT('Ctrl Pts',(-60.1299471689708,-27.1128327042649,
-27.14995));
#243767=CARTESIAN_POINT('Ctrl Pts',(-60.1228187178762,-27.1041813790389,
-27.14995));
#243768=CARTESIAN_POINT('Ctrl Pts',(-60.1192544923289,-27.0998557164259,
-27.14995));
#243769=CARTESIAN_POINT('Ctrl Pts',(-60.1158492999601,-27.0958373343259,
-27.14995));
#243770=CARTESIAN_POINT('Ctrl Pts',(-60.1126231807877,-27.0921164159072,
-27.14995));
#243771=CARTESIAN_POINT('Ctrl Pts',(-60.1093970616152,-27.0883954974885,
-27.14995));
#243772=CARTESIAN_POINT('Ctrl Pts',(-60.1071557123175,-27.0858589013014,
-27.14995));
#243773=CARTESIAN_POINT('Ctrl Pts',(-60.1035059146068,-27.0818289508923,
-27.14995));
#243774=CARTESIAN_POINT('Ctrl Pts',(-60.0962063191852,-27.0737690500741,
-27.14995));
#243775=CARTESIAN_POINT('Ctrl Pts',(-60.0881358252403,-27.0653231937789,
-27.14995));
#243776=CARTESIAN_POINT('Ctrl Pts',(-60.0802510129,-27.0575828777573,-27.14995));
#243777=CARTESIAN_POINT('Ctrl Pts',(-60.0763086067298,-27.0537127197465,
-27.14995));
#243778=CARTESIAN_POINT('Ctrl Pts',(-60.0726275116169,-27.0501964597785,
-27.14995));
#243779=CARTESIAN_POINT('Ctrl Pts',(-60.068073229236,-27.0460154954056,
-27.14995));
#243780=CARTESIAN_POINT('Ctrl Pts',(-60.0635189468552,-27.0418345310327,
-27.14995));
#243781=CARTESIAN_POINT('Ctrl Pts',(-60.0608270167709,-27.0394009294251,
-27.14995));
#243782=CARTESIAN_POINT('Ctrl Pts',(-60.0551300882665,-27.0353595333066,
-27.14995));
#243783=CARTESIAN_POINT('Ctrl Pts',(-60.049433159762,-27.0313181371882,
-27.14995));
#243784=CARTESIAN_POINT('Ctrl Pts',(-60.0442902943263,-27.0276890843295,
-27.14995));
#243785=CARTESIAN_POINT('Ctrl Pts',(-60.0397289987587,-27.0244536454528,
-27.14995));
#243786=CARTESIAN_POINT('Ctrl Pts',(-60.0374483509749,-27.0228359260145,
-27.14995));
#243787=CARTESIAN_POINT('Ctrl Pts',(-60.0353125919848,-27.0213175666086,
-27.14995));
#243788=CARTESIAN_POINT('Ctrl Pts',(-60.0333232381725,-27.0198996133675,
-27.14995));
#243789=CARTESIAN_POINT('Ctrl Pts',(-60.0313338843601,-27.0184816601264,
-27.14995));
#243790=CARTESIAN_POINT('Ctrl Pts',(-60.0305214001357,-27.0179021513849,
-27.14995));
#243791=CARTESIAN_POINT('Ctrl Pts',(-60.0277868739454,-27.0159622808878,
-27.14995));
#243792=CARTESIAN_POINT('Ctrl Pts',(-60.0250523477551,-27.0140224103907,
-27.14995));
#243793=CARTESIAN_POINT('Ctrl Pts',(-60.0225438971918,-27.0122427021784,
-27.14995));
#243794=CARTESIAN_POINT('Ctrl Pts',(-60.0202643910877,-27.010625425684,
-27.14995));
#243795=CARTESIAN_POINT('Ctrl Pts',(-60.0179848849835,-27.0090081491896,
-27.14995));
#243796=CARTESIAN_POINT('Ctrl Pts',(-60.0175503464132,-27.0087004971746,
-27.14995));
#243797=CARTESIAN_POINT('Ctrl Pts',(-60.0141152667846,-27.0062636546787,
-27.14995));
#243798=CARTESIAN_POINT('Ctrl Pts',(-60.0072451122419,-27.0013899730315,
-27.14995));
#243799=CARTESIAN_POINT('Ctrl Pts',(-60.0026514387729,-26.9981429986844,
-27.14995));
#243800=CARTESIAN_POINT('Ctrl Pts',(-59.9987583829376,-26.9958773894365,
-27.14995));
#243801=CARTESIAN_POINT('',(-60.0785790019143,-28.6323101147099,-27.14995));
#243802=CARTESIAN_POINT('Ctrl Pts',(-60.0785790019143,-28.6323101147099,
-27.14995));
#243803=CARTESIAN_POINT('Ctrl Pts',(-60.1258286923341,-28.5202492179071,
-27.14995));
#243804=CARTESIAN_POINT('Ctrl Pts',(-60.1730775948717,-28.4178603385288,
-27.1499499999982));
#243805=CARTESIAN_POINT('Ctrl Pts',(-60.2584466045542,-28.193908983491,
-27.1499499999982));
#243806=CARTESIAN_POINT('Ctrl Pts',(-60.2916736659582,-28.0851185333452,
-27.14995));
#243807=CARTESIAN_POINT('Ctrl Pts',(-60.3119370945392,-27.9655515603093,
-27.14995));
#243808=CARTESIAN_POINT('',(-60.0745809370706,-28.6418766476167,-27.1499500000522));
#243809=CARTESIAN_POINT('Ctrl Pts',(-60.0745809362347,-28.6418766496844,
-27.14995));
#243810=CARTESIAN_POINT('Ctrl Pts',(-60.0752422385998,-28.6402801245457,
-27.14995));
#243811=CARTESIAN_POINT('Ctrl Pts',(-60.0759060662479,-28.638684646748,
-27.1499500000006));
#243812=CARTESIAN_POINT('Ctrl Pts',(-60.0772387597021,-28.6354957964475,
-27.1499500000006));
#243813=CARTESIAN_POINT('Ctrl Pts',(-60.0779076244668,-28.6339024264159,
-27.14995));
#243814=CARTESIAN_POINT('Ctrl Pts',(-60.0785790019143,-28.6323101147099,
-27.14995));
#243815=CARTESIAN_POINT('',(-57.855180104188,-33.9999842387537,-27.14995));
#243816=CARTESIAN_POINT('',(-60.2627421407299,-28.1876153178796,-27.14995));
#243817=CARTESIAN_POINT('',(-58.2526348815488,-33.7356511576002,-27.14995));
#243818=CARTESIAN_POINT('Ctrl Pts',(-57.8551801041881,-33.9999842387536,
-27.14995));
#243819=CARTESIAN_POINT('Ctrl Pts',(-57.8844567986838,-33.9293040458406,
-27.14995));
#243820=CARTESIAN_POINT('Ctrl Pts',(-57.9260258713737,-33.8474501205147,
-27.14995));
#243821=CARTESIAN_POINT('Ctrl Pts',(-57.9971602307868,-33.7539381089864,
-27.14995));
#243822=CARTESIAN_POINT('Ctrl Pts',(-58.0308423626586,-33.7180928013356,
-27.14995));
#243823=CARTESIAN_POINT('Ctrl Pts',(-58.0818873760537,-33.6855661818695,
-27.14995));
#243824=CARTESIAN_POINT('Ctrl Pts',(-58.1031888603429,-33.6757705412644,
-27.14995));
#243825=CARTESIAN_POINT('Ctrl Pts',(-58.1368964656122,-33.6687990467782,
-27.14995));
#243826=CARTESIAN_POINT('Ctrl Pts',(-58.1547533666348,-33.6685040991281,
-27.14995));
#243827=CARTESIAN_POINT('Ctrl Pts',(-58.1837596142463,-33.674737141348,
-27.14995));
#243828=CARTESIAN_POINT('Ctrl Pts',(-58.1998209469314,-33.6822762393232,
-27.14995));
#243829=CARTESIAN_POINT('Ctrl Pts',(-58.2272377777507,-33.7022330937833,
-27.14995));
#243830=CARTESIAN_POINT('Ctrl Pts',(-58.242259343044,-33.7195847204375,
-27.14995));
#243831=CARTESIAN_POINT('Ctrl Pts',(-58.2526348815488,-33.7356511576002,
-27.14995));
#243832=CARTESIAN_POINT('Origin',(-40.1177331105385,-29.5848091660776,-27.14995));
#243833=CARTESIAN_POINT('Origin',(0.,2.17747716649809E-16,-28.54995));
#243834=CARTESIAN_POINT('',(-2.46951155546522E-15,59.91999999,-28.54995));
#243835=CARTESIAN_POINT('Origin',(-1.73472347597681E-15,53.91999999,-28.54995));
#243836=CARTESIAN_POINT('',(-2.10211751572101E-15,56.91999999,-28.54995));
#243837=CARTESIAN_POINT('Origin',(-1.73472347597681E-15,53.91999999,-28.54995));
#243838=CARTESIAN_POINT('Origin',(-1.73472347597681E-15,53.91999999,-45.5205127484771));
#243839=CARTESIAN_POINT('',(-2.10211751572101E-15,56.91999999,-27.14995));
#243840=CARTESIAN_POINT('',(-2.10211751572101E-15,56.91999999,-45.5205127484771));
#243841=CARTESIAN_POINT('Origin',(-1.73472347597681E-15,53.91999999,-27.14995));
#243842=CARTESIAN_POINT('Origin',(-1.73472347597681E-15,53.91999999,-45.5205127484771));
#243843=CARTESIAN_POINT('',(-2.46951155546522E-15,59.91999999,-45.5205127484771));
#243844=CARTESIAN_POINT('Origin',(0.,0.,-27.14995));
#243845=CARTESIAN_POINT('Origin',(12.9675000200281,-12.967500020028,-28.54995));
#243846=CARTESIAN_POINT('',(72.8875000100282,-12.9675000200274,-28.54995));
#243847=CARTESIAN_POINT('Origin',(66.8875000100282,-12.9675000200274,-28.54995));
#243848=CARTESIAN_POINT('',(69.8875000100282,-12.9675000200274,-28.54995));
#243849=CARTESIAN_POINT('Origin',(66.8875000100282,-12.9675000200274,-28.54995));
#243850=CARTESIAN_POINT('Origin',(66.8875000100282,-12.9675000200274,-45.5205127484772));
#243851=CARTESIAN_POINT('',(69.8875000100282,-12.9675000200274,-27.14995));
#243852=CARTESIAN_POINT('',(69.8875000100282,-12.9675000200274,-45.5205127484772));
#243853=CARTESIAN_POINT('Origin',(66.8875000100282,-12.9675000200274,-27.14995));
#243854=CARTESIAN_POINT('Origin',(66.8875000100282,-12.9675000200274,-45.5205127484772));
#243855=CARTESIAN_POINT('',(72.8875000100282,-12.9675000200274,-45.5205127484772));
#243856=CARTESIAN_POINT('Origin',(0.,0.,-27.14995));
#243857=CARTESIAN_POINT('Origin',(-12.9675000200281,-12.9675000200282,-28.54995));
#243858=CARTESIAN_POINT('',(-72.8875000100282,-12.9675000200284,-28.54995));
#243859=CARTESIAN_POINT('Origin',(-66.8875000100282,-12.9675000200284,-28.54995));
#243860=CARTESIAN_POINT('',(-69.8875000100282,-12.9675000200284,-28.54995));
#243861=CARTESIAN_POINT('Origin',(-66.8875000100282,-12.9675000200284,-28.54995));
#243862=CARTESIAN_POINT('Origin',(-66.8875000100282,-12.9675000200284,-45.5205127484772));
#243863=CARTESIAN_POINT('',(-69.8875000100282,-12.9675000200284,-27.14995));
#243864=CARTESIAN_POINT('',(-69.8875000100282,-12.9675000200284,-45.5205127484772));
#243865=CARTESIAN_POINT('Origin',(-66.8875000100282,-12.9675000200284,-27.14995));
#243866=CARTESIAN_POINT('Origin',(-66.8875000100282,-12.9675000200284,-45.5205127484772));
#243867=CARTESIAN_POINT('',(-72.8875000100282,-12.9675000200284,-19.1495981543667));
#243868=CARTESIAN_POINT('Ctrl Pts',(-63.0894692252869,-17.612385611532,
-27.14995));
#243869=CARTESIAN_POINT('Ctrl Pts',(-63.5471016769306,-17.9865825869362,
-27.14995));
#243870=CARTESIAN_POINT('Ctrl Pts',(-64.0759568113924,-18.3017783306405,
-27.1170384642544));
#243871=CARTESIAN_POINT('Ctrl Pts',(-65.3769931585463,-18.8297394406605,
-26.9140019035161));
#243872=CARTESIAN_POINT('Ctrl Pts',(-66.1724941403793,-18.9675000200284,
-26.6941821528334));
#243873=CARTESIAN_POINT('Ctrl Pts',(-67.7431470572572,-18.9675000200284,
-26.0493222880549));
#243874=CARTESIAN_POINT('Ctrl Pts',(-68.5842584032391,-18.7773839207075,
-25.5566509641909));
#243875=CARTESIAN_POINT('Ctrl Pts',(-70.0405902601868,-18.1339073024589,
-24.3988971850764));
#243876=CARTESIAN_POINT('Ctrl Pts',(-70.6574511542138,-17.6828302500813,
-23.7346108572202));
#243877=CARTESIAN_POINT('Ctrl Pts',(-71.6953344410442,-16.644946963251,
-22.3309543073884));
#243878=CARTESIAN_POINT('Ctrl Pts',(-72.1391640112646,-15.965192613364,
-21.4806501260797));
#243879=CARTESIAN_POINT('Ctrl Pts',(-72.5723511030316,-14.9230055464081,
-20.3496274930716));
#243880=CARTESIAN_POINT('Ctrl Pts',(-72.6783812619408,-14.5802499618463,
-20.0034708627134));
#243881=CARTESIAN_POINT('Ctrl Pts',(-72.7936053444643,-14.0406964652972,
-19.5690738680634));
#243882=CARTESIAN_POINT('Ctrl Pts',(-72.8242996686683,-13.8590796780428,
-19.4400001816203));
#243883=CARTESIAN_POINT('Ctrl Pts',(-72.8706981898791,-13.4592683047818,
-19.2329336835229));
#243884=CARTESIAN_POINT('Ctrl Pts',(-72.8875000100282,-13.2439920760961,
-19.1495981543667));
#243885=CARTESIAN_POINT('Ctrl Pts',(-72.8875000100282,-12.9675000200284,
-19.1495981543667));
#243886=CARTESIAN_POINT('',(-72.8875000100282,-12.9675000200284,-45.5205127484772));
#243887=CARTESIAN_POINT('Ctrl Pts',(-72.8875000100282,-12.9675000200284,
-19.1495981543667));
#243888=CARTESIAN_POINT('Ctrl Pts',(-72.8875000100282,-12.7143686770247,
-19.1495981543667));
#243889=CARTESIAN_POINT('Ctrl Pts',(-72.8731254021373,-12.5111144844339,
-19.220932038759));
#243890=CARTESIAN_POINT('Ctrl Pts',(-72.8323299217736,-12.1338327493845,
-19.4050676822193));
#243891=CARTESIAN_POINT('Ctrl Pts',(-72.8051266450376,-11.9616848910719,
-19.5215236887874));
#243892=CARTESIAN_POINT('Ctrl Pts',(-72.7033687071041,-11.4523905224552,
-19.9151662946502));
#243893=CARTESIAN_POINT('Ctrl Pts',(-72.609889943601,-11.1300135832241,
-20.2316301675614));
#243894=CARTESIAN_POINT('Ctrl Pts',(-72.2319065968022,-10.1522326657623,
-21.2677761539189));
#243895=CARTESIAN_POINT('Ctrl Pts',(-71.8480681919679,-9.51569868903438,
-22.0510777895308));
#243896=CARTESIAN_POINT('Ctrl Pts',(-70.8903178012519,-8.44072115508987,
-23.4642017994411));
#243897=CARTESIAN_POINT('Ctrl Pts',(-70.2528967393358,-7.92767447817741,
-24.1985795660467));
#243898=CARTESIAN_POINT('Ctrl Pts',(-68.7170274778242,-7.19008180081177,
-25.4763223240037));
#243899=CARTESIAN_POINT('Ctrl Pts',(-67.8170490374015,-6.96750002002839,
-26.018980498083));
#243900=CARTESIAN_POINT('Ctrl Pts',(-66.1804258126876,-6.96750002002839,
-26.6909256618053));
#243901=CARTESIAN_POINT('Ctrl Pts',(-65.3934975758082,-7.10219196742949,
-26.9096248240429));
#243902=CARTESIAN_POINT('Ctrl Pts',(-64.0901992025078,-7.6247696746572,
-27.1161425394507));
#243903=CARTESIAN_POINT('Ctrl Pts',(-63.5528101105262,-7.94374978023574,
-27.14995));
#243904=CARTESIAN_POINT('Ctrl Pts',(-63.0894692252869,-8.3226144285248,
-27.14995));
#243905=CARTESIAN_POINT('Origin',(0.,0.,-27.14995));
#243906=CARTESIAN_POINT('Origin',(0.,-25.9350000400563,-28.54995));
#243907=CARTESIAN_POINT('',(2.46951155546522E-15,-85.8550000300563,-28.54995));
#243908=CARTESIAN_POINT('Origin',(1.73472347597681E-15,-79.8550000300563,
-28.54995));
#243909=CARTESIAN_POINT('',(2.10211751572101E-15,-82.8550000300563,-28.54995));
#243910=CARTESIAN_POINT('Origin',(1.73472347597681E-15,-79.8550000300563,
-28.54995));
#243911=CARTESIAN_POINT('Origin',(1.73472347597681E-15,-79.8550000300563,
-45.5205127484772));
#243912=CARTESIAN_POINT('',(2.10211751572101E-15,-82.8550000300563,-27.14995));
#243913=CARTESIAN_POINT('',(2.10211751572101E-15,-82.8550000300563,-45.5205127484772));
#243914=CARTESIAN_POINT('Origin',(1.73472347597681E-15,-79.8550000300563,
-27.14995));
#243915=CARTESIAN_POINT('Origin',(1.73472347597681E-15,-79.8550000300563,
-45.5205127484772));
#243916=CARTESIAN_POINT('',(9.99935396488397E-16,-85.8550000300563,-27.14995));
#243917=CARTESIAN_POINT('Origin',(1.73472347597681E-15,-79.8550000300563,
-27.14995));
#243918=CARTESIAN_POINT('',(2.46951155546522E-15,-85.8550000300563,-45.5205127484772));
#243919=CARTESIAN_POINT('Origin',(1.73472347597681E-15,-79.8550000300563,
-27.14995));
#243920=CARTESIAN_POINT('Origin',(0.,0.,-27.14995));
#243921=CARTESIAN_POINT('Origin',(-55.0820026611041,-35.7832125649284,-33.0452518248346));
#243922=CARTESIAN_POINT('',(-52.4032186345485,-42.2503692925074,-33.0452518248346));
#243923=CARTESIAN_POINT('Origin',(-55.0820026611041,-35.7832125649284,-33.0452518248346));
#243924=CARTESIAN_POINT('Origin',(-55.0820026611041,-35.7832125649284,-33.0452518248346));
#243925=CARTESIAN_POINT('Origin',(-54.8649619663051,-35.6933113655558,-32.9597467890032));
#243926=CARTESIAN_POINT('Origin',(-58.1205723882901,-37.0418293561452,-34.2423223264744));
#243927=CARTESIAN_POINT('',(-60.5940855103344,-31.6841242185413,-34.3278273623058));
#243928=CARTESIAN_POINT('Origin',(-58.3376130830891,-37.1317305555178,-34.3278273623058));
#243929=CARTESIAN_POINT('',(-60.5981652751394,-31.4944723962724,-34.3027835171364));
#243930=CARTESIAN_POINT('Origin',(-60.3770448155354,-31.5942230191687,-34.2423223264744));
#243931=CARTESIAN_POINT('',(-55.9499213956124,-42.7163258114444,-34.3027835171364));
#243932=CARTESIAN_POINT('Origin',(-58.2740433353759,-37.1053991038583,-34.3027835171364));
#243933=CARTESIAN_POINT('Origin',(-58.2740433353759,-37.1053991038583,-34.3027835171364));
#243934=CARTESIAN_POINT('Origin',(-57.3795491045205,-36.7348874619736,-33.9503898734876));
#243935=CARTESIAN_POINT('',(-54.8822573706237,-43.1979644247475,-34.0108510641496));
#243936=CARTESIAN_POINT('',(-60.183782732589,-30.398949994626,-34.0108510641496));
#243937=CARTESIAN_POINT('Origin',(-57.5330200516063,-36.7984572096868,-34.0108510641496));
#243938=CARTESIAN_POINT('Origin',(-57.5330200516063,-36.7984572096868,-34.0108510641496));
#243939=CARTESIAN_POINT('',(-60.0583331310761,-30.2677307343945,-33.9503898734876));
#243940=CARTESIAN_POINT('Origin',(-59.9626622729849,-30.4987006175224,-33.9503898734876));
#243941=CARTESIAN_POINT('',(-54.7007650779648,-43.2020441895526,-33.9503898734876));
#243942=CARTESIAN_POINT('Origin',(-57.3795491045205,-36.7348874619736,-33.9503898734876));
#243943=CARTESIAN_POINT('Origin',(-57.3795491045205,-36.7348874619736,-33.9503898734876));
#243944=CARTESIAN_POINT('Origin',(-56.4399049639283,-34.7833755446169,-30.7021592582377));
#243945=CARTESIAN_POINT('',(-57.886842929255,-35.3827168737675,-31.2721928304471));
#243946=CARTESIAN_POINT('',(-59.679932565128,-36.125438919497,-31.9785958103411));
#243947=CARTESIAN_POINT('',(-56.4399049639283,-34.7833755446169,-30.7021592582377));
#243948=CARTESIAN_POINT('',(-59.4423249965411,-34.4647200715469,-34.3278273623058));
#243949=CARTESIAN_POINT('Ctrl Pts',(-59.6799325651279,-36.125438919497,
-31.9785958103412));
#243950=CARTESIAN_POINT('Ctrl Pts',(-58.934586262998,-35.0355570872307,
-32.9063798090518));
#243951=CARTESIAN_POINT('Ctrl Pts',(-59.442324996541,-34.464720071547,-34.3278273623057));
#243952=CARTESIAN_POINT('',(-57.6492353606681,-33.7219980258176,-33.6214243824119));
#243953=CARTESIAN_POINT('',(-56.2022973953414,-33.1226566966669,-33.0513908102024));
#243954=CARTESIAN_POINT('Ctrl Pts',(-57.649235360668,-33.7219980258177,
-33.6214243824119));
#243955=CARTESIAN_POINT('Ctrl Pts',(-57.4063046536298,-34.402522117505,
-32.3043002133772));
#243956=CARTESIAN_POINT('Ctrl Pts',(-57.8868429292549,-35.3827168737677,
-31.2721928304472));
#243957=CARTESIAN_POINT('Origin',(-55.3351930504764,-37.4503860285879,-30.7021592582377));
#243958=CARTESIAN_POINT('',(-56.782131015803,-38.0497273577386,-31.2721928304472));
#243959=CARTESIAN_POINT('',(-58.575220651676,-38.7924494034679,-31.9785958103411));
#243960=CARTESIAN_POINT('',(-55.3351930504764,-37.4503860285879,-30.7021592582377));
#243961=CARTESIAN_POINT('Ctrl Pts',(-58.575220651676,-38.7924494034677,
-31.978595810341));
#243962=CARTESIAN_POINT('Ctrl Pts',(-58.5010340905656,-37.1994217531912,
-31.7317640330694));
#243963=CARTESIAN_POINT('Ctrl Pts',(-59.6799325651279,-36.1254389194971,
-31.978595810341));
#243964=CARTESIAN_POINT('Ctrl Pts',(-57.8868429292551,-35.3827168737676,
-31.2721928304471));
#243965=CARTESIAN_POINT('Ctrl Pts',(-56.9727524811973,-36.5663867834655,
-31.1296844373948));
#243966=CARTESIAN_POINT('Ctrl Pts',(-56.782131015803,-38.0497273577387,
-31.2721928304471));
#243967=CARTESIAN_POINT('Origin',(-53.9928735684375,-38.4566776646086,-33.0513908102024));
#243968=CARTESIAN_POINT('',(-55.4398115337641,-39.0560189937595,-33.6214243824119));
#243969=CARTESIAN_POINT('',(-57.2329011696371,-39.7987410394886,-34.3278273623058));
#243970=CARTESIAN_POINT('',(-53.9928735684375,-38.4566776646086,-33.0513908102024));
#243971=CARTESIAN_POINT('Ctrl Pts',(-57.2329011696371,-39.7987410394885,
-34.3278273623054));
#243972=CARTESIAN_POINT('Ctrl Pts',(-57.2775183928202,-39.0360728131871,
-32.9063798090518));
#243973=CARTESIAN_POINT('Ctrl Pts',(-58.5752206516756,-38.792449403468,
-31.9785958103413));
#243974=CARTESIAN_POINT('Ctrl Pts',(-56.782131015803,-38.0497273577387,
-31.2721928304471));
#243975=CARTESIAN_POINT('Ctrl Pts',(-55.7492367834519,-38.4030378434613,
-32.3043002133771));
#243976=CARTESIAN_POINT('Ctrl Pts',(-55.4398115337641,-39.0560189937594,
-33.6214243824119));
#243977=CARTESIAN_POINT('Origin',(-53.7552659998506,-36.7959588166585,-35.4006223621673));
#243978=CARTESIAN_POINT('',(-55.2022039651772,-37.3953001458094,-35.9706559343767));
#243979=CARTESIAN_POINT('',(-56.9952936010502,-38.1380221915386,-36.6770589142706));
#243980=CARTESIAN_POINT('',(-53.7552659998506,-36.7959588166585,-35.4006223621673));
#243981=CARTESIAN_POINT('Ctrl Pts',(-56.9952936010502,-38.1380221915386,
-36.6770589142705));
#243982=CARTESIAN_POINT('Ctrl Pts',(-56.4875548675072,-38.7088592072223,
-35.2556113610166));
#243983=CARTESIAN_POINT('Ctrl Pts',(-57.2329011696371,-39.7987410394886,
-34.3278273623059));
#243984=CARTESIAN_POINT('Ctrl Pts',(-55.4398115337641,-39.0560189937594,
-33.6214243824119));
#243985=CARTESIAN_POINT('Ctrl Pts',(-54.959273258139,-38.0758242374967,
-34.6535317653419));
#243986=CARTESIAN_POINT('Ctrl Pts',(-55.2022039651772,-37.3953001458093,
-35.9706559343767));
#243987=CARTESIAN_POINT('Origin',(-54.8599779133025,-34.1289483326876,-35.4006223621673));
#243988=CARTESIAN_POINT('',(-56.3069158786292,-34.7282896618384,-35.9706559343767));
#243989=CARTESIAN_POINT('',(-58.1000055145022,-35.4710117075677,-36.6770589142706));
#243990=CARTESIAN_POINT('',(-54.8599779133025,-34.1289483326876,-35.4006223621673));
#243991=CARTESIAN_POINT('Ctrl Pts',(-58.100005514502,-35.4710117075679,
-36.6770589142706));
#243992=CARTESIAN_POINT('Ctrl Pts',(-56.9211070399398,-36.5449945412619,
-36.430227136999));
#243993=CARTESIAN_POINT('Ctrl Pts',(-56.9952936010502,-38.1380221915383,
-36.6770589142706));
#243994=CARTESIAN_POINT('Ctrl Pts',(-55.2022039651772,-37.3953001458093,
-35.9706559343767));
#243995=CARTESIAN_POINT('Ctrl Pts',(-55.3928254305715,-35.9119595715362,
-35.8281475413243));
#243996=CARTESIAN_POINT('Ctrl Pts',(-56.3069158786292,-34.7282896618384,
-35.9706559343767));
#243997=CARTESIAN_POINT('Origin',(-56.2022973953414,-33.1226566966669,-33.0513908102024));
#243998=CARTESIAN_POINT('Ctrl Pts',(-59.4423249965407,-34.464720071547,
-34.3278273623061));
#243999=CARTESIAN_POINT('Ctrl Pts',(-58.1446227376852,-34.7083434812661,
-35.2556113610166));
#244000=CARTESIAN_POINT('Ctrl Pts',(-58.1000055145022,-35.4710117075675,
-36.6770589142702));
#244001=CARTESIAN_POINT('Ctrl Pts',(-56.3069158786292,-34.7282896618385,
-35.9706559343767));
#244002=CARTESIAN_POINT('Ctrl Pts',(-56.6163411283169,-34.0753085115404,
-34.6535317653419));
#244003=CARTESIAN_POINT('Ctrl Pts',(-57.6492353606681,-33.7219980258177,
-33.6214243824118));
#244004=CARTESIAN_POINT('Origin',(-56.6012875246971,-36.4125209605368,-33.6437870756545));
#244005=CARTESIAN_POINT('',(-55.0975854818894,-35.7896671806377,-33.0513908102024));
#244006=CARTESIAN_POINT('',(-57.7493378217924,-33.6408823630029,-33.6437870756545));
#244007=CARTESIAN_POINT('Origin',(-58.3376130830891,-37.1317305555178,-34.3278273623058));
#244008=CARTESIAN_POINT('Origin',(-58.3376130830891,-37.1317305555178,-34.3278273623058));
#244009=CARTESIAN_POINT('Origin',(-58.3376130830891,-37.1317305555178,-34.3278273623058));
#244010=CARTESIAN_POINT('Origin',(-58.3376130830891,-37.1317305555178,-34.3278273623058));
#244011=CARTESIAN_POINT('Origin',(-58.3376130830891,-37.1317305555178,-34.3278273623058));
#244012=CARTESIAN_POINT('Origin',(-58.3376130830891,-37.1317305555178,-34.3278273623058));
#244013=CARTESIAN_POINT('Origin',(-58.3376130830891,-37.1317305555178,-34.3278273623058));
#244014=CARTESIAN_POINT('Origin',(-58.3376130830891,-37.1317305555178,-34.3278273623058));
#244015=CARTESIAN_POINT('Origin',(-58.3376130830891,-37.1317305555178,-34.3278273623058));
#244016=CARTESIAN_POINT('Origin',(-58.3376130830891,-37.1317305555178,-34.3278273623058));
#244017=CARTESIAN_POINT('Origin',(-58.3376130830891,-37.1317305555178,-34.3278273623058));
#244018=CARTESIAN_POINT('Origin',(-58.3376130830891,-37.1317305555178,-34.3278273623058));
#244019=CARTESIAN_POINT('Origin',(-58.3376130830891,-37.1317305555178,-34.3278273623058));
#244020=CARTESIAN_POINT('',(-56.0415124888986,-42.6750077505855,-34.3278273623058));
#244021=CARTESIAN_POINT('Origin',(-58.3376130830891,-37.1317305555178,-34.3278273623058));
#244022=CARTESIAN_POINT('Origin',(-58.3376130830891,-37.1317305555178,-34.3278273623058));
#244023=CARTESIAN_POINT('',(-55.6588290565335,-43.5988872830968,-34.3278273623058));
#244024=CARTESIAN_POINT('Ctrl Pts',(-43.4805771074156,-59.5712767529309,
-39.2399080357013));
#244025=CARTESIAN_POINT('Ctrl Pts',(-43.4150727209207,-59.5358440364426,
-39.2223070534893));
#244026=CARTESIAN_POINT('Ctrl Pts',(-43.2883193276586,-59.4590682572254,
-39.1867578392588));
#244027=CARTESIAN_POINT('Ctrl Pts',(-43.1106712693135,-59.32658002426,-39.1324031814995));
#244028=CARTESIAN_POINT('Ctrl Pts',(-43.0005921597408,-59.2266373021163,
-39.0954660506179));
#244029=CARTESIAN_POINT('Ctrl Pts',(-42.8948534568781,-59.1207134074407,
-39.0581733199915));
#244030=CARTESIAN_POINT('Ctrl Pts',(-42.7951360401793,-59.0104958554849,
-39.0211184761739));
#244031=CARTESIAN_POINT('Ctrl Pts',(-42.6850011896347,-58.8622904152127,
-38.9753582681256));
#244032=CARTESIAN_POINT('Ctrl Pts',(-42.6055727997797,-58.7375004045667,
-38.939089851323));
#244033=CARTESIAN_POINT('Ctrl Pts',(-42.5503788594446,-58.6407591922129,
-38.9120596161462));
#244034=CARTESIAN_POINT('Ctrl Pts',(-42.5165536369311,-58.5741539171446,
-38.8941613358138));
#244035=CARTESIAN_POINT('Ctrl Pts',(-42.4842288567228,-58.5064298632496,
-38.8763157156907));
#244036=CARTESIAN_POINT('Ctrl Pts',(-42.4689425396028,-58.4722695523732,
-38.8674882509199));
#244037=CARTESIAN_POINT('Ctrl Pts',(-42.4257123024776,-58.3690064948315,
-38.8413136266604));
#244038=CARTESIAN_POINT('Ctrl Pts',(-42.3750272156063,-58.229152189777,
-38.8072100415055));
#244039=CARTESIAN_POINT('Ctrl Pts',(-42.3380647902547,-58.0850119200902,
-38.7746901633276));
#244040=CARTESIAN_POINT('Ctrl Pts',(-42.3155659796374,-57.9752818499468,
-38.7509105250088));
#244041=CARTESIAN_POINT('Ctrl Pts',(-42.3089374211558,-57.9384266221928,
-38.7430843922672));
#244042=CARTESIAN_POINT('Ctrl Pts',(-42.297458012674,-57.864178756387,-38.7276438637217));
#244043=CARTESIAN_POINT('Ctrl Pts',(-42.292601515188,-57.8267325312259,
-38.720018782004));
#244044=CARTESIAN_POINT('Ctrl Pts',(-42.2847289916893,-57.7514526301959,
-38.7050196673963));
#244045=CARTESIAN_POINT('Ctrl Pts',(-42.2817363521424,-57.7138759968928,
-38.6976962453237));
#244046=CARTESIAN_POINT('Ctrl Pts',(-42.277596992864,-57.6387184974263,
-38.6833720377019));
#244047=CARTESIAN_POINT('Ctrl Pts',(-42.2741651307842,-57.5260409596698,
-38.6623829091612));
#244048=CARTESIAN_POINT('Ctrl Pts',(-42.2805893100654,-57.3760354719141,
-38.6363740800325));
#244049=CARTESIAN_POINT('Ctrl Pts',(-42.2937061680812,-57.2637038035873,
-38.618370061439));
#244050=CARTESIAN_POINT('Ctrl Pts',(-42.3043247017591,-57.1888547452426,
-38.6067079534822));
#244051=CARTESIAN_POINT('Ctrl Pts',(-42.3105743117123,-57.1514345461221,
-38.6010450635964));
#244052=CARTESIAN_POINT('Ctrl Pts',(-42.3249704170347,-57.0766935209607,
-38.590076215021));
#244053=CARTESIAN_POINT('Ctrl Pts',(-42.3331592025312,-57.0392159768686,
-38.5847494243559));
#244054=CARTESIAN_POINT('Ctrl Pts',(-42.3512949844302,-56.9651221381903,
-38.5745673038812));
#244055=CARTESIAN_POINT('Ctrl Pts',(-42.3712216906218,-56.8916587034686,
-38.564820665347));
#244056=CARTESIAN_POINT('Ctrl Pts',(-42.4063979707918,-56.7834465224234,
-38.5515118436));
#244057=CARTESIAN_POINT('Ctrl Pts',(-42.4468320479729,-56.6771725078319,
-38.5395042677724));
#244058=CARTESIAN_POINT('Ctrl Pts',(-42.4925290654744,-56.5728473165674,
-38.5288039137004));
#244059=CARTESIAN_POINT('Ctrl Pts',(-42.5265325119253,-56.5046058456765,
-38.5225509073062));
#244060=CARTESIAN_POINT('Ctrl Pts',(-42.5623338475306,-56.4370293947697,
-38.5167461666044));
#244061=CARTESIAN_POINT('Ctrl Pts',(-42.5811223641794,-56.4035923099625,
-38.5140693065785));
#244062=CARTESIAN_POINT('Ctrl Pts',(-42.620584523009,-56.3373241998654,
-38.5091697400817));
#244063=CARTESIAN_POINT('Ctrl Pts',(-42.6411082254821,-56.3047465904101,
-38.5069659500128));
#244064=CARTESIAN_POINT('Ctrl Pts',(-42.7048067991197,-56.2090283357163,
-38.501110858935));
#244065=CARTESIAN_POINT('Ctrl Pts',(-42.7502234543428,-56.1476408662828,
-38.4981890389281));
#244066=CARTESIAN_POINT('Ctrl Pts',(-42.8467942323831,-56.0297655581676,
-38.4942910511033));
#244067=CARTESIAN_POINT('Ctrl Pts',(-42.8979715413934,-55.9732420482176,
-38.4933125989996));
#244068=CARTESIAN_POINT('Ctrl Pts',(-42.9790570553347,-55.8921695883033,
-38.4933149859729));
#244069=CARTESIAN_POINT('Ctrl Pts',(-43.0068374106561,-55.8657400908868,
-38.4935622007431));
#244070=CARTESIAN_POINT('Ctrl Pts',(-43.0495800649421,-55.8270637749536,
-38.4943063068789));
#244071=CARTESIAN_POINT('Ctrl Pts',(-43.0640222060113,-55.8143203511958,
-38.494617152342));
#244072=CARTESIAN_POINT('Ctrl Pts',(-43.0932714774893,-55.7891564261061,
-38.4953646906773));
#244073=CARTESIAN_POINT('Ctrl Pts',(-43.1080901283632,-55.7767277938553,
-38.4958020036096));
#244074=CARTESIAN_POINT('Ctrl Pts',(-43.1528523310046,-55.7401327167866,
-38.4972962980169));
#244075=CARTESIAN_POINT('Ctrl Pts',(-43.2134913856688,-55.6930468850421,
-38.4997758707861));
#244076=CARTESIAN_POINT('Ctrl Pts',(-43.3385569247743,-55.6055389451161,
-38.5066450244003));
#244077=CARTESIAN_POINT('Ctrl Pts',(-43.4691986576013,-55.5278792007279,
-38.5163302992824));
#244078=CARTESIAN_POINT('Ctrl Pts',(-43.5713395927684,-55.4769743237494,
-38.5256877381308));
#244079=CARTESIAN_POINT('Ctrl Pts',(-43.6403672861995,-55.4446857735354,
-38.5323951500278));
#244080=CARTESIAN_POINT('Ctrl Pts',(-43.6753577685123,-55.4293620157832,
-38.5359845633874));
#244081=CARTESIAN_POINT('Ctrl Pts',(-43.7462462065788,-55.4003985583156,
-38.5436333065981));
#244082=CARTESIAN_POINT('Ctrl Pts',(-43.7822717759725,-55.3867204456352,
-38.5477088862383));
#244083=CARTESIAN_POINT('Ctrl Pts',(-43.8543821738219,-55.3613797848081,
-38.5562346427694));
#244084=CARTESIAN_POINT('Ctrl Pts',(-43.890622407919,-55.349649082917,-38.5607007444526));
#244085=CARTESIAN_POINT('Ctrl Pts',(-43.9997560709039,-55.3172704656441,
-38.5746802407103));
#244086=CARTESIAN_POINT('Ctrl Pts',(-44.1098017310836,-55.290468361793,
-38.5898286859852));
#244087=CARTESIAN_POINT('Ctrl Pts',(-44.2583166685835,-55.2656490138239,
-38.612301023075));
#244088=CARTESIAN_POINT('Ctrl Pts',(-44.3705972700495,-55.2524997368729,
-38.6302900391873));
#244089=CARTESIAN_POINT('Ctrl Pts',(-44.446056048267,-55.2474029004138,
-38.6430428201589));
#244090=CARTESIAN_POINT('Ctrl Pts',(-44.5218128020516,-55.2441636366351,
-38.65617756452));
#244091=CARTESIAN_POINT('Ctrl Pts',(-44.5599089424743,-55.2434808562086,
-38.6629497802385));
#244092=CARTESIAN_POINT('Ctrl Pts',(-44.6354869543582,-55.2439911084578,
-38.6767130108817));
#244093=CARTESIAN_POINT('Ctrl Pts',(-44.6731456892459,-55.2451740103824,
-38.6837342374529));
#244094=CARTESIAN_POINT('Ctrl Pts',(-44.7481014788608,-55.2493620066237,
-38.6980304684339));
#244095=CARTESIAN_POINT('Ctrl Pts',(-44.860046548974,-55.2583760573225,
-38.7198650218829));
#244096=CARTESIAN_POINT('Ctrl Pts',(-45.0073845433675,-55.2811507310277,
-38.7505067688753));
#244097=CARTESIAN_POINT('Ctrl Pts',(-45.1528189888476,-55.3146135839333,
-38.7826550300594));
#244098=CARTESIAN_POINT('Ctrl Pts',(-45.2248832056965,-55.3349380951144,
-38.7992310848652));
#244099=CARTESIAN_POINT('Ctrl Pts',(-45.2966462681613,-55.3570913336823,
-38.8160672125853));
#244100=CARTESIAN_POINT('Ctrl Pts',(-45.3323638946335,-55.3690863290504,
-38.8246135819642));
#244101=CARTESIAN_POINT('Ctrl Pts',(-45.4027951436545,-55.3946744461232,
-38.841798196801));
#244102=CARTESIAN_POINT('Ctrl Pts',(-45.4376370321487,-55.4083060218429,
-38.85046633842));
#244103=CARTESIAN_POINT('Ctrl Pts',(-45.5409345111852,-55.4516493275196,
-38.8766665754573));
#244104=CARTESIAN_POINT('Ctrl Pts',(-45.6082182891413,-55.4838201174091,
-38.8944064774514));
#244105=CARTESIAN_POINT('Ctrl Pts',(-45.7067749877369,-55.5369855856676,
-38.9214216121435));
#244106=CARTESIAN_POINT('Ctrl Pts',(-45.7392219877795,-55.5555212114618,
-38.9304915704334));
#244107=CARTESIAN_POINT('Ctrl Pts',(-45.8033556832395,-55.5942722159849,
-38.9487787872477));
#244108=CARTESIAN_POINT('Ctrl Pts',(-45.8348443691401,-55.6143675312756,
-38.9579395118015));
#244109=CARTESIAN_POINT('Ctrl Pts',(-45.9274099842789,-55.6766589025306,
-38.9854159162723));
#244110=CARTESIAN_POINT('Ctrl Pts',(-45.9867610865919,-55.7209353156014,
-39.0037703637879));
#244111=CARTESIAN_POINT('Ctrl Pts',(-46.1007337830098,-55.8148102393793,
-39.0405190865864));
#244112=CARTESIAN_POINT('Ctrl Pts',(-46.1826971388658,-55.889219933262,
-39.0681181728269));
#244113=CARTESIAN_POINT('Ctrl Pts',(-46.259356574729,-55.9696687352924,
-39.0957737179551));
#244114=CARTESIAN_POINT('Ctrl Pts',(-46.309266807939,-56.024663053365,-39.1142236413887));
#244115=CARTESIAN_POINT('Ctrl Pts',(-46.3336138177017,-56.0528284109483,
-39.1234510495426));
#244116=CARTESIAN_POINT('Ctrl Pts',(-46.3692509284248,-56.0961546965833,
-39.1373141736981));
#244117=CARTESIAN_POINT('Ctrl Pts',(-46.3809719555493,-56.1107655250657,
-39.14193505412));
#244118=CARTESIAN_POINT('Ctrl Pts',(-46.4039850968433,-56.1401806715041,
-39.1511314768264));
#244119=CARTESIAN_POINT('Ctrl Pts',(-46.4153001903629,-56.1550126624776,
-39.1557159133813));
#244120=CARTESIAN_POINT('Ctrl Pts',(-46.4486370096885,-56.1998310060263,
-39.1694131182659));
#244121=CARTESIAN_POINT('Ctrl Pts',(-46.4700835091466,-56.2301795317326,
-39.1784826054425));
#244122=CARTESIAN_POINT('Ctrl Pts',(-46.532071913686,-56.3225583984772,
-39.2054898733524));
#244123=CARTESIAN_POINT('Ctrl Pts',(-46.5894197348374,-56.4176636744323,
-39.23211607576));
#244124=CARTESIAN_POINT('Ctrl Pts',(-46.6566074362748,-56.5498680842415,
-39.2668544229849));
#244125=CARTESIAN_POINT('Ctrl Pts',(-46.6870820302515,-56.617790568625,
-39.2839693714534));
#244126=CARTESIAN_POINT('Ctrl Pts',(-46.7159729830272,-56.6866360545619,
-39.3009558869148));
#244127=CARTESIAN_POINT('Ctrl Pts',(-46.7296188023799,-56.7214992889704,
-39.3093799218186));
#244128=CARTESIAN_POINT('Ctrl Pts',(-46.7553216997643,-56.7922546384013,
-39.3261176641085));
#244129=CARTESIAN_POINT('Ctrl Pts',(-46.7672996943011,-56.8279354881579,
-39.3343809787628));
#244130=CARTESIAN_POINT('Ctrl Pts',(-46.8004530502947,-56.9353633959568,
-39.358737163018));
#244131=CARTESIAN_POINT('Ctrl Pts',(-46.8189795501832,-57.0077635587999,
-39.3744658121213));
#244132=CARTESIAN_POINT('Ctrl Pts',(-46.848916211803,-57.1540080946302,
-39.4048998290393));
#244133=CARTESIAN_POINT('Ctrl Pts',(-46.866048617508,-57.2647966217996,
-39.4269646939479));
#244134=CARTESIAN_POINT('Ctrl Pts',(-46.875074749658,-57.3772756893033,
-39.4478819384746));
#244135=CARTESIAN_POINT('Ctrl Pts',(-46.8792542953452,-57.4526370309597,
-39.4615663943076));
#244136=CARTESIAN_POINT('Ctrl Pts',(-46.8804258736835,-57.4905390832845,
-39.4682843608713));
#244137=CARTESIAN_POINT('Ctrl Pts',(-46.8808837743635,-57.566610437341,
-39.4814341960201));
#244138=CARTESIAN_POINT('Ctrl Pts',(-46.8801708637706,-57.604491394965,
-39.4878166677226));
#244139=CARTESIAN_POINT('Ctrl Pts',(-46.8768913879562,-57.6800597985945,
-39.5002231148134));
#244140=CARTESIAN_POINT('Ctrl Pts',(-46.8691896925243,-57.7930657109158,
-39.5182849936093));
#244141=CARTESIAN_POINT('Ctrl Pts',(-46.8479069711518,-57.9423669591112,
-39.540205996752));
#244142=CARTESIAN_POINT('Ctrl Pts',(-46.8236459543104,-58.053306681129,
-39.5550278422771));
#244143=CARTESIAN_POINT('Ctrl Pts',(-46.8055990109883,-58.1270324939452,
-39.5645447403379));
#244144=CARTESIAN_POINT('Ctrl Pts',(-46.7956339676918,-58.1637938532181,
-39.5691227921436));
#244145=CARTESIAN_POINT('Ctrl Pts',(-46.7738161327052,-58.2370162077019,
-39.5779016468881));
#244146=CARTESIAN_POINT('Ctrl Pts',(-46.7619036278491,-58.2736352268715,
-39.5821192203466));
#244147=CARTESIAN_POINT('Ctrl Pts',(-46.7364059718256,-58.3458255995332,
-39.5900871854462));
#244148=CARTESIAN_POINT('Ctrl Pts',(-46.7091836493705,-58.4171862986019,
-39.5976163356366));
#244149=CARTESIAN_POINT('Ctrl Pts',(-46.663274408039,-58.5216699086648,
-39.6076014242402));
#244150=CARTESIAN_POINT('Ctrl Pts',(-46.6123207377325,-58.6236436013082,
-39.616293729045));
#244151=CARTESIAN_POINT('Ctrl Pts',(-46.5563244858032,-58.7230996041114,
-39.6236943138341));
#244152=CARTESIAN_POINT('Ctrl Pts',(-46.515607032986,-58.7877140896312,
-39.6277619492082));
#244153=CARTESIAN_POINT('Ctrl Pts',(-46.4731710833873,-58.8514710047945,
-39.6313905635194));
#244154=CARTESIAN_POINT('Ctrl Pts',(-46.4511086137465,-58.8829006319494,
-39.6329844599904));
#244155=CARTESIAN_POINT('Ctrl Pts',(-46.4051673201274,-58.9449633016888,
-39.6357273485653));
#244156=CARTESIAN_POINT('Ctrl Pts',(-46.381447994276,-58.975377588932,-39.6368662598532));
#244157=CARTESIAN_POINT('Ctrl Pts',(-46.3084068909562,-59.0643493136614,
-39.6395761233691));
#244158=CARTESIAN_POINT('Ctrl Pts',(-46.2570407846102,-59.1209150453974,
-39.6404603784325));
#244159=CARTESIAN_POINT('Ctrl Pts',(-46.1491379755941,-59.228544463199,
-39.6404138814247));
#244160=CARTESIAN_POINT('Ctrl Pts',(-46.0925836555155,-59.2796343044913,
-39.6394845811684));
#244161=CARTESIAN_POINT('Ctrl Pts',(-46.0038529437629,-59.3521266125547,
-39.6367223387528));
#244162=CARTESIAN_POINT('Ctrl Pts',(-45.9736068078661,-59.3756113554055,
-39.6355721163029));
#244163=CARTESIAN_POINT('Ctrl Pts',(-45.9272656961273,-59.4097723546528,
-39.6334997725088));
#244164=CARTESIAN_POINT('Ctrl Pts',(-45.9116419215573,-59.4209912820171,
-39.6327502808957));
#244165=CARTESIAN_POINT('Ctrl Pts',(-45.8800804794677,-59.4430610802669,
-39.6311351339295));
#244166=CARTESIAN_POINT('Ctrl Pts',(-45.8321587971618,-59.4756823489919,
-39.628531354857));
#244167=CARTESIAN_POINT('Ctrl Pts',(-45.7834097108732,-59.5062438963941,
-39.6254355071979));
#244168=CARTESIAN_POINT('Ctrl Pts',(-45.717633106262,-59.5452481912826,
-39.6208773262667));
#244169=CARTESIAN_POINT('Ctrl Pts',(-45.6178307490054,-59.601113548897,
-39.6133952897297));
#244170=CARTESIAN_POINT('Ctrl Pts',(-45.4802897643185,-59.6652183443042,
-39.6008811885904));
#244171=CARTESIAN_POINT('Ctrl Pts',(-45.3738098009101,-59.7055766782111,
-39.5896017905935));
#244172=CARTESIAN_POINT('Ctrl Pts',(-45.3020778813705,-59.7307512119865,
-39.5816566825671));
#244173=CARTESIAN_POINT('Ctrl Pts',(-45.2658207311094,-59.7424779859237,
-39.5774690651077));
#244174=CARTESIAN_POINT('Ctrl Pts',(-45.1926264675053,-59.7641596016776,
-39.5686715125846));
#244175=CARTESIAN_POINT('Ctrl Pts',(-45.1555073907618,-59.7741562512684,
-39.5640376159893));
#244176=CARTESIAN_POINT('Ctrl Pts',(-45.0441315765335,-59.8011904590316,
-39.5496210468413));
#244177=CARTESIAN_POINT('Ctrl Pts',(-44.9324484012679,-59.8224577850013,
-39.5341534065747));
#244178=CARTESIAN_POINT('Ctrl Pts',(-44.8203079610257,-59.8353953605365,
-39.5171556909205));
#244179=CARTESIAN_POINT('Ctrl Pts',(-44.7080184564226,-59.8455760612675,
-39.4996502778008));
#244180=CARTESIAN_POINT('Ctrl Pts',(-44.6329372249224,-59.8486931621852,
-39.4873001861445));
#244181=CARTESIAN_POINT('Ctrl Pts',(-44.5200834441659,-59.8478515133141,
-39.4677634802869));
#244182=CARTESIAN_POINT('Ctrl Pts',(-44.4823810871712,-59.8466449718289,
-39.4610736497974));
#244183=CARTESIAN_POINT('Ctrl Pts',(-44.4258051079382,-59.8434394706745,
-39.4507883432074));
#244184=CARTESIAN_POINT('Ctrl Pts',(-44.4069254589855,-59.8421361346926,
-39.4473147915973));
#244185=CARTESIAN_POINT('Ctrl Pts',(-44.3691376542581,-59.8390581625153,
-39.4402793331445));
#244186=CARTESIAN_POINT('Ctrl Pts',(-44.3502459350849,-59.8372838734483,
-39.4367203104461));
#244187=CARTESIAN_POINT('Ctrl Pts',(-44.2562487381671,-59.8272835659938,
-39.4188041728073));
#244188=CARTESIAN_POINT('Ctrl Pts',(-44.1080045765469,-59.8040393501646,
-39.3892226636159));
#244189=CARTESIAN_POINT('Ctrl Pts',(-43.9639303529155,-59.7668593120831,
-39.3578670379715));
#244190=CARTESIAN_POINT('Ctrl Pts',(-43.8219159040518,-59.7227861654643,
-39.3256251231267));
#244191=CARTESIAN_POINT('Ctrl Pts',(-43.7519290534068,-59.6972943066161,
-39.3090578287531));
#244192=CARTESIAN_POINT('Ctrl Pts',(-43.665783177736,-59.6610675807531,
-39.2877890488175));
#244193=CARTESIAN_POINT('Ctrl Pts',(-43.6486106666635,-59.653596197985,
-39.2835041280971));
#244194=CARTESIAN_POINT('Ctrl Pts',(-43.6144193015916,-59.6382222359849,
-39.2748825183767));
#244195=CARTESIAN_POINT('Ctrl Pts',(-43.597366582891,-59.6303022352814,
-39.2705368924251));
#244196=CARTESIAN_POINT('Ctrl Pts',(-43.5465994182959,-59.605961903298,
-39.2574616452183));
#244197=CARTESIAN_POINT('Ctrl Pts',(-43.513329300663,-59.588993111175,-39.2487085268073));
#244198=CARTESIAN_POINT('Ctrl Pts',(-43.4805771074156,-59.5712767529309,
-39.2399080357013));
#244199=CARTESIAN_POINT('Ctrl Pts',(-43.8341420587998,-57.9817357678076,
-41.1268248734572));
#244200=CARTESIAN_POINT('Ctrl Pts',(-43.8090823387197,-57.9680163597508,
-41.1092238912453));
#244201=CARTESIAN_POINT('Ctrl Pts',(-43.7605654269547,-57.9383371077444,
-41.0736746770147));
#244202=CARTESIAN_POINT('Ctrl Pts',(-43.6924895655639,-57.8872515755908,
-41.019320019256));
#244203=CARTESIAN_POINT('Ctrl Pts',(-43.6502497090231,-57.8487916199066,
-40.9823828883729));
#244204=CARTESIAN_POINT('Ctrl Pts',(-43.6096433745973,-57.8080652293815,
-40.945090157748));
#244205=CARTESIAN_POINT('Ctrl Pts',(-43.5713160673933,-57.7657212262301,
-40.9080353139296));
#244206=CARTESIAN_POINT('Ctrl Pts',(-43.5288984657655,-57.7088609123343,
-40.8622751058818));
#244207=CARTESIAN_POINT('Ctrl Pts',(-43.4982484100127,-57.6610280687967,
-40.826006689079));
#244208=CARTESIAN_POINT('Ctrl Pts',(-43.4769169762936,-57.6239677344727,
-40.798976453902));
#244209=CARTESIAN_POINT('Ctrl Pts',(-43.4638199758968,-57.5984660781933,
-40.7810781735695));
#244210=CARTESIAN_POINT('Ctrl Pts',(-43.4512904535732,-57.5725430453748,
-40.7632325534464));
#244211=CARTESIAN_POINT('Ctrl Pts',(-43.4453582046716,-57.5594707895743,
-40.7544050886758));
#244212=CARTESIAN_POINT('Ctrl Pts',(-43.4285595200757,-57.5199648485381,
-40.7282304644163));
#244213=CARTESIAN_POINT('Ctrl Pts',(-43.4088016745783,-57.4664867157472,
-40.6941268792613));
#244214=CARTESIAN_POINT('Ctrl Pts',(-43.3942530508608,-57.4114223976644,
-40.6616070010832));
#244215=CARTESIAN_POINT('Ctrl Pts',(-43.3853242538269,-57.3695231591805,
-40.6378273627645));
#244216=CARTESIAN_POINT('Ctrl Pts',(-43.3826786150667,-57.3554536366825,
-40.630001230023));
#244217=CARTESIAN_POINT('Ctrl Pts',(-43.378062215599,-57.3271160344971,
-40.6145607014775));
#244218=CARTESIAN_POINT('Ctrl Pts',(-43.3760891270041,-57.3128275119467,
-40.60693561976));
#244219=CARTESIAN_POINT('Ctrl Pts',(-43.3728422231051,-57.2841093232557,
-40.5919365051523));
#244220=CARTESIAN_POINT('Ctrl Pts',(-43.3715781643254,-57.2697777029377,
-40.5846130830795));
#244221=CARTESIAN_POINT('Ctrl Pts',(-43.3697526802575,-57.2411194243864,
-40.5702888754578));
#244222=CARTESIAN_POINT('Ctrl Pts',(-43.3680717796799,-57.1981642741791,
-40.5492997469169));
#244223=CARTESIAN_POINT('Ctrl Pts',(-43.3700185838812,-57.1410182421193,
-40.5232909177883));
#244224=CARTESIAN_POINT('Ctrl Pts',(-43.3746384661022,-57.0982543712987,
-40.505286899195));
#244225=CARTESIAN_POINT('Ctrl Pts',(-43.3784319419536,-57.0697666559562,
-40.4936247912381));
#244226=CARTESIAN_POINT('Ctrl Pts',(-43.3806866868643,-57.0555278483981,
-40.4879619013523));
#244227=CARTESIAN_POINT('Ctrl Pts',(-43.3859186984709,-57.0270949764048,
-40.476993052777));
#244228=CARTESIAN_POINT('Ctrl Pts',(-43.3889115442249,-57.0128413374093,
-40.4716662621118));
#244229=CARTESIAN_POINT('Ctrl Pts',(-43.3955695423488,-56.984668670318,
-40.4614841416371));
#244230=CARTESIAN_POINT('Ctrl Pts',(-43.4029115329907,-56.9567427536229,
-40.4517375031029));
#244231=CARTESIAN_POINT('Ctrl Pts',(-43.4159439893498,-56.915628788467,
-40.4384286813559));
#244232=CARTESIAN_POINT('Ctrl Pts',(-43.4309850942545,-56.8752725380991,
-40.4264211055283));
#244233=CARTESIAN_POINT('Ctrl Pts',(-43.4480370013178,-56.8356780486645,
-40.4157207514563));
#244234=CARTESIAN_POINT('Ctrl Pts',(-43.4607570961379,-56.8097932355363,
-40.409467745062));
#244235=CARTESIAN_POINT('Ctrl Pts',(-43.4741642201056,-56.7841683331057,
-40.4036630043601));
#244236=CARTESIAN_POINT('Ctrl Pts',(-43.4812071336048,-56.7714928975767,
-40.4009861443346));
#244237=CARTESIAN_POINT('Ctrl Pts',(-43.4960130774609,-56.7463797512019,
-40.3960865778375));
#244238=CARTESIAN_POINT('Ctrl Pts',(-43.5037198572985,-56.7340380787953,
-40.3938827877695));
#244239=CARTESIAN_POINT('Ctrl Pts',(-43.527657505214,-56.6977883833479,
-40.3880276966888));
#244240=CARTESIAN_POINT('Ctrl Pts',(-43.5447483375558,-56.6745564757614,
-40.3851058766842));
#244241=CARTESIAN_POINT('Ctrl Pts',(-43.5811328114983,-56.629979998045,
-40.3812078888591));
#244242=CARTESIAN_POINT('Ctrl Pts',(-43.6004351631962,-56.6086219171049,
-40.3802294367552));
#244243=CARTESIAN_POINT('Ctrl Pts',(-43.6310475296952,-56.578014570072,
-40.3802318237287));
#244244=CARTESIAN_POINT('Ctrl Pts',(-43.6415402048873,-56.5680413281089,
-40.3804790384992));
#244245=CARTESIAN_POINT('Ctrl Pts',(-43.6576911458811,-56.5534539772523,
-40.3812231446347));
#244246=CARTESIAN_POINT('Ctrl Pts',(-43.6631494628181,-56.5486488515781,
-40.3815339900979));
#244247=CARTESIAN_POINT('Ctrl Pts',(-43.6742063152013,-56.5391628964206,
-40.3822815284329));
#244248=CARTESIAN_POINT('Ctrl Pts',(-43.6798092119243,-56.534479009001,
-40.3827188413654));
#244249=CARTESIAN_POINT('Ctrl Pts',(-43.6967370434146,-56.5206915949946,
-40.3842131357726));
#244250=CARTESIAN_POINT('Ctrl Pts',(-43.7196778600618,-56.5029622466235,
-40.386692708542));
#244251=CARTESIAN_POINT('Ctrl Pts',(-43.7670264629127,-56.4700551612604,
-40.3935618621563));
#244252=CARTESIAN_POINT('Ctrl Pts',(-43.8165352419067,-56.4409186299576,
-40.4032471370382));
#244253=CARTESIAN_POINT('Ctrl Pts',(-43.8552784957563,-56.4218759376155,
-40.4126045758866));
#244254=CARTESIAN_POINT('Ctrl Pts',(-43.8814691350842,-56.4098116142502,
-40.4193119877837));
#244255=CARTESIAN_POINT('Ctrl Pts',(-43.8947490665381,-56.4040935548973,
-40.4229014011429));
#244256=CARTESIAN_POINT('Ctrl Pts',(-43.9216608718689,-56.3933018151258,
-40.430550144354));
#244257=CARTESIAN_POINT('Ctrl Pts',(-43.9353412421961,-56.3882139347518,
-40.434625723994));
#244258=CARTESIAN_POINT('Ctrl Pts',(-43.9627318697344,-56.3788058930362,
-40.4431514805252));
#244259=CARTESIAN_POINT('Ctrl Pts',(-43.9765011076412,-56.3744602994329,
-40.4476175822086));
#244260=CARTESIAN_POINT('Ctrl Pts',(-44.0179764085085,-56.3624961934912,
-40.4615970784657));
#244261=CARTESIAN_POINT('Ctrl Pts',(-44.0598195105868,-56.3526585058303,
-40.4767455237411));
#244262=CARTESIAN_POINT('Ctrl Pts',(-44.1163310625808,-56.3437038269143,
-40.4992178608308));
#244263=CARTESIAN_POINT('Ctrl Pts',(-44.1590753545772,-56.3390714325247,
-40.5172068769433));
#244264=CARTESIAN_POINT('Ctrl Pts',(-44.1878153726385,-56.337382052278,
-40.5299596579145));
#244265=CARTESIAN_POINT('Ctrl Pts',(-44.2166756293141,-56.3364007867548,
-40.5430944022758));
#244266=CARTESIAN_POINT('Ctrl Pts',(-44.2311921171808,-56.3362675100036,
-40.5498666179945));
#244267=CARTESIAN_POINT('Ctrl Pts',(-44.2599977007373,-56.3367129587916,
-40.5636298486377));
#244268=CARTESIAN_POINT('Ctrl Pts',(-44.2743541649932,-56.3372884158027,
-40.5706510752088));
#244269=CARTESIAN_POINT('Ctrl Pts',(-44.3029357424357,-56.3391317429585,
-40.5849473061899));
#244270=CARTESIAN_POINT('Ctrl Pts',(-44.3456316213443,-56.3429350642169,
-40.6067818596389));
#244271=CARTESIAN_POINT('Ctrl Pts',(-44.4018650235691,-56.3520939287388,
-40.6374236066311));
#244272=CARTESIAN_POINT('Ctrl Pts',(-44.4574103376146,-56.3653147883305,
-40.6695718678152));
#244273=CARTESIAN_POINT('Ctrl Pts',(-44.4849466005937,-56.3732907222196,
-40.686147922621));
#244274=CARTESIAN_POINT('Ctrl Pts',(-44.512374392093,-56.3819617528141,
-40.7029840503412));
#244275=CARTESIAN_POINT('Ctrl Pts',(-44.5260289861432,-56.3866462995878,
-40.7115304197201));
#244276=CARTESIAN_POINT('Ctrl Pts',(-44.5529609776699,-56.3966203919845,
-40.7287150345567));
#244277=CARTESIAN_POINT('Ctrl Pts',(-44.5662873943758,-56.4019250012471,
-40.737383176176));
#244278=CARTESIAN_POINT('Ctrl Pts',(-44.6058068395674,-56.4187668411382,
-40.7635834132132));
#244279=CARTESIAN_POINT('Ctrl Pts',(-44.6315615859976,-56.4312362585519,
-40.7813233152079));
#244280=CARTESIAN_POINT('Ctrl Pts',(-44.6693071486035,-56.4518014713652,
-40.8083384498991));
#244281=CARTESIAN_POINT('Ctrl Pts',(-44.6817372625133,-56.458965010373,
-40.8174084081892));
#244282=CARTESIAN_POINT('Ctrl Pts',(-44.7063132537473,-56.473929075182,
-40.8356956250034));
#244283=CARTESIAN_POINT('Ctrl Pts',(-44.7183832523531,-56.4816832398284,
-40.8448563495594));
#244284=CARTESIAN_POINT('Ctrl Pts',(-44.7538754102704,-56.505703003501,
-40.8723327540241));
#244285=CARTESIAN_POINT('Ctrl Pts',(-44.7766465418209,-56.5227549736834,
-40.8906872015444));
#244286=CARTESIAN_POINT('Ctrl Pts',(-44.8204030914552,-56.5588699415109,
-40.9274359243417));
#244287=CARTESIAN_POINT('Ctrl Pts',(-44.851893062885,-56.5874690797881,
-40.9550350105826));
#244288=CARTESIAN_POINT('Ctrl Pts',(-44.8813802932551,-56.6183507815631,
-40.982690555711));
#244289=CARTESIAN_POINT('Ctrl Pts',(-44.9005867815582,-56.6394533348067,
-41.0011404791447));
#244290=CARTESIAN_POINT('Ctrl Pts',(-44.9099603095753,-56.6502571213647,
-41.0103678872986));
#244291=CARTESIAN_POINT('Ctrl Pts',(-44.9236872082217,-56.6668706184025,
-41.0242310114538));
#244292=CARTESIAN_POINT('Ctrl Pts',(-44.9282031316495,-56.6724722064122,
-41.0288518918758));
#244293=CARTESIAN_POINT('Ctrl Pts',(-44.9370720489983,-56.6837477093971,
-41.038048314582));
#244294=CARTESIAN_POINT('Ctrl Pts',(-44.9414338933841,-56.6894322363092,
-41.0426327511372));
#244295=CARTESIAN_POINT('Ctrl Pts',(-44.9542884395491,-56.7066066663578,
-41.0563299560217));
#244296=CARTESIAN_POINT('Ctrl Pts',(-44.9625629539304,-56.7182326826763,
-41.0653994431984));
#244297=CARTESIAN_POINT('Ctrl Pts',(-44.9864941991718,-56.7536111473724,
-41.0924067111081));
#244298=CARTESIAN_POINT('Ctrl Pts',(-45.0086645271567,-56.7900134244028,
-41.1190329135161));
#244299=CARTESIAN_POINT('Ctrl Pts',(-45.034704630644,-56.8405768845403,
-41.1537712607408));
#244300=CARTESIAN_POINT('Ctrl Pts',(-45.0465408860903,-56.8665423758261,
-41.1708862092094));
#244301=CARTESIAN_POINT('Ctrl Pts',(-45.0577761134165,-56.8928546179869,
-41.1878727246706));
#244302=CARTESIAN_POINT('Ctrl Pts',(-45.0630901582258,-56.906176087846,
-41.1962967595746));
#244303=CARTESIAN_POINT('Ctrl Pts',(-45.0731156002939,-56.9332061371524,
-41.2130345018643));
#244304=CARTESIAN_POINT('Ctrl Pts',(-45.0777961712447,-56.9468340019015,
-41.2212978165198));
#244305=CARTESIAN_POINT('Ctrl Pts',(-45.0907786540592,-56.9878560258786,
-41.2456540007716));
#244306=CARTESIAN_POINT('Ctrl Pts',(-45.0980724298404,-57.0154910056487,
-41.2613826498774));
#244307=CARTESIAN_POINT('Ctrl Pts',(-45.1099506000897,-57.0712899900431,
-41.2918166667949));
#244308=CARTESIAN_POINT('Ctrl Pts',(-45.1168338059478,-57.11354441615,-41.3138815317038));
#244309=CARTESIAN_POINT('Ctrl Pts',(-45.1206309792415,-57.1564190282566,
-41.3347987762303));
#244310=CARTESIAN_POINT('Ctrl Pts',(-45.1224627479043,-57.1851396939165,
-41.3484832320635));
#244311=CARTESIAN_POINT('Ctrl Pts',(-45.1230291819396,-57.199581674993,
-41.3552011986272));
#244312=CARTESIAN_POINT('Ctrl Pts',(-45.1234439819388,-57.2285619504273,
-41.3683510337761));
#244313=CARTESIAN_POINT('Ctrl Pts',(-45.1232917301137,-57.2429904040975,
-41.3747335054784));
#244314=CARTESIAN_POINT('Ctrl Pts',(-45.122279779691,-57.2717682086368,
-41.3871399525693));
#244315=CARTESIAN_POINT('Ctrl Pts',(-45.1196997436484,-57.3147947598186,
-41.4052018313649));
#244316=CARTESIAN_POINT('Ctrl Pts',(-45.1120557453653,-57.3716084168758,
-41.4271228345082));
#244317=CARTESIAN_POINT('Ctrl Pts',(-45.1031553338884,-57.4137999065974,
-41.4419446800329));
#244318=CARTESIAN_POINT('Ctrl Pts',(-45.09650693546,-57.4418330021969,-41.4514615780937));
#244319=CARTESIAN_POINT('Ctrl Pts',(-45.092823442876,-57.4558081403435,
-41.4560396298995));
#244320=CARTESIAN_POINT('Ctrl Pts',(-45.08473584999,-57.4836385233421,-41.464818484644));
#244321=CARTESIAN_POINT('Ctrl Pts',(-45.0803094818206,-57.4975537933777,
-41.4690360581021));
#244322=CARTESIAN_POINT('Ctrl Pts',(-45.0708158371377,-57.5249803724867,
-41.4770040232021));
#244323=CARTESIAN_POINT('Ctrl Pts',(-45.060662137239,-57.5520858826269,
-41.4845331733926));
#244324=CARTESIAN_POINT('Ctrl Pts',(-45.0434887903859,-57.591755117417,
-41.4945182619959));
#244325=CARTESIAN_POINT('Ctrl Pts',(-45.0243848727922,-57.6304534586566,
-41.5032105668009));
#244326=CARTESIAN_POINT('Ctrl Pts',(-45.0033512023575,-57.6681778817651,
-41.51061115159));
#244327=CARTESIAN_POINT('Ctrl Pts',(-44.9880328234845,-57.692673879575,
-41.5146787869643));
#244328=CARTESIAN_POINT('Ctrl Pts',(-44.9720568870916,-57.7168380825906,
-41.5183074012753));
#244329=CARTESIAN_POINT('Ctrl Pts',(-44.9637457009402,-57.7287466936453,
-41.5199012977462));
#244330=CARTESIAN_POINT('Ctrl Pts',(-44.9464287138105,-57.7522550306847,
-41.5226441863212));
#244331=CARTESIAN_POINT('Ctrl Pts',(-44.9374830238235,-57.7637718882179,
-41.5237830976086));
#244332=CARTESIAN_POINT('Ctrl Pts',(-44.9099214446927,-57.7974515399035,
-41.5264929611258));
#244333=CARTESIAN_POINT('Ctrl Pts',(-44.8905204729439,-57.8188493934961,
-41.5273772161885));
#244334=CARTESIAN_POINT('Ctrl Pts',(-44.8497318000032,-57.8595330722204,
-41.5273307191807));
#244335=CARTESIAN_POINT('Ctrl Pts',(-44.8283374647208,-57.878828810327,
-41.5264014189239));
#244336=CARTESIAN_POINT('Ctrl Pts',(-44.7947479986672,-57.9061820008563,
-41.5236391765087));
#244337=CARTESIAN_POINT('Ctrl Pts',(-44.7832945060713,-57.9150388128137,
-41.5224889540588));
#244338=CARTESIAN_POINT('Ctrl Pts',(-44.7657408175914,-57.9279147771907,
-41.5204166102647));
#244339=CARTESIAN_POINT('Ctrl Pts',(-44.7598217545323,-57.9321421746299,
-41.5196671186517));
#244340=CARTESIAN_POINT('Ctrl Pts',(-44.7478629508254,-57.9404557426351,
-41.5180519716851));
#244341=CARTESIAN_POINT('Ctrl Pts',(-44.7297025277655,-57.9527400844071,
-41.5154481926132));
#244342=CARTESIAN_POINT('Ctrl Pts',(-44.711220794734,-57.9642369190977,
-41.5123523449538));
#244343=CARTESIAN_POINT('Ctrl Pts',(-44.6862770262529,-57.9788987855805,
-41.5077941640223));
#244344=CARTESIAN_POINT('Ctrl Pts',(-44.6484202704456,-57.9998814948776,
-41.5003121274858));
#244345=CARTESIAN_POINT('Ctrl Pts',(-44.5962108390282,-58.0238874022289,
-41.4877980263462));
#244346=CARTESIAN_POINT('Ctrl Pts',(-44.5557649369164,-58.0389385823793,
-41.4765186283493));
#244347=CARTESIAN_POINT('Ctrl Pts',(-44.5285120653069,-58.048310487242,
-41.4685735203231));
#244348=CARTESIAN_POINT('Ctrl Pts',(-44.5147341086114,-58.0526671867402,
-41.4643859028639));
#244349=CARTESIAN_POINT('Ctrl Pts',(-44.4869140318333,-58.0607029371288,
-41.4555883503401));
#244350=CARTESIAN_POINT('Ctrl Pts',(-44.4728027150897,-58.0643973546439,
-41.4509544537452));
#244351=CARTESIAN_POINT('Ctrl Pts',(-44.4304531283686,-58.0743536715507,
-41.4365378845966));
#244352=CARTESIAN_POINT('Ctrl Pts',(-44.3879697631396,-58.0821103913619,
-41.4210702443308));
#244353=CARTESIAN_POINT('Ctrl Pts',(-44.3452880889881,-58.0866896268435,
-41.4040725286766));
#244354=CARTESIAN_POINT('Ctrl Pts',(-44.3025416355467,-58.090217180745,
-41.3865671155567));
#244355=CARTESIAN_POINT('Ctrl Pts',(-44.2739489581488,-58.0911687787978,
-41.3742170239002));
#244356=CARTESIAN_POINT('Ctrl Pts',(-44.2309555122234,-58.090491506171,
-41.3546803180427));
#244357=CARTESIAN_POINT('Ctrl Pts',(-44.2165895018292,-58.0899123697243,
-41.347990487553));
#244358=CARTESIAN_POINT('Ctrl Pts',(-44.1950278537333,-58.0885113544661,
-41.337705180963));
#244359=CARTESIAN_POINT('Ctrl Pts',(-44.1878319550126,-58.0879547296283,
-41.3342316293533));
#244360=CARTESIAN_POINT('Ctrl Pts',(-44.1734279164018,-58.0866616594573,
-41.3271961709002));
#244361=CARTESIAN_POINT('Ctrl Pts',(-44.1662260389348,-58.0859253983809,
-41.3236371482021));
#244362=CARTESIAN_POINT('Ctrl Pts',(-44.130389101081,-58.0818150523559,
-41.3057210105631));
#244363=CARTESIAN_POINT('Ctrl Pts',(-44.073848260417,-58.0724828543971,
-41.2761395013722));
#244364=CARTESIAN_POINT('Ctrl Pts',(-44.0188545174212,-58.0578491440998,
-41.2447838757269));
#244365=CARTESIAN_POINT('Ctrl Pts',(-43.9646246641704,-58.0405931079736,
-41.2125419608827));
#244366=CARTESIAN_POINT('Ctrl Pts',(-43.9378880325505,-58.0306505669816,
-41.1959746665064));
#244367=CARTESIAN_POINT('Ctrl Pts',(-43.9049634769563,-58.0165631445999,
-41.174705886574));
#244368=CARTESIAN_POINT('Ctrl Pts',(-43.898399460067,-58.0136596367661,
-41.1704209658528));
#244369=CARTESIAN_POINT('Ctrl Pts',(-43.8853286348063,-58.0076886655405,
-41.1617993561325));
#244370=CARTESIAN_POINT('Ctrl Pts',(-43.8788088737381,-58.0046144513738,
-41.157453730181));
#244371=CARTESIAN_POINT('Ctrl Pts',(-43.8593967360427,-57.9951717320096,
-41.1443784829743));
#244372=CARTESIAN_POINT('Ctrl Pts',(-43.8466719188398,-57.9885954718361,
-41.1356253645631));
#244373=CARTESIAN_POINT('Ctrl Pts',(-43.8341420587998,-57.9817357678076,
-41.1268248734572));
#244374=CARTESIAN_POINT('',(-43.4124018854943,-55.8022015878058,-38.9060745433569));
#244375=CARTESIAN_POINT('',(-42.5465470395476,-57.084443392074,-38.9933901058265));
#244376=CARTESIAN_POINT('Ctrl Pts',(-43.412401749244,-55.8022014449206,
-38.9060739147518));
#244377=CARTESIAN_POINT('Ctrl Pts',(-43.4091603539247,-55.8043237908914,
-38.905838575256));
#244378=CARTESIAN_POINT('Ctrl Pts',(-43.405924519186,-55.8064559313723,
-38.9056064596797));
#244379=CARTESIAN_POINT('Ctrl Pts',(-43.4026942423849,-55.8085978727799,
-38.9053775693585));
#244380=CARTESIAN_POINT('Ctrl Pts',(-43.37514439206,-55.8268657082684,-38.9034254474569));
#244381=CARTESIAN_POINT('Ctrl Pts',(-43.3479995130707,-55.8458475490097,
-38.9017082880385));
#244382=CARTESIAN_POINT('Ctrl Pts',(-43.3212654553579,-55.8655537371234,
-38.9002297378292));
#244383=CARTESIAN_POINT('Ctrl Pts',(-43.2945313976451,-55.8852599252372,
-38.89875118762));
#244384=CARTESIAN_POINT('Ctrl Pts',(-43.2682103054482,-55.9056892935197,
-38.8975114527738));
#244385=CARTESIAN_POINT('Ctrl Pts',(-43.2423046180206,-55.9268610072553,
-38.8965152565023));
#244386=CARTESIAN_POINT('Ctrl Pts',(-43.2293517743068,-55.9374468641231,
-38.8960171583666));
#244387=CARTESIAN_POINT('Ctrl Pts',(-43.2164877853448,-55.9482328356115,
-38.8955798454342));
#244388=CARTESIAN_POINT('Ctrl Pts',(-43.2037924561014,-55.9591521490568,
-38.8952060762666));
#244389=CARTESIAN_POINT('Ctrl Pts',(-43.191097126858,-55.9700714625021,
-38.894832307099));
#244390=CARTESIAN_POINT('Ctrl Pts',(-43.1785604553322,-55.9811311728431,
-38.8945214616358));
#244391=CARTESIAN_POINT('Ctrl Pts',(-43.1661929384724,-55.9923201879255,
-38.8942734262572));
#244392=CARTESIAN_POINT('Ctrl Pts',(-43.1414579047527,-56.0146982180903,
-38.8937773555001));
#244393=CARTESIAN_POINT('Ctrl Pts',(-43.117344267243,-56.0376373429099,
-38.8935301407298));
#244394=CARTESIAN_POINT('Ctrl Pts',(-43.0938842149535,-56.0610936119007,
-38.893529345072));
#244395=CARTESIAN_POINT('Ctrl Pts',(-43.0469641103745,-56.1080061498824,
-38.8935277537564));
#244396=CARTESIAN_POINT('Ctrl Pts',(-43.0025474813891,-56.1570710705973,
-38.8945062058602));
#244397=CARTESIAN_POINT('Ctrl Pts',(-42.9606448514092,-56.2082353818757,
-38.8964551997726));
#244398=CARTESIAN_POINT('Ctrl Pts',(-42.9187422214293,-56.2593996931541,
-38.8984041936851));
#244399=CARTESIAN_POINT('Ctrl Pts',(-42.8793334746424,-56.3126943660298,
-38.9013260136914));
#244400=CARTESIAN_POINT('Ctrl Pts',(-42.8424899550942,-56.3680976795844,
-38.9052294077438));
#244401=CARTESIAN_POINT('Ctrl Pts',(-42.8240681953201,-56.3957993363617,
-38.9071811047699));
#244402=CARTESIAN_POINT('Ctrl Pts',(-42.8062629627728,-56.4240849025666,
-38.9093848948387));
#244403=CARTESIAN_POINT('Ctrl Pts',(-42.7891466755666,-56.452854472693,
-38.9118346780871));
#244404=CARTESIAN_POINT('Ctrl Pts',(-42.7720303883604,-56.4816240428195,
-38.9142844613354));
#244405=CARTESIAN_POINT('Ctrl Pts',(-42.7557331147215,-56.5106575807864,
-38.9169613213614));
#244406=CARTESIAN_POINT('Ctrl Pts',(-42.7402073536177,-56.5399968434848,
-38.9198636917123));
#244407=CARTESIAN_POINT('Ctrl Pts',(-42.7246815925139,-56.5693361061833,
-38.9227660620632));
#244408=CARTESIAN_POINT('Ctrl Pts',(-42.7099369818181,-56.5989648901808,
-38.9258925623446));
#244409=CARTESIAN_POINT('Ctrl Pts',(-42.6959610908403,-56.6288786279515,
-38.9292392096901));
#244410=CARTESIAN_POINT('Ctrl Pts',(-42.6819851998625,-56.6587923657221,
-38.9325858570355));
#244411=CARTESIAN_POINT('Ctrl Pts',(-42.6687780682593,-56.6889910719312,
-38.9361526631523));
#244412=CARTESIAN_POINT('Ctrl Pts',(-42.6563331490266,-56.719472363895,
-38.9399372898988));
#244413=CARTESIAN_POINT('Ctrl Pts',(-42.643888229794,-56.7499536558588,
-38.9437219166453));
#244414=CARTESIAN_POINT('Ctrl Pts',(-42.6322055381297,-56.7807175391602,
-38.9477243688907));
#244415=CARTESIAN_POINT('Ctrl Pts',(-42.6212841673493,-56.8117637261138,
-38.9519438796553));
#244416=CARTESIAN_POINT('Ctrl Pts',(-42.6103627965688,-56.8428099130675,
-38.9561633904199));
#244417=CARTESIAN_POINT('Ctrl Pts',(-42.6002027387397,-56.8741384006643,
-38.9605999581383));
#244418=CARTESIAN_POINT('Ctrl Pts',(-42.5908086952621,-56.9057509847877,
-38.9652543723165));
#244419=CARTESIAN_POINT('Ctrl Pts',(-42.5814146517845,-56.9373635689111,
-38.9699087864947));
#244420=CARTESIAN_POINT('Ctrl Pts',(-42.5727856698931,-56.9692679586228,
-38.9747824586382));
#244421=CARTESIAN_POINT('Ctrl Pts',(-42.5649349981973,-57.0014449365778,
-38.9798735188755));
#244422=CARTESIAN_POINT('Ctrl Pts',(-42.5582279477202,-57.0289346372945,
-38.9842229553717));
#244423=CARTESIAN_POINT('Ctrl Pts',(-42.5520784846546,-57.0566978718422,
-38.9887444451878));
#244424=CARTESIAN_POINT('Ctrl Pts',(-42.5465468336536,-57.0844434303275,
-38.9933892883181));
#244425=CARTESIAN_POINT('Ctrl Pts',(-43.4124020554461,-55.8022017898837,
-38.9060751583925));
#244426=CARTESIAN_POINT('Ctrl Pts',(-43.3061848450385,-55.8790363393388,
-38.9101809968017));
#244427=CARTESIAN_POINT('Ctrl Pts',(-43.2069727235914,-55.9648033290264,
-38.9151474711616));
#244428=CARTESIAN_POINT('Ctrl Pts',(-43.031358609741,-56.1455355255316,
-38.9261117869001));
#244429=CARTESIAN_POINT('Ctrl Pts',(-42.9541369537678,-56.2389770816702,
-38.9319838163158));
#244430=CARTESIAN_POINT('Ctrl Pts',(-42.8824499129319,-56.3415276713087,
-38.9385899207548));
#244431=CARTESIAN_POINT('Ctrl Pts',(-42.880249864589,-56.3446921073219,
-38.9387939270245));
#244432=CARTESIAN_POINT('Ctrl Pts',(-42.8735245664188,-56.3544183519727,
-38.93942145924));
#244433=CARTESIAN_POINT('Ctrl Pts',(-42.8690260301994,-56.3609982673211,
-38.9398466822262));
#244434=CARTESIAN_POINT('Ctrl Pts',(-42.7971306143081,-56.4673582778772,
-38.9467316408428));
#244435=CARTESIAN_POINT('Ctrl Pts',(-42.7376562988331,-56.5724855808993,
-38.9536292675083));
#244436=CARTESIAN_POINT('Ctrl Pts',(-42.6273438404767,-56.8117291221827,
-38.971053016757));
#244437=CARTESIAN_POINT('Ctrl Pts',(-42.5803525009342,-56.9465451572024,
-38.9817005915576));
#244438=CARTESIAN_POINT('Ctrl Pts',(-42.5465476043924,-57.084443479682,
-38.9933907057792));
#244439=CARTESIAN_POINT('Ctrl Pts',(-44.5079524583208,-59.1441977614012,
-52.99995));
#244440=CARTESIAN_POINT('Ctrl Pts',(-43.5445019199415,-59.1441977614012,
-52.9416166666667));
#244441=CARTESIAN_POINT('Ctrl Pts',(-43.0627766507519,-58.309825119875,
-52.8832833333334));
#244442=CARTESIAN_POINT('Ctrl Pts',(-42.5810513815623,-57.4754524783487,
-52.82495));
#244443=CARTESIAN_POINT('Ctrl Pts',(-43.0627766507519,-56.6410798368225,
-52.7666166666667));
#244444=CARTESIAN_POINT('Ctrl Pts',(-43.5445019199415,-55.8067071952963,
-52.7082833333333));
#244445=CARTESIAN_POINT('Ctrl Pts',(-44.5079524583208,-55.8067071952963,
-52.64995));
#244446=CARTESIAN_POINT('Ctrl Pts',(-45.4714029967,-55.8067071952963,-52.5916166666666));
#244447=CARTESIAN_POINT('Ctrl Pts',(-45.9531282658897,-56.6410798368225,
-52.5332833333334));
#244448=CARTESIAN_POINT('Ctrl Pts',(-46.4348535350793,-57.4754524783487,
-52.4749500000001));
#244449=CARTESIAN_POINT('Ctrl Pts',(-45.9531282658897,-58.309825119875,
-52.4166166666667));
#244450=CARTESIAN_POINT('Ctrl Pts',(-45.4714029967,-59.1441977614012,-52.3582833333334));
#244451=CARTESIAN_POINT('Ctrl Pts',(-44.5079524583208,-59.1441977614012,
-52.29995));
#244452=CARTESIAN_POINT('Ctrl Pts',(-43.5445019199415,-59.1441977614012,
-52.2416166666667));
#244453=CARTESIAN_POINT('Ctrl Pts',(-43.0627766507519,-58.309825119875,
-52.1832833333333));
#244454=CARTESIAN_POINT('Ctrl Pts',(-42.5810513815623,-57.4754524783487,
-52.12495));
#244455=CARTESIAN_POINT('Ctrl Pts',(-43.0627766507519,-56.6410798368225,
-52.0666166666667));
#244456=CARTESIAN_POINT('Ctrl Pts',(-43.5445019199415,-55.8067071952963,
-52.0082833333333));
#244457=CARTESIAN_POINT('Ctrl Pts',(-44.5079524583208,-55.8067071952963,
-51.94995));
#244458=CARTESIAN_POINT('Ctrl Pts',(-45.4714029967,-55.8067071952963,-51.8916166666667));
#244459=CARTESIAN_POINT('Ctrl Pts',(-45.9531282658897,-56.6410798368225,
-51.8332833333334));
#244460=CARTESIAN_POINT('Ctrl Pts',(-46.4348535350793,-57.4754524783487,
-51.77495));
#244461=CARTESIAN_POINT('Ctrl Pts',(-45.9531282658897,-58.309825119875,
-51.7166166666667));
#244462=CARTESIAN_POINT('Ctrl Pts',(-45.4714029967,-59.1441977614012,-51.6582833333333));
#244463=CARTESIAN_POINT('Ctrl Pts',(-44.5079524583208,-59.1441977614012,
-51.59995));
#244464=CARTESIAN_POINT('Ctrl Pts',(-43.5445019199415,-59.1441977614012,
-51.5416166666667));
#244465=CARTESIAN_POINT('Ctrl Pts',(-43.0627766507519,-58.309825119875,
-51.4832833333334));
#244466=CARTESIAN_POINT('Ctrl Pts',(-42.5810513815623,-57.4754524783487,
-51.42495));
#244467=CARTESIAN_POINT('Ctrl Pts',(-43.0627766507519,-56.6410798368225,
-51.3666166666667));
#244468=CARTESIAN_POINT('Ctrl Pts',(-43.5445019199415,-55.8067071952963,
-51.3082833333333));
#244469=CARTESIAN_POINT('Ctrl Pts',(-44.5079524583208,-55.8067071952963,
-51.24995));
#244470=CARTESIAN_POINT('Ctrl Pts',(-45.4714029967,-55.8067071952963,-51.1916166666667));
#244471=CARTESIAN_POINT('Ctrl Pts',(-45.9531282658897,-56.6410798368225,
-51.1332833333334));
#244472=CARTESIAN_POINT('Ctrl Pts',(-46.4348535350793,-57.4754524783487,
-51.07495));
#244473=CARTESIAN_POINT('Ctrl Pts',(-45.9531282658897,-58.309825119875,
-51.0166166666667));
#244474=CARTESIAN_POINT('Ctrl Pts',(-45.4714029967,-59.1441977614012,-50.9582833333334));
#244475=CARTESIAN_POINT('Ctrl Pts',(-44.5079524583208,-59.1441977614012,
-50.89995));
#244476=CARTESIAN_POINT('Ctrl Pts',(-43.5445019199415,-59.1441977614012,
-50.8416166666667));
#244477=CARTESIAN_POINT('Ctrl Pts',(-43.0627766507519,-58.309825119875,
-50.7832833333333));
#244478=CARTESIAN_POINT('Ctrl Pts',(-42.5810513815623,-57.4754524783487,
-50.72495));
#244479=CARTESIAN_POINT('Ctrl Pts',(-43.0627766507519,-56.6410798368225,
-50.6666166666667));
#244480=CARTESIAN_POINT('Ctrl Pts',(-43.5445019199415,-55.8067071952963,
-50.6082833333334));
#244481=CARTESIAN_POINT('Ctrl Pts',(-44.5079524583208,-55.8067071952963,
-50.54995));
#244482=CARTESIAN_POINT('Ctrl Pts',(-45.4714029967,-55.8067071952963,-50.4916166666667));
#244483=CARTESIAN_POINT('Ctrl Pts',(-45.9531282658897,-56.6410798368225,
-50.4332833333333));
#244484=CARTESIAN_POINT('Ctrl Pts',(-46.4348535350793,-57.4754524783487,
-50.37495));
#244485=CARTESIAN_POINT('Ctrl Pts',(-45.9531282658897,-58.309825119875,
-50.3166166666667));
#244486=CARTESIAN_POINT('Ctrl Pts',(-45.4714029967,-59.1441977614012,-50.2582833333334));
#244487=CARTESIAN_POINT('Ctrl Pts',(-44.5079524583208,-59.1441977614012,
-50.19995));
#244488=CARTESIAN_POINT('Ctrl Pts',(-43.5445019199415,-59.1441977614012,
-50.1416166666667));
#244489=CARTESIAN_POINT('Ctrl Pts',(-43.0627766507519,-58.309825119875,
-50.0832833333334));
#244490=CARTESIAN_POINT('Ctrl Pts',(-42.5810513815623,-57.4754524783487,
-50.02495));
#244491=CARTESIAN_POINT('Ctrl Pts',(-43.0627766507519,-56.6410798368225,
-49.9666166666667));
#244492=CARTESIAN_POINT('Ctrl Pts',(-43.5445019199415,-55.8067071952963,
-49.9082833333334));
#244493=CARTESIAN_POINT('Ctrl Pts',(-44.5079524583208,-55.8067071952963,
-49.84995));
#244494=CARTESIAN_POINT('Ctrl Pts',(-45.4714029967,-55.8067071952963,-49.7916166666667));
#244495=CARTESIAN_POINT('Ctrl Pts',(-45.9531282658897,-56.6410798368225,
-49.7332833333334));
#244496=CARTESIAN_POINT('Ctrl Pts',(-46.4348535350793,-57.4754524783487,
-49.67495));
#244497=CARTESIAN_POINT('Ctrl Pts',(-45.9531282658897,-58.309825119875,
-49.6166166666667));
#244498=CARTESIAN_POINT('Ctrl Pts',(-45.4714029967,-59.1441977614012,-49.5582833333334));
#244499=CARTESIAN_POINT('Ctrl Pts',(-44.5079524583208,-59.1441977614012,
-49.49995));
#244500=CARTESIAN_POINT('Ctrl Pts',(-43.5445019199415,-59.1441977614012,
-49.4416166666667));
#244501=CARTESIAN_POINT('Ctrl Pts',(-43.0627766507519,-58.309825119875,
-49.3832833333334));
#244502=CARTESIAN_POINT('Ctrl Pts',(-42.5810513815623,-57.4754524783487,
-49.32495));
#244503=CARTESIAN_POINT('Ctrl Pts',(-43.0627766507519,-56.6410798368225,
-49.2666166666667));
#244504=CARTESIAN_POINT('Ctrl Pts',(-43.5445019199415,-55.8067071952963,
-49.2082833333334));
#244505=CARTESIAN_POINT('Ctrl Pts',(-44.5079524583208,-55.8067071952963,
-49.14995));
#244506=CARTESIAN_POINT('Ctrl Pts',(-45.4714029967,-55.8067071952963,-49.0916166666667));
#244507=CARTESIAN_POINT('Ctrl Pts',(-45.9531282658897,-56.6410798368225,
-49.0332833333333));
#244508=CARTESIAN_POINT('Ctrl Pts',(-46.4348535350793,-57.4754524783487,
-48.97495));
#244509=CARTESIAN_POINT('Ctrl Pts',(-45.9531282658897,-58.309825119875,
-48.9166166666667));
#244510=CARTESIAN_POINT('Ctrl Pts',(-45.4714029967,-59.1441977614012,-48.8582833333333));
#244511=CARTESIAN_POINT('Ctrl Pts',(-44.5079524583208,-59.1441977614012,
-48.79995));
#244512=CARTESIAN_POINT('Ctrl Pts',(-43.5445019199415,-59.1441977614012,
-48.7416166666667));
#244513=CARTESIAN_POINT('Ctrl Pts',(-43.0627766507519,-58.309825119875,
-48.6832833333334));
#244514=CARTESIAN_POINT('Ctrl Pts',(-42.5810513815623,-57.4754524783487,
-48.62495));
#244515=CARTESIAN_POINT('Ctrl Pts',(-43.0627766507519,-56.6410798368225,
-48.5666166666667));
#244516=CARTESIAN_POINT('Ctrl Pts',(-43.5445019199415,-55.8067071952963,
-48.5082833333334));
#244517=CARTESIAN_POINT('Ctrl Pts',(-44.5079524583208,-55.8067071952963,
-48.44995));
#244518=CARTESIAN_POINT('Ctrl Pts',(-45.4714029967,-55.8067071952963,-48.3916166666667));
#244519=CARTESIAN_POINT('Ctrl Pts',(-45.9531282658897,-56.6410798368225,
-48.3332833333334));
#244520=CARTESIAN_POINT('Ctrl Pts',(-46.4348535350793,-57.4754524783487,
-48.27495));
#244521=CARTESIAN_POINT('Ctrl Pts',(-45.9531282658897,-58.309825119875,
-48.2166166666667));
#244522=CARTESIAN_POINT('Ctrl Pts',(-45.4714029967,-59.1441977614012,-48.1582833333334));
#244523=CARTESIAN_POINT('Ctrl Pts',(-44.5079524583208,-59.1441977614012,
-48.09995));
#244524=CARTESIAN_POINT('Ctrl Pts',(-43.5445019199415,-59.1441977614012,
-48.0416166666667));
#244525=CARTESIAN_POINT('Ctrl Pts',(-43.0627766507519,-58.309825119875,
-47.9832833333334));
#244526=CARTESIAN_POINT('Ctrl Pts',(-42.5810513815623,-57.4754524783487,
-47.92495));
#244527=CARTESIAN_POINT('Ctrl Pts',(-43.0627766507519,-56.6410798368225,
-47.8666166666667));
#244528=CARTESIAN_POINT('Ctrl Pts',(-43.5445019199415,-55.8067071952963,
-47.8082833333333));
#244529=CARTESIAN_POINT('Ctrl Pts',(-44.5079524583208,-55.8067071952963,
-47.74995));
#244530=CARTESIAN_POINT('Ctrl Pts',(-45.4714029967,-55.8067071952963,-47.6916166666667));
#244531=CARTESIAN_POINT('Ctrl Pts',(-45.9531282658897,-56.6410798368225,
-47.6332833333333));
#244532=CARTESIAN_POINT('Ctrl Pts',(-46.4348535350793,-57.4754524783487,
-47.57495));
#244533=CARTESIAN_POINT('Ctrl Pts',(-45.9531282658897,-58.309825119875,
-47.5166166666667));
#244534=CARTESIAN_POINT('Ctrl Pts',(-45.4714029967,-59.1441977614012,-47.4582833333333));
#244535=CARTESIAN_POINT('Ctrl Pts',(-44.5079524583208,-59.1441977614012,
-47.39995));
#244536=CARTESIAN_POINT('Ctrl Pts',(-43.5445019199415,-59.1441977614012,
-47.3416166666666));
#244537=CARTESIAN_POINT('Ctrl Pts',(-43.0627766507519,-58.309825119875,
-47.2832833333333));
#244538=CARTESIAN_POINT('Ctrl Pts',(-42.5810513815623,-57.4754524783487,
-47.22495));
#244539=CARTESIAN_POINT('Ctrl Pts',(-43.0627766507519,-56.6410798368225,
-47.1666166666667));
#244540=CARTESIAN_POINT('Ctrl Pts',(-43.5445019199415,-55.8067071952963,
-47.1082833333333));
#244541=CARTESIAN_POINT('Ctrl Pts',(-44.5079524583208,-55.8067071952963,
-47.04995));
#244542=CARTESIAN_POINT('Ctrl Pts',(-45.4714029967,-55.8067071952963,-46.9916166666667));
#244543=CARTESIAN_POINT('Ctrl Pts',(-45.9531282658897,-56.6410798368225,
-46.9332833333334));
#244544=CARTESIAN_POINT('Ctrl Pts',(-46.4348535350793,-57.4754524783487,
-46.87495));
#244545=CARTESIAN_POINT('Ctrl Pts',(-45.9531282658897,-58.309825119875,
-46.8166166666667));
#244546=CARTESIAN_POINT('Ctrl Pts',(-45.4714029967,-59.1441977614012,-46.7582833333333));
#244547=CARTESIAN_POINT('Ctrl Pts',(-44.5079524583208,-59.1441977614012,
-46.69995));
#244548=CARTESIAN_POINT('Ctrl Pts',(-43.5445019199415,-59.1441977614012,
-46.6416166666666));
#244549=CARTESIAN_POINT('Ctrl Pts',(-43.0627766507519,-58.309825119875,
-46.5832833333334));
#244550=CARTESIAN_POINT('Ctrl Pts',(-42.5810513815623,-57.4754524783487,
-46.52495));
#244551=CARTESIAN_POINT('Ctrl Pts',(-43.0627766507519,-56.6410798368225,
-46.4666166666667));
#244552=CARTESIAN_POINT('Ctrl Pts',(-43.5445019199415,-55.8067071952963,
-46.4082833333333));
#244553=CARTESIAN_POINT('Ctrl Pts',(-44.5079524583208,-55.8067071952963,
-46.34995));
#244554=CARTESIAN_POINT('Ctrl Pts',(-45.4714029967,-55.8067071952963,-46.2916166666667));
#244555=CARTESIAN_POINT('Ctrl Pts',(-45.9531282658897,-56.6410798368225,
-46.2332833333334));
#244556=CARTESIAN_POINT('Ctrl Pts',(-46.4348535350793,-57.4754524783487,
-46.17495));
#244557=CARTESIAN_POINT('Ctrl Pts',(-45.9531282658897,-58.309825119875,
-46.1166166666667));
#244558=CARTESIAN_POINT('Ctrl Pts',(-45.4714029967,-59.1441977614012,-46.0582833333333));
#244559=CARTESIAN_POINT('Ctrl Pts',(-44.5079524583208,-59.1441977614012,
-45.99995));
#244560=CARTESIAN_POINT('Ctrl Pts',(-43.5445019199415,-59.1441977614012,
-45.9416166666667));
#244561=CARTESIAN_POINT('Ctrl Pts',(-43.0627766507519,-58.309825119875,
-45.8832833333333));
#244562=CARTESIAN_POINT('Ctrl Pts',(-42.5810513815623,-57.4754524783487,
-45.82495));
#244563=CARTESIAN_POINT('Ctrl Pts',(-43.0627766507519,-56.6410798368225,
-45.7666166666667));
#244564=CARTESIAN_POINT('Ctrl Pts',(-43.5445019199415,-55.8067071952963,
-45.7082833333333));
#244565=CARTESIAN_POINT('Ctrl Pts',(-44.5079524583208,-55.8067071952963,
-45.64995));
#244566=CARTESIAN_POINT('Ctrl Pts',(-45.4714029967,-55.8067071952963,-45.5916166666667));
#244567=CARTESIAN_POINT('Ctrl Pts',(-45.9531282658897,-56.6410798368225,
-45.5332833333333));
#244568=CARTESIAN_POINT('Ctrl Pts',(-46.4348535350793,-57.4754524783487,
-45.47495));
#244569=CARTESIAN_POINT('Ctrl Pts',(-45.9531282658897,-58.309825119875,
-45.4166166666667));
#244570=CARTESIAN_POINT('Ctrl Pts',(-45.4714029967,-59.1441977614012,-45.3582833333333));
#244571=CARTESIAN_POINT('Ctrl Pts',(-44.5079524583208,-59.1441977614012,
-45.29995));
#244572=CARTESIAN_POINT('Ctrl Pts',(-43.5445019199415,-59.1441977614012,
-45.2416166666667));
#244573=CARTESIAN_POINT('Ctrl Pts',(-43.0627766507519,-58.309825119875,
-45.1832833333334));
#244574=CARTESIAN_POINT('Ctrl Pts',(-42.5810513815623,-57.4754524783487,
-45.12495));
#244575=CARTESIAN_POINT('Ctrl Pts',(-43.0627766507519,-56.6410798368225,
-45.0666166666667));
#244576=CARTESIAN_POINT('Ctrl Pts',(-43.5445019199415,-55.8067071952963,
-45.0082833333334));
#244577=CARTESIAN_POINT('Ctrl Pts',(-44.5079524583208,-55.8067071952963,
-44.94995));
#244578=CARTESIAN_POINT('Ctrl Pts',(-45.4714029967,-55.8067071952963,-44.8916166666667));
#244579=CARTESIAN_POINT('Ctrl Pts',(-45.9531282658897,-56.6410798368225,
-44.8332833333334));
#244580=CARTESIAN_POINT('Ctrl Pts',(-46.4348535350793,-57.4754524783487,
-44.77495));
#244581=CARTESIAN_POINT('Ctrl Pts',(-45.9531282658897,-58.309825119875,
-44.7166166666667));
#244582=CARTESIAN_POINT('Ctrl Pts',(-45.4714029967,-59.1441977614012,-44.6582833333334));
#244583=CARTESIAN_POINT('Ctrl Pts',(-44.5079524583208,-59.1441977614012,
-44.59995));
#244584=CARTESIAN_POINT('Ctrl Pts',(-43.5445019199415,-59.1441977614012,
-44.5416166666667));
#244585=CARTESIAN_POINT('Ctrl Pts',(-43.0627766507519,-58.309825119875,
-44.4832833333334));
#244586=CARTESIAN_POINT('Ctrl Pts',(-42.5810513815623,-57.4754524783487,
-44.42495));
#244587=CARTESIAN_POINT('Ctrl Pts',(-43.0627766507519,-56.6410798368225,
-44.3666166666667));
#244588=CARTESIAN_POINT('Ctrl Pts',(-43.5445019199415,-55.8067071952963,
-44.3082833333334));
#244589=CARTESIAN_POINT('Ctrl Pts',(-44.5079524583208,-55.8067071952963,
-44.24995));
#244590=CARTESIAN_POINT('Ctrl Pts',(-45.4714029967,-55.8067071952963,-44.1916166666667));
#244591=CARTESIAN_POINT('Ctrl Pts',(-45.9531282658897,-56.6410798368225,
-44.1332833333334));
#244592=CARTESIAN_POINT('Ctrl Pts',(-46.4348535350793,-57.4754524783487,
-44.07495));
#244593=CARTESIAN_POINT('Ctrl Pts',(-45.9531282658897,-58.309825119875,
-44.0166166666667));
#244594=CARTESIAN_POINT('Ctrl Pts',(-45.4714029967,-59.1441977614012,-43.9582833333334));
#244595=CARTESIAN_POINT('Ctrl Pts',(-44.5079524583208,-59.1441977614012,
-43.89995));
#244596=CARTESIAN_POINT('Ctrl Pts',(-43.5445019199415,-59.1441977614012,
-43.8416166666667));
#244597=CARTESIAN_POINT('Ctrl Pts',(-43.0627766507519,-58.309825119875,
-43.7832833333334));
#244598=CARTESIAN_POINT('Ctrl Pts',(-42.5810513815623,-57.4754524783487,
-43.72495));
#244599=CARTESIAN_POINT('Ctrl Pts',(-43.0627766507519,-56.6410798368225,
-43.6666166666667));
#244600=CARTESIAN_POINT('Ctrl Pts',(-43.5445019199415,-55.8067071952963,
-43.6082833333333));
#244601=CARTESIAN_POINT('Ctrl Pts',(-44.5079524583208,-55.8067071952963,
-43.54995));
#244602=CARTESIAN_POINT('Ctrl Pts',(-45.4714029967,-55.8067071952963,-43.4916166666667));
#244603=CARTESIAN_POINT('Ctrl Pts',(-45.9531282658897,-56.6410798368225,
-43.4332833333333));
#244604=CARTESIAN_POINT('Ctrl Pts',(-46.4348535350793,-57.4754524783487,
-43.37495));
#244605=CARTESIAN_POINT('Ctrl Pts',(-45.9531282658897,-58.309825119875,
-43.3166166666667));
#244606=CARTESIAN_POINT('Ctrl Pts',(-45.4714029967,-59.1441977614012,-43.2582833333333));
#244607=CARTESIAN_POINT('Ctrl Pts',(-44.5079524583208,-59.1441977614012,
-43.19995));
#244608=CARTESIAN_POINT('Ctrl Pts',(-43.5445019199415,-59.1441977614012,
-43.1416166666667));
#244609=CARTESIAN_POINT('Ctrl Pts',(-43.0627766507519,-58.309825119875,
-43.0832833333333));
#244610=CARTESIAN_POINT('Ctrl Pts',(-42.5810513815623,-57.4754524783487,
-43.02495));
#244611=CARTESIAN_POINT('Ctrl Pts',(-43.0627766507519,-56.6410798368225,
-42.9666166666667));
#244612=CARTESIAN_POINT('Ctrl Pts',(-43.5445019199415,-55.8067071952963,
-42.9082833333333));
#244613=CARTESIAN_POINT('Ctrl Pts',(-44.5079524583208,-55.8067071952963,
-42.84995));
#244614=CARTESIAN_POINT('Ctrl Pts',(-45.4714029967,-55.8067071952963,-42.7916166666667));
#244615=CARTESIAN_POINT('Ctrl Pts',(-45.9531282658897,-56.6410798368225,
-42.7332833333334));
#244616=CARTESIAN_POINT('Ctrl Pts',(-46.4348535350793,-57.4754524783487,
-42.67495));
#244617=CARTESIAN_POINT('Ctrl Pts',(-45.9531282658897,-58.309825119875,
-42.6166166666667));
#244618=CARTESIAN_POINT('Ctrl Pts',(-45.4714029967,-59.1441977614012,-42.5582833333333));
#244619=CARTESIAN_POINT('Ctrl Pts',(-44.5079524583208,-59.1441977614012,
-42.49995));
#244620=CARTESIAN_POINT('Ctrl Pts',(-43.5445019199415,-59.1441977614012,
-42.4416166666667));
#244621=CARTESIAN_POINT('Ctrl Pts',(-43.0627766507519,-58.309825119875,
-42.3832833333333));
#244622=CARTESIAN_POINT('Ctrl Pts',(-42.5810513815623,-57.4754524783487,
-42.32495));
#244623=CARTESIAN_POINT('Ctrl Pts',(-43.0627766507519,-56.6410798368225,
-42.2666166666667));
#244624=CARTESIAN_POINT('Ctrl Pts',(-43.5445019199415,-55.8067071952963,
-42.2082833333333));
#244625=CARTESIAN_POINT('Ctrl Pts',(-44.5079524583208,-55.8067071952963,
-42.14995));
#244626=CARTESIAN_POINT('Ctrl Pts',(-45.4714029967,-55.8067071952963,-42.0916166666667));
#244627=CARTESIAN_POINT('Ctrl Pts',(-45.9531282658897,-56.6410798368225,
-42.0332833333334));
#244628=CARTESIAN_POINT('Ctrl Pts',(-46.4348535350793,-57.4754524783487,
-41.97495));
#244629=CARTESIAN_POINT('Ctrl Pts',(-45.9531282658897,-58.309825119875,
-41.9166166666667));
#244630=CARTESIAN_POINT('Ctrl Pts',(-45.4714029967,-59.1441977614012,-41.8582833333333));
#244631=CARTESIAN_POINT('Ctrl Pts',(-44.5079524583208,-59.1441977614012,
-41.79995));
#244632=CARTESIAN_POINT('Ctrl Pts',(-43.5445019199415,-59.1441977614012,
-41.7416166666667));
#244633=CARTESIAN_POINT('Ctrl Pts',(-43.0627766507519,-58.309825119875,
-41.6832833333333));
#244634=CARTESIAN_POINT('Ctrl Pts',(-42.5810513815623,-57.4754524783487,
-41.62495));
#244635=CARTESIAN_POINT('Ctrl Pts',(-43.0627766507519,-56.6410798368225,
-41.5666166666667));
#244636=CARTESIAN_POINT('Ctrl Pts',(-43.5445019199415,-55.8067071952963,
-41.5082833333334));
#244637=CARTESIAN_POINT('Ctrl Pts',(-44.5079524583208,-55.8067071952963,
-41.44995));
#244638=CARTESIAN_POINT('Ctrl Pts',(-45.4714029967,-55.8067071952963,-41.3916166666667));
#244639=CARTESIAN_POINT('Ctrl Pts',(-45.9531282658897,-56.6410798368225,
-41.3332833333334));
#244640=CARTESIAN_POINT('Ctrl Pts',(-46.4348535350793,-57.4754524783487,
-41.27495));
#244641=CARTESIAN_POINT('Ctrl Pts',(-45.9531282658897,-58.309825119875,
-41.2166166666667));
#244642=CARTESIAN_POINT('Ctrl Pts',(-45.4714029967,-59.1441977614012,-41.1582833333333));
#244643=CARTESIAN_POINT('Ctrl Pts',(-44.5079524583208,-59.1441977614012,
-41.09995));
#244644=CARTESIAN_POINT('Ctrl Pts',(-43.5445019199415,-59.1441977614012,
-41.0416166666667));
#244645=CARTESIAN_POINT('Ctrl Pts',(-43.0627766507519,-58.309825119875,
-40.9832833333333));
#244646=CARTESIAN_POINT('Ctrl Pts',(-42.5810513815623,-57.4754524783487,
-40.92495));
#244647=CARTESIAN_POINT('Ctrl Pts',(-43.0627766507519,-56.6410798368225,
-40.8666166666667));
#244648=CARTESIAN_POINT('Ctrl Pts',(-43.5445019199415,-55.8067071952963,
-40.8082833333334));
#244649=CARTESIAN_POINT('Ctrl Pts',(-44.5079524583208,-55.8067071952963,
-40.74995));
#244650=CARTESIAN_POINT('Ctrl Pts',(-45.4714029967,-55.8067071952963,-40.6916166666667));
#244651=CARTESIAN_POINT('Ctrl Pts',(-45.9531282658897,-56.6410798368225,
-40.6332833333334));
#244652=CARTESIAN_POINT('Ctrl Pts',(-46.4348535350793,-57.4754524783487,
-40.57495));
#244653=CARTESIAN_POINT('Ctrl Pts',(-45.9531282658897,-58.309825119875,
-40.5166166666667));
#244654=CARTESIAN_POINT('Ctrl Pts',(-45.4714029967,-59.1441977614012,-40.4582833333333));
#244655=CARTESIAN_POINT('Ctrl Pts',(-44.5079524583208,-59.1441977614012,
-40.39995));
#244656=CARTESIAN_POINT('Ctrl Pts',(-43.5445019199415,-59.1441977614012,
-40.3416166666667));
#244657=CARTESIAN_POINT('Ctrl Pts',(-43.0627766507519,-58.309825119875,
-40.2832833333334));
#244658=CARTESIAN_POINT('Ctrl Pts',(-42.5810513815623,-57.4754524783487,
-40.22495));
#244659=CARTESIAN_POINT('Ctrl Pts',(-43.0627766507519,-56.6410798368225,
-40.1666166666667));
#244660=CARTESIAN_POINT('Ctrl Pts',(-43.5445019199415,-55.8067071952963,
-40.1082833333334));
#244661=CARTESIAN_POINT('Ctrl Pts',(-44.5079524583208,-55.8067071952963,
-40.04995));
#244662=CARTESIAN_POINT('Ctrl Pts',(-45.4714029967,-55.8067071952963,-39.9916166666667));
#244663=CARTESIAN_POINT('Ctrl Pts',(-45.9531282658897,-56.6410798368225,
-39.9332833333333));
#244664=CARTESIAN_POINT('Ctrl Pts',(-46.4348535350793,-57.4754524783487,
-39.87495));
#244665=CARTESIAN_POINT('Ctrl Pts',(-45.9531282658897,-58.309825119875,
-39.8166166666667));
#244666=CARTESIAN_POINT('Ctrl Pts',(-45.4714029967,-59.1441977614012,-39.7582833333334));
#244667=CARTESIAN_POINT('Ctrl Pts',(-44.5079524583208,-59.1441977614012,
-39.69995));
#244668=CARTESIAN_POINT('Ctrl Pts',(-43.5445019199415,-59.1441977614012,
-39.6416166666667));
#244669=CARTESIAN_POINT('Ctrl Pts',(-43.0627766507519,-58.309825119875,
-39.5832833333333));
#244670=CARTESIAN_POINT('Ctrl Pts',(-42.5810513815623,-57.4754524783487,
-39.52495));
#244671=CARTESIAN_POINT('Ctrl Pts',(-43.0627766507519,-56.6410798368225,
-39.4666166666667));
#244672=CARTESIAN_POINT('Ctrl Pts',(-43.5445019199415,-55.8067071952963,
-39.4082833333334));
#244673=CARTESIAN_POINT('Ctrl Pts',(-44.5079524583208,-55.8067071952963,
-39.34995));
#244674=CARTESIAN_POINT('Ctrl Pts',(-45.4714029967,-55.8067071952963,-39.2916166666667));
#244675=CARTESIAN_POINT('Ctrl Pts',(-45.9531282658897,-56.6410798368225,
-39.2332833333333));
#244676=CARTESIAN_POINT('Ctrl Pts',(-46.4348535350793,-57.4754524783487,
-39.17495));
#244677=CARTESIAN_POINT('Ctrl Pts',(-45.9531282658897,-58.309825119875,
-39.1166166666667));
#244678=CARTESIAN_POINT('Ctrl Pts',(-45.4714029967,-59.1441977614012,-39.0582833333334));
#244679=CARTESIAN_POINT('Ctrl Pts',(-44.5079524583208,-59.1441977614012,
-38.99995));
#244680=CARTESIAN_POINT('Ctrl Pts',(-43.5445019199415,-59.1441977614012,
-38.9416166666667));
#244681=CARTESIAN_POINT('Ctrl Pts',(-43.0627766507519,-58.309825119875,
-38.8832833333334));
#244682=CARTESIAN_POINT('Ctrl Pts',(-42.5810513815623,-57.4754524783487,
-38.82495));
#244683=CARTESIAN_POINT('Ctrl Pts',(-43.0627766507519,-56.6410798368225,
-38.7666166666667));
#244684=CARTESIAN_POINT('Ctrl Pts',(-43.5445019199415,-55.8067071952963,
-38.7082833333334));
#244685=CARTESIAN_POINT('Ctrl Pts',(-44.5079524583208,-55.8067071952963,
-38.64995));
#244686=CARTESIAN_POINT('Ctrl Pts',(-45.4714029967,-55.8067071952963,-38.5916166666667));
#244687=CARTESIAN_POINT('Ctrl Pts',(-45.9531282658897,-56.6410798368225,
-38.5332833333334));
#244688=CARTESIAN_POINT('Ctrl Pts',(-46.4348535350793,-57.4754524783487,
-38.47495));
#244689=CARTESIAN_POINT('Ctrl Pts',(-45.9531282658897,-58.309825119875,
-38.4166166666667));
#244690=CARTESIAN_POINT('Ctrl Pts',(-45.4714029967,-59.1441977614012,-38.3582833333333));
#244691=CARTESIAN_POINT('Ctrl Pts',(-44.5079524583208,-59.1441977614012,
-38.29995));
#244692=CARTESIAN_POINT('Ctrl Pts',(-43.5445019199415,-59.1441977614012,
-38.2416166666667));
#244693=CARTESIAN_POINT('Ctrl Pts',(-43.0627766507519,-58.309825119875,
-38.1832833333333));
#244694=CARTESIAN_POINT('Ctrl Pts',(-42.5810513815623,-57.4754524783487,
-38.12495));
#244695=CARTESIAN_POINT('Ctrl Pts',(-43.0627766507519,-56.6410798368225,
-38.0666166666667));
#244696=CARTESIAN_POINT('Ctrl Pts',(-43.5445019199415,-55.8067071952963,
-38.0082833333333));
#244697=CARTESIAN_POINT('Ctrl Pts',(-44.5079524583208,-55.8067071952963,
-37.94995));
#244698=CARTESIAN_POINT('Ctrl Pts',(-45.4714029967,-55.8067071952963,-37.8916166666667));
#244699=CARTESIAN_POINT('Ctrl Pts',(-45.9531282658897,-56.6410798368225,
-37.8332833333334));
#244700=CARTESIAN_POINT('Ctrl Pts',(-46.4348535350793,-57.4754524783487,
-37.77495));
#244701=CARTESIAN_POINT('Ctrl Pts',(-45.9531282658897,-58.309825119875,
-37.7166166666667));
#244702=CARTESIAN_POINT('Ctrl Pts',(-45.4714029967,-59.1441977614012,-37.6582833333333));
#244703=CARTESIAN_POINT('Ctrl Pts',(-44.5079524583208,-59.1441977614012,
-37.59995));
#244704=CARTESIAN_POINT('Ctrl Pts',(-43.5445019199415,-59.1441977614012,
-37.5416166666667));
#244705=CARTESIAN_POINT('Ctrl Pts',(-43.0627766507519,-58.309825119875,
-37.4832833333334));
#244706=CARTESIAN_POINT('Ctrl Pts',(-42.5810513815623,-57.4754524783487,
-37.42495));
#244707=CARTESIAN_POINT('Ctrl Pts',(-43.0627766507519,-56.6410798368225,
-37.3666166666667));
#244708=CARTESIAN_POINT('Ctrl Pts',(-43.5445019199415,-55.8067071952963,
-37.3082833333333));
#244709=CARTESIAN_POINT('Ctrl Pts',(-44.5079524583208,-55.8067071952963,
-37.24995));
#244710=CARTESIAN_POINT('Ctrl Pts',(-45.4714029967,-55.8067071952963,-37.1916166666667));
#244711=CARTESIAN_POINT('Ctrl Pts',(-45.9531282658897,-56.6410798368225,
-37.1332833333334));
#244712=CARTESIAN_POINT('Ctrl Pts',(-46.4348535350793,-57.4754524783487,
-37.07495));
#244713=CARTESIAN_POINT('Ctrl Pts',(-45.9531282658897,-58.309825119875,
-37.0166166666667));
#244714=CARTESIAN_POINT('Ctrl Pts',(-45.8905850977848,-58.418153064699,
-37.0090431559831));
#244715=CARTESIAN_POINT('Ctrl Pts',(-45.8125914103809,-58.5159466035015,
-37.0009024189827));
#244716=CARTESIAN_POINT('Ctrl Pts',(-44.5079524583208,-59.5441932447742,
-53.2308875));
#244717=CARTESIAN_POINT('Ctrl Pts',(-43.3135644199415,-59.5441932447742,
-53.1725541666667));
#244718=CARTESIAN_POINT('Ctrl Pts',(-42.7163704007519,-58.5098228615615,
-53.1142208333334));
#244719=CARTESIAN_POINT('Ctrl Pts',(-42.1191763815623,-57.4754524783487,
-53.0558875000001));
#244720=CARTESIAN_POINT('Ctrl Pts',(-42.7163704007519,-56.4410820951361,
-52.9975541666667));
#244721=CARTESIAN_POINT('Ctrl Pts',(-43.3135644199415,-55.4067117119233,
-52.9392208333334));
#244722=CARTESIAN_POINT('Ctrl Pts',(-44.5079524583208,-55.4067117119234,
-52.8808875));
#244723=CARTESIAN_POINT('Ctrl Pts',(-45.7023404967,-55.4067117119233,-52.8225541666667));
#244724=CARTESIAN_POINT('Ctrl Pts',(-46.2995345158897,-56.4410820951361,
-52.7642208333334));
#244725=CARTESIAN_POINT('Ctrl Pts',(-46.8967285350793,-57.4754524783487,
-52.7058875));
#244726=CARTESIAN_POINT('Ctrl Pts',(-46.2995345158897,-58.5098228615615,
-52.6475541666667));
#244727=CARTESIAN_POINT('Ctrl Pts',(-45.7023404967,-59.5441932447742,-52.5892208333333));
#244728=CARTESIAN_POINT('Ctrl Pts',(-44.5079524583208,-59.5441932447742,
-52.5308875));
#244729=CARTESIAN_POINT('Ctrl Pts',(-43.3135644199415,-59.5441932447742,
-52.4725541666667));
#244730=CARTESIAN_POINT('Ctrl Pts',(-42.7163704007519,-58.5098228615615,
-52.4142208333334));
#244731=CARTESIAN_POINT('Ctrl Pts',(-42.1191763815623,-57.4754524783487,
-52.3558875000001));
#244732=CARTESIAN_POINT('Ctrl Pts',(-42.7163704007519,-56.4410820951361,
-52.2975541666667));
#244733=CARTESIAN_POINT('Ctrl Pts',(-43.3135644199415,-55.4067117119233,
-52.2392208333334));
#244734=CARTESIAN_POINT('Ctrl Pts',(-44.5079524583208,-55.4067117119234,
-52.1808875));
#244735=CARTESIAN_POINT('Ctrl Pts',(-45.7023404967,-55.4067117119233,-52.1225541666667));
#244736=CARTESIAN_POINT('Ctrl Pts',(-46.2995345158897,-56.4410820951361,
-52.0642208333334));
#244737=CARTESIAN_POINT('Ctrl Pts',(-46.8967285350793,-57.4754524783487,
-52.0058875));
#244738=CARTESIAN_POINT('Ctrl Pts',(-46.2995345158897,-58.5098228615615,
-51.9475541666667));
#244739=CARTESIAN_POINT('Ctrl Pts',(-45.7023404967,-59.5441932447742,-51.8892208333334));
#244740=CARTESIAN_POINT('Ctrl Pts',(-44.5079524583208,-59.5441932447742,
-51.8308875));
#244741=CARTESIAN_POINT('Ctrl Pts',(-43.3135644199415,-59.5441932447742,
-51.7725541666667));
#244742=CARTESIAN_POINT('Ctrl Pts',(-42.7163704007519,-58.5098228615615,
-51.7142208333334));
#244743=CARTESIAN_POINT('Ctrl Pts',(-42.1191763815623,-57.4754524783487,
-51.6558875));
#244744=CARTESIAN_POINT('Ctrl Pts',(-42.7163704007519,-56.4410820951361,
-51.5975541666667));
#244745=CARTESIAN_POINT('Ctrl Pts',(-43.3135644199415,-55.4067117119233,
-51.5392208333333));
#244746=CARTESIAN_POINT('Ctrl Pts',(-44.5079524583208,-55.4067117119234,
-51.4808875));
#244747=CARTESIAN_POINT('Ctrl Pts',(-45.7023404967,-55.4067117119233,-51.4225541666667));
#244748=CARTESIAN_POINT('Ctrl Pts',(-46.2995345158897,-56.4410820951361,
-51.3642208333334));
#244749=CARTESIAN_POINT('Ctrl Pts',(-46.8967285350793,-57.4754524783487,
-51.3058875));
#244750=CARTESIAN_POINT('Ctrl Pts',(-46.2995345158897,-58.5098228615615,
-51.2475541666667));
#244751=CARTESIAN_POINT('Ctrl Pts',(-45.7023404967,-59.5441932447742,-51.1892208333334));
#244752=CARTESIAN_POINT('Ctrl Pts',(-44.5079524583208,-59.5441932447742,
-51.1308875));
#244753=CARTESIAN_POINT('Ctrl Pts',(-43.3135644199415,-59.5441932447742,
-51.0725541666667));
#244754=CARTESIAN_POINT('Ctrl Pts',(-42.7163704007519,-58.5098228615615,
-51.0142208333334));
#244755=CARTESIAN_POINT('Ctrl Pts',(-42.1191763815623,-57.4754524783487,
-50.9558875));
#244756=CARTESIAN_POINT('Ctrl Pts',(-42.7163704007519,-56.4410820951361,
-50.8975541666667));
#244757=CARTESIAN_POINT('Ctrl Pts',(-43.3135644199415,-55.4067117119233,
-50.8392208333333));
#244758=CARTESIAN_POINT('Ctrl Pts',(-44.5079524583208,-55.4067117119234,
-50.7808875));
#244759=CARTESIAN_POINT('Ctrl Pts',(-45.7023404967,-55.4067117119233,-50.7225541666667));
#244760=CARTESIAN_POINT('Ctrl Pts',(-46.2995345158897,-56.4410820951361,
-50.6642208333333));
#244761=CARTESIAN_POINT('Ctrl Pts',(-46.8967285350793,-57.4754524783487,
-50.6058875));
#244762=CARTESIAN_POINT('Ctrl Pts',(-46.2995345158897,-58.5098228615615,
-50.5475541666667));
#244763=CARTESIAN_POINT('Ctrl Pts',(-45.7023404967,-59.5441932447742,-50.4892208333333));
#244764=CARTESIAN_POINT('Ctrl Pts',(-44.5079524583208,-59.5441932447742,
-50.4308875));
#244765=CARTESIAN_POINT('Ctrl Pts',(-43.3135644199415,-59.5441932447742,
-50.3725541666667));
#244766=CARTESIAN_POINT('Ctrl Pts',(-42.7163704007519,-58.5098228615615,
-50.3142208333334));
#244767=CARTESIAN_POINT('Ctrl Pts',(-42.1191763815623,-57.4754524783487,
-50.2558875));
#244768=CARTESIAN_POINT('Ctrl Pts',(-42.7163704007519,-56.4410820951361,
-50.1975541666667));
#244769=CARTESIAN_POINT('Ctrl Pts',(-43.3135644199415,-55.4067117119233,
-50.1392208333333));
#244770=CARTESIAN_POINT('Ctrl Pts',(-44.5079524583208,-55.4067117119234,
-50.0808875));
#244771=CARTESIAN_POINT('Ctrl Pts',(-45.7023404967,-55.4067117119233,-50.0225541666667));
#244772=CARTESIAN_POINT('Ctrl Pts',(-46.2995345158897,-56.4410820951361,
-49.9642208333334));
#244773=CARTESIAN_POINT('Ctrl Pts',(-46.8967285350793,-57.4754524783487,
-49.9058875));
#244774=CARTESIAN_POINT('Ctrl Pts',(-46.2995345158897,-58.5098228615615,
-49.8475541666667));
#244775=CARTESIAN_POINT('Ctrl Pts',(-45.7023404967,-59.5441932447742,-49.7892208333333));
#244776=CARTESIAN_POINT('Ctrl Pts',(-44.5079524583208,-59.5441932447742,
-49.7308875));
#244777=CARTESIAN_POINT('Ctrl Pts',(-43.3135644199415,-59.5441932447742,
-49.6725541666667));
#244778=CARTESIAN_POINT('Ctrl Pts',(-42.7163704007519,-58.5098228615615,
-49.6142208333334));
#244779=CARTESIAN_POINT('Ctrl Pts',(-42.1191763815623,-57.4754524783487,
-49.5558875));
#244780=CARTESIAN_POINT('Ctrl Pts',(-42.7163704007519,-56.4410820951361,
-49.4975541666667));
#244781=CARTESIAN_POINT('Ctrl Pts',(-43.3135644199415,-55.4067117119233,
-49.4392208333333));
#244782=CARTESIAN_POINT('Ctrl Pts',(-44.5079524583208,-55.4067117119234,
-49.3808875));
#244783=CARTESIAN_POINT('Ctrl Pts',(-45.7023404967,-55.4067117119233,-49.3225541666667));
#244784=CARTESIAN_POINT('Ctrl Pts',(-46.2995345158897,-56.4410820951361,
-49.2642208333334));
#244785=CARTESIAN_POINT('Ctrl Pts',(-46.8967285350793,-57.4754524783487,
-49.2058875));
#244786=CARTESIAN_POINT('Ctrl Pts',(-46.2995345158897,-58.5098228615615,
-49.1475541666667));
#244787=CARTESIAN_POINT('Ctrl Pts',(-45.7023404967,-59.5441932447742,-49.0892208333333));
#244788=CARTESIAN_POINT('Ctrl Pts',(-44.5079524583208,-59.5441932447742,
-49.0308875));
#244789=CARTESIAN_POINT('Ctrl Pts',(-43.3135644199415,-59.5441932447742,
-48.9725541666667));
#244790=CARTESIAN_POINT('Ctrl Pts',(-42.7163704007519,-58.5098228615615,
-48.9142208333334));
#244791=CARTESIAN_POINT('Ctrl Pts',(-42.1191763815623,-57.4754524783487,
-48.8558875));
#244792=CARTESIAN_POINT('Ctrl Pts',(-42.7163704007519,-56.4410820951361,
-48.7975541666667));
#244793=CARTESIAN_POINT('Ctrl Pts',(-43.3135644199415,-55.4067117119233,
-48.7392208333334));
#244794=CARTESIAN_POINT('Ctrl Pts',(-44.5079524583208,-55.4067117119234,
-48.6808875));
#244795=CARTESIAN_POINT('Ctrl Pts',(-45.7023404967,-55.4067117119233,-48.6225541666667));
#244796=CARTESIAN_POINT('Ctrl Pts',(-46.2995345158897,-56.4410820951361,
-48.5642208333334));
#244797=CARTESIAN_POINT('Ctrl Pts',(-46.8967285350793,-57.4754524783487,
-48.5058875));
#244798=CARTESIAN_POINT('Ctrl Pts',(-46.2995345158897,-58.5098228615615,
-48.4475541666667));
#244799=CARTESIAN_POINT('Ctrl Pts',(-45.7023404967,-59.5441932447742,-48.3892208333334));
#244800=CARTESIAN_POINT('Ctrl Pts',(-44.5079524583208,-59.5441932447742,
-48.3308875));
#244801=CARTESIAN_POINT('Ctrl Pts',(-43.3135644199415,-59.5441932447742,
-48.2725541666667));
#244802=CARTESIAN_POINT('Ctrl Pts',(-42.7163704007519,-58.5098228615615,
-48.2142208333334));
#244803=CARTESIAN_POINT('Ctrl Pts',(-42.1191763815623,-57.4754524783487,
-48.1558875));
#244804=CARTESIAN_POINT('Ctrl Pts',(-42.7163704007519,-56.4410820951361,
-48.0975541666667));
#244805=CARTESIAN_POINT('Ctrl Pts',(-43.3135644199415,-55.4067117119233,
-48.0392208333334));
#244806=CARTESIAN_POINT('Ctrl Pts',(-44.5079524583208,-55.4067117119234,
-47.9808875));
#244807=CARTESIAN_POINT('Ctrl Pts',(-45.7023404967,-55.4067117119233,-47.9225541666667));
#244808=CARTESIAN_POINT('Ctrl Pts',(-46.2995345158897,-56.4410820951361,
-47.8642208333334));
#244809=CARTESIAN_POINT('Ctrl Pts',(-46.8967285350793,-57.4754524783487,
-47.8058875000001));
#244810=CARTESIAN_POINT('Ctrl Pts',(-46.2995345158897,-58.5098228615615,
-47.7475541666667));
#244811=CARTESIAN_POINT('Ctrl Pts',(-45.7023404967,-59.5441932447742,-47.6892208333334));
#244812=CARTESIAN_POINT('Ctrl Pts',(-44.5079524583208,-59.5441932447742,
-47.6308875));
#244813=CARTESIAN_POINT('Ctrl Pts',(-43.3135644199415,-59.5441932447742,
-47.5725541666667));
#244814=CARTESIAN_POINT('Ctrl Pts',(-42.7163704007519,-58.5098228615615,
-47.5142208333333));
#244815=CARTESIAN_POINT('Ctrl Pts',(-42.1191763815623,-57.4754524783487,
-47.4558875));
#244816=CARTESIAN_POINT('Ctrl Pts',(-42.7163704007519,-56.4410820951361,
-47.3975541666667));
#244817=CARTESIAN_POINT('Ctrl Pts',(-43.3135644199415,-55.4067117119233,
-47.3392208333334));
#244818=CARTESIAN_POINT('Ctrl Pts',(-44.5079524583208,-55.4067117119234,
-47.2808875));
#244819=CARTESIAN_POINT('Ctrl Pts',(-45.7023404967,-55.4067117119233,-47.2225541666667));
#244820=CARTESIAN_POINT('Ctrl Pts',(-46.2995345158897,-56.4410820951361,
-47.1642208333334));
#244821=CARTESIAN_POINT('Ctrl Pts',(-46.8967285350793,-57.4754524783487,
-47.1058875));
#244822=CARTESIAN_POINT('Ctrl Pts',(-46.2995345158897,-58.5098228615615,
-47.0475541666667));
#244823=CARTESIAN_POINT('Ctrl Pts',(-45.7023404967,-59.5441932447742,-46.9892208333334));
#244824=CARTESIAN_POINT('Ctrl Pts',(-44.5079524583208,-59.5441932447742,
-46.9308875));
#244825=CARTESIAN_POINT('Ctrl Pts',(-43.3135644199415,-59.5441932447742,
-46.8725541666667));
#244826=CARTESIAN_POINT('Ctrl Pts',(-42.7163704007519,-58.5098228615615,
-46.8142208333334));
#244827=CARTESIAN_POINT('Ctrl Pts',(-42.1191763815623,-57.4754524783487,
-46.7558875));
#244828=CARTESIAN_POINT('Ctrl Pts',(-42.7163704007519,-56.4410820951361,
-46.6975541666667));
#244829=CARTESIAN_POINT('Ctrl Pts',(-43.3135644199415,-55.4067117119233,
-46.6392208333334));
#244830=CARTESIAN_POINT('Ctrl Pts',(-44.5079524583208,-55.4067117119234,
-46.5808875));
#244831=CARTESIAN_POINT('Ctrl Pts',(-45.7023404967,-55.4067117119233,-46.5225541666667));
#244832=CARTESIAN_POINT('Ctrl Pts',(-46.2995345158897,-56.4410820951361,
-46.4642208333334));
#244833=CARTESIAN_POINT('Ctrl Pts',(-46.8967285350793,-57.4754524783487,
-46.4058875));
#244834=CARTESIAN_POINT('Ctrl Pts',(-46.2995345158897,-58.5098228615615,
-46.3475541666667));
#244835=CARTESIAN_POINT('Ctrl Pts',(-45.7023404967,-59.5441932447742,-46.2892208333334));
#244836=CARTESIAN_POINT('Ctrl Pts',(-44.5079524583208,-59.5441932447742,
-46.2308875));
#244837=CARTESIAN_POINT('Ctrl Pts',(-43.3135644199415,-59.5441932447742,
-46.1725541666667));
#244838=CARTESIAN_POINT('Ctrl Pts',(-42.7163704007519,-58.5098228615615,
-46.1142208333334));
#244839=CARTESIAN_POINT('Ctrl Pts',(-42.1191763815623,-57.4754524783487,
-46.0558875));
#244840=CARTESIAN_POINT('Ctrl Pts',(-42.7163704007519,-56.4410820951361,
-45.9975541666667));
#244841=CARTESIAN_POINT('Ctrl Pts',(-43.3135644199415,-55.4067117119233,
-45.9392208333333));
#244842=CARTESIAN_POINT('Ctrl Pts',(-44.5079524583208,-55.4067117119234,
-45.8808875));
#244843=CARTESIAN_POINT('Ctrl Pts',(-45.7023404967,-55.4067117119233,-45.8225541666667));
#244844=CARTESIAN_POINT('Ctrl Pts',(-46.2995345158897,-56.4410820951361,
-45.7642208333334));
#244845=CARTESIAN_POINT('Ctrl Pts',(-46.8967285350793,-57.4754524783487,
-45.7058875));
#244846=CARTESIAN_POINT('Ctrl Pts',(-46.2995345158897,-58.5098228615615,
-45.6475541666667));
#244847=CARTESIAN_POINT('Ctrl Pts',(-45.7023404967,-59.5441932447742,-45.5892208333334));
#244848=CARTESIAN_POINT('Ctrl Pts',(-44.5079524583208,-59.5441932447742,
-45.5308875));
#244849=CARTESIAN_POINT('Ctrl Pts',(-43.3135644199415,-59.5441932447742,
-45.4725541666667));
#244850=CARTESIAN_POINT('Ctrl Pts',(-42.7163704007519,-58.5098228615615,
-45.4142208333334));
#244851=CARTESIAN_POINT('Ctrl Pts',(-42.1191763815623,-57.4754524783487,
-45.3558875));
#244852=CARTESIAN_POINT('Ctrl Pts',(-42.7163704007519,-56.4410820951361,
-45.2975541666667));
#244853=CARTESIAN_POINT('Ctrl Pts',(-43.3135644199415,-55.4067117119233,
-45.2392208333333));
#244854=CARTESIAN_POINT('Ctrl Pts',(-44.5079524583208,-55.4067117119234,
-45.1808875));
#244855=CARTESIAN_POINT('Ctrl Pts',(-45.7023404967,-55.4067117119233,-45.1225541666667));
#244856=CARTESIAN_POINT('Ctrl Pts',(-46.2995345158897,-56.4410820951361,
-45.0642208333334));
#244857=CARTESIAN_POINT('Ctrl Pts',(-46.8967285350793,-57.4754524783487,
-45.0058875));
#244858=CARTESIAN_POINT('Ctrl Pts',(-46.2995345158897,-58.5098228615615,
-44.9475541666667));
#244859=CARTESIAN_POINT('Ctrl Pts',(-45.7023404967,-59.5441932447742,-44.8892208333333));
#244860=CARTESIAN_POINT('Ctrl Pts',(-44.5079524583208,-59.5441932447742,
-44.8308875));
#244861=CARTESIAN_POINT('Ctrl Pts',(-43.3135644199415,-59.5441932447742,
-44.7725541666667));
#244862=CARTESIAN_POINT('Ctrl Pts',(-42.7163704007519,-58.5098228615615,
-44.7142208333334));
#244863=CARTESIAN_POINT('Ctrl Pts',(-42.1191763815623,-57.4754524783487,
-44.6558875));
#244864=CARTESIAN_POINT('Ctrl Pts',(-42.7163704007519,-56.4410820951361,
-44.5975541666667));
#244865=CARTESIAN_POINT('Ctrl Pts',(-43.3135644199415,-55.4067117119233,
-44.5392208333333));
#244866=CARTESIAN_POINT('Ctrl Pts',(-44.5079524583208,-55.4067117119234,
-44.4808875000001));
#244867=CARTESIAN_POINT('Ctrl Pts',(-45.7023404967,-55.4067117119233,-44.4225541666667));
#244868=CARTESIAN_POINT('Ctrl Pts',(-46.2995345158897,-56.4410820951361,
-44.3642208333333));
#244869=CARTESIAN_POINT('Ctrl Pts',(-46.8967285350793,-57.4754524783487,
-44.3058875));
#244870=CARTESIAN_POINT('Ctrl Pts',(-46.2995345158897,-58.5098228615615,
-44.2475541666667));
#244871=CARTESIAN_POINT('Ctrl Pts',(-45.7023404967,-59.5441932447742,-44.1892208333334));
#244872=CARTESIAN_POINT('Ctrl Pts',(-44.5079524583208,-59.5441932447742,
-44.1308875000001));
#244873=CARTESIAN_POINT('Ctrl Pts',(-43.3135644199415,-59.5441932447742,
-44.0725541666667));
#244874=CARTESIAN_POINT('Ctrl Pts',(-42.7163704007519,-58.5098228615615,
-44.0142208333334));
#244875=CARTESIAN_POINT('Ctrl Pts',(-42.1191763815623,-57.4754524783487,
-43.9558875));
#244876=CARTESIAN_POINT('Ctrl Pts',(-42.7163704007519,-56.4410820951361,
-43.8975541666667));
#244877=CARTESIAN_POINT('Ctrl Pts',(-43.3135644199415,-55.4067117119233,
-43.8392208333333));
#244878=CARTESIAN_POINT('Ctrl Pts',(-44.5079524583208,-55.4067117119234,
-43.7808875));
#244879=CARTESIAN_POINT('Ctrl Pts',(-45.7023404967,-55.4067117119233,-43.7225541666667));
#244880=CARTESIAN_POINT('Ctrl Pts',(-46.2995345158897,-56.4410820951361,
-43.6642208333334));
#244881=CARTESIAN_POINT('Ctrl Pts',(-46.8967285350793,-57.4754524783487,
-43.6058875));
#244882=CARTESIAN_POINT('Ctrl Pts',(-46.2995345158897,-58.5098228615615,
-43.5475541666667));
#244883=CARTESIAN_POINT('Ctrl Pts',(-45.7023404967,-59.5441932447742,-43.4892208333333));
#244884=CARTESIAN_POINT('Ctrl Pts',(-44.5079524583208,-59.5441932447742,
-43.4308875));
#244885=CARTESIAN_POINT('Ctrl Pts',(-43.3135644199415,-59.5441932447742,
-43.3725541666667));
#244886=CARTESIAN_POINT('Ctrl Pts',(-42.7163704007519,-58.5098228615615,
-43.3142208333334));
#244887=CARTESIAN_POINT('Ctrl Pts',(-42.1191763815623,-57.4754524783487,
-43.2558875));
#244888=CARTESIAN_POINT('Ctrl Pts',(-42.7163704007519,-56.4410820951361,
-43.1975541666667));
#244889=CARTESIAN_POINT('Ctrl Pts',(-43.3135644199415,-55.4067117119233,
-43.1392208333334));
#244890=CARTESIAN_POINT('Ctrl Pts',(-44.5079524583208,-55.4067117119234,
-43.0808875));
#244891=CARTESIAN_POINT('Ctrl Pts',(-45.7023404967,-55.4067117119233,-43.0225541666667));
#244892=CARTESIAN_POINT('Ctrl Pts',(-46.2995345158897,-56.4410820951361,
-42.9642208333334));
#244893=CARTESIAN_POINT('Ctrl Pts',(-46.8967285350793,-57.4754524783487,
-42.9058875));
#244894=CARTESIAN_POINT('Ctrl Pts',(-46.2995345158897,-58.5098228615615,
-42.8475541666667));
#244895=CARTESIAN_POINT('Ctrl Pts',(-45.7023404967,-59.5441932447742,-42.7892208333334));
#244896=CARTESIAN_POINT('Ctrl Pts',(-44.5079524583208,-59.5441932447742,
-42.7308875000001));
#244897=CARTESIAN_POINT('Ctrl Pts',(-43.3135644199415,-59.5441932447742,
-42.6725541666667));
#244898=CARTESIAN_POINT('Ctrl Pts',(-42.7163704007519,-58.5098228615615,
-42.6142208333334));
#244899=CARTESIAN_POINT('Ctrl Pts',(-42.1191763815623,-57.4754524783487,
-42.5558875));
#244900=CARTESIAN_POINT('Ctrl Pts',(-42.7163704007519,-56.4410820951361,
-42.4975541666667));
#244901=CARTESIAN_POINT('Ctrl Pts',(-43.3135644199415,-55.4067117119233,
-42.4392208333334));
#244902=CARTESIAN_POINT('Ctrl Pts',(-44.5079524583208,-55.4067117119234,
-42.3808875000001));
#244903=CARTESIAN_POINT('Ctrl Pts',(-45.7023404967,-55.4067117119233,-42.3225541666667));
#244904=CARTESIAN_POINT('Ctrl Pts',(-46.2995345158897,-56.4410820951361,
-42.2642208333334));
#244905=CARTESIAN_POINT('Ctrl Pts',(-46.8967285350793,-57.4754524783487,
-42.2058875));
#244906=CARTESIAN_POINT('Ctrl Pts',(-46.2995345158897,-58.5098228615615,
-42.1475541666667));
#244907=CARTESIAN_POINT('Ctrl Pts',(-45.7023404967,-59.5441932447742,-42.0892208333334));
#244908=CARTESIAN_POINT('Ctrl Pts',(-44.5079524583208,-59.5441932447742,
-42.0308875000001));
#244909=CARTESIAN_POINT('Ctrl Pts',(-43.3135644199415,-59.5441932447742,
-41.9725541666667));
#244910=CARTESIAN_POINT('Ctrl Pts',(-42.7163704007519,-58.5098228615615,
-41.9142208333334));
#244911=CARTESIAN_POINT('Ctrl Pts',(-42.1191763815623,-57.4754524783487,
-41.8558875));
#244912=CARTESIAN_POINT('Ctrl Pts',(-42.7163704007519,-56.4410820951361,
-41.7975541666667));
#244913=CARTESIAN_POINT('Ctrl Pts',(-43.3135644199415,-55.4067117119233,
-41.7392208333334));
#244914=CARTESIAN_POINT('Ctrl Pts',(-44.5079524583208,-55.4067117119234,
-41.6808875000001));
#244915=CARTESIAN_POINT('Ctrl Pts',(-45.7023404967,-55.4067117119233,-41.6225541666667));
#244916=CARTESIAN_POINT('Ctrl Pts',(-46.2995345158897,-56.4410820951361,
-41.5642208333334));
#244917=CARTESIAN_POINT('Ctrl Pts',(-46.8967285350793,-57.4754524783487,
-41.5058875));
#244918=CARTESIAN_POINT('Ctrl Pts',(-46.2995345158897,-58.5098228615615,
-41.4475541666667));
#244919=CARTESIAN_POINT('Ctrl Pts',(-45.7023404967,-59.5441932447742,-41.3892208333334));
#244920=CARTESIAN_POINT('Ctrl Pts',(-44.5079524583208,-59.5441932447742,
-41.3308875000001));
#244921=CARTESIAN_POINT('Ctrl Pts',(-43.3135644199415,-59.5441932447742,
-41.2725541666667));
#244922=CARTESIAN_POINT('Ctrl Pts',(-42.7163704007519,-58.5098228615615,
-41.2142208333333));
#244923=CARTESIAN_POINT('Ctrl Pts',(-42.1191763815623,-57.4754524783487,
-41.1558875));
#244924=CARTESIAN_POINT('Ctrl Pts',(-42.7163704007519,-56.4410820951361,
-41.0975541666667));
#244925=CARTESIAN_POINT('Ctrl Pts',(-43.3135644199415,-55.4067117119233,
-41.0392208333333));
#244926=CARTESIAN_POINT('Ctrl Pts',(-44.5079524583208,-55.4067117119234,
-40.9808875000001));
#244927=CARTESIAN_POINT('Ctrl Pts',(-45.7023404967,-55.4067117119233,-40.9225541666667));
#244928=CARTESIAN_POINT('Ctrl Pts',(-46.2995345158897,-56.4410820951361,
-40.8642208333334));
#244929=CARTESIAN_POINT('Ctrl Pts',(-46.8967285350793,-57.4754524783487,
-40.8058875));
#244930=CARTESIAN_POINT('Ctrl Pts',(-46.2995345158897,-58.5098228615615,
-40.7475541666667));
#244931=CARTESIAN_POINT('Ctrl Pts',(-45.7023404967,-59.5441932447742,-40.6892208333333));
#244932=CARTESIAN_POINT('Ctrl Pts',(-44.5079524583208,-59.5441932447742,
-40.6308875));
#244933=CARTESIAN_POINT('Ctrl Pts',(-43.3135644199415,-59.5441932447742,
-40.5725541666667));
#244934=CARTESIAN_POINT('Ctrl Pts',(-42.7163704007519,-58.5098228615615,
-40.5142208333333));
#244935=CARTESIAN_POINT('Ctrl Pts',(-42.1191763815623,-57.4754524783487,
-40.4558875));
#244936=CARTESIAN_POINT('Ctrl Pts',(-42.7163704007519,-56.4410820951361,
-40.3975541666667));
#244937=CARTESIAN_POINT('Ctrl Pts',(-43.3135644199415,-55.4067117119233,
-40.3392208333333));
#244938=CARTESIAN_POINT('Ctrl Pts',(-44.5079524583208,-55.4067117119234,
-40.2808875));
#244939=CARTESIAN_POINT('Ctrl Pts',(-45.7023404967,-55.4067117119233,-40.2225541666667));
#244940=CARTESIAN_POINT('Ctrl Pts',(-46.2995345158897,-56.4410820951361,
-40.1642208333333));
#244941=CARTESIAN_POINT('Ctrl Pts',(-46.8967285350793,-57.4754524783487,
-40.1058875));
#244942=CARTESIAN_POINT('Ctrl Pts',(-46.2995345158897,-58.5098228615615,
-40.0475541666667));
#244943=CARTESIAN_POINT('Ctrl Pts',(-45.7023404967,-59.5441932447742,-39.9892208333333));
#244944=CARTESIAN_POINT('Ctrl Pts',(-44.5079524583208,-59.5441932447742,
-39.9308875));
#244945=CARTESIAN_POINT('Ctrl Pts',(-43.3135644199415,-59.5441932447742,
-39.8725541666667));
#244946=CARTESIAN_POINT('Ctrl Pts',(-42.7163704007519,-58.5098228615615,
-39.8142208333334));
#244947=CARTESIAN_POINT('Ctrl Pts',(-42.1191763815623,-57.4754524783487,
-39.7558875));
#244948=CARTESIAN_POINT('Ctrl Pts',(-42.7163704007519,-56.4410820951361,
-39.6975541666667));
#244949=CARTESIAN_POINT('Ctrl Pts',(-43.3135644199415,-55.4067117119233,
-39.6392208333334));
#244950=CARTESIAN_POINT('Ctrl Pts',(-44.5079524583208,-55.4067117119234,
-39.5808875000001));
#244951=CARTESIAN_POINT('Ctrl Pts',(-45.7023404967,-55.4067117119233,-39.5225541666667));
#244952=CARTESIAN_POINT('Ctrl Pts',(-46.2995345158897,-56.4410820951361,
-39.4642208333333));
#244953=CARTESIAN_POINT('Ctrl Pts',(-46.8967285350793,-57.4754524783487,
-39.4058875));
#244954=CARTESIAN_POINT('Ctrl Pts',(-46.2995345158897,-58.5098228615615,
-39.3475541666667));
#244955=CARTESIAN_POINT('Ctrl Pts',(-45.7023404967,-59.5441932447742,-39.2892208333334));
#244956=CARTESIAN_POINT('Ctrl Pts',(-44.5079524583208,-59.5441932447742,
-39.2308875));
#244957=CARTESIAN_POINT('Ctrl Pts',(-43.3135644199415,-59.5441932447742,
-39.1725541666667));
#244958=CARTESIAN_POINT('Ctrl Pts',(-42.7163704007519,-58.5098228615615,
-39.1142208333333));
#244959=CARTESIAN_POINT('Ctrl Pts',(-42.1191763815623,-57.4754524783487,
-39.0558875));
#244960=CARTESIAN_POINT('Ctrl Pts',(-42.7163704007519,-56.4410820951361,
-38.9975541666667));
#244961=CARTESIAN_POINT('Ctrl Pts',(-43.3135644199415,-55.4067117119233,
-38.9392208333334));
#244962=CARTESIAN_POINT('Ctrl Pts',(-44.5079524583208,-55.4067117119234,
-38.8808875));
#244963=CARTESIAN_POINT('Ctrl Pts',(-45.7023404967,-55.4067117119233,-38.8225541666667));
#244964=CARTESIAN_POINT('Ctrl Pts',(-46.2995345158897,-56.4410820951361,
-38.7642208333333));
#244965=CARTESIAN_POINT('Ctrl Pts',(-46.8967285350793,-57.4754524783487,
-38.7058875));
#244966=CARTESIAN_POINT('Ctrl Pts',(-46.2995345158897,-58.5098228615615,
-38.6475541666667));
#244967=CARTESIAN_POINT('Ctrl Pts',(-45.7023404967,-59.5441932447742,-38.5892208333334));
#244968=CARTESIAN_POINT('Ctrl Pts',(-44.5079524583208,-59.5441932447742,
-38.5308875));
#244969=CARTESIAN_POINT('Ctrl Pts',(-43.3135644199415,-59.5441932447742,
-38.4725541666667));
#244970=CARTESIAN_POINT('Ctrl Pts',(-42.7163704007519,-58.5098228615615,
-38.4142208333334));
#244971=CARTESIAN_POINT('Ctrl Pts',(-42.1191763815623,-57.4754524783487,
-38.3558875));
#244972=CARTESIAN_POINT('Ctrl Pts',(-42.7163704007519,-56.4410820951361,
-38.2975541666667));
#244973=CARTESIAN_POINT('Ctrl Pts',(-43.3135644199415,-55.4067117119233,
-38.2392208333333));
#244974=CARTESIAN_POINT('Ctrl Pts',(-44.5079524583208,-55.4067117119234,
-38.1808875000001));
#244975=CARTESIAN_POINT('Ctrl Pts',(-45.7023404967,-55.4067117119233,-38.1225541666667));
#244976=CARTESIAN_POINT('Ctrl Pts',(-46.2995345158897,-56.4410820951361,
-38.0642208333334));
#244977=CARTESIAN_POINT('Ctrl Pts',(-46.8967285350793,-57.4754524783487,
-38.0058875));
#244978=CARTESIAN_POINT('Ctrl Pts',(-46.2995345158897,-58.5098228615615,
-37.9475541666667));
#244979=CARTESIAN_POINT('Ctrl Pts',(-45.7023404967,-59.5441932447742,-37.8892208333334));
#244980=CARTESIAN_POINT('Ctrl Pts',(-44.5079524583208,-59.5441932447742,
-37.8308875));
#244981=CARTESIAN_POINT('Ctrl Pts',(-43.3135644199415,-59.5441932447742,
-37.7725541666667));
#244982=CARTESIAN_POINT('Ctrl Pts',(-42.7163704007519,-58.5098228615615,
-37.7142208333333));
#244983=CARTESIAN_POINT('Ctrl Pts',(-42.1191763815623,-57.4754524783487,
-37.6558875));
#244984=CARTESIAN_POINT('Ctrl Pts',(-42.7163704007519,-56.4410820951361,
-37.5975541666667));
#244985=CARTESIAN_POINT('Ctrl Pts',(-43.3135644199415,-55.4067117119233,
-37.5392208333334));
#244986=CARTESIAN_POINT('Ctrl Pts',(-44.5079524583208,-55.4067117119234,
-37.4808875));
#244987=CARTESIAN_POINT('Ctrl Pts',(-45.7023404967,-55.4067117119233,-37.4225541666667));
#244988=CARTESIAN_POINT('Ctrl Pts',(-46.2995345158897,-56.4410820951361,
-37.3642208333333));
#244989=CARTESIAN_POINT('Ctrl Pts',(-46.8967285350793,-57.4754524783487,
-37.3058875));
#244990=CARTESIAN_POINT('Ctrl Pts',(-46.2995345158897,-58.5098228615615,
-37.2475541666667));
#244991=CARTESIAN_POINT('Ctrl Pts',(-46.2219998538691,-58.6441168355289,
-37.239980655983));
#244992=CARTESIAN_POINT('Ctrl Pts',(-46.1253112086366,-58.7653513237809,
-37.2318399189827));
#244993=CARTESIAN_POINT('Ctrl Pts',(-43.4124017072694,-55.802201528474,
-38.9060754033995));
#244994=CARTESIAN_POINT('Ctrl Pts',(-43.3649158658203,-55.8332929240044,
-38.9093809723611));
#244995=CARTESIAN_POINT('Ctrl Pts',(-43.3188133243802,-55.8663716512136,
-38.9126746807634));
#244996=CARTESIAN_POINT('Ctrl Pts',(-43.2743250866905,-55.9012347622251,
-38.9159389233579));
#244997=CARTESIAN_POINT('Ctrl Pts',(-43.2296908678756,-55.9362122710289,
-38.9192138770489));
#244998=CARTESIAN_POINT('Ctrl Pts',(-43.1866820205791,-55.972985308453,
-38.9224591311364));
#244999=CARTESIAN_POINT('Ctrl Pts',(-43.1454915293058,-56.0113153370374,
-38.925657963383));
#245000=CARTESIAN_POINT('Ctrl Pts',(-43.1039234831771,-56.0499967012809,
-38.9288861163445));
#245001=CARTESIAN_POINT('Ctrl Pts',(-43.064207623636,-56.0902630655489,
-38.9320669558098));
#245002=CARTESIAN_POINT('Ctrl Pts',(-43.0264951685045,-56.1318445720534,
-38.9351849561294));
#245003=CARTESIAN_POINT('Ctrl Pts',(-42.9885545942382,-56.1736776012247,
-38.9383218169429));
#245004=CARTESIAN_POINT('Ctrl Pts',(-42.9526418729829,-56.2168409968285,
-38.9413950476852));
#245005=CARTESIAN_POINT('Ctrl Pts',(-42.9188598747448,-56.2610457456956,
-38.9443910067074));
#245006=CARTESIAN_POINT('Ctrl Pts',(-42.8846518529637,-56.3058079590324,
-38.9474247476591));
#245007=CARTESIAN_POINT('Ctrl Pts',(-42.852628641587,-56.3516372104306,
-38.9503792335294));
#245008=CARTESIAN_POINT('Ctrl Pts',(-42.8228435979642,-56.3982301413591,
-38.9532429054736));
#245009=CARTESIAN_POINT('Ctrl Pts',(-42.8065246134638,-56.4237580313726,
-38.9548118881705));
#245010=CARTESIAN_POINT('Ctrl Pts',(-42.7908765577231,-56.4495151786358,
-38.9563536575169));
#245011=CARTESIAN_POINT('Ctrl Pts',(-42.7759016507518,-56.4754524783487,
-38.9578666666668));
#245012=CARTESIAN_POINT('Ctrl Pts',(-42.7486194549309,-56.5227066276525,
-38.9606231587095));
#245013=CARTESIAN_POINT('Ctrl Pts',(-42.7229732223034,-56.571599774412,
-38.9634751990818));
#245014=CARTESIAN_POINT('Ctrl Pts',(-42.699209382297,-56.6219610565873,
-38.9664128682174));
#245015=CARTESIAN_POINT('Ctrl Pts',(-42.6756509453961,-56.6718870402692,
-38.9693251455661));
#245016=CARTESIAN_POINT('Ctrl Pts',(-42.6539431678017,-56.7232556458407,
-38.9723215636153));
#245017=CARTESIAN_POINT('Ctrl Pts',(-42.6343032293951,-56.7758552387935,
-38.9753898218966));
#245018=CARTESIAN_POINT('Ctrl Pts',(-42.6148606751112,-56.827926198494,
-38.9784272437538));
#245019=CARTESIAN_POINT('Ctrl Pts',(-42.5974451867678,-56.881203113289,
-38.9815350449805));
#245020=CARTESIAN_POINT('Ctrl Pts',(-42.582235617094,-56.93544112293,-38.9846989841965));
#245021=CARTESIAN_POINT('Ctrl Pts',(-42.5685080995495,-56.9843940680093,
-38.9875546225892));
#245022=CARTESIAN_POINT('Ctrl Pts',(-42.5565774230983,-57.0341291617399,
-38.9904559466857));
#245023=CARTESIAN_POINT('Ctrl Pts',(-42.5465468989916,-57.0844431661648,
-38.9933911308716));
#245024=CARTESIAN_POINT('Ctrl Pts',(43.4805771074156,-59.5712767529309,
-39.2399080357013));
#245025=CARTESIAN_POINT('Ctrl Pts',(43.4150727209207,-59.5358440364426,
-39.2223070534893));
#245026=CARTESIAN_POINT('Ctrl Pts',(43.2883193276586,-59.4590682572254,
-39.1867578392588));
#245027=CARTESIAN_POINT('Ctrl Pts',(43.1106712693135,-59.32658002426,-39.1324031814995));
#245028=CARTESIAN_POINT('Ctrl Pts',(43.0005921597408,-59.2266373021163,
-39.0954660506179));
#245029=CARTESIAN_POINT('Ctrl Pts',(42.8948534568781,-59.1207134074407,
-39.0581733199915));
#245030=CARTESIAN_POINT('Ctrl Pts',(42.7951360401793,-59.0104958554849,
-39.0211184761739));
#245031=CARTESIAN_POINT('Ctrl Pts',(42.6850011896347,-58.8622904152127,
-38.9753582681256));
#245032=CARTESIAN_POINT('Ctrl Pts',(42.6055727997797,-58.7375004045667,
-38.939089851323));
#245033=CARTESIAN_POINT('Ctrl Pts',(42.5503788594446,-58.6407591922129,
-38.9120596161462));
#245034=CARTESIAN_POINT('Ctrl Pts',(42.5165536369311,-58.5741539171446,
-38.8941613358138));
#245035=CARTESIAN_POINT('Ctrl Pts',(42.4842288567228,-58.5064298632496,
-38.8763157156907));
#245036=CARTESIAN_POINT('Ctrl Pts',(42.4689425396028,-58.4722695523732,
-38.8674882509199));
#245037=CARTESIAN_POINT('Ctrl Pts',(42.4257123024776,-58.3690064948315,
-38.8413136266604));
#245038=CARTESIAN_POINT('Ctrl Pts',(42.3750272156063,-58.229152189777,-38.8072100415055));
#245039=CARTESIAN_POINT('Ctrl Pts',(42.3380647902547,-58.0850119200902,
-38.7746901633276));
#245040=CARTESIAN_POINT('Ctrl Pts',(42.3155659796374,-57.9752818499468,
-38.7509105250088));
#245041=CARTESIAN_POINT('Ctrl Pts',(42.3089374211558,-57.9384266221928,
-38.7430843922672));
#245042=CARTESIAN_POINT('Ctrl Pts',(42.297458012674,-57.864178756387,-38.7276438637217));
#245043=CARTESIAN_POINT('Ctrl Pts',(42.292601515188,-57.8267325312259,-38.720018782004));
#245044=CARTESIAN_POINT('Ctrl Pts',(42.2847289916893,-57.7514526301959,
-38.7050196673963));
#245045=CARTESIAN_POINT('Ctrl Pts',(42.2817363521424,-57.7138759968928,
-38.6976962453237));
#245046=CARTESIAN_POINT('Ctrl Pts',(42.277596992864,-57.6387184974263,-38.6833720377019));
#245047=CARTESIAN_POINT('Ctrl Pts',(42.2741651307842,-57.5260409596698,
-38.6623829091612));
#245048=CARTESIAN_POINT('Ctrl Pts',(42.2805893100654,-57.3760354719141,
-38.6363740800325));
#245049=CARTESIAN_POINT('Ctrl Pts',(42.2937061680812,-57.2637038035873,
-38.618370061439));
#245050=CARTESIAN_POINT('Ctrl Pts',(42.3043247017591,-57.1888547452426,
-38.6067079534822));
#245051=CARTESIAN_POINT('Ctrl Pts',(42.3105743117123,-57.1514345461221,
-38.6010450635964));
#245052=CARTESIAN_POINT('Ctrl Pts',(42.3249704170347,-57.0766935209607,
-38.590076215021));
#245053=CARTESIAN_POINT('Ctrl Pts',(42.3331592025312,-57.0392159768686,
-38.5847494243559));
#245054=CARTESIAN_POINT('Ctrl Pts',(42.3512949844302,-56.9651221381903,
-38.5745673038812));
#245055=CARTESIAN_POINT('Ctrl Pts',(42.3712216906218,-56.8916587034686,
-38.564820665347));
#245056=CARTESIAN_POINT('Ctrl Pts',(42.4063979707918,-56.7834465224234,
-38.5515118436));
#245057=CARTESIAN_POINT('Ctrl Pts',(42.4468320479729,-56.6771725078319,
-38.5395042677724));
#245058=CARTESIAN_POINT('Ctrl Pts',(42.4925290654744,-56.5728473165674,
-38.5288039137004));
#245059=CARTESIAN_POINT('Ctrl Pts',(42.5265325119253,-56.5046058456765,
-38.5225509073062));
#245060=CARTESIAN_POINT('Ctrl Pts',(42.5623338475306,-56.4370293947697,
-38.5167461666044));
#245061=CARTESIAN_POINT('Ctrl Pts',(42.5811223641794,-56.4035923099625,
-38.5140693065785));
#245062=CARTESIAN_POINT('Ctrl Pts',(42.620584523009,-56.3373241998654,-38.5091697400817));
#245063=CARTESIAN_POINT('Ctrl Pts',(42.6411082254821,-56.3047465904101,
-38.5069659500128));
#245064=CARTESIAN_POINT('Ctrl Pts',(42.7048067991197,-56.2090283357163,
-38.501110858935));
#245065=CARTESIAN_POINT('Ctrl Pts',(42.7502234543428,-56.1476408662828,
-38.4981890389281));
#245066=CARTESIAN_POINT('Ctrl Pts',(42.8467942323831,-56.0297655581676,
-38.4942910511033));
#245067=CARTESIAN_POINT('Ctrl Pts',(42.8979715413934,-55.9732420482176,
-38.4933125989996));
#245068=CARTESIAN_POINT('Ctrl Pts',(42.9790570553347,-55.8921695883033,
-38.4933149859729));
#245069=CARTESIAN_POINT('Ctrl Pts',(43.0068374106561,-55.8657400908868,
-38.4935622007431));
#245070=CARTESIAN_POINT('Ctrl Pts',(43.0495800649421,-55.8270637749536,
-38.4943063068789));
#245071=CARTESIAN_POINT('Ctrl Pts',(43.0640222060113,-55.8143203511958,
-38.494617152342));
#245072=CARTESIAN_POINT('Ctrl Pts',(43.0932714774893,-55.7891564261061,
-38.4953646906773));
#245073=CARTESIAN_POINT('Ctrl Pts',(43.1080901283632,-55.7767277938553,
-38.4958020036096));
#245074=CARTESIAN_POINT('Ctrl Pts',(43.1528523310046,-55.7401327167866,
-38.4972962980169));
#245075=CARTESIAN_POINT('Ctrl Pts',(43.2134913856688,-55.6930468850421,
-38.4997758707861));
#245076=CARTESIAN_POINT('Ctrl Pts',(43.3385569247743,-55.6055389451161,
-38.5066450244003));
#245077=CARTESIAN_POINT('Ctrl Pts',(43.4691986576013,-55.5278792007279,
-38.5163302992824));
#245078=CARTESIAN_POINT('Ctrl Pts',(43.5713395927684,-55.4769743237494,
-38.5256877381308));
#245079=CARTESIAN_POINT('Ctrl Pts',(43.6403672861995,-55.4446857735354,
-38.5323951500278));
#245080=CARTESIAN_POINT('Ctrl Pts',(43.6753577685123,-55.4293620157832,
-38.5359845633874));
#245081=CARTESIAN_POINT('Ctrl Pts',(43.7462462065788,-55.4003985583156,
-38.5436333065981));
#245082=CARTESIAN_POINT('Ctrl Pts',(43.7822717759725,-55.3867204456352,
-38.5477088862383));
#245083=CARTESIAN_POINT('Ctrl Pts',(43.8543821738219,-55.3613797848081,
-38.5562346427694));
#245084=CARTESIAN_POINT('Ctrl Pts',(43.890622407919,-55.349649082917,-38.5607007444526));
#245085=CARTESIAN_POINT('Ctrl Pts',(43.9997560709039,-55.3172704656441,
-38.5746802407103));
#245086=CARTESIAN_POINT('Ctrl Pts',(44.1098017310836,-55.290468361793,-38.5898286859852));
#245087=CARTESIAN_POINT('Ctrl Pts',(44.2583166685835,-55.2656490138239,
-38.612301023075));
#245088=CARTESIAN_POINT('Ctrl Pts',(44.3705972700495,-55.2524997368729,
-38.6302900391873));
#245089=CARTESIAN_POINT('Ctrl Pts',(44.446056048267,-55.2474029004138,-38.6430428201589));
#245090=CARTESIAN_POINT('Ctrl Pts',(44.5218128020516,-55.2441636366351,
-38.65617756452));
#245091=CARTESIAN_POINT('Ctrl Pts',(44.5599089424743,-55.2434808562086,
-38.6629497802385));
#245092=CARTESIAN_POINT('Ctrl Pts',(44.6354869543582,-55.2439911084578,
-38.6767130108817));
#245093=CARTESIAN_POINT('Ctrl Pts',(44.6731456892459,-55.2451740103824,
-38.6837342374529));
#245094=CARTESIAN_POINT('Ctrl Pts',(44.7481014788608,-55.2493620066237,
-38.6980304684339));
#245095=CARTESIAN_POINT('Ctrl Pts',(44.860046548974,-55.2583760573225,-38.7198650218829));
#245096=CARTESIAN_POINT('Ctrl Pts',(45.0073845433675,-55.2811507310277,
-38.7505067688753));
#245097=CARTESIAN_POINT('Ctrl Pts',(45.1528189888476,-55.3146135839333,
-38.7826550300594));
#245098=CARTESIAN_POINT('Ctrl Pts',(45.2248832056965,-55.3349380951144,
-38.7992310848652));
#245099=CARTESIAN_POINT('Ctrl Pts',(45.2966462681613,-55.3570913336823,
-38.8160672125853));
#245100=CARTESIAN_POINT('Ctrl Pts',(45.3323638946335,-55.3690863290504,
-38.8246135819642));
#245101=CARTESIAN_POINT('Ctrl Pts',(45.4027951436545,-55.3946744461232,
-38.841798196801));
#245102=CARTESIAN_POINT('Ctrl Pts',(45.4376370321487,-55.4083060218429,
-38.85046633842));
#245103=CARTESIAN_POINT('Ctrl Pts',(45.5409345111852,-55.4516493275196,
-38.8766665754573));
#245104=CARTESIAN_POINT('Ctrl Pts',(45.6082182891413,-55.4838201174091,
-38.8944064774514));
#245105=CARTESIAN_POINT('Ctrl Pts',(45.7067749877369,-55.5369855856676,
-38.9214216121435));
#245106=CARTESIAN_POINT('Ctrl Pts',(45.7392219877795,-55.5555212114618,
-38.9304915704334));
#245107=CARTESIAN_POINT('Ctrl Pts',(45.8033556832395,-55.5942722159849,
-38.9487787872477));
#245108=CARTESIAN_POINT('Ctrl Pts',(45.8348443691401,-55.6143675312756,
-38.9579395118015));
#245109=CARTESIAN_POINT('Ctrl Pts',(45.9274099842789,-55.6766589025306,
-38.9854159162723));
#245110=CARTESIAN_POINT('Ctrl Pts',(45.9867610865919,-55.7209353156014,
-39.0037703637879));
#245111=CARTESIAN_POINT('Ctrl Pts',(46.1007337830098,-55.8148102393793,
-39.0405190865864));
#245112=CARTESIAN_POINT('Ctrl Pts',(46.1826971388658,-55.889219933262,-39.0681181728269));
#245113=CARTESIAN_POINT('Ctrl Pts',(46.259356574729,-55.9696687352924,-39.0957737179551));
#245114=CARTESIAN_POINT('Ctrl Pts',(46.309266807939,-56.024663053365,-39.1142236413887));
#245115=CARTESIAN_POINT('Ctrl Pts',(46.3336138177017,-56.0528284109483,
-39.1234510495426));
#245116=CARTESIAN_POINT('Ctrl Pts',(46.3692509284248,-56.0961546965833,
-39.1373141736981));
#245117=CARTESIAN_POINT('Ctrl Pts',(46.3809719555493,-56.1107655250657,
-39.14193505412));
#245118=CARTESIAN_POINT('Ctrl Pts',(46.4039850968433,-56.1401806715041,
-39.1511314768264));
#245119=CARTESIAN_POINT('Ctrl Pts',(46.4153001903629,-56.1550126624776,
-39.1557159133813));
#245120=CARTESIAN_POINT('Ctrl Pts',(46.4486370096885,-56.1998310060263,
-39.1694131182659));
#245121=CARTESIAN_POINT('Ctrl Pts',(46.4700835091466,-56.2301795317326,
-39.1784826054425));
#245122=CARTESIAN_POINT('Ctrl Pts',(46.532071913686,-56.3225583984772,-39.2054898733524));
#245123=CARTESIAN_POINT('Ctrl Pts',(46.5894197348374,-56.4176636744323,
-39.23211607576));
#245124=CARTESIAN_POINT('Ctrl Pts',(46.6566074362748,-56.5498680842415,
-39.2668544229849));
#245125=CARTESIAN_POINT('Ctrl Pts',(46.6870820302515,-56.617790568625,-39.2839693714534));
#245126=CARTESIAN_POINT('Ctrl Pts',(46.7159729830272,-56.6866360545619,
-39.3009558869148));
#245127=CARTESIAN_POINT('Ctrl Pts',(46.7296188023799,-56.7214992889704,
-39.3093799218186));
#245128=CARTESIAN_POINT('Ctrl Pts',(46.7553216997643,-56.7922546384013,
-39.3261176641085));
#245129=CARTESIAN_POINT('Ctrl Pts',(46.7672996943011,-56.8279354881579,
-39.3343809787628));
#245130=CARTESIAN_POINT('Ctrl Pts',(46.8004530502947,-56.9353633959568,
-39.358737163018));
#245131=CARTESIAN_POINT('Ctrl Pts',(46.8189795501832,-57.0077635587999,
-39.3744658121213));
#245132=CARTESIAN_POINT('Ctrl Pts',(46.848916211803,-57.1540080946302,-39.4048998290393));
#245133=CARTESIAN_POINT('Ctrl Pts',(46.866048617508,-57.2647966217996,-39.4269646939479));
#245134=CARTESIAN_POINT('Ctrl Pts',(46.875074749658,-57.3772756893033,-39.4478819384746));
#245135=CARTESIAN_POINT('Ctrl Pts',(46.8792542953452,-57.4526370309597,
-39.4615663943076));
#245136=CARTESIAN_POINT('Ctrl Pts',(46.8804258736835,-57.4905390832845,
-39.4682843608713));
#245137=CARTESIAN_POINT('Ctrl Pts',(46.8808837743635,-57.566610437341,-39.4814341960201));
#245138=CARTESIAN_POINT('Ctrl Pts',(46.8801708637706,-57.604491394965,-39.4878166677226));
#245139=CARTESIAN_POINT('Ctrl Pts',(46.8768913879562,-57.6800597985945,
-39.5002231148134));
#245140=CARTESIAN_POINT('Ctrl Pts',(46.8691896925243,-57.7930657109158,
-39.5182849936093));
#245141=CARTESIAN_POINT('Ctrl Pts',(46.8479069711518,-57.9423669591112,
-39.540205996752));
#245142=CARTESIAN_POINT('Ctrl Pts',(46.8236459543104,-58.053306681129,-39.5550278422771));
#245143=CARTESIAN_POINT('Ctrl Pts',(46.8055990109883,-58.1270324939452,
-39.5645447403379));
#245144=CARTESIAN_POINT('Ctrl Pts',(46.7956339676918,-58.1637938532181,
-39.5691227921436));
#245145=CARTESIAN_POINT('Ctrl Pts',(46.7738161327052,-58.2370162077019,
-39.5779016468881));
#245146=CARTESIAN_POINT('Ctrl Pts',(46.7619036278491,-58.2736352268715,
-39.5821192203466));
#245147=CARTESIAN_POINT('Ctrl Pts',(46.7364059718256,-58.3458255995332,
-39.5900871854462));
#245148=CARTESIAN_POINT('Ctrl Pts',(46.7091836493705,-58.4171862986019,
-39.5976163356366));
#245149=CARTESIAN_POINT('Ctrl Pts',(46.663274408039,-58.5216699086648,-39.6076014242402));
#245150=CARTESIAN_POINT('Ctrl Pts',(46.6123207377325,-58.6236436013082,
-39.616293729045));
#245151=CARTESIAN_POINT('Ctrl Pts',(46.5563244858032,-58.7230996041114,
-39.6236943138341));
#245152=CARTESIAN_POINT('Ctrl Pts',(46.515607032986,-58.7877140896312,-39.6277619492082));
#245153=CARTESIAN_POINT('Ctrl Pts',(46.4731710833873,-58.8514710047945,
-39.6313905635194));
#245154=CARTESIAN_POINT('Ctrl Pts',(46.4511086137465,-58.8829006319494,
-39.6329844599904));
#245155=CARTESIAN_POINT('Ctrl Pts',(46.4051673201274,-58.9449633016888,
-39.6357273485653));
#245156=CARTESIAN_POINT('Ctrl Pts',(46.381447994276,-58.975377588932,-39.6368662598532));
#245157=CARTESIAN_POINT('Ctrl Pts',(46.3084068909562,-59.0643493136614,
-39.6395761233691));
#245158=CARTESIAN_POINT('Ctrl Pts',(46.2570407846102,-59.1209150453974,
-39.6404603784325));
#245159=CARTESIAN_POINT('Ctrl Pts',(46.1491379755941,-59.228544463199,-39.6404138814247));
#245160=CARTESIAN_POINT('Ctrl Pts',(46.0925836555155,-59.2796343044913,
-39.6394845811684));
#245161=CARTESIAN_POINT('Ctrl Pts',(46.0038529437629,-59.3521266125547,
-39.6367223387528));
#245162=CARTESIAN_POINT('Ctrl Pts',(45.9736068078661,-59.3756113554055,
-39.6355721163029));
#245163=CARTESIAN_POINT('Ctrl Pts',(45.9272656961273,-59.4097723546528,
-39.6334997725088));
#245164=CARTESIAN_POINT('Ctrl Pts',(45.9116419215573,-59.4209912820171,
-39.6327502808957));
#245165=CARTESIAN_POINT('Ctrl Pts',(45.8800804794677,-59.4430610802669,
-39.6311351339295));
#245166=CARTESIAN_POINT('Ctrl Pts',(45.8321587971618,-59.4756823489919,
-39.628531354857));
#245167=CARTESIAN_POINT('Ctrl Pts',(45.7834097108732,-59.5062438963941,
-39.6254355071979));
#245168=CARTESIAN_POINT('Ctrl Pts',(45.717633106262,-59.5452481912826,-39.6208773262667));
#245169=CARTESIAN_POINT('Ctrl Pts',(45.6178307490054,-59.601113548897,-39.6133952897297));
#245170=CARTESIAN_POINT('Ctrl Pts',(45.4802897643185,-59.6652183443042,
-39.6008811885904));
#245171=CARTESIAN_POINT('Ctrl Pts',(45.3738098009101,-59.7055766782111,
-39.5896017905935));
#245172=CARTESIAN_POINT('Ctrl Pts',(45.3020778813705,-59.7307512119865,
-39.5816566825671));
#245173=CARTESIAN_POINT('Ctrl Pts',(45.2658207311094,-59.7424779859237,
-39.5774690651077));
#245174=CARTESIAN_POINT('Ctrl Pts',(45.1926264675053,-59.7641596016776,
-39.5686715125846));
#245175=CARTESIAN_POINT('Ctrl Pts',(45.1555073907618,-59.7741562512684,
-39.5640376159893));
#245176=CARTESIAN_POINT('Ctrl Pts',(45.0441315765335,-59.8011904590316,
-39.5496210468413));
#245177=CARTESIAN_POINT('Ctrl Pts',(44.9324484012679,-59.8224577850013,
-39.5341534065747));
#245178=CARTESIAN_POINT('Ctrl Pts',(44.8203079610257,-59.8353953605365,
-39.5171556909205));
#245179=CARTESIAN_POINT('Ctrl Pts',(44.7080184564226,-59.8455760612675,
-39.4996502778008));
#245180=CARTESIAN_POINT('Ctrl Pts',(44.6329372249224,-59.8486931621852,
-39.4873001861445));
#245181=CARTESIAN_POINT('Ctrl Pts',(44.5200834441659,-59.8478515133141,
-39.4677634802869));
#245182=CARTESIAN_POINT('Ctrl Pts',(44.4823810871712,-59.8466449718289,
-39.4610736497974));
#245183=CARTESIAN_POINT('Ctrl Pts',(44.4258051079382,-59.8434394706745,
-39.4507883432074));
#245184=CARTESIAN_POINT('Ctrl Pts',(44.4069254589855,-59.8421361346926,
-39.4473147915973));
#245185=CARTESIAN_POINT('Ctrl Pts',(44.3691376542581,-59.8390581625153,
-39.4402793331445));
#245186=CARTESIAN_POINT('Ctrl Pts',(44.3502459350849,-59.8372838734483,
-39.4367203104461));
#245187=CARTESIAN_POINT('Ctrl Pts',(44.2562487381671,-59.8272835659938,
-39.4188041728073));
#245188=CARTESIAN_POINT('Ctrl Pts',(44.1080045765469,-59.8040393501646,
-39.3892226636159));
#245189=CARTESIAN_POINT('Ctrl Pts',(43.9639303529155,-59.7668593120831,
-39.3578670379715));
#245190=CARTESIAN_POINT('Ctrl Pts',(43.8219159040518,-59.7227861654643,
-39.3256251231267));
#245191=CARTESIAN_POINT('Ctrl Pts',(43.7519290534068,-59.6972943066161,
-39.3090578287531));
#245192=CARTESIAN_POINT('Ctrl Pts',(43.665783177736,-59.6610675807531,-39.2877890488175));
#245193=CARTESIAN_POINT('Ctrl Pts',(43.6486106666635,-59.653596197985,-39.2835041280971));
#245194=CARTESIAN_POINT('Ctrl Pts',(43.6144193015916,-59.6382222359849,
-39.2748825183767));
#245195=CARTESIAN_POINT('Ctrl Pts',(43.597366582891,-59.6303022352814,-39.2705368924251));
#245196=CARTESIAN_POINT('Ctrl Pts',(43.5465994182959,-59.605961903298,-39.2574616452183));
#245197=CARTESIAN_POINT('Ctrl Pts',(43.513329300663,-59.588993111175,-39.2487085268073));
#245198=CARTESIAN_POINT('Ctrl Pts',(43.4805771074156,-59.5712767529309,
-39.2399080357013));
#245199=CARTESIAN_POINT('Ctrl Pts',(43.8903154257419,-57.7291941381088,
-41.4266127101804));
#245200=CARTESIAN_POINT('Ctrl Pts',(43.8716814361492,-57.7189244770852,
-41.4090117279687));
#245201=CARTESIAN_POINT('Ctrl Pts',(43.8355945080866,-57.6967277837834,
-41.3734625137379));
#245202=CARTESIAN_POINT('Ctrl Pts',(43.7849271573585,-57.6585752750105,
-41.3191078559793));
#245203=CARTESIAN_POINT('Ctrl Pts',(43.753465403225,-57.62988352171,-41.2821707250961));
#245204=CARTESIAN_POINT('Ctrl Pts',(43.7232071092872,-57.5995155202448,
-41.2448779944712));
#245205=CARTESIAN_POINT('Ctrl Pts',(43.694633283399,-57.5679550683129,-41.2078231506529));
#245206=CARTESIAN_POINT('Ctrl Pts',(43.6629744005209,-57.5256074013359,
-41.162062942605));
#245207=CARTESIAN_POINT('Ctrl Pts',(43.6400741040405,-57.4900012877665,
-41.1257945258022));
#245208=CARTESIAN_POINT('Ctrl Pts',(43.624122646482,-57.4624228770549,-41.0987642906252));
#245209=CARTESIAN_POINT('Ctrl Pts',(43.6143188854815,-57.4434516436916,
-41.0808660102928));
#245210=CARTESIAN_POINT('Ctrl Pts',(43.6049343759216,-57.4241698350281,
-41.0630203901697));
#245211=CARTESIAN_POINT('Ctrl Pts',(43.6004882740613,-57.4144479878336,
-41.054192925399));
#245212=CARTESIAN_POINT('Ctrl Pts',(43.5878889573419,-57.3850715912746,
-41.0280183011396));
#245213=CARTESIAN_POINT('Ctrl Pts',(43.5730447416356,-57.3453166524842,
-40.9939147159844));
#245214=CARTESIAN_POINT('Ctrl Pts',(43.5620571572655,-57.3044044614592,
-40.9613948378065));
#245215=CARTESIAN_POINT('Ctrl Pts',(43.5552843243605,-57.2732819874194,
-40.9376151994878));
#245216=CARTESIAN_POINT('Ctrl Pts',(43.5532714802541,-57.2628325912303,
-40.9297890667463));
#245217=CARTESIAN_POINT('Ctrl Pts',(43.5497454556161,-57.2417890776549,
-40.9143485382007));
#245218=CARTESIAN_POINT('Ctrl Pts',(43.5482304746054,-57.2311797832666,
-40.9067234564832));
#245219=CARTESIAN_POINT('Ctrl Pts',(43.5457184756399,-57.2098591834555,
-40.8917243418755));
#245220=CARTESIAN_POINT('Ctrl Pts',(43.5447290487245,-57.199220662917,-40.8844009198028));
#245221=CARTESIAN_POINT('Ctrl Pts',(43.5432711863927,-57.1779500447907,
-40.8700767121812));
#245222=CARTESIAN_POINT('Ctrl Pts',(43.5418684734652,-57.1460721839032,
-40.8490875836402));
#245223=CARTESIAN_POINT('Ctrl Pts',(43.5431039253892,-57.1036793909824,
-40.8230787545116));
#245224=CARTESIAN_POINT('Ctrl Pts',(43.5463738329101,-57.0719682486671,
-40.8050747359183));
#245225=CARTESIAN_POINT('Ctrl Pts',(43.5490829635055,-57.0508462881094,
-40.7934126279614));
#245226=CARTESIAN_POINT('Ctrl Pts',(43.5507030159248,-57.0402904723448,
-40.7877497380755));
#245227=CARTESIAN_POINT('Ctrl Pts',(43.5544790630841,-57.019214904491,-40.7767808895002));
#245228=CARTESIAN_POINT('Ctrl Pts',(43.5566463931059,-57.0086510117152,
-40.7714540988351));
#245229=CARTESIAN_POINT('Ctrl Pts',(43.5614808344627,-56.9877741662596,
-40.7612719783604));
#245230=CARTESIAN_POINT('Ctrl Pts',(43.5668234022498,-56.9670831174431,
-40.7515253398262));
#245231=CARTESIAN_POINT('Ctrl Pts',(43.5763377125496,-56.9366295208774,
-40.7382165180791));
#245232=CARTESIAN_POINT('Ctrl Pts',(43.5873444561754,-56.9067460923864,
-40.7262089422516));
#245233=CARTESIAN_POINT('Ctrl Pts',(43.5998453117462,-56.8774358278222,
-40.7155085881795));
#245234=CARTESIAN_POINT('Ctrl Pts',(43.6091839698139,-56.8582805167828,
-40.7092555817853));
#245235=CARTESIAN_POINT('Ctrl Pts',(43.6190331668358,-56.8393207538612,
-40.7034508410834));
#245236=CARTESIAN_POINT('Ctrl Pts',(43.6242099732076,-56.8299438685379,
-40.7007739810578));
#245237=CARTESIAN_POINT('Ctrl Pts',(43.6350986096338,-56.8113693026126,
-40.6958744145609));
#245238=CARTESIAN_POINT('Ctrl Pts',(43.6407690742328,-56.8022426567881,
-40.6936706244929));
#245239=CARTESIAN_POINT('Ctrl Pts',(43.6583896223854,-56.7754411523649,
-40.6878155334118));
#245240=CARTESIAN_POINT('Ctrl Pts',(43.6709801307092,-56.7582712890167,
-40.6848937134075));
#245241=CARTESIAN_POINT('Ctrl Pts',(43.6978023804218,-56.725340315416,-40.6809957255822));
#245242=CARTESIAN_POINT('Ctrl Pts',(43.7120405319879,-56.7095692151415,
-40.6800172734785));
#245243=CARTESIAN_POINT('Ctrl Pts',(43.7346338722206,-56.6869796178674,
-40.680019660452));
#245244=CARTESIAN_POINT('Ctrl Pts',(43.7423799312797,-56.6796208977126,
-40.6802668752224));
#245245=CARTESIAN_POINT('Ctrl Pts',(43.7543060585229,-56.6688607312791,
-40.681010981358));
#245246=CARTESIAN_POINT('Ctrl Pts',(43.7583370517177,-56.6653168192219,
-40.6813218268212));
#245247=CARTESIAN_POINT('Ctrl Pts',(43.7665035456834,-56.6583217341419,
-40.6820693651562));
#245248=CARTESIAN_POINT('Ctrl Pts',(43.7706422703,-56.6548683091639,-40.6825066780886));
#245249=CARTESIAN_POINT('Ctrl Pts',(43.7831478581881,-56.6447045100584,
-40.6840009724959));
#245250=CARTESIAN_POINT('Ctrl Pts',(43.8000992888712,-56.6316392340345,
-40.6864805452653));
#245251=CARTESIAN_POINT('Ctrl Pts',(43.8351004518507,-56.6074069729907,
-40.6933496988796));
#245252=CARTESIAN_POINT('Ctrl Pts',(43.8717190640765,-56.5859796680779,
-40.7030349737613));
#245253=CARTESIAN_POINT('Ctrl Pts',(43.9003898794618,-56.5719991465823,
-40.7123924126099));
#245254=CARTESIAN_POINT('Ctrl Pts',(43.919774692733,-56.5631479893168,-40.719099824507));
#245255=CARTESIAN_POINT('Ctrl Pts',(43.9296053152689,-56.5589560552736,
-40.722689237866));
#245256=CARTESIAN_POINT('Ctrl Pts',(43.9495302416178,-56.551051384942,-40.7303379810773));
#245257=CARTESIAN_POINT('Ctrl Pts',(43.959660471973,-56.5473282955902,-40.7344135607172));
#245258=CARTESIAN_POINT('Ctrl Pts',(43.9799461530017,-56.5404515818703,
-40.7429393172485));
#245259=CARTESIAN_POINT('Ctrl Pts',(43.9901452646573,-56.5372793127045,
-40.7474054189318));
#245260=CARTESIAN_POINT('Ctrl Pts',(44.0208712025373,-56.5285586047056,
-40.7613849151889));
#245261=CARTESIAN_POINT('Ctrl Pts',(44.0518784813599,-56.521416173947,-40.7765333604643));
#245262=CARTESIAN_POINT('Ctrl Pts',(44.0937728041468,-56.5149820273198,
-40.799005697554));
#245263=CARTESIAN_POINT('Ctrl Pts',(44.1254693703652,-56.5117027703592,
-40.8169947136667));
#245264=CARTESIAN_POINT('Ctrl Pts',(44.1467868482481,-56.5105547568045,
-40.8297474946377));
#245265=CARTESIAN_POINT('Ctrl Pts',(44.1681963264173,-56.50993223545,-40.842882238999));
#245266=CARTESIAN_POINT('Ctrl Pts',(44.1789665479467,-56.509886262238,-40.8496544547178));
#245267=CARTESIAN_POINT('Ctrl Pts',(44.2003410646824,-56.5103214152413,
-40.8634176853611));
#245268=CARTESIAN_POINT('Ctrl Pts',(44.2109953322312,-56.5108003631786,
-40.8704389119319));
#245269=CARTESIAN_POINT('Ctrl Pts',(44.2322091102727,-56.5122711761573,
-40.8847351429132));
#245270=CARTESIAN_POINT('Ctrl Pts',(44.2639028799147,-56.5152466319394,
-40.9065696963621));
#245271=CARTESIAN_POINT('Ctrl Pts',(44.305661850593,-56.5222422564611,-40.9372114433545));
#245272=CARTESIAN_POINT('Ctrl Pts',(44.346925841944,-56.532247127269,-40.9693597045385));
#245273=CARTESIAN_POINT('Ctrl Pts',(44.3673876336497,-56.53826115526,-40.9859357593442));
#245274=CARTESIAN_POINT('Ctrl Pts',(44.3877715667723,-56.5447901720246,
-41.0027718870644));
#245275=CARTESIAN_POINT('Ctrl Pts',(44.3979208506631,-56.5483132560745,
-41.0113182564434));
#245276=CARTESIAN_POINT('Ctrl Pts',(44.4179418071922,-56.5558066378292,
-41.02850287128));
#245277=CARTESIAN_POINT('Ctrl Pts',(44.4278499085732,-56.5597882829787,
-41.0371710128992));
#245278=CARTESIAN_POINT('Ctrl Pts',(44.4572364860018,-56.5724196473794,
-41.0633712499365));
#245279=CARTESIAN_POINT('Ctrl Pts',(44.4763932211824,-56.581758968269,-41.0811111519311));
#245280=CARTESIAN_POINT('Ctrl Pts',(44.5044772880921,-56.5971447477014,
-41.1081262866225));
#245281=CARTESIAN_POINT('Ctrl Pts',(44.5137271775895,-56.6025015227711,
-41.1171962449124));
#245282=CARTESIAN_POINT('Ctrl Pts',(44.5320183562985,-56.6136863880645,
-41.1354834617267));
#245283=CARTESIAN_POINT('Ctrl Pts',(44.5410031705763,-56.6194798267371,
-41.144644186283));
#245284=CARTESIAN_POINT('Ctrl Pts',(44.5674276642847,-56.6374191091633,
-41.1721205907467));
#245285=CARTESIAN_POINT('Ctrl Pts',(44.5843870769067,-56.6501457393646,
-41.1904750382678));
#245286=CARTESIAN_POINT('Ctrl Pts',(44.616987890196,-56.6770839740703,-41.2272237610649));
#245287=CARTESIAN_POINT('Ctrl Pts',(44.640458797708,-56.6984048650555,-41.2548228473058));
#245288=CARTESIAN_POINT('Ctrl Pts',(44.6624514458289,-56.7214114906953,
-41.2824783924342));
#245289=CARTESIAN_POINT('Ctrl Pts',(44.6767798128067,-56.7371294193188,
-41.3009283158679));
#245290=CARTESIAN_POINT('Ctrl Pts',(44.683774397772,-56.7451748501741,-41.3101557240219));
#245291=CARTESIAN_POINT('Ctrl Pts',(44.6940202659092,-56.7575442973705,
-41.324018848177));
#245292=CARTESIAN_POINT('Ctrl Pts',(44.6973914635031,-56.7617145235639,
-41.328639728599));
#245293=CARTESIAN_POINT('Ctrl Pts',(44.7040131878578,-56.770108052971,-41.3378361513053));
#245294=CARTESIAN_POINT('Ctrl Pts',(44.7072703203268,-56.7743392575068,
-41.3424205878605));
#245295=CARTESIAN_POINT('Ctrl Pts',(44.7168707027477,-56.7871217033085,
-41.3561177927451));
#245296=CARTESIAN_POINT('Ctrl Pts',(44.7230524906066,-56.7957731420119,
-41.3651872799216));
#245297=CARTESIAN_POINT('Ctrl Pts',(44.7409373255192,-56.8220955492914,
-41.3921945478314));
#245298=CARTESIAN_POINT('Ctrl Pts',(44.7575187561203,-56.8491712652862,
-41.4188207502394));
#245299=CARTESIAN_POINT('Ctrl Pts',(44.7770214494108,-56.88676384976,-41.453559097464));
#245300=CARTESIAN_POINT('Ctrl Pts',(44.7858965000619,-56.9060633365117,
-41.4706740459328));
#245301=CARTESIAN_POINT('Ctrl Pts',(44.7943266372896,-56.9256180211132,
-41.4876605613939));
#245302=CARTESIAN_POINT('Ctrl Pts',(44.7983169540911,-56.9355169983302,
-41.4960845962979));
#245303=CARTESIAN_POINT('Ctrl Pts',(44.8058516078422,-56.9556000996462,
-41.5128223385875));
#245304=CARTESIAN_POINT('Ctrl Pts',(44.8093727854448,-56.9657242505397,
-41.5210856532432));
#245305=CARTESIAN_POINT('Ctrl Pts',(44.8191505788346,-56.9961959016236,
-41.5454418374945));
#245306=CARTESIAN_POINT('Ctrl Pts',(44.8246597322132,-57.0167187198372,
-41.5611704866007));
#245307=CARTESIAN_POINT('Ctrl Pts',(44.8336688220904,-57.0581479791523,
-41.5916045035181));
#245308=CARTESIAN_POINT('Ctrl Pts',(44.8389236650083,-57.0895139074259,
-41.613669368427));
#245309=CARTESIAN_POINT('Ctrl Pts',(44.8418900765893,-57.1213299669285,
-41.6345866129535));
#245310=CARTESIAN_POINT('Ctrl Pts',(44.8433488372948,-57.142640498193,-41.6482710687869));
#245311=CARTESIAN_POINT('Ctrl Pts',(44.8438191277705,-57.1533552116615,
-41.6549890353504));
#245312=CARTESIAN_POINT('Ctrl Pts',(44.8442270800594,-57.1748537940466,
-41.6681388704993));
#245313=CARTESIAN_POINT('Ctrl Pts',(44.8441639040618,-57.1855561823783,
-41.6745213422017));
#245314=CARTESIAN_POINT('Ctrl Pts',(44.8435122114514,-57.2069000331791,
-41.6869277892926));
#245315=CARTESIAN_POINT('Ctrl Pts',(44.8417458896958,-57.2388084678274,
-41.7049896680882));
#245316=CARTESIAN_POINT('Ctrl Pts',(44.8362687719071,-57.2809279665006,
-41.7269106712316));
#245317=CARTESIAN_POINT('Ctrl Pts',(44.8298088085522,-57.3121969378441,
-41.7417325167562));
#245318=CARTESIAN_POINT('Ctrl Pts',(44.8249713776488,-57.3329705079708,
-41.751249414817));
#245319=CARTESIAN_POINT('Ctrl Pts',(44.8222858794974,-57.3433254378487,
-41.7558274666229));
#245320=CARTESIAN_POINT('Ctrl Pts',(44.8163797073795,-57.3639440769784,
-41.7646063213672));
#245321=CARTESIAN_POINT('Ctrl Pts',(44.8131427147447,-57.3742522416544,
-41.7688238948253));
#245322=CARTESIAN_POINT('Ctrl Pts',(44.8061917406462,-57.3945668799698,
-41.7767918599254));
#245323=CARTESIAN_POINT('Ctrl Pts',(44.7987498536529,-57.4146412549335,
-41.7843210101159));
#245324=CARTESIAN_POINT('Ctrl Pts',(44.7861419817956,-57.4440129710611,
-41.7943060987191));
#245325=CARTESIAN_POINT('Ctrl Pts',(44.7720982599006,-57.4726583092559,
-41.8029984035242));
#245326=CARTESIAN_POINT('Ctrl Pts',(44.7566193423106,-57.5005749992605,
-41.8103989883131));
#245327=CARTESIAN_POINT('Ctrl Pts',(44.7453362941317,-57.518697088903,-41.8144666236875));
#245328=CARTESIAN_POINT('Ctrl Pts',(44.7335642473644,-57.5365709174371,
-41.8180952379985));
#245329=CARTESIAN_POINT('Ctrl Pts',(44.7274378249752,-57.5453780864623,
-41.8196891344695));
#245330=CARTESIAN_POINT('Ctrl Pts',(44.7146685840676,-57.5627610237142,
-41.8224320230444));
#245331=CARTESIAN_POINT('Ctrl Pts',(44.7080700862024,-57.5712755128024,
-41.8235709343319));
#245332=CARTESIAN_POINT('Ctrl Pts',(44.6877341610586,-57.5961705213949,
-41.8262807978491));
#245333=CARTESIAN_POINT('Ctrl Pts',(44.6734117165454,-57.6119810052107,
-41.8271650529119));
#245334=CARTESIAN_POINT('Ctrl Pts',(44.6432859415473,-57.6420285404153,
-41.827118555904));
#245335=CARTESIAN_POINT('Ctrl Pts',(44.6274777219699,-57.6562729242579,
-41.8261892556471));
#245336=CARTESIAN_POINT('Ctrl Pts',(44.6026489360012,-57.6764545436153,
-41.823427013232));
#245337=CARTESIAN_POINT('Ctrl Pts',(44.5941811636919,-57.6829873126311,
-41.8222767907821));
#245338=CARTESIAN_POINT('Ctrl Pts',(44.5812011369499,-57.6924815728277,
-41.820204446988));
#245339=CARTESIAN_POINT('Ctrl Pts',(44.5768239301145,-57.6955981764101,
-41.8194549553751));
#245340=CARTESIAN_POINT('Ctrl Pts',(44.5679795363474,-57.7017261947271,
-41.8178398084084));
#245341=CARTESIAN_POINT('Ctrl Pts',(44.554547495243,-57.7107794649358,-41.8152360293365));
#245342=CARTESIAN_POINT('Ctrl Pts',(44.5408745509057,-57.7192473537464,
-41.812140181677));
#245343=CARTESIAN_POINT('Ctrl Pts',(44.5224181841827,-57.7300417662926,
-41.8075820007456));
#245344=CARTESIAN_POINT('Ctrl Pts',(44.494403164631,-57.7454824222945,-41.8000999642091));
#245345=CARTESIAN_POINT('Ctrl Pts',(44.4557509611988,-57.7631175354143,
-41.7875858630695));
#245346=CARTESIAN_POINT('Ctrl Pts',(44.4257963579031,-57.7741479888816,
-41.7763064650726));
#245347=CARTESIAN_POINT('Ctrl Pts',(44.4056101875344,-57.781009218212,-41.7683613570464));
#245348=CARTESIAN_POINT('Ctrl Pts',(44.3954036594654,-57.7841949818065,
-41.7641737395871));
#245349=CARTESIAN_POINT('Ctrl Pts',(44.3747925009816,-57.7900627169564,
-41.7553761870634));
#245350=CARTESIAN_POINT('Ctrl Pts',(44.3643365899562,-57.7927558542442,
-41.7507422904685));
#245351=CARTESIAN_POINT('Ctrl Pts',(44.3329536886806,-57.7999988857253,
-41.7363257213199));
#245352=CARTESIAN_POINT('Ctrl Pts',(44.3014645871824,-57.8056090798854,
-41.7208580810542));
#245353=CARTESIAN_POINT('Ctrl Pts',(44.2698183189435,-57.8088603667088,
-41.7038603653999));
#245354=CARTESIAN_POINT('Ctrl Pts',(44.2381206623806,-57.8113308880715,
-41.6863549522799));
#245355=CARTESIAN_POINT('Ctrl Pts',(44.2169139506954,-57.8119384373532,
-41.6740048606234));
#245356=CARTESIAN_POINT('Ctrl Pts',(44.1850197107514,-57.811287280344,-41.6544681547659));
#245357=CARTESIAN_POINT('Ctrl Pts',(44.1743613109546,-57.8108078241776,
-41.6477783242763));
#245358=CARTESIAN_POINT('Ctrl Pts',(44.1583626375358,-57.8096935003687,
-41.6374930176863));
#245359=CARTESIAN_POINT('Ctrl Pts',(44.1530230189312,-57.809255510817,-41.6340194660765));
#245360=CARTESIAN_POINT('Ctrl Pts',(44.1423341247923,-57.8082460206643,
-41.6269840076234));
#245361=CARTESIAN_POINT('Ctrl Pts',(44.1369894952372,-57.8076746784434,
-41.6234249849254));
#245362=CARTESIAN_POINT('Ctrl Pts',(44.1103928894951,-57.8045001122898,
-41.6055088472864));
#245363=CARTESIAN_POINT('Ctrl Pts',(44.0684216046586,-57.7973782151022,
-41.5759273380954));
#245364=CARTESIAN_POINT('Ctrl Pts',(44.0275807082801,-57.78632659952,-41.5445717124501));
#245365=CARTESIAN_POINT('Ctrl Pts',(43.9872978152183,-57.7733311875938,
-41.5123297976061));
#245366=CARTESIAN_POINT('Ctrl Pts',(43.9674326520914,-57.7658590768128,
-41.4957625032292));
#245367=CARTESIAN_POINT('Ctrl Pts',(43.942963744406,-57.7552890823142,-41.4744937232973));
#245368=CARTESIAN_POINT('Ctrl Pts',(43.938085174092,-57.7531113051098,-41.4702088025761));
#245369=CARTESIAN_POINT('Ctrl Pts',(43.9283699185172,-57.7486342535987,
-41.4615871928557));
#245370=CARTESIAN_POINT('Ctrl Pts',(43.9235236029976,-57.7463299238453,
-41.4572415669043));
#245371=CARTESIAN_POINT('Ctrl Pts',(43.9090930604083,-57.739254093668,-41.4441663196977));
#245372=CARTESIAN_POINT('Ctrl Pts',(43.8996324205383,-57.7343289686206,
-41.4354132012863));
#245373=CARTESIAN_POINT('Ctrl Pts',(43.8903154257419,-57.7291941381088,
-41.4266127101804));
#245374=CARTESIAN_POINT('',(44.1169604895359,-55.514043408345,-38.9933921916852));
#245375=CARTESIAN_POINT('',(42.8346996263142,-56.3799038065431,-38.9060746154351));
#245376=CARTESIAN_POINT('Ctrl Pts',(44.1169605045695,-55.5140434467185,
-38.9933921503467));
#245377=CARTESIAN_POINT('Ctrl Pts',(44.0897504669453,-55.5194672282592,
-38.9888363220206));
#245378=CARTESIAN_POINT('Ctrl Pts',(44.0626342052293,-55.5254611820674,
-38.9844176545342));
#245379=CARTESIAN_POINT('Ctrl Pts',(44.035612307405,-55.5320287845437,-38.9801370974184));
#245380=CARTESIAN_POINT('Ctrl Pts',(44.0037536535162,-55.5397719480894,
-38.9750903465021));
#245381=CARTESIAN_POINT('Ctrl Pts',(43.9720261635144,-55.5483124608923,
-38.9702355631519));
#245382=CARTESIAN_POINT('Ctrl Pts',(43.9404317247268,-55.5576620265682,
-38.9655757312954));
#245383=CARTESIAN_POINT('Ctrl Pts',(43.9088372843841,-55.5670115927043,
-38.9609158992096));
#245384=CARTESIAN_POINT('Ctrl Pts',(43.8773631496921,-55.5771759127617,
-38.9564497975263));
#245385=CARTESIAN_POINT('Ctrl Pts',(43.8460504835165,-55.5881565885239,
-38.9521869192607));
#245386=CARTESIAN_POINT('Ctrl Pts',(43.8147378173409,-55.5991372642861,
-38.9479240409952));
#245387=CARTESIAN_POINT('Ctrl Pts',(43.783451665776,-55.6109933882688,-38.943848461355));
#245388=CARTESIAN_POINT('Ctrl Pts',(43.7526711697336,-55.6235480058908,
-38.9400240897496));
#245389=CARTESIAN_POINT('Ctrl Pts',(43.7218906736911,-55.6361026235129,
-38.9361997181442));
#245390=CARTESIAN_POINT('Ctrl Pts',(43.6915050002909,-55.6493890121587,
-38.9326103047847));
#245391=CARTESIAN_POINT('Ctrl Pts',(43.661534024224,-55.6633885075075,-38.9292565988362));
#245392=CARTESIAN_POINT('Ctrl Pts',(43.6315630481571,-55.6773880028563,
-38.9259028928876));
#245393=CARTESIAN_POINT('Ctrl Pts',(43.6019980471442,-55.692103160754,-38.9227836007446));
#245394=CARTESIAN_POINT('Ctrl Pts',(43.5728356374758,-55.7075279772239,
-38.9198969730841));
#245395=CARTESIAN_POINT('Ctrl Pts',(43.5145108357497,-55.738377600849,-38.9141237195064));
#245396=CARTESIAN_POINT('Ctrl Pts',(43.4577942192328,-55.7720615501898,
-38.9092810747706));
#245397=CARTESIAN_POINT('Ctrl Pts',(43.4026941814562,-55.8085977570299,
-38.9053773125136));
#245398=CARTESIAN_POINT('Ctrl Pts',(43.3751441635105,-55.826865859825,-38.9034254314518));
#245399=CARTESIAN_POINT('Ctrl Pts',(43.3479989433793,-55.8458479689402,
-38.9017082565312));
#245400=CARTESIAN_POINT('Ctrl Pts',(43.3212654553579,-55.8655537371234,
-38.9002297378292));
#245401=CARTESIAN_POINT('Ctrl Pts',(43.2945319332195,-55.885259530455,-38.8987512172404));
#245402=CARTESIAN_POINT('Ctrl Pts',(43.2682103298005,-55.9056892736175,
-38.8975114537103));
#245403=CARTESIAN_POINT('Ctrl Pts',(43.2423046180206,-55.9268610072553,
-38.8965152565023));
#245404=CARTESIAN_POINT('Ctrl Pts',(43.2293517743067,-55.9374468641231,
-38.8960171583666));
#245405=CARTESIAN_POINT('Ctrl Pts',(43.2164877853448,-55.9482328356115,
-38.8955798454342));
#245406=CARTESIAN_POINT('Ctrl Pts',(43.2037924561014,-55.9591521490568,
-38.8952060762666));
#245407=CARTESIAN_POINT('Ctrl Pts',(43.191097126858,-55.9700714625021,-38.8948323070989));
#245408=CARTESIAN_POINT('Ctrl Pts',(43.1785604553322,-55.9811311728431,
-38.8945214616358));
#245409=CARTESIAN_POINT('Ctrl Pts',(43.1661929384724,-55.9923201879255,
-38.8942734262572));
#245410=CARTESIAN_POINT('Ctrl Pts',(43.1414579047527,-56.0146982180904,
-38.8937773555001));
#245411=CARTESIAN_POINT('Ctrl Pts',(43.117344267243,-56.0376373429098,-38.8935301407297));
#245412=CARTESIAN_POINT('Ctrl Pts',(43.0938842149535,-56.0610936119007,
-38.8935293450719));
#245413=CARTESIAN_POINT('Ctrl Pts',(43.0469641103745,-56.1080061498823,
-38.8935277537563));
#245414=CARTESIAN_POINT('Ctrl Pts',(43.0025474813891,-56.1570710705974,
-38.8945062058602));
#245415=CARTESIAN_POINT('Ctrl Pts',(42.9606448514092,-56.2082353818758,
-38.8964551997727));
#245416=CARTESIAN_POINT('Ctrl Pts',(42.9187422214293,-56.2593996931541,
-38.8984041936851));
#245417=CARTESIAN_POINT('Ctrl Pts',(42.8793334746424,-56.3126943660299,
-38.9013260136915));
#245418=CARTESIAN_POINT('Ctrl Pts',(42.8424899550942,-56.3680976795844,
-38.9052294077438));
#245419=CARTESIAN_POINT('Ctrl Pts',(42.8398779414905,-56.372025485898,-38.9055061380478));
#245420=CARTESIAN_POINT('Ctrl Pts',(42.8372783432785,-56.3759650434577,
-38.9057879244666));
#245421=CARTESIAN_POINT('Ctrl Pts',(42.8346994073709,-56.3799036571657,
-38.906073887373));
#245422=CARTESIAN_POINT('Ctrl Pts',(42.8346999571654,-56.3799040703247,
-38.9060752480495));
#245423=CARTESIAN_POINT('Ctrl Pts',(42.9101948352659,-56.2755386802039,
-38.9101094563356));
#245424=CARTESIAN_POINT('Ctrl Pts',(42.9944552171636,-56.1777247440651,
-38.9149819711245));
#245425=CARTESIAN_POINT('Ctrl Pts',(43.1750149383427,-56.0013540627946,
-38.9259216140551));
#245426=CARTESIAN_POINT('Ctrl Pts',(43.2698921661549,-55.922757935853,-38.931882518117));
#245427=CARTESIAN_POINT('Ctrl Pts',(43.3738733865066,-55.8500563343114,
-38.9385804803669));
#245428=CARTESIAN_POINT('Ctrl Pts',(43.3770600568266,-55.847840486669,-38.9387859039925));
#245429=CARTESIAN_POINT('Ctrl Pts',(43.3868444233345,-55.8410742771104,
-38.9394171105667));
#245430=CARTESIAN_POINT('Ctrl Pts',(43.393460399576,-55.8365509664054,-38.9398445749671));
#245431=CARTESIAN_POINT('Ctrl Pts',(43.4984963686718,-55.7655548257614,
-38.9466415987992));
#245432=CARTESIAN_POINT('Ctrl Pts',(43.6024979667475,-55.7065542689109,
-38.9534619752777));
#245433=CARTESIAN_POINT('Ctrl Pts',(43.8415689376835,-55.5957793032466,
-38.9708427154357));
#245434=CARTESIAN_POINT('Ctrl Pts',(43.9774091399379,-55.5482478649706,
-38.9815644662213));
#245435=CARTESIAN_POINT('Ctrl Pts',(44.1169604613867,-55.5140433046816,
-38.9933922348093));
#245436=CARTESIAN_POINT('Ctrl Pts',(46.1766977413729,-57.4754524783491,
-52.99995));
#245437=CARTESIAN_POINT('Ctrl Pts',(46.1766977413729,-56.5120019399699,
-52.9416166666667));
#245438=CARTESIAN_POINT('Ctrl Pts',(45.3423250998467,-56.0302766707802,
-52.8832833333334));
#245439=CARTESIAN_POINT('Ctrl Pts',(44.5079524583205,-55.5485514015906,
-52.82495));
#245440=CARTESIAN_POINT('Ctrl Pts',(43.6735798167943,-56.0302766707802,
-52.7666166666667));
#245441=CARTESIAN_POINT('Ctrl Pts',(42.839207175268,-56.5120019399698,-52.7082833333333));
#245442=CARTESIAN_POINT('Ctrl Pts',(42.839207175268,-57.4754524783491,-52.64995));
#245443=CARTESIAN_POINT('Ctrl Pts',(42.839207175268,-58.4389030167283,-52.5916166666666));
#245444=CARTESIAN_POINT('Ctrl Pts',(43.6735798167943,-58.920628285918,-52.5332833333334));
#245445=CARTESIAN_POINT('Ctrl Pts',(44.5079524583205,-59.4023535551075,
-52.4749500000001));
#245446=CARTESIAN_POINT('Ctrl Pts',(45.3423250998467,-58.920628285918,-52.4166166666667));
#245447=CARTESIAN_POINT('Ctrl Pts',(46.1766977413729,-58.4389030167283,
-52.3582833333334));
#245448=CARTESIAN_POINT('Ctrl Pts',(46.1766977413729,-57.4754524783491,
-52.29995));
#245449=CARTESIAN_POINT('Ctrl Pts',(46.1766977413729,-56.5120019399699,
-52.2416166666667));
#245450=CARTESIAN_POINT('Ctrl Pts',(45.3423250998467,-56.0302766707802,
-52.1832833333333));
#245451=CARTESIAN_POINT('Ctrl Pts',(44.5079524583205,-55.5485514015906,
-52.12495));
#245452=CARTESIAN_POINT('Ctrl Pts',(43.6735798167943,-56.0302766707802,
-52.0666166666667));
#245453=CARTESIAN_POINT('Ctrl Pts',(42.839207175268,-56.5120019399698,-52.0082833333333));
#245454=CARTESIAN_POINT('Ctrl Pts',(42.839207175268,-57.4754524783491,-51.94995));
#245455=CARTESIAN_POINT('Ctrl Pts',(42.839207175268,-58.4389030167283,-51.8916166666667));
#245456=CARTESIAN_POINT('Ctrl Pts',(43.6735798167943,-58.920628285918,-51.8332833333334));
#245457=CARTESIAN_POINT('Ctrl Pts',(44.5079524583205,-59.4023535551075,
-51.77495));
#245458=CARTESIAN_POINT('Ctrl Pts',(45.3423250998467,-58.920628285918,-51.7166166666667));
#245459=CARTESIAN_POINT('Ctrl Pts',(46.1766977413729,-58.4389030167283,
-51.6582833333333));
#245460=CARTESIAN_POINT('Ctrl Pts',(46.1766977413729,-57.4754524783491,
-51.59995));
#245461=CARTESIAN_POINT('Ctrl Pts',(46.1766977413729,-56.5120019399699,
-51.5416166666667));
#245462=CARTESIAN_POINT('Ctrl Pts',(45.3423250998467,-56.0302766707802,
-51.4832833333334));
#245463=CARTESIAN_POINT('Ctrl Pts',(44.5079524583205,-55.5485514015906,
-51.42495));
#245464=CARTESIAN_POINT('Ctrl Pts',(43.6735798167943,-56.0302766707802,
-51.3666166666667));
#245465=CARTESIAN_POINT('Ctrl Pts',(42.839207175268,-56.5120019399698,-51.3082833333333));
#245466=CARTESIAN_POINT('Ctrl Pts',(42.839207175268,-57.4754524783491,-51.24995));
#245467=CARTESIAN_POINT('Ctrl Pts',(42.839207175268,-58.4389030167283,-51.1916166666667));
#245468=CARTESIAN_POINT('Ctrl Pts',(43.6735798167943,-58.920628285918,-51.1332833333334));
#245469=CARTESIAN_POINT('Ctrl Pts',(44.5079524583205,-59.4023535551075,
-51.07495));
#245470=CARTESIAN_POINT('Ctrl Pts',(45.3423250998467,-58.920628285918,-51.0166166666667));
#245471=CARTESIAN_POINT('Ctrl Pts',(46.1766977413729,-58.4389030167283,
-50.9582833333334));
#245472=CARTESIAN_POINT('Ctrl Pts',(46.1766977413729,-57.4754524783491,
-50.89995));
#245473=CARTESIAN_POINT('Ctrl Pts',(46.1766977413729,-56.5120019399699,
-50.8416166666667));
#245474=CARTESIAN_POINT('Ctrl Pts',(45.3423250998467,-56.0302766707802,
-50.7832833333333));
#245475=CARTESIAN_POINT('Ctrl Pts',(44.5079524583205,-55.5485514015906,
-50.72495));
#245476=CARTESIAN_POINT('Ctrl Pts',(43.6735798167943,-56.0302766707802,
-50.6666166666667));
#245477=CARTESIAN_POINT('Ctrl Pts',(42.839207175268,-56.5120019399698,-50.6082833333334));
#245478=CARTESIAN_POINT('Ctrl Pts',(42.839207175268,-57.4754524783491,-50.54995));
#245479=CARTESIAN_POINT('Ctrl Pts',(42.839207175268,-58.4389030167283,-50.4916166666667));
#245480=CARTESIAN_POINT('Ctrl Pts',(43.6735798167943,-58.920628285918,-50.4332833333333));
#245481=CARTESIAN_POINT('Ctrl Pts',(44.5079524583205,-59.4023535551075,
-50.37495));
#245482=CARTESIAN_POINT('Ctrl Pts',(45.3423250998467,-58.920628285918,-50.3166166666667));
#245483=CARTESIAN_POINT('Ctrl Pts',(46.1766977413729,-58.4389030167283,
-50.2582833333334));
#245484=CARTESIAN_POINT('Ctrl Pts',(46.1766977413729,-57.4754524783491,
-50.19995));
#245485=CARTESIAN_POINT('Ctrl Pts',(46.1766977413729,-56.5120019399699,
-50.1416166666667));
#245486=CARTESIAN_POINT('Ctrl Pts',(45.3423250998467,-56.0302766707802,
-50.0832833333334));
#245487=CARTESIAN_POINT('Ctrl Pts',(44.5079524583205,-55.5485514015906,
-50.02495));
#245488=CARTESIAN_POINT('Ctrl Pts',(43.6735798167943,-56.0302766707802,
-49.9666166666667));
#245489=CARTESIAN_POINT('Ctrl Pts',(42.839207175268,-56.5120019399698,-49.9082833333334));
#245490=CARTESIAN_POINT('Ctrl Pts',(42.839207175268,-57.4754524783491,-49.84995));
#245491=CARTESIAN_POINT('Ctrl Pts',(42.839207175268,-58.4389030167283,-49.7916166666667));
#245492=CARTESIAN_POINT('Ctrl Pts',(43.6735798167943,-58.920628285918,-49.7332833333334));
#245493=CARTESIAN_POINT('Ctrl Pts',(44.5079524583205,-59.4023535551075,
-49.67495));
#245494=CARTESIAN_POINT('Ctrl Pts',(45.3423250998467,-58.920628285918,-49.6166166666667));
#245495=CARTESIAN_POINT('Ctrl Pts',(46.1766977413729,-58.4389030167283,
-49.5582833333334));
#245496=CARTESIAN_POINT('Ctrl Pts',(46.1766977413729,-57.4754524783491,
-49.49995));
#245497=CARTESIAN_POINT('Ctrl Pts',(46.1766977413729,-56.5120019399699,
-49.4416166666667));
#245498=CARTESIAN_POINT('Ctrl Pts',(45.3423250998467,-56.0302766707802,
-49.3832833333334));
#245499=CARTESIAN_POINT('Ctrl Pts',(44.5079524583205,-55.5485514015906,
-49.32495));
#245500=CARTESIAN_POINT('Ctrl Pts',(43.6735798167943,-56.0302766707802,
-49.2666166666667));
#245501=CARTESIAN_POINT('Ctrl Pts',(42.839207175268,-56.5120019399698,-49.2082833333334));
#245502=CARTESIAN_POINT('Ctrl Pts',(42.839207175268,-57.4754524783491,-49.14995));
#245503=CARTESIAN_POINT('Ctrl Pts',(42.839207175268,-58.4389030167283,-49.0916166666667));
#245504=CARTESIAN_POINT('Ctrl Pts',(43.6735798167943,-58.920628285918,-49.0332833333333));
#245505=CARTESIAN_POINT('Ctrl Pts',(44.5079524583205,-59.4023535551075,
-48.97495));
#245506=CARTESIAN_POINT('Ctrl Pts',(45.3423250998467,-58.920628285918,-48.9166166666667));
#245507=CARTESIAN_POINT('Ctrl Pts',(46.1766977413729,-58.4389030167283,
-48.8582833333333));
#245508=CARTESIAN_POINT('Ctrl Pts',(46.1766977413729,-57.4754524783491,
-48.79995));
#245509=CARTESIAN_POINT('Ctrl Pts',(46.1766977413729,-56.5120019399699,
-48.7416166666667));
#245510=CARTESIAN_POINT('Ctrl Pts',(45.3423250998467,-56.0302766707802,
-48.6832833333334));
#245511=CARTESIAN_POINT('Ctrl Pts',(44.5079524583205,-55.5485514015906,
-48.62495));
#245512=CARTESIAN_POINT('Ctrl Pts',(43.6735798167943,-56.0302766707802,
-48.5666166666667));
#245513=CARTESIAN_POINT('Ctrl Pts',(42.839207175268,-56.5120019399698,-48.5082833333334));
#245514=CARTESIAN_POINT('Ctrl Pts',(42.839207175268,-57.4754524783491,-48.44995));
#245515=CARTESIAN_POINT('Ctrl Pts',(42.839207175268,-58.4389030167283,-48.3916166666667));
#245516=CARTESIAN_POINT('Ctrl Pts',(43.6735798167943,-58.920628285918,-48.3332833333334));
#245517=CARTESIAN_POINT('Ctrl Pts',(44.5079524583205,-59.4023535551075,
-48.27495));
#245518=CARTESIAN_POINT('Ctrl Pts',(45.3423250998467,-58.920628285918,-48.2166166666667));
#245519=CARTESIAN_POINT('Ctrl Pts',(46.1766977413729,-58.4389030167283,
-48.1582833333334));
#245520=CARTESIAN_POINT('Ctrl Pts',(46.1766977413729,-57.4754524783491,
-48.09995));
#245521=CARTESIAN_POINT('Ctrl Pts',(46.1766977413729,-56.5120019399699,
-48.0416166666667));
#245522=CARTESIAN_POINT('Ctrl Pts',(45.3423250998467,-56.0302766707802,
-47.9832833333334));
#245523=CARTESIAN_POINT('Ctrl Pts',(44.5079524583205,-55.5485514015906,
-47.92495));
#245524=CARTESIAN_POINT('Ctrl Pts',(43.6735798167943,-56.0302766707802,
-47.8666166666667));
#245525=CARTESIAN_POINT('Ctrl Pts',(42.839207175268,-56.5120019399698,-47.8082833333333));
#245526=CARTESIAN_POINT('Ctrl Pts',(42.839207175268,-57.4754524783491,-47.74995));
#245527=CARTESIAN_POINT('Ctrl Pts',(42.839207175268,-58.4389030167283,-47.6916166666667));
#245528=CARTESIAN_POINT('Ctrl Pts',(43.6735798167943,-58.920628285918,-47.6332833333333));
#245529=CARTESIAN_POINT('Ctrl Pts',(44.5079524583205,-59.4023535551075,
-47.57495));
#245530=CARTESIAN_POINT('Ctrl Pts',(45.3423250998467,-58.920628285918,-47.5166166666667));
#245531=CARTESIAN_POINT('Ctrl Pts',(46.1766977413729,-58.4389030167283,
-47.4582833333333));
#245532=CARTESIAN_POINT('Ctrl Pts',(46.1766977413729,-57.4754524783491,
-47.39995));
#245533=CARTESIAN_POINT('Ctrl Pts',(46.1766977413729,-56.5120019399699,
-47.3416166666666));
#245534=CARTESIAN_POINT('Ctrl Pts',(45.3423250998467,-56.0302766707802,
-47.2832833333333));
#245535=CARTESIAN_POINT('Ctrl Pts',(44.5079524583205,-55.5485514015906,
-47.22495));
#245536=CARTESIAN_POINT('Ctrl Pts',(43.6735798167943,-56.0302766707802,
-47.1666166666667));
#245537=CARTESIAN_POINT('Ctrl Pts',(42.839207175268,-56.5120019399698,-47.1082833333333));
#245538=CARTESIAN_POINT('Ctrl Pts',(42.839207175268,-57.4754524783491,-47.04995));
#245539=CARTESIAN_POINT('Ctrl Pts',(42.839207175268,-58.4389030167283,-46.9916166666667));
#245540=CARTESIAN_POINT('Ctrl Pts',(43.6735798167943,-58.920628285918,-46.9332833333334));
#245541=CARTESIAN_POINT('Ctrl Pts',(44.5079524583205,-59.4023535551075,
-46.87495));
#245542=CARTESIAN_POINT('Ctrl Pts',(45.3423250998467,-58.920628285918,-46.8166166666667));
#245543=CARTESIAN_POINT('Ctrl Pts',(46.1766977413729,-58.4389030167283,
-46.7582833333333));
#245544=CARTESIAN_POINT('Ctrl Pts',(46.1766977413729,-57.4754524783491,
-46.69995));
#245545=CARTESIAN_POINT('Ctrl Pts',(46.1766977413729,-56.5120019399699,
-46.6416166666666));
#245546=CARTESIAN_POINT('Ctrl Pts',(45.3423250998467,-56.0302766707802,
-46.5832833333334));
#245547=CARTESIAN_POINT('Ctrl Pts',(44.5079524583205,-55.5485514015906,
-46.52495));
#245548=CARTESIAN_POINT('Ctrl Pts',(43.6735798167943,-56.0302766707802,
-46.4666166666667));
#245549=CARTESIAN_POINT('Ctrl Pts',(42.839207175268,-56.5120019399698,-46.4082833333333));
#245550=CARTESIAN_POINT('Ctrl Pts',(42.839207175268,-57.4754524783491,-46.34995));
#245551=CARTESIAN_POINT('Ctrl Pts',(42.839207175268,-58.4389030167283,-46.2916166666667));
#245552=CARTESIAN_POINT('Ctrl Pts',(43.6735798167943,-58.920628285918,-46.2332833333334));
#245553=CARTESIAN_POINT('Ctrl Pts',(44.5079524583205,-59.4023535551075,
-46.17495));
#245554=CARTESIAN_POINT('Ctrl Pts',(45.3423250998467,-58.920628285918,-46.1166166666667));
#245555=CARTESIAN_POINT('Ctrl Pts',(46.1766977413729,-58.4389030167283,
-46.0582833333333));
#245556=CARTESIAN_POINT('Ctrl Pts',(46.1766977413729,-57.4754524783491,
-45.99995));
#245557=CARTESIAN_POINT('Ctrl Pts',(46.1766977413729,-56.5120019399699,
-45.9416166666667));
#245558=CARTESIAN_POINT('Ctrl Pts',(45.3423250998467,-56.0302766707802,
-45.8832833333333));
#245559=CARTESIAN_POINT('Ctrl Pts',(44.5079524583205,-55.5485514015906,
-45.82495));
#245560=CARTESIAN_POINT('Ctrl Pts',(43.6735798167943,-56.0302766707802,
-45.7666166666667));
#245561=CARTESIAN_POINT('Ctrl Pts',(42.839207175268,-56.5120019399698,-45.7082833333333));
#245562=CARTESIAN_POINT('Ctrl Pts',(42.839207175268,-57.4754524783491,-45.64995));
#245563=CARTESIAN_POINT('Ctrl Pts',(42.839207175268,-58.4389030167283,-45.5916166666667));
#245564=CARTESIAN_POINT('Ctrl Pts',(43.6735798167943,-58.920628285918,-45.5332833333333));
#245565=CARTESIAN_POINT('Ctrl Pts',(44.5079524583205,-59.4023535551075,
-45.47495));
#245566=CARTESIAN_POINT('Ctrl Pts',(45.3423250998467,-58.920628285918,-45.4166166666667));
#245567=CARTESIAN_POINT('Ctrl Pts',(46.1766977413729,-58.4389030167283,
-45.3582833333333));
#245568=CARTESIAN_POINT('Ctrl Pts',(46.1766977413729,-57.4754524783491,
-45.29995));
#245569=CARTESIAN_POINT('Ctrl Pts',(46.1766977413729,-56.5120019399699,
-45.2416166666667));
#245570=CARTESIAN_POINT('Ctrl Pts',(45.3423250998467,-56.0302766707802,
-45.1832833333334));
#245571=CARTESIAN_POINT('Ctrl Pts',(44.5079524583205,-55.5485514015906,
-45.12495));
#245572=CARTESIAN_POINT('Ctrl Pts',(43.6735798167943,-56.0302766707802,
-45.0666166666667));
#245573=CARTESIAN_POINT('Ctrl Pts',(42.839207175268,-56.5120019399698,-45.0082833333334));
#245574=CARTESIAN_POINT('Ctrl Pts',(42.839207175268,-57.4754524783491,-44.94995));
#245575=CARTESIAN_POINT('Ctrl Pts',(42.839207175268,-58.4389030167283,-44.8916166666667));
#245576=CARTESIAN_POINT('Ctrl Pts',(43.6735798167943,-58.920628285918,-44.8332833333334));
#245577=CARTESIAN_POINT('Ctrl Pts',(44.5079524583205,-59.4023535551075,
-44.77495));
#245578=CARTESIAN_POINT('Ctrl Pts',(45.3423250998467,-58.920628285918,-44.7166166666667));
#245579=CARTESIAN_POINT('Ctrl Pts',(46.1766977413729,-58.4389030167283,
-44.6582833333334));
#245580=CARTESIAN_POINT('Ctrl Pts',(46.1766977413729,-57.4754524783491,
-44.59995));
#245581=CARTESIAN_POINT('Ctrl Pts',(46.1766977413729,-56.5120019399699,
-44.5416166666667));
#245582=CARTESIAN_POINT('Ctrl Pts',(45.3423250998467,-56.0302766707802,
-44.4832833333334));
#245583=CARTESIAN_POINT('Ctrl Pts',(44.5079524583205,-55.5485514015906,
-44.42495));
#245584=CARTESIAN_POINT('Ctrl Pts',(43.6735798167943,-56.0302766707802,
-44.3666166666667));
#245585=CARTESIAN_POINT('Ctrl Pts',(42.839207175268,-56.5120019399698,-44.3082833333334));
#245586=CARTESIAN_POINT('Ctrl Pts',(42.839207175268,-57.4754524783491,-44.24995));
#245587=CARTESIAN_POINT('Ctrl Pts',(42.839207175268,-58.4389030167283,-44.1916166666667));
#245588=CARTESIAN_POINT('Ctrl Pts',(43.6735798167943,-58.920628285918,-44.1332833333334));
#245589=CARTESIAN_POINT('Ctrl Pts',(44.5079524583205,-59.4023535551075,
-44.07495));
#245590=CARTESIAN_POINT('Ctrl Pts',(45.3423250998467,-58.920628285918,-44.0166166666667));
#245591=CARTESIAN_POINT('Ctrl Pts',(46.1766977413729,-58.4389030167283,
-43.9582833333334));
#245592=CARTESIAN_POINT('Ctrl Pts',(46.1766977413729,-57.4754524783491,
-43.89995));
#245593=CARTESIAN_POINT('Ctrl Pts',(46.1766977413729,-56.5120019399699,
-43.8416166666667));
#245594=CARTESIAN_POINT('Ctrl Pts',(45.3423250998467,-56.0302766707802,
-43.7832833333334));
#245595=CARTESIAN_POINT('Ctrl Pts',(44.5079524583205,-55.5485514015906,
-43.72495));
#245596=CARTESIAN_POINT('Ctrl Pts',(43.6735798167943,-56.0302766707802,
-43.6666166666667));
#245597=CARTESIAN_POINT('Ctrl Pts',(42.839207175268,-56.5120019399698,-43.6082833333333));
#245598=CARTESIAN_POINT('Ctrl Pts',(42.839207175268,-57.4754524783491,-43.54995));
#245599=CARTESIAN_POINT('Ctrl Pts',(42.839207175268,-58.4389030167283,-43.4916166666667));
#245600=CARTESIAN_POINT('Ctrl Pts',(43.6735798167943,-58.920628285918,-43.4332833333333));
#245601=CARTESIAN_POINT('Ctrl Pts',(44.5079524583205,-59.4023535551075,
-43.37495));
#245602=CARTESIAN_POINT('Ctrl Pts',(45.3423250998467,-58.920628285918,-43.3166166666667));
#245603=CARTESIAN_POINT('Ctrl Pts',(46.1766977413729,-58.4389030167283,
-43.2582833333333));
#245604=CARTESIAN_POINT('Ctrl Pts',(46.1766977413729,-57.4754524783491,
-43.19995));
#245605=CARTESIAN_POINT('Ctrl Pts',(46.1766977413729,-56.5120019399699,
-43.1416166666667));
#245606=CARTESIAN_POINT('Ctrl Pts',(45.3423250998467,-56.0302766707802,
-43.0832833333333));
#245607=CARTESIAN_POINT('Ctrl Pts',(44.5079524583205,-55.5485514015906,
-43.02495));
#245608=CARTESIAN_POINT('Ctrl Pts',(43.6735798167943,-56.0302766707802,
-42.9666166666667));
#245609=CARTESIAN_POINT('Ctrl Pts',(42.839207175268,-56.5120019399698,-42.9082833333333));
#245610=CARTESIAN_POINT('Ctrl Pts',(42.839207175268,-57.4754524783491,-42.84995));
#245611=CARTESIAN_POINT('Ctrl Pts',(42.839207175268,-58.4389030167283,-42.7916166666667));
#245612=CARTESIAN_POINT('Ctrl Pts',(43.6735798167943,-58.920628285918,-42.7332833333334));
#245613=CARTESIAN_POINT('Ctrl Pts',(44.5079524583205,-59.4023535551075,
-42.67495));
#245614=CARTESIAN_POINT('Ctrl Pts',(45.3423250998467,-58.920628285918,-42.6166166666667));
#245615=CARTESIAN_POINT('Ctrl Pts',(46.1766977413729,-58.4389030167283,
-42.5582833333333));
#245616=CARTESIAN_POINT('Ctrl Pts',(46.1766977413729,-57.4754524783491,
-42.49995));
#245617=CARTESIAN_POINT('Ctrl Pts',(46.1766977413729,-56.5120019399699,
-42.4416166666667));
#245618=CARTESIAN_POINT('Ctrl Pts',(45.3423250998467,-56.0302766707802,
-42.3832833333333));
#245619=CARTESIAN_POINT('Ctrl Pts',(44.5079524583205,-55.5485514015906,
-42.32495));
#245620=CARTESIAN_POINT('Ctrl Pts',(43.6735798167943,-56.0302766707802,
-42.2666166666667));
#245621=CARTESIAN_POINT('Ctrl Pts',(42.839207175268,-56.5120019399698,-42.2082833333333));
#245622=CARTESIAN_POINT('Ctrl Pts',(42.839207175268,-57.4754524783491,-42.14995));
#245623=CARTESIAN_POINT('Ctrl Pts',(42.839207175268,-58.4389030167283,-42.0916166666667));
#245624=CARTESIAN_POINT('Ctrl Pts',(43.6735798167943,-58.920628285918,-42.0332833333334));
#245625=CARTESIAN_POINT('Ctrl Pts',(44.5079524583205,-59.4023535551075,
-41.97495));
#245626=CARTESIAN_POINT('Ctrl Pts',(45.3423250998467,-58.920628285918,-41.9166166666667));
#245627=CARTESIAN_POINT('Ctrl Pts',(46.1766977413729,-58.4389030167283,
-41.8582833333333));
#245628=CARTESIAN_POINT('Ctrl Pts',(46.1766977413729,-57.4754524783491,
-41.79995));
#245629=CARTESIAN_POINT('Ctrl Pts',(46.1766977413729,-56.5120019399699,
-41.7416166666667));
#245630=CARTESIAN_POINT('Ctrl Pts',(45.3423250998467,-56.0302766707802,
-41.6832833333333));
#245631=CARTESIAN_POINT('Ctrl Pts',(44.5079524583205,-55.5485514015906,
-41.62495));
#245632=CARTESIAN_POINT('Ctrl Pts',(43.6735798167943,-56.0302766707802,
-41.5666166666667));
#245633=CARTESIAN_POINT('Ctrl Pts',(42.839207175268,-56.5120019399698,-41.5082833333334));
#245634=CARTESIAN_POINT('Ctrl Pts',(42.839207175268,-57.4754524783491,-41.44995));
#245635=CARTESIAN_POINT('Ctrl Pts',(42.839207175268,-58.4389030167283,-41.3916166666667));
#245636=CARTESIAN_POINT('Ctrl Pts',(43.6735798167943,-58.920628285918,-41.3332833333334));
#245637=CARTESIAN_POINT('Ctrl Pts',(44.5079524583205,-59.4023535551075,
-41.27495));
#245638=CARTESIAN_POINT('Ctrl Pts',(45.3423250998467,-58.920628285918,-41.2166166666667));
#245639=CARTESIAN_POINT('Ctrl Pts',(46.1766977413729,-58.4389030167283,
-41.1582833333333));
#245640=CARTESIAN_POINT('Ctrl Pts',(46.1766977413729,-57.4754524783491,
-41.09995));
#245641=CARTESIAN_POINT('Ctrl Pts',(46.1766977413729,-56.5120019399699,
-41.0416166666667));
#245642=CARTESIAN_POINT('Ctrl Pts',(45.3423250998467,-56.0302766707802,
-40.9832833333333));
#245643=CARTESIAN_POINT('Ctrl Pts',(44.5079524583205,-55.5485514015906,
-40.92495));
#245644=CARTESIAN_POINT('Ctrl Pts',(43.6735798167943,-56.0302766707802,
-40.8666166666667));
#245645=CARTESIAN_POINT('Ctrl Pts',(42.839207175268,-56.5120019399698,-40.8082833333334));
#245646=CARTESIAN_POINT('Ctrl Pts',(42.839207175268,-57.4754524783491,-40.74995));
#245647=CARTESIAN_POINT('Ctrl Pts',(42.839207175268,-58.4389030167283,-40.6916166666667));
#245648=CARTESIAN_POINT('Ctrl Pts',(43.6735798167943,-58.920628285918,-40.6332833333334));
#245649=CARTESIAN_POINT('Ctrl Pts',(44.5079524583205,-59.4023535551075,
-40.57495));
#245650=CARTESIAN_POINT('Ctrl Pts',(45.3423250998467,-58.920628285918,-40.5166166666667));
#245651=CARTESIAN_POINT('Ctrl Pts',(46.1766977413729,-58.4389030167283,
-40.4582833333333));
#245652=CARTESIAN_POINT('Ctrl Pts',(46.1766977413729,-57.4754524783491,
-40.39995));
#245653=CARTESIAN_POINT('Ctrl Pts',(46.1766977413729,-56.5120019399699,
-40.3416166666667));
#245654=CARTESIAN_POINT('Ctrl Pts',(45.3423250998467,-56.0302766707802,
-40.2832833333334));
#245655=CARTESIAN_POINT('Ctrl Pts',(44.5079524583205,-55.5485514015906,
-40.22495));
#245656=CARTESIAN_POINT('Ctrl Pts',(43.6735798167943,-56.0302766707802,
-40.1666166666667));
#245657=CARTESIAN_POINT('Ctrl Pts',(42.839207175268,-56.5120019399698,-40.1082833333334));
#245658=CARTESIAN_POINT('Ctrl Pts',(42.839207175268,-57.4754524783491,-40.04995));
#245659=CARTESIAN_POINT('Ctrl Pts',(42.839207175268,-58.4389030167283,-39.9916166666667));
#245660=CARTESIAN_POINT('Ctrl Pts',(43.6735798167943,-58.920628285918,-39.9332833333333));
#245661=CARTESIAN_POINT('Ctrl Pts',(44.5079524583205,-59.4023535551075,
-39.87495));
#245662=CARTESIAN_POINT('Ctrl Pts',(45.3423250998467,-58.920628285918,-39.8166166666667));
#245663=CARTESIAN_POINT('Ctrl Pts',(46.1766977413729,-58.4389030167283,
-39.7582833333334));
#245664=CARTESIAN_POINT('Ctrl Pts',(46.1766977413729,-57.4754524783491,
-39.69995));
#245665=CARTESIAN_POINT('Ctrl Pts',(46.1766977413729,-56.5120019399699,
-39.6416166666667));
#245666=CARTESIAN_POINT('Ctrl Pts',(45.3423250998467,-56.0302766707802,
-39.5832833333333));
#245667=CARTESIAN_POINT('Ctrl Pts',(44.5079524583205,-55.5485514015906,
-39.52495));
#245668=CARTESIAN_POINT('Ctrl Pts',(43.6735798167943,-56.0302766707802,
-39.4666166666667));
#245669=CARTESIAN_POINT('Ctrl Pts',(42.839207175268,-56.5120019399698,-39.4082833333334));
#245670=CARTESIAN_POINT('Ctrl Pts',(42.839207175268,-57.4754524783491,-39.34995));
#245671=CARTESIAN_POINT('Ctrl Pts',(42.839207175268,-58.4389030167283,-39.2916166666667));
#245672=CARTESIAN_POINT('Ctrl Pts',(43.6735798167943,-58.920628285918,-39.2332833333333));
#245673=CARTESIAN_POINT('Ctrl Pts',(44.5079524583205,-59.4023535551075,
-39.17495));
#245674=CARTESIAN_POINT('Ctrl Pts',(45.3423250998467,-58.920628285918,-39.1166166666667));
#245675=CARTESIAN_POINT('Ctrl Pts',(46.1766977413729,-58.4389030167283,
-39.0582833333334));
#245676=CARTESIAN_POINT('Ctrl Pts',(46.1766977413729,-57.4754524783491,
-38.99995));
#245677=CARTESIAN_POINT('Ctrl Pts',(46.1766977413729,-56.5120019399699,
-38.9416166666667));
#245678=CARTESIAN_POINT('Ctrl Pts',(45.3423250998467,-56.0302766707802,
-38.8832833333334));
#245679=CARTESIAN_POINT('Ctrl Pts',(44.5079524583205,-55.5485514015906,
-38.82495));
#245680=CARTESIAN_POINT('Ctrl Pts',(43.6735798167943,-56.0302766707802,
-38.7666166666667));
#245681=CARTESIAN_POINT('Ctrl Pts',(42.839207175268,-56.5120019399698,-38.7082833333334));
#245682=CARTESIAN_POINT('Ctrl Pts',(42.839207175268,-57.4754524783491,-38.64995));
#245683=CARTESIAN_POINT('Ctrl Pts',(42.839207175268,-58.4389030167283,-38.5916166666667));
#245684=CARTESIAN_POINT('Ctrl Pts',(43.6735798167943,-58.920628285918,-38.5332833333334));
#245685=CARTESIAN_POINT('Ctrl Pts',(44.5079524583205,-59.4023535551075,
-38.47495));
#245686=CARTESIAN_POINT('Ctrl Pts',(45.3423250998467,-58.920628285918,-38.4166166666667));
#245687=CARTESIAN_POINT('Ctrl Pts',(46.1766977413729,-58.4389030167283,
-38.3582833333333));
#245688=CARTESIAN_POINT('Ctrl Pts',(46.1766977413729,-57.4754524783491,
-38.29995));
#245689=CARTESIAN_POINT('Ctrl Pts',(46.1766977413729,-56.5120019399699,
-38.2416166666667));
#245690=CARTESIAN_POINT('Ctrl Pts',(45.3423250998467,-56.0302766707802,
-38.1832833333333));
#245691=CARTESIAN_POINT('Ctrl Pts',(44.5079524583205,-55.5485514015906,
-38.12495));
#245692=CARTESIAN_POINT('Ctrl Pts',(43.6735798167943,-56.0302766707802,
-38.0666166666667));
#245693=CARTESIAN_POINT('Ctrl Pts',(42.839207175268,-56.5120019399698,-38.0082833333333));
#245694=CARTESIAN_POINT('Ctrl Pts',(42.839207175268,-57.4754524783491,-37.94995));
#245695=CARTESIAN_POINT('Ctrl Pts',(42.839207175268,-58.4389030167283,-37.8916166666667));
#245696=CARTESIAN_POINT('Ctrl Pts',(43.6735798167943,-58.920628285918,-37.8332833333334));
#245697=CARTESIAN_POINT('Ctrl Pts',(44.5079524583205,-59.4023535551075,
-37.77495));
#245698=CARTESIAN_POINT('Ctrl Pts',(45.3423250998467,-58.920628285918,-37.7166166666667));
#245699=CARTESIAN_POINT('Ctrl Pts',(46.1766977413729,-58.4389030167283,
-37.6582833333333));
#245700=CARTESIAN_POINT('Ctrl Pts',(46.1766977413729,-57.4754524783491,
-37.59995));
#245701=CARTESIAN_POINT('Ctrl Pts',(46.1766977413729,-56.5120019399699,
-37.5416166666667));
#245702=CARTESIAN_POINT('Ctrl Pts',(45.3423250998467,-56.0302766707802,
-37.4832833333334));
#245703=CARTESIAN_POINT('Ctrl Pts',(44.5079524583205,-55.5485514015906,
-37.42495));
#245704=CARTESIAN_POINT('Ctrl Pts',(43.6735798167943,-56.0302766707802,
-37.3666166666667));
#245705=CARTESIAN_POINT('Ctrl Pts',(42.839207175268,-56.5120019399698,-37.3082833333333));
#245706=CARTESIAN_POINT('Ctrl Pts',(42.839207175268,-57.4754524783491,-37.24995));
#245707=CARTESIAN_POINT('Ctrl Pts',(42.839207175268,-58.4389030167283,-37.1916166666667));
#245708=CARTESIAN_POINT('Ctrl Pts',(43.6735798167943,-58.920628285918,-37.1332833333334));
#245709=CARTESIAN_POINT('Ctrl Pts',(44.5079524583205,-59.4023535551075,
-37.07495));
#245710=CARTESIAN_POINT('Ctrl Pts',(45.3423250998467,-58.920628285918,-37.0166166666667));
#245711=CARTESIAN_POINT('Ctrl Pts',(45.4506530446707,-58.8580851178131,
-37.0090431559831));
#245712=CARTESIAN_POINT('Ctrl Pts',(45.5484465834733,-58.7800914304091,
-37.0009024189827));
#245713=CARTESIAN_POINT('Ctrl Pts',(46.5766932247459,-57.4754524783491,
-53.2308875));
#245714=CARTESIAN_POINT('Ctrl Pts',(46.5766932247459,-56.2810644399698,
-53.1725541666667));
#245715=CARTESIAN_POINT('Ctrl Pts',(45.5423228415332,-55.6838704207802,
-53.1142208333334));
#245716=CARTESIAN_POINT('Ctrl Pts',(44.5079524583205,-55.0866764015906,
-53.0558875000001));
#245717=CARTESIAN_POINT('Ctrl Pts',(43.4735820751078,-55.6838704207802,
-52.9975541666667));
#245718=CARTESIAN_POINT('Ctrl Pts',(42.4392116918951,-56.2810644399698,
-52.9392208333334));
#245719=CARTESIAN_POINT('Ctrl Pts',(42.439211691895,-57.4754524783491,-52.8808875));
#245720=CARTESIAN_POINT('Ctrl Pts',(42.4392116918951,-58.6698405167284,
-52.8225541666667));
#245721=CARTESIAN_POINT('Ctrl Pts',(43.4735820751078,-59.267034535918,-52.7642208333334));
#245722=CARTESIAN_POINT('Ctrl Pts',(44.5079524583205,-59.8642285551076,
-52.7058875));
#245723=CARTESIAN_POINT('Ctrl Pts',(45.5423228415332,-59.267034535918,-52.6475541666667));
#245724=CARTESIAN_POINT('Ctrl Pts',(46.5766932247459,-58.6698405167284,
-52.5892208333333));
#245725=CARTESIAN_POINT('Ctrl Pts',(46.5766932247459,-57.4754524783491,
-52.5308875));
#245726=CARTESIAN_POINT('Ctrl Pts',(46.5766932247459,-56.2810644399698,
-52.4725541666667));
#245727=CARTESIAN_POINT('Ctrl Pts',(45.5423228415332,-55.6838704207802,
-52.4142208333334));
#245728=CARTESIAN_POINT('Ctrl Pts',(44.5079524583205,-55.0866764015906,
-52.3558875000001));
#245729=CARTESIAN_POINT('Ctrl Pts',(43.4735820751078,-55.6838704207802,
-52.2975541666667));
#245730=CARTESIAN_POINT('Ctrl Pts',(42.4392116918951,-56.2810644399698,
-52.2392208333334));
#245731=CARTESIAN_POINT('Ctrl Pts',(42.439211691895,-57.4754524783491,-52.1808875));
#245732=CARTESIAN_POINT('Ctrl Pts',(42.4392116918951,-58.6698405167284,
-52.1225541666667));
#245733=CARTESIAN_POINT('Ctrl Pts',(43.4735820751078,-59.267034535918,-52.0642208333334));
#245734=CARTESIAN_POINT('Ctrl Pts',(44.5079524583205,-59.8642285551076,
-52.0058875));
#245735=CARTESIAN_POINT('Ctrl Pts',(45.5423228415332,-59.267034535918,-51.9475541666667));
#245736=CARTESIAN_POINT('Ctrl Pts',(46.5766932247459,-58.6698405167284,
-51.8892208333334));
#245737=CARTESIAN_POINT('Ctrl Pts',(46.5766932247459,-57.4754524783491,
-51.8308875));
#245738=CARTESIAN_POINT('Ctrl Pts',(46.5766932247459,-56.2810644399698,
-51.7725541666667));
#245739=CARTESIAN_POINT('Ctrl Pts',(45.5423228415332,-55.6838704207802,
-51.7142208333334));
#245740=CARTESIAN_POINT('Ctrl Pts',(44.5079524583205,-55.0866764015906,
-51.6558875));
#245741=CARTESIAN_POINT('Ctrl Pts',(43.4735820751078,-55.6838704207802,
-51.5975541666667));
#245742=CARTESIAN_POINT('Ctrl Pts',(42.4392116918951,-56.2810644399698,
-51.5392208333333));
#245743=CARTESIAN_POINT('Ctrl Pts',(42.439211691895,-57.4754524783491,-51.4808875));
#245744=CARTESIAN_POINT('Ctrl Pts',(42.4392116918951,-58.6698405167284,
-51.4225541666667));
#245745=CARTESIAN_POINT('Ctrl Pts',(43.4735820751078,-59.267034535918,-51.3642208333334));
#245746=CARTESIAN_POINT('Ctrl Pts',(44.5079524583205,-59.8642285551076,
-51.3058875));
#245747=CARTESIAN_POINT('Ctrl Pts',(45.5423228415332,-59.267034535918,-51.2475541666667));
#245748=CARTESIAN_POINT('Ctrl Pts',(46.5766932247459,-58.6698405167284,
-51.1892208333334));
#245749=CARTESIAN_POINT('Ctrl Pts',(46.5766932247459,-57.4754524783491,
-51.1308875));
#245750=CARTESIAN_POINT('Ctrl Pts',(46.5766932247459,-56.2810644399698,
-51.0725541666667));
#245751=CARTESIAN_POINT('Ctrl Pts',(45.5423228415332,-55.6838704207802,
-51.0142208333334));
#245752=CARTESIAN_POINT('Ctrl Pts',(44.5079524583205,-55.0866764015906,
-50.9558875));
#245753=CARTESIAN_POINT('Ctrl Pts',(43.4735820751078,-55.6838704207802,
-50.8975541666667));
#245754=CARTESIAN_POINT('Ctrl Pts',(42.4392116918951,-56.2810644399698,
-50.8392208333333));
#245755=CARTESIAN_POINT('Ctrl Pts',(42.439211691895,-57.4754524783491,-50.7808875));
#245756=CARTESIAN_POINT('Ctrl Pts',(42.4392116918951,-58.6698405167284,
-50.7225541666667));
#245757=CARTESIAN_POINT('Ctrl Pts',(43.4735820751078,-59.267034535918,-50.6642208333333));
#245758=CARTESIAN_POINT('Ctrl Pts',(44.5079524583205,-59.8642285551076,
-50.6058875));
#245759=CARTESIAN_POINT('Ctrl Pts',(45.5423228415332,-59.267034535918,-50.5475541666667));
#245760=CARTESIAN_POINT('Ctrl Pts',(46.5766932247459,-58.6698405167284,
-50.4892208333333));
#245761=CARTESIAN_POINT('Ctrl Pts',(46.5766932247459,-57.4754524783491,
-50.4308875));
#245762=CARTESIAN_POINT('Ctrl Pts',(46.5766932247459,-56.2810644399698,
-50.3725541666667));
#245763=CARTESIAN_POINT('Ctrl Pts',(45.5423228415332,-55.6838704207802,
-50.3142208333334));
#245764=CARTESIAN_POINT('Ctrl Pts',(44.5079524583205,-55.0866764015906,
-50.2558875));
#245765=CARTESIAN_POINT('Ctrl Pts',(43.4735820751078,-55.6838704207802,
-50.1975541666667));
#245766=CARTESIAN_POINT('Ctrl Pts',(42.4392116918951,-56.2810644399698,
-50.1392208333333));
#245767=CARTESIAN_POINT('Ctrl Pts',(42.439211691895,-57.4754524783491,-50.0808875));
#245768=CARTESIAN_POINT('Ctrl Pts',(42.4392116918951,-58.6698405167284,
-50.0225541666667));
#245769=CARTESIAN_POINT('Ctrl Pts',(43.4735820751078,-59.267034535918,-49.9642208333334));
#245770=CARTESIAN_POINT('Ctrl Pts',(44.5079524583205,-59.8642285551076,
-49.9058875));
#245771=CARTESIAN_POINT('Ctrl Pts',(45.5423228415332,-59.267034535918,-49.8475541666667));
#245772=CARTESIAN_POINT('Ctrl Pts',(46.5766932247459,-58.6698405167284,
-49.7892208333333));
#245773=CARTESIAN_POINT('Ctrl Pts',(46.5766932247459,-57.4754524783491,
-49.7308875));
#245774=CARTESIAN_POINT('Ctrl Pts',(46.5766932247459,-56.2810644399698,
-49.6725541666667));
#245775=CARTESIAN_POINT('Ctrl Pts',(45.5423228415332,-55.6838704207802,
-49.6142208333334));
#245776=CARTESIAN_POINT('Ctrl Pts',(44.5079524583205,-55.0866764015906,
-49.5558875));
#245777=CARTESIAN_POINT('Ctrl Pts',(43.4735820751078,-55.6838704207802,
-49.4975541666667));
#245778=CARTESIAN_POINT('Ctrl Pts',(42.4392116918951,-56.2810644399698,
-49.4392208333333));
#245779=CARTESIAN_POINT('Ctrl Pts',(42.439211691895,-57.4754524783491,-49.3808875));
#245780=CARTESIAN_POINT('Ctrl Pts',(42.4392116918951,-58.6698405167284,
-49.3225541666667));
#245781=CARTESIAN_POINT('Ctrl Pts',(43.4735820751078,-59.267034535918,-49.2642208333334));
#245782=CARTESIAN_POINT('Ctrl Pts',(44.5079524583205,-59.8642285551076,
-49.2058875));
#245783=CARTESIAN_POINT('Ctrl Pts',(45.5423228415332,-59.267034535918,-49.1475541666667));
#245784=CARTESIAN_POINT('Ctrl Pts',(46.5766932247459,-58.6698405167284,
-49.0892208333333));
#245785=CARTESIAN_POINT('Ctrl Pts',(46.5766932247459,-57.4754524783491,
-49.0308875));
#245786=CARTESIAN_POINT('Ctrl Pts',(46.5766932247459,-56.2810644399698,
-48.9725541666667));
#245787=CARTESIAN_POINT('Ctrl Pts',(45.5423228415332,-55.6838704207802,
-48.9142208333334));
#245788=CARTESIAN_POINT('Ctrl Pts',(44.5079524583205,-55.0866764015906,
-48.8558875));
#245789=CARTESIAN_POINT('Ctrl Pts',(43.4735820751078,-55.6838704207802,
-48.7975541666667));
#245790=CARTESIAN_POINT('Ctrl Pts',(42.4392116918951,-56.2810644399698,
-48.7392208333334));
#245791=CARTESIAN_POINT('Ctrl Pts',(42.439211691895,-57.4754524783491,-48.6808875));
#245792=CARTESIAN_POINT('Ctrl Pts',(42.4392116918951,-58.6698405167284,
-48.6225541666667));
#245793=CARTESIAN_POINT('Ctrl Pts',(43.4735820751078,-59.267034535918,-48.5642208333334));
#245794=CARTESIAN_POINT('Ctrl Pts',(44.5079524583205,-59.8642285551076,
-48.5058875));
#245795=CARTESIAN_POINT('Ctrl Pts',(45.5423228415332,-59.267034535918,-48.4475541666667));
#245796=CARTESIAN_POINT('Ctrl Pts',(46.5766932247459,-58.6698405167284,
-48.3892208333334));
#245797=CARTESIAN_POINT('Ctrl Pts',(46.5766932247459,-57.4754524783491,
-48.3308875));
#245798=CARTESIAN_POINT('Ctrl Pts',(46.5766932247459,-56.2810644399698,
-48.2725541666667));
#245799=CARTESIAN_POINT('Ctrl Pts',(45.5423228415332,-55.6838704207802,
-48.2142208333334));
#245800=CARTESIAN_POINT('Ctrl Pts',(44.5079524583205,-55.0866764015906,
-48.1558875));
#245801=CARTESIAN_POINT('Ctrl Pts',(43.4735820751078,-55.6838704207802,
-48.0975541666667));
#245802=CARTESIAN_POINT('Ctrl Pts',(42.4392116918951,-56.2810644399698,
-48.0392208333334));
#245803=CARTESIAN_POINT('Ctrl Pts',(42.439211691895,-57.4754524783491,-47.9808875));
#245804=CARTESIAN_POINT('Ctrl Pts',(42.4392116918951,-58.6698405167284,
-47.9225541666667));
#245805=CARTESIAN_POINT('Ctrl Pts',(43.4735820751078,-59.267034535918,-47.8642208333334));
#245806=CARTESIAN_POINT('Ctrl Pts',(44.5079524583205,-59.8642285551076,
-47.8058875000001));
#245807=CARTESIAN_POINT('Ctrl Pts',(45.5423228415332,-59.267034535918,-47.7475541666667));
#245808=CARTESIAN_POINT('Ctrl Pts',(46.5766932247459,-58.6698405167284,
-47.6892208333334));
#245809=CARTESIAN_POINT('Ctrl Pts',(46.5766932247459,-57.4754524783491,
-47.6308875));
#245810=CARTESIAN_POINT('Ctrl Pts',(46.5766932247459,-56.2810644399698,
-47.5725541666667));
#245811=CARTESIAN_POINT('Ctrl Pts',(45.5423228415332,-55.6838704207802,
-47.5142208333333));
#245812=CARTESIAN_POINT('Ctrl Pts',(44.5079524583205,-55.0866764015906,
-47.4558875));
#245813=CARTESIAN_POINT('Ctrl Pts',(43.4735820751078,-55.6838704207802,
-47.3975541666667));
#245814=CARTESIAN_POINT('Ctrl Pts',(42.4392116918951,-56.2810644399698,
-47.3392208333334));
#245815=CARTESIAN_POINT('Ctrl Pts',(42.439211691895,-57.4754524783491,-47.2808875));
#245816=CARTESIAN_POINT('Ctrl Pts',(42.4392116918951,-58.6698405167284,
-47.2225541666667));
#245817=CARTESIAN_POINT('Ctrl Pts',(43.4735820751078,-59.267034535918,-47.1642208333334));
#245818=CARTESIAN_POINT('Ctrl Pts',(44.5079524583205,-59.8642285551076,
-47.1058875));
#245819=CARTESIAN_POINT('Ctrl Pts',(45.5423228415332,-59.267034535918,-47.0475541666667));
#245820=CARTESIAN_POINT('Ctrl Pts',(46.5766932247459,-58.6698405167284,
-46.9892208333334));
#245821=CARTESIAN_POINT('Ctrl Pts',(46.5766932247459,-57.4754524783491,
-46.9308875));
#245822=CARTESIAN_POINT('Ctrl Pts',(46.5766932247459,-56.2810644399698,
-46.8725541666667));
#245823=CARTESIAN_POINT('Ctrl Pts',(45.5423228415332,-55.6838704207802,
-46.8142208333334));
#245824=CARTESIAN_POINT('Ctrl Pts',(44.5079524583205,-55.0866764015906,
-46.7558875));
#245825=CARTESIAN_POINT('Ctrl Pts',(43.4735820751078,-55.6838704207802,
-46.6975541666667));
#245826=CARTESIAN_POINT('Ctrl Pts',(42.4392116918951,-56.2810644399698,
-46.6392208333334));
#245827=CARTESIAN_POINT('Ctrl Pts',(42.439211691895,-57.4754524783491,-46.5808875));
#245828=CARTESIAN_POINT('Ctrl Pts',(42.4392116918951,-58.6698405167284,
-46.5225541666667));
#245829=CARTESIAN_POINT('Ctrl Pts',(43.4735820751078,-59.267034535918,-46.4642208333334));
#245830=CARTESIAN_POINT('Ctrl Pts',(44.5079524583205,-59.8642285551076,
-46.4058875));
#245831=CARTESIAN_POINT('Ctrl Pts',(45.5423228415332,-59.267034535918,-46.3475541666667));
#245832=CARTESIAN_POINT('Ctrl Pts',(46.5766932247459,-58.6698405167284,
-46.2892208333334));
#245833=CARTESIAN_POINT('Ctrl Pts',(46.5766932247459,-57.4754524783491,
-46.2308875));
#245834=CARTESIAN_POINT('Ctrl Pts',(46.5766932247459,-56.2810644399698,
-46.1725541666667));
#245835=CARTESIAN_POINT('Ctrl Pts',(45.5423228415332,-55.6838704207802,
-46.1142208333334));
#245836=CARTESIAN_POINT('Ctrl Pts',(44.5079524583205,-55.0866764015906,
-46.0558875));
#245837=CARTESIAN_POINT('Ctrl Pts',(43.4735820751078,-55.6838704207802,
-45.9975541666667));
#245838=CARTESIAN_POINT('Ctrl Pts',(42.4392116918951,-56.2810644399698,
-45.9392208333333));
#245839=CARTESIAN_POINT('Ctrl Pts',(42.439211691895,-57.4754524783491,-45.8808875));
#245840=CARTESIAN_POINT('Ctrl Pts',(42.4392116918951,-58.6698405167284,
-45.8225541666667));
#245841=CARTESIAN_POINT('Ctrl Pts',(43.4735820751078,-59.267034535918,-45.7642208333334));
#245842=CARTESIAN_POINT('Ctrl Pts',(44.5079524583205,-59.8642285551076,
-45.7058875));
#245843=CARTESIAN_POINT('Ctrl Pts',(45.5423228415332,-59.267034535918,-45.6475541666667));
#245844=CARTESIAN_POINT('Ctrl Pts',(46.5766932247459,-58.6698405167284,
-45.5892208333334));
#245845=CARTESIAN_POINT('Ctrl Pts',(46.5766932247459,-57.4754524783491,
-45.5308875));
#245846=CARTESIAN_POINT('Ctrl Pts',(46.5766932247459,-56.2810644399698,
-45.4725541666667));
#245847=CARTESIAN_POINT('Ctrl Pts',(45.5423228415332,-55.6838704207802,
-45.4142208333334));
#245848=CARTESIAN_POINT('Ctrl Pts',(44.5079524583205,-55.0866764015906,
-45.3558875));
#245849=CARTESIAN_POINT('Ctrl Pts',(43.4735820751078,-55.6838704207802,
-45.2975541666667));
#245850=CARTESIAN_POINT('Ctrl Pts',(42.4392116918951,-56.2810644399698,
-45.2392208333333));
#245851=CARTESIAN_POINT('Ctrl Pts',(42.439211691895,-57.4754524783491,-45.1808875));
#245852=CARTESIAN_POINT('Ctrl Pts',(42.4392116918951,-58.6698405167284,
-45.1225541666667));
#245853=CARTESIAN_POINT('Ctrl Pts',(43.4735820751078,-59.267034535918,-45.0642208333334));
#245854=CARTESIAN_POINT('Ctrl Pts',(44.5079524583205,-59.8642285551076,
-45.0058875));
#245855=CARTESIAN_POINT('Ctrl Pts',(45.5423228415332,-59.267034535918,-44.9475541666667));
#245856=CARTESIAN_POINT('Ctrl Pts',(46.5766932247459,-58.6698405167284,
-44.8892208333333));
#245857=CARTESIAN_POINT('Ctrl Pts',(46.5766932247459,-57.4754524783491,
-44.8308875));
#245858=CARTESIAN_POINT('Ctrl Pts',(46.5766932247459,-56.2810644399698,
-44.7725541666667));
#245859=CARTESIAN_POINT('Ctrl Pts',(45.5423228415332,-55.6838704207802,
-44.7142208333334));
#245860=CARTESIAN_POINT('Ctrl Pts',(44.5079524583205,-55.0866764015906,
-44.6558875));
#245861=CARTESIAN_POINT('Ctrl Pts',(43.4735820751078,-55.6838704207802,
-44.5975541666667));
#245862=CARTESIAN_POINT('Ctrl Pts',(42.4392116918951,-56.2810644399698,
-44.5392208333333));
#245863=CARTESIAN_POINT('Ctrl Pts',(42.439211691895,-57.4754524783491,-44.4808875000001));
#245864=CARTESIAN_POINT('Ctrl Pts',(42.4392116918951,-58.6698405167284,
-44.4225541666667));
#245865=CARTESIAN_POINT('Ctrl Pts',(43.4735820751078,-59.267034535918,-44.3642208333333));
#245866=CARTESIAN_POINT('Ctrl Pts',(44.5079524583205,-59.8642285551076,
-44.3058875));
#245867=CARTESIAN_POINT('Ctrl Pts',(45.5423228415332,-59.267034535918,-44.2475541666667));
#245868=CARTESIAN_POINT('Ctrl Pts',(46.5766932247459,-58.6698405167284,
-44.1892208333334));
#245869=CARTESIAN_POINT('Ctrl Pts',(46.5766932247459,-57.4754524783491,
-44.1308875000001));
#245870=CARTESIAN_POINT('Ctrl Pts',(46.5766932247459,-56.2810644399698,
-44.0725541666667));
#245871=CARTESIAN_POINT('Ctrl Pts',(45.5423228415332,-55.6838704207802,
-44.0142208333334));
#245872=CARTESIAN_POINT('Ctrl Pts',(44.5079524583205,-55.0866764015906,
-43.9558875));
#245873=CARTESIAN_POINT('Ctrl Pts',(43.4735820751078,-55.6838704207802,
-43.8975541666667));
#245874=CARTESIAN_POINT('Ctrl Pts',(42.4392116918951,-56.2810644399698,
-43.8392208333333));
#245875=CARTESIAN_POINT('Ctrl Pts',(42.439211691895,-57.4754524783491,-43.7808875));
#245876=CARTESIAN_POINT('Ctrl Pts',(42.4392116918951,-58.6698405167284,
-43.7225541666667));
#245877=CARTESIAN_POINT('Ctrl Pts',(43.4735820751078,-59.267034535918,-43.6642208333334));
#245878=CARTESIAN_POINT('Ctrl Pts',(44.5079524583205,-59.8642285551076,
-43.6058875));
#245879=CARTESIAN_POINT('Ctrl Pts',(45.5423228415332,-59.267034535918,-43.5475541666667));
#245880=CARTESIAN_POINT('Ctrl Pts',(46.5766932247459,-58.6698405167284,
-43.4892208333333));
#245881=CARTESIAN_POINT('Ctrl Pts',(46.5766932247459,-57.4754524783491,
-43.4308875));
#245882=CARTESIAN_POINT('Ctrl Pts',(46.5766932247459,-56.2810644399698,
-43.3725541666667));
#245883=CARTESIAN_POINT('Ctrl Pts',(45.5423228415332,-55.6838704207802,
-43.3142208333334));
#245884=CARTESIAN_POINT('Ctrl Pts',(44.5079524583205,-55.0866764015906,
-43.2558875));
#245885=CARTESIAN_POINT('Ctrl Pts',(43.4735820751078,-55.6838704207802,
-43.1975541666667));
#245886=CARTESIAN_POINT('Ctrl Pts',(42.4392116918951,-56.2810644399698,
-43.1392208333334));
#245887=CARTESIAN_POINT('Ctrl Pts',(42.439211691895,-57.4754524783491,-43.0808875));
#245888=CARTESIAN_POINT('Ctrl Pts',(42.4392116918951,-58.6698405167284,
-43.0225541666667));
#245889=CARTESIAN_POINT('Ctrl Pts',(43.4735820751078,-59.267034535918,-42.9642208333334));
#245890=CARTESIAN_POINT('Ctrl Pts',(44.5079524583205,-59.8642285551076,
-42.9058875));
#245891=CARTESIAN_POINT('Ctrl Pts',(45.5423228415332,-59.267034535918,-42.8475541666667));
#245892=CARTESIAN_POINT('Ctrl Pts',(46.5766932247459,-58.6698405167284,
-42.7892208333334));
#245893=CARTESIAN_POINT('Ctrl Pts',(46.5766932247459,-57.4754524783491,
-42.7308875000001));
#245894=CARTESIAN_POINT('Ctrl Pts',(46.5766932247459,-56.2810644399698,
-42.6725541666667));
#245895=CARTESIAN_POINT('Ctrl Pts',(45.5423228415332,-55.6838704207802,
-42.6142208333334));
#245896=CARTESIAN_POINT('Ctrl Pts',(44.5079524583205,-55.0866764015906,
-42.5558875));
#245897=CARTESIAN_POINT('Ctrl Pts',(43.4735820751078,-55.6838704207802,
-42.4975541666667));
#245898=CARTESIAN_POINT('Ctrl Pts',(42.4392116918951,-56.2810644399698,
-42.4392208333334));
#245899=CARTESIAN_POINT('Ctrl Pts',(42.439211691895,-57.4754524783491,-42.3808875000001));
#245900=CARTESIAN_POINT('Ctrl Pts',(42.4392116918951,-58.6698405167284,
-42.3225541666667));
#245901=CARTESIAN_POINT('Ctrl Pts',(43.4735820751078,-59.267034535918,-42.2642208333334));
#245902=CARTESIAN_POINT('Ctrl Pts',(44.5079524583205,-59.8642285551076,
-42.2058875));
#245903=CARTESIAN_POINT('Ctrl Pts',(45.5423228415332,-59.267034535918,-42.1475541666667));
#245904=CARTESIAN_POINT('Ctrl Pts',(46.5766932247459,-58.6698405167284,
-42.0892208333334));
#245905=CARTESIAN_POINT('Ctrl Pts',(46.5766932247459,-57.4754524783491,
-42.0308875000001));
#245906=CARTESIAN_POINT('Ctrl Pts',(46.5766932247459,-56.2810644399698,
-41.9725541666667));
#245907=CARTESIAN_POINT('Ctrl Pts',(45.5423228415332,-55.6838704207802,
-41.9142208333334));
#245908=CARTESIAN_POINT('Ctrl Pts',(44.5079524583205,-55.0866764015906,
-41.8558875));
#245909=CARTESIAN_POINT('Ctrl Pts',(43.4735820751078,-55.6838704207802,
-41.7975541666667));
#245910=CARTESIAN_POINT('Ctrl Pts',(42.4392116918951,-56.2810644399698,
-41.7392208333334));
#245911=CARTESIAN_POINT('Ctrl Pts',(42.439211691895,-57.4754524783491,-41.6808875000001));
#245912=CARTESIAN_POINT('Ctrl Pts',(42.4392116918951,-58.6698405167284,
-41.6225541666667));
#245913=CARTESIAN_POINT('Ctrl Pts',(43.4735820751078,-59.267034535918,-41.5642208333334));
#245914=CARTESIAN_POINT('Ctrl Pts',(44.5079524583205,-59.8642285551076,
-41.5058875));
#245915=CARTESIAN_POINT('Ctrl Pts',(45.5423228415332,-59.267034535918,-41.4475541666667));
#245916=CARTESIAN_POINT('Ctrl Pts',(46.5766932247459,-58.6698405167284,
-41.3892208333334));
#245917=CARTESIAN_POINT('Ctrl Pts',(46.5766932247459,-57.4754524783491,
-41.3308875000001));
#245918=CARTESIAN_POINT('Ctrl Pts',(46.5766932247459,-56.2810644399698,
-41.2725541666667));
#245919=CARTESIAN_POINT('Ctrl Pts',(45.5423228415332,-55.6838704207802,
-41.2142208333333));
#245920=CARTESIAN_POINT('Ctrl Pts',(44.5079524583205,-55.0866764015906,
-41.1558875));
#245921=CARTESIAN_POINT('Ctrl Pts',(43.4735820751078,-55.6838704207802,
-41.0975541666667));
#245922=CARTESIAN_POINT('Ctrl Pts',(42.4392116918951,-56.2810644399698,
-41.0392208333333));
#245923=CARTESIAN_POINT('Ctrl Pts',(42.439211691895,-57.4754524783491,-40.9808875000001));
#245924=CARTESIAN_POINT('Ctrl Pts',(42.4392116918951,-58.6698405167284,
-40.9225541666667));
#245925=CARTESIAN_POINT('Ctrl Pts',(43.4735820751078,-59.267034535918,-40.8642208333334));
#245926=CARTESIAN_POINT('Ctrl Pts',(44.5079524583205,-59.8642285551076,
-40.8058875));
#245927=CARTESIAN_POINT('Ctrl Pts',(45.5423228415332,-59.267034535918,-40.7475541666667));
#245928=CARTESIAN_POINT('Ctrl Pts',(46.5766932247459,-58.6698405167284,
-40.6892208333333));
#245929=CARTESIAN_POINT('Ctrl Pts',(46.5766932247459,-57.4754524783491,
-40.6308875));
#245930=CARTESIAN_POINT('Ctrl Pts',(46.5766932247459,-56.2810644399698,
-40.5725541666667));
#245931=CARTESIAN_POINT('Ctrl Pts',(45.5423228415332,-55.6838704207802,
-40.5142208333333));
#245932=CARTESIAN_POINT('Ctrl Pts',(44.5079524583205,-55.0866764015906,
-40.4558875));
#245933=CARTESIAN_POINT('Ctrl Pts',(43.4735820751078,-55.6838704207802,
-40.3975541666667));
#245934=CARTESIAN_POINT('Ctrl Pts',(42.4392116918951,-56.2810644399698,
-40.3392208333333));
#245935=CARTESIAN_POINT('Ctrl Pts',(42.439211691895,-57.4754524783491,-40.2808875));
#245936=CARTESIAN_POINT('Ctrl Pts',(42.4392116918951,-58.6698405167284,
-40.2225541666667));
#245937=CARTESIAN_POINT('Ctrl Pts',(43.4735820751078,-59.267034535918,-40.1642208333333));
#245938=CARTESIAN_POINT('Ctrl Pts',(44.5079524583205,-59.8642285551076,
-40.1058875));
#245939=CARTESIAN_POINT('Ctrl Pts',(45.5423228415332,-59.267034535918,-40.0475541666667));
#245940=CARTESIAN_POINT('Ctrl Pts',(46.5766932247459,-58.6698405167284,
-39.9892208333333));
#245941=CARTESIAN_POINT('Ctrl Pts',(46.5766932247459,-57.4754524783491,
-39.9308875));
#245942=CARTESIAN_POINT('Ctrl Pts',(46.5766932247459,-56.2810644399698,
-39.8725541666667));
#245943=CARTESIAN_POINT('Ctrl Pts',(45.5423228415332,-55.6838704207802,
-39.8142208333334));
#245944=CARTESIAN_POINT('Ctrl Pts',(44.5079524583205,-55.0866764015906,
-39.7558875));
#245945=CARTESIAN_POINT('Ctrl Pts',(43.4735820751078,-55.6838704207802,
-39.6975541666667));
#245946=CARTESIAN_POINT('Ctrl Pts',(42.4392116918951,-56.2810644399698,
-39.6392208333334));
#245947=CARTESIAN_POINT('Ctrl Pts',(42.439211691895,-57.4754524783491,-39.5808875000001));
#245948=CARTESIAN_POINT('Ctrl Pts',(42.4392116918951,-58.6698405167284,
-39.5225541666667));
#245949=CARTESIAN_POINT('Ctrl Pts',(43.4735820751078,-59.267034535918,-39.4642208333333));
#245950=CARTESIAN_POINT('Ctrl Pts',(44.5079524583205,-59.8642285551076,
-39.4058875));
#245951=CARTESIAN_POINT('Ctrl Pts',(45.5423228415332,-59.267034535918,-39.3475541666667));
#245952=CARTESIAN_POINT('Ctrl Pts',(46.5766932247459,-58.6698405167284,
-39.2892208333334));
#245953=CARTESIAN_POINT('Ctrl Pts',(46.5766932247459,-57.4754524783491,
-39.2308875));
#245954=CARTESIAN_POINT('Ctrl Pts',(46.5766932247459,-56.2810644399698,
-39.1725541666667));
#245955=CARTESIAN_POINT('Ctrl Pts',(45.5423228415332,-55.6838704207802,
-39.1142208333333));
#245956=CARTESIAN_POINT('Ctrl Pts',(44.5079524583205,-55.0866764015906,
-39.0558875));
#245957=CARTESIAN_POINT('Ctrl Pts',(43.4735820751078,-55.6838704207802,
-38.9975541666667));
#245958=CARTESIAN_POINT('Ctrl Pts',(42.4392116918951,-56.2810644399698,
-38.9392208333334));
#245959=CARTESIAN_POINT('Ctrl Pts',(42.439211691895,-57.4754524783491,-38.8808875));
#245960=CARTESIAN_POINT('Ctrl Pts',(42.4392116918951,-58.6698405167284,
-38.8225541666667));
#245961=CARTESIAN_POINT('Ctrl Pts',(43.4735820751078,-59.267034535918,-38.7642208333333));
#245962=CARTESIAN_POINT('Ctrl Pts',(44.5079524583205,-59.8642285551076,
-38.7058875));
#245963=CARTESIAN_POINT('Ctrl Pts',(45.5423228415332,-59.267034535918,-38.6475541666667));
#245964=CARTESIAN_POINT('Ctrl Pts',(46.5766932247459,-58.6698405167284,
-38.5892208333334));
#245965=CARTESIAN_POINT('Ctrl Pts',(46.5766932247459,-57.4754524783491,
-38.5308875));
#245966=CARTESIAN_POINT('Ctrl Pts',(46.5766932247459,-56.2810644399698,
-38.4725541666667));
#245967=CARTESIAN_POINT('Ctrl Pts',(45.5423228415332,-55.6838704207802,
-38.4142208333334));
#245968=CARTESIAN_POINT('Ctrl Pts',(44.5079524583205,-55.0866764015906,
-38.3558875));
#245969=CARTESIAN_POINT('Ctrl Pts',(43.4735820751078,-55.6838704207802,
-38.2975541666667));
#245970=CARTESIAN_POINT('Ctrl Pts',(42.4392116918951,-56.2810644399698,
-38.2392208333333));
#245971=CARTESIAN_POINT('Ctrl Pts',(42.439211691895,-57.4754524783491,-38.1808875000001));
#245972=CARTESIAN_POINT('Ctrl Pts',(42.4392116918951,-58.6698405167284,
-38.1225541666667));
#245973=CARTESIAN_POINT('Ctrl Pts',(43.4735820751078,-59.267034535918,-38.0642208333334));
#245974=CARTESIAN_POINT('Ctrl Pts',(44.5079524583205,-59.8642285551076,
-38.0058875));
#245975=CARTESIAN_POINT('Ctrl Pts',(45.5423228415332,-59.267034535918,-37.9475541666667));
#245976=CARTESIAN_POINT('Ctrl Pts',(46.5766932247459,-58.6698405167284,
-37.8892208333334));
#245977=CARTESIAN_POINT('Ctrl Pts',(46.5766932247459,-57.4754524783491,
-37.8308875));
#245978=CARTESIAN_POINT('Ctrl Pts',(46.5766932247459,-56.2810644399698,
-37.7725541666667));
#245979=CARTESIAN_POINT('Ctrl Pts',(45.5423228415332,-55.6838704207802,
-37.7142208333333));
#245980=CARTESIAN_POINT('Ctrl Pts',(44.5079524583205,-55.0866764015906,
-37.6558875));
#245981=CARTESIAN_POINT('Ctrl Pts',(43.4735820751078,-55.6838704207802,
-37.5975541666667));
#245982=CARTESIAN_POINT('Ctrl Pts',(42.4392116918951,-56.2810644399698,
-37.5392208333334));
#245983=CARTESIAN_POINT('Ctrl Pts',(42.439211691895,-57.4754524783491,-37.4808875));
#245984=CARTESIAN_POINT('Ctrl Pts',(42.4392116918951,-58.6698405167284,
-37.4225541666667));
#245985=CARTESIAN_POINT('Ctrl Pts',(43.4735820751078,-59.267034535918,-37.3642208333333));
#245986=CARTESIAN_POINT('Ctrl Pts',(44.5079524583205,-59.8642285551076,
-37.3058875));
#245987=CARTESIAN_POINT('Ctrl Pts',(45.5423228415332,-59.267034535918,-37.2475541666667));
#245988=CARTESIAN_POINT('Ctrl Pts',(45.6766168155006,-59.1894998738974,
-37.239980655983));
#245989=CARTESIAN_POINT('Ctrl Pts',(45.7978513037526,-59.0928112286649,
-37.2318399189827));
#245990=CARTESIAN_POINT('Ctrl Pts',(42.8346997657407,-56.3799037924606,
-38.9060754358215));
#245991=CARTESIAN_POINT('Ctrl Pts',(42.8657912775273,-56.3324177857128,
-38.9093809684272));
#245992=CARTESIAN_POINT('Ctrl Pts',(42.8988701072886,-56.2863150958481,
-38.9126746506026));
#245993=CARTESIAN_POINT('Ctrl Pts',(42.9337333069081,-56.2418267252429,
-38.9159388745174));
#245994=CARTESIAN_POINT('Ctrl Pts',(42.9687109169304,-56.1971923573553,
-38.9192138106209));
#245995=CARTESIAN_POINT('Ctrl Pts',(43.0054840427986,-56.1541833777436,
-38.9224590546962));
#245996=CARTESIAN_POINT('Ctrl Pts',(43.0438141464837,-56.1129927698216,
-38.9256578819596));
#245997=CARTESIAN_POINT('Ctrl Pts',(43.0824956090267,-56.0714245817847,
-38.9288860317707));
#245998=CARTESIAN_POINT('Ctrl Pts',(43.1227620598465,-56.0317085984475,
-38.9320668731519));
#245999=CARTESIAN_POINT('Ctrl Pts',(43.1643436400644,-55.9939960368214,
-38.9351848778962));
#246000=CARTESIAN_POINT('Ctrl Pts',(43.2061767575094,-55.9560553426152,
-38.9383217442196));
#246001=CARTESIAN_POINT('Ctrl Pts',(43.2493402292857,-55.9201425202975,
-38.9413949829685));
#246002=CARTESIAN_POINT('Ctrl Pts',(43.2935450408245,-55.8863604391545,
-38.944390949966));
#246003=CARTESIAN_POINT('Ctrl Pts',(43.3383073424745,-55.8521523144312,
-38.947424700678));
#246004=CARTESIAN_POINT('Ctrl Pts',(43.3841366695237,-55.8201290211542,
-38.9503791961889));
#246005=CARTESIAN_POINT('Ctrl Pts',(43.4307296615396,-55.7903439160353,
-38.953242875097));
#246006=CARTESIAN_POINT('Ctrl Pts',(43.4562577073261,-55.7740248196576,
-38.9548118691264));
#246007=CARTESIAN_POINT('Ctrl Pts',(43.4820150081877,-55.7583766645963,
-38.9563536487424));
#246008=CARTESIAN_POINT('Ctrl Pts',(43.5079524583204,-55.7434016707801,
-38.9578666666668));
#246009=CARTESIAN_POINT('Ctrl Pts',(43.5552055679399,-55.7161200752212,
-38.9606230980613));
#246010=CARTESIAN_POINT('Ctrl Pts',(43.6040973111767,-55.6904744504906,
-38.9634751033216));
#246011=CARTESIAN_POINT('Ctrl Pts',(43.6544568310304,-55.6667111967904,
-38.9664127263806));
#246012=CARTESIAN_POINT('Ctrl Pts',(43.7043813282697,-55.643153218136,-38.9693249732551));
#246013=CARTESIAN_POINT('Ctrl Pts',(43.7557481097746,-55.6214458968395,
-38.9723213509202));
#246014=CARTESIAN_POINT('Ctrl Pts',(43.8083455435853,-55.6018063857908,
-38.9753895242081));
#246015=CARTESIAN_POINT('Ctrl Pts',(43.8604147804534,-55.5823640997575,
-38.9784268861116));
#246016=CARTESIAN_POINT('Ctrl Pts',(43.9136896632225,-55.5649488835336,
-38.9815345847811));
#246017=CARTESIAN_POINT('Ctrl Pts',(43.9679253295305,-55.5497395667206,
-38.9846983459951));
#246018=CARTESIAN_POINT('Ctrl Pts',(44.0168892084326,-55.5360086181159,
-38.9875545849152));
#246019=CARTESIAN_POINT('Ctrl Pts',(44.0666354001336,-55.52407545424,-38.9904564724688));
#246020=CARTESIAN_POINT('Ctrl Pts',(44.1169605007733,-55.5140434474753,
-38.9933921501253));
#246021=CARTESIAN_POINT('Ctrl Pts',(-50.8662592829675,-43.9775643489266,
-38.2016959289287));
#246022=CARTESIAN_POINT('Ctrl Pts',(-50.9206074996482,-43.8969602231097,
-38.2028048079744));
#246023=CARTESIAN_POINT('Ctrl Pts',(-50.9634706458651,-43.817641350392,
-38.2391813181835));
#246024=CARTESIAN_POINT('Ctrl Pts',(-50.6165344156739,-43.8081147605988,
-38.1265410889715));
#246025=CARTESIAN_POINT('Ctrl Pts',(-50.6707175035488,-43.7281782205006,
-38.1277074258953));
#246026=CARTESIAN_POINT('Ctrl Pts',(-50.7134583474186,-43.6493859440548,
-38.1636515730652));
#246027=CARTESIAN_POINT('Ctrl Pts',(-50.367254897517,-43.6381237449266,
-38.0514121363637));
#246028=CARTESIAN_POINT('Ctrl Pts',(-50.4211897771984,-43.558806022001,
-38.0526121686946));
#246029=CARTESIAN_POINT('Ctrl Pts',(-50.4638460929301,-43.480574245264,
-38.0881367070155));
#246030=CARTESIAN_POINT('Ctrl Pts',(-50.1184449162637,-43.4675617326621,
-37.9763108762634));
#246031=CARTESIAN_POINT('Ctrl Pts',(-50.1720495177334,-43.3888135426178,
-37.9775209986779));
#246032=CARTESIAN_POINT('Ctrl Pts',(-50.2146583013983,-43.3111769590637,
-38.012638623582));
#246033=CARTESIAN_POINT('',(-50.1228968347622,-43.4706134770457,-37.9776546393185));
#246034=CARTESIAN_POINT('',(-50.8662598031175,-43.9775646659832,-38.2016934855357));
#246035=CARTESIAN_POINT('Origin',(-163.821120857268,123.708346813688,-40.9343427676646));
#246036=CARTESIAN_POINT('',(-50.9629628917746,-43.8185802311495,-38.2387520398483));
#246037=CARTESIAN_POINT('Origin',(-50.2413380988264,-43.5197615250917,-38.4894964491189));
#246038=CARTESIAN_POINT('Origin',(-50.7629779210076,-43.9145999846305,-38.6868437920595));
#246039=CARTESIAN_POINT('Ctrl Pts',(-52.1463598473653,-42.4957105173844,
-39.6163034956207));
#246040=CARTESIAN_POINT('Ctrl Pts',(-52.1778331585616,-42.407856341012,
-39.2820037515321));
#246041=CARTESIAN_POINT('Ctrl Pts',(-51.8651142120726,-42.3571081800691,
-39.1398680265747));
#246042=CARTESIAN_POINT('Ctrl Pts',(-52.138908792049,-42.7327637189233,
-39.5106313066209));
#246043=CARTESIAN_POINT('Ctrl Pts',(-52.1408096255332,-42.6362970896441,
-39.208392993337));
#246044=CARTESIAN_POINT('Ctrl Pts',(-51.8563466958888,-42.5839200186503,
-39.0796163834337));
#246045=CARTESIAN_POINT('Ctrl Pts',(-52.1182999697365,-42.9653720232436,
-39.3935075242519));
#246046=CARTESIAN_POINT('Ctrl Pts',(-52.0958067489885,-42.8676463321302,
-39.1251861092046));
#246047=CARTESIAN_POINT('Ctrl Pts',(-51.8388838770158,-42.8062228472946,
-39.0116982544704));
#246048=CARTESIAN_POINT('Ctrl Pts',(-52.0320114860966,-43.3497261830944,
-39.161530854536));
#246049=CARTESIAN_POINT('Ctrl Pts',(-51.9795767898205,-43.2501370823012,
-38.9567426032799));
#246050=CARTESIAN_POINT('Ctrl Pts',(-51.7752900045357,-43.1727371404884,
-38.8742643034118));
#246051=CARTESIAN_POINT('Ctrl Pts',(-51.9821559399578,-43.506114175996,
-39.0559812260102));
#246052=CARTESIAN_POINT('Ctrl Pts',(-51.9220107796067,-43.40483234188,-38.8805374882183));
#246053=CARTESIAN_POINT('Ctrl Pts',(-51.7396064271064,-43.3216378204905,
-38.8110241554243));
#246054=CARTESIAN_POINT('Ctrl Pts',(-51.8587029432334,-43.7273337947907,
-38.8735991626261));
#246055=CARTESIAN_POINT('Ctrl Pts',(-51.7966191070807,-43.6242584279089,
-38.7452143542829));
#246056=CARTESIAN_POINT('Ctrl Pts',(-51.6539357945151,-43.5318198667555,
-38.699791068918));
#246057=CARTESIAN_POINT('Ctrl Pts',(-51.8101033942497,-43.7971217698189,
-38.8100520149236));
#246058=CARTESIAN_POINT('Ctrl Pts',(-51.7496889766211,-43.6930275230314,
-38.6980706314006));
#246059=CARTESIAN_POINT('Ctrl Pts',(-51.6204903967813,-43.598045469751,
-38.6607426239999));
#246060=CARTESIAN_POINT('Ctrl Pts',(-51.6873370041662,-43.9236094312998,
-38.674885570098));
#246061=CARTESIAN_POINT('Ctrl Pts',(-51.6361098819405,-43.8172559764407,
-38.5963460304981));
#246062=CARTESIAN_POINT('Ctrl Pts',(-51.5368137528036,-43.7178768472947,
-38.5767876614047));
#246063=CARTESIAN_POINT('Ctrl Pts',(-51.6135281175597,-43.9798771251562,
-38.6036544036492));
#246064=CARTESIAN_POINT('Ctrl Pts',(-51.5698336784193,-43.8726832305444,
-38.541955894343));
#246065=CARTESIAN_POINT('Ctrl Pts',(-51.4868275908931,-43.7710708483964,
-38.5321195958186));
#246066=CARTESIAN_POINT('Ctrl Pts',(-51.4291465383277,-44.058604748282,
-38.459510380713));
#246067=CARTESIAN_POINT('Ctrl Pts',(-51.4095099680441,-43.9497005422073,
-38.4289632372181));
#246068=CARTESIAN_POINT('Ctrl Pts',(-51.3629645413757,-43.8451599264395,
-38.440265964053));
#246069=CARTESIAN_POINT('Ctrl Pts',(-51.319068965668,-44.078041978234,-38.388630302131));
#246070=CARTESIAN_POINT('Ctrl Pts',(-51.3156521245987,-43.9687081271715,
-38.3713923008305));
#246071=CARTESIAN_POINT('Ctrl Pts',(-51.2894661655026,-43.8631892410449,
-38.3942946312693));
#246072=CARTESIAN_POINT('Ctrl Pts',(-51.089300024305,-44.0616597869013,
-38.2737385514644));
#246073=CARTESIAN_POINT('Ctrl Pts',(-51.1234504711255,-43.9521135664641,
-38.2731895662586));
#246074=CARTESIAN_POINT('Ctrl Pts',(-51.1369785556538,-43.8467829646352,
-38.3177691970519));
#246075=CARTESIAN_POINT('Ctrl Pts',(-50.9704089609615,-44.0259726799371,
-38.2301338295288));
#246076=CARTESIAN_POINT('Ctrl Pts',(-51.0249939553012,-43.9165958222839,
-38.2325205502091));
#246077=CARTESIAN_POINT('Ctrl Pts',(-51.0586423830823,-43.8125622297662,
-38.2875269246531));
#246078=CARTESIAN_POINT('Ctrl Pts',(-50.8660311843248,-43.9777851953718,
-38.2016761331321));
#246079=CARTESIAN_POINT('Ctrl Pts',(-50.9393056690222,-43.8691613854929,
-38.2030936955718));
#246080=CARTESIAN_POINT('Ctrl Pts',(-50.9899108736213,-43.7663745378293,
-38.2666882799375));
#246081=CARTESIAN_POINT('',(-51.855727616252,-42.5504169941763,-39.0864710348602));
#246082=CARTESIAN_POINT('',(-52.1363779744195,-42.6975314190816,-39.5221562288903));
#246083=CARTESIAN_POINT('Origin',(-51.6375959493,-42.6626531820611,-39.5221562583896));
#246084=CARTESIAN_POINT('Ctrl Pts',(-50.8662613636147,-43.9775656172223,
-38.2016861553823));
#246085=CARTESIAN_POINT('Ctrl Pts',(-50.9078004219846,-43.9967461943322,
-38.2130183288712));
#246086=CARTESIAN_POINT('Ctrl Pts',(-50.949269083369,-44.0129893917626,
-38.2259372986406));
#246087=CARTESIAN_POINT('Ctrl Pts',(-50.9903956935496,-44.0262820941249,
-38.2403937622755));
#246088=CARTESIAN_POINT('Ctrl Pts',(-51.0314585596062,-44.0395541934843,
-38.2548278191376));
#246089=CARTESIAN_POINT('Ctrl Pts',(-51.0721796277597,-44.0498849023057,
-38.2707944285533));
#246090=CARTESIAN_POINT('Ctrl Pts',(-51.1123002988897,-44.0572683454116,
-38.2881944319024));
#246091=CARTESIAN_POINT('Ctrl Pts',(-51.1298439799964,-44.0604969247866,
-38.2958029813462));
#246092=CARTESIAN_POINT('Ctrl Pts',(-51.1472730853109,-44.0631620602905,
-38.3036849773209));
#246093=CARTESIAN_POINT('Ctrl Pts',(-51.1645672900365,-44.0652637097802,
-38.3118293100208));
#246094=CARTESIAN_POINT('Ctrl Pts',(-51.2041865851273,-44.0700783787768,
-38.3304871625023));
#246095=CARTESIAN_POINT('Ctrl Pts',(-51.2430955061505,-44.0719352464437,
-38.3505244284462));
#246096=CARTESIAN_POINT('Ctrl Pts',(-51.2810711000578,-44.0708391843286,
-38.3717770661348));
#246097=CARTESIAN_POINT('Ctrl Pts',(-51.2893225981018,-44.0706010273055,
-38.3763949293537));
#246098=CARTESIAN_POINT('Ctrl Pts',(-51.2975301585805,-44.0702234828254,
-38.381070026873));
#246099=CARTESIAN_POINT('Ctrl Pts',(-51.3056917160415,-44.0697066461471,
-38.385800442706));
#246100=CARTESIAN_POINT('Ctrl Pts',(-51.3285533264544,-44.0682589177148,
-38.3990509680356));
#246101=CARTESIAN_POINT('Ctrl Pts',(-51.3510535722672,-44.0657181870734,
-38.412735840956));
#246102=CARTESIAN_POINT('Ctrl Pts',(-51.373150782787,-44.0620871882793,
-38.4268099888037));
#246103=CARTESIAN_POINT('Ctrl Pts',(-51.3841993880469,-44.0602716888823,
-38.4338470627276));
#246104=CARTESIAN_POINT('Ctrl Pts',(-51.3951472928094,-44.058183636393,
-38.4409813696671));
#246105=CARTESIAN_POINT('Ctrl Pts',(-51.4059898777672,-44.0558234574321,
-38.4482069490058));
#246106=CARTESIAN_POINT('Ctrl Pts',(-51.4126979836034,-44.054363258566,
-38.4526772806766));
#246107=CARTESIAN_POINT('Ctrl Pts',(-51.4197316537442,-44.05270078671,-38.4574288435828));
#246108=CARTESIAN_POINT('Ctrl Pts',(-51.4264092843737,-44.0510178394573,
-38.462005765729));
#246109=CARTESIAN_POINT('Ctrl Pts',(-51.4305249803831,-44.0499805704503,
-38.4648267094525));
#246110=CARTESIAN_POINT('Ctrl Pts',(-51.4345059407379,-44.04893567481,-38.4675802974087));
#246111=CARTESIAN_POINT('Ctrl Pts',(-51.4381973259372,-44.047927018598,
-38.470151265276));
#246112=CARTESIAN_POINT('Ctrl Pts',(-51.4751679454563,-44.0378249449793,
-38.4959004812708));
#246113=CARTESIAN_POINT('Ctrl Pts',(-51.5113692337529,-44.0243189447717,
-38.523077931443));
#246114=CARTESIAN_POINT('Ctrl Pts',(-51.5465460185733,-44.0074090900157,
-38.5515565059206));
#246115=CARTESIAN_POINT('Ctrl Pts',(-51.5815815540112,-43.9905671353408,
-38.5799207271087));
#246116=CARTESIAN_POINT('Ctrl Pts',(-51.6156000740549,-43.9703486034704,
-38.6095753079235));
#246117=CARTESIAN_POINT('Ctrl Pts',(-51.6483730590436,-43.9467609115004,
-38.6403493423971));
#246118=CARTESIAN_POINT('Ctrl Pts',(-51.6810670486091,-43.9232300748858,
-38.6710491996824));
#246119=CARTESIAN_POINT('Ctrl Pts',(-51.7125208832909,-43.8963463259735,
-38.7028626106144));
#246120=CARTESIAN_POINT('Ctrl Pts',(-51.7425412958989,-43.8661241919007,
-38.7355810510177));
#246121=CARTESIAN_POINT('Ctrl Pts',(-51.7471512174186,-43.8614832941205,
-38.7406052805137));
#246122=CARTESIAN_POINT('Ctrl Pts',(-51.7517274126434,-43.8567636886518,
-38.7456507856083));
#246123=CARTESIAN_POINT('Ctrl Pts',(-51.7562692654992,-43.8519654422891,
-38.7507167429485));
#246124=CARTESIAN_POINT('Ctrl Pts',(-51.7718585546465,-43.8354961174734,
-38.7681049491038));
#246125=CARTESIAN_POINT('Ctrl Pts',(-51.7870429900321,-43.8181002779942,
-38.785734261531));
#246126=CARTESIAN_POINT('Ctrl Pts',(-51.8017998436459,-43.7997809435826,
-38.8035700068467));
#246127=CARTESIAN_POINT('Ctrl Pts',(-51.8091782704528,-43.7906212763769,
-38.8124878795046));
#246128=CARTESIAN_POINT('Ctrl Pts',(-51.8164498539091,-43.781230743038,
-38.821457325757));
#246129=CARTESIAN_POINT('Ctrl Pts',(-51.8236120869667,-43.7716097649364,
-38.8304738402603));
#246130=CARTESIAN_POINT('Ctrl Pts',(-51.8271932034955,-43.7667992758857,
-38.8349820975119));
#246131=CARTESIAN_POINT('Ctrl Pts',(-51.8307469855887,-43.7619311761192,
-38.8395021196075));
#246132=CARTESIAN_POINT('Ctrl Pts',(-51.8342731412247,-43.7570055208757,
-38.8440333338866));
#246133=CARTESIAN_POINT('Ctrl Pts',(-51.8368130664596,-43.7534575220512,
-38.8472972129322));
#246134=CARTESIAN_POINT('Ctrl Pts',(-51.8397709257302,-43.7492575266246,
-38.8511273425434));
#246135=CARTESIAN_POINT('Ctrl Pts',(-51.8422112091579,-43.745749784102,
-38.8543131150123));
#246136=CARTESIAN_POINT('Ctrl Pts',(-51.8431587495307,-43.7443877588472,
-38.855550122156));
#246137=CARTESIAN_POINT('Ctrl Pts',(-51.8440288232728,-43.7431301746906,
-38.8566896765824));
#246138=CARTESIAN_POINT('Ctrl Pts',(-51.8447684504413,-43.7420559457143,
-38.857659973624));
#246139=CARTESIAN_POINT('Ctrl Pts',(-51.869619022372,-43.7059631606182,
-38.8902607723163));
#246140=CARTESIAN_POINT('Ctrl Pts',(-51.8933616238456,-43.6664604414045,
-38.92383760287));
#246141=CARTESIAN_POINT('Ctrl Pts',(-51.9157806930845,-43.6235568924935,
-38.9582211922616));
#246142=CARTESIAN_POINT('Ctrl Pts',(-51.9315329386519,-43.5934116964125,
-38.9823800339073));
#246143=CARTESIAN_POINT('Ctrl Pts',(-51.9466321814526,-43.5615877106783,
-39.0069361696535));
#246144=CARTESIAN_POINT('Ctrl Pts',(-51.9610125958872,-43.528090184004,
-39.0318184615583));
#246145=CARTESIAN_POINT('Ctrl Pts',(-51.9784361220784,-43.4875040773932,
-39.0619662202806));
#246146=CARTESIAN_POINT('Ctrl Pts',(-51.9948036328542,-43.444461108997,
-39.0925930961632));
#246147=CARTESIAN_POINT('Ctrl Pts',(-52.0100167926752,-43.3989739076197,
-39.1235551946763));
#246148=CARTESIAN_POINT('Ctrl Pts',(-52.0176233725858,-43.376230306931,
-39.1390362439329));
#246149=CARTESIAN_POINT('Ctrl Pts',(-52.0249417103708,-43.3528757033714,
-39.1546008212855));
#246150=CARTESIAN_POINT('Ctrl Pts',(-52.031961741472,-43.3289119934329,
-39.1702294612548));
#246151=CARTESIAN_POINT('Ctrl Pts',(-52.0354717570227,-43.3169301384636,
-39.1780437812394));
#246152=CARTESIAN_POINT('Ctrl Pts',(-52.0389072222062,-43.304796009584,
-39.1858741093882));
#246153=CARTESIAN_POINT('Ctrl Pts',(-52.0422670274971,-43.2925098629238,
-39.1937179293146));
#246154=CARTESIAN_POINT('Ctrl Pts',(-52.0439469301426,-43.2863667895937,
-39.1976398392779));
#246155=CARTESIAN_POINT('Ctrl Pts',(-52.0456079194934,-43.2801857119935,
-39.201565121674));
#246156=CARTESIAN_POINT('Ctrl Pts',(-52.0472498669231,-43.2739666631534,
-39.2054934588666));
#246157=CARTESIAN_POINT('Ctrl Pts',(-52.0485785941713,-43.2689339687429,
-39.2086724209779));
#246158=CARTESIAN_POINT('Ctrl Pts',(-52.050139501498,-43.2629252013346,
-39.2124478593144));
#246159=CARTESIAN_POINT('Ctrl Pts',(-52.0513379881636,-43.2582496014946,
-39.215376408652));
#246160=CARTESIAN_POINT('Ctrl Pts',(-52.0516205068005,-43.2571474247819,
-39.2160667540606));
#246161=CARTESIAN_POINT('Ctrl Pts',(-52.0518831318285,-43.2561193454742,
-39.2167100295185));
#246162=CARTESIAN_POINT('Ctrl Pts',(-52.0521184614956,-43.2551956366398,
-39.2172873150054));
#246163=CARTESIAN_POINT('Ctrl Pts',(-52.0649863542751,-43.2046869762132,
-39.2488534487757));
#246164=CARTESIAN_POINT('Ctrl Pts',(-52.0768350792428,-43.1508768626302,
-39.281128278774));
#246165=CARTESIAN_POINT('Ctrl Pts',(-52.0874657593684,-43.0937769205883,
-39.3139294576404));
#246166=CARTESIAN_POINT('Ctrl Pts',(-52.098456883128,-43.0347409490196,
-39.347842792641));
#246167=CARTESIAN_POINT('Ctrl Pts',(-52.1081448988321,-42.9721882462489,
-39.3823185300744));
#246168=CARTESIAN_POINT('Ctrl Pts',(-52.1163489521921,-42.9061392731944,
-39.417111092746));
#246169=CARTESIAN_POINT('Ctrl Pts',(-52.1241330629832,-42.843471162526,
-39.4501227213469));
#246170=CARTESIAN_POINT('Ctrl Pts',(-52.1305810127062,-42.7776556479445,
-39.4834186547465));
#246171=CARTESIAN_POINT('Ctrl Pts',(-52.1355813145032,-42.708716260349,
-39.5167597484441));
#246172=CARTESIAN_POINT('Ctrl Pts',(-52.1358510742276,-42.704997070797,
-39.5185584567247));
#246173=CARTESIAN_POINT('Ctrl Pts',(-52.1361166319404,-42.7012687906537,
-39.5203572909574));
#246174=CARTESIAN_POINT('Ctrl Pts',(-52.1363779740716,-42.6975314240561,
-39.5221562118214));
#246175=CARTESIAN_POINT('',(-51.2551520560089,-43.9396089457538,-38.3574184111583));
#246176=CARTESIAN_POINT('Ctrl Pts',(-51.2549749806985,-43.9395355987587,
-38.3573338134652));
#246177=CARTESIAN_POINT('Ctrl Pts',(-51.2311912050884,-43.9296840363366,
-38.3459729646063));
#246178=CARTESIAN_POINT('Ctrl Pts',(-51.2072412883732,-43.9197636560154,
-38.3352762701445));
#246179=CARTESIAN_POINT('Ctrl Pts',(-51.1631138496503,-43.9014854724236,
-38.316377625375));
#246180=CARTESIAN_POINT('Ctrl Pts',(-51.1425648781377,-43.8929738097303,
-38.3078789583852));
#246181=CARTESIAN_POINT('Ctrl Pts',(-51.1120978131143,-43.8803539381919,
-38.2955513131889));
#246182=CARTESIAN_POINT('Ctrl Pts',(-51.1015315829945,-43.8759772623731,
-38.2913264303936));
#246183=CARTESIAN_POINT('Ctrl Pts',(-51.0866459456191,-43.8698114294876,
-38.2854361560059));
#246184=CARTESIAN_POINT('Ctrl Pts',(-51.0822429209912,-43.8679876369713,
-38.283701557845));
#246185=CARTESIAN_POINT('Ctrl Pts',(-51.0758876115541,-43.8653551816094,
-38.2812086804991));
#246186=CARTESIAN_POINT('Ctrl Pts',(-51.0739305078821,-43.8645445227255,
-38.2804424886344));
#246187=CARTESIAN_POINT('Ctrl Pts',(-51.0710119900097,-43.8633356330407,
-38.2793021155487));
#246188=CARTESIAN_POINT('Ctrl Pts',(-51.0700503307405,-43.8629373007292,
-38.27892671662));
#246189=CARTESIAN_POINT('Ctrl Pts',(-51.0686079713225,-43.8623398558964,
-38.2783642040776));
#246190=CARTESIAN_POINT('Ctrl Pts',(-51.0681272830895,-43.8621407483109,
-38.2781768273618));
#246191=CARTESIAN_POINT('Ctrl Pts',(-51.0674057880406,-43.8618418952765,
-38.2778957157717));
#246192=CARTESIAN_POINT('Ctrl Pts',(-51.0671649926649,-43.8617421545661,
-38.2778019185543));
#246193=CARTESIAN_POINT('Ctrl Pts',(-51.0668036221895,-43.8615924700141,
-38.2776611872062));
#246194=CARTESIAN_POINT('Ctrl Pts',(-51.0666830508817,-43.8615425277432,
-38.2776142377835));
#246195=CARTESIAN_POINT('Ctrl Pts',(-51.0575674890041,-43.8577667383849,
-38.2740651411923));
#246196=CARTESIAN_POINT('Ctrl Pts',(-51.0485165904603,-43.8540177334563,
-38.2705724504896));
#246197=CARTESIAN_POINT('Ctrl Pts',(-51.0245088795784,-43.8440734140075,
-38.2613952017063));
#246198=CARTESIAN_POINT('Ctrl Pts',(-51.0093159881586,-43.8377803123299,
-38.2556783811805));
#246199=CARTESIAN_POINT('Ctrl Pts',(-50.9838482215668,-43.8272312180042,
-38.2462842461313));
#246200=CARTESIAN_POINT('Ctrl Pts',(-50.9733963020293,-43.8229018911788,
-38.2424824569401));
#246201=CARTESIAN_POINT('Ctrl Pts',(-50.9629628917746,-43.8185802311496,
-38.2387520398482));
#246202=CARTESIAN_POINT('',(-51.3131709192528,-43.8514488225354,-38.4111555278088));
#246203=CARTESIAN_POINT('Ctrl Pts',(-51.3131706199324,-43.8514490160907,
-38.4111560835884));
#246204=CARTESIAN_POINT('Ctrl Pts',(-51.3069386016551,-43.8640094387329,
-38.4034254897557));
#246205=CARTESIAN_POINT('Ctrl Pts',(-51.3002063680618,-43.8760898419399,
-38.3960439531634));
#246206=CARTESIAN_POINT('Ctrl Pts',(-51.2930358474315,-43.887681591147,
-38.3889937580458));
#246207=CARTESIAN_POINT('Ctrl Pts',(-51.2857753960681,-43.8994187209419,
-38.3818551412852));
#246208=CARTESIAN_POINT('Ctrl Pts',(-51.2780655250384,-43.9106546759655,
-38.3750568369513));
#246209=CARTESIAN_POINT('Ctrl Pts',(-51.2699335264417,-43.9213447836983,
-38.3685638057529));
#246210=CARTESIAN_POINT('Ctrl Pts',(-51.2651534708457,-43.9276285168645,
-38.3647471486611));
#246211=CARTESIAN_POINT('Ctrl Pts',(-51.2602268679523,-43.9337229911979,
-38.3610355849099));
#246212=CARTESIAN_POINT('Ctrl Pts',(-51.2551536659444,-43.939613984762,
-38.357418527837));
#246213=CARTESIAN_POINT('Ctrl Pts',(-51.855727616252,-42.5504169941763,
-39.0864710348602));
#246214=CARTESIAN_POINT('Ctrl Pts',(-51.8458743174447,-42.7008613470123,
-39.042782114243));
#246215=CARTESIAN_POINT('Ctrl Pts',(-51.8311705584223,-42.8391342171477,
-38.9977676632627));
#246216=CARTESIAN_POINT('Ctrl Pts',(-51.8014482670023,-43.0284553089955,
-38.9290723862128));
#246217=CARTESIAN_POINT('Ctrl Pts',(-51.7846711206524,-43.1185939468382,
-38.8944295129609));
#246218=CARTESIAN_POINT('Ctrl Pts',(-51.7616665101479,-43.2158800024417,
-38.8536552611055));
#246219=CARTESIAN_POINT('Ctrl Pts',(-51.7492971647288,-43.262558791895,
-38.8331972272602));
#246220=CARTESIAN_POINT('Ctrl Pts',(-51.7428945957875,-43.2854077086099,
-38.8229527559164));
#246221=CARTESIAN_POINT('Ctrl Pts',(-51.7401038255464,-43.2950950611959,
-38.8185591959896));
#246222=CARTESIAN_POINT('Ctrl Pts',(-51.7382328961144,-43.3015299608571,
-38.8156294996974));
#246223=CARTESIAN_POINT('Ctrl Pts',(-51.7376125178611,-43.3036541572315,
-38.8146605651198));
#246224=CARTESIAN_POINT('Ctrl Pts',(-51.7160874290895,-43.3763411190383,
-38.7813111028424));
#246225=CARTESIAN_POINT('Ctrl Pts',(-51.6936601975632,-43.4385690812335,
-38.7501513027776));
#246226=CARTESIAN_POINT('Ctrl Pts',(-51.6566553067176,-43.5226975170906,
-38.7039720702541));
#246227=CARTESIAN_POINT('Ctrl Pts',(-51.6373120808315,-43.5624582890849,
-38.681022058614));
#246228=CARTESIAN_POINT('Ctrl Pts',(-51.6132516816768,-43.6048274098125,
-38.6545338045479));
#246229=CARTESIAN_POINT('Ctrl Pts',(-51.6008456012002,-43.6250088569449,
-38.6413662782202));
#246230=CARTESIAN_POINT('Ctrl Pts',(-51.595447894416,-43.6334432541016,
-38.6357399840156));
#246231=CARTESIAN_POINT('Ctrl Pts',(-51.5918314348969,-43.639018470814,
-38.63199294011));
#246232=CARTESIAN_POINT('Ctrl Pts',(-51.5906499275888,-43.6408284542711,
-38.6307721667191));
#246233=CARTESIAN_POINT('Ctrl Pts',(-51.5094055996291,-43.7627195584335,
-38.5475952000448));
#246234=CARTESIAN_POINT('Ctrl Pts',(-51.418063219401,-43.8314895829832,
-38.474608352185));
#246235=CARTESIAN_POINT('Ctrl Pts',(-51.3131710690959,-43.8514487256653,
-38.4111552499418));
#246236=CARTESIAN_POINT('Ctrl Pts',(-52.3762811131638,-39.2667566979623,
-40.1997763344591));
#246237=CARTESIAN_POINT('Ctrl Pts',(-52.3787524417377,-39.2314150528153,
-39.8684983696827));
#246238=CARTESIAN_POINT('Ctrl Pts',(-52.0729733445211,-39.1963583849098,
-39.7409428796644));
#246239=CARTESIAN_POINT('Ctrl Pts',(-52.2944317444485,-40.4372572032816,
-40.074293523619));
#246240=CARTESIAN_POINT('Ctrl Pts',(-52.298594212147,-40.3777311420296,
-39.7508319554676));
#246241=CARTESIAN_POINT('Ctrl Pts',(-51.9996196710719,-40.3410025908912,
-39.6210810788317));
#246242=CARTESIAN_POINT('Ctrl Pts',(-52.2140974212184,-41.5860915487537,
-39.8473838284864));
#246243=CARTESIAN_POINT('Ctrl Pts',(-52.2193926604804,-41.5103660993754,
-39.5325747394078));
#246244=CARTESIAN_POINT('Ctrl Pts',(-51.9268724548342,-41.4641473693466,
-39.4019228714579));
#246245=CARTESIAN_POINT('Ctrl Pts',(-52.1363779744299,-42.6975314189331,
-39.5221562583896));
#246246=CARTESIAN_POINT('Ctrl Pts',(-52.1426275598539,-42.6081581835409,
-39.2152367329798));
#246247=CARTESIAN_POINT('Ctrl Pts',(-51.855727616252,-42.5504169941763,
-39.0864710348602));
#246248=CARTESIAN_POINT('',(-52.0729733445211,-39.1963583849098,-39.7409428796644));
#246249=CARTESIAN_POINT('',(-52.3762811131638,-39.2667566979623,-40.1997763344591));
#246250=CARTESIAN_POINT('Origin',(-51.8774990880339,-39.2318784610903,-40.1997763344591));
#246251=CARTESIAN_POINT('Origin',(-52.5931625893807,-36.1652070894527,-23.5673415363821));
#246252=CARTESIAN_POINT('Origin',(-52.1460600630305,-36.065931493028,-23.2795421339938));
#246253=CARTESIAN_POINT('Ctrl Pts',(-52.0729733445211,-39.1963583849098,
-39.7409428796644));
#246254=CARTESIAN_POINT('Ctrl Pts',(-52.3787524417377,-39.2314150528153,
-39.8684983696827));
#246255=CARTESIAN_POINT('Ctrl Pts',(-52.3762811131638,-39.2667566979623,
-40.1997763344591));
#246256=CARTESIAN_POINT('Ctrl Pts',(-52.100888629852,-38.7607556577822,
-39.7865571684177));
#246257=CARTESIAN_POINT('Ctrl Pts',(-52.4109286028315,-38.8364874603624,
-39.9107687095326));
#246258=CARTESIAN_POINT('Ctrl Pts',(-52.4029815901681,-38.8849220874284,
-40.2475330828085));
#246259=CARTESIAN_POINT('Ctrl Pts',(-52.2102585591639,-38.3472834992403,
-39.8504420494694));
#246260=CARTESIAN_POINT('Ctrl Pts',(-52.5175719298667,-38.4659927236101,
-39.9706931604272));
#246261=CARTESIAN_POINT('Ctrl Pts',(-52.4996604569693,-38.5219332431804,
-40.3132835285224));
#246262=CARTESIAN_POINT('Ctrl Pts',(-52.3973403582525,-37.9591679226684,
-39.9296369918383));
#246263=CARTESIAN_POINT('Ctrl Pts',(-52.6906835816361,-38.1229388123735,
-40.0447034978031));
#246264=CARTESIAN_POINT('Ctrl Pts',(-52.6630979669894,-38.1805575254669,
-40.3940322392211));
#246265=CARTESIAN_POINT('',(-52.3973403582525,-37.9591679226684,-39.9296369918383));
#246266=CARTESIAN_POINT('',(-52.6630979669894,-38.1805575254669,-40.3940322392211));
#246267=CARTESIAN_POINT('Origin',(-52.2121187508304,-37.964646093179,-40.3940322392211));
#246268=CARTESIAN_POINT('Ctrl Pts',(-52.3762811131638,-39.2667566979623,
-40.1997763344591));
#246269=CARTESIAN_POINT('Ctrl Pts',(-52.3813348028011,-39.1944855690943,
-40.2088154151));
#246270=CARTESIAN_POINT('Ctrl Pts',(-52.3890106866762,-39.1212990642225,
-40.2186994462388));
#246271=CARTESIAN_POINT('Ctrl Pts',(-52.399580537506,-39.0474991337333,
-40.2294606094852));
#246272=CARTESIAN_POINT('Ctrl Pts',(-52.4098707578906,-38.975651615605,
-40.2399370810253));
#246273=CARTESIAN_POINT('Ctrl Pts',(-52.4229039093203,-38.9032227962493,
-40.251244856509));
#246274=CARTESIAN_POINT('Ctrl Pts',(-52.4388845253147,-38.8304840396482,
-40.263398639784));
#246275=CARTESIAN_POINT('Ctrl Pts',(-52.4546982516725,-38.7585049123794,
-40.2754254980096));
#246276=CARTESIAN_POINT('Ctrl Pts',(-52.4733983143613,-38.6862223928386,
-40.2882807703834));
#246277=CARTESIAN_POINT('Ctrl Pts',(-52.4951355715001,-38.6138907219804,
-40.3019641257189));
#246278=CARTESIAN_POINT('Ctrl Pts',(-52.5169079265806,-38.5414422611912,
-40.3156695748081));
#246279=CARTESIAN_POINT('Ctrl Pts',(-52.5417274476098,-38.4689446114306,
-40.3302057758585));
#246280=CARTESIAN_POINT('Ctrl Pts',(-52.5696958444338,-38.3966427428268,
-40.3455578235737));
#246281=CARTESIAN_POINT('Ctrl Pts',(-52.5976642412578,-38.3243408742229,
-40.3609098712888));
#246282=CARTESIAN_POINT('Ctrl Pts',(-52.6287816069157,-38.2522349026372,
-40.3770777354374));
#246283=CARTESIAN_POINT('Ctrl Pts',(-52.6630979669894,-38.1805575254669,
-40.3940322392211));
#246284=CARTESIAN_POINT('Ctrl Pts',(-52.3973403582525,-37.9591679226684,
-39.9296369918383));
#246285=CARTESIAN_POINT('Ctrl Pts',(-52.3381595240891,-38.0819431134417,
-39.9045847271404));
#246286=CARTESIAN_POINT('Ctrl Pts',(-52.2869524009769,-38.2068368043554,
-39.8811490804055));
#246287=CARTESIAN_POINT('Ctrl Pts',(-52.2436543900273,-38.3338051377694,
-39.859375557193));
#246288=CARTESIAN_POINT('Ctrl Pts',(-52.2004721855357,-38.4604338769931,
-39.8376602702492));
#246289=CARTESIAN_POINT('Ctrl Pts',(-52.1651567780144,-38.5891263087813,
-39.8175981380879));
#246290=CARTESIAN_POINT('Ctrl Pts',(-52.1376916733654,-38.7198578257722,
-39.7992419918224));
#246291=CARTESIAN_POINT('Ctrl Pts',(-52.1103657443256,-38.8499268789298,
-39.7809788627825));
#246292=CARTESIAN_POINT('Ctrl Pts',(-52.090810706346,-38.9820145333958,
-39.7644043901133));
#246293=CARTESIAN_POINT('Ctrl Pts',(-52.0790583244375,-39.1161133203773,
-39.7495795137018));
#246294=CARTESIAN_POINT('Ctrl Pts',(-52.0767210815741,-39.1427820787019,
-39.7466312316546));
#246295=CARTESIAN_POINT('Ctrl Pts',(-52.0746925946574,-39.169530428859,
-39.7437521782701));
#246296=CARTESIAN_POINT('Ctrl Pts',(-52.0729733445211,-39.1963583849098,
-39.7409428796644));
#246297=CARTESIAN_POINT('Ctrl Pts',(-52.3973403582526,-37.9591679226684,
-39.9296369918383));
#246298=CARTESIAN_POINT('Ctrl Pts',(-52.6906835816361,-38.1229388123734,
-40.0447034978031));
#246299=CARTESIAN_POINT('Ctrl Pts',(-52.6630979669894,-38.1805575254669,
-40.3940322392211));
#246300=CARTESIAN_POINT('Ctrl Pts',(-53.1457424766041,-36.406550234656,
-40.2464484764969));
#246301=CARTESIAN_POINT('Ctrl Pts',(-53.4384326164932,-36.5566079867106,
-40.3650991663767));
#246302=CARTESIAN_POINT('Ctrl Pts',(-53.4324663318346,-36.573559978192,
-40.7170573734051));
#246303=CARTESIAN_POINT('Ctrl Pts',(-53.8198487743995,-34.8177779595407,
-40.2933158502147));
#246304=CARTESIAN_POINT('Ctrl Pts',(-54.1268603779516,-34.9318568554821,
-40.4136350441051));
#246305=CARTESIAN_POINT('Ctrl Pts',(-54.1287347135875,-34.9307380700991,
-40.7648390575021));
#246306=CARTESIAN_POINT('Ctrl Pts',(-54.5679521612331,-32.7869698119953,
-40.01447771336));
#246307=CARTESIAN_POINT('Ctrl Pts',(-54.8877444086082,-32.8830970178215,
-40.1309118165611));
#246308=CARTESIAN_POINT('Ctrl Pts',(-54.9060208033569,-32.8327777738735,
-40.4805364040184));
#246309=CARTESIAN_POINT('Ctrl Pts',(-54.7126522107998,-32.3789049161325,
-39.9414701040553));
#246310=CARTESIAN_POINT('Ctrl Pts',(-55.0357525196778,-32.4702090184626,
-40.0565968968413));
#246311=CARTESIAN_POINT('Ctrl Pts',(-55.0566283970611,-32.4113164265585,
-40.4060976883517));
#246312=CARTESIAN_POINT('Ctrl Pts',(-54.9880779906355,-31.5720202326829,
-39.7641101894595));
#246313=CARTESIAN_POINT('Ctrl Pts',(-55.3180333651333,-31.6546255096238,
-39.8762742785657));
#246314=CARTESIAN_POINT('Ctrl Pts',(-55.3438236830459,-31.5781288928756,
-40.2252589174025));
#246315=CARTESIAN_POINT('Ctrl Pts',(-55.1194549413204,-31.1714661595765,
-39.6595567410297));
#246316=CARTESIAN_POINT('Ctrl Pts',(-55.4530870881607,-31.2497493955288,
-39.7698680960119));
#246317=CARTESIAN_POINT('Ctrl Pts',(-55.4810874242724,-31.1646108621852,
-40.1186537766862));
#246318=CARTESIAN_POINT('Ctrl Pts',(-55.4956573107256,-29.9783108281782,
-39.2999034309858));
#246319=CARTESIAN_POINT('Ctrl Pts',(-55.8415244394745,-30.042499694056,
-39.4035145580109));
#246320=CARTESIAN_POINT('Ctrl Pts',(-55.8749613596854,-29.9331076843543,
-39.7519370004083));
#246321=CARTESIAN_POINT('Ctrl Pts',(-55.7225896344932,-29.1941586468675,
-38.9989859405087));
#246322=CARTESIAN_POINT('Ctrl Pts',(-56.077077518843,-29.2501138114284,
-39.0964197551406));
#246323=CARTESIAN_POINT('Ctrl Pts',(-56.1136890638183,-29.1241139971889,
-39.4451035675999));
#246324=CARTESIAN_POINT('Ctrl Pts',(-55.9280282803564,-28.4214833957092,
-38.6389054336786));
#246325=CARTESIAN_POINT('Ctrl Pts',(-56.2902455608578,-28.4766057597396,
-38.7328054198089));
#246326=CARTESIAN_POINT('Ctrl Pts',(-56.3309570935689,-28.3272991455305,
-39.0779244525544));
#246327=CARTESIAN_POINT('',(-55.9280282803564,-28.4214833957092,-38.6389054336786));
#246328=CARTESIAN_POINT('',(-56.3309570935689,-28.3272991455305,-39.0779244525544));
#246329=CARTESIAN_POINT('Origin',(-55.8485682509781,-28.1957658625034,-39.0779244525544));
#246330=CARTESIAN_POINT('Ctrl Pts',(-52.6630979669894,-38.1805575254669,
-40.3940322392211));
#246331=CARTESIAN_POINT('Ctrl Pts',(-52.8760451560815,-37.7357697928196,
-40.4834397291488));
#246332=CARTESIAN_POINT('Ctrl Pts',(-53.0834983485661,-37.2880132084225,
-40.551761385336));
#246333=CARTESIAN_POINT('Ctrl Pts',(-53.2853549466339,-36.8374221904802,
-40.5989778505683));
#246334=CARTESIAN_POINT('Ctrl Pts',(-53.4478491683769,-36.4746971793296,
-40.6369870256205));
#246335=CARTESIAN_POINT('Ctrl Pts',(-53.6067170909194,-36.1101352784612,
-40.6613205359031));
#246336=CARTESIAN_POINT('Ctrl Pts',(-53.7619142086117,-35.7438031016591,
-40.6719908480972));
#246337=CARTESIAN_POINT('Ctrl Pts',(-53.9359086942521,-35.3331010240432,
-40.6839535411514));
#246338=CARTESIAN_POINT('Ctrl Pts',(-54.105287952085,-34.9201765391549,
-40.6787343711124));
#246339=CARTESIAN_POINT('Ctrl Pts',(-54.2699948688641,-34.5051333001102,
-40.6563333253597));
#246340=CARTESIAN_POINT('Ctrl Pts',(-54.3523483272536,-34.2976116805879,
-40.6451328024833));
#246341=CARTESIAN_POINT('Ctrl Pts',(-54.4335338407837,-34.089560425584,
-40.629636810339));
#246342=CARTESIAN_POINT('Ctrl Pts',(-54.5135451044598,-33.8809928709033,
-40.6098453486404));
#246343=CARTESIAN_POINT('Ctrl Pts',(-54.5555679147339,-33.7714508592289,
-40.5994506516715));
#246344=CARTESIAN_POINT('Ctrl Pts',(-54.5974060491286,-33.6614000385814,
-40.5878321906909));
#246345=CARTESIAN_POINT('Ctrl Pts',(-54.6388378415948,-33.5514189685314,
-40.5750457578139));
#246346=CARTESIAN_POINT('Ctrl Pts',(-54.6762920172485,-33.4519965184991,
-40.5634868733328));
#246347=CARTESIAN_POINT('Ctrl Pts',(-54.7134142984132,-33.3526311541021,
-40.5509741559631));
#246348=CARTESIAN_POINT('Ctrl Pts',(-54.7500504083475,-33.2537548873174,
-40.5375839610123));
#246349=CARTESIAN_POINT('Ctrl Pts',(-54.7502214650147,-33.2532932268219,
-40.5375214412162));
#246350=CARTESIAN_POINT('Ctrl Pts',(-54.7503925152058,-33.2528315659145,
-40.5374589009037));
#246351=CARTESIAN_POINT('Ctrl Pts',(-54.7505635589241,-33.2523699045864,
-40.5373963400742));
#246352=CARTESIAN_POINT('Ctrl Pts',(-54.8109190055075,-33.0894654968639,
-40.5153207745943));
#246353=CARTESIAN_POINT('Ctrl Pts',(-54.8704399382255,-32.9265623149063,
-40.4906380116614));
#246354=CARTESIAN_POINT('Ctrl Pts',(-54.9291455224067,-32.7636633303162,
-40.4633905681202));
#246355=CARTESIAN_POINT('Ctrl Pts',(-54.9873071697268,-32.6022736870193,
-40.4363955858928));
#246356=CARTESIAN_POINT('Ctrl Pts',(-55.0446688758138,-32.4408869522044,
-40.4068828775015));
#246357=CARTESIAN_POINT('Ctrl Pts',(-55.1012324203421,-32.2795110730784,
-40.3748470776743));
#246358=CARTESIAN_POINT('Ctrl Pts',(-55.1333863062824,-32.18777598727,-40.3566361352335));
#246359=CARTESIAN_POINT('Ctrl Pts',(-55.1652819353429,-32.0960445994109,
-40.3376090518113));
#246360=CARTESIAN_POINT('Ctrl Pts',(-55.19691646867,-32.0043213810441,-40.3177586380898));
#246361=CARTESIAN_POINT('Ctrl Pts',(-55.1980200095687,-32.0011217029651,
-40.3170661751041));
#246362=CARTESIAN_POINT('Ctrl Pts',(-55.1991232004239,-31.9979221280785,
-40.3163727298852));
#246363=CARTESIAN_POINT('Ctrl Pts',(-55.2002260400535,-31.994722659717,
-40.3156783028771));
#246364=CARTESIAN_POINT('Ctrl Pts',(-55.2636031512567,-31.8108581551368,
-40.2757715235684));
#246365=CARTESIAN_POINT('Ctrl Pts',(-55.325951793402,-31.6269964981267,
-40.2325819377435));
#246366=CARTESIAN_POINT('Ctrl Pts',(-55.3872684018359,-31.443178847248,
-40.1861063713614));
#246367=CARTESIAN_POINT('Ctrl Pts',(-55.429027236798,-31.3179923579394,
-40.1544548244822));
#246368=CARTESIAN_POINT('Ctrl Pts',(-55.4703078146834,-31.192825294027,
-40.1212791854428));
#246369=CARTESIAN_POINT('Ctrl Pts',(-55.5111134058755,-31.0676789074495,
-40.0865765609729));
#246370=CARTESIAN_POINT('Ctrl Pts',(-55.530477816035,-31.0082903313041,
-40.0701083311491));
#246371=CARTESIAN_POINT('Ctrl Pts',(-55.5499419887612,-30.9482684207738,
-40.0531149583656));
#246372=CARTESIAN_POINT('Ctrl Pts',(-55.5691505247735,-30.8887074115548,
-40.0359028676874));
#246373=CARTESIAN_POINT('Ctrl Pts',(-55.5835906458874,-30.843932099879,
-40.02296358518));
#246374=CARTESIAN_POINT('Ctrl Pts',(-55.5978866951893,-30.7994170631401,
-40.0099017258433));
#246375=CARTESIAN_POINT('Ctrl Pts',(-55.6118945080683,-30.7556237400288,
-39.9968653099877));
#246376=CARTESIAN_POINT('Ctrl Pts',(-55.6120559180998,-30.7551191158079,
-39.9967150932257));
#246377=CARTESIAN_POINT('Ctrl Pts',(-55.6122173197593,-30.7546144941026,
-39.9965648522302));
#246378=CARTESIAN_POINT('Ctrl Pts',(-55.6123787130472,-30.7541098749132,
-39.9964145870016));
#246379=CARTESIAN_POINT('Ctrl Pts',(-55.7548384822693,-30.3086890385658,
-39.8637774118964));
#246380=CARTESIAN_POINT('Ctrl Pts',(-55.8907835748029,-29.8652112734624,
-39.7123085185695));
#246381=CARTESIAN_POINT('Ctrl Pts',(-56.0204269822374,-29.4238800047714,
-39.5419882937266));
#246382=CARTESIAN_POINT('Ctrl Pts',(-56.1282497940572,-29.0568302698414,
-39.4003350780657));
#246383=CARTESIAN_POINT('Ctrl Pts',(-56.2317142317968,-28.6912651936965,
-39.2456431279436));
#246384=CARTESIAN_POINT('Ctrl Pts',(-56.3309570935689,-28.3272991455305,
-39.0779244525544));
#246385=CARTESIAN_POINT('Ctrl Pts',(-55.9280282803564,-28.4214833957092,
-38.6389054336786));
#246386=CARTESIAN_POINT('Ctrl Pts',(-55.8595025109934,-28.6792156535855,
-38.7590132822262));
#246387=CARTESIAN_POINT('Ctrl Pts',(-55.7888458358274,-28.9372393566178,
-38.8720750899543));
#246388=CARTESIAN_POINT('Ctrl Pts',(-55.7160933944967,-29.1952948017582,
-38.9780896749729));
#246389=CARTESIAN_POINT('Ctrl Pts',(-55.6418369701219,-29.4586849271757,
-39.08629585845));
#246390=CARTESIAN_POINT('Ctrl Pts',(-55.565397089092,-29.7221081267061,
-39.1871602619621));
#246391=CARTESIAN_POINT('Ctrl Pts',(-55.4868336072826,-29.9852798369313,
-39.2807323450087));
#246392=CARTESIAN_POINT('Ctrl Pts',(-55.4082701254731,-30.2484515471565,
-39.3743044280552));
#246393=CARTESIAN_POINT('Ctrl Pts',(-55.3275829838991,-30.5113717428164,
-39.4605842051981));
#246394=CARTESIAN_POINT('Ctrl Pts',(-55.2448557311221,-30.773747715777,
-39.5396723043484));
#246395=CARTESIAN_POINT('Ctrl Pts',(-55.2035971806928,-30.9046024456088,
-39.5791159002327));
#246396=CARTESIAN_POINT('Ctrl Pts',(-55.1618285510732,-31.0353297545122,
-39.6167686677692));
#246397=CARTESIAN_POINT('Ctrl Pts',(-55.1195602217546,-31.165894991039,
-39.6526370728405));
#246398=CARTESIAN_POINT('Ctrl Pts',(-55.0429685311297,-31.4024837648001,
-39.7176318769577));
#246399=CARTESIAN_POINT('Ctrl Pts',(-54.964737103265,-31.6385337089141,
-39.776762889674));
#246400=CARTESIAN_POINT('Ctrl Pts',(-54.8849569483814,-31.8737910274784,
-39.8300923327622));
#246401=CARTESIAN_POINT('Ctrl Pts',(-54.8734583654024,-31.9076982792613,
-39.8377786179977));
#246402=CARTESIAN_POINT('Ctrl Pts',(-54.8619276465711,-31.941589052632,
-39.8453444670309));
#246403=CARTESIAN_POINT('Ctrl Pts',(-54.8503651007177,-31.9754625744077,
-39.8527901467574));
#246404=CARTESIAN_POINT('Ctrl Pts',(-54.8385632459024,-32.0100371733883,
-39.8603899290412));
#246405=CARTESIAN_POINT('Ctrl Pts',(-54.8267234728141,-32.044606447891,
-39.8678659505221));
#246406=CARTESIAN_POINT('Ctrl Pts',(-54.814851167199,-32.0791552626038,
-39.8752157882416));
#246407=CARTESIAN_POINT('Ctrl Pts',(-54.7610765509181,-32.2356412320839,
-39.9085062640686));
#246408=CARTESIAN_POINT('Ctrl Pts',(-54.7066122033027,-32.391776105291,
-39.9392266524732));
#246409=CARTESIAN_POINT('Ctrl Pts',(-54.6514895234034,-32.547506073265,
-39.9674256651062));
#246410=CARTESIAN_POINT('Ctrl Pts',(-54.5925932920716,-32.7138968988899,
-39.9975551068242));
#246411=CARTESIAN_POINT('Ctrl Pts',(-54.5329450048582,-32.8798272445593,
-40.0248067697069));
#246412=CARTESIAN_POINT('Ctrl Pts',(-54.4725652945174,-33.045235666278,
-40.0491901836131));
#246413=CARTESIAN_POINT('Ctrl Pts',(-54.459998567761,-33.0796618406867,
-40.0542650622142));
#246414=CARTESIAN_POINT('Ctrl Pts',(-54.4476988874635,-33.1132505315278,
-40.0590994196371));
#246415=CARTESIAN_POINT('Ctrl Pts',(-54.4350351962782,-33.1477240550659,
-40.0639400649739));
#246416=CARTESIAN_POINT('Ctrl Pts',(-54.4297277455465,-33.1621721748955,
-40.0659688168014));
#246417=CARTESIAN_POINT('Ctrl Pts',(-54.4243561818974,-33.1767756701395,
-40.0679980885883));
#246418=CARTESIAN_POINT('Ctrl Pts',(-54.4188732977944,-33.1916610504326,
-40.0700434285701));
#246419=CARTESIAN_POINT('Ctrl Pts',(-54.4186927565832,-33.1921511984162,
-40.0701107778248));
#246420=CARTESIAN_POINT('Ctrl Pts',(-54.4185122071696,-33.192641346441,
-40.0701781023605));
#246421=CARTESIAN_POINT('Ctrl Pts',(-54.4183316495574,-33.193131494494,
-40.0702454021735));
#246422=CARTESIAN_POINT('Ctrl Pts',(-54.3216825238763,-33.455498614907,
-40.1062697381429));
#246423=CARTESIAN_POINT('Ctrl Pts',(-54.2227641565077,-33.7177318491769,
-40.1353601491472));
#246424=CARTESIAN_POINT('Ctrl Pts',(-54.1216389171421,-33.9795830238138,
-40.1573801871496));
#246425=CARTESIAN_POINT('Ctrl Pts',(-54.0207235880817,-34.2408906619379,
-40.1793545171475));
#246426=CARTESIAN_POINT('Ctrl Pts',(-53.9176105406912,-34.5018178209743,
-40.1942877778114));
#246427=CARTESIAN_POINT('Ctrl Pts',(-53.8123757322959,-34.7621244357644,
-40.202093896917));
#246428=CARTESIAN_POINT('Ctrl Pts',(-53.7030310371878,-35.0325971801243,
-40.2102048796478));
#246429=CARTESIAN_POINT('Ctrl Pts',(-53.5913955171586,-35.3023999113141,
-40.2106207756592));
#246430=CARTESIAN_POINT('Ctrl Pts',(-53.4775703714016,-35.571270916981,
-40.2033021049399));
#246431=CARTESIAN_POINT('Ctrl Pts',(-53.3681804343619,-35.8296653357723,
-40.1962686069911));
#246432=CARTESIAN_POINT('Ctrl Pts',(-53.2567682858326,-36.0871992674317,
-40.1820918925141));
#246433=CARTESIAN_POINT('Ctrl Pts',(-53.1434378897113,-36.3436472007061,
-40.160787752568));
#246434=CARTESIAN_POINT('Ctrl Pts',(-53.0300324555901,-36.6002649325572,
-40.1394695067853));
#246435=CARTESIAN_POINT('Ctrl Pts',(-52.9147062402528,-36.8557952264196,
-40.1110143971545));
#246436=CARTESIAN_POINT('Ctrl Pts',(-52.7975772000339,-37.1100188075254,
-40.075488166563));
#246437=CARTESIAN_POINT('Ctrl Pts',(-52.6802158407442,-37.3647466272557,
-40.0398914716284));
#246438=CARTESIAN_POINT('Ctrl Pts',(-52.5610445063604,-37.6181625450243,
-39.997195584507));
#246439=CARTESIAN_POINT('Ctrl Pts',(-52.4401955774352,-37.8700527012338,
-39.9475166832538));
#246440=CARTESIAN_POINT('Ctrl Pts',(-52.4259337762717,-37.8997791320335,
-39.9416539038482));
#246441=CARTESIAN_POINT('Ctrl Pts',(-52.411648626526,-37.9294843209584,
-39.9356939278134));
#246442=CARTESIAN_POINT('Ctrl Pts',(-52.3973403582526,-37.9591679226684,
-39.9296369918383));
#246443=CARTESIAN_POINT('Ctrl Pts',(-55.9280282803564,-28.4214833957092,
-38.6389054336786));
#246444=CARTESIAN_POINT('Ctrl Pts',(-56.2902455608578,-28.4766057597396,
-38.7328054198089));
#246445=CARTESIAN_POINT('Ctrl Pts',(-56.3309570935689,-28.3272991455305,
-39.0779244525544));
#246446=CARTESIAN_POINT('Ctrl Pts',(-55.9771522644365,-28.2367232142716,
-38.552803881023));
#246447=CARTESIAN_POINT('Ctrl Pts',(-56.3140818024757,-28.2791502561168,
-38.6345461846056));
#246448=CARTESIAN_POINT('Ctrl Pts',(-56.3829126567059,-28.1367558595196,
-38.9462184848765));
#246449=CARTESIAN_POINT('Ctrl Pts',(-56.0135219001012,-28.0528579818781,
-38.461315834925));
#246450=CARTESIAN_POINT('Ctrl Pts',(-56.3268630274838,-28.0775147348304,
-38.5284708636181));
#246451=CARTESIAN_POINT('Ctrl Pts',(-56.4167006885852,-27.9458326698372,
-38.8064076909433));
#246452=CARTESIAN_POINT('Ctrl Pts',(-56.0471103898057,-27.685962661452,
-38.2659355865592));
#246453=CARTESIAN_POINT('Ctrl Pts',(-56.3080000147378,-27.6770507033699,
-38.3033918191236));
#246454=CARTESIAN_POINT('Ctrl Pts',(-56.4275000344708,-27.560942607285,
-38.5081858145621));
#246455=CARTESIAN_POINT('Ctrl Pts',(-56.0452301422673,-27.5003069580262,
-38.1605763563824));
#246456=CARTESIAN_POINT('Ctrl Pts',(-56.2793394878168,-27.4741008831429,
-38.1827126614319));
#246457=CARTESIAN_POINT('Ctrl Pts',(-56.4055238530003,-27.3641600613333,
-38.3474070423507));
#246458=CARTESIAN_POINT('Ctrl Pts',(-56.0042558232646,-27.3241842272071,
-38.0522584541458));
#246459=CARTESIAN_POINT('Ctrl Pts',(-56.2039767728891,-27.2781673895146,
-38.0563752154928));
#246460=CARTESIAN_POINT('Ctrl Pts',(-56.3272010881867,-27.1739053137705,
-38.1827403312291));
#246461=CARTESIAN_POINT('',(-56.329970462594,-27.1806936516958,-38.1886113251078));
#246462=CARTESIAN_POINT('',(-56.3105671034289,-27.2343570385725,-38.1841758734895));
#246463=CARTESIAN_POINT('Ctrl Pts',(-56.3299705172648,-27.1806936804351,
-38.1886114231063));
#246464=CARTESIAN_POINT('Ctrl Pts',(-56.3269691615845,-27.189692744714,
-38.1876467081772));
#246465=CARTESIAN_POINT('Ctrl Pts',(-56.3238524112746,-27.1986710864456,
-38.186802403549));
#246466=CARTESIAN_POINT('Ctrl Pts',(-56.3173870154762,-27.2165616053026,
-38.1853313182445));
#246467=CARTESIAN_POINT('Ctrl Pts',(-56.3140355294396,-27.2254811086767,
-38.1847041131599));
#246468=CARTESIAN_POINT('Ctrl Pts',(-56.3105671034163,-27.2343570378499,
-38.1841758742811));
#246469=CARTESIAN_POINT('Ctrl Pts',(-56.3309570935689,-28.3272991455305,
-39.0779244525544));
#246470=CARTESIAN_POINT('Ctrl Pts',(-56.3461201068511,-28.2716898863449,
-39.039486617472));
#246471=CARTESIAN_POINT('Ctrl Pts',(-56.3593682732299,-28.2173779774047,
-39.0012762447384));
#246472=CARTESIAN_POINT('Ctrl Pts',(-56.3707008719059,-28.1643327425414,
-38.9633572404796));
#246473=CARTESIAN_POINT('Ctrl Pts',(-56.3824169834641,-28.1094923738794,
-38.9241549977484));
#246474=CARTESIAN_POINT('Ctrl Pts',(-56.3920860246955,-28.0560058960518,
-38.885264239361));
#246475=CARTESIAN_POINT('Ctrl Pts',(-56.399764516406,-28.0038471393053,
-38.8467574908829));
#246476=CARTESIAN_POINT('Ctrl Pts',(-56.4079112481125,-27.948507703726,
-38.805902572942));
#246477=CARTESIAN_POINT('Ctrl Pts',(-56.413817471714,-27.8946628690484,
-38.7654800016931));
#246478=CARTESIAN_POINT('Ctrl Pts',(-56.4176100874624,-27.8422896230681,
-38.7255774452514));
#246479=CARTESIAN_POINT('Ctrl Pts',(-56.4197909465699,-27.812173555936,
-38.7026323700314));
#246480=CARTESIAN_POINT('Ctrl Pts',(-56.4212739875461,-27.7825442284572,
-38.6798592538911));
#246481=CARTESIAN_POINT('Ctrl Pts',(-56.4220909106037,-27.753398352269,
-38.6572747578281));
#246482=CARTESIAN_POINT('Ctrl Pts',(-56.423134269861,-27.7161737697971,
-38.6284302506032));
#246483=CARTESIAN_POINT('Ctrl Pts',(-56.4231257094644,-27.679634330352,
-38.5998063072248));
#246484=CARTESIAN_POINT('Ctrl Pts',(-56.4220192345237,-27.6438642774849,
-38.5715055700834));
#246485=CARTESIAN_POINT('Ctrl Pts',(-56.420876952977,-27.6069366708922,
-38.5422889935433));
#246486=CARTESIAN_POINT('Ctrl Pts',(-56.4185647847815,-27.5708289824376,
-38.5134168402244));
#246487=CARTESIAN_POINT('Ctrl Pts',(-56.4150800085523,-27.5356115188146,
-38.4849833562604));
#246488=CARTESIAN_POINT('Ctrl Pts',(-56.4113982623776,-27.4984034591139,
-38.4549427269819));
#246489=CARTESIAN_POINT('Ctrl Pts',(-56.4064077337896,-27.4621890975008,
-38.4253917770801));
#246490=CARTESIAN_POINT('Ctrl Pts',(-56.4001551812337,-27.427027248806,
-38.3964211901481));
#246491=CARTESIAN_POINT('Ctrl Pts',(-56.3936726956335,-27.3905723488592,
-38.3663852310843));
#246492=CARTESIAN_POINT('Ctrl Pts',(-56.3858340302463,-27.3552486854546,
-38.336973041202));
#246493=CARTESIAN_POINT('Ctrl Pts',(-56.3767393875982,-27.3210976288266,
-38.3082647183813));
#246494=CARTESIAN_POINT('Ctrl Pts',(-56.3670679856636,-27.284780798367,
-38.2777357861724));
#246495=CARTESIAN_POINT('Ctrl Pts',(-56.3559765593455,-27.2497899684099,
-38.2480028279519));
#246496=CARTESIAN_POINT('Ctrl Pts',(-56.3436339365408,-27.2161491683113,
-38.2191392545631));
#246497=CARTESIAN_POINT('Ctrl Pts',(-56.3392349416417,-27.2041593578492,
-38.2088520802636));
#246498=CARTESIAN_POINT('Ctrl Pts',(-56.3346774134342,-27.1923408141125,
-38.1986751391635));
#246499=CARTESIAN_POINT('Ctrl Pts',(-56.3299702222398,-27.1806939286319,
-38.1886111170349));
#246500=CARTESIAN_POINT('',(-56.0373082460296,-27.7729550357457,-38.311656138237));
#246501=CARTESIAN_POINT('Ctrl Pts',(-56.0373052066298,-27.7730130613194,
-38.3116877705396));
#246502=CARTESIAN_POINT('Ctrl Pts',(-56.035646130788,-27.8046657328717,
-38.3289427060704));
#246503=CARTESIAN_POINT('Ctrl Pts',(-56.0333127894923,-27.8368271237374,
-38.3462766787704));
#246504=CARTESIAN_POINT('Ctrl Pts',(-56.0303381943686,-27.8694105448201,
-38.3636295168291));
#246505=CARTESIAN_POINT('Ctrl Pts',(-56.0286759911365,-27.8876181547931,
-38.3733262796857));
#246506=CARTESIAN_POINT('Ctrl Pts',(-56.0268051262239,-27.9059830603538,
-38.3830432285537));
#246507=CARTESIAN_POINT('Ctrl Pts',(-56.0247195628867,-27.9245020533413,
-38.3927754207108));
#246508=CARTESIAN_POINT('Ctrl Pts',(-56.0182865355039,-27.9816248397191,
-38.4227948679862));
#246509=CARTESIAN_POINT('Ctrl Pts',(-56.0098655697242,-28.0401765970223,
-38.4529489814088));
#246510=CARTESIAN_POINT('Ctrl Pts',(-55.9994204528404,-28.100180513741,
-38.4831776867009));
#246511=CARTESIAN_POINT('Ctrl Pts',(-55.9893894320084,-28.1578055786693,
-38.5122079767289));
#246512=CARTESIAN_POINT('Ctrl Pts',(-55.97749145665,-28.2167699428144,-38.54130703125));
#246513=CARTESIAN_POINT('Ctrl Pts',(-55.9637414575256,-28.2770983741972,
-38.5704249033626));
#246514=CARTESIAN_POINT('Ctrl Pts',(-55.9529641626647,-28.3243839985543,
-38.593247587978));
#246515=CARTESIAN_POINT('Ctrl Pts',(-55.9410499212476,-28.3725077114536,
-38.6160818879126));
#246516=CARTESIAN_POINT('Ctrl Pts',(-55.9280282803564,-28.4214833957092,
-38.6389054336786));
#246517=CARTESIAN_POINT('Ctrl Pts',(-56.3105671031579,-27.2343570385113,
-38.1841758742417));
#246518=CARTESIAN_POINT('Ctrl Pts',(-56.2731836457653,-27.3300237523219,
-38.1784823996949));
#246519=CARTESIAN_POINT('Ctrl Pts',(-56.22815914317,-27.425144703044,-38.1927583058393));
#246520=CARTESIAN_POINT('Ctrl Pts',(-56.1357812725437,-27.6032305524574,
-38.2400026082589));
#246521=CARTESIAN_POINT('Ctrl Pts',(-56.086002246048,-27.6908676735014,
-38.2742157055539));
#246522=CARTESIAN_POINT('Ctrl Pts',(-56.037313485634,-27.7728550057779,
-38.3116016074841));
#246523=CARTESIAN_POINT('Ctrl Pts',(-53.5049272332164,-45.5904441965002,
-27.0918908718704));
#246524=CARTESIAN_POINT('Ctrl Pts',(-53.2176708121394,-45.0562509145002,
-26.9551461919307));
#246525=CARTESIAN_POINT('Ctrl Pts',(-53.1622384417568,-44.6469455848382,
-27.4198764587519));
#246526=CARTESIAN_POINT('Ctrl Pts',(-53.3401376735643,-45.6078127141537,
-27.1200911635315));
#246527=CARTESIAN_POINT('Ctrl Pts',(-53.1337365804956,-45.0871086122264,
-27.0122080197638));
#246528=CARTESIAN_POINT('Ctrl Pts',(-53.063726008764,-44.7100871047333,
-27.4303518614045));
#246529=CARTESIAN_POINT('Ctrl Pts',(-53.1566042596039,-45.6113895454731,
-27.1349070389393));
#246530=CARTESIAN_POINT('Ctrl Pts',(-53.0245060734752,-45.1301223401293,
-27.0637831794719));
#246531=CARTESIAN_POINT('Ctrl Pts',(-52.9589297219542,-44.7746345958153,
-27.4136386124325));
#246532=CARTESIAN_POINT('Ctrl Pts',(-52.8631376063666,-45.5875376591559,
-27.1460905313543));
#246533=CARTESIAN_POINT('Ctrl Pts',(-52.8151221132255,-45.2071015764094,
-27.1155083247184));
#246534=CARTESIAN_POINT('Ctrl Pts',(-52.7848678380642,-44.9023469842384,
-27.3473769064844));
#246535=CARTESIAN_POINT('Ctrl Pts',(-52.762004727618,-45.5747306984873,
-27.1480089070401));
#246536=CARTESIAN_POINT('Ctrl Pts',(-52.73999642702,-45.2344272993809,-27.1285847238272));
#246537=CARTESIAN_POINT('Ctrl Pts',(-52.7241510212094,-44.9506058502004,
-27.317579614679));
#246538=CARTESIAN_POINT('Ctrl Pts',(-52.6073879775618,-45.5460939686536,
-27.1494556764823));
#246539=CARTESIAN_POINT('Ctrl Pts',(-52.6148381830911,-45.2827523418283,
-27.1414548626328));
#246540=CARTESIAN_POINT('Ctrl Pts',(-52.6220773103498,-45.0491834799539,
-27.263203350593));
#246541=CARTESIAN_POINT('Ctrl Pts',(-52.5551162511329,-45.5349159989873,
-27.1497020573719));
#246542=CARTESIAN_POINT('Ctrl Pts',(-52.5715747382081,-45.2994028420944,
-27.1446544886293));
#246543=CARTESIAN_POINT('Ctrl Pts',(-52.5864288471625,-45.0855251832409,
-27.243489825349));
#246544=CARTESIAN_POINT('Ctrl Pts',(-52.4764210340132,-45.5150283699019,
-27.1498873098043));
#246545=CARTESIAN_POINT('Ctrl Pts',(-52.5008596531919,-45.334079330316,
-27.1478520318169));
#246546=CARTESIAN_POINT('Ctrl Pts',(-52.5238148016628,-45.1638876910866,
-27.2098971119021));
#246547=CARTESIAN_POINT('Ctrl Pts',(-52.4501261696617,-45.5078812506388,
-27.149918608058));
#246548=CARTESIAN_POINT('Ctrl Pts',(-52.4766859109803,-45.3462185725822,
-27.1486382797322));
#246549=CARTESIAN_POINT('Ctrl Pts',(-52.5018689863788,-45.192276719095,
-27.198669824253));
#246550=CARTESIAN_POINT('Ctrl Pts',(-52.4105457516782,-45.4960245236483,
-27.1499421164755));
#246551=CARTESIAN_POINT('Ctrl Pts',(-52.4374156231595,-45.3700061187084,
-27.1494236542118));
#246552=CARTESIAN_POINT('Ctrl Pts',(-52.4634217751467,-45.2479034668112,
-27.1813235487131));
#246553=CARTESIAN_POINT('Ctrl Pts',(-52.397352190851,-45.4918856766869,
-27.1499460403929));
#246554=CARTESIAN_POINT('Ctrl Pts',(-52.4242270113872,-45.3778792225278,
-27.1496188303446));
#246555=CARTESIAN_POINT('Ctrl Pts',(-52.450381510263,-45.2667337504327,
-27.1756979157076));
#246556=CARTESIAN_POINT('Ctrl Pts',(-52.3776026724743,-45.4853183606142,
-27.1499490074433));
#246557=CARTESIAN_POINT('Ctrl Pts',(-52.4007513598026,-45.3991513814277,
-27.1498212851494));
#246558=CARTESIAN_POINT('Ctrl Pts',(-52.4235369397624,-45.3142904301389,
-27.1653223320967));
#246559=CARTESIAN_POINT('Ctrl Pts',(-52.3710211458483,-45.483069951052,
-27.1499495102509));
#246560=CARTESIAN_POINT('Ctrl Pts',(-52.392612848151,-45.4068824448819,
-27.1498709642282));
#246561=CARTESIAN_POINT('Ctrl Pts',(-52.4139394359862,-45.3315890395918,
-27.161969255845));
#246562=CARTESIAN_POINT('Ctrl Pts',(-52.3611723955272,-45.4795723115674,
-27.1499498834281));
#246563=CARTESIAN_POINT('Ctrl Pts',(-52.3791731661577,-45.4211953896253,
-27.1499196186609));
#246564=CARTESIAN_POINT('Ctrl Pts',(-52.3970410441707,-45.3632394127332,
-27.1572535611551));
#246565=CARTESIAN_POINT('Ctrl Pts',(-52.357893820504,-45.4783859538111,
-27.1499499446124));
#246566=CARTESIAN_POINT('Ctrl Pts',(-52.3744966404333,-45.4264035092904,
-27.1499315299618));
#246567=CARTESIAN_POINT('Ctrl Pts',(-52.3910025434165,-45.3747156667379,
-27.1557336710171));
#246568=CARTESIAN_POINT('Ctrl Pts',(-52.3529857957684,-45.4765600171004,
-27.1499499883959));
#246569=CARTESIAN_POINT('Ctrl Pts',(-52.3667871434141,-45.435788327086,
-27.1499431389266));
#246570=CARTESIAN_POINT('Ctrl Pts',(-52.3805378126143,-45.3951641548607,
-27.153605667294));
#246571=CARTESIAN_POINT('Ctrl Pts',(-52.3513512437753,-45.4759437807972,
-27.1499499950419));
#246572=CARTESIAN_POINT('Ctrl Pts',(-52.3640896356265,-45.439210366248,
-27.1499459628841));
#246573=CARTESIAN_POINT('Ctrl Pts',(-52.3767900903855,-45.4025844806719,
-27.1529187439664));
#246574=CARTESIAN_POINT('Ctrl Pts',(-52.3480894402565,-45.4746884282277,
-27.1499500007674));
#246575=CARTESIAN_POINT('Ctrl Pts',(-52.358361049002,-45.4467890388277,
-27.149949596787));
#246576=CARTESIAN_POINT('Ctrl Pts',(-52.3686148330815,-45.4189361333146,
-27.151673524296));
#246577=CARTESIAN_POINT('Ctrl Pts',(-52.3464615330207,-45.4740496677423,
-27.1499499999556));
#246578=CARTESIAN_POINT('Ctrl Pts',(-52.354091925022,-45.4531300726578,
-27.1499503254651));
#246579=CARTESIAN_POINT('Ctrl Pts',(-52.3621865654577,-45.4322306539423,
-27.1509264737703));
#246580=CARTESIAN_POINT('Ctrl Pts',(-52.34484211086,-45.473387463513,-27.149949999795));
#246581=CARTESIAN_POINT('Ctrl Pts',(-52.3544411585185,-45.4495909622675,
-27.1499505193682));
#246582=CARTESIAN_POINT('Ctrl Pts',(-52.3640275639789,-45.4258258009784,
-27.1512670021823));
#246583=CARTESIAN_POINT('',(-53.1622408850506,-44.6469488027857,-27.4198793594831));
#246584=CARTESIAN_POINT('Ctrl Pts',(-52.3451506921103,-45.473503287774,
-27.1499501432945));
#246585=CARTESIAN_POINT('Ctrl Pts',(-52.3820649490763,-45.3843464938679,
-27.1499647742885));
#246586=CARTESIAN_POINT('Ctrl Pts',(-52.4255740573844,-45.3010011843873,
-27.1640868107759));
#246587=CARTESIAN_POINT('Ctrl Pts',(-52.5068084427536,-45.1823953595046,
-27.2020720172523));
#246588=CARTESIAN_POINT('Ctrl Pts',(-52.53660370576,-45.1439054140081,-27.2175412386481));
#246589=CARTESIAN_POINT('Ctrl Pts',(-52.586580167937,-45.0869019409087,
-27.2442488546962));
#246590=CARTESIAN_POINT('Ctrl Pts',(-52.6041258972165,-45.0680161745429,
-27.2537272597621));
#246591=CARTESIAN_POINT('Ctrl Pts',(-52.631952259695,-45.0396571638826,
-27.2686754446952));
#246592=CARTESIAN_POINT('Ctrl Pts',(-52.6414789512766,-45.0301983315303,
-27.2737797996278));
#246593=CARTESIAN_POINT('Ctrl Pts',(-52.6610625104122,-45.0112249171893,
-27.2842080852999));
#246594=CARTESIAN_POINT('Ctrl Pts',(-52.6725722732524,-45.0003652292174,
-27.290294169548));
#246595=CARTESIAN_POINT('Ctrl Pts',(-52.7525080504857,-44.9263566788015,
-27.3322280681073));
#246596=CARTESIAN_POINT('Ctrl Pts',(-52.8274152663173,-44.8683372625527,
-27.3682550785334));
#246597=CARTESIAN_POINT('Ctrl Pts',(-52.9889951430861,-44.7566940244181,
-27.4166930620214));
#246598=CARTESIAN_POINT('Ctrl Pts',(-53.0756516339733,-44.7024568188154,
-27.4290805984111));
#246599=CARTESIAN_POINT('Ctrl Pts',(-53.1622384085562,-44.6469454777987,
-27.4198761157188));
#246600=CARTESIAN_POINT('Origin',(-53.6334240605191,-45.2802247659028,-28.0338316716305));
#246601=CARTESIAN_POINT('Ctrl Pts',(-54.1729863252367,-45.4155339669028,
-26.8184100191364));
#246602=CARTESIAN_POINT('Ctrl Pts',(-53.4948062719818,-45.0018366342789,
-26.6524889540493));
#246603=CARTESIAN_POINT('Ctrl Pts',(-53.5626783369365,-44.363661901133,
-27.1491860078999));
#246604=CARTESIAN_POINT('Ctrl Pts',(-54.0985832939867,-45.4543288404299,
-26.8878842623322));
#246605=CARTESIAN_POINT('Ctrl Pts',(-53.4663807315788,-44.9982803860136,
-26.6936892350566));
#246606=CARTESIAN_POINT('Ctrl Pts',(-53.5158499791776,-44.4021217230785,
-27.2295107442058));
#246607=CARTESIAN_POINT('Ctrl Pts',(-54.0039121656008,-45.4910386121189,
-26.9442182302923));
#246608=CARTESIAN_POINT('Ctrl Pts',(-53.4359975789415,-44.9961164351359,
-26.7410719889231));
#246609=CARTESIAN_POINT('Ctrl Pts',(-53.4577716218956,-44.446641152384,
-27.2926084953181));
#246610=CARTESIAN_POINT('Ctrl Pts',(-53.7733799776403,-45.5533648819636,
-27.0359103001593));
#246611=CARTESIAN_POINT('Ctrl Pts',(-53.3470483842575,-45.0123168742401,
-26.8487365913724));
#246612=CARTESIAN_POINT('Ctrl Pts',(-53.3195631540916,-44.544459526392,
-27.3849932634619));
#246613=CARTESIAN_POINT('Ctrl Pts',(-53.6402578408342,-45.5778984718822,
-27.0696657788991));
#246614=CARTESIAN_POINT('Ctrl Pts',(-53.2906043022484,-45.0299634766633,
-26.9058257418929));
#246615=CARTESIAN_POINT('Ctrl Pts',(-53.2410272830333,-44.5963709464781,
-27.4125980820349));
#246616=CARTESIAN_POINT('Ctrl Pts',(-53.4944417351013,-45.5914386672807,
-27.0936350023709));
#246617=CARTESIAN_POINT('Ctrl Pts',(-53.2121096349814,-45.0580990514851,
-26.9588617892535));
#246618=CARTESIAN_POINT('Ctrl Pts',(-53.1561130272964,-44.6507276720235,
-27.4206373946492));
#246619=CARTESIAN_POINT('',(-53.5592639447716,-44.3666367581605,-27.1547933762998));
#246620=CARTESIAN_POINT('Origin',(-54.427442714539,-44.7262215362818,-27.496793978795));
#246621=CARTESIAN_POINT('Ctrl Pts',(-53.1622457766273,-44.6469552539754,
-27.4198856202721));
#246622=CARTESIAN_POINT('Ctrl Pts',(-53.1829616413124,-44.6336777614326,
-27.4176857913189));
#246623=CARTESIAN_POINT('Ctrl Pts',(-53.203825483367,-44.620248346138,-27.4142375777492));
#246624=CARTESIAN_POINT('Ctrl Pts',(-53.2246773472487,-44.606676467706,
-27.4094115119876));
#246625=CARTESIAN_POINT('Ctrl Pts',(-53.2420734725691,-44.5953538301051,
-27.4053852606525));
#246626=CARTESIAN_POINT('Ctrl Pts',(-53.2594606276377,-44.5839326590593,
-27.4004000481084));
#246627=CARTESIAN_POINT('Ctrl Pts',(-53.276734970572,-44.5724432363545,
-27.3943871326634));
#246628=CARTESIAN_POINT('Ctrl Pts',(-53.2957250867575,-44.559812627312,
-27.3877769846915));
#246629=CARTESIAN_POINT('Ctrl Pts',(-53.3145785223172,-44.5470989704662,
-27.3799245457684));
#246630=CARTESIAN_POINT('Ctrl Pts',(-53.3331483702287,-44.5343766610789,
-27.3707499894093));
#246631=CARTESIAN_POINT('Ctrl Pts',(-53.3424332941844,-44.5280155063852,
-27.3661627112298));
#246632=CARTESIAN_POINT('Ctrl Pts',(-53.3516472121374,-44.5216527584649,
-27.361245110394));
#246633=CARTESIAN_POINT('Ctrl Pts',(-53.3607713708089,-44.5153011412843,
-27.3559885994396));
#246634=CARTESIAN_POINT('Ctrl Pts',(-53.3659497709643,-44.5116962921602,
-27.353005275922));
#246635=CARTESIAN_POINT('Ctrl Pts',(-53.3713666791296,-44.5079151244326,
-27.3497435082216));
#246636=CARTESIAN_POINT('Ctrl Pts',(-53.3765597693778,-44.504264785144,
-27.3464883543585));
#246637=CARTESIAN_POINT('Ctrl Pts',(-53.3805167212274,-44.5014833551844,
-27.3440080417733));
#246638=CARTESIAN_POINT('Ctrl Pts',(-53.3843446775867,-44.4987785077191,
-27.3415321022123));
#246639=CARTESIAN_POINT('Ctrl Pts',(-53.3878557727717,-44.4962946745248,
-27.339194797945));
#246640=CARTESIAN_POINT('Ctrl Pts',(-53.4040938620753,-44.4848074595393,
-27.3283852489511));
#246641=CARTESIAN_POINT('Ctrl Pts',(-53.4201817297529,-44.4732534524402,
-27.3162930153253));
#246642=CARTESIAN_POINT('Ctrl Pts',(-53.4359540056218,-44.4617216985649,
-27.3028611096342));
#246643=CARTESIAN_POINT('Ctrl Pts',(-53.4428340594993,-44.4566914106963,
-27.2970019529976));
#246644=CARTESIAN_POINT('Ctrl Pts',(-53.4498511634597,-44.4515321157807,
-27.2907002087151));
#246645=CARTESIAN_POINT('Ctrl Pts',(-53.4567248436233,-44.4464263008861,
-27.2841946017466));
#246646=CARTESIAN_POINT('Ctrl Pts',(-53.4636552526535,-44.4412783474158,
-27.2776353036402));
#246647=CARTESIAN_POINT('Ctrl Pts',(-53.4704396513325,-44.4361851635385,
-27.2708689417737));
#246648=CARTESIAN_POINT('Ctrl Pts',(-53.4768392779086,-44.4313447726754,
-27.2641606808037));
#246649=CARTESIAN_POINT('Ctrl Pts',(-53.4786432337058,-44.4299803413208,
-27.2622697257421));
#246650=CARTESIAN_POINT('Ctrl Pts',(-53.4804169154806,-44.428636041392,
-27.2603834997713));
#246651=CARTESIAN_POINT('Ctrl Pts',(-53.4821556626255,-44.4273163903631,
-27.2585081884501));
#246652=CARTESIAN_POINT('Ctrl Pts',(-53.4894649357621,-44.4217688960977,
-27.2506248324929));
#246653=CARTESIAN_POINT('Ctrl Pts',(-53.496801847095,-44.4161533979149,
-27.242244797274));
#246654=CARTESIAN_POINT('Ctrl Pts',(-53.5039434369036,-44.4106261624368,
-27.2335970890786));
#246655=CARTESIAN_POINT('Ctrl Pts',(-53.5105049481577,-44.4055478789221,
-27.2256517945201));
#246656=CARTESIAN_POINT('Ctrl Pts',(-53.5169020275297,-44.4005444852192,
-27.2174809284803));
#246657=CARTESIAN_POINT('Ctrl Pts',(-53.522998259727,-44.3957400324566,
-27.2092754392718));
#246658=CARTESIAN_POINT('Ctrl Pts',(-53.5256916414775,-44.393617372923,
-27.2056501648116));
#246659=CARTESIAN_POINT('Ctrl Pts',(-53.5282004467817,-44.3916302581029,
-27.2022014922256));
#246660=CARTESIAN_POINT('Ctrl Pts',(-53.5309532960349,-44.3894455369061,
-27.1983202529587));
#246661=CARTESIAN_POINT('Ctrl Pts',(-53.5333769026166,-44.387522109873,
-27.1949032125881));
#246662=CARTESIAN_POINT('Ctrl Pts',(-53.5359898668883,-44.3854453842273,
-27.191150857536));
#246663=CARTESIAN_POINT('Ctrl Pts',(-53.5390481116965,-44.3829894685758,
-27.1866366971472));
#246664=CARTESIAN_POINT('Ctrl Pts',(-53.5407261265692,-44.3816419430349,
-27.1841598423676));
#246665=CARTESIAN_POINT('Ctrl Pts',(-53.5425375417721,-44.3801802906758,
-27.1814534500025));
#246666=CARTESIAN_POINT('Ctrl Pts',(-53.5445179248843,-44.3785677202971,
-27.1784452999289));
#246667=CARTESIAN_POINT('Ctrl Pts',(-53.5486210827242,-44.3752266340442,
-27.1722127106478));
#246668=CARTESIAN_POINT('Ctrl Pts',(-53.5517998805691,-44.3725906371767,
-27.1671864609521));
#246669=CARTESIAN_POINT('Ctrl Pts',(-53.5541506530685,-44.3706553907933,
-27.1633939311691));
#246670=CARTESIAN_POINT('Ctrl Pts',(-53.556524588143,-44.3687010760866,
-27.1595640329225));
#246671=CARTESIAN_POINT('Ctrl Pts',(-53.5580541187007,-44.3674611371709,
-27.1569920294027));
#246672=CARTESIAN_POINT('Ctrl Pts',(-53.5587877855783,-44.3669315765437,
-27.1556906963517));
#246673=CARTESIAN_POINT('Ctrl Pts',(-53.5590432140006,-44.3667472083521,
-27.1552376331725));
#246674=CARTESIAN_POINT('Ctrl Pts',(-53.559201727648,-44.3666489657124,
-27.1549384692066));
#246675=CARTESIAN_POINT('Ctrl Pts',(-53.5592639447716,-44.3666367581605,
-27.1547933762998));
#246676=CARTESIAN_POINT('Ctrl Pts',(-53.559279935343,-44.3666167387913,
-27.1547738354693));
#246677=CARTESIAN_POINT('Ctrl Pts',(-53.4929150197559,-45.0016832826959,
-26.6555125209271));
#246678=CARTESIAN_POINT('Ctrl Pts',(-54.1676134446955,-45.4183137084154,
-26.8233719893975));
#246679=CARTESIAN_POINT('Ctrl Pts',(-53.759714509971,-44.159109532608,-26.8641791075324));
#246680=CARTESIAN_POINT('Ctrl Pts',(-53.6168204963237,-44.9093405275666,
-26.4380889960535));
#246681=CARTESIAN_POINT('Ctrl Pts',(-54.3266292023091,-45.3366816698438,
-26.6781230301639));
#246682=CARTESIAN_POINT('Ctrl Pts',(-53.9467562705573,-44.0476837299281,
-26.5065585291096));
#246683=CARTESIAN_POINT('Ctrl Pts',(-53.7163262343164,-44.9073871865944,
-26.1875635549992));
#246684=CARTESIAN_POINT('Ctrl Pts',(-54.4936741569865,-45.3076755243593,
-26.4992996221132));
#246685=CARTESIAN_POINT('Ctrl Pts',(-54.0990511533284,-44.0351983215918,
-26.1331099517669));
#246686=CARTESIAN_POINT('Ctrl Pts',(-53.7768128357869,-44.9677898415763,
-25.9705199042206));
#246687=CARTESIAN_POINT('Ctrl Pts',(-54.6449756149829,-45.3273946390668,
-26.3125400475463));
#246688=CARTESIAN_POINT('',(-53.559279935343,-44.3666167387913,-27.1547738354693));
#246689=CARTESIAN_POINT('Ctrl Pts',(-60.2219860711698,-29.2531258014113,
-26.1331099517669));
#246690=CARTESIAN_POINT('Ctrl Pts',(-60.6535709595361,-28.3658271140614,
-25.9705199042206));
#246691=CARTESIAN_POINT('Ctrl Pts',(-61.5217337387322,-28.7254319115519,
-26.3125400475463));
#246692=CARTESIAN_POINT('Ctrl Pts',(-60.1224375724058,-29.1357973637293,
-26.5091584767853));
#246693=CARTESIAN_POINT('Ctrl Pts',(-60.5674386476715,-28.3657673146916,
-26.1892157116101));
#246694=CARTESIAN_POINT('Ctrl Pts',(-61.3999932287862,-28.6317653934777,
-26.500551642367));
#246695=CARTESIAN_POINT('Ctrl Pts',(-60.0697340205019,-28.9211346043095,
-26.8686373631129));
#246696=CARTESIAN_POINT('Ctrl Pts',(-60.4987668584442,-28.2916785253826,
-26.4414259312258));
#246697=CARTESIAN_POINT('Ctrl Pts',(-61.3023268669242,-28.4910580092523,
-26.6804294767723));
#246698=CARTESIAN_POINT('Ctrl Pts',(-60.0746583928549,-28.6371017026725,
-27.1547738354693));
#246699=CARTESIAN_POINT('Ctrl Pts',(-60.4767911707101,-28.1411147611284,
-26.6555125209271));
#246700=CARTESIAN_POINT('Ctrl Pts',(-61.2484772015156,-28.3235963933842,
-26.8233719893975));
#246701=CARTESIAN_POINT('',(-60.0746608288527,-28.637079928768,-27.1547905454732));
#246702=CARTESIAN_POINT('',(-60.0745809376059,-28.6418766419159,-27.1499500046874));
#246703=CARTESIAN_POINT('Origin',(-60.9428211720509,-28.996706500163,-27.496793978795));
#246704=CARTESIAN_POINT('Ctrl Pts',(-60.844966001754,-27.666686296169,-27.1052376108796));
#246705=CARTESIAN_POINT('Ctrl Pts',(-60.2994052311052,-27.862800659529,
-26.9851894460117));
#246706=CARTESIAN_POINT('Ctrl Pts',(-59.9789660757281,-28.0995786058708,
-27.4232256967097));
#246707=CARTESIAN_POINT('Ctrl Pts',(-60.9625188062383,-27.8006555414775,
-27.0805352245546));
#246708=CARTESIAN_POINT('Ctrl Pts',(-60.3447014319684,-27.9607038681006,
-26.9244775354546));
#246709=CARTESIAN_POINT('Ctrl Pts',(-60.0056441485464,-28.2188680374461,
-27.4213854663284));
#246710=CARTESIAN_POINT('Ctrl Pts',(-61.0541543765889,-27.9302946525346,
-27.0441985004279));
#246711=CARTESIAN_POINT('Ctrl Pts',(-60.3764775334752,-28.0237347066717,
-26.858283774367));
#246712=CARTESIAN_POINT('Ctrl Pts',(-60.0281768266373,-28.3265373252776,
-27.3933984485104));
#246713=CARTESIAN_POINT('Ctrl Pts',(-61.1938025120114,-28.1730269430135,
-26.9370053822956));
#246714=CARTESIAN_POINT('Ctrl Pts',(-60.4367689858647,-28.1111042957933,
-26.7320775605175));
#246715=CARTESIAN_POINT('Ctrl Pts',(-60.0617095819124,-28.5222327395198,
-27.2855146773129));
#246716=CARTESIAN_POINT('Ctrl Pts',(-61.2391009664971,-28.2820540015562,
-26.8673782615866));
#246717=CARTESIAN_POINT('Ctrl Pts',(-60.4637526568036,-28.1314416114958,
-26.6767248536642));
#246718=CARTESIAN_POINT('Ctrl Pts',(-60.0722222978374,-28.6067470756235,
-27.2066250416898));
#246719=CARTESIAN_POINT('Ctrl Pts',(-61.2616496374058,-28.368733778436,
-26.7820215656129));
#246720=CARTESIAN_POINT('Ctrl Pts',(-60.4895512830636,-28.1510794068988,
-26.6321340393296));
#246721=CARTESIAN_POINT('Ctrl Pts',(-60.0775655158368,-28.6712003044384,
-27.1069552801944));
#246722=CARTESIAN_POINT('',(-59.9921334535065,-28.1581281070072,-27.4198788482142));
#246723=CARTESIAN_POINT('Origin',(-60.7731046378674,-28.043511085052,-28.0338316716305));
#246724=CARTESIAN_POINT('Ctrl Pts',(-60.0746608288527,-28.637079928768,
-27.1547905454732));
#246725=CARTESIAN_POINT('Ctrl Pts',(-60.0745597917545,-28.6368564728994,
-27.1552819564429));
#246726=CARTESIAN_POINT('Ctrl Pts',(-60.0743992696367,-28.635573735643,
-27.1570485778493));
#246727=CARTESIAN_POINT('Ctrl Pts',(-60.0741584639655,-28.6332063693261,
-27.1600818130461));
#246728=CARTESIAN_POINT('Ctrl Pts',(-60.0739199748378,-28.6308617770044,
-27.1630858686084));
#246729=CARTESIAN_POINT('Ctrl Pts',(-60.0736028577126,-28.6274531695012,
-27.1673324792244));
#246730=CARTESIAN_POINT('Ctrl Pts',(-60.0731533921911,-28.6229201453569,
-27.1727994271334));
#246731=CARTESIAN_POINT('Ctrl Pts',(-60.0729827771374,-28.6211994301504,
-27.1748746555242));
#246732=CARTESIAN_POINT('Ctrl Pts',(-60.0727927342046,-28.6193163369742,
-27.177125565431));
#246733=CARTESIAN_POINT('Ctrl Pts',(-60.072578963976,-28.6172662809877,
-27.1795502902216));
#246734=CARTESIAN_POINT('Ctrl Pts',(-60.0721368775343,-28.6130266730578,
-27.1845647300795));
#246735=CARTESIAN_POINT('Ctrl Pts',(-60.0717521348559,-28.6096020511089,
-27.188527632882));
#246736=CARTESIAN_POINT('Ctrl Pts',(-60.071415717113,-28.6066382940892,
-27.1919084760572));
#246737=CARTESIAN_POINT('Ctrl Pts',(-60.0710288730816,-28.603230293954,
-27.1957960801764));
#246738=CARTESIAN_POINT('Ctrl Pts',(-60.0707052101654,-28.6004306127975,
-27.1989138452128));
#246739=CARTESIAN_POINT('Ctrl Pts',(-60.0703847997515,-28.5976487042245,
-27.2019560952377));
#246740=CARTESIAN_POINT('Ctrl Pts',(-60.0701357660212,-28.5954865114892,
-27.2043206340894));
#246741=CARTESIAN_POINT('Ctrl Pts',(-60.0698879348767,-28.59333416891,-27.2066392349029));
#246742=CARTESIAN_POINT('Ctrl Pts',(-60.0695992250175,-28.5908999407258,
-27.2092316651229));
#246743=CARTESIAN_POINT('Ctrl Pts',(-60.0687200962936,-28.583487655174,
-27.2171256798202));
#246744=CARTESIAN_POINT('Ctrl Pts',(-60.0678153539134,-28.5761854144752,
-27.2245640965939));
#246745=CARTESIAN_POINT('Ctrl Pts',(-60.0668681916812,-28.568727145558,
-27.2318214504281));
#246746=CARTESIAN_POINT('Ctrl Pts',(-60.06592907555,-28.5613322343037,-27.2390171533641));
#246747=CARTESIAN_POINT('Ctrl Pts',(-60.0649484332206,-28.5537835801611,
-27.2460350541153));
#246748=CARTESIAN_POINT('Ctrl Pts',(-60.063873374386,-28.5457910961666,
-27.2531269287546));
#246749=CARTESIAN_POINT('Ctrl Pts',(-60.0636074376708,-28.543813999777,
-27.2548812419011));
#246750=CARTESIAN_POINT('Ctrl Pts',(-60.0633355367877,-28.5418096082398,
-27.2566399957809));
#246751=CARTESIAN_POINT('Ctrl Pts',(-60.0630564862275,-28.5397732639399,
-27.2584068206655));
#246752=CARTESIAN_POINT('Ctrl Pts',(-60.0605116265829,-28.5212023984059,
-27.2745197478142));
#246753=CARTESIAN_POINT('Ctrl Pts',(-60.0577294240748,-28.5021745059489,
-27.289270645353));
#246754=CARTESIAN_POINT('Ctrl Pts',(-60.054737528402,-28.4828917423689,
-27.3026952770944));
#246755=CARTESIAN_POINT('Ctrl Pts',(-60.0532415805655,-28.4732503605789,
-27.3094075929651));
#246756=CARTESIAN_POINT('Ctrl Pts',(-60.0516935979333,-28.4635449380373,
-27.3157886794781));
#246757=CARTESIAN_POINT('Ctrl Pts',(-60.0500992168557,-28.4537985636733,
-27.3218448706633));
#246758=CARTESIAN_POINT('Ctrl Pts',(-60.0491851062695,-28.4482106499004,
-27.3253170822642));
#246759=CARTESIAN_POINT('Ctrl Pts',(-60.0483032371289,-28.4429277771905,
-27.328501753937));
#246760=CARTESIAN_POINT('Ctrl Pts',(-60.0473767034212,-28.437407468587,
-27.3317127204619));
#246761=CARTESIAN_POINT('Ctrl Pts',(-60.0466871877869,-28.4332993189782,
-27.3341022844918));
#246762=CARTESIAN_POINT('Ctrl Pts',(-60.0459721797416,-28.4290592947978,
-27.3365060899411));
#246763=CARTESIAN_POINT('Ctrl Pts',(-60.0451838338097,-28.4244580371654,
-27.3390462004825));
#246764=CARTESIAN_POINT('Ctrl Pts',(-60.04122942221,-28.401377729628,-27.3517876153646));
#246765=CARTESIAN_POINT('Ctrl Pts',(-60.037005635401,-28.3778607369677,
-27.3629374174089));
#246766=CARTESIAN_POINT('Ctrl Pts',(-60.0325473374862,-28.3541327475903,
-27.372575464053));
#246767=CARTESIAN_POINT('Ctrl Pts',(-60.0280704554034,-28.330305849403,
-27.3822536863609));
#246768=CARTESIAN_POINT('Ctrl Pts',(-60.0233574971758,-28.3062666481107,
-27.3904078485879));
#246769=CARTESIAN_POINT('Ctrl Pts',(-60.018474744767,-28.2822058428692,
-27.3971390011105));
#246770=CARTESIAN_POINT('Ctrl Pts',(-60.0135217812117,-28.2577990572095,
-27.4039669437006));
#246771=CARTESIAN_POINT('Ctrl Pts',(-60.008394606897,-28.2333704035156,
-27.4093309698207));
#246772=CARTESIAN_POINT('Ctrl Pts',(-60.0031874462669,-28.2090737209063,
-27.4133524650949));
#246773=CARTESIAN_POINT('Ctrl Pts',(-59.9995313655727,-28.1920143984598,
-27.4161760598096));
#246774=CARTESIAN_POINT('Ctrl Pts',(-59.9958363978412,-28.1750191601907,
-27.4183381480339));
#246775=CARTESIAN_POINT('Ctrl Pts',(-59.992140178489,-28.1581271757,-27.4198841015071));
#246776=CARTESIAN_POINT('Ctrl Pts',(-59.9921300883295,-28.1581285421428,
-27.4198764587517));
#246777=CARTESIAN_POINT('Ctrl Pts',(-60.320749267504,-27.9079025729579,
-26.9551461919303));
#246778=CARTESIAN_POINT('Ctrl Pts',(-60.9016019229534,-27.7332918440739,
-27.0918908718699));
#246779=CARTESIAN_POINT('Ctrl Pts',(-59.9671190756674,-28.0438219358925,
-27.430351861608));
#246780=CARTESIAN_POINT('Ctrl Pts',(-60.2832184902842,-27.8267324213398,
-27.0122080197432));
#246781=CARTESIAN_POINT('Ctrl Pts',(-60.797359504462,-27.6044866323707,
-27.1200911635279));
#246782=CARTESIAN_POINT('Ctrl Pts',(-59.938658879413,-27.9240778021679,
-27.4136386124499));
#246783=CARTESIAN_POINT('Ctrl Pts',(-60.2363961568897,-27.7190794903775,
-27.0637831794859));
#246784=CARTESIAN_POINT('Ctrl Pts',(-60.6701109845517,-27.4721797090988,
-27.1349070389388));
#246785=CARTESIAN_POINT('Ctrl Pts',(-59.9058848368889,-27.7106911677997,
-27.3473769064724));
#246786=CARTESIAN_POINT('Ctrl Pts',(-60.1427718787375,-27.5165901322075,
-27.1155083247124));
#246787=CARTESIAN_POINT('Ctrl Pts',(-60.445732893452,-27.2815332790988,
-27.1460905313549));
#246788=CARTESIAN_POINT('Ctrl Pts',(-59.8970757353221,-27.633633723506,
-27.3175796146788));
#246789=CARTESIAN_POINT('Ctrl Pts',(-60.1089722005848,-27.4441460460438,
-27.1285847238195));
#246790=CARTESIAN_POINT('Ctrl Pts',(-60.3651652603529,-27.2190774234678,
-27.1480089070405));
#246791=CARTESIAN_POINT('Ctrl Pts',(-59.8946036326632,-27.4917517999077,
-27.2632033505944));
#246792=CARTESIAN_POINT('Ctrl Pts',(-60.0546429227938,-27.3214748378271,
-27.1414548626368));
#246793=CARTESIAN_POINT('Ctrl Pts',(-60.2355854820384,-27.1299960968794,
-27.1494556764824));
#246794=CARTESIAN_POINT('Ctrl Pts',(-59.8950938274304,-27.4408470650292,
-27.2434898253561));
#246795=CARTESIAN_POINT('Ctrl Pts',(-60.0358247291844,-27.2791092809321,
-27.1446544886278));
#246796=CARTESIAN_POINT('Ctrl Pts',(-60.1907197716695,-27.1009384228054,
-27.1497020573719));
#246797=CARTESIAN_POINT('Ctrl Pts',(-59.9062296719677,-27.3411615881386,
-27.2098971118952));
#246798=CARTESIAN_POINT('Ctrl Pts',(-60.0103415930171,-27.2045861847983,
-27.1478520318177));
#246799=CARTESIAN_POINT('Ctrl Pts',(-60.1210111726076,-27.0593551785227,
-27.1498873098043));
#246800=CARTESIAN_POINT('Ctrl Pts',(-59.9107857113893,-27.3055694790947,
-27.198669824241));
#246801=CARTESIAN_POINT('Ctrl Pts',(-60.001831916504,-27.1789090272168,
-27.148638279731));
#246802=CARTESIAN_POINT('Ctrl Pts',(-60.0973641192197,-27.0458156781241,
-27.149918608058));
#246803=CARTESIAN_POINT('Ctrl Pts',(-59.9229334781053,-27.2390491448428,
-27.1813235487183));
#246804=CARTESIAN_POINT('Ctrl Pts',(-59.9908839648439,-27.1343204052552,
-27.1494236542124));
#246805=CARTESIAN_POINT('Ctrl Pts',(-60.0609925652013,-27.0262120682258,
-27.1499421164754));
#246806=CARTESIAN_POINT('Ctrl Pts',(-59.9270276396052,-27.2165132639013,
-27.1756979157175));
#246807=CARTESIAN_POINT('Ctrl Pts',(-59.9871253331188,-27.1194275233503,
-27.1496188303448));
#246808=CARTESIAN_POINT('Ctrl Pts',(-60.0487367021204,-27.0198094186492,
-27.1499460403929));
#246809=CARTESIAN_POINT('Ctrl Pts',(-59.941673312503,-27.1639036353,-27.1653223320947));
#246810=CARTESIAN_POINT('Ctrl Pts',(-59.9855672285123,-27.0877860430869,
-27.1498212851493));
#246811=CARTESIAN_POINT('Ctrl Pts',(-60.030127890022,-27.0104881940086,
-27.1499490074433));
#246812=CARTESIAN_POINT('Ctrl Pts',(-59.9471188165433,-27.1448852112603,
-27.1619692558456));
#246813=CARTESIAN_POINT('Ctrl Pts',(-59.9852791191255,-27.0765645589215,
-27.1498709642282));
#246814=CARTESIAN_POINT('Ctrl Pts',(-60.0238841822655,-27.0074242175497,
-27.1499495102509));
#246815=CARTESIAN_POINT('Ctrl Pts',(-59.9575500425786,-27.1105560503329,
-27.1572535611545));
#246816=CARTESIAN_POINT('Ctrl Pts',(-59.98589660914,-27.0569404883559,-27.149919618661));
#246817=CARTESIAN_POINT('Ctrl Pts',(-60.0144468595299,-27.0029333040085,
-27.1499498834281));
#246818=CARTESIAN_POINT('Ctrl Pts',(-59.9613951148011,-27.0981712484174,
-27.1557336710108));
#246819=CARTESIAN_POINT('Ctrl Pts',(-59.9862725028326,-27.0499509885438,
-27.1499315299619));
#246820=CARTESIAN_POINT('Ctrl Pts',(-60.0112896752839,-27.0014538829912,
-27.1499499446124));
#246821=CARTESIAN_POINT('Ctrl Pts',(-59.9684546972765,-27.0763123017486,
-27.1536056672944));
#246822=CARTESIAN_POINT('Ctrl Pts',(-59.9874571335005,-27.0378634826494,
-27.1499431389266));
#246823=CARTESIAN_POINT('Ctrl Pts',(-60.0065280454809,-26.999274517649,
-27.1499499883959));
#246824=CARTESIAN_POINT('Ctrl Pts',(-59.9710516202097,-27.0684152991668,
-27.1529187439602));
#246825=CARTESIAN_POINT('Ctrl Pts',(-59.9879694545663,-27.0335363094633,
-27.149945962884));
#246826=CARTESIAN_POINT('Ctrl Pts',(-60.0049364978137,-26.9985544597188,
-27.1499499950418));
#246827=CARTESIAN_POINT('Ctrl Pts',(-59.9768332047617,-27.0510721549069,
-27.1516735242969));
#246828=CARTESIAN_POINT('Ctrl Pts',(-59.9892776628721,-27.0241266562837,
-27.149949596787));
#246829=CARTESIAN_POINT('Ctrl Pts',(-60.001742386112,-26.9971356846468,
-27.1499500007674));
#246830=CARTESIAN_POINT('Ctrl Pts',(-59.9816883788974,-27.0371260374492,
-27.1509264737607));
#246831=CARTESIAN_POINT('Ctrl Pts',(-59.9907427244201,-27.0166241416866,
-27.1499503254652));
#246832=CARTESIAN_POINT('Ctrl Pts',(-60.0001396099956,-26.9964362522719,
-27.1499499999556));
#246833=CARTESIAN_POINT('Ctrl Pts',(-59.9784612462896,-27.0429567353391,
-27.1512670021965));
#246834=CARTESIAN_POINT('Ctrl Pts',(-59.9884871407403,-27.0193736162006,
-27.1499505193683));
#246835=CARTESIAN_POINT('Ctrl Pts',(-59.998526256503,-26.9957593969819,
-27.149949999795));
#246836=CARTESIAN_POINT('Ctrl Pts',(-59.9921299933151,-28.1581286133368,
-27.4198761139792));
#246837=CARTESIAN_POINT('Ctrl Pts',(-59.9701579252025,-28.0576651497413,
-27.4290779346156));
#246838=CARTESIAN_POINT('Ctrl Pts',(-59.9472412910225,-27.9580348996117,
-27.4166918460736));
#246839=CARTESIAN_POINT('Ctrl Pts',(-59.9207601538973,-27.8131235425062,
-27.3803603832272));
#246840=CARTESIAN_POINT('Ctrl Pts',(-59.9132588707421,-27.7653999402845,
-27.365309683848));
#246841=CARTESIAN_POINT('Ctrl Pts',(-59.9047658007748,-27.6938927948674,
-27.3402656049488));
#246842=CARTESIAN_POINT('Ctrl Pts',(-59.9023893111735,-27.6700639391975,
-27.3315068947973));
#246843=CARTESIAN_POINT('Ctrl Pts',(-59.8995467614903,-27.6341899840966,
-27.3180027950516));
#246844=CARTESIAN_POINT('Ctrl Pts',(-59.8987191770273,-27.6222100030513,
-27.3134404804139));
#246845=CARTESIAN_POINT('Ctrl Pts',(-59.8973051909472,-27.5981804781832,
-27.3042363771492));
#246846=CARTESIAN_POINT('Ctrl Pts',(-59.8967949914569,-27.588104634047,
-27.3003548689801));
#246847=CARTESIAN_POINT('Ctrl Pts',(-59.8919058191163,-27.4614630196987,
-27.2515720110604));
#246848=CARTESIAN_POINT('Ctrl Pts',(-59.8984591636505,-27.363138339122,
-27.2147413151307));
#246849=CARTESIAN_POINT('Ctrl Pts',(-59.9337022752968,-27.1747284561612,
-27.1640852704678));
#246850=CARTESIAN_POINT('Ctrl Pts',(-59.9618895982155,-27.0850253725664,
-27.1499500046719));
#246851=CARTESIAN_POINT('Ctrl Pts',(-59.9987583566445,-26.9958774289692,
-27.1499500000015));
#246852=CARTESIAN_POINT('Ctrl Pts',(-51.0753935148582,-44.2778743810374,
-38.2852384570399));
#246853=CARTESIAN_POINT('Ctrl Pts',(-51.221272714641,-44.0620551258768,
-38.2881244881786));
#246854=CARTESIAN_POINT('Ctrl Pts',(-51.322393361958,-43.857597022718,-38.4139756691106));
#246855=CARTESIAN_POINT('Ctrl Pts',(-50.5589168178961,-43.9265466949758,
-38.1296723017668));
#246856=CARTESIAN_POINT('Ctrl Pts',(-50.70387613966,-43.7144228107189,-38.13287636152));
#246857=CARTESIAN_POINT('Ctrl Pts',(-50.804491208013,-43.5123432497905,
-38.2555902237865));
#246858=CARTESIAN_POINT('Ctrl Pts',(-50.0437957213916,-43.5725655138355,
-37.9740538460248));
#246859=CARTESIAN_POINT('Ctrl Pts',(-50.18735261211,-43.3638960195065,-37.9774448600074));
#246860=CARTESIAN_POINT('Ctrl Pts',(-50.2878807263347,-43.164578596265,
-38.0971582664596));
#246861=CARTESIAN_POINT('Ctrl Pts',(-49.530715885079,-43.2159674697984,
-37.8185383057006));
#246862=CARTESIAN_POINT('Ctrl Pts',(-49.6723958234993,-43.010504571894,
-37.8219861814962));
#246863=CARTESIAN_POINT('Ctrl Pts',(-49.7732408306752,-42.814351716493,
-37.9388383832698));
#246864=CARTESIAN_POINT('',(-49.8728085526386,-42.8820630203836,-37.9694624807979));
#246865=CARTESIAN_POINT('Ctrl Pts',(-51.3131710686973,-43.8514487258803,
-38.411155249868));
#246866=CARTESIAN_POINT('Ctrl Pts',(-50.8316561824108,-43.5304148924606,
-38.2638929263568));
#246867=CARTESIAN_POINT('Ctrl Pts',(-50.3514791746876,-43.2073574749185,
-38.1166580156441));
#246868=CARTESIAN_POINT('Ctrl Pts',(-49.8728085497775,-42.8820630221025,
-37.9694624863033));
#246869=CARTESIAN_POINT('',(-49.5640573010087,-43.2391345629747,-37.8286434305113));
#246870=CARTESIAN_POINT('Ctrl Pts',(-49.5640573010554,-43.2391345629941,
-37.8286434303062));
#246871=CARTESIAN_POINT('Ctrl Pts',(-49.8494633692686,-43.3573536272316,
-37.904735709135));
#246872=CARTESIAN_POINT('Ctrl Pts',(-50.135471903199,-43.4758222409351,
-37.9876583178626));
#246873=CARTESIAN_POINT('Ctrl Pts',(-50.6978706344543,-43.7087754228824,
-38.1635076732467));
#246874=CARTESIAN_POINT('Ctrl Pts',(-50.9785707207733,-43.8250452056,-38.257673825788));
#246875=CARTESIAN_POINT('Ctrl Pts',(-51.2549749806985,-43.9395355987587,
-38.3573338134652));
#246876=CARTESIAN_POINT('',(-49.5398530052707,-43.2223193698252,-37.8213061206858));
#246877=CARTESIAN_POINT('',(-49.5398418208422,-43.2223097035821,-37.82130434093));
#246878=CARTESIAN_POINT('Ctrl Pts',(-49.8728085512757,-42.8820630232987,
-37.969462486706));
#246879=CARTESIAN_POINT('Ctrl Pts',(-49.835317068268,-42.9487641223396,
-37.9279035533955));
#246880=CARTESIAN_POINT('Ctrl Pts',(-49.7850972385136,-43.010927571904,
-37.8943460529194));
#246881=CARTESIAN_POINT('Ctrl Pts',(-49.6691607843692,-43.1241681864113,
-37.8451396851236));
#246882=CARTESIAN_POINT('Ctrl Pts',(-49.6055190626502,-43.1745010780307,
-37.8290666430855));
#246883=CARTESIAN_POINT('Ctrl Pts',(-49.5398550048227,-43.2223190381248,
-37.8213083592913));
#246884=CARTESIAN_POINT('Ctrl Pts',(-56.0567428479854,-26.4451399126818,
-36.7328353710964));
#246885=CARTESIAN_POINT('Ctrl Pts',(-56.9256533237087,-26.804455625982,
-37.0750745754352));
#246886=CARTESIAN_POINT('Ctrl Pts',(-56.5501269894349,-27.7316757551251,
-37.0532039630469));
#246887=CARTESIAN_POINT('Ctrl Pts',(-56.0161159413416,-26.4316774197765,
-36.8592602097566));
#246888=CARTESIAN_POINT('Ctrl Pts',(-56.8812242910574,-26.792771568599,
-37.2001343692902));
#246889=CARTESIAN_POINT('Ctrl Pts',(-56.4634891944676,-27.7025207485233,
-37.3037739683117));
#246890=CARTESIAN_POINT('Ctrl Pts',(-55.9865950568036,-26.3938324397214,
-36.9856616450977));
#246891=CARTESIAN_POINT('Ctrl Pts',(-56.8463391109411,-26.7573474025772,
-37.3259290836403));
#246892=CARTESIAN_POINT('Ctrl Pts',(-56.3975727115578,-27.6239813543799,
-37.5536697174369));
#246893=CARTESIAN_POINT('Ctrl Pts',(-55.9639108205415,-26.3064676587972,
-37.1605584951606));
#246894=CARTESIAN_POINT('Ctrl Pts',(-56.8116611688153,-26.6724967553174,
-37.5031641308945));
#246895=CARTESIAN_POINT('Ctrl Pts',(-56.3372700934347,-27.4430605475982,
-37.8969608391351));
#246896=CARTESIAN_POINT('Ctrl Pts',(-55.9598677494703,-26.2742284930919,
-37.2140109224323));
#246897=CARTESIAN_POINT('Ctrl Pts',(-56.8032368383072,-26.6410057827481,
-37.5576570896612));
#246898=CARTESIAN_POINT('Ctrl Pts',(-56.3237384842937,-27.3763245447103,
-38.0014758126155));
#246899=CARTESIAN_POINT('Ctrl Pts',(-55.9584332691836,-26.2015366731774,
-37.3161182781239));
#246900=CARTESIAN_POINT('Ctrl Pts',(-56.7915392176745,-26.5690973896552,
-37.6629529996084));
#246901=CARTESIAN_POINT('Ctrl Pts',(-56.3079807609824,-27.2255973278124,
-38.1999509624373));
#246902=CARTESIAN_POINT('Ctrl Pts',(-55.9611416957481,-26.1605953720209,
-37.3652108762889));
#246903=CARTESIAN_POINT('Ctrl Pts',(-56.7882693648106,-26.5282588226261,
-37.7141900108042));
#246904=CARTESIAN_POINT('Ctrl Pts',(-56.3058507535083,-27.1405858754377,
-38.2947398804766));
#246905=CARTESIAN_POINT('Ctrl Pts',(-55.9735854550226,-26.0733128348902,
-37.4552148376231));
#246906=CARTESIAN_POINT('Ctrl Pts',(-56.787283226926,-26.4397664909511,
-37.8097324411522));
#246907=CARTESIAN_POINT('Ctrl Pts',(-56.3133653432169,-26.9588185181872,
-38.4667780711462));
#246908=CARTESIAN_POINT('Ctrl Pts',(-55.9832537988535,-26.0268975082167,
-37.4964217183786));
#246909=CARTESIAN_POINT('Ctrl Pts',(-56.7894489037504,-26.3921445172251,
-37.8543040547116));
#246910=CARTESIAN_POINT('Ctrl Pts',(-56.3228479854743,-26.8619028223475,
-38.5446064466135));
#246911=CARTESIAN_POINT('Ctrl Pts',(-56.0096187269497,-25.9285721559953,
-37.5713719240169));
#246912=CARTESIAN_POINT('Ctrl Pts',(-56.7994567234388,-26.2891407664831,
-37.93719686714));
#246913=CARTESIAN_POINT('Ctrl Pts',(-56.3532675293309,-26.6560036746519,
-38.6838766227473));
#246914=CARTESIAN_POINT('Ctrl Pts',(-56.0264911179296,-25.876428712841,
-37.6051403493443));
#246915=CARTESIAN_POINT('Ctrl Pts',(-56.8073578500169,-26.2335499771157,
-37.975588088565));
#246916=CARTESIAN_POINT('Ctrl Pts',(-56.3744282312934,-26.5465004149421,
-38.745296875714));
#246917=CARTESIAN_POINT('Ctrl Pts',(-56.0847411249187,-25.7176419731692,
-37.6904448613398));
#246918=CARTESIAN_POINT('Ctrl Pts',(-56.8397912948059,-26.061143575332,
-38.0745256106056));
#246919=CARTESIAN_POINT('Ctrl Pts',(-56.4527962216696,-26.2131202154147,
-38.896893054692));
#246920=CARTESIAN_POINT('Ctrl Pts',(-56.1352426205228,-25.6049974448028,
-37.7283114705867));
#246921=CARTESIAN_POINT('Ctrl Pts',(-56.8741681320632,-25.932461502415,
-38.1225595342041));
#246922=CARTESIAN_POINT('Ctrl Pts',(-56.5266192379674,-25.9765570154852,
-38.9582311572884));
#246923=CARTESIAN_POINT('Ctrl Pts',(-56.1839719359073,-25.4898819665406,
-37.7383677470617));
#246924=CARTESIAN_POINT('Ctrl Pts',(-56.9226955196534,-25.8032369518573,
-38.135248020605));
#246925=CARTESIAN_POINT('Ctrl Pts',(-56.6168337454475,-25.7433245796562,
-38.9744601000404));
#246926=CARTESIAN_POINT('',(-56.5352472331774,-27.7260285737871,-37.0969113483379));
#246927=CARTESIAN_POINT('',(-56.0497678863462,-26.4425442437853,-36.7548912050127));
#246928=CARTESIAN_POINT('Origin',(-55.6670844539814,-27.3664237762966,-36.7548912050122));
#246929=CARTESIAN_POINT('',(-56.1804995572509,-25.4980753298431,-37.7376053587295));
#246930=CARTESIAN_POINT('Ctrl Pts',(-56.1804996992808,-25.4980753614798,
-37.7376050690768));
#246931=CARTESIAN_POINT('Ctrl Pts',(-56.1721547081557,-25.517745210166,
-37.7356615392445));
#246932=CARTESIAN_POINT('Ctrl Pts',(-56.1633474000913,-25.5383093620459,
-37.7328132500983));
#246933=CARTESIAN_POINT('Ctrl Pts',(-56.1541372930473,-25.5597695621204,
-37.7288569014977));
#246934=CARTESIAN_POINT('Ctrl Pts',(-56.1514769713159,-25.5659682996971,
-37.7277141178026));
#246935=CARTESIAN_POINT('Ctrl Pts',(-56.1487833323961,-25.5722416757009,
-37.7264788095946));
#246936=CARTESIAN_POINT('Ctrl Pts',(-56.1460585738842,-25.5785894156077,
-37.725145914588));
#246937=CARTESIAN_POINT('Ctrl Pts',(-56.1399796001049,-25.5927513107933,
-37.7221722074649));
#246938=CARTESIAN_POINT('Ctrl Pts',(-56.133753323915,-25.6072872660305,
-37.7187172178508));
#246939=CARTESIAN_POINT('Ctrl Pts',(-56.127401266824,-25.6221863641009,
-37.7147184532386));
#246940=CARTESIAN_POINT('Ctrl Pts',(-56.1242252382785,-25.6296359131361,
-37.7127190709326));
#246941=CARTESIAN_POINT('Ctrl Pts',(-56.121017807697,-25.6371762469106,
-37.7105836624425));
#246942=CARTESIAN_POINT('Ctrl Pts',(-56.117782435604,-25.6448052112892,
-37.7083042395931));
#246943=CARTESIAN_POINT('Ctrl Pts',(-56.1161647495575,-25.6486196934784,
-37.7071645281684));
#246944=CARTESIAN_POINT('Ctrl Pts',(-56.1145400807257,-25.6524563334436,
-37.7059888081935));
#246945=CARTESIAN_POINT('Ctrl Pts',(-56.1129088768668,-25.6563148191995,
-37.704776053173));
#246946=CARTESIAN_POINT('Ctrl Pts',(-56.1119212824668,-25.6586508968786,
-37.7040418040107));
#246947=CARTESIAN_POINT('Ctrl Pts',(-56.1106283545974,-25.6617120181857,
-37.7030640373722));
#246948=CARTESIAN_POINT('Ctrl Pts',(-56.1095810891675,-25.6641951359811,
-37.7022571329218));
#246949=CARTESIAN_POINT('Ctrl Pts',(-56.1088985924495,-25.6658133692363,
-37.7017312780396));
#246950=CARTESIAN_POINT('Ctrl Pts',(-56.1083201206434,-25.667186413911,
-37.7012794811119));
#246951=CARTESIAN_POINT('Ctrl Pts',(-56.1079961185751,-25.6679554802017,
-37.7010256371487));
#246952=CARTESIAN_POINT('Ctrl Pts',(-56.1047114345681,-25.6757521580389,
-37.6984522054096));
#246953=CARTESIAN_POINT('Ctrl Pts',(-56.1008359754091,-25.6849538000702,
-37.6952903021413));
#246954=CARTESIAN_POINT('Ctrl Pts',(-56.0964078629411,-25.6955756054257,
-37.6913867676171));
#246955=CARTESIAN_POINT('Ctrl Pts',(-56.0919797504732,-25.7061974107812,
-37.687483233093));
#246956=CARTESIAN_POINT('Ctrl Pts',(-56.0869979055547,-25.7182397591171,
-37.6828377562645));
#246957=CARTESIAN_POINT('Ctrl Pts',(-56.0815361707356,-25.7316992647335,
-37.6772557977095));
#246958=CARTESIAN_POINT('Ctrl Pts',(-56.0767092572323,-25.7435943624561,
-37.6723226341605));
#246959=CARTESIAN_POINT('Ctrl Pts',(-56.0714975515571,-25.7565942408721,
-37.6666519605074));
#246960=CARTESIAN_POINT('Ctrl Pts',(-56.0659762650254,-25.7706842877089,
-37.6600785155475));
#246961=CARTESIAN_POINT('Ctrl Pts',(-56.0621264069709,-25.7805089327426,
-37.6554950131556));
#246962=CARTESIAN_POINT('Ctrl Pts',(-56.0581267025653,-25.7908632519376,
-37.6504721261128));
#246963=CARTESIAN_POINT('Ctrl Pts',(-56.0540156952128,-25.8017372274691,
-37.6449482157837));
#246964=CARTESIAN_POINT('Ctrl Pts',(-56.0523569770774,-25.8061246826281,
-37.6427194165004));
#246965=CARTESIAN_POINT('Ctrl Pts',(-56.0505076302188,-25.811057589218,
-37.6401707669867));
#246966=CARTESIAN_POINT('Ctrl Pts',(-56.0487318534611,-25.8158450653948,
-37.637648186208));
#246967=CARTESIAN_POINT('Ctrl Pts',(-56.0477552145813,-25.8184780739365,
-37.6362608212391));
#246968=CARTESIAN_POINT('Ctrl Pts',(-56.0468004020449,-25.8210673534648,
-37.6348821415423));
#246969=CARTESIAN_POINT('Ctrl Pts',(-56.0459080583341,-25.8234999233763,
-37.6335753185341));
#246970=CARTESIAN_POINT('Ctrl Pts',(-56.045160120874,-25.8255388352205,
-37.6324799761569));
#246971=CARTESIAN_POINT('Ctrl Pts',(-56.0444554474835,-25.8274690560493,
-37.6314343381085));
#246972=CARTESIAN_POINT('Ctrl Pts',(-56.0438170325454,-25.8292240855981,
-37.6304777193087));
#246973=CARTESIAN_POINT('Ctrl Pts',(-56.0362567591205,-25.8500075956098,
-37.6191491941467));
#246974=CARTESIAN_POINT('Ctrl Pts',(-56.02931845791,-25.8701426530822,-37.6073098766025));
#246975=CARTESIAN_POINT('Ctrl Pts',(-56.0229752198237,-25.8895467790827,
-37.5951388123388));
#246976=CARTESIAN_POINT('Ctrl Pts',(-56.0162785047191,-25.9100322002368,
-37.5822895153734));
#246977=CARTESIAN_POINT('Ctrl Pts',(-56.0102448833575,-25.9297031511995,
-37.5690703868155));
#246978=CARTESIAN_POINT('Ctrl Pts',(-56.0048282449515,-25.9484996069876,
-37.5556484966893));
#246979=CARTESIAN_POINT('Ctrl Pts',(-56.0019374570599,-25.9585310255028,
-37.5484854124016));
#246980=CARTESIAN_POINT('Ctrl Pts',(-55.9992221728258,-25.9683139641521,
-37.5412638620756));
#246981=CARTESIAN_POINT('Ctrl Pts',(-55.9966740556322,-25.9778429475711,
-37.534004721751));
#246982=CARTESIAN_POINT('Ctrl Pts',(-55.9951913800419,-25.9833875870214,
-37.5297808382527));
#246983=CARTESIAN_POINT('Ctrl Pts',(-55.9937630386758,-25.9888492806145,
-37.5255438327704));
#246984=CARTESIAN_POINT('Ctrl Pts',(-55.9923857319884,-25.9942300976549,
-37.5212950898624));
#246985=CARTESIAN_POINT('Ctrl Pts',(-55.9880037727898,-26.011349393555,
-37.5077775354653));
#246986=CARTESIAN_POINT('Ctrl Pts',(-55.9842072046152,-26.0274324169427,
-37.4943285285434));
#246987=CARTESIAN_POINT('Ctrl Pts',(-55.9808899258191,-26.0426836271918,
-37.4809469087161));
#246988=CARTESIAN_POINT('Ctrl Pts',(-55.9774338122668,-26.0585731311112,
-37.4670052413193));
#246989=CARTESIAN_POINT('Ctrl Pts',(-55.974498085135,-26.0735596866835,
-37.4531366392436));
#246990=CARTESIAN_POINT('Ctrl Pts',(-55.9719986222037,-26.087847946888,
-37.4393035224131));
#246991=CARTESIAN_POINT('Ctrl Pts',(-55.9702448851522,-26.0978732411258,
-37.4295975774998));
#246992=CARTESIAN_POINT('Ctrl Pts',(-55.9687066805805,-26.1075541977658,
-37.4199083357066));
#246993=CARTESIAN_POINT('Ctrl Pts',(-55.9673642825326,-26.1169544197451,
-37.4102131602444));
#246994=CARTESIAN_POINT('Ctrl Pts',(-55.9672678347631,-26.1176298009733,
-37.4095165873842));
#246995=CARTESIAN_POINT('Ctrl Pts',(-55.9671724168607,-26.1183037484222,
-37.4088199099095));
#246996=CARTESIAN_POINT('Ctrl Pts',(-55.9670780227245,-26.1189762775923,
-37.4081231265292));
#246997=CARTESIAN_POINT('Ctrl Pts',(-55.9648434489261,-26.1348969281966,
-37.3916283107813));
#246998=CARTESIAN_POINT('Ctrl Pts',(-55.9630287311143,-26.1509346460944,
-37.3741059408746));
#246999=CARTESIAN_POINT('Ctrl Pts',(-55.96170828606,-26.1668761819019,-37.3556204411724));
#247000=CARTESIAN_POINT('Ctrl Pts',(-55.9603820323537,-26.1828878446978,
-37.3370536235569));
#247001=CARTESIAN_POINT('Ctrl Pts',(-55.9595544937755,-26.1988023789265,
-37.3175151190445));
#247002=CARTESIAN_POINT('Ctrl Pts',(-55.9592940442026,-26.2143746264578,
-37.2971137790707));
#247003=CARTESIAN_POINT('Ctrl Pts',(-55.9591607998138,-26.222341291868,
-37.2866765798698));
#247004=CARTESIAN_POINT('Ctrl Pts',(-55.9591758576328,-26.230217912011,
-37.2760142599166));
#247005=CARTESIAN_POINT('Ctrl Pts',(-55.9593475633682,-26.2379689077822,
-37.2651458023614));
#247006=CARTESIAN_POINT('Ctrl Pts',(-55.9598305616365,-26.2597720090362,
-37.2345734620393));
#247007=CARTESIAN_POINT('Ctrl Pts',(-55.9615201312929,-26.2807531775857,
-37.2022137984117));
#247008=CARTESIAN_POINT('Ctrl Pts',(-55.964565507656,-26.3005184935725,
-37.1680104276273));
#247009=CARTESIAN_POINT('Ctrl Pts',(-55.9657901137843,-26.3084665184464,
-37.1542565750731));
#247010=CARTESIAN_POINT('Ctrl Pts',(-55.9672335016317,-26.3162182494181,
-37.1402047360869));
#247011=CARTESIAN_POINT('Ctrl Pts',(-55.9689034868341,-26.3237494563216,
-37.1258518969158));
#247012=CARTESIAN_POINT('Ctrl Pts',(-55.9697156062902,-26.3274119077281,
-37.1188720626497));
#247013=CARTESIAN_POINT('Ctrl Pts',(-55.9705815899045,-26.3310227930614,
-37.111820163739));
#247014=CARTESIAN_POINT('Ctrl Pts',(-55.9715024848901,-26.3345790848028,
-37.1046968313216));
#247015=CARTESIAN_POINT('Ctrl Pts',(-55.9751208331207,-26.3485523413963,
-37.0767080837981));
#247016=CARTESIAN_POINT('Ctrl Pts',(-55.9795661956742,-26.3615529551416,
-37.0478335973107));
#247017=CARTESIAN_POINT('Ctrl Pts',(-55.9848552614668,-26.3733867099384,
-37.0182655556123));
#247018=CARTESIAN_POINT('Ctrl Pts',(-55.9901546423669,-26.3852435437551,
-36.9886398482424));
#247019=CARTESIAN_POINT('Ctrl Pts',(-55.9963009301748,-26.3959285868322,
-36.9583183373182));
#247020=CARTESIAN_POINT('Ctrl Pts',(-56.0032806792625,-26.4052809700527,
-36.9275198794518));
#247021=CARTESIAN_POINT('Ctrl Pts',(-56.0102641509324,-26.4146383412771,
-36.8967049955237));
#247022=CARTESIAN_POINT('Ctrl Pts',(-56.0180818130719,-26.4226612919738,
-36.8654132065517));
#247023=CARTESIAN_POINT('Ctrl Pts',(-56.0266918657886,-26.4292285506241,
-36.8338816445531));
#247024=CARTESIAN_POINT('Ctrl Pts',(-56.0338493648503,-26.4346878839377,
-36.8076695953536));
#247025=CARTESIAN_POINT('Ctrl Pts',(-56.041553878962,-26.4391418905252,
-36.7812923423983));
#247026=CARTESIAN_POINT('Ctrl Pts',(-56.0497678863463,-26.4425442437853,
-36.7548912050128));
#247027=CARTESIAN_POINT('Ctrl Pts',(-56.3299706459847,-27.1806933304988,
-38.1886114270112));
#247028=CARTESIAN_POINT('Ctrl Pts',(-56.3437769035186,-27.1393066339906,
-38.193039662463));
#247029=CARTESIAN_POINT('Ctrl Pts',(-56.3564803637532,-27.0977146430855,
-38.1960409587767));
#247030=CARTESIAN_POINT('Ctrl Pts',(-56.3680979352093,-27.056004561509,
-38.1976404253347));
#247031=CARTESIAN_POINT('Ctrl Pts',(-56.3800510880585,-27.0130896560733,
-38.1992860935639));
#247032=CARTESIAN_POINT('Ctrl Pts',(-56.3908561640652,-26.9700488132131,
-38.1994477244899));
#247033=CARTESIAN_POINT('Ctrl Pts',(-56.4005166943456,-26.9269475570461,
-38.1981091053726));
#247034=CARTESIAN_POINT('Ctrl Pts',(-56.4040961557844,-26.9109774932987,
-38.1976131144309));
#247035=CARTESIAN_POINT('Ctrl Pts',(-56.4075182298872,-26.8949989247735,
-38.196910746293));
#247036=CARTESIAN_POINT('Ctrl Pts',(-56.4107820091105,-26.8790146182937,
-38.1959998501665));
#247037=CARTESIAN_POINT('Ctrl Pts',(-56.4197273242927,-26.8352050804409,
-38.1935032802724));
#247038=CARTESIAN_POINT('Ctrl Pts',(-56.4274760433765,-26.7913422802906,
-38.189480689052));
#247039=CARTESIAN_POINT('Ctrl Pts',(-56.4339768310141,-26.7474071238096,
-38.1839506306335));
#247040=CARTESIAN_POINT('Ctrl Pts',(-56.4344734020574,-26.7440510802489,
-38.1835282099929));
#247041=CARTESIAN_POINT('Ctrl Pts',(-56.4349626672844,-26.7406946136967,
-38.1830969864374));
#247042=CARTESIAN_POINT('Ctrl Pts',(-56.4354445914514,-26.7373377156824,
-38.1826569655605));
#247043=CARTESIAN_POINT('Ctrl Pts',(-56.4419501218732,-26.6920226979891,
-38.1767170907896));
#247044=CARTESIAN_POINT('Ctrl Pts',(-56.4470910724675,-26.6468479021783,
-38.1691966063775));
#247045=CARTESIAN_POINT('Ctrl Pts',(-56.450788998755,-26.6017985919294,
-38.1601708188183));
#247046=CARTESIAN_POINT('Ctrl Pts',(-56.4531572262878,-26.5729480934145,
-38.1543905200937));
#247047=CARTESIAN_POINT('Ctrl Pts',(-56.4549325771593,-26.5441489691068,
-38.1479926699768));
#247048=CARTESIAN_POINT('Ctrl Pts',(-56.4560836745012,-26.5153977768571,
-38.14100084909));
#247049=CARTESIAN_POINT('Ctrl Pts',(-56.4570386769814,-26.4915444858214,
-38.1352001178704));
#247050=CARTESIAN_POINT('Ctrl Pts',(-56.4575638982276,-26.4677219169545,
-38.1289906679363));
#247051=CARTESIAN_POINT('Ctrl Pts',(-56.4576378137927,-26.4439320606186,
-38.1223923804602));
#247052=CARTESIAN_POINT('Ctrl Pts',(-56.4576780029057,-26.4309971229861,
-38.1188047826295));
#247053=CARTESIAN_POINT('Ctrl Pts',(-56.4575863209636,-26.4180682023607,
-38.1151026029789));
#247054=CARTESIAN_POINT('Ctrl Pts',(-56.4573583944686,-26.4051487944763,
-38.1112876037085));
#247055=CARTESIAN_POINT('Ctrl Pts',(-56.4570348307297,-26.3868084434738,
-38.1058718426829));
#247056=CARTESIAN_POINT('Ctrl Pts',(-56.4564370919895,-26.3684842352767,
-38.1002302193718));
#247057=CARTESIAN_POINT('Ctrl Pts',(-56.4555535507852,-26.350174320246,
-38.0943733011292));
#247058=CARTESIAN_POINT('Ctrl Pts',(-56.4550955081205,-26.340682151426,
-38.0913369759125));
#247059=CARTESIAN_POINT('Ctrl Pts',(-56.4545387351896,-26.3308044692514,
-38.0881165337714));
#247060=CARTESIAN_POINT('Ctrl Pts',(-56.4539112632845,-26.321149637431,
-38.0849073026169));
#247061=CARTESIAN_POINT('Ctrl Pts',(-56.4533283735237,-26.312180785495,
-38.0819260886932));
#247062=CARTESIAN_POINT('Ctrl Pts',(-56.4526850619369,-26.3034039575018,
-38.0789551544803));
#247063=CARTESIAN_POINT('Ctrl Pts',(-56.4520336712243,-26.2952855196118,
-38.0761685452557));
#247064=CARTESIAN_POINT('Ctrl Pts',(-56.4489043128688,-26.2562835796778,
-38.0627813435463));
#247065=CARTESIAN_POINT('Ctrl Pts',(-56.444386387158,-26.217066609373,-38.0483345530097));
#247066=CARTESIAN_POINT('Ctrl Pts',(-56.4383206844836,-26.1776021530648,
-38.032981847176));
#247067=CARTESIAN_POINT('Ctrl Pts',(-56.4338992703069,-26.1488357073674,
-38.0217909473136));
#247068=CARTESIAN_POINT('Ctrl Pts',(-56.4286554571048,-26.1199385485611,
-38.0101193157026));
#247069=CARTESIAN_POINT('Ctrl Pts',(-56.4225389178063,-26.0909056213828,
-37.998038048118));
#247070=CARTESIAN_POINT('Ctrl Pts',(-56.4213234888835,-26.0851364343173,
-37.9956373569215));
#247071=CARTESIAN_POINT('Ctrl Pts',(-56.4200733065636,-26.0793629877505,
-37.9932198357306));
#247072=CARTESIAN_POINT('Ctrl Pts',(-56.4187877641046,-26.0735858933992,
-37.9907856426935));
#247073=CARTESIAN_POINT('Ctrl Pts',(-56.412400971856,-26.0448843120847,
-37.9786921602017));
#247074=CARTESIAN_POINT('Ctrl Pts',(-56.405165059693,-26.0160109209669,
-37.9662294042276));
#247075=CARTESIAN_POINT('Ctrl Pts',(-56.3970073796387,-25.9870111882494,
-37.9534493683309));
#247076=CARTESIAN_POINT('Ctrl Pts',(-56.3921075449972,-25.9695927685497,
-37.9457731586502));
#247077=CARTESIAN_POINT('Ctrl Pts',(-56.3868771908374,-25.9521216702897,
-37.9379863926414));
#247078=CARTESIAN_POINT('Ctrl Pts',(-56.3813044015347,-25.9345959421817,
-37.9301082422528));
#247079=CARTESIAN_POINT('Ctrl Pts',(-56.3785180068833,-25.9258330781278,
-37.9261691670585));
#247080=CARTESIAN_POINT('Ctrl Pts',(-56.3756459973473,-25.9170565567473,
-37.9222072490867));
#247081=CARTESIAN_POINT('Ctrl Pts',(-56.3726869268393,-25.9082661430612,
-37.9182250284407));
#247082=CARTESIAN_POINT('Ctrl Pts',(-56.3712073915853,-25.9038709362181,
-37.9162339181176));
#247083=CARTESIAN_POINT('Ctrl Pts',(-56.3697060905476,-25.8994722563214,
-37.9142377323202));
#247084=CARTESIAN_POINT('Ctrl Pts',(-56.3681828424972,-25.8950700745533,
-37.9122367943842));
#247085=CARTESIAN_POINT('Ctrl Pts',(-56.3669710243399,-25.8915679241342,
-37.9106449506121));
#247086=CARTESIAN_POINT('Ctrl Pts',(-56.3654774223584,-25.8873033214185,
-37.9087037044428));
#247087=CARTESIAN_POINT('Ctrl Pts',(-56.3643408295022,-25.8840911501479,
-37.9072401091671));
#247088=CARTESIAN_POINT('Ctrl Pts',(-56.3640487320537,-25.8832656416757,
-37.9068639740865));
#247089=CARTESIAN_POINT('Ctrl Pts',(-56.3637804176812,-25.8825094376191,
-37.9065193163851));
#247090=CARTESIAN_POINT('Ctrl Pts',(-56.3635470749447,-25.8818529950945,
-37.9062200511035));
#247091=CARTESIAN_POINT('Ctrl Pts',(-56.3559220562341,-25.8604022029829,
-37.8964408593217));
#247092=CARTESIAN_POINT('Ctrl Pts',(-56.3474085676981,-25.8377868512682,
-37.8860858805099));
#247093=CARTESIAN_POINT('Ctrl Pts',(-56.3378749583545,-25.8140733963192,
-37.8752267949122));
#247094=CARTESIAN_POINT('Ctrl Pts',(-56.328842437291,-25.7916063249726,
-37.8649384648732));
#247095=CARTESIAN_POINT('Ctrl Pts',(-56.3188936191063,-25.7681544980646,
-37.8541980336547));
#247096=CARTESIAN_POINT('Ctrl Pts',(-56.3079341570525,-25.7437537778324,
-37.8431049637893));
#247097=CARTESIAN_POINT('Ctrl Pts',(-56.2975795165837,-25.7206996640498,
-37.8326240889445));
#247098=CARTESIAN_POINT('Ctrl Pts',(-56.2863224087543,-25.6967991089898,
-37.8218290008965));
#247099=CARTESIAN_POINT('Ctrl Pts',(-56.274105561681,-25.6720524972858,
-37.8108317796241));
#247100=CARTESIAN_POINT('Ctrl Pts',(-56.2621445138239,-25.6478240359556,
-37.8000648207562));
#247101=CARTESIAN_POINT('Ctrl Pts',(-56.2492633010286,-25.622785034932,
-37.7891046168325));
#247102=CARTESIAN_POINT('Ctrl Pts',(-56.2354338835942,-25.5968983561643,
-37.7780764398159));
#247103=CARTESIAN_POINT('Ctrl Pts',(-56.2215469023249,-25.5709039261838,
-37.7670023589017));
#247104=CARTESIAN_POINT('Ctrl Pts',(-56.2067037293098,-25.544054901184,
-37.7558602365061));
#247105=CARTESIAN_POINT('Ctrl Pts',(-56.1909044158831,-25.5162703670661,
-37.7447898421755));
#247106=CARTESIAN_POINT('Ctrl Pts',(-56.1874809063733,-25.5102498132477,
-37.7423910290597));
#247107=CARTESIAN_POINT('Ctrl Pts',(-56.1840126093571,-25.5041851725429,
-37.7399956157948));
#247108=CARTESIAN_POINT('Ctrl Pts',(-56.1804996997125,-25.498075361193,
-37.7376050692572));
#247109=CARTESIAN_POINT('Origin',(-57.2992117475353,-25.881758760926,-37.0968023399421));
#247110=CARTESIAN_POINT('Origin',(-59.8906867066747,-29.1158971114318,-24.194539546945));
#247111=CARTESIAN_POINT('',(-59.5084684665646,-28.5649662692455,-28.4686772617213));
#247112=CARTESIAN_POINT('',(-58.9433054279041,-27.6410867367342,-28.14995));
#247113=CARTESIAN_POINT('Origin',(-58.560621995539,-28.5649662692455,-28.14995));
#247114=CARTESIAN_POINT('',(-59.0583147116521,-27.6887251418614,-27.8079298566744));
#247115=CARTESIAN_POINT('',(-59.428784774735,-28.924571066736,-28.4919701433257));
#247116=CARTESIAN_POINT('',(-56.4622101753633,-27.6957756338847,-37.3141124660878));
#247117=CARTESIAN_POINT('Origin',(-58.560621995539,-28.5649662692455,-28.14995));
#247118=CARTESIAN_POINT('Ctrl Pts',(-59.998518160033,-26.9957779612784,
-27.14995));
#247119=CARTESIAN_POINT('Ctrl Pts',(-60.6454255730951,-27.2637357853683,
-27.14995));
#247120=CARTESIAN_POINT('Ctrl Pts',(-60.8666809392289,-27.3553827587689,
-26.4919701433257));
#247121=CARTESIAN_POINT('Ctrl Pts',(-59.9484159856373,-27.1167353102034,
-27.14995));
#247122=CARTESIAN_POINT('Ctrl Pts',(-60.5825424694076,-27.4155490271209,
-27.1499500000068));
#247123=CARTESIAN_POINT('Ctrl Pts',(-60.7664765904384,-27.5972974566192,
-26.4919701433347));
#247124=CARTESIAN_POINT('Ctrl Pts',(-59.8808474404287,-27.230351027148,
-27.1759773253793));
#247125=CARTESIAN_POINT('Ctrl Pts',(-60.5059399274626,-27.5624213738311,
-27.189969500269));
#247126=CARTESIAN_POINT('Ctrl Pts',(-60.6488436389318,-27.8317793422431,
-26.5440247940841));
#247127=CARTESIAN_POINT('Ctrl Pts',(-59.720909171428,-27.4259018040837,
-27.2761636095982));
#247128=CARTESIAN_POINT('Ctrl Pts',(-60.3438449576235,-27.8117580695072,
-27.3392652319674));
#247129=CARTESIAN_POINT('Ctrl Pts',(-60.3963453125034,-28.2507898651562,
-26.7443973625222));
#247130=CARTESIAN_POINT('Ctrl Pts',(-59.6286113898652,-27.5077381405927,
-27.3502831612192));
#247131=CARTESIAN_POINT('Ctrl Pts',(-60.25750475067,-27.9147957782208,-27.4500905748289));
#247132=CARTESIAN_POINT('Ctrl Pts',(-60.2615973195289,-28.4351100777821,
-26.8926364657637));
#247133=CARTESIAN_POINT('Ctrl Pts',(-59.4332702873462,-27.6271977754378,
-27.5354032764078));
#247134=CARTESIAN_POINT('Ctrl Pts',(-60.0950932878165,-28.0555284666377,
-27.714377456199));
#247135=CARTESIAN_POINT('Ctrl Pts',(-59.9954138159282,-28.7255983981058,
-27.2628766961414));
#247136=CARTESIAN_POINT('Ctrl Pts',(-59.3303038024737,-27.6647740853107,
-27.6463310241559));
#247137=CARTESIAN_POINT('Ctrl Pts',(-60.018639255483,-28.0922015151602,
-27.8698850835747));
#247138=CARTESIAN_POINT('Ctrl Pts',(-59.8640830067033,-28.8316522445216,
-27.4847321916381));
#247139=CARTESIAN_POINT('Ctrl Pts',(-59.1292987784775,-27.6899559312547,
-27.888202111114));
#247140=CARTESIAN_POINT('Ctrl Pts',(-59.8921803917124,-28.0961466343177,
-28.1867324885194));
#247141=CARTESIAN_POINT('Ctrl Pts',(-59.6247383514533,-28.9493941482113,
-27.968474365553));
#247142=CARTESIAN_POINT('Ctrl Pts',(-59.0313551773641,-27.6775581371241,
-28.0190267086425));
#247143=CARTESIAN_POINT('Ctrl Pts',(-59.8428062390324,-28.0610797847622,
-28.3489305637492));
#247144=CARTESIAN_POINT('Ctrl Pts',(-59.5168345241973,-28.9610424671195,
-28.23012356061));
#247145=CARTESIAN_POINT('Ctrl Pts',(-58.9433054279041,-27.6410867367342,
-28.14995));
#247146=CARTESIAN_POINT('Ctrl Pts',(-59.8114682071001,-28.0006915342247,
-28.4919701433256));
#247147=CARTESIAN_POINT('Ctrl Pts',(-59.428784774735,-28.924571066736,-28.4919701433257));
#247148=CARTESIAN_POINT('Ctrl Pts',(-60.0746608288527,-28.637079928768,
-27.1547905454732));
#247149=CARTESIAN_POINT('Ctrl Pts',(-60.0444600479327,-28.667752613367,
-27.1992006472175));
#247150=CARTESIAN_POINT('Ctrl Pts',(-60.0141620017611,-28.6965907066387,
-27.2457865562304));
#247151=CARTESIAN_POINT('Ctrl Pts',(-59.9839608794947,-28.7233395120922,
-27.2943231462453));
#247152=CARTESIAN_POINT('Ctrl Pts',(-59.9534054378562,-28.750402134359,
-27.3434291672218));
#247153=CARTESIAN_POINT('Ctrl Pts',(-59.9229495475082,-28.7753257426137,
-27.3945314828291));
#247154=CARTESIAN_POINT('Ctrl Pts',(-59.8927990300297,-28.7978772501937,
-27.4473527189011));
#247155=CARTESIAN_POINT('Ctrl Pts',(-59.8623328067314,-28.8206648944234,
-27.5007270457002));
#247156=CARTESIAN_POINT('Ctrl Pts',(-59.832178773856,-28.8410300714376,
-27.5558559437987));
#247157=CARTESIAN_POINT('Ctrl Pts',(-59.8025485290152,-28.8587698654644,
-27.6124156554068));
#247158=CARTESIAN_POINT('Ctrl Pts',(-59.7829193828322,-28.8705219455461,
-27.6498847635154));
#247159=CARTESIAN_POINT('Ctrl Pts',(-59.7635200854943,-28.881122619247,
-27.6879810424222));
#247160=CARTESIAN_POINT('Ctrl Pts',(-59.7444106790783,-28.8905231963665,
-27.7266032785955));
#247161=CARTESIAN_POINT('Ctrl Pts',(-59.7141853858534,-28.9053920621874,
-27.7876919585852));
#247162=CARTESIAN_POINT('Ctrl Pts',(-59.6846932959222,-28.917253071195,
-27.8500820237121));
#247163=CARTESIAN_POINT('Ctrl Pts',(-59.6561316380727,-28.9260738700217,
-27.9133068574047));
#247164=CARTESIAN_POINT('Ctrl Pts',(-59.628803824998,-28.9345136161588,
-27.9738004199962));
#247165=CARTESIAN_POINT('Ctrl Pts',(-59.6023280103622,-28.9401705089795,
-28.035057253628));
#247166=CARTESIAN_POINT('Ctrl Pts',(-59.5768604082263,-28.9430655183748,
-28.0966587861506));
#247167=CARTESIAN_POINT('Ctrl Pts',(-59.551602297407,-28.9459367140114,
-28.1577535969929));
#247168=CARTESIAN_POINT('Ctrl Pts',(-59.5273361425688,-28.9460913671025,
-28.2191866992274));
#247169=CARTESIAN_POINT('Ctrl Pts',(-59.5041940479805,-28.9435966619134,
-28.2805521290657));
#247170=CARTESIAN_POINT('Ctrl Pts',(-59.4814573360743,-28.9411456567565,
-28.3408426137454));
#247171=CARTESIAN_POINT('Ctrl Pts',(-59.4598058222201,-28.9361374839187,
-28.4010671409335));
#247172=CARTESIAN_POINT('Ctrl Pts',(-59.439341970719,-28.9286789989135,
-28.4608532721926));
#247173=CARTESIAN_POINT('Ctrl Pts',(-59.4357869697836,-28.9273833033711,
-28.4712393792527));
#247174=CARTESIAN_POINT('Ctrl Pts',(-59.4322677512012,-28.9260137628254,
-28.4816123002776));
#247175=CARTESIAN_POINT('Ctrl Pts',(-59.428784774735,-28.924571066736,-28.4919701433257));
#247176=CARTESIAN_POINT('Ctrl Pts',(-58.9433054279041,-27.6410867367342,
-28.14995));
#247177=CARTESIAN_POINT('Ctrl Pts',(-58.9613748712486,-27.648571345232,
-28.1230821098565));
#247178=CARTESIAN_POINT('Ctrl Pts',(-58.9791315286144,-27.6547427046832,
-28.0973015822799));
#247179=CARTESIAN_POINT('Ctrl Pts',(-58.9964342459705,-27.6598302215434,
-28.0726669650116));
#247180=CARTESIAN_POINT('Ctrl Pts',(-59.0144311387734,-27.6651218467652,
-28.0470440205289));
#247181=CARTESIAN_POINT('Ctrl Pts',(-59.0319371483571,-27.6692410795885,
-28.0226604247913));
#247182=CARTESIAN_POINT('Ctrl Pts',(-59.0488314419348,-27.6724253459282,
-27.9995447185591));
#247183=CARTESIAN_POINT('Ctrl Pts',(-59.068041016188,-27.6760460004654,
-27.9732611173396));
#247184=CARTESIAN_POINT('Ctrl Pts',(-59.086460041634,-27.6784586319551,
-27.9486159224461));
#247185=CARTESIAN_POINT('Ctrl Pts',(-59.1039586602071,-27.6799782867226,
-27.9256083236474));
#247186=CARTESIAN_POINT('Ctrl Pts',(-59.1211642581416,-27.6814724943265,
-27.9029859953353));
#247187=CARTESIAN_POINT('Ctrl Pts',(-59.1374778388352,-27.6821028285425,
-27.881949932047));
#247188=CARTESIAN_POINT('Ctrl Pts',(-59.1528052574349,-27.6821364137596,
-27.8624791903457));
#247189=CARTESIAN_POINT('Ctrl Pts',(-59.1690851883618,-27.6821720861078,
-27.8417984522337));
#247190=CARTESIAN_POINT('Ctrl Pts',(-59.1842533698988,-27.6815349481643,
-27.8228824131788));
#247191=CARTESIAN_POINT('Ctrl Pts',(-59.1982293897907,-27.6805062024526,
-27.8056852997811));
#247192=CARTESIAN_POINT('Ctrl Pts',(-59.2028122682947,-27.6801688663122,
-27.8000461920859));
#247193=CARTESIAN_POINT('Ctrl Pts',(-59.2072672152542,-27.6797890985914,
-27.7945917577315));
#247194=CARTESIAN_POINT('Ctrl Pts',(-59.2115920807886,-27.679375851391,
-27.7893200190977));
#247195=CARTESIAN_POINT('Ctrl Pts',(-59.2126299161687,-27.6792766847089,
-27.7880549631497));
#247196=CARTESIAN_POINT('Ctrl Pts',(-59.2136602613722,-27.6791755879617,
-27.786800428185));
#247197=CARTESIAN_POINT('Ctrl Pts',(-59.2146831346899,-27.679072706751,
-27.7855564027394));
#247198=CARTESIAN_POINT('Ctrl Pts',(-59.2157060080076,-27.6789698255402,
-27.7843123772939));
#247199=CARTESIAN_POINT('Ctrl Pts',(-59.2159304130621,-27.6789487784925,
-27.7840390885988));
#247200=CARTESIAN_POINT('Ctrl Pts',(-59.217729308674,-27.6787588260363,
-27.7818558257232));
#247201=CARTESIAN_POINT('Ctrl Pts',(-59.2217623561684,-27.6783329607041,
-27.7769610431625));
#247202=CARTESIAN_POINT('Ctrl Pts',(-59.2257866159072,-27.6778681563496,
-27.7720978874654));
#247203=CARTESIAN_POINT('Ctrl Pts',(-59.2298015448288,-27.677365154145,
-27.7672666579805));
#247204=CARTESIAN_POINT('Ctrl Pts',(-59.2564471047789,-27.6740269193568,
-27.7352036209043));
#247205=CARTESIAN_POINT('Ctrl Pts',(-59.2826719347528,-27.6690086662134,
-27.7045578880862));
#247206=CARTESIAN_POINT('Ctrl Pts',(-59.3083322835412,-27.6625830507753,
-27.6753684982175));
#247207=CARTESIAN_POINT('Ctrl Pts',(-59.3339926323296,-27.6561574353372,
-27.6461791083489));
#247208=CARTESIAN_POINT('Ctrl Pts',(-59.3590887994654,-27.6483243303831,
-27.6184457481429));
#247209=CARTESIAN_POINT('Ctrl Pts',(-59.3835121576981,-27.6393314235105,
-27.5921760116137));
#247210=CARTESIAN_POINT('Ctrl Pts',(-59.4102021141836,-27.6295039341529,
-27.5634683245637));
#247211=CARTESIAN_POINT('Ctrl Pts',(-59.4360869695798,-27.6182918335755,
-27.5365103467925));
#247212=CARTESIAN_POINT('Ctrl Pts',(-59.461058297068,-27.6059926956016,
-27.51128325361));
#247213=CARTESIAN_POINT('Ctrl Pts',(-59.4790883909822,-27.5971123261924,
-27.4930684887171));
#247214=CARTESIAN_POINT('Ctrl Pts',(-59.4966429912841,-27.5876646717946,
-27.4757554313279));
#247215=CARTESIAN_POINT('Ctrl Pts',(-59.5136917085776,-27.5777545780401,
-27.459327532637));
#247216=CARTESIAN_POINT('Ctrl Pts',(-59.5171569791665,-27.5757402824289,
-27.455988447755));
#247217=CARTESIAN_POINT('Ctrl Pts',(-59.5202646758599,-27.5739061150911,
-27.4530084899692));
#247218=CARTESIAN_POINT('Ctrl Pts',(-59.523617795358,-27.5718989259609,
-27.4498080531444));
#247219=CARTESIAN_POINT('Ctrl Pts',(-59.5258853753984,-27.5705415445697,
-27.4476437262635));
#247220=CARTESIAN_POINT('Ctrl Pts',(-59.5282650669352,-27.5691043972,-27.4453790651482));
#247221=CARTESIAN_POINT('Ctrl Pts',(-59.5309409555251,-27.5674680334054,
-27.4428432437218));
#247222=CARTESIAN_POINT('Ctrl Pts',(-59.5623318535266,-27.5482718197956,
-27.4130954761778));
#247223=CARTESIAN_POINT('Ctrl Pts',(-59.5927659836345,-27.5270383018031,
-27.3856317423159));
#247224=CARTESIAN_POINT('Ctrl Pts',(-59.6220731179921,-27.5041279599908,
-27.3604797898221));
#247225=CARTESIAN_POINT('Ctrl Pts',(-59.6423059120638,-27.4883113256403,
-27.3431156125847));
#247226=CARTESIAN_POINT('Ctrl Pts',(-59.6620022705099,-27.4716947429332,
-27.3268527561149));
#247227=CARTESIAN_POINT('Ctrl Pts',(-59.6811150169812,-27.4543872636165,
-27.3116941131195));
#247228=CARTESIAN_POINT('Ctrl Pts',(-59.6966942407607,-27.4402795531553,
-27.2993379668287));
#247229=CARTESIAN_POINT('Ctrl Pts',(-59.7119961768362,-27.4256086581483,
-27.2876298176573));
#247230=CARTESIAN_POINT('Ctrl Pts',(-59.7268826337955,-27.4105236752065,
-27.2766669971972));
#247231=CARTESIAN_POINT('Ctrl Pts',(-59.74173904001,-27.3954691437667,-27.2657263069808));
#247232=CARTESIAN_POINT('Ctrl Pts',(-59.7561813657372,-27.3800025679289,
-27.2555280942016));
#247233=CARTESIAN_POINT('Ctrl Pts',(-59.7700924498725,-27.364298936964,
-27.2461293656728));
#247234=CARTESIAN_POINT('Ctrl Pts',(-59.7806770832468,-27.352350394723,
-27.2389780829479));
#247235=CARTESIAN_POINT('Ctrl Pts',(-59.7909545612152,-27.3402652046939,
-27.2322888317529));
#247236=CARTESIAN_POINT('Ctrl Pts',(-59.8008824303336,-27.328128780816,
-27.2260707188289));
#247237=CARTESIAN_POINT('Ctrl Pts',(-59.8041054693502,-27.3241887442165,
-27.2240520358341));
#247238=CARTESIAN_POINT('Ctrl Pts',(-59.8072916110025,-27.3202435181017,
-27.2220829617867));
#247239=CARTESIAN_POINT('Ctrl Pts',(-59.8104397189014,-27.3162962998181,
-27.2201632624574));
#247240=CARTESIAN_POINT('Ctrl Pts',(-59.8437952720307,-27.2744738294958,
-27.1998232248763));
#247241=CARTESIAN_POINT('Ctrl Pts',(-59.874727000118,-27.230098430282,-27.1838933969132));
#247242=CARTESIAN_POINT('Ctrl Pts',(-59.902952727294,-27.1838915675732,
-27.1723878666496));
#247243=CARTESIAN_POINT('Ctrl Pts',(-59.9311901022577,-27.1376656368799,
-27.160877588449));
#247244=CARTESIAN_POINT('Ctrl Pts',(-59.9567191564442,-27.0896067866201,
-27.1537949386769));
#247245=CARTESIAN_POINT('Ctrl Pts',(-59.9792844971738,-27.0403941998065,
-27.1511419396506));
#247246=CARTESIAN_POINT('Ctrl Pts',(-59.9860436278898,-27.0256532609866,
-27.1503472710736));
#247247=CARTESIAN_POINT('Ctrl Pts',(-59.9925370376024,-27.0108085114896,
-27.1499499750118));
#247248=CARTESIAN_POINT('Ctrl Pts',(-59.9987583477721,-26.9958774502974,
-27.1499499662059));
#247249=CARTESIAN_POINT('Ctrl Pts',(-50.4237575282656,-42.512871148214,
-37.0628442249021));
#247250=CARTESIAN_POINT('Ctrl Pts',(-50.0392469284306,-43.4351970348678,
-37.0691716931121));
#247251=CARTESIAN_POINT('Ctrl Pts',(-49.1714197666586,-43.0765237853397,
-36.7274049322981));
#247252=CARTESIAN_POINT('Ctrl Pts',(-50.3416577002277,-42.4769411182047,
-37.3090186906075));
#247253=CARTESIAN_POINT('Ctrl Pts',(-49.9919063191206,-43.4299470769918,
-37.1948592375177));
#247254=CARTESIAN_POINT('Ctrl Pts',(-49.1176720095218,-43.0532992273906,
-36.8471157789082));
#247255=CARTESIAN_POINT('Ctrl Pts',(-50.2401291906866,-42.4884206957375,
-37.5546625905171));
#247256=CARTESIAN_POINT('Ctrl Pts',(-49.936763884108,-43.4500767701373,
-37.3136659503387));
#247257=CARTESIAN_POINT('Ctrl Pts',(-49.0542361384641,-43.0537900902966,
-36.9665683337155));
#247258=CARTESIAN_POINT('Ctrl Pts',(-50.0695743278833,-42.5755840840409,
-37.8959436915621));
#247259=CARTESIAN_POINT('Ctrl Pts',(-49.8496587474524,-43.5105080802159,
-37.4712316264487));
#247260=CARTESIAN_POINT('Ctrl Pts',(-48.9513522923176,-43.0900782943884,
-37.1325273165808));
#247261=CARTESIAN_POINT('Ctrl Pts',(-50.0111449417175,-42.6150505005841,
-38.0027616853659));
#247262=CARTESIAN_POINT('Ctrl Pts',(-49.8204425668583,-43.5351648198003,
-37.5194682740609));
#247263=CARTESIAN_POINT('Ctrl Pts',(-48.9166267233427,-43.1075285409369,
-37.1844709706788));
#247264=CARTESIAN_POINT('Ctrl Pts',(-49.8898699570401,-42.7151860559833,
-38.2053146722979));
#247265=CARTESIAN_POINT('Ctrl Pts',(-49.7612063443368,-43.5929894582252,
-37.6090332432771));
#247266=CARTESIAN_POINT('Ctrl Pts',(-48.8455389394235,-43.1532669776793,
-37.2829687310632));
#247267=CARTESIAN_POINT('Ctrl Pts',(-49.8264028016164,-42.7766563905902,
-38.3017849985497));
#247268=CARTESIAN_POINT('Ctrl Pts',(-49.7309236615698,-43.626585368299,
-37.6505782223522));
#247269=CARTESIAN_POINT('Ctrl Pts',(-48.8088280035253,-43.1819400457003,
-37.3298804131014));
#247270=CARTESIAN_POINT('Ctrl Pts',(-49.6998636398414,-42.9166438821161,
-38.4757993599315));
#247271=CARTESIAN_POINT('Ctrl Pts',(-49.6717558147567,-43.6995260307251,
-37.7240763018152));
#247272=CARTESIAN_POINT('Ctrl Pts',(-48.7365799885116,-43.2482138864143,
-37.4145002189235));
#247273=CARTESIAN_POINT('Ctrl Pts',(-49.636377638708,-42.9953419367724,
-38.5542040553824));
#247274=CARTESIAN_POINT('Ctrl Pts',(-49.6426863188407,-43.7390132802502,
-37.7563474788299));
#247275=CARTESIAN_POINT('Ctrl Pts',(-48.7007915109969,-43.2858867144277,
-37.4526268655564));
#247276=CARTESIAN_POINT('Ctrl Pts',(-49.5089673406965,-43.1703662790524,
-38.6935914165869));
#247277=CARTESIAN_POINT('Ctrl Pts',(-49.5852286190754,-43.8240110418488,
-37.8128274533556));
#247278=CARTESIAN_POINT('Ctrl Pts',(-48.6298942465199,-43.3704186966852,
-37.5204081363966));
#247279=CARTESIAN_POINT('Ctrl Pts',(-49.4452086173444,-43.2667004006212,
-38.7541455640211));
#247280=CARTESIAN_POINT('Ctrl Pts',(-49.5569626986225,-43.8694639105835,
-37.8367864581829));
#247281=CARTESIAN_POINT('Ctrl Pts',(-48.5948903577209,-43.4172909280656,
-37.5498543766621));
#247282=CARTESIAN_POINT('Ctrl Pts',(-49.2615126569161,-43.5701125808966,
-38.9014161879009));
#247283=CARTESIAN_POINT('Ctrl Pts',(-49.4760987284841,-44.0097527471331,
-37.8945457008393));
#247284=CARTESIAN_POINT('Ctrl Pts',(-48.4954434049397,-43.5658475318205,
-37.6214690391308));
#247285=CARTESIAN_POINT('Ctrl Pts',(-49.1445110616521,-43.7995630731719,
-38.957158320864));
#247286=CARTESIAN_POINT('Ctrl Pts',(-49.4258287509964,-44.1113431434592,
-37.9153346356675));
#247287=CARTESIAN_POINT('Ctrl Pts',(-48.4340663781108,-43.6793802666741,
-37.6485752564667));
#247288=CARTESIAN_POINT('Ctrl Pts',(-49.0438717682238,-44.0349657503363,
-38.9651091877403));
#247289=CARTESIAN_POINT('Ctrl Pts',(-49.3817941333223,-44.2147893101095,
-37.9183446714817));
#247290=CARTESIAN_POINT('Ctrl Pts',(-48.3833370225155,-43.7969102160512,
-37.6524415864869));
#247291=CARTESIAN_POINT('',(-48.3869818477026,-43.7885141789011,-37.6521262739199));
#247292=CARTESIAN_POINT('Ctrl Pts',(-48.3869820185779,-43.7885142818768,
-37.6521255977635));
#247293=CARTESIAN_POINT('Ctrl Pts',(-48.3941923230744,-43.7855029913321,
-37.6532372055275));
#247294=CARTESIAN_POINT('Ctrl Pts',(-48.40472479657,-43.7811582841343,-37.6548675123769));
#247295=CARTESIAN_POINT('Ctrl Pts',(-48.4185542648403,-43.7754695476231,
-37.6570112368262));
#247296=CARTESIAN_POINT('Ctrl Pts',(-48.4332645964769,-43.7694184689384,
-37.6592915050889));
#247297=CARTESIAN_POINT('Ctrl Pts',(-48.4517063655238,-43.7618503879438,
-37.662153381686));
#247298=CARTESIAN_POINT('Ctrl Pts',(-48.4738977492675,-43.7527517588849,
-37.6656002137221));
#247299=CARTESIAN_POINT('Ctrl Pts',(-48.4777287835395,-43.7511810069139,
-37.6661952614132));
#247300=CARTESIAN_POINT('Ctrl Pts',(-48.4816716525774,-43.7495645474523,
-37.6668077446633));
#247301=CARTESIAN_POINT('Ctrl Pts',(-48.4857265410659,-43.7479021557398,
-37.6674376688176));
#247302=CARTESIAN_POINT('Ctrl Pts',(-48.5038894581431,-43.740455863959,
-37.6702592655672));
#247303=CARTESIAN_POINT('Ctrl Pts',(-48.5242907044421,-43.7320882445654,
-37.6734280242068));
#247304=CARTESIAN_POINT('Ctrl Pts',(-48.5469302210382,-43.7227990263846,
-37.6769467634094));
#247305=CARTESIAN_POINT('Ctrl Pts',(-48.5552184355614,-43.7193982897696,
-37.6782349563457));
#247306=CARTESIAN_POINT('Ctrl Pts',(-48.5638066266517,-43.7158735854635,
-37.6795699967092));
#247307=CARTESIAN_POINT('Ctrl Pts',(-48.5726946772116,-43.7122230706351,
-37.6809516127904));
#247308=CARTESIAN_POINT('Ctrl Pts',(-48.5892776962156,-43.7054120656387,
-37.68352938455));
#247309=CARTESIAN_POINT('Ctrl Pts',(-48.6069047406048,-43.6981667414177,
-37.6862702702229));
#247310=CARTESIAN_POINT('Ctrl Pts',(-48.6255745808139,-43.690481744612,
-37.6891773653139));
#247311=CARTESIAN_POINT('Ctrl Pts',(-48.6349095009184,-43.6866392462091,
-37.6906309128593));
#247312=CARTESIAN_POINT('Ctrl Pts',(-48.6445051011876,-43.6826868018733,
-37.6921260606455));
#247313=CARTESIAN_POINT('Ctrl Pts',(-48.6543610548145,-43.6786234447101,
-37.6936635574224));
#247314=CARTESIAN_POINT('Ctrl Pts',(-48.6592890316279,-43.6765917661285,
-37.6944323058108));
#247315=CARTESIAN_POINT('Ctrl Pts',(-48.6642820944631,-43.6745323555192,
-37.6952116459788));
#247316=CARTESIAN_POINT('Ctrl Pts',(-48.6693401861212,-43.6724450617448,
-37.6960017001812));
#247317=CARTESIAN_POINT('Ctrl Pts',(-48.6743982777794,-43.6703577679704,
-37.6967917543835));
#247318=CARTESIAN_POINT('Ctrl Pts',(-48.6809273732975,-43.6676617725024,
-37.6978124741394));
#247319=CARTESIAN_POINT('Ctrl Pts',(-48.6847094771468,-43.6660993562588,
-37.698404148648));
#247320=CARTESIAN_POINT('Ctrl Pts',(-48.7123065729498,-43.6546987833301,
-37.7027214542398));
#247321=CARTESIAN_POINT('Ctrl Pts',(-48.7387413992479,-43.6436924952179,
-37.7068525271263));
#247322=CARTESIAN_POINT('Ctrl Pts',(-48.7640030878273,-43.6330656769537,
-37.7107829608343));
#247323=CARTESIAN_POINT('Ctrl Pts',(-48.7909189728857,-43.6217429889221,
-37.7149707688498));
#247324=CARTESIAN_POINT('Ctrl Pts',(-48.8165033200792,-43.6108520387734,
-37.7189299873399));
#247325=CARTESIAN_POINT('Ctrl Pts',(-48.8407654011673,-43.6004175398603,
-37.7226755849429));
#247326=CARTESIAN_POINT('Ctrl Pts',(-48.8436635160472,-43.599171134968,
-37.7231229980113));
#247327=CARTESIAN_POINT('Ctrl Pts',(-48.8465427863071,-43.5979312796092,
-37.7235674059532));
#247328=CARTESIAN_POINT('Ctrl Pts',(-48.8494032448022,-43.5966980430636,
-37.7240088692827));
#247329=CARTESIAN_POINT('Ctrl Pts',(-48.8595586364947,-43.5923197239264,
-37.7255761820184));
#247330=CARTESIAN_POINT('Ctrl Pts',(-48.8694763091597,-43.5880221626812,
-37.727104110795));
#247331=CARTESIAN_POINT('Ctrl Pts',(-48.8791523850949,-43.583810866203,
-37.7285943817753));
#247332=CARTESIAN_POINT('Ctrl Pts',(-48.892954490905,-43.5778038071453,
-37.7307201275729));
#247333=CARTESIAN_POINT('Ctrl Pts',(-48.9062809742503,-43.571946621652,
-37.7327581161945));
#247334=CARTESIAN_POINT('Ctrl Pts',(-48.9191161911195,-43.5662657232329,
-37.7347219845827));
#247335=CARTESIAN_POINT('Ctrl Pts',(-48.9300329149347,-43.5614339545377,
-37.736392311545));
#247336=CARTESIAN_POINT('Ctrl Pts',(-48.9405984373613,-43.5567226003328,
-37.7380053451827));
#247337=CARTESIAN_POINT('Ctrl Pts',(-48.9508131358863,-43.552133008746,
-37.7395604493697));
#247338=CARTESIAN_POINT('Ctrl Pts',(-48.9559204851488,-43.5498382129526,
-37.7403380014632));
#247339=CARTESIAN_POINT('Ctrl Pts',(-48.9609401364647,-43.547573871151,
-37.7411010587111));
#247340=CARTESIAN_POINT('Ctrl Pts',(-48.9658721830952,-43.5453402239186,
-37.7418494793756));
#247341=CARTESIAN_POINT('Ctrl Pts',(-48.9683382064105,-43.5442234003024,
-37.7422236897079));
#247342=CARTESIAN_POINT('Ctrl Pts',(-48.9707823289942,-43.5431142510686,
-37.7425942403847));
#247343=CARTESIAN_POINT('Ctrl Pts',(-48.9732045651145,-43.5420128103547,
-37.742961110882));
#247344=CARTESIAN_POINT('Ctrl Pts',(-48.9756268012349,-43.5409113696408,
-37.7433279813792));
#247345=CARTESIAN_POINT('Ctrl Pts',(-48.9768890918041,-43.5403372625218,
-37.7435191631628));
#247346=CARTESIAN_POINT('Ctrl Pts',(-48.980405629973,-43.5387316505353,
-37.7440506597886));
#247347=CARTESIAN_POINT('Ctrl Pts',(-49.0162112906282,-43.5223831864575,
-37.749462399093));
#247348=CARTESIAN_POINT('Ctrl Pts',(-49.0511276808107,-43.5059828258899,
-37.7547048280429));
#247349=CARTESIAN_POINT('Ctrl Pts',(-49.0850703209528,-43.4895147250152,
-37.7597506223924));
#247350=CARTESIAN_POINT('Ctrl Pts',(-49.1076241559372,-43.4785721811212,
-37.763103396739));
#247351=CARTESIAN_POINT('Ctrl Pts',(-49.1297489180256,-43.4676007829305,
-37.766369148453));
#247352=CARTESIAN_POINT('Ctrl Pts',(-49.1514279942163,-43.4566051623532,
-37.7695413736243));
#247353=CARTESIAN_POINT('Ctrl Pts',(-49.1832043343191,-43.440488212718,
-37.7741910969354));
#247354=CARTESIAN_POINT('Ctrl Pts',(-49.2140118419065,-43.4243167890084,
-37.7786635108871));
#247355=CARTESIAN_POINT('Ctrl Pts',(-49.2438645278442,-43.4080568268287,
-37.7829115278891));
#247356=CARTESIAN_POINT('Ctrl Pts',(-49.275440482448,-43.3908582461476,
-37.7874047648558));
#247357=CARTESIAN_POINT('Ctrl Pts',(-49.3059481203,-43.3735617149496,-37.7916467356859));
#247358=CARTESIAN_POINT('Ctrl Pts',(-49.3354042005926,-43.3561704676905,
-37.7956243930565));
#247359=CARTESIAN_POINT('Ctrl Pts',(-49.3678131316066,-43.3370358195272,
-37.8000007941949));
#247360=CARTESIAN_POINT('Ctrl Pts',(-49.3989490230391,-43.3177876585055,
-37.8040571104969));
#247361=CARTESIAN_POINT('Ctrl Pts',(-49.4288357902375,-43.2984632285755,
-37.8078297319575));
#247362=CARTESIAN_POINT('Ctrl Pts',(-49.4364798994516,-43.2935206380335,
-37.8087946516584));
#247363=CARTESIAN_POINT('Ctrl Pts',(-49.4440423047,-43.2885731615757,-37.8097412644242));
#247364=CARTESIAN_POINT('Ctrl Pts',(-49.4515234297442,-43.2836215894803,
-37.810670665132));
#247365=CARTESIAN_POINT('Ctrl Pts',(-49.4823256120956,-43.2632343849215,
-37.8144973048295));
#247366=CARTESIAN_POINT('Ctrl Pts',(-49.5117715503363,-43.2427689466307,
-37.8179862888973));
#247367=CARTESIAN_POINT('Ctrl Pts',(-49.539850477956,-43.2223212301653,
-37.8213021121719));
#247368=CARTESIAN_POINT('',(-49.1686140212331,-43.0753365939135,-36.7336343834465));
#247369=CARTESIAN_POINT('Ctrl Pts',(-49.1686140214361,-43.0753365934265,
-36.7336343834471));
#247370=CARTESIAN_POINT('Ctrl Pts',(-49.1683337750584,-43.075220511576,
-36.7342546446349));
#247371=CARTESIAN_POINT('Ctrl Pts',(-49.1673315732913,-43.0748009644702,
-36.7364762491404));
#247372=CARTESIAN_POINT('Ctrl Pts',(-49.1655731415317,-43.0741060083359,
-36.7403419878483));
#247373=CARTESIAN_POINT('Ctrl Pts',(-49.1639046758595,-43.0734466080223,
-36.7440099449906));
#247374=CARTESIAN_POINT('Ctrl Pts',(-49.1615552406925,-43.0725394115718,
-36.749158251366));
#247375=CARTESIAN_POINT('Ctrl Pts',(-49.1584774905419,-43.0714549440963,
-36.7558211532992));
#247376=CARTESIAN_POINT('Ctrl Pts',(-49.1554493667226,-43.0703879628168,
-36.7623766211126));
#247377=CARTESIAN_POINT('Ctrl Pts',(-49.151716128663,-43.069149267846,-36.7703985066625));
#247378=CARTESIAN_POINT('Ctrl Pts',(-49.1472163071513,-43.0678524373069,
-36.7799140437103));
#247379=CARTESIAN_POINT('Ctrl Pts',(-49.1431401300286,-43.0666776993841,
-36.7885337221405));
#247380=CARTESIAN_POINT('Ctrl Pts',(-49.1384346443936,-43.0654556929127,
-36.7983792211052));
#247381=CARTESIAN_POINT('Ctrl Pts',(-49.1330435616248,-43.0643059188313,
-36.8094633528079));
#247382=CARTESIAN_POINT('Ctrl Pts',(-49.128280821557,-43.0632901534794,
-36.8192556042798));
#247383=CARTESIAN_POINT('Ctrl Pts',(-49.1229843241211,-43.0623311285456,
-36.8300117719329));
#247384=CARTESIAN_POINT('Ctrl Pts',(-49.1170958753251,-43.0615332342699,
-36.8417600935923));
#247385=CARTESIAN_POINT('Ctrl Pts',(-49.1101501782072,-43.0605920811474,
-36.8556177811971));
#247386=CARTESIAN_POINT('Ctrl Pts',(-49.1023827525068,-43.059874088312,
-36.8708531503353));
#247387=CARTESIAN_POINT('Ctrl Pts',(-49.0936988710649,-43.0595999877853,
-36.8874724047507));
#247388=CARTESIAN_POINT('Ctrl Pts',(-49.0858463594793,-43.0593521288554,
-36.9025005795036));
#247389=CARTESIAN_POINT('Ctrl Pts',(-49.0772442151559,-43.0594676696369,
-36.9186604878903));
#247390=CARTESIAN_POINT('Ctrl Pts',(-49.0678179136489,-43.0601492850026,
-36.9359343013193));
#247391=CARTESIAN_POINT('Ctrl Pts',(-49.0586745427887,-43.0608104416682,
-36.9526896408587));
#247392=CARTESIAN_POINT('Ctrl Pts',(-49.0487557305991,-43.0620042891318,
-36.9704929824581));
#247393=CARTESIAN_POINT('Ctrl Pts',(-49.0379957893748,-43.0639516440868,
-36.9892956075429));
#247394=CARTESIAN_POINT('Ctrl Pts',(-49.0305212063224,-43.0653044085713,
-37.0023571828686));
#247395=CARTESIAN_POINT('Ctrl Pts',(-49.0226405847877,-43.0670215909623,
-37.0159006128308));
#247396=CARTESIAN_POINT('Ctrl Pts',(-49.0143347106628,-43.0691871639097,
-37.029896478983));
#247397=CARTESIAN_POINT('Ctrl Pts',(-49.0101817736003,-43.0702699503835,
-37.036894412059));
#247398=CARTESIAN_POINT('Ctrl Pts',(-49.0059224867822,-43.0714649806154,
-37.0440054089939));
#247399=CARTESIAN_POINT('Ctrl Pts',(-49.0015548172672,-43.0727834636932,
-37.051224538183));
#247400=CARTESIAN_POINT('Ctrl Pts',(-48.9993709825097,-43.073442705232,
-37.0548341027775));
#247401=CARTESIAN_POINT('Ctrl Pts',(-48.9971600554548,-43.0741328172138,
-37.0584706883975));
#247402=CARTESIAN_POINT('Ctrl Pts',(-48.9949218013837,-43.0748552442512,
-37.0621336079249));
#247403=CARTESIAN_POINT('Ctrl Pts',(-48.9947516515637,-43.074910162427,
-37.0624120593779));
#247404=CARTESIAN_POINT('Ctrl Pts',(-48.9945823225945,-43.0749649498015,
-37.0626890625254));
#247405=CARTESIAN_POINT('Ctrl Pts',(-48.9944107145094,-43.0750206127534,
-37.0629696859303));
#247406=CARTESIAN_POINT('Ctrl Pts',(-48.9929547407522,-43.0754928737024,
-37.0653505779076));
#247407=CARTESIAN_POINT('Ctrl Pts',(-48.9910589517925,-43.0761221560178,
-37.0684394409689));
#247408=CARTESIAN_POINT('Ctrl Pts',(-48.9896342939045,-43.0766054080036,
-37.0707525726143));
#247409=CARTESIAN_POINT('Ctrl Pts',(-48.9890179860343,-43.0768144631071,
-37.0717532347733));
#247410=CARTESIAN_POINT('Ctrl Pts',(-48.9884900444376,-43.0769953611969,
-37.072608999683));
#247411=CARTESIAN_POINT('Ctrl Pts',(-48.988124835575,-43.0771209443097,
-37.0732006352929));
#247412=CARTESIAN_POINT('Ctrl Pts',(-48.9871657946507,-43.0774507264069,
-37.0747542743754));
#247413=CARTESIAN_POINT('Ctrl Pts',(-48.9862068882847,-43.0777847567456,
-37.0763044684413));
#247414=CARTESIAN_POINT('Ctrl Pts',(-48.9852481546861,-43.0781229928334,
-37.0778511718949));
#247415=CARTESIAN_POINT('Ctrl Pts',(-48.96949840413,-43.0836794206261,-37.1032598919126));
#247416=CARTESIAN_POINT('Ctrl Pts',(-48.9539049319844,-43.0903185138448,
-37.1275604547439));
#247417=CARTESIAN_POINT('Ctrl Pts',(-48.9385790570763,-43.0978238481727,
-37.150682142485));
#247418=CARTESIAN_POINT('Ctrl Pts',(-48.9223950612735,-43.1057494184902,
-37.1750984514786));
#247419=CARTESIAN_POINT('Ctrl Pts',(-48.9065095058817,-43.1146407285902,
-37.1982002688633));
#247420=CARTESIAN_POINT('Ctrl Pts',(-48.8910609812166,-43.1241913276533,
-37.2199301095669));
#247421=CARTESIAN_POINT('Ctrl Pts',(-48.8877410902348,-43.126243753266,
-37.224599856598));
#247422=CARTESIAN_POINT('Ctrl Pts',(-48.8844414069668,-43.1283264551359,
-37.2292063289032));
#247423=CARTESIAN_POINT('Ctrl Pts',(-48.8811633453352,-43.1304361250316,
-37.2337490904038));
#247424=CARTESIAN_POINT('Ctrl Pts',(-48.87925775696,-43.1316625090599,-37.2363898685463));
#247425=CARTESIAN_POINT('Ctrl Pts',(-48.8773584741306,-43.1328991103173,
-37.2390101440911));
#247426=CARTESIAN_POINT('Ctrl Pts',(-48.8754660681914,-43.134145042483,
-37.2416094617211));
#247427=CARTESIAN_POINT('Ctrl Pts',(-48.8633226216908,-43.1421401085966,
-37.2582891148152));
#247428=CARTESIAN_POINT('Ctrl Pts',(-48.8514789480032,-43.1505096699715,
-37.2740888990657));
#247429=CARTESIAN_POINT('Ctrl Pts',(-48.8399944210421,-43.159099822315,
-37.2890302768204));
#247430=CARTESIAN_POINT('Ctrl Pts',(-48.834685217634,-43.1630709798779,
-37.295937554235));
#247431=CARTESIAN_POINT('Ctrl Pts',(-48.8294523536931,-43.1670898452388,
-37.3026617223202));
#247432=CARTESIAN_POINT('Ctrl Pts',(-48.8242997622521,-43.1711439171208,
-37.309206443355));
#247433=CARTESIAN_POINT('Ctrl Pts',(-48.8161505895126,-43.1775557066917,
-37.3195573634414));
#247434=CARTESIAN_POINT('Ctrl Pts',(-48.8082033886358,-43.1840546475917,
-37.329458206654));
#247435=CARTESIAN_POINT('Ctrl Pts',(-48.8004734072819,-43.1905952224304,
-37.3389225331823));
#247436=CARTESIAN_POINT('Ctrl Pts',(-48.796608416605,-43.1938655098497,
-37.3436546964465));
#247437=CARTESIAN_POINT('Ctrl Pts',(-48.7927977248867,-43.1971462475385,
-37.3482776875658));
#247438=CARTESIAN_POINT('Ctrl Pts',(-48.7890429180782,-43.2004323433745,
-37.3527934738198));
#247439=CARTESIAN_POINT('Ctrl Pts',(-48.7869512675521,-43.2022628940351,
-37.3553090351191));
#247440=CARTESIAN_POINT('Ctrl Pts',(-48.7852402434882,-43.2037739309092,
-37.3573565500108));
#247441=CARTESIAN_POINT('Ctrl Pts',(-48.783302773363,-43.2054983650398,
-37.3596657888437));
#247442=CARTESIAN_POINT('Ctrl Pts',(-48.7817622121791,-43.2068695326521,
-37.3615019584258));
#247443=CARTESIAN_POINT('Ctrl Pts',(-48.7800784456113,-43.2083758932927,
-37.3635034554526));
#247444=CARTESIAN_POINT('Ctrl Pts',(-48.7779479513844,-43.2103018304306,
-37.3660211095965));
#247445=CARTESIAN_POINT('Ctrl Pts',(-48.7761984141342,-43.2118833877622,
-37.3680885780985));
#247446=CARTESIAN_POINT('Ctrl Pts',(-48.7744507032931,-43.2134753302845,
-37.370145189086));
#247447=CARTESIAN_POINT('Ctrl Pts',(-48.7727050281733,-43.215077463822,
-37.3721906661398));
#247448=CARTESIAN_POINT('Ctrl Pts',(-48.749680734094,-43.2362085398765,
-37.3991691483819));
#247449=CARTESIAN_POINT('Ctrl Pts',(-48.7269086677561,-43.2591448935121,
-37.4243779608413));
#247450=CARTESIAN_POINT('Ctrl Pts',(-48.7044148467678,-43.2837824910303,
-37.4477732221221));
#247451=CARTESIAN_POINT('Ctrl Pts',(-48.6913853473366,-43.2980537685965,
-37.4613248789841));
#247452=CARTESIAN_POINT('Ctrl Pts',(-48.6784491398924,-43.3128951477292,
-37.4742687062647));
#247453=CARTESIAN_POINT('Ctrl Pts',(-48.6656107043938,-43.3282806397202,
-37.4866016703672));
#247454=CARTESIAN_POINT('Ctrl Pts',(-48.6460866766756,-43.3516780990231,
-37.5053570033683));
#247455=CARTESIAN_POINT('Ctrl Pts',(-48.6268227356246,-43.3763363759805,
-37.5226335144684));
#247456=CARTESIAN_POINT('Ctrl Pts',(-48.6080585338523,-43.40181969179,-37.5382668320716));
#247457=CARTESIAN_POINT('Ctrl Pts',(-48.5924087617698,-43.4230733581684,
-37.5513053753761));
#247458=CARTESIAN_POINT('Ctrl Pts',(-48.577106383062,-43.4449007487233,
-37.5632014659455));
#247459=CARTESIAN_POINT('Ctrl Pts',(-48.5622752927423,-43.4670574296315,
-37.5738817239087));
#247460=CARTESIAN_POINT('Ctrl Pts',(-48.5609740374997,-43.4690014200306,
-37.5748187920114));
#247461=CARTESIAN_POINT('Ctrl Pts',(-48.5596754374432,-43.4709494581627,
-37.5757471545326));
#247462=CARTESIAN_POINT('Ctrl Pts',(-48.5583795328176,-43.4729014153975,
-37.5766668154231));
#247463=CARTESIAN_POINT('Ctrl Pts',(-48.5393600363684,-43.501549545024,
-37.5901643265022));
#247464=CARTESIAN_POINT('Ctrl Pts',(-48.5210197611396,-43.530904729223,
-37.6017244902742));
#247465=CARTESIAN_POINT('Ctrl Pts',(-48.5034701459434,-43.560633202674,
-37.611456384112));
#247466=CARTESIAN_POINT('Ctrl Pts',(-48.4857114947968,-43.59071577618,-37.6213041959147));
#247467=CARTESIAN_POINT('Ctrl Pts',(-48.4687624047102,-43.6211806953529,
-37.6292799395048));
#247468=CARTESIAN_POINT('Ctrl Pts',(-48.4527142239903,-43.6517295750421,
-37.6355052155685));
#247469=CARTESIAN_POINT('Ctrl Pts',(-48.4363750855775,-43.6828323138703,
-37.6418433575073));
#247470=CARTESIAN_POINT('Ctrl Pts',(-48.4209697936999,-43.7140221500743,
-37.6463669886134));
#247471=CARTESIAN_POINT('Ctrl Pts',(-48.4065704198427,-43.7450317991596,
-37.6492131468641));
#247472=CARTESIAN_POINT('Ctrl Pts',(-48.3998182147374,-43.7595729530278,
-37.6505477774155));
#247473=CARTESIAN_POINT('Ctrl Pts',(-48.3932868585182,-43.7740751531259,
-37.6515136723023));
#247474=CARTESIAN_POINT('Ctrl Pts',(-48.3869820185779,-43.7885142818768,
-37.6521255977635));
#247475=CARTESIAN_POINT('',(-50.4194602329978,-42.5110618584059,-37.075654526771));
#247476=CARTESIAN_POINT('Origin',(-49.5512974538022,-42.1514570609157,-36.7336343834439));
#247477=CARTESIAN_POINT('',(-49.9605657445604,-42.6569090739569,-38.0871380980686));
#247478=CARTESIAN_POINT('Origin',(-49.6622328036899,-44.3390837210073,-37.0757458603726));
#247479=CARTESIAN_POINT('Ctrl Pts',(-49.8728085593972,-42.8820630175426,
-37.969462470141));
#247480=CARTESIAN_POINT('Ctrl Pts',(-49.8921616460598,-42.8476319404765,
-37.9909151727652));
#247481=CARTESIAN_POINT('Ctrl Pts',(-49.9092258698084,-42.811480340848,
-38.0115509623024));
#247482=CARTESIAN_POINT('Ctrl Pts',(-49.9385737864525,-42.7361810737982,
-38.050911317004));
#247483=CARTESIAN_POINT('Ctrl Pts',(-49.9508224032009,-42.6971223001809,
-38.0695891203786));
#247484=CARTESIAN_POINT('Ctrl Pts',(-49.96056574456,-42.6569090739567,-38.0871380980685));
#247485=CARTESIAN_POINT('Origin',(-48.14917985945,-41.570680937293,-40.903319168463));
#247486=CARTESIAN_POINT('',(-52.0550036453325,-44.2709183219374,-28.14995));
#247487=CARTESIAN_POINT('',(-53.3058498568936,-43.7066435869166,-28.4919701433257));
#247488=CARTESIAN_POINT('Origin',(-52.4376870776976,-43.3470387894261,-28.14995));
#247489=CARTESIAN_POINT('',(-49.017342638646,-41.9302857347835,-41.2453393117887));
#247490=CARTESIAN_POINT('',(-53.3850683564681,-44.8218491641236,-24.194539546945));
#247491=CARTESIAN_POINT('Ctrl Pts',(-52.0550036453325,-44.2709183219374,
-28.14995));
#247492=CARTESIAN_POINT('Ctrl Pts',(-52.9231664245284,-44.6305231194279,
-28.4919701433257));
#247493=CARTESIAN_POINT('Ctrl Pts',(-53.3058498568936,-43.7066435869166,
-28.4919701433257));
#247494=CARTESIAN_POINT('Ctrl Pts',(-52.1435820782265,-44.3076087101758,
-28.0182405965214));
#247495=CARTESIAN_POINT('Ctrl Pts',(-52.9884077964684,-44.6098608177916,
-28.3480901147829));
#247496=CARTESIAN_POINT('Ctrl Pts',(-53.3944282897846,-43.743333975162,
-28.228551336368));
#247497=CARTESIAN_POINT('Ctrl Pts',(-52.2220105281705,-44.3686099077136,
-27.8866328738247));
#247498=CARTESIAN_POINT('Ctrl Pts',(-53.048435044978,-44.620231423514,-28.1848168586396));
#247499=CARTESIAN_POINT('Ctrl Pts',(-53.4627751400873,-43.8286743072844,
-27.9653358909753));
#247500=CARTESIAN_POINT('Ctrl Pts',(-52.3467027906606,-44.5299708800253,
-27.6435487102698));
#247501=CARTESIAN_POINT('Ctrl Pts',(-53.1352121592815,-44.7138087590227,
-27.8661586695385));
#247502=CARTESIAN_POINT('Ctrl Pts',(-53.5486784427678,-44.0836801124388,
-27.479167563865));
#247503=CARTESIAN_POINT('Ctrl Pts',(-52.3929000186986,-44.6302588784236,
-27.5321945097562));
#247504=CARTESIAN_POINT('Ctrl Pts',(-53.1631899467114,-44.794885409667,
-27.7098964514495));
#247505=CARTESIAN_POINT('Ctrl Pts',(-53.5661839363464,-44.2532360852968,
-27.2564591628373));
#247506=CARTESIAN_POINT('Ctrl Pts',(-52.4459516145522,-44.8547560303666,
-27.3468433305442));
#247507=CARTESIAN_POINT('Ctrl Pts',(-53.1776753975914,-45.0117760871578,
-27.4450855646671));
#247508=CARTESIAN_POINT('Ctrl Pts',(-53.5476330292888,-44.6505969708682,
-26.8857568044149));
#247509=CARTESIAN_POINT('Ctrl Pts',(-52.452784611166,-44.9788747485428,
-27.2729210180269));
#247510=CARTESIAN_POINT('Ctrl Pts',(-53.1651856643124,-45.1471482079303,
-27.3344565761127));
#247511=CARTESIAN_POINT('Ctrl Pts',(-53.5115841014411,-44.8782418126584,
-26.7379121793796));
#247512=CARTESIAN_POINT('Ctrl Pts',(-52.4260229733029,-45.2319244248767,
-27.1738560637643));
#247513=CARTESIAN_POINT('Ctrl Pts',(-53.1017995598561,-45.4406484702319,
-27.1867616325076));
#247514=CARTESIAN_POINT('Ctrl Pts',(-53.3914367413948,-45.356744566022,
-26.539782270854));
#247515=CARTESIAN_POINT('Ctrl Pts',(-52.3924488199414,-45.3607304740787,
-27.1487530935363));
#247516=CARTESIAN_POINT('Ctrl Pts',(-53.0510858309516,-45.5998124623687,
-27.1481429616664));
#247517=CARTESIAN_POINT('Ctrl Pts',(-53.3074055923412,-45.6073645701926,
-26.4895763391844));
#247518=CARTESIAN_POINT('Ctrl Pts',(-52.3412129907762,-45.4820634699211,
-27.1499944128911));
#247519=CARTESIAN_POINT('Ctrl Pts',(-52.9872085841078,-45.752243332221,
-27.1500170503128));
#247520=CARTESIAN_POINT('Ctrl Pts',(-53.2057691169878,-45.8503754979613,
-26.4920589691078));
#247521=CARTESIAN_POINT('Ctrl Pts',(-52.3451505088232,-45.4735032149087,
-27.1499504714879));
#247522=CARTESIAN_POINT('Ctrl Pts',(-52.3627366640159,-45.4303973965223,
-27.149955201081));
#247523=CARTESIAN_POINT('Ctrl Pts',(-52.3783532542793,-45.3862784926915,
-27.1532451336684));
#247524=CARTESIAN_POINT('Ctrl Pts',(-52.391705759617,-45.3414941638924,
-27.1598205284727));
#247525=CARTESIAN_POINT('Ctrl Pts',(-52.3961646350242,-45.3265390871288,
-27.162016286156));
#247526=CARTESIAN_POINT('Ctrl Pts',(-52.4003708846481,-45.3115102106125,
-27.1645784468541));
#247527=CARTESIAN_POINT('Ctrl Pts',(-52.4043130646239,-45.2964216897362,
-27.1675069834584));
#247528=CARTESIAN_POINT('Ctrl Pts',(-52.4096690785004,-45.275921781643,
-27.1714858182115));
#247529=CARTESIAN_POINT('Ctrl Pts',(-52.4144998716781,-45.2554681891212,
-27.1761072098123));
#247530=CARTESIAN_POINT('Ctrl Pts',(-52.4188376180112,-45.2349418246403,
-27.1813926878448));
#247531=CARTESIAN_POINT('Ctrl Pts',(-52.4231338832753,-45.2146117500013,
-27.1866276218246));
#247532=CARTESIAN_POINT('Ctrl Pts',(-52.4269465681568,-45.1942098686581,
-27.1925141192982));
#247533=CARTESIAN_POINT('Ctrl Pts',(-52.4302758447408,-45.1736199006748,
-27.199112847856));
#247534=CARTESIAN_POINT('Ctrl Pts',(-52.4334702013726,-45.1538643474436,
-27.20544416092));
#247535=CARTESIAN_POINT('Ctrl Pts',(-52.4362195192742,-45.1339352959373,
-27.2124313525265));
#247536=CARTESIAN_POINT('Ctrl Pts',(-52.438494965569,-45.1137349982039,
-27.220162175848));
#247537=CARTESIAN_POINT('Ctrl Pts',(-52.4388077184374,-45.1109585314193,
-27.2212247529671));
#247538=CARTESIAN_POINT('Ctrl Pts',(-52.4391111205152,-45.108180141414,
-27.2223002129721));
#247539=CARTESIAN_POINT('Ctrl Pts',(-52.4394050835699,-45.1053999392664,
-27.2233886092791));
#247540=CARTESIAN_POINT('Ctrl Pts',(-52.4434186911884,-45.0674406095399,
-27.2382489655034));
#247541=CARTESIAN_POINT('Ctrl Pts',(-52.4456709126751,-45.0291509483473,
-27.2555192111601));
#247542=CARTESIAN_POINT('Ctrl Pts',(-52.4460185726721,-44.9908310284022,
-27.2752228594763));
#247543=CARTESIAN_POINT('Ctrl Pts',(-52.4462187383754,-44.9687682837951,
-27.2865672610631));
#247544=CARTESIAN_POINT('Ctrl Pts',(-52.4457875494046,-44.9466963412302,
-27.298717887852));
#247545=CARTESIAN_POINT('Ctrl Pts',(-52.4446976007478,-44.9246794826073,
-27.3116756346609));
#247546=CARTESIAN_POINT('Ctrl Pts',(-52.4429172619991,-44.8887168101594,
-27.332841015796));
#247547=CARTESIAN_POINT('Ctrl Pts',(-52.4393794287248,-44.8528972178532,
-27.3561617363975));
#247548=CARTESIAN_POINT('Ctrl Pts',(-52.4339628625585,-44.8175267802565,
-27.3816307628944));
#247549=CARTESIAN_POINT('Ctrl Pts',(-52.431069078058,-44.79863022828,-27.3952375151907));
#247550=CARTESIAN_POINT('Ctrl Pts',(-52.4276390143528,-44.7798625814266,
-27.4094571301389));
#247551=CARTESIAN_POINT('Ctrl Pts',(-52.423654105959,-44.761276036307,-27.4242857303512));
#247552=CARTESIAN_POINT('Ctrl Pts',(-52.4227084790016,-44.7568654109244,
-27.4278045876786));
#247553=CARTESIAN_POINT('Ctrl Pts',(-52.4216502220477,-44.7521007131266,
-27.4316525297199));
#247554=CARTESIAN_POINT('Ctrl Pts',(-52.4206177053084,-44.7476164130445,
-27.4353204873094));
#247555=CARTESIAN_POINT('Ctrl Pts',(-52.4202128499573,-44.745858094932,
-27.4367587131523));
#247556=CARTESIAN_POINT('Ctrl Pts',(-52.4198123437877,-44.7441426586176,
-27.4381688899413));
#247557=CARTESIAN_POINT('Ctrl Pts',(-52.4194259738441,-44.7425074883477,
-27.4395189486769));
#247558=CARTESIAN_POINT('Ctrl Pts',(-52.4190941693375,-44.7411032464454,
-27.4406783441735));
#247559=CARTESIAN_POINT('Ctrl Pts',(-52.4187728116493,-44.7397582037023,
-27.4417933739563));
#247560=CARTESIAN_POINT('Ctrl Pts',(-52.4184684924213,-44.7384957856129,
-27.442843360707));
#247561=CARTESIAN_POINT('Ctrl Pts',(-52.4122187620994,-44.7125698108868,
-27.464406684453));
#247562=CARTESIAN_POINT('Ctrl Pts',(-52.404731444009,-44.6865268769795,
-27.4876002411829));
#247563=CARTESIAN_POINT('Ctrl Pts',(-52.3958714578284,-44.6606022207932,
-27.5124732459137));
#247564=CARTESIAN_POINT('Ctrl Pts',(-52.3870114716477,-44.6346775646069,
-27.5373462506445));
#247565=CARTESIAN_POINT('Ctrl Pts',(-52.3767786586423,-44.6088708924118,
-27.5638990563341));
#247566=CARTESIAN_POINT('Ctrl Pts',(-52.3650469817685,-44.5834604974678,
-27.5921469614712));
#247567=CARTESIAN_POINT('Ctrl Pts',(-52.3536937597227,-44.5588698222236,
-27.619483611023));
#247568=CARTESIAN_POINT('Ctrl Pts',(-52.3409355488873,-44.5346481494281,
-27.6484094417132));
#247569=CARTESIAN_POINT('Ctrl Pts',(-52.3266618289586,-44.5110837509137,
-27.6789131759605));
#247570=CARTESIAN_POINT('Ctrl Pts',(-52.3138131594986,-44.4898719596604,
-27.7063714980095));
#247571=CARTESIAN_POINT('Ctrl Pts',(-52.2997365041,-44.4691930457479,-27.7351082044668));
#247572=CARTESIAN_POINT('Ctrl Pts',(-52.2843566594156,-44.4492903938695,
-27.7650907920472));
#247573=CARTESIAN_POINT('Ctrl Pts',(-52.2837186874352,-44.4484648111348,
-27.7663345010161));
#247574=CARTESIAN_POINT('Ctrl Pts',(-52.2830784779469,-44.4476405726622,
-27.767580343073));
#247575=CARTESIAN_POINT('Ctrl Pts',(-52.2824360261253,-44.4468176910827,
-27.7688283177016));
#247576=CARTESIAN_POINT('Ctrl Pts',(-52.2813248295301,-44.4453944198295,
-27.7709868377828));
#247577=CARTESIAN_POINT('Ctrl Pts',(-52.2802069226367,-44.4439752050525,
-27.773151741833));
#247578=CARTESIAN_POINT('Ctrl Pts',(-52.2790823052009,-44.4425601308152,
-27.7753230093723));
#247579=CARTESIAN_POINT('Ctrl Pts',(-52.2780757844132,-44.4412936542423,
-27.7772662710044));
#247580=CARTESIAN_POINT('Ctrl Pts',(-52.2766634267718,-44.4395338119596,
-27.7799843776605));
#247581=CARTESIAN_POINT('Ctrl Pts',(-52.2759205732601,-44.4386144114997,
-27.7814106877139));
#247582=CARTESIAN_POINT('Ctrl Pts',(-52.2758334131032,-44.438506536815,
-27.7815780388889));
#247583=CARTESIAN_POINT('Ctrl Pts',(-52.2757555052074,-44.4384101877566,
-27.7817275847392));
#247584=CARTESIAN_POINT('Ctrl Pts',(-52.2756886070813,-44.4383274928831,
-27.7818559746203));
#247585=CARTESIAN_POINT('Ctrl Pts',(-52.2676800702558,-44.4284278891467,
-27.7972258384781));
#247586=CARTESIAN_POINT('Ctrl Pts',(-52.2586467068395,-44.4178780252673,
-27.8142376774287));
#247587=CARTESIAN_POINT('Ctrl Pts',(-52.2484496368236,-44.4068934908634,
-27.8329545686498));
#247588=CARTESIAN_POINT('Ctrl Pts',(-52.2386193771832,-44.39630409361,-27.8509981733398));
#247589=CARTESIAN_POINT('Ctrl Pts',(-52.2277071249877,-44.3853106597761,
-27.8706270447069));
#247590=CARTESIAN_POINT('Ctrl Pts',(-52.215582220397,-44.3741516473034,
-27.8918817944962));
#247591=CARTESIAN_POINT('Ctrl Pts',(-52.2042196016309,-44.3636941955698,
-27.911800270309));
#247592=CARTESIAN_POINT('Ctrl Pts',(-52.1917916195219,-44.3530914633972,
-27.9331470466369));
#247593=CARTESIAN_POINT('Ctrl Pts',(-52.1781914581759,-44.3425794767405,
-27.9559337338037));
#247594=CARTESIAN_POINT('Ctrl Pts',(-52.165085428788,-44.332449420005,-27.9778925167962));
#247595=CARTESIAN_POINT('Ctrl Pts',(-52.1508905243962,-44.3224035921207,
-28.0011889148053));
#247596=CARTESIAN_POINT('Ctrl Pts',(-52.1355169284213,-44.31269102401,-28.025806121144));
#247597=CARTESIAN_POINT('Ctrl Pts',(-52.120939443385,-44.3034814144607,
-28.0491485426324));
#247598=CARTESIAN_POINT('Ctrl Pts',(-52.1053019503684,-44.2945715114819,
-28.0736787774362));
#247599=CARTESIAN_POINT('Ctrl Pts',(-52.0885370500198,-44.2862079032681,
-28.0993528411084));
#247600=CARTESIAN_POINT('Ctrl Pts',(-52.0778243289322,-44.2808635826806,
-28.1157584908639));
#247601=CARTESIAN_POINT('Ctrl Pts',(-52.0666514599927,-44.2757430047416,
-28.1326305840812));
#247602=CARTESIAN_POINT('Ctrl Pts',(-52.0550036453325,-44.2709183219374,
-28.14995));
#247603=CARTESIAN_POINT('Ctrl Pts',(-53.3058498568936,-43.7066435869166,
-28.4919701433257));
#247604=CARTESIAN_POINT('Ctrl Pts',(-53.325878097415,-43.7149395557728,
-28.4324091977161));
#247605=CARTESIAN_POINT('Ctrl Pts',(-53.3450421162736,-43.7257975480542,
-28.3723481914006));
#247606=CARTESIAN_POINT('Ctrl Pts',(-53.3631923272661,-43.7392286476817,
-28.3121551709553));
#247607=CARTESIAN_POINT('Ctrl Pts',(-53.3817311398638,-43.7529473112873,
-28.2506733994109));
#247608=CARTESIAN_POINT('Ctrl Pts',(-53.3992119966698,-43.7693504901722,
-28.1890545402301));
#247609=CARTESIAN_POINT('Ctrl Pts',(-53.4154902120498,-43.7884000440542,
-28.1277059557092));
#247610=CARTESIAN_POINT('Ctrl Pts',(-53.4318778232817,-43.807577618246,
-28.0659450851662));
#247611=CARTESIAN_POINT('Ctrl Pts',(-53.4470463242961,-43.8294371266463,
-28.0044589051888));
#247612=CARTESIAN_POINT('Ctrl Pts',(-53.4608667701963,-43.8538903731411,
-27.9436674521647));
#247613=CARTESIAN_POINT('Ctrl Pts',(-53.4746634610095,-43.8783015885027,
-27.8829804897104));
#247614=CARTESIAN_POINT('Ctrl Pts',(-53.4871165121676,-43.9052973926726,
-27.8229866659694));
#247615=CARTESIAN_POINT('Ctrl Pts',(-53.4981196516723,-43.934743987147,
-27.7640964128422));
#247616=CARTESIAN_POINT('Ctrl Pts',(-53.5007377563813,-43.9417505571923,
-27.7500839713058));
#247617=CARTESIAN_POINT('Ctrl Pts',(-53.503273878774,-43.9488956857912,
-27.7361339461954));
#247618=CARTESIAN_POINT('Ctrl Pts',(-53.5057267914276,-43.9561772098616,
-27.7222517274201));
#247619=CARTESIAN_POINT('Ctrl Pts',(-53.516015172449,-43.98671849063,-27.6640248044291));
#247620=CARTESIAN_POINT('Ctrl Pts',(-53.524834739455,-44.0196559383853,
-27.607006864364));
#247621=CARTESIAN_POINT('Ctrl Pts',(-53.5321633779772,-44.0547175334498,
-27.5515400465457));
#247622=CARTESIAN_POINT('Ctrl Pts',(-53.539448489013,-44.0895708847729,
-27.4964026666108));
#247623=CARTESIAN_POINT('Ctrl Pts',(-53.5452603272204,-44.1265226675562,
-27.4427986309046));
#247624=CARTESIAN_POINT('Ctrl Pts',(-53.5496025507427,-44.1652740000725,
-27.3910329022814));
#247625=CARTESIAN_POINT('Ctrl Pts',(-53.5538697570887,-44.2033558563332,
-27.3401614893866));
#247626=CARTESIAN_POINT('Ctrl Pts',(-53.5567177527472,-44.2431750607486,
-27.2910658408008));
#247627=CARTESIAN_POINT('Ctrl Pts',(-53.5581740600656,-44.2844256199221,
-27.2439978212674));
#247628=CARTESIAN_POINT('Ctrl Pts',(-53.5591211928104,-44.3112535805061,
-27.2133863823412));
#247629=CARTESIAN_POINT('Ctrl Pts',(-53.5594801618893,-44.3386865381858,
-27.1836317992188));
#247630=CARTESIAN_POINT('Ctrl Pts',(-53.5592639447716,-44.3666367581605,
-27.1547933762998));
#247631=CARTESIAN_POINT('Ctrl Pts',(-55.7504626785233,-26.3185679674161,
-36.6521851368644));
#247632=CARTESIAN_POINT('Ctrl Pts',(-55.5392505223476,-26.2310810277901,
-37.5833004572826));
#247633=CARTESIAN_POINT('Ctrl Pts',(-55.8969434195062,-25.3423960630483,
-37.6224808631404));
#247634=CARTESIAN_POINT('Ctrl Pts',(-55.9208644997853,-26.3891507128358,
-36.6974706218906));
#247635=CARTESIAN_POINT('Ctrl Pts',(-55.6480848386771,-26.2761616776646,
-37.5999312032258));
#247636=CARTESIAN_POINT('Ctrl Pts',(-55.996440168022,-25.3971431190627,
-37.6496522218102));
#247637=CARTESIAN_POINT('Ctrl Pts',(-56.0836332067825,-26.456571718804,
-36.762150428292));
#247638=CARTESIAN_POINT('Ctrl Pts',(-55.7548998347942,-26.3204058977241,
-37.6301299838414));
#247639=CARTESIAN_POINT('Ctrl Pts',(-56.0914939922152,-25.4493175282016,
-37.6884594400956));
#247640=CARTESIAN_POINT('Ctrl Pts',(-56.2387979627755,-26.5208430651387,
-36.8455500552174));
#247641=CARTESIAN_POINT('Ctrl Pts',(-55.8586323634263,-26.3633733179405,
-37.6741999657538));
#247642=CARTESIAN_POINT('Ctrl Pts',(-56.182121826823,-25.498964054333,-37.7384998141522));
#247643=CARTESIAN_POINT('',(-55.8969434190161,-25.3423960644772,-37.6224808629378));
#247644=CARTESIAN_POINT('Origin',(-55.5095456070917,-25.1140012264302,-39.2553865411486));
#247645=CARTESIAN_POINT('',(-55.7504626788662,-26.3185679665883,-36.6521851368644));
#247646=CARTESIAN_POINT('Origin',(-55.1862083484817,-26.0848461712916,-39.1409509186699));
#247647=CARTESIAN_POINT('Origin',(-56.1331461108883,-25.3946884349048,-36.6521851368644));
#247648=CARTESIAN_POINT('Ctrl Pts',(-55.8969434195062,-25.3423960630483,
-37.6224808631404));
#247649=CARTESIAN_POINT('Ctrl Pts',(-55.5392505223476,-26.23108102779,-37.5833004572826));
#247650=CARTESIAN_POINT('Ctrl Pts',(-55.7504626785233,-26.3185679674161,
-36.6521851368644));
#247651=CARTESIAN_POINT('Ctrl Pts',(-55.0816420516339,-25.0053755109404,
-37.405845897407));
#247652=CARTESIAN_POINT('Ctrl Pts',(-54.7245658074498,-25.8936275698287,
-37.3661635279098));
#247653=CARTESIAN_POINT('Ctrl Pts',(-54.9353008930509,-25.9809169003452,
-36.4355501696994));
#247654=CARTESIAN_POINT('Ctrl Pts',(-54.2663041831515,-24.6683705249141,
-37.1893551119314));
#247655=CARTESIAN_POINT('Ctrl Pts',(-53.9096353215527,-25.5560723101748,
-37.1490863785069));
#247656=CARTESIAN_POINT('Ctrl Pts',(-54.1201064257051,-25.643252295999,
-36.2190593841676));
#247657=CARTESIAN_POINT('Ctrl Pts',(-53.45092477896,-24.3313834513715,-36.9730300997693));
#247658=CARTESIAN_POINT('Ctrl Pts',(-53.094385962218,-25.218384968819,-36.9320687979064));
#247659=CARTESIAN_POINT('Ctrl Pts',(-53.3048743824714,-25.3055721272105,
-36.0027343734933));
#247660=CARTESIAN_POINT('',(-53.3048743827289,-25.3055721265897,-36.0027343734921));
#247661=CARTESIAN_POINT('',(-53.4509247784284,-24.3313834527923,-36.973030099559));
#247662=CARTESIAN_POINT('Origin',(-53.6875578148366,-24.3816925946992,-36.0027343734933));
#247663=CARTESIAN_POINT('Origin',(2171.9425404878,-684.86429331655,-7395.89927355314));
#247664=CARTESIAN_POINT('Origin',(1653.54988594156,681.696820180718,-7571.86104389537));
#247665=CARTESIAN_POINT('Origin',(-53.6875578148366,-24.3816925946992,-36.0027343734933));
#247666=CARTESIAN_POINT('',(-52.7094196628928,-24.1737364557848,-36.0027343734933));
#247667=CARTESIAN_POINT('Origin',(-53.6875578148366,-24.3816925946992,-36.0027343734933));
#247668=CARTESIAN_POINT('Origin',(-53.6875578148366,-24.3816925946992,-36.0027343734933));
#247669=CARTESIAN_POINT('Origin',(-53.6875578148366,-24.3816925946992,-55.24995));
#247670=CARTESIAN_POINT('',(-53.3048743824714,-25.3055721272105,-28.64995));
#247671=CARTESIAN_POINT('',(-52.7094196628928,-24.1737364557848,-28.64995));
#247672=CARTESIAN_POINT('Origin',(-53.6875578148365,-24.3816925946992,-28.64995));
#247673=CARTESIAN_POINT('',(-52.7094196628929,-24.1737364557848,-55.24995));
#247674=CARTESIAN_POINT('',(-53.3048743824714,-25.3055721272105,-36.0027343734933));
#247675=CARTESIAN_POINT('Ctrl Pts',(-52.7094196628928,-24.1737364557848,
-28.64995));
#247676=CARTESIAN_POINT('Ctrl Pts',(-52.5364563745167,-24.9872829667439,
-28.64995));
#247677=CARTESIAN_POINT('Ctrl Pts',(-53.3048743824714,-25.3055721272105,
-28.64995));
#247678=CARTESIAN_POINT('Ctrl Pts',(-52.709419661177,-24.1737364638552,
-28.4522245494749));
#247679=CARTESIAN_POINT('Ctrl Pts',(-52.5364564758209,-24.9872830087068,
-28.4725838150348));
#247680=CARTESIAN_POINT('Ctrl Pts',(-53.3048744251021,-25.3055721448687,
-28.584041512097));
#247681=CARTESIAN_POINT('Ctrl Pts',(-52.7478129283917,-24.18436087427,-28.2540622406394));
#247682=CARTESIAN_POINT('Ctrl Pts',(-52.5661365121454,-24.9995768822825,
-28.2939908458137));
#247683=CARTESIAN_POINT('Ctrl Pts',(-53.3173284366389,-25.3107307653532,
-28.5179874195064));
#247684=CARTESIAN_POINT('Ctrl Pts',(-52.8580751908351,-24.2149033446468,
-27.980658832839));
#247685=CARTESIAN_POINT('Ctrl Pts',(-52.652344235038,-25.0352852902864,
-28.0433521906345));
#247686=CARTESIAN_POINT('Ctrl Pts',(-53.3530964953807,-25.3255463803838,
-28.4268529412997));
#247687=CARTESIAN_POINT('Ctrl Pts',(-52.9030108008295,-24.227353663694,
-27.8942996676949));
#247688=CARTESIAN_POINT('Ctrl Pts',(-52.6878047550409,-25.0499735186003,
-27.9629661172779));
#247689=CARTESIAN_POINT('Ctrl Pts',(-53.3676733222451,-25.3315842997674,
-28.3980665530275));
#247690=CARTESIAN_POINT('Ctrl Pts',(-53.0090582923966,-24.2567524735255,
-27.7310236386286));
#247691=CARTESIAN_POINT('Ctrl Pts',(-52.7723574461003,-25.0849963899722,
-27.8083075481136));
#247692=CARTESIAN_POINT('Ctrl Pts',(-53.4020750585865,-25.3458339655292,
-28.343641215747));
#247693=CARTESIAN_POINT('Ctrl Pts',(-53.0705147380728,-24.2737967964412,
-27.6541049946696));
#247694=CARTESIAN_POINT('Ctrl Pts',(-52.8218880255259,-25.1055126277224,
-27.7338993339231));
#247695=CARTESIAN_POINT('Ctrl Pts',(-53.4220117490162,-25.354092013094,
-28.3180016675465));
#247696=CARTESIAN_POINT('Ctrl Pts',(-53.271425280039,-24.329554436308,-27.4475644489341));
#247697=CARTESIAN_POINT('Ctrl Pts',(-52.986650618978,-25.1737595285021,
-27.5280515041845));
#247698=CARTESIAN_POINT('Ctrl Pts',(-53.487189224505,-25.3810894074027,
-28.2491548109981));
#247699=CARTESIAN_POINT('Ctrl Pts',(-53.4327530160742,-24.374374360655,
-27.3369024763037));
#247700=CARTESIAN_POINT('Ctrl Pts',(-53.1222572959679,-25.2299296532595,
-27.4101121807186));
#247701=CARTESIAN_POINT('Ctrl Pts',(-53.5395274002361,-25.4027685896203,
-28.2122674917371));
#247702=CARTESIAN_POINT('Ctrl Pts',(-53.7793279888276,-24.4708259099888,
-27.1890241015641));
#247703=CARTESIAN_POINT('Ctrl Pts',(-53.4249980376239,-25.3553289743366,
-27.233364160377));
#247704=CARTESIAN_POINT('Ctrl Pts',(-53.6519699663366,-25.4493438254873,
-28.1629747008856));
#247705=CARTESIAN_POINT('Ctrl Pts',(-53.9688606392783,-24.5236518439783,
-27.14995));
#247706=CARTESIAN_POINT('Ctrl Pts',(-53.5971493048004,-25.4266363639807,
-27.1731944252321));
#247707=CARTESIAN_POINT('Ctrl Pts',(-53.7134648732951,-25.4748158499664,
-28.1499500287456));
#247708=CARTESIAN_POINT('Ctrl Pts',(-54.1572878000337,-24.5762611252212,
-27.14995));
#247709=CARTESIAN_POINT('Ctrl Pts',(-53.7746043676686,-25.5001406577324,
-27.14995));
#247710=CARTESIAN_POINT('Ctrl Pts',(-53.7746043676686,-25.5001406577325,
-28.14995));
#247711=CARTESIAN_POINT('',(-53.7746043676686,-25.5001406577325,-28.14995));
#247712=CARTESIAN_POINT('Origin',(-54.1572878000337,-24.5762611252212,-28.14995));
#247713=CARTESIAN_POINT('Ctrl Pts',(-52.7094196628928,-24.1737364557848,
-28.64995));
#247714=CARTESIAN_POINT('Ctrl Pts',(-52.7094196623825,-24.1737364581851,
-28.5911408946036));
#247715=CARTESIAN_POINT('Ctrl Pts',(-52.7128129245313,-24.1746866093358,
-28.5317681320255));
#247716=CARTESIAN_POINT('Ctrl Pts',(-52.7197005445987,-24.1766085300182,
-28.4722462243672));
#247717=CARTESIAN_POINT('Ctrl Pts',(-52.7264036735814,-24.1784789703302,
-28.4143186644234));
#247718=CARTESIAN_POINT('Ctrl Pts',(-52.736416539613,-24.1812698432637,
-28.3562495690729));
#247719=CARTESIAN_POINT('Ctrl Pts',(-52.7498419130618,-24.1850037883381,
-28.2984688589346));
#247720=CARTESIAN_POINT('Ctrl Pts',(-52.7627900625724,-24.1886050050396,
-28.242742046079));
#247721=CARTESIAN_POINT('Ctrl Pts',(-52.7789125032754,-24.1930834657548,
-28.1872833154782));
#247722=CARTESIAN_POINT('Ctrl Pts',(-52.7983093839467,-24.1984616617822,
-28.1325264875571));
#247723=CARTESIAN_POINT('Ctrl Pts',(-52.8031630965455,-24.1998074564107,
-28.1188245985753));
#247724=CARTESIAN_POINT('Ctrl Pts',(-52.8082218780349,-24.2012095986938,
-28.1051669098548));
#247725=CARTESIAN_POINT('Ctrl Pts',(-52.8134873707718,-24.2026684605618,
-28.0915607337429));
#247726=CARTESIAN_POINT('Ctrl Pts',(-52.8160396530933,-24.203375598059,
-28.0849655669677));
#247727=CARTESIAN_POINT('Ctrl Pts',(-52.8186421023036,-24.2040965209239,
-28.0783783736381));
#247728=CARTESIAN_POINT('Ctrl Pts',(-52.8212948296775,-24.2048312666952,
-28.0718006689512));
#247729=CARTESIAN_POINT('Ctrl Pts',(-52.8382986680715,-24.2095409471842,
-28.0296379391516));
#247730=CARTESIAN_POINT('Ctrl Pts',(-52.8572442526181,-24.2147843387079,
-27.9880389891984));
#247731=CARTESIAN_POINT('Ctrl Pts',(-52.878156523599,-24.2205704318867,
-27.947193588991));
#247732=CARTESIAN_POINT('Ctrl Pts',(-52.8990687945799,-24.2263565250655,
-27.9063481887835));
#247733=CARTESIAN_POINT('Ctrl Pts',(-52.9219478322349,-24.2326853437507,
-27.8662563850818));
#247734=CARTESIAN_POINT('Ctrl Pts',(-52.9467712010785,-24.2395527832638,
-27.8270804380994));
#247735=CARTESIAN_POINT('Ctrl Pts',(-52.949825104249,-24.2403976522835,
-27.8222608042517));
#247736=CARTESIAN_POINT('Ctrl Pts',(-52.9529075011859,-24.2412504051661,
-27.8174563757837));
#247737=CARTESIAN_POINT('Ctrl Pts',(-52.9560186463722,-24.2421111243394,
-27.8126668029462));
#247738=CARTESIAN_POINT('Ctrl Pts',(-52.9780675057062,-24.2482110890927,
-27.7787228333006));
#247739=CARTESIAN_POINT('Ctrl Pts',(-53.0016171799217,-24.2547269870702,
-27.7455215338308));
#247740=CARTESIAN_POINT('Ctrl Pts',(-53.0265760983851,-24.2616377598036,
-27.7132033055052));
#247741=CARTESIAN_POINT('Ctrl Pts',(-53.0289546891742,-24.2622963580675,
-27.7101233707585));
#247742=CARTESIAN_POINT('Ctrl Pts',(-53.0313461012784,-24.2629585489486,
-27.7070514878665));
#247743=CARTESIAN_POINT('Ctrl Pts',(-53.0337502686034,-24.2636243179425,
-27.7039877996));
#247744=CARTESIAN_POINT('Ctrl Pts',(-53.049345815812,-24.2679430821423,
-27.6841140185629));
#247745=CARTESIAN_POINT('Ctrl Pts',(-53.0654807379639,-24.2724132274182,
-27.6645804228689));
#247746=CARTESIAN_POINT('Ctrl Pts',(-53.0821467732563,-24.2770331862523,
-27.6454233566967));
#247747=CARTESIAN_POINT('Ctrl Pts',(-53.0904797909025,-24.2793431656693,
-27.6358448236106));
#247748=CARTESIAN_POINT('Ctrl Pts',(-53.0989456970375,-24.2816906220258,
-27.6263605258861));
#247749=CARTESIAN_POINT('Ctrl Pts',(-53.107543962866,-24.2840754684918,
-27.6169758713563));
#247750=CARTESIAN_POINT('Ctrl Pts',(-53.1118430957802,-24.2852678917247,
-27.6122835440914));
#247751=CARTESIAN_POINT('Ctrl Pts',(-53.1161753245165,-24.2864696637492,
-27.6076161364291));
#247752=CARTESIAN_POINT('Ctrl Pts',(-53.1205406140096,-24.2876807803625,
-27.6029743847767));
#247753=CARTESIAN_POINT('Ctrl Pts',(-53.1227232587562,-24.2882863386692,
-27.6006535089506));
#247754=CARTESIAN_POINT('Ctrl Pts',(-53.1249141690336,-24.2888942331957,
-27.5983390477616));
#247755=CARTESIAN_POINT('Ctrl Pts',(-53.1271133420458,-24.289504463756,
-27.5960310976378));
#247756=CARTESIAN_POINT('Ctrl Pts',(-53.1290394097302,-24.2900389125492,
-27.5940097613784));
#247757=CARTESIAN_POINT('Ctrl Pts',(-53.1316083240647,-24.2907518064033,
-27.5913323973162));
#247758=CARTESIAN_POINT('Ctrl Pts',(-53.1331478191429,-24.291179042896,
-27.5897360553741));
#247759=CARTESIAN_POINT('Ctrl Pts',(-53.1333661106969,-24.2912396225752,
-27.5895097032615));
#247760=CARTESIAN_POINT('Ctrl Pts',(-53.1335636543095,-24.2912944447278,
-27.5893050130261));
#247761=CARTESIAN_POINT('Ctrl Pts',(-53.1337356439429,-24.2913421754602,
-27.5891268809258));
#247762=CARTESIAN_POINT('Ctrl Pts',(-53.1349790940228,-24.2916872589505,
-27.5878390220597));
#247763=CARTESIAN_POINT('Ctrl Pts',(-53.1362288224179,-24.292034158616,
-27.5865494247887));
#247764=CARTESIAN_POINT('Ctrl Pts',(-53.1374848551265,-24.2923828799776,
-27.5852581657108));
#247765=CARTESIAN_POINT('Ctrl Pts',(-53.1573367030932,-24.2978944907865,
-27.5648495579378));
#247766=CARTESIAN_POINT('Ctrl Pts',(-53.1788814445988,-24.3038939694486,
-27.5439062900081));
#247767=CARTESIAN_POINT('Ctrl Pts',(-53.2022803852861,-24.3104194037623,
-27.5226638270178));
#247768=CARTESIAN_POINT('Ctrl Pts',(-53.2241989150423,-24.316531985015,
-27.5027653383055));
#247769=CARTESIAN_POINT('Ctrl Pts',(-53.2477448421254,-24.3231061872658,
-27.4826043546765));
#247770=CARTESIAN_POINT('Ctrl Pts',(-53.2730374239921,-24.330169670055,
-27.4624174062464));
#247771=CARTESIAN_POINT('Ctrl Pts',(-53.2974626786647,-24.3369909335745,
-27.4429227038444));
#247772=CARTESIAN_POINT('Ctrl Pts',(-53.32351725015,-24.34426860855,-27.4234036353704));
#247773=CARTESIAN_POINT('Ctrl Pts',(-53.3512899421954,-24.3520224739381,
-27.4041157829931));
#247774=CARTESIAN_POINT('Ctrl Pts',(-53.3776321832186,-24.3593769713192,
-27.3858213643135));
#247775=CARTESIAN_POINT('Ctrl Pts',(-53.4055203797343,-24.3671599432765,
-27.367734961942));
#247776=CARTESIAN_POINT('Ctrl Pts',(-53.4350087013824,-24.3753822836722,
-27.3501144502417));
#247777=CARTESIAN_POINT('Ctrl Pts',(-53.4606967054725,-24.3825449671316,
-27.3347647880254));
#247778=CARTESIAN_POINT('Ctrl Pts',(-53.4875988516975,-24.3900410344375,
-27.3197691139046));
#247779=CARTESIAN_POINT('Ctrl Pts',(-53.5157338737957,-24.3978729492133,
-27.3053249748031));
#247780=CARTESIAN_POINT('Ctrl Pts',(-53.5444237498552,-24.4058593180685,
-27.2905959811964));
#247781=CARTESIAN_POINT('Ctrl Pts',(-53.5745393269424,-24.414230882692,
-27.2763718188066));
#247782=CARTESIAN_POINT('Ctrl Pts',(-53.6059083724541,-24.4229441848809,
-27.2629869669082));
#247783=CARTESIAN_POINT('Ctrl Pts',(-53.6209445451166,-24.4271207453735,
-27.2565711853336));
#247784=CARTESIAN_POINT('Ctrl Pts',(-53.6363003452189,-24.4313846413295,
-27.250334067976));
#247785=CARTESIAN_POINT('Ctrl Pts',(-53.6519543084626,-24.4357303721746,
-27.2443059491307));
#247786=CARTESIAN_POINT('Ctrl Pts',(-53.6881882089995,-24.445789344254,
-27.2303527888184));
#247787=CARTESIAN_POINT('Ctrl Pts',(-53.725938196618,-24.4562659038156,
-27.2175466562902));
#247788=CARTESIAN_POINT('Ctrl Pts',(-53.7651942802866,-24.4671634152115,
-27.2061405089377));
#247789=CARTESIAN_POINT('Ctrl Pts',(-53.8008938818551,-24.4770736451316,
-27.1957677239357));
#247790=CARTESIAN_POINT('Ctrl Pts',(-53.837839120707,-24.4873320299336,
-27.1865530465471));
#247791=CARTESIAN_POINT('Ctrl Pts',(-53.8759926239344,-24.4979329922837,
-27.1787222605505));
#247792=CARTESIAN_POINT('Ctrl Pts',(-53.9129275881487,-24.5081953832024,
-27.1711415726428));
#247793=CARTESIAN_POINT('Ctrl Pts',(-53.9509952084681,-24.5187789120278,
-27.1648577255513));
#247794=CARTESIAN_POINT('Ctrl Pts',(-53.9901288761984,-24.5296696175481,
-27.1601094004118));
#247795=CARTESIAN_POINT('Ctrl Pts',(-54.0275148318809,-24.540073943479,
-27.1555731357699));
#247796=CARTESIAN_POINT('Ctrl Pts',(-54.0658739630156,-24.5507586832984,
-27.1524383207612));
#247797=CARTESIAN_POINT('Ctrl Pts',(-54.1051139954855,-24.5617023371624,
-27.1509446747599));
#247798=CARTESIAN_POINT('Ctrl Pts',(-54.1223393936945,-24.5665063289994,
-27.1502890013179));
#247799=CARTESIAN_POINT('Ctrl Pts',(-54.1397340652788,-24.571360083541,
-27.14995));
#247800=CARTESIAN_POINT('Ctrl Pts',(-54.1572878000336,-24.5762611252214,
-27.14995));
#247801=CARTESIAN_POINT('Ctrl Pts',(-53.7746043676686,-25.5001406577325,
-28.14995));
#247802=CARTESIAN_POINT('Ctrl Pts',(-53.7400313146559,-25.485820030282,
-28.14995));
#247803=CARTESIAN_POINT('Ctrl Pts',(-53.7054590384781,-25.471499724607,
-28.1541104421107));
#247804=CARTESIAN_POINT('Ctrl Pts',(-53.6718442132407,-25.4575760080969,
-28.1621235025489));
#247805=CARTESIAN_POINT('Ctrl Pts',(-53.6457564066785,-25.4467700848063,
-28.1683422815909));
#247806=CARTESIAN_POINT('Ctrl Pts',(-53.6202442011515,-25.4362025832709,
-28.1768826771709));
#247807=CARTESIAN_POINT('Ctrl Pts',(-53.5957486758074,-25.4260562044559,
-28.187621076324));
#247808=CARTESIAN_POINT('Ctrl Pts',(-53.562916032086,-25.4124564781379,
-28.2020143187052));
#247809=CARTESIAN_POINT('Ctrl Pts',(-53.5314342202936,-25.3994162847254,
-28.2205659399078));
#247810=CARTESIAN_POINT('Ctrl Pts',(-53.5022513514982,-25.3873283446814,
-28.242657912297));
#247811=CARTESIAN_POINT('Ctrl Pts',(-53.4814624525329,-25.3787173007832,
-28.2583954939983));
#247812=CARTESIAN_POINT('Ctrl Pts',(-53.461840238405,-25.3705895135676,
-28.2759308966333));
#247813=CARTESIAN_POINT('Ctrl Pts',(-53.4437375711116,-25.3630911432596,
-28.2950527119614));
#247814=CARTESIAN_POINT('Ctrl Pts',(-53.4271303962018,-25.3562122261793,
-28.3125948413394));
#247815=CARTESIAN_POINT('Ctrl Pts',(-53.4116292338695,-25.3497914345087,
-28.3316389938391));
#247816=CARTESIAN_POINT('Ctrl Pts',(-53.3975863960872,-25.3439747006451,
-28.3517369823159));
#247817=CARTESIAN_POINT('Ctrl Pts',(-53.3932029374535,-25.3421590126289,
-28.3580105505558));
#247818=CARTESIAN_POINT('Ctrl Pts',(-53.3889617532722,-25.3404022566205,
-28.3643871416707));
#247819=CARTESIAN_POINT('Ctrl Pts',(-53.3848741883221,-25.338709131781,
-28.3708538828368));
#247820=CARTESIAN_POINT('Ctrl Pts',(-53.3717588132892,-25.3332765655668,
-28.3916030909026));
#247821=CARTESIAN_POINT('Ctrl Pts',(-53.3601568354504,-25.3284708689956,
-28.4132788617422));
#247822=CARTESIAN_POINT('Ctrl Pts',(-53.3500641460493,-25.3242903401649,
-28.4359756086709));
#247823=CARTESIAN_POINT('Ctrl Pts',(-53.3491805785529,-25.3239243545245,
-28.4379626021337));
#247824=CARTESIAN_POINT('Ctrl Pts',(-53.348308605256,-25.323563171359,-28.4399574365791));
#247825=CARTESIAN_POINT('Ctrl Pts',(-53.3474482388699,-25.3232067959332,
-28.4419601846317));
#247826=CARTESIAN_POINT('Ctrl Pts',(-53.3452788063953,-25.3223081875796,
-28.4470101572176));
#247827=CARTESIAN_POINT('Ctrl Pts',(-53.3431878049941,-25.3214420664403,
-28.4520995820139));
#247828=CARTESIAN_POINT('Ctrl Pts',(-53.3411738091334,-25.3206078420402,
-28.4572311007019));
#247829=CARTESIAN_POINT('Ctrl Pts',(-53.3367395978111,-25.3187711315721,
-28.4685291568261));
#247830=CARTESIAN_POINT('Ctrl Pts',(-53.3327048917567,-25.3170999016042,
-28.4799940523333));
#247831=CARTESIAN_POINT('Ctrl Pts',(-53.3290655208329,-25.315592424809,
-28.4916214078187));
#247832=CARTESIAN_POINT('Ctrl Pts',(-53.3209950143511,-25.3122495115691,
-28.5174057122425));
#247833=CARTESIAN_POINT('Ctrl Pts',(-53.3148900299868,-25.3097207442473,
-28.5439203032342));
#247834=CARTESIAN_POINT('Ctrl Pts',(-53.3108262630393,-25.3080374768633,
-28.5708597425681));
#247835=CARTESIAN_POINT('Ctrl Pts',(-53.3068954035518,-25.3064092615518,
-28.5969181145328));
#247836=CARTESIAN_POINT('Ctrl Pts',(-53.3048743824714,-25.3055721272105,
-28.6233752345599));
#247837=CARTESIAN_POINT('Ctrl Pts',(-53.3048743824714,-25.3055721272105,
-28.64995));
#247838=CARTESIAN_POINT('Origin',(0.757869275948407,-1.82965828450052,-28.14995));
#247839=CARTESIAN_POINT('',(-53.9354576832443,-25.5667682825966,-28.14995));
#247840=CARTESIAN_POINT('Ctrl Pts',(-45.8309904068109,-42.7275323570066,
-36.9730300997693));
#247841=CARTESIAN_POINT('Ctrl Pts',(-46.2060841796464,-41.8482165540222,
-36.9320687979064));
#247842=CARTESIAN_POINT('Ctrl Pts',(-46.4165725998998,-41.9354037124137,
-36.0027343734933));
#247843=CARTESIAN_POINT('Ctrl Pts',(-46.7534506368482,-43.1104816252375,
-37.2179244522577));
#247844=CARTESIAN_POINT('Ctrl Pts',(-47.1290415487049,-42.2305180137903,
-37.1777580130411));
#247845=CARTESIAN_POINT('Ctrl Pts',(-47.3394696831815,-42.3176802009835,
-36.2476287235887));
#247846=CARTESIAN_POINT('Ctrl Pts',(-47.6758891195153,-43.4933769026755,
-37.463031047121));
#247847=CARTESIAN_POINT('Ctrl Pts',(-48.0515862359126,-42.6126485351233,
-37.4235224076789));
#247848=CARTESIAN_POINT('Ctrl Pts',(-48.2623182897497,-42.6999366098412,
-36.4927353185438));
#247849=CARTESIAN_POINT('Ctrl Pts',(-48.5983086357822,-43.8762256986891,
-37.7083189393204));
#247850=CARTESIAN_POINT('Ctrl Pts',(-48.9738234376089,-42.9946516917827,
-37.6693623947416));
#247851=CARTESIAN_POINT('Ctrl Pts',(-49.1851254866488,-43.0821758662522,
-36.7380232130444));
#247852=CARTESIAN_POINT('',(-46.4165725996979,-41.9354037129011,-36.0027343734932));
#247853=CARTESIAN_POINT('Origin',(1674.91246247384,671.062426055257,-7635.73196693816));
#247854=CARTESIAN_POINT('',(-45.8309904070058,-42.727532356592,-36.9730300996838));
#247855=CARTESIAN_POINT('Origin',(1064.10886932915,2004.44184216393,-7418.93704427589));
#247856=CARTESIAN_POINT('Origin',(-46.0338891675347,-42.859283244925,-36.0027343734933));
#247857=CARTESIAN_POINT('Origin',(-46.0338891675347,-42.859283244925,-36.0027343734933));
#247858=CARTESIAN_POINT('',(-45.1951938513423,-42.314682320764,-36.0027343734933));
#247859=CARTESIAN_POINT('Origin',(-46.0338891675347,-42.8592832449249,-36.0027343734933));
#247860=CARTESIAN_POINT('Origin',(-46.0338891675347,-42.8592832449249,-36.0027343734933));
#247861=CARTESIAN_POINT('Origin',(-46.0338891675347,-42.8592832449249,-55.24995));
#247862=CARTESIAN_POINT('',(-45.1951938513423,-42.314682320764,-28.64995));
#247863=CARTESIAN_POINT('',(-46.4165725998998,-41.9354037124137,-28.64995));
#247864=CARTESIAN_POINT('Origin',(-46.0338891675347,-42.8592832449249,-28.64995));
#247865=CARTESIAN_POINT('',(-46.4165725998998,-41.9354037124137,-7.34233313511216E-15));
#247866=CARTESIAN_POINT('',(-45.1951938513423,-42.314682320764,-55.24995));
#247867=CARTESIAN_POINT('Ctrl Pts',(-46.5036191527319,-43.0538517754469,
-27.14995));
#247868=CARTESIAN_POINT('Ctrl Pts',(-46.886302585097,-42.1299722429357,
-27.1499500000001));
#247869=CARTESIAN_POINT('Ctrl Pts',(-46.886302585097,-42.1299722429356,
-28.14995));
#247870=CARTESIAN_POINT('Ctrl Pts',(-46.3336353463682,-42.9580702414852,
-27.14995));
#247871=CARTESIAN_POINT('Ctrl Pts',(-46.7093272072494,-42.0566666412253,
-27.1731316302543));
#247872=CARTESIAN_POINT('Ctrl Pts',(-46.8253261772413,-42.104714987817,
-28.149950041602));
#247873=CARTESIAN_POINT('Ctrl Pts',(-46.1640497973707,-42.8624134989651,
-27.1881541167863));
#247874=CARTESIAN_POINT('Ctrl Pts',(-46.5389139774209,-41.9860791702219,
-27.2322497625617));
#247875=CARTESIAN_POINT('Ctrl Pts',(-46.7644730427604,-42.0795087942021,
-28.1626847185045));
#247876=CARTESIAN_POINT('Ctrl Pts',(-45.9273486281662,-42.7287775839517,
-27.2996074426928));
#247877=CARTESIAN_POINT('Ctrl Pts',(-46.3089587420652,-41.8908285929994,
-27.3662354207734));
#247878=CARTESIAN_POINT('Ctrl Pts',(-46.6795127713057,-42.0443170975027,
-28.1998358077765));
#247879=CARTESIAN_POINT('Ctrl Pts',(-45.8524382410723,-42.6864641790425,
-27.3451208446555));
#247880=CARTESIAN_POINT('Ctrl Pts',(-46.2379326487285,-41.8614086218567,
-27.4172101718477));
#247881=CARTESIAN_POINT('Ctrl Pts',(-46.6526207729806,-42.0331780670771,
-28.2150069437025));
#247882=CARTESIAN_POINT('Ctrl Pts',(-45.7105338998473,-42.6062770391952,
-27.4527521127821));
#247883=CARTESIAN_POINT('Ctrl Pts',(-46.1056152152263,-41.8066009463618,
-27.5319438042374));
#247884=CARTESIAN_POINT('Ctrl Pts',(-46.6016724405327,-42.0120745767969,
-28.2508840421101));
#247885=CARTESIAN_POINT('Ctrl Pts',(-45.6430616909817,-42.5681325640035,
-27.515614264563));
#247886=CARTESIAN_POINT('Ctrl Pts',(-46.0437329340899,-41.7809684662446,
-27.5963774980067));
#247887=CARTESIAN_POINT('Ctrl Pts',(-46.5774442952742,-42.0020389504397,
-28.2718380908663));
#247888=CARTESIAN_POINT('Ctrl Pts',(-45.461192857402,-42.4652810208128,
-27.7222891160844));
#247889=CARTESIAN_POINT('Ctrl Pts',(-45.8798463955735,-41.7130844393005,
-27.8008611479946));
#247890=CARTESIAN_POINT('Ctrl Pts',(-46.5121314621695,-41.9749854891707,
-28.3407297000044));
#247891=CARTESIAN_POINT('Ctrl Pts',(-45.3628210526023,-42.4095997698276,
-27.889382888041));
#247892=CARTESIAN_POINT('Ctrl Pts',(-45.7931967067073,-41.6771929629972,
-27.958995177229));
#247893=CARTESIAN_POINT('Ctrl Pts',(-46.4767944547823,-41.9603484214572,
-28.3964276298892));
#247894=CARTESIAN_POINT('Ctrl Pts',(-45.2305230591413,-42.3346964000699,
-28.2517820805544));
#247895=CARTESIAN_POINT('Ctrl Pts',(-45.6784095350839,-41.6296465597236,
-28.2919200601672));
#247896=CARTESIAN_POINT('Ctrl Pts',(-46.4292667992664,-41.9406618219547,
-28.5172273596426));
#247897=CARTESIAN_POINT('Ctrl Pts',(-45.1951938541106,-42.3146823164992,
-28.4504081177447));
#247898=CARTESIAN_POINT('Ctrl Pts',(-45.648154654201,-41.6171145777345,
-28.4709599502677));
#247899=CARTESIAN_POINT('Ctrl Pts',(-46.4165726261775,-41.9354037232982,
-28.5834360396918));
#247900=CARTESIAN_POINT('Ctrl Pts',(-45.1951938513414,-42.3146823207637,
-28.6499499999994));
#247901=CARTESIAN_POINT('Ctrl Pts',(-45.6481545919442,-41.6171145519467,
-28.6499499999995));
#247902=CARTESIAN_POINT('Ctrl Pts',(-46.4165725998989,-41.9354037124133,
-28.64995));
#247903=CARTESIAN_POINT('',(-46.886302585097,-42.1299722429356,-28.14995));
#247904=CARTESIAN_POINT('Origin',(-46.5036191527319,-43.0538517754469,-28.14995));
#247905=CARTESIAN_POINT('Ctrl Pts',(-46.4165725998989,-41.9354037124133,
-28.64995));
#247906=CARTESIAN_POINT('Ctrl Pts',(-46.4165725998989,-41.9354037124133,
-28.6226248135972));
#247907=CARTESIAN_POINT('Ctrl Pts',(-46.4187109381147,-41.9362894411032,
-28.5954211970934));
#247908=CARTESIAN_POINT('Ctrl Pts',(-46.4228669716073,-41.9380109265415,
-28.5686411074116));
#247909=CARTESIAN_POINT('Ctrl Pts',(-46.4270499742658,-41.9397435829741,
-28.5416872374458));
#247910=CARTESIAN_POINT('Ctrl Pts',(-46.433277320163,-41.9423230341023,
-28.5151609373024));
#247911=CARTESIAN_POINT('Ctrl Pts',(-46.4414722606413,-41.9457174895913,
-28.489381232746));
#247912=CARTESIAN_POINT('Ctrl Pts',(-46.4427468468602,-41.9462454404895,
-28.4853716299623));
#247913=CARTESIAN_POINT('Ctrl Pts',(-46.4440691143792,-41.946793141629,
-28.4813801353776));
#247914=CARTESIAN_POINT('Ctrl Pts',(-46.4454388651654,-41.9473605109817,
-28.4774080096258));
#247915=CARTESIAN_POINT('Ctrl Pts',(-46.4478264096847,-41.9483494643023,
-28.4704843946408));
#247916=CARTESIAN_POINT('Ctrl Pts',(-46.45035857188,-41.9493983202258,-28.463618983549));
#247917=CARTESIAN_POINT('Ctrl Pts',(-46.4530306270243,-41.950505121706,
-28.4568274947659));
#247918=CARTESIAN_POINT('Ctrl Pts',(-46.456999039382,-41.9521488919256,
-28.446741090647));
#247919=CARTESIAN_POINT('Ctrl Pts',(-46.4612903227467,-41.9539263996952,
-28.4367870158134));
#247920=CARTESIAN_POINT('Ctrl Pts',(-46.4658757275553,-41.9558257365559,
-28.4270122638807));
#247921=CARTESIAN_POINT('Ctrl Pts',(-46.4765029911984,-41.9602276932878,
-28.4043580228328));
#247922=CARTESIAN_POINT('Ctrl Pts',(-46.4887247847145,-41.9652901259187,
-28.3826189531785));
#247923=CARTESIAN_POINT('Ctrl Pts',(-46.5023672130988,-41.9709410047792,
-28.3619996399708));
#247924=CARTESIAN_POINT('Ctrl Pts',(-46.5160732539531,-41.9766182327875,
-28.3412841821907));
#247925=CARTESIAN_POINT('Ctrl Pts',(-46.5312140385135,-41.9828897510974,
-28.3216976523455));
#247926=CARTESIAN_POINT('Ctrl Pts',(-46.5476531664069,-41.9896990608245,
-28.3034746152985));
#247927=CARTESIAN_POINT('Ctrl Pts',(-46.5502931718124,-41.9907925868682,
-28.3005481269458));
#247928=CARTESIAN_POINT('Ctrl Pts',(-46.5529667295821,-41.9919000107562,
-28.2976568837582));
#247929=CARTESIAN_POINT('Ctrl Pts',(-46.5556733480225,-41.9930211288223,
-28.2948019573763));
#247930=CARTESIAN_POINT('Ctrl Pts',(-46.5774801822152,-42.0020538152974,
-28.2718002275009));
#247931=CARTESIAN_POINT('Ctrl Pts',(-46.6017003997271,-42.0120861578744,
-28.2508643378562));
#247932=CARTESIAN_POINT('Ctrl Pts',(-46.6271465968548,-42.0226263178355,
-28.2329454764323));
#247933=CARTESIAN_POINT('Ctrl Pts',(-46.6526206528053,-42.0331780172989,
-28.2150069972093));
#247934=CARTESIAN_POINT('Ctrl Pts',(-46.679496989526,-42.0443105604755,
-28.1998426732967));
#247935=CARTESIAN_POINT('Ctrl Pts',(-46.7078328490258,-42.0560476577818,
-28.1874520771524));
#247936=CARTESIAN_POINT('Ctrl Pts',(-46.7371092175932,-42.0681743266994,
-28.1746502188044));
#247937=CARTESIAN_POINT('Ctrl Pts',(-46.7675446777706,-42.080781107082,
-28.1650444274588));
#247938=CARTESIAN_POINT('Ctrl Pts',(-46.7986350690308,-42.0936591688014,
-28.1587550972375));
#247939=CARTESIAN_POINT('Ctrl Pts',(-46.827431271788,-42.1055869465283,
-28.152929862465));
#247940=CARTESIAN_POINT('Ctrl Pts',(-46.8567902372224,-42.1177478281885,
-28.14995));
#247941=CARTESIAN_POINT('Ctrl Pts',(-46.886302585097,-42.1299722429356,
-28.14995));
#247942=CARTESIAN_POINT('Ctrl Pts',(-46.5036191527319,-43.0538517754469,
-27.14995));
#247943=CARTESIAN_POINT('Ctrl Pts',(-46.2744683037554,-42.9247311243421,
-27.14995));
#247944=CARTESIAN_POINT('Ctrl Pts',(-46.0777393610381,-42.8132290539286,
-27.2181464165627));
#247945=CARTESIAN_POINT('Ctrl Pts',(-45.8475944848875,-42.683304170092,
-27.3484057282222));
#247946=CARTESIAN_POINT('Ctrl Pts',(-45.7811408576611,-42.6458517787015,
-27.39666449696));
#247947=CARTESIAN_POINT('Ctrl Pts',(-45.6954623428615,-42.597586077303,
-27.4694662134751));
#247948=CARTESIAN_POINT('Ctrl Pts',(-45.6692215721777,-42.5828065424626,
-27.4938232175497));
#247949=CARTESIAN_POINT('Ctrl Pts',(-45.6330713242968,-42.5624303622357,
-27.5298221771973));
#247950=CARTESIAN_POINT('Ctrl Pts',(-45.6157982810954,-42.552690123496,
-27.5476894082045));
#247951=CARTESIAN_POINT('Ctrl Pts',(-45.5969866223692,-42.5420696469704,
-27.5681755773823));
#247952=CARTESIAN_POINT('Ctrl Pts',(-45.5879077094426,-42.536939971722,
-27.578314372819));
#247953=CARTESIAN_POINT('Ctrl Pts',(-45.5840859290262,-42.5347796725811,
-27.5826356936761));
#247954=CARTESIAN_POINT('Ctrl Pts',(-45.5815533520825,-42.533347884816,
-27.5855111018876));
#247955=CARTESIAN_POINT('Ctrl Pts',(-45.581048615305,-42.5330625581288,
-27.5860830286103));
#247956=CARTESIAN_POINT('Ctrl Pts',(-45.4507253194287,-42.4593606968009,
-27.7352703996687));
#247957=CARTESIAN_POINT('Ctrl Pts',(-45.3532470316574,-42.4040488934299,
-27.9086811930516));
#247958=CARTESIAN_POINT('Ctrl Pts',(-45.2255529238554,-42.3317558836558,
-28.2735063897175));
#247959=CARTESIAN_POINT('Ctrl Pts',(-45.1951938513423,-42.3146823207641,
-28.4647367626832));
#247960=CARTESIAN_POINT('Ctrl Pts',(-45.1951938513423,-42.314682320764,
-28.64995));
#247961=CARTESIAN_POINT('Origin',(3.82683432365091,-22.2062953451411,-28.14995));
#247962=CARTESIAN_POINT('',(8.02885449088512,-19.3833694022149,-28.14995));
#247963=CARTESIAN_POINT('Origin',(-65.4282127731639,-49.8102829151368,-43.9323406555977));
#247964=CARTESIAN_POINT('Ctrl Pts',(-49.5640573010081,-43.2391345629745,
-37.8286434305112));
#247965=CARTESIAN_POINT('Ctrl Pts',(-49.842046725293,-43.3542815527096,
-37.9027583562636));
#247966=CARTESIAN_POINT('Ctrl Pts',(-50.1228968347622,-43.4706134770457,
-37.9776546393184));
#247967=CARTESIAN_POINT('Origin',(-74.5160435483921,-43.8330558721564,-27.1488937903833));
#247968=CARTESIAN_POINT('Origin',(-58.8891135228643,-37.3601695173274,-20.9925312105213));
#247969=CARTESIAN_POINT('Origin',(8.02885449088512,-19.383369402215,-4.55788165120213E-15));
#247970=CARTESIAN_POINT('Origin',(1.1405527083135,-2.75353781701182,-1.76005755589152E-15));
#247971=CARTESIAN_POINT('Origin',(-55.5229609888525,-26.2243336820917,-41.2453393117887));
#247972=CARTESIAN_POINT('Origin',(-26.5085260991663,-68.3364732839715,-55.24995));
#247973=CARTESIAN_POINT('',(-26.299256677934,-65.343781133192,-39.1625636424987));
#247974=CARTESIAN_POINT('',(-26.299256677934,-65.343781133192,-52.64995));
#247975=CARTESIAN_POINT('',(-26.299256677934,-65.343781133192,-52.64995));
#247976=CARTESIAN_POINT('',(-25.2130575054386,-65.6305979870176,-52.64995));
#247977=CARTESIAN_POINT('Origin',(-26.5085260991663,-68.3364732839715,-52.64995));
#247978=CARTESIAN_POINT('',(-25.2130575054386,-65.6305979870176,-39.0779244525544));
#247979=CARTESIAN_POINT('',(-25.2130575054386,-65.6305979870176,-55.24995));
#247980=CARTESIAN_POINT('Ctrl Pts',(-26.299256677934,-65.343781133192,-39.1625636424987));
#247981=CARTESIAN_POINT('Ctrl Pts',(-26.2191817227488,-65.3493805195246,
-39.150717625587));
#247982=CARTESIAN_POINT('Ctrl Pts',(-26.1398068688508,-65.3581562279599,
-39.1400968863451));
#247983=CARTESIAN_POINT('Ctrl Pts',(-26.0611578132232,-65.3700172137199,
-39.1307129226473));
#247984=CARTESIAN_POINT('Ctrl Pts',(-25.9815936509173,-65.3820162058069,
-39.121219773559));
#247985=CARTESIAN_POINT('Ctrl Pts',(-25.902771422632,-65.3971727049329,
-39.1129923480007));
#247986=CARTESIAN_POINT('Ctrl Pts',(-25.8247155096153,-65.4154455405877,
-39.1060425498786));
#247987=CARTESIAN_POINT('Ctrl Pts',(-25.7467575651693,-65.4336954418673,
-39.0991014745011));
#247988=CARTESIAN_POINT('Ctrl Pts',(-25.6695631782055,-65.4550540670665,
-39.0934348214525));
#247989=CARTESIAN_POINT('Ctrl Pts',(-25.5931671353121,-65.4795312181795,
-39.0890544498735));
#247990=CARTESIAN_POINT('Ctrl Pts',(-25.5176849950404,-65.5037155565796,
-39.0847264793471));
#247991=CARTESIAN_POINT('Ctrl Pts',(-25.4429814678376,-65.5309446076645,
-39.0816541995771));
#247992=CARTESIAN_POINT('Ctrl Pts',(-25.3691120394327,-65.5612731829912,
-39.079849049173));
#247993=CARTESIAN_POINT('Ctrl Pts',(-25.3166630024623,-65.5828071870157,
-39.0785673497971));
#247994=CARTESIAN_POINT('Ctrl Pts',(-25.2646348944175,-65.6059047250466,
-39.0779244527868));
#247995=CARTESIAN_POINT('Ctrl Pts',(-25.2130575054386,-65.6305979870177,
-39.0779244525544));
#247996=CARTESIAN_POINT('Origin',(-55.3689732639433,13.5410260791383,-55.24995));
#247997=CARTESIAN_POINT('',(-52.3762811131638,13.3317566579059,-39.1625636424987));
#247998=CARTESIAN_POINT('',(-52.3762811131638,13.3317566579059,-52.64995));
#247999=CARTESIAN_POINT('',(-52.3762811131638,13.3317566579059,-52.64995));
#248000=CARTESIAN_POINT('',(-52.6630979669895,12.2455574854105,-52.64995));
#248001=CARTESIAN_POINT('Origin',(-55.3689732639433,13.5410260791383,-52.64995));
#248002=CARTESIAN_POINT('',(-52.6630979669895,12.2455574854105,-39.0779244525544));
#248003=CARTESIAN_POINT('',(-52.6630979669895,12.2455574854105,-55.24995));
#248004=CARTESIAN_POINT('Ctrl Pts',(-52.3762811131638,13.3317566579059,
-39.1625636424987));
#248005=CARTESIAN_POINT('Ctrl Pts',(-52.3818804994966,13.2516817027191,
-39.1507176255866));
#248006=CARTESIAN_POINT('Ctrl Pts',(-52.390656207932,13.1723068488195,-39.1400968863444));
#248007=CARTESIAN_POINT('Ctrl Pts',(-52.4025171936925,13.0936577931905,
-39.1307129226464));
#248008=CARTESIAN_POINT('Ctrl Pts',(-52.4145161857798,13.0140936308831,
-39.1212197735579));
#248009=CARTESIAN_POINT('Ctrl Pts',(-52.4296726849063,12.9352714025963,
-39.1129923479995));
#248010=CARTESIAN_POINT('Ctrl Pts',(-52.4479455205616,12.8572154895783,
-39.1060425498774));
#248011=CARTESIAN_POINT('Ctrl Pts',(-52.4661954218418,12.779257545131,-39.0991014744999));
#248012=CARTESIAN_POINT('Ctrl Pts',(-52.4875540470417,12.7020631581658,
-39.0934348214514));
#248013=CARTESIAN_POINT('Ctrl Pts',(-52.5120311981555,12.6256671152711,
-39.0890544498725));
#248014=CARTESIAN_POINT('Ctrl Pts',(-52.5362155365564,12.5501849749981,
-39.0847264793463));
#248015=CARTESIAN_POINT('Ctrl Pts',(-52.5634445876421,12.4754814477942,
-39.0816541995765));
#248016=CARTESIAN_POINT('Ctrl Pts',(-52.5937731629698,12.4016120193881,
-39.0798490491726));
#248017=CARTESIAN_POINT('Ctrl Pts',(-52.6153071669924,12.3491629824233,
-39.078567349797));
#248018=CARTESIAN_POINT('Ctrl Pts',(-52.638404705021,12.297134874384,-39.0779244527868));
#248019=CARTESIAN_POINT('Ctrl Pts',(-52.6630979669895,12.2455574854105,
-39.0779244525544));
#248020=CARTESIAN_POINT('Origin',(-26.5085260991666,42.4014732439151,-55.24995));
#248021=CARTESIAN_POINT('',(-25.2130575054389,39.6955979469612,-39.0779244525544));
#248022=CARTESIAN_POINT('',(-25.2130575054389,39.6955979469612,-52.64995));
#248023=CARTESIAN_POINT('',(-25.2130575054389,39.6955979469612,-55.24995));
#248024=CARTESIAN_POINT('',(-26.2992566779342,39.4087810931356,-52.64995));
#248025=CARTESIAN_POINT('Origin',(-26.5085260991666,42.4014732439151,-52.64995));
#248026=CARTESIAN_POINT('',(-26.2992566779342,39.4087810931356,-39.1625636424987));
#248027=CARTESIAN_POINT('',(-26.2992566779342,39.4087810931356,-37.9059960127943));
#248028=CARTESIAN_POINT('Ctrl Pts',(-25.2130575054389,39.6955979469613,
-39.0779244525544));
#248029=CARTESIAN_POINT('Ctrl Pts',(-25.2853758087053,39.6609747362246,
-39.0779244528815));
#248030=CARTESIAN_POINT('Ctrl Pts',(-25.358578777861,39.6294870816771,-39.0791883715014));
#248031=CARTESIAN_POINT('Ctrl Pts',(-25.4325893318994,39.6010518340479,
-39.0817049219424));
#248032=CARTESIAN_POINT('Ctrl Pts',(-25.5078024392622,39.5721545590496,
-39.0842623623096));
#248033=CARTESIAN_POINT('Ctrl Pts',(-25.5838503061877,39.5464092486697,
-39.0881134717398));
#248034=CARTESIAN_POINT('Ctrl Pts',(-25.6606832984686,39.5237723238568,
-39.0932464046122));
#248035=CARTESIAN_POINT('Ctrl Pts',(-25.737639668794,39.5010990487803,-39.0983875799231));
#248036=CARTESIAN_POINT('Ctrl Pts',(-25.8153845108865,39.4815438876141,
-39.1048146986732));
#248037=CARTESIAN_POINT('Ctrl Pts',(-25.893887314254,39.4651116919121,-39.112515858085));
#248038=CARTESIAN_POINT('Ctrl Pts',(-25.9717768804289,39.4488078589327,
-39.1201568586595));
#248039=CARTESIAN_POINT('Ctrl Pts',(-26.0504134462025,39.4355782885041,
-39.1290520728958));
#248040=CARTESIAN_POINT('Ctrl Pts',(-26.1297738690388,39.4254781585406,
-39.1391898747846));
#248041=CARTESIAN_POINT('Ctrl Pts',(-26.1859090101704,39.4183338893862,
-39.1463607909599));
#248042=CARTESIAN_POINT('Ctrl Pts',(-26.242406487351,39.4127564457215,-39.154153418384));
#248043=CARTESIAN_POINT('Ctrl Pts',(-26.2992566779342,39.4087810931356,
-39.1625636424987));
#248044=CARTESIAN_POINT('Ctrl Pts',(-25.2130575054389,39.6955979469612,
-39.0779244525544));
#248045=CARTESIAN_POINT('Ctrl Pts',(-25.2130575054388,39.6955979469612,
-37.9059960127943));
#248046=CARTESIAN_POINT('Ctrl Pts',(-24.7220243175171,38.669965539032,-37.6224808631404));
#248047=CARTESIAN_POINT('Ctrl Pts',(-25.5571787362036,39.5308459913215,
-39.077924454111));
#248048=CARTESIAN_POINT('Ctrl Pts',(-25.5933889787397,39.5135099307705,
-37.9059960140155));
#248049=CARTESIAN_POINT('Ctrl Pts',(-25.2415430286799,38.4212400498976,
-37.6224808645859));
#248050=CARTESIAN_POINT('Ctrl Pts',(-25.9205756959913,39.4352610469465,
-39.1065428641433));
#248051=CARTESIAN_POINT('Ctrl Pts',(-26.0004074167487,39.4148955857669,
-37.9286345805798));
#248052=CARTESIAN_POINT('Ctrl Pts',(-25.7896847017763,38.2763141299578,
-37.6510924855219));
#248053=CARTESIAN_POINT('Ctrl Pts',(-26.2992566779342,39.4087810931356,
-39.1625636424987));
#248054=CARTESIAN_POINT('Ctrl Pts',(-26.4161222952889,39.4006090530882,
-37.971813107807));
#248055=CARTESIAN_POINT('Ctrl Pts',(-26.3607251006129,38.2350705817238,
-37.7071200530847));
#248056=CARTESIAN_POINT('',(-24.7220243175171,38.669965539032,-37.6224808631404));
#248057=CARTESIAN_POINT('Origin',(-24.5653232085749,38.3426602984844,-39.0779244525544));
#248058=CARTESIAN_POINT('',(-26.3607251006129,38.2350705817238,-37.7071200530847));
#248059=CARTESIAN_POINT('Origin',(-26.194621967318,37.9124350177459,-39.1625636424987));
#248060=CARTESIAN_POINT('Ctrl Pts',(-26.3607251006129,38.2350705817238,
-37.7071200530847));
#248061=CARTESIAN_POINT('Ctrl Pts',(-26.2011255350992,38.2465977037834,
-37.6914609588104));
#248062=CARTESIAN_POINT('Ctrl Pts',(-26.0435569434565,38.2662022062977,
-37.6779662189505));
#248063=CARTESIAN_POINT('Ctrl Pts',(-25.8880107550447,38.2938462174384,
-37.6666367941389));
#248064=CARTESIAN_POINT('Ctrl Pts',(-25.7326779997653,38.3214522967729,
-37.6553229150289));
#248065=CARTESIAN_POINT('Ctrl Pts',(-25.5793619804298,38.3570758581462,
-37.6461683926629));
#248066=CARTESIAN_POINT('Ctrl Pts',(-25.4280646493686,38.4007283517996,
-37.6391871086171));
#248067=CARTESIAN_POINT('Ctrl Pts',(-25.2772986540836,38.4442275437957,
-37.6322303418973));
#248068=CARTESIAN_POINT('Ctrl Pts',(-25.1285370763277,38.4956993999497,
-37.6274315578454));
#248069=CARTESIAN_POINT('Ctrl Pts',(-24.9817940407081,38.5552037278875,
-37.624817614644));
#248070=CARTESIAN_POINT('Ctrl Pts',(-24.8944876056226,38.5906065033751,
-37.6232624194589));
#248071=CARTESIAN_POINT('Ctrl Pts',(-24.8078959327013,38.6288535270284,
-37.6224808633793));
#248072=CARTESIAN_POINT('Ctrl Pts',(-24.7220243175172,38.669965539032,-37.6224808631404));
#248073=CARTESIAN_POINT('Origin',(-48.2118204350716,29.879557875893,235.35105));
#248074=CARTESIAN_POINT('',(-50.4542306878656,31.8724442896568,-41.3499258784557));
#248075=CARTESIAN_POINT('',(-50.4542306878656,31.8724442896568,-52.64995));
#248076=CARTESIAN_POINT('',(-50.4542306878656,31.8724442896567,235.35105));
#248077=CARTESIAN_POINT('',(-51.2045125858511,30.0888272971254,-52.64995));
#248078=CARTESIAN_POINT('Origin',(-48.2118204350716,29.879557875893,-52.64995));
#248079=CARTESIAN_POINT('',(-51.2045125858511,30.0888272971254,-41.2737227474219));
#248080=CARTESIAN_POINT('',(-51.2045125858511,30.0888272971253,235.35105));
#248081=CARTESIAN_POINT('Ctrl Pts',(-50.4542306878656,31.8724442896568,
-41.3499258784557));
#248082=CARTESIAN_POINT('Ctrl Pts',(-50.6751042513768,31.6239157533749,
-41.3499258753262));
#248083=CARTESIAN_POINT('Ctrl Pts',(-50.8500106529935,31.3458145441506,
-41.3433504080566));
#248084=CARTESIAN_POINT('Ctrl Pts',(-51.1065500370229,30.7342489164072,
-41.3171858838447));
#248085=CARTESIAN_POINT('Ctrl Pts',(-51.1815637992349,30.4170102355187,
-41.298307134608));
#248086=CARTESIAN_POINT('Ctrl Pts',(-51.2045125858511,30.0888272971254,
-41.2737227474219));
#248087=CARTESIAN_POINT('Origin',(-42.8470578959213,35.2443204150433,235.35105));
#248088=CARTESIAN_POINT('',(-43.0563273171537,38.2370125658228,-41.2737227474219));
#248089=CARTESIAN_POINT('',(-43.0563273171537,38.2370125658228,-52.64995));
#248090=CARTESIAN_POINT('',(-43.0563273171537,38.2370125658227,235.35105));
#248091=CARTESIAN_POINT('',(-44.839944309685,37.4867306678373,-52.64995));
#248092=CARTESIAN_POINT('Origin',(-42.8470578959213,35.2443204150433,-52.64995));
#248093=CARTESIAN_POINT('',(-44.839944309685,37.4867306678373,-41.3499258784557));
#248094=CARTESIAN_POINT('',(-44.839944309685,37.4867306678373,235.35105));
#248095=CARTESIAN_POINT('Ctrl Pts',(-43.0563273171537,38.2370125658228,
-41.2737227474219));
#248096=CARTESIAN_POINT('Ctrl Pts',(-43.3844623716888,38.2140671259236,
-41.2983034469791));
#248097=CARTESIAN_POINT('Ctrl Pts',(-43.7019124525045,38.1390166933963,
-41.3171960016465));
#248098=CARTESIAN_POINT('Ctrl Pts',(-44.3136937257824,37.8823162829827,
-41.3433633063114));
#248099=CARTESIAN_POINT('Ctrl Pts',(-44.5912415362924,37.707759080253,-41.3499257769023));
#248100=CARTESIAN_POINT('Ctrl Pts',(-44.839944309685,37.4867306678373,-41.3499258784558));
#248101=CARTESIAN_POINT('Origin',(-44.0630480057168,38.1666157975539,235.35105));
#248102=CARTESIAN_POINT('',(-44.0630480057168,38.166615797554,-52.64995));
#248103=CARTESIAN_POINT('Ctrl Pts',(-26.2992566779342,39.4087810931356,
-39.1625636424987));
#248104=CARTESIAN_POINT('Ctrl Pts',(-31.903874175502,39.0168680593679,-39.7153157040946));
#248105=CARTESIAN_POINT('Ctrl Pts',(-37.4870209577723,38.6264564042711,
-40.4393222961257));
#248106=CARTESIAN_POINT('Ctrl Pts',(-43.0563273171537,38.2370125658228,
-41.2737227474219));
#248107=CARTESIAN_POINT('Ctrl Pts',(-44.0845625322695,36.6367696109743,
-39.8944822890418));
#248108=CARTESIAN_POINT('Ctrl Pts',(-44.8399443096851,37.4867306678373,
-40.1779974386957));
#248109=CARTESIAN_POINT('Ctrl Pts',(-44.839944309685,37.4867306678373,-41.3499258784558));
#248110=CARTESIAN_POINT('Ctrl Pts',(-43.9595274298496,36.7478914351849,
-39.8944822858058));
#248111=CARTESIAN_POINT('Ctrl Pts',(-44.6149072014685,37.6867267800097,
-40.1779974336417));
#248112=CARTESIAN_POINT('Ctrl Pts',(-44.5912415343056,37.7077590820187,
-41.3499258752894));
#248113=CARTESIAN_POINT('Ctrl Pts',(-43.8200866324971,36.835758129222,-39.887919815423));
#248114=CARTESIAN_POINT('Ctrl Pts',(-44.3663746862182,37.849051706332,-40.1674920635188));
#248115=CARTESIAN_POINT('Ctrl Pts',(-44.3136937213669,37.8823162857708,
-41.343363404867));
#248116=CARTESIAN_POINT('Ctrl Pts',(-43.5128927223798,36.9652495181622,
-39.8617525114841));
#248117=CARTESIAN_POINT('Ctrl Pts',(-43.8196015906779,38.1008702319186,
-40.1253788430241));
#248118=CARTESIAN_POINT('Ctrl Pts',(-43.7019124427066,38.1390166965721,
-41.3171961008681));
#248119=CARTESIAN_POINT('Ctrl Pts',(-43.3535628849498,37.0032968338361,
-39.8428593266731));
#248120=CARTESIAN_POINT('Ctrl Pts',(-43.5344232858197,38.1836802846001,
-40.0946545134465));
#248121=CARTESIAN_POINT('Ctrl Pts',(-43.3844623592655,38.214067128441,-41.2983035466937));
#248122=CARTESIAN_POINT('Ctrl Pts',(-43.1889493654704,37.0152446912691,
-39.8182791580079));
#248123=CARTESIAN_POINT('Ctrl Pts',(-43.23812030497,38.224300361751,-40.0543903140502));
#248124=CARTESIAN_POINT('Ctrl Pts',(-43.0563273171537,38.2370125658228,
-41.2737227474219));
#248125=CARTESIAN_POINT('',(-43.1889493654704,37.0152446912691,-39.8182791580079));
#248126=CARTESIAN_POINT('Origin',(-42.9516926065375,36.740666490433,-41.2737227474219));
#248127=CARTESIAN_POINT('',(-44.0845625322695,36.6367696109743,-39.8944822890418));
#248128=CARTESIAN_POINT('Origin',(-43.8435011028032,36.3655255414403,-41.3499258784558));
#248129=CARTESIAN_POINT('Ctrl Pts',(-44.0845625322695,36.6367696109743,
-39.8944822890418));
#248130=CARTESIAN_POINT('Ctrl Pts',(-43.9941797939522,36.7170950246701,
-39.8944822890418));
#248131=CARTESIAN_POINT('Ctrl Pts',(-43.8962901478109,36.7852564677648,
-39.8910542505833));
#248132=CARTESIAN_POINT('Ctrl Pts',(-43.7909432593834,36.8413335920192,
-39.8842118316082));
#248133=CARTESIAN_POINT('Ctrl Pts',(-43.7506303648289,36.8627925191003,
-39.8815934560799));
#248134=CARTESIAN_POINT('Ctrl Pts',(-43.7092251907661,36.8824814307078,
-39.8784749689682));
#248135=CARTESIAN_POINT('Ctrl Pts',(-43.6667294913925,36.9004031219782,
-39.8748566639276));
#248136=CARTESIAN_POINT('Ctrl Pts',(-43.6666496039709,36.9004368128629,
-39.8748498618967));
#248137=CARTESIAN_POINT('Ctrl Pts',(-43.666569712705,36.9004704974974,-39.8748430581001));
#248138=CARTESIAN_POINT('Ctrl Pts',(-43.6664898175948,36.9005041758817,
-39.8748362525378));
#248139=CARTESIAN_POINT('Ctrl Pts',(-43.5643771770594,36.9435479709187,
-39.8661381741221));
#248140=CARTESIAN_POINT('Ctrl Pts',(-43.4597085659162,36.9748052400737,
-39.8548713027025));
#248141=CARTESIAN_POINT('Ctrl Pts',(-43.3525514979881,36.9944348238143,
-39.8410580051272));
#248142=CARTESIAN_POINT('Ctrl Pts',(-43.2986448352414,37.0043097240054,
-39.8341090582383));
#248143=CARTESIAN_POINT('Ctrl Pts',(-43.2441082468331,37.0112411932519,
-39.8265155089205));
#248144=CARTESIAN_POINT('Ctrl Pts',(-43.1889493654704,37.0152446912691,
-39.8182791580079));
#248145=CARTESIAN_POINT('Origin',(0.,-12.9675000200282,235.35105));
#248146=CARTESIAN_POINT('Origin',(0.,-12.9675000200281,-52.64995));
#248147=CARTESIAN_POINT('Origin',(0.,-12.9675000200281,-41.3499258784557));
#248148=CARTESIAN_POINT('Ctrl Pts',(-49.9827447112974,30.221449345442,-39.8182791580079));
#248149=CARTESIAN_POINT('Ctrl Pts',(-51.1918003817794,30.2706202849417,
-40.0543903140502));
#248150=CARTESIAN_POINT('Ctrl Pts',(-51.204512585851,30.0888272971254,-41.2737227474219));
#248151=CARTESIAN_POINT('Ctrl Pts',(-49.970795119399,30.3860867600489,-39.8428628946809));
#248152=CARTESIAN_POINT('Ctrl Pts',(-51.1511744833359,30.5669657276558,
-40.0946602834914));
#248153=CARTESIAN_POINT('Ctrl Pts',(-51.1815637992349,30.4170102355187,
-41.298307134608));
#248154=CARTESIAN_POINT('Ctrl Pts',(-49.9327664722994,30.5453106517579,
-39.8617422945218));
#248155=CARTESIAN_POINT('Ctrl Pts',(-51.0684082345096,30.8519555741622,
-40.125362313696));
#248156=CARTESIAN_POINT('Ctrl Pts',(-51.1065500370229,30.7342489164072,
-41.3171858838447));
#248157=CARTESIAN_POINT('Ctrl Pts',(-49.8033560611762,30.8523961753476,
-39.8879068185516));
#248158=CARTESIAN_POINT('Ctrl Pts',(-50.8167365053657,31.3985364985707,
-40.1674712617341));
#248159=CARTESIAN_POINT('Ctrl Pts',(-50.8500106529935,31.3458145441506,
-41.3433504080566));
#248160=CARTESIAN_POINT('Ctrl Pts',(-49.715313604986,30.9921150076825,-39.8944822858423));
#248161=CARTESIAN_POINT('Ctrl Pts',(-50.6540845266555,31.647567268839,-40.1779974337035));
#248162=CARTESIAN_POINT('Ctrl Pts',(-50.6751042513768,31.6239157533749,
-41.3499258753262));
#248163=CARTESIAN_POINT('Ctrl Pts',(-49.6042696310026,31.1170625122411,
-39.8944822890418));
#248164=CARTESIAN_POINT('Ctrl Pts',(-50.4542306878656,31.8724442896567,
-40.1779974386957));
#248165=CARTESIAN_POINT('Ctrl Pts',(-50.4542306878656,31.8724442896568,
-41.3499258784558));
#248166=CARTESIAN_POINT('',(-49.6042696310026,31.1170625122412,-39.8944822890418));
#248167=CARTESIAN_POINT('Origin',(-49.3330255614686,30.8760010827748,-41.3499258784557));
#248168=CARTESIAN_POINT('',(-49.9827447112974,30.221449345442,-39.8182791580079));
#248169=CARTESIAN_POINT('Origin',(-49.7081665104613,29.9841925865092,-41.2737227474219));
#248170=CARTESIAN_POINT('Ctrl Pts',(-49.9827447112974,30.221449345442,-39.8182791580079));
#248171=CARTESIAN_POINT('Ctrl Pts',(-49.974247842649,30.3385164122215,-39.8357596691873));
#248172=CARTESIAN_POINT('Ctrl Pts',(-49.9525777122483,30.4527365881441,
-39.8503404873507));
#248173=CARTESIAN_POINT('Ctrl Pts',(-49.9175649839551,30.5640807882622,
-39.8620074889827));
#248174=CARTESIAN_POINT('Ctrl Pts',(-49.903287657114,30.6094842062316,-39.8667650044257));
#248175=CARTESIAN_POINT('Ctrl Pts',(-49.8867911421682,30.6544092836455,
-39.871037881299));
#248176=CARTESIAN_POINT('Ctrl Pts',(-49.8680615705257,30.6988535344112,
-39.8748246333721));
#248177=CARTESIAN_POINT('Ctrl Pts',(-49.8680277409604,30.6989338101224,
-39.8748314730468));
#248178=CARTESIAN_POINT('Ctrl Pts',(-49.8679939050224,30.699014082039,-39.8748383109414));
#248179=CARTESIAN_POINT('Ctrl Pts',(-49.8679600627116,30.6990943501611,
-39.8748451470561));
#248180=CARTESIAN_POINT('Ctrl Pts',(-49.8342106733128,30.7791420788837,
-39.8816624916982));
#248181=CARTESIAN_POINT('Ctrl Pts',(-49.7941455915935,30.8553753559231,
-39.8867070324262));
#248182=CARTESIAN_POINT('Ctrl Pts',(-49.747789476607,30.9277322498084,-39.889976576145));
#248183=CARTESIAN_POINT('Ctrl Pts',(-49.7052516615012,30.9941291895568,
-39.8929768113077));
#248184=CARTESIAN_POINT('Ctrl Pts',(-49.6574159846451,31.0572618495022,
-39.8944822890418));
#248185=CARTESIAN_POINT('Ctrl Pts',(-49.6042696310026,31.1170625122411,
-39.8944822890418));
#248186=CARTESIAN_POINT('Origin',(-51.1341158175823,31.0955479856884,235.35105));
#248187=CARTESIAN_POINT('',(-51.1341158175823,31.0955479856884,-52.64995));
#248188=CARTESIAN_POINT('Ctrl Pts',(-51.2045125858511,30.0888272971254,
-41.2737227474219));
#248189=CARTESIAN_POINT('Ctrl Pts',(-51.5939564242993,24.519520937744,-40.4393222961257));
#248190=CARTESIAN_POINT('Ctrl Pts',(-51.9843680793961,18.9363741554737,
-39.7153157040947));
#248191=CARTESIAN_POINT('Ctrl Pts',(-52.3762811131638,13.3317566579059,
-39.1625636424987));
#248192=CARTESIAN_POINT('Ctrl Pts',(-52.3762811131638,13.3317566579059,
-39.1625636424987));
#248193=CARTESIAN_POINT('Ctrl Pts',(-52.3681090731164,13.4486222752606,
-37.971813107807));
#248194=CARTESIAN_POINT('Ctrl Pts',(-51.202570601752,13.3932250805846,-37.7071200530847));
#248195=CARTESIAN_POINT('Ctrl Pts',(-52.4027610669746,12.9530756759645,
-39.1065428641427));
#248196=CARTESIAN_POINT('Ctrl Pts',(-52.3823956057955,13.0329073967221,
-37.9286345805849));
#248197=CARTESIAN_POINT('Ctrl Pts',(-51.243814149994,12.8221846817494,-37.6510924855238));
#248198=CARTESIAN_POINT('Ctrl Pts',(-52.4983460113501,12.5896787161743,
-39.0779244541051));
#248199=CARTESIAN_POINT('Ctrl Pts',(-52.4810099507979,12.6258889587099,
-37.9059960140017));
#248200=CARTESIAN_POINT('Ctrl Pts',(-51.3887400699185,12.2740430086498,
-37.6224808645841));
#248201=CARTESIAN_POINT('Ctrl Pts',(-52.6630979669895,12.2455574854105,
-39.0779244525544));
#248202=CARTESIAN_POINT('Ctrl Pts',(-52.6630979669895,12.2455574854105,
-37.9059960127943));
#248203=CARTESIAN_POINT('Ctrl Pts',(-51.6374655590603,11.7545242974889,
-37.6224808631404));
#248204=CARTESIAN_POINT('',(-51.202570601752,13.3932250805846,-37.7071200530847));
#248205=CARTESIAN_POINT('Origin',(-50.8799350377741,13.2271219472897,-39.1625636424987));
#248206=CARTESIAN_POINT('',(-51.6374655590603,11.7545242974889,-37.6224808631404));
#248207=CARTESIAN_POINT('Origin',(-51.3101603185126,11.5978231885467,-39.0779244525544));
#248208=CARTESIAN_POINT('Ctrl Pts',(-51.6374655590603,11.7545242974889,
-37.6224808631404));
#248209=CARTESIAN_POINT('Ctrl Pts',(-51.5683401737289,11.898908096752,-37.6224808635416));
#248210=CARTESIAN_POINT('Ctrl Pts',(-51.5073117137531,12.0453267862122,
-37.6246896514879));
#248211=CARTESIAN_POINT('Ctrl Pts',(-51.4542914421326,12.1937580895559,
-37.6290723471549));
#248212=CARTESIAN_POINT('Ctrl Pts',(-51.401143473863,12.3425468822047,-37.6334655983234));
#248213=CARTESIAN_POINT('Ctrl Pts',(-51.3560423053795,12.4933581163811,
-37.6400432640145));
#248214=CARTESIAN_POINT('Ctrl Pts',(-51.3189474852191,12.6461827680856,
-37.6487836824747));
#248215=CARTESIAN_POINT('Ctrl Pts',(-51.281768224475,12.7993553013203,-37.6575439971369));
#248216=CARTESIAN_POINT('Ctrl Pts',(-51.2526317828013,12.9545505495527,
-37.6684769421211));
#248217=CARTESIAN_POINT('Ctrl Pts',(-51.2315467536768,13.1117710662236,
-37.6815739017301));
#248218=CARTESIAN_POINT('Ctrl Pts',(-51.2190600923228,13.2048778548359,
-37.6893299877397));
#248219=CARTESIAN_POINT('Ctrl Pts',(-51.2093980530995,13.2986951308913,
-37.6978452571967));
#248220=CARTESIAN_POINT('Ctrl Pts',(-51.202570601752,13.3932250805846,-37.7071200530847));
#248221=CARTESIAN_POINT('Origin',(-42.8470578959211,-61.1793204550998,235.35105));
#248222=CARTESIAN_POINT('',(-44.8399443096849,-63.4217307078938,-41.3499258784557));
#248223=CARTESIAN_POINT('',(-44.8399443096849,-63.4217307078937,-52.64995));
#248224=CARTESIAN_POINT('',(-44.8399443096849,-63.4217307078938,235.35105));
#248225=CARTESIAN_POINT('',(-43.0563273171535,-64.1720126058792,-52.64995));
#248226=CARTESIAN_POINT('Origin',(-42.8470578959211,-61.1793204550997,-52.64995));
#248227=CARTESIAN_POINT('',(-43.0563273171535,-64.1720126058792,-41.273722747422));
#248228=CARTESIAN_POINT('',(-43.0563273171535,-64.1720126058792,235.35105));
#248229=CARTESIAN_POINT('Ctrl Pts',(-44.8399443096849,-63.4217307078938,
-41.3499258784557));
#248230=CARTESIAN_POINT('Ctrl Pts',(-44.5914157734028,-63.6426042714052,
-41.3499258753244));
#248231=CARTESIAN_POINT('Ctrl Pts',(-44.3133145641792,-63.8175106730215,
-41.3433504080572));
#248232=CARTESIAN_POINT('Ctrl Pts',(-43.7017489364349,-64.0740500570513,
-41.3171858838442));
#248233=CARTESIAN_POINT('Ctrl Pts',(-43.3845102555472,-64.1490638192631,
-41.2983071346081));
#248234=CARTESIAN_POINT('Ctrl Pts',(-43.0563273171535,-64.1720126058792,
-41.273722747422));
#248235=CARTESIAN_POINT('Origin',(-48.2118204350714,-55.8145579159494,235.35105));
#248236=CARTESIAN_POINT('',(-51.2045125858509,-56.0238273371818,-41.2737227474219));
#248237=CARTESIAN_POINT('',(-51.2045125858509,-56.0238273371818,-52.64995));
#248238=CARTESIAN_POINT('',(-51.2045125858509,-56.0238273371818,235.35105));
#248239=CARTESIAN_POINT('',(-50.4542306878654,-57.8074443297132,-52.64995));
#248240=CARTESIAN_POINT('Origin',(-48.2118204350714,-55.8145579159494,-52.64995));
#248241=CARTESIAN_POINT('',(-50.4542306878654,-57.8074443297132,-41.3499258784557));
#248242=CARTESIAN_POINT('',(-50.4542306878654,-57.8074443297133,235.35105));
#248243=CARTESIAN_POINT('Ctrl Pts',(-51.2045125858509,-56.0238273371818,
-41.2737227474219));
#248244=CARTESIAN_POINT('Ctrl Pts',(-51.1815671459517,-56.3519623917163,
-41.2983034469768));
#248245=CARTESIAN_POINT('Ctrl Pts',(-51.106516713424,-56.6694124725336,
-41.317196001646));
#248246=CARTESIAN_POINT('Ctrl Pts',(-50.8498163030113,-57.2811937458096,
-41.343363306312));
#248247=CARTESIAN_POINT('Ctrl Pts',(-50.6752591002806,-57.5587415563211,
-41.3499257769023));
#248248=CARTESIAN_POINT('Ctrl Pts',(-50.4542306878654,-57.8074443297132,
-41.3499258784557));
#248249=CARTESIAN_POINT('Origin',(-51.1341158175821,-57.030548025745,235.35105));
#248250=CARTESIAN_POINT('Ctrl Pts',(-52.1363779740716,-42.6975314240561,
-39.5221562118214));
#248251=CARTESIAN_POINT('Ctrl Pts',(-51.8249654425107,-47.1509381060673,
-40.0158159854806));
#248252=CARTESIAN_POINT('Ctrl Pts',(-51.5144316274106,-51.5917785572367,
-40.6097076503739));
#248253=CARTESIAN_POINT('Ctrl Pts',(-51.2045125858509,-56.0238273371818,
-41.2737227474219));
#248254=CARTESIAN_POINT('',(-52.3762811131638,-39.2667566979623,-52.64995));
#248255=CARTESIAN_POINT('',(-52.3762811131638,-39.2667566979623,-37.9059960127943));
#248256=CARTESIAN_POINT('',(-51.1341158175821,-57.0305480257449,-52.64995));
#248257=CARTESIAN_POINT('Ctrl Pts',(-49.6042696310024,-57.0520625522976,
-39.8944822890418));
#248258=CARTESIAN_POINT('Ctrl Pts',(-50.4542306878655,-57.8074443297132,
-40.1779974386957));
#248259=CARTESIAN_POINT('Ctrl Pts',(-50.4542306878654,-57.8074443297132,
-41.3499258784558));
#248260=CARTESIAN_POINT('Ctrl Pts',(-49.7153914552119,-56.9270274498771,
-39.8944822858055));
#248261=CARTESIAN_POINT('Ctrl Pts',(-50.6542268000352,-57.5824072214955,
-40.177997433644));
#248262=CARTESIAN_POINT('Ctrl Pts',(-50.6752591020463,-57.5587415543343,
-41.3499258752894));
#248263=CARTESIAN_POINT('Ctrl Pts',(-49.8032581492502,-56.7875866525247,
-39.887919815423));
#248264=CARTESIAN_POINT('Ctrl Pts',(-50.8165517263607,-57.3338747062451,
-40.1674920635201));
#248265=CARTESIAN_POINT('Ctrl Pts',(-50.8498163057994,-57.2811937413941,
-41.3433634048676));
#248266=CARTESIAN_POINT('Ctrl Pts',(-49.9327495381902,-56.4803927424085,
-39.8617525114842));
#248267=CARTESIAN_POINT('Ctrl Pts',(-51.0683702519462,-56.7871016107072,
-40.125378843023));
#248268=CARTESIAN_POINT('Ctrl Pts',(-51.1065167165998,-56.6694124627357,
-41.3171961008675));
#248269=CARTESIAN_POINT('Ctrl Pts',(-49.9707968538638,-56.3210629049775,
-39.8428593266729));
#248270=CARTESIAN_POINT('Ctrl Pts',(-51.1511803046297,-56.5019233058474,
-40.094654513445));
#248271=CARTESIAN_POINT('Ctrl Pts',(-51.1815671484691,-56.351962379293,
-41.2983035466914));
#248272=CARTESIAN_POINT('Ctrl Pts',(-49.9827447112972,-56.1564493854985,
-39.8182791580079));
#248273=CARTESIAN_POINT('Ctrl Pts',(-51.1918003817792,-56.2056203249981,
-40.0543903140502));
#248274=CARTESIAN_POINT('Ctrl Pts',(-51.2045125858509,-56.0238273371818,
-41.2737227474219));
#248275=CARTESIAN_POINT('',(-49.9827447112972,-56.1564493854985,-39.8182791580079));
#248276=CARTESIAN_POINT('Origin',(-49.7081665104611,-55.9191926265656,-41.2737227474219));
#248277=CARTESIAN_POINT('',(-49.6042696310024,-57.0520625522976,-39.8944822890418));
#248278=CARTESIAN_POINT('Origin',(-49.3330255614684,-56.8110011228313,-41.3499258784558));
#248279=CARTESIAN_POINT('Ctrl Pts',(-49.6042696310024,-57.0520625522976,
-39.8944822890418));
#248280=CARTESIAN_POINT('Ctrl Pts',(-49.6845950444292,-56.9616798142831,
-39.8944822890418));
#248281=CARTESIAN_POINT('Ctrl Pts',(-49.7527564873363,-56.8637901684946,
-39.8910542506063));
#248282=CARTESIAN_POINT('Ctrl Pts',(-49.8088336114838,-56.75844328047,-39.884211831677));
#248283=CARTESIAN_POINT('Ctrl Pts',(-49.8302925387837,-56.7181303855818,
-39.8815934561345));
#248284=CARTESIAN_POINT('Ctrl Pts',(-49.8499814505791,-56.6767252111662,
-39.8784749689999));
#248285=CARTESIAN_POINT('Ctrl Pts',(-49.8679031420063,-56.6342295114207,
-39.8748566639276));
#248286=CARTESIAN_POINT('Ctrl Pts',(-49.867936832891,-56.6341496239991,
-39.8748498618967));
#248287=CARTESIAN_POINT('Ctrl Pts',(-49.8679705175255,-56.6340697327332,
-39.8748430581001));
#248288=CARTESIAN_POINT('Ctrl Pts',(-49.8680041959098,-56.6339898376229,
-39.8748362525379));
#248289=CARTESIAN_POINT('Ctrl Pts',(-49.9110479907906,-56.531877197458,
-39.8661381741537));
#248290=CARTESIAN_POINT('Ctrl Pts',(-49.9423052598749,-56.4272085867039,
-39.8548713027842));
#248291=CARTESIAN_POINT('Ctrl Pts',(-49.9619348436287,-56.3200515191826,
-39.8410580052776));
#248292=CARTESIAN_POINT('Ctrl Pts',(-49.9718097439335,-56.2661448560562,
-39.8341090583478));
#248293=CARTESIAN_POINT('Ctrl Pts',(-49.9787412132511,-56.2116082672591,
-39.8265155089799));
#248294=CARTESIAN_POINT('Ctrl Pts',(-49.9827447112972,-56.1564493854985,
-39.8182791580079));
#248295=CARTESIAN_POINT('Origin',(0.,-12.9675000200282,235.35105));
#248296=CARTESIAN_POINT('Origin',(0.,-12.9675000200281,-52.64995));
#248297=CARTESIAN_POINT('Origin',(0.,-12.9675000200281,-41.3499258784557));
#248298=CARTESIAN_POINT('Ctrl Pts',(-43.1889493654702,-62.9502447313255,
-39.8182791580079));
#248299=CARTESIAN_POINT('Ctrl Pts',(-43.2381203049698,-64.1593004018075,
-40.0543903140503));
#248300=CARTESIAN_POINT('Ctrl Pts',(-43.0563273171535,-64.1720126058792,
-41.2737227474219));
#248301=CARTESIAN_POINT('Ctrl Pts',(-43.3535867800773,-62.9382951394238,
-39.8428628946803));
#248302=CARTESIAN_POINT('Ctrl Pts',(-43.5344657476846,-64.1186745033647,
-40.0946602834885));
#248303=CARTESIAN_POINT('Ctrl Pts',(-43.3845102555472,-64.1490638192631,
-41.2983071346081));
#248304=CARTESIAN_POINT('Ctrl Pts',(-43.5128106717856,-62.900266492328,
-39.8617422945218));
#248305=CARTESIAN_POINT('Ctrl Pts',(-43.8194555941901,-64.0359082545366,
-40.1253623136954));
#248306=CARTESIAN_POINT('Ctrl Pts',(-43.7017489364349,-64.0740500570513,
-41.3171858838442));
#248307=CARTESIAN_POINT('Ctrl Pts',(-43.8198961953762,-62.7708560812039,
-39.8879068185516));
#248308=CARTESIAN_POINT('Ctrl Pts',(-44.3660365185992,-63.784236525395,
-40.1674712617347));
#248309=CARTESIAN_POINT('Ctrl Pts',(-44.3133145641792,-63.8175106730215,
-41.3433504080572));
#248310=CARTESIAN_POINT('Ctrl Pts',(-43.9596150277081,-62.6828136250119,
-39.8944822858415));
#248311=CARTESIAN_POINT('Ctrl Pts',(-44.6150672888654,-63.6215845466811,
-40.1779974336972));
#248312=CARTESIAN_POINT('Ctrl Pts',(-44.5914157734028,-63.6426042714052,
-41.3499258753244));
#248313=CARTESIAN_POINT('Ctrl Pts',(-44.0845625322693,-62.5717696510307,
-39.8944822890418));
#248314=CARTESIAN_POINT('Ctrl Pts',(-44.8399443096849,-63.4217307078938,
-40.1779974386957));
#248315=CARTESIAN_POINT('Ctrl Pts',(-44.8399443096849,-63.4217307078937,
-41.3499258784558));
#248316=CARTESIAN_POINT('',(-44.0845625322693,-62.5717696510307,-39.8944822890418));
#248317=CARTESIAN_POINT('Origin',(-43.843501102803,-62.3005255814968,-41.3499258784557));
#248318=CARTESIAN_POINT('',(-43.1889493654702,-62.9502447313255,-39.8182791580079));
#248319=CARTESIAN_POINT('Origin',(-42.9516926065373,-62.6756665304895,-41.2737227474219));
#248320=CARTESIAN_POINT('Ctrl Pts',(-43.1889493654702,-62.9502447313255,
-39.8182791580079));
#248321=CARTESIAN_POINT('Ctrl Pts',(-43.3060164327879,-62.941747862638,
-39.8357596692676));
#248322=CARTESIAN_POINT('Ctrl Pts',(-43.4202366092229,-62.9200777320772,
-39.8503404874849));
#248323=CARTESIAN_POINT('Ctrl Pts',(-43.5315808098265,-62.8850650035002,
-39.8620074891437));
#248324=CARTESIAN_POINT('Ctrl Pts',(-43.576984227273,-62.8707876767701,
-39.8667650045221));
#248325=CARTESIAN_POINT('Ctrl Pts',(-43.6219093041748,-62.8542911619851,
-39.8710378813417));
#248326=CARTESIAN_POINT('Ctrl Pts',(-43.6663535544392,-62.8355615905537,
-39.8748246333721));
#248327=CARTESIAN_POINT('Ctrl Pts',(-43.6664338301504,-62.8355277609885,
-39.8748314730468));
#248328=CARTESIAN_POINT('Ctrl Pts',(-43.6665141020671,-62.8354939250504,
-39.8748383109414));
#248329=CARTESIAN_POINT('Ctrl Pts',(-43.6665943701892,-62.8354600827397,
-39.8748451470561));
#248330=CARTESIAN_POINT('Ctrl Pts',(-43.7466420990545,-62.8017106932806,
-39.8816624917103));
#248331=CARTESIAN_POINT('Ctrl Pts',(-43.8228753762229,-62.7616456114789,
-39.8867070324442));
#248332=CARTESIAN_POINT('Ctrl Pts',(-43.8952322702234,-62.7152894963873,
-39.8899765761625));
#248333=CARTESIAN_POINT('Ctrl Pts',(-43.9616292098301,-62.6727516813436,
-39.8929768113136));
#248334=CARTESIAN_POINT('Ctrl Pts',(-44.0247618696465,-62.62491600457,-39.8944822890418));
#248335=CARTESIAN_POINT('Ctrl Pts',(-44.0845625322693,-62.5717696510307,
-39.8944822890418));
#248336=CARTESIAN_POINT('Origin',(-44.0630480057166,-64.1016158376104,235.35105));
#248337=CARTESIAN_POINT('',(-44.0630480057166,-64.1016158376104,-52.64995));
#248338=CARTESIAN_POINT('Ctrl Pts',(-43.0563273171535,-64.1720126058792,
-41.273722747422));
#248339=CARTESIAN_POINT('Ctrl Pts',(-37.4870209577721,-64.5614564443275,
-40.4393222961258));
#248340=CARTESIAN_POINT('Ctrl Pts',(-31.9038741755017,-64.9518680994243,
-39.7153157040947));
#248341=CARTESIAN_POINT('Ctrl Pts',(-26.299256677934,-65.343781133192,-39.1625636424987));
#248342=CARTESIAN_POINT('Ctrl Pts',(-26.299256677934,-65.343781133192,-39.1625636424987));
#248343=CARTESIAN_POINT('Ctrl Pts',(-26.4161222952887,-65.3356090931445,
-37.971813107807));
#248344=CARTESIAN_POINT('Ctrl Pts',(-26.3607251006126,-64.1700706217802,
-37.7071200530847));
#248345=CARTESIAN_POINT('Ctrl Pts',(-25.9205756959923,-65.3702610870028,
-39.1065428641436));
#248346=CARTESIAN_POINT('Ctrl Pts',(-26.0004074167526,-65.3498956258429,
-37.9286345805822));
#248347=CARTESIAN_POINT('Ctrl Pts',(-25.7896847017718,-64.2113141700146,
-37.6510924855215));
#248348=CARTESIAN_POINT('Ctrl Pts',(-25.5571787362025,-65.4658460313782,
-39.0779244541051));
#248349=CARTESIAN_POINT('Ctrl Pts',(-25.5933889787346,-65.4485099708086,
-37.9059960140076));
#248350=CARTESIAN_POINT('Ctrl Pts',(-25.2415430286856,-64.3562400899596,
-37.6224808645879));
#248351=CARTESIAN_POINT('Ctrl Pts',(-25.2130575054386,-65.6305979870176,
-39.0779244525544));
#248352=CARTESIAN_POINT('Ctrl Pts',(-25.2130575054386,-65.6305979870177,
-37.9059960127943));
#248353=CARTESIAN_POINT('Ctrl Pts',(-24.722024317517,-64.6049655790884,
-37.6224808631404));
#248354=CARTESIAN_POINT('',(-26.3607251006126,-64.1700706217802,-37.7071200530847));
#248355=CARTESIAN_POINT('Origin',(-26.1946219673178,-63.8474350578023,-39.1625636424987));
#248356=CARTESIAN_POINT('',(-24.722024317517,-64.6049655790884,-37.6224808631404));
#248357=CARTESIAN_POINT('Origin',(-24.5653232085747,-64.2776603385407,-39.0779244525544));
#248358=CARTESIAN_POINT('Ctrl Pts',(-24.722024317517,-64.6049655790884,
-37.6224808631404));
#248359=CARTESIAN_POINT('Ctrl Pts',(-24.8664081169227,-64.5358401936933,
-37.6224808635427));
#248360=CARTESIAN_POINT('Ctrl Pts',(-25.0128268065285,-64.4748117336668,
-37.6246896514935));
#248361=CARTESIAN_POINT('Ctrl Pts',(-25.1612581100212,-64.4217914620098,
-37.629072347169));
#248362=CARTESIAN_POINT('Ctrl Pts',(-25.3100469028066,-64.3686434937081,
-37.6334655983456));
#248363=CARTESIAN_POINT('Ctrl Pts',(-25.4608581371227,-64.3235423252056,
-37.6400432640483));
#248364=CARTESIAN_POINT('Ctrl Pts',(-25.6136827889703,-64.2864475050405,
-37.648783682524));
#248365=CARTESIAN_POINT('Ctrl Pts',(-25.7668553223293,-64.2492682442964,
-37.6575439972006));
#248366=CARTESIAN_POINT('Ctrl Pts',(-25.9220505706891,-64.2201318026351,
-37.6684769422025));
#248367=CARTESIAN_POINT('Ctrl Pts',(-26.0792710874908,-64.1990467735369,
-37.6815739018329));
#248368=CARTESIAN_POINT('Ctrl Pts',(-26.1723778756961,-64.1865601122634,
-37.6893299878148));
#248369=CARTESIAN_POINT('Ctrl Pts',(-26.2661951513385,-64.1768980730961,
-37.6978452572376));
#248370=CARTESIAN_POINT('Ctrl Pts',(-26.3607251006126,-64.1700706217802,
-37.7071200530847));
#248371=CARTESIAN_POINT('Ctrl Pts',(-43.9586137318958,-64.1089185934363,
-41.4098789472402));
#248372=CARTESIAN_POINT('Ctrl Pts',(-44.1434687505058,-64.0959922713062,
-40.1874603719527));
#248373=CARTESIAN_POINT('Ctrl Pts',(-44.0941462007501,-62.8828332296677,
-39.9541044945113));
#248374=CARTESIAN_POINT('Ctrl Pts',(-37.7893866621767,-64.5403129745774,
-40.4723364366453));
#248375=CARTESIAN_POINT('Ctrl Pts',(-37.983387269697,-64.5267471306234,
-39.2654008360683));
#248376=CARTESIAN_POINT('Ctrl Pts',(-37.9047806371077,-63.3320208489792,
-39.0165447742965));
#248377=CARTESIAN_POINT('Ctrl Pts',(-31.6035178480626,-64.9728710598491,
-39.6662697593448));
#248378=CARTESIAN_POINT('Ctrl Pts',(-31.7696060423701,-64.9612570419197,
-38.4686952332404));
#248379=CARTESIAN_POINT('Ctrl Pts',(-31.6931000950573,-63.7835313257006,
-38.2104625119264));
#248380=CARTESIAN_POINT('Ctrl Pts',(-25.390939784773,-65.4072968377652,
-39.074508439621));
#248381=CARTESIAN_POINT('Ctrl Pts',(-25.503745040343,-65.3994087258724,
-37.8837048863563));
#248382=CARTESIAN_POINT('Ctrl Pts',(-25.4475537226946,-64.2343331337137,
-37.6186845317716));
#248383=CARTESIAN_POINT('Ctrl Pts',(-26.3607251006126,-64.1700706217802,
-37.7071200530847));
#248384=CARTESIAN_POINT('Ctrl Pts',(-26.9782676591259,-64.1254684477288,
-37.7677101762428));
#248385=CARTESIAN_POINT('Ctrl Pts',(-27.5952002861798,-64.0809650014557,
-37.830358117877));
#248386=CARTESIAN_POINT('Ctrl Pts',(-28.2117112797203,-64.0365095004908,
-37.894983680275));
#248387=CARTESIAN_POINT('Ctrl Pts',(-28.8402455667364,-63.9911870214179,
-37.9608695804625));
#248388=CARTESIAN_POINT('Ctrl Pts',(-29.4683415491132,-63.9459140349067,
-38.0288109893072));
#248389=CARTESIAN_POINT('Ctrl Pts',(-30.0961447214576,-63.9006435374936,
-38.0987229249114));
#248390=CARTESIAN_POINT('Ctrl Pts',(-30.7311061421422,-63.854856863232,
-38.1694320004778));
#248391=CARTESIAN_POINT('Ctrl Pts',(-31.365767875829,-63.8090724214961,
-38.2421567951076));
#248392=CARTESIAN_POINT('Ctrl Pts',(-32.0002275449116,-63.7632534702054,
-38.3168093867271));
#248393=CARTESIAN_POINT('Ctrl Pts',(-32.6418016585458,-63.7169207330836,
-38.39229908707));
#248394=CARTESIAN_POINT('Ctrl Pts',(-33.283168966963,-63.6705524205074,
-38.4697600610882));
#248395=CARTESIAN_POINT('Ctrl Pts',(-33.9243792500023,-63.6241272043221,
-38.5491013957037));
#248396=CARTESIAN_POINT('Ctrl Pts',(-34.5727070787781,-63.5771866601574,
-38.6293234329419));
#248397=CARTESIAN_POINT('Ctrl Pts',(-35.2208741753138,-63.5301876833421,
-38.7114678071238));
#248398=CARTESIAN_POINT('Ctrl Pts',(-35.8688829127333,-63.4831293271622,
-38.7954405439891));
#248399=CARTESIAN_POINT('Ctrl Pts',(-36.528007916167,-63.4352637084019,
-38.8808537911855));
#248400=CARTESIAN_POINT('Ctrl Pts',(-37.1869689079169,-63.3873363978492,
-38.9681586684062));
#248401=CARTESIAN_POINT('Ctrl Pts',(-37.8457206741843,-63.3393720909894,
-39.0572562817087));
#248402=CARTESIAN_POINT('Ctrl Pts',(-38.5108024898544,-63.290946887556,
-39.1472100480005));
#248403=CARTESIAN_POINT('Ctrl Pts',(-39.1756707976568,-63.2424837816027,
-39.2389911692744));
#248404=CARTESIAN_POINT('Ctrl Pts',(-39.840234097892,-63.1940375338189,
-39.3324978732434));
#248405=CARTESIAN_POINT('Ctrl Pts',(-40.5151066360261,-63.144839749058,
-39.4274551280569));
#248406=CARTESIAN_POINT('Ctrl Pts',(-41.1896644203457,-63.095659160954,
-39.524191918062));
#248407=CARTESIAN_POINT('Ctrl Pts',(-41.8637688574652,-63.0465861854865,
-39.6226016607987));
#248408=CARTESIAN_POINT('Ctrl Pts',(-42.3057074499343,-63.014414254088,
-39.6871184638273));
#248409=CARTESIAN_POINT('Ctrl Pts',(-42.7474503238866,-62.9822892633039,
-39.7523543070286));
#248410=CARTESIAN_POINT('Ctrl Pts',(-43.1889493654702,-62.9502447313255,
-39.8182791580079));
#248411=CARTESIAN_POINT('Origin',(0.,-12.9675000200281,-41.3499258784557));
#248412=CARTESIAN_POINT('Origin',(0.,-12.9675000200281,-39.8944822890418));
#248413=CARTESIAN_POINT('Ctrl Pts',(-51.14141857343,30.9911137115562,-41.409878947203));
#248414=CARTESIAN_POINT('Ctrl Pts',(-51.1284922512846,31.175968730169,-40.1874603718989));
#248415=CARTESIAN_POINT('Ctrl Pts',(-49.9153332096598,31.1266461804112,
-39.9541044944637));
#248416=CARTESIAN_POINT('Ctrl Pts',(-51.5728129545556,24.8218866420576,
-40.4723364365686));
#248417=CARTESIAN_POINT('Ctrl Pts',(-51.5592471107002,25.0158872495489,
-39.2654008361028));
#248418=CARTESIAN_POINT('Ctrl Pts',(-50.3645208289796,24.9372806169763,
-39.0165447742893));
#248419=CARTESIAN_POINT('Ctrl Pts',(-52.0053710398143,18.6360178281302,
-39.6662697593861));
#248420=CARTESIAN_POINT('Ctrl Pts',(-51.9937570218959,18.8021060224485,
-38.4686952333466));
#248421=CARTESIAN_POINT('Ctrl Pts',(-50.8160313056482,18.7256000751318,
-38.2104625119396));
#248422=CARTESIAN_POINT('Ctrl Pts',(-52.4397968177151,12.4234397650578,
-39.0745084396475));
#248423=CARTESIAN_POINT('Ctrl Pts',(-52.4319087058198,12.5362450206276,
-37.883704886372));
#248424=CARTESIAN_POINT('Ctrl Pts',(-51.266833113666,12.4800537029801,-37.618684531802));
#248425=CARTESIAN_POINT('Ctrl Pts',(-51.202570601752,13.3932250805846,-37.7071200530847));
#248426=CARTESIAN_POINT('Ctrl Pts',(-51.1579684277001,14.0107676390858,
-37.7677101762413));
#248427=CARTESIAN_POINT('Ctrl Pts',(-51.1134649814269,14.6277002661276,
-37.830358117874));
#248428=CARTESIAN_POINT('Ctrl Pts',(-51.0690094804622,15.2442112596561,
-37.8949836802706));
#248429=CARTESIAN_POINT('Ctrl Pts',(-51.023687001393,15.8727455466137,-37.9608695804517));
#248430=CARTESIAN_POINT('Ctrl Pts',(-50.9784140148859,16.5008415289319,
-38.0288109892898));
#248431=CARTESIAN_POINT('Ctrl Pts',(-50.9331435174771,17.1286447012179,
-38.0987229248871));
#248432=CARTESIAN_POINT('Ctrl Pts',(-50.8873568432167,17.7636061218883,
-38.1694320004514));
#248433=CARTESIAN_POINT('Ctrl Pts',(-50.8415724014823,18.3982678555611,
-38.2421567950793));
#248434=CARTESIAN_POINT('Ctrl Pts',(-50.7957534501932,19.0327275246296,
-38.3168093866967));
#248435=CARTESIAN_POINT('Ctrl Pts',(-50.749420713076,19.6743016382088,-38.3922990870328));
#248436=CARTESIAN_POINT('Ctrl Pts',(-50.7030524005045,20.315668946571,-38.4697600610437));
#248437=CARTESIAN_POINT('Ctrl Pts',(-50.656627184324,20.9568792295554,-38.5491013956518));
#248438=CARTESIAN_POINT('Ctrl Pts',(-50.6096866401672,21.6052070582347,
-38.6293234328774));
#248439=CARTESIAN_POINT('Ctrl Pts',(-50.5626876633598,22.2533741546739,
-38.7114678070461));
#248440=CARTESIAN_POINT('Ctrl Pts',(-50.5156293071878,22.9013828919971,
-38.7954405438977));
#248441=CARTESIAN_POINT('Ctrl Pts',(-50.4677636884305,23.5605078954009,
-38.8808537910891));
#248442=CARTESIAN_POINT('Ctrl Pts',(-50.4198363778808,24.2194688871211,
-38.9681586683046));
#248443=CARTESIAN_POINT('Ctrl Pts',(-50.3718720710237,24.8782206533588,
-39.0572562816017));
#248444=CARTESIAN_POINT('Ctrl Pts',(-50.3234468675883,25.5433024690615,
-39.1472100478965));
#248445=CARTESIAN_POINT('Ctrl Pts',(-50.2749837616329,26.2081707768964,
-39.2389911691736));
#248446=CARTESIAN_POINT('Ctrl Pts',(-50.2265375138466,26.8727340771642,
-39.3324978731459));
#248447=CARTESIAN_POINT('Ctrl Pts',(-50.1773397290819,27.5476066153477,
-39.4274551279651));
#248448=CARTESIAN_POINT('Ctrl Pts',(-50.1281591409739,28.2221643997166,
-39.524191917976));
#248449=CARTESIAN_POINT('Ctrl Pts',(-50.0790861655016,28.8962688368852,
-39.6226016607187));
#248450=CARTESIAN_POINT('Ctrl Pts',(-50.0469142340889,29.3382074295385,
-39.6871184637734));
#248451=CARTESIAN_POINT('Ctrl Pts',(-50.0147892432904,29.7799503036747,
-39.7523543070014));
#248452=CARTESIAN_POINT('Ctrl Pts',(-49.9827447112974,30.221449345442,-39.8182791580079));
#248453=CARTESIAN_POINT('Origin',(0.,-12.9675000200281,-41.3499258784557));
#248454=CARTESIAN_POINT('Origin',(0.,-12.9675000200281,-39.8944822890418));
#248455=CARTESIAN_POINT('Ctrl Pts',(-25.390939784986,39.4722967976939,-39.0745084396377));
#248456=CARTESIAN_POINT('Ctrl Pts',(-25.5037450405553,39.4644086857989,
-37.8837048863654));
#248457=CARTESIAN_POINT('Ctrl Pts',(-25.4475537229077,38.2993330936448,
-37.6186845317924));
#248458=CARTESIAN_POINT('Ctrl Pts',(-31.6035178481249,39.0378710197884,
-39.6662697593827));
#248459=CARTESIAN_POINT('Ctrl Pts',(-31.7696060424436,39.0262570018692,
-38.4686952333224));
#248460=CARTESIAN_POINT('Ctrl Pts',(-31.6931000951265,37.8485312856233,
-38.2104625119342));
#248461=CARTESIAN_POINT('Ctrl Pts',(-37.78938666212,38.6053129345249,-40.4723364365685));
#248462=CARTESIAN_POINT('Ctrl Pts',(-37.9833872696133,38.59174709065,-39.2654008361018));
#248463=CARTESIAN_POINT('Ctrl Pts',(-37.9047806370375,37.397020808928,-39.0165447742889));
#248464=CARTESIAN_POINT('Ctrl Pts',(-43.9586137316839,38.1739185533947,
-41.4098789472187));
#248465=CARTESIAN_POINT('Ctrl Pts',(-44.143468750297,38.1609922312524,-40.1874603719145));
#248466=CARTESIAN_POINT('Ctrl Pts',(-44.0941462005395,36.9478331896271,
-39.9541044944794));
#248467=CARTESIAN_POINT('Ctrl Pts',(-43.1889493654703,37.0152446912691,
-39.8182791580079));
#248468=CARTESIAN_POINT('Ctrl Pts',(-42.4904603455135,37.0659418652793,
-39.7139804388393));
#248469=CARTESIAN_POINT('Ctrl Pts',(-41.7913631998226,37.1168384172332,
-39.6114063013225));
#248470=CARTESIAN_POINT('Ctrl Pts',(-41.0918404324428,37.1678090072805,
-39.5106756721723));
#248471=CARTESIAN_POINT('Ctrl Pts',(-40.4273733396133,37.2162252724371,
-39.4149930276158));
#248472=CARTESIAN_POINT('Ctrl Pts',(-39.7625221889097,37.264708707939,-39.3209737511287));
#248473=CARTESIAN_POINT('Ctrl Pts',(-39.0974046393108,37.3131849458321,
-39.2287197708965));
#248474=CARTESIAN_POINT('Ctrl Pts',(-38.4397880037208,37.3611144892467,
-39.1375061919785));
#248475=CARTESIAN_POINT('Ctrl Pts',(-37.7819111637672,37.4090371649522,
-39.0480183173054));
#248476=CARTESIAN_POINT('Ctrl Pts',(-37.1238471677498,37.4569106864784,
-38.9603546652988));
#248477=CARTESIAN_POINT('Ctrl Pts',(-36.4731112694083,37.5042510959609,
-38.873667222002));
#248478=CARTESIAN_POINT('Ctrl Pts',(-35.8221925731159,37.551543640539,-38.7887635990717));
#248479=CARTESIAN_POINT('Ctrl Pts',(-35.1711185085701,37.5987738016015,
-38.7057390601872));
#248480=CARTESIAN_POINT('Ctrl Pts',(-34.5272799080192,37.6454790882318,
-38.623637182939));
#248481=CARTESIAN_POINT('Ctrl Pts',(-33.8832895753389,37.6921236016348,
-38.5433728568344));
#248482=CARTESIAN_POINT('Ctrl Pts',(-33.2391284750776,37.738716035705,-38.4650382046873));
#248483=CARTESIAN_POINT('Ctrl Pts',(-32.6058302106908,37.7845227564434,
-38.3880245520065));
#248484=CARTESIAN_POINT('Ctrl Pts',(-31.9723670273983,37.8302794124422,
-38.3128760397775));
#248485=CARTESIAN_POINT('Ctrl Pts',(-31.3386741185916,37.8760126096808,
-38.2396802084161));
#248486=CARTESIAN_POINT('Ctrl Pts',(-30.7112206329954,37.9212955118816,
-38.1672050727778));
#248487=CARTESIAN_POINT('Ctrl Pts',(-30.0835420992274,37.9665556913751,
-38.09664435461));
#248488=CARTESIAN_POINT('Ctrl Pts',(-29.4555270109952,38.0118330876516,
-38.0280830339018));
#248489=CARTESIAN_POINT('Ctrl Pts',(-28.8372567832138,38.0564079181513,
-37.9605855737842));
#248490=CARTESIAN_POINT('Ctrl Pts',(-28.2186604708678,38.1009997405071,
-37.8950259435464));
#248491=CARTESIAN_POINT('Ctrl Pts',(-27.5995823364983,38.1456560947805,
-37.8314852283597));
#248492=CARTESIAN_POINT('Ctrl Pts',(-27.1868647446055,38.1754269136404,
-37.789124871075));
#248493=CARTESIAN_POINT('Ctrl Pts',(-26.7739319975608,38.2052266046837,
-37.7476618043058));
#248494=CARTESIAN_POINT('Ctrl Pts',(-26.3607251006129,38.2350705817238,
-37.7071200530847));
#248495=CARTESIAN_POINT('Origin',(26.5085260991663,-68.3364732839715,-55.24995));
#248496=CARTESIAN_POINT('',(26.299256677934,-65.343781133192,-39.1625636424987));
#248497=CARTESIAN_POINT('',(26.299256677934,-65.343781133192,-52.64995));
#248498=CARTESIAN_POINT('',(26.299256677934,-65.343781133192,-52.64995));
#248499=CARTESIAN_POINT('',(25.2130575054386,-65.6305979870176,-39.0779244525544));
#248500=CARTESIAN_POINT('Ctrl Pts',(26.299256677934,-65.343781133192,-39.1625636424987));
#248501=CARTESIAN_POINT('Ctrl Pts',(26.2254373064082,-65.3489430865025,
-39.1516430551934));
#248502=CARTESIAN_POINT('Ctrl Pts',(26.1520152366826,-65.3567479315796,
-39.1417380677395));
#248503=CARTESIAN_POINT('Ctrl Pts',(26.0791903717072,-65.3672001454729,
-39.1328886242715));
#248504=CARTESIAN_POINT('Ctrl Pts',(26.0033259821766,-65.3780886081775,
-39.1236698275513));
#248505=CARTESIAN_POINT('Ctrl Pts',(25.9281098779661,-65.3918504119504,
-39.1155967042653));
#248506=CARTESIAN_POINT('Ctrl Pts',(25.8537553847433,-65.4084357764527,
-39.1086925042226));
#248507=CARTESIAN_POINT('Ctrl Pts',(25.7824469356956,-65.4243416964353,
-39.1020711451678));
#248508=CARTESIAN_POINT('Ctrl Pts',(25.711930945636,-65.4428441967757,-39.0965247723696));
#248509=CARTESIAN_POINT('Ctrl Pts',(25.6423830881242,-65.4638512240535,
-39.0920542502616));
#248510=CARTESIAN_POINT('Ctrl Pts',(25.5726544940153,-65.4849128430724,
-39.087572110442));
#248511=CARTESIAN_POINT('Ctrl Pts',(25.5038991449303,-65.5084919753254,
-39.0841714266781));
#248512=CARTESIAN_POINT('Ctrl Pts',(25.4362806067455,-65.5344490373293,
-39.081833571492));
#248513=CARTESIAN_POINT('Ctrl Pts',(25.3682218634524,-65.5605750830409,
-39.0794804965774));
#248514=CARTESIAN_POINT('Ctrl Pts',(25.3013148512129,-65.5891100638622,
-39.0782041359531));
#248515=CARTESIAN_POINT('Ctrl Pts',(25.2357116044156,-65.6198650319822,
-39.0779656809084));
#248516=CARTESIAN_POINT('Ctrl Pts',(25.2281428273083,-65.6234132938444,
-39.0779381698754));
#248517=CARTESIAN_POINT('Ctrl Pts',(25.2205913875361,-65.626991055221,-39.0779244525544));
#248518=CARTESIAN_POINT('Ctrl Pts',(25.2130575054386,-65.6305979870176,
-39.0779244525544));
#248519=CARTESIAN_POINT('',(25.2130575054386,-65.6305979870176,-52.64995));
#248520=CARTESIAN_POINT('',(25.2130575054386,-65.6305979870176,-55.24995));
#248521=CARTESIAN_POINT('Origin',(26.5085260991663,-68.3364732839715,-52.64995));
#248522=CARTESIAN_POINT('Origin',(55.3689732639432,-39.4760261191947,-55.24995));
#248523=CARTESIAN_POINT('',(52.6630979669894,-38.1805575254669,-39.0779244525544));
#248524=CARTESIAN_POINT('',(52.6630979669894,-38.1805575254669,-52.64995));
#248525=CARTESIAN_POINT('',(52.6630979669894,-38.1805575254669,-55.24995));
#248526=CARTESIAN_POINT('',(52.3762811131638,-39.2667566979623,-39.1625636424987));
#248527=CARTESIAN_POINT('Ctrl Pts',(52.6630979669894,-38.1805575254669,
-39.0779244525544));
#248528=CARTESIAN_POINT('Ctrl Pts',(52.6318538057676,-38.2458179296431,
-39.0779244525544));
#248529=CARTESIAN_POINT('Ctrl Pts',(52.6028021694694,-38.3123970248505,
-39.0789553362961));
#248530=CARTESIAN_POINT('Ctrl Pts',(52.5761369448303,-38.380144816412,-39.0810581140022));
#248531=CARTESIAN_POINT('Ctrl Pts',(52.5486170513734,-38.4500640475814,
-39.0832282895481));
#248532=CARTESIAN_POINT('Ctrl Pts',(52.5236393921055,-38.5212281199008,
-39.0865403103588));
#248533=CARTESIAN_POINT('Ctrl Pts',(52.5013651848038,-38.5934555718355,
-39.091017145468));
#248534=CARTESIAN_POINT('Ctrl Pts',(52.4799837840479,-38.6627879648801,
-39.095314537707));
#248535=CARTESIAN_POINT('Ctrl Pts',(52.4610932034441,-38.7331000345627,
-39.1006851051596));
#248536=CARTESIAN_POINT('Ctrl Pts',(52.4447889514025,-38.804217595539,-39.1071295131387));
#248537=CARTESIAN_POINT('Ctrl Pts',(52.4284881332189,-38.8753201783607,
-39.1135725638534));
#248538=CARTESIAN_POINT('Ctrl Pts',(52.4147725871611,-38.9472278341315,
-39.1210889899846));
#248539=CARTESIAN_POINT('Ctrl Pts',(52.4036908710759,-39.0197541971,-39.1296602879662));
#248540=CARTESIAN_POINT('Ctrl Pts',(52.3925835339235,-39.0924482419338,
-39.1382514028967));
#248541=CARTESIAN_POINT('Ctrl Pts',(52.3841222371824,-39.1657637734407,
-39.1479022534551));
#248542=CARTESIAN_POINT('Ctrl Pts',(52.3783083555277,-39.2395020072502,
-39.158575180387));
#248543=CARTESIAN_POINT('Ctrl Pts',(52.377592552146,-39.248580636685,-39.1598892279794));
#248544=CARTESIAN_POINT('Ctrl Pts',(52.3769168204106,-39.2576656607894,
-39.1612187453113));
#248545=CARTESIAN_POINT('Ctrl Pts',(52.3762811131638,-39.2667566979623,
-39.1625636424987));
#248546=CARTESIAN_POINT('',(52.3762811131638,-39.2667566979623,-52.64995));
#248547=CARTESIAN_POINT('',(52.3762811131638,-39.2667566979623,-37.9059960127943));
#248548=CARTESIAN_POINT('Origin',(55.3689732639432,-39.4760261191947,-52.64995));
#248549=CARTESIAN_POINT('Origin',(55.3689732639433,13.5410260791383,-55.24995));
#248550=CARTESIAN_POINT('',(52.3762811131638,13.3317566579059,-39.1625636424987));
#248551=CARTESIAN_POINT('',(52.3762811131638,13.3317566579059,-52.64995));
#248552=CARTESIAN_POINT('',(52.3762811131638,13.3317566579059,-52.64995));
#248553=CARTESIAN_POINT('',(52.6630979669895,12.2455574854105,-39.0779244525544));
#248554=CARTESIAN_POINT('Ctrl Pts',(52.3762811131638,13.3317566579059,-39.1625636424987));
#248555=CARTESIAN_POINT('Ctrl Pts',(52.3814430664743,13.257937286379,-39.1516430551932));
#248556=CARTESIAN_POINT('Ctrl Pts',(52.3892479115517,13.1845152166523,-39.1417380677392));
#248557=CARTESIAN_POINT('Ctrl Pts',(52.3997001254452,13.1116903516758,-39.1328886242711));
#248558=CARTESIAN_POINT('Ctrl Pts',(52.4105885881499,13.0358259621455,-39.1236698275509));
#248559=CARTESIAN_POINT('Ctrl Pts',(52.4243503919228,12.9606098579354,-39.115596704265));
#248560=CARTESIAN_POINT('Ctrl Pts',(52.4409357564251,12.8862553647129,-39.1086925042223));
#248561=CARTESIAN_POINT('Ctrl Pts',(52.4568416764079,12.8149469156643,-39.1020711451675));
#248562=CARTESIAN_POINT('Ctrl Pts',(52.4753441767486,12.7444309256038,-39.0965247723692));
#248563=CARTESIAN_POINT('Ctrl Pts',(52.4963512040269,12.6748830680911,-39.0920542502613));
#248564=CARTESIAN_POINT('Ctrl Pts',(52.5174128230462,12.6051544739813,-39.0875721104417));
#248565=CARTESIAN_POINT('Ctrl Pts',(52.5409919552997,12.5363991248954,-39.0841714266778));
#248566=CARTESIAN_POINT('Ctrl Pts',(52.5669490173042,12.4687805867097,-39.0818335714918));
#248567=CARTESIAN_POINT('Ctrl Pts',(52.5930750630163,12.4007218434158,-39.0794804965772));
#248568=CARTESIAN_POINT('Ctrl Pts',(52.6216100438381,12.3338148311756,-39.078204135953));
#248569=CARTESIAN_POINT('Ctrl Pts',(52.6523650119588,12.2682115843776,-39.0779656809083));
#248570=CARTESIAN_POINT('Ctrl Pts',(52.6559132738194,12.2606428072736,-39.0779381698754));
#248571=CARTESIAN_POINT('Ctrl Pts',(52.6594910351945,12.2530913675048,-39.0779244525544));
#248572=CARTESIAN_POINT('Ctrl Pts',(52.6630979669895,12.2455574854105,-39.0779244525544));
#248573=CARTESIAN_POINT('',(52.6630979669895,12.2455574854105,-52.64995));
#248574=CARTESIAN_POINT('',(52.6630979669895,12.2455574854105,-55.24995));
#248575=CARTESIAN_POINT('Origin',(55.3689732639433,13.5410260791383,-52.64995));
#248576=CARTESIAN_POINT('Origin',(26.5085260991666,42.4014732439151,-55.24995));
#248577=CARTESIAN_POINT('',(25.2130575054389,39.6955979469612,-39.0779244525544));
#248578=CARTESIAN_POINT('',(25.2130575054389,39.6955979469612,-52.64995));
#248579=CARTESIAN_POINT('',(25.2130575054389,39.6955979469612,-55.24995));
#248580=CARTESIAN_POINT('',(26.2992566779342,39.4087810931356,-39.1625636424987));
#248581=CARTESIAN_POINT('Ctrl Pts',(25.2130575054389,39.6955979469612,-39.0779244525544));
#248582=CARTESIAN_POINT('Ctrl Pts',(25.2783179096223,39.6643537857359,-39.0779244525544));
#248583=CARTESIAN_POINT('Ctrl Pts',(25.3448970048371,39.6353021494348,-39.0789553362963));
#248584=CARTESIAN_POINT('Ctrl Pts',(25.4126447964065,39.6086369247934,-39.081058114003));
#248585=CARTESIAN_POINT('Ctrl Pts',(25.4825640275743,39.5811170313378,-39.083228289549));
#248586=CARTESIAN_POINT('Ctrl Pts',(25.553728099892,39.5561393720712,-39.0865403103599));
#248587=CARTESIAN_POINT('Ctrl Pts',(25.625955551825,39.5338651647706,-39.0910171454692));
#248588=CARTESIAN_POINT('Ctrl Pts',(25.6952879448785,39.5124837640123,-39.0953145377089));
#248589=CARTESIAN_POINT('Ctrl Pts',(25.7656000145702,39.4935931834069,-39.1006851051625));
#248590=CARTESIAN_POINT('Ctrl Pts',(25.8367175755558,39.4772889313643,-39.1071295131429));
#248591=CARTESIAN_POINT('Ctrl Pts',(25.9078201583872,39.4609881131796,-39.1135725638588));
#248592=CARTESIAN_POINT('Ctrl Pts',(25.9797278141677,39.4472725671214,-39.1210889899916));
#248593=CARTESIAN_POINT('Ctrl Pts',(26.0522541771461,39.4361908510365,-39.1296602879749));
#248594=CARTESIAN_POINT('Ctrl Pts',(26.1249482219899,39.4250835138844,-39.1382514029073));
#248595=CARTESIAN_POINT('Ctrl Pts',(26.198263753507,39.4166222171442,-39.1479022534678));
#248596=CARTESIAN_POINT('Ctrl Pts',(26.2720019873267,39.4108083354913,-39.1585751804022));
#248597=CARTESIAN_POINT('Ctrl Pts',(26.2810806167268,39.4100925321126,-39.1598892279896));
#248598=CARTESIAN_POINT('Ctrl Pts',(26.2901656407963,39.4094168003799,-39.1612187453165));
#248599=CARTESIAN_POINT('Ctrl Pts',(26.2992566779342,39.4087810931356,-39.1625636424987));
#248600=CARTESIAN_POINT('',(26.2992566779342,39.4087810931356,-52.64995));
#248601=CARTESIAN_POINT('',(26.2992566779342,39.4087810931356,-37.9059960127943));
#248602=CARTESIAN_POINT('Origin',(26.5085260991666,42.4014732439151,-52.64995));
#248603=CARTESIAN_POINT('Origin',(0.,-12.9675000200281,-55.24995));
#248604=CARTESIAN_POINT('Origin',(0.,-12.9675000200281,-39.0779244525544));
#248605=CARTESIAN_POINT('Origin',(0.,-12.9675000200281,-52.64995));
#248606=CARTESIAN_POINT('Ctrl Pts',(24.7220243175171,38.669965539032,-37.6224808631404));
#248607=CARTESIAN_POINT('Ctrl Pts',(25.2130575054388,39.6955979469612,-37.9059960127943));
#248608=CARTESIAN_POINT('Ctrl Pts',(25.2130575054389,39.6955979469612,-39.0779244525544));
#248609=CARTESIAN_POINT('Ctrl Pts',(25.2415430286799,38.4212400498976,-37.6224808645859));
#248610=CARTESIAN_POINT('Ctrl Pts',(25.5933889787397,39.5135099307705,-37.9059960140155));
#248611=CARTESIAN_POINT('Ctrl Pts',(25.5571787362036,39.5308459913215,-39.077924454111));
#248612=CARTESIAN_POINT('Ctrl Pts',(25.7896847017763,38.2763141299578,-37.6510924855219));
#248613=CARTESIAN_POINT('Ctrl Pts',(26.0004074167487,39.4148955857669,-37.9286345805798));
#248614=CARTESIAN_POINT('Ctrl Pts',(25.9205756959913,39.4352610469465,-39.1065428641433));
#248615=CARTESIAN_POINT('Ctrl Pts',(26.3607251006129,38.2350705817238,-37.7071200530847));
#248616=CARTESIAN_POINT('Ctrl Pts',(26.4161222952889,39.4006090530882,-37.971813107807));
#248617=CARTESIAN_POINT('Ctrl Pts',(26.2992566779342,39.4087810931356,-39.1625636424987));
#248618=CARTESIAN_POINT('',(24.7220243175171,38.669965539032,-37.6224808631404));
#248619=CARTESIAN_POINT('Origin',(24.5653232085749,38.3426602984844,-39.0779244525544));
#248620=CARTESIAN_POINT('',(26.3607251006129,38.2350705817238,-37.7071200530847));
#248621=CARTESIAN_POINT('Ctrl Pts',(26.3607251006129,38.2350705817238,-37.7071200530847));
#248622=CARTESIAN_POINT('Ctrl Pts',(26.2011255350992,38.2465977037834,-37.6914609588104));
#248623=CARTESIAN_POINT('Ctrl Pts',(26.0435569434565,38.2662022062977,-37.6779662189505));
#248624=CARTESIAN_POINT('Ctrl Pts',(25.8880107550447,38.2938462174384,-37.6666367941389));
#248625=CARTESIAN_POINT('Ctrl Pts',(25.7326779997654,38.3214522967729,-37.6553229150289));
#248626=CARTESIAN_POINT('Ctrl Pts',(25.5793619804298,38.3570758581462,-37.6461683926629));
#248627=CARTESIAN_POINT('Ctrl Pts',(25.4280646493686,38.4007283517996,-37.6391871086171));
#248628=CARTESIAN_POINT('Ctrl Pts',(25.2772986540836,38.4442275437957,-37.6322303418973));
#248629=CARTESIAN_POINT('Ctrl Pts',(25.1285370763278,38.4956993999497,-37.6274315578455));
#248630=CARTESIAN_POINT('Ctrl Pts',(24.9817940407082,38.5552037278875,-37.624817614644));
#248631=CARTESIAN_POINT('Ctrl Pts',(24.8944876056227,38.590606503375,-37.623262419459));
#248632=CARTESIAN_POINT('Ctrl Pts',(24.8078959327013,38.6288535270284,-37.6224808633793));
#248633=CARTESIAN_POINT('Ctrl Pts',(24.7220243175172,38.669965539032,-37.6224808631404));
#248634=CARTESIAN_POINT('Origin',(26.194621967318,37.9124350177459,-39.1625636424987));
#248635=CARTESIAN_POINT('Origin',(48.2118204350716,29.879557875893,235.35105));
#248636=CARTESIAN_POINT('',(50.4542306878656,31.8724442896568,-41.3499258784557));
#248637=CARTESIAN_POINT('',(50.4542306878656,31.8724442896568,-52.64995));
#248638=CARTESIAN_POINT('',(50.4542306878656,31.8724442896567,235.35105));
#248639=CARTESIAN_POINT('',(51.2045125858511,30.0888272971254,-41.2737227474219));
#248640=CARTESIAN_POINT('Ctrl Pts',(50.4542306878656,31.8724442896568,-41.3499258784557));
#248641=CARTESIAN_POINT('Ctrl Pts',(50.5181129933322,31.8005634560272,-41.3499258784558));
#248642=CARTESIAN_POINT('Ctrl Pts',(50.5788912011241,31.7252093793369,-41.3493408309145));
#248643=CARTESIAN_POINT('Ctrl Pts',(50.6361616709643,31.6466372662856,-41.3481707358316));
#248644=CARTESIAN_POINT('Ctrl Pts',(50.6929598518543,31.5687131091685,-41.3470102901017));
#248645=CARTESIAN_POINT('Ctrl Pts',(50.7463075433695,31.4876238374954,-41.3452744063958));
#248646=CARTESIAN_POINT('Ctrl Pts',(50.7958274996612,31.403666628624,-41.3429630847142));
#248647=CARTESIAN_POINT('Ctrl Pts',(50.8449448069292,31.3203920796478,-41.3406705564946));
#248648=CARTESIAN_POINT('Ctrl Pts',(50.8902960139758,31.2342961473852,-41.3378119100797));
#248649=CARTESIAN_POINT('Ctrl Pts',(50.9315346868522,31.1457152076104,-41.3343871454692));
#248650=CARTESIAN_POINT('Ctrl Pts',(50.9722785909486,31.0581970344193,-41.3310034701201));
#248651=CARTESIAN_POINT('Ctrl Pts',(51.0090077268708,30.9682532960156,-41.3270671793063));
#248652=CARTESIAN_POINT('Ctrl Pts',(51.0414142689238,30.8762517784658,-41.3225782730277));
#248653=CARTESIAN_POINT('Ctrl Pts',(51.0735998270302,30.784877629871,-41.3181199771185));
#248654=CARTESIAN_POINT('Ctrl Pts',(51.1015212128023,30.6914738422423,-41.3131165767449));
#248655=CARTESIAN_POINT('Ctrl Pts',(51.1249078316996,30.5964412831547,-41.3075680719069));
#248656=CARTESIAN_POINT('Ctrl Pts',(51.1480518192897,30.5023946671032,-41.3020771316527));
#248657=CARTESIAN_POINT('Ctrl Pts',(51.1667543600226,30.4067531287956,-41.2960523389518));
#248658=CARTESIAN_POINT('Ctrl Pts',(51.1807881805032,30.3099420375285,-41.2894936938044));
#248659=CARTESIAN_POINT('Ctrl Pts',(51.191385421931,30.2368378882726,-41.2845411189755));
#248660=CARTESIAN_POINT('Ctrl Pts',(51.1993211964125,30.1630676248948,-41.279284136848));
#248661=CARTESIAN_POINT('Ctrl Pts',(51.2045125858511,30.0888272971254,-41.2737227474219));
#248662=CARTESIAN_POINT('',(51.2045125858511,30.0888272971254,-52.64995));
#248663=CARTESIAN_POINT('',(51.2045125858511,30.0888272971253,235.35105));
#248664=CARTESIAN_POINT('Origin',(48.2118204350716,29.879557875893,-52.64995));
#248665=CARTESIAN_POINT('Origin',(42.8470578959213,35.2443204150433,235.35105));
#248666=CARTESIAN_POINT('',(43.0563273171537,38.2370125658228,-41.2737227474219));
#248667=CARTESIAN_POINT('',(43.0563273171537,38.2370125658228,-52.64995));
#248668=CARTESIAN_POINT('',(43.0563273171537,38.2370125658227,235.35105));
#248669=CARTESIAN_POINT('',(44.839944309685,37.4867306678373,-41.3499258784557));
#248670=CARTESIAN_POINT('Ctrl Pts',(43.0563273171537,38.2370125658227,-41.2737227474219));
#248671=CARTESIAN_POINT('Ctrl Pts',(43.154629171652,38.2301386305295,-41.2810866008773));
#248672=CARTESIAN_POINT('Ctrl Pts',(43.2521056977309,38.2184516355055,-41.2879167524659));
#248673=CARTESIAN_POINT('Ctrl Pts',(43.3483058302563,38.2021490964115,-41.2942132021878));
#248674=CARTESIAN_POINT('Ctrl Pts',(43.4452418270719,38.1857218542009,-41.3005578153829));
#248675=CARTESIAN_POINT('Ctrl Pts',(43.5408815832291,38.1646084828715,-41.3063605305851));
#248676=CARTESIAN_POINT('Ctrl Pts',(43.6347991557083,38.1390507492245,-41.3116213477944));
#248677=CARTESIAN_POINT('Ctrl Pts',(43.7294452772313,38.1132947559556,-41.3169229748677));
#248678=CARTESIAN_POINT('Ctrl Pts',(43.8223421816389,38.0830255004283,-41.3216742639821));
#248679=CARTESIAN_POINT('Ctrl Pts',(43.9130933638555,38.0485258962993,-41.3258752151377));
#248680=CARTESIAN_POINT('Ctrl Pts',(44.0049695254192,38.01359862455,-41.3301282425657));
#248681=CARTESIAN_POINT('Ctrl Pts',(44.0946462283388,37.9743357949492,-41.3338172031509));
#248682=CARTESIAN_POINT('Ctrl Pts',(44.1817555311144,37.9310623495449,-41.3369420968931));
#248683=CARTESIAN_POINT('Ctrl Pts',(44.2694569033968,37.8874947807043,-41.3400882300923));
#248684=CARTESIAN_POINT('Ctrl Pts',(44.3545557283222,37.8398622590698,-41.3426626026266));
#248685=CARTESIAN_POINT('Ctrl Pts',(44.4367228234257,37.7885227297703,-41.3446652144958));
#248686=CARTESIAN_POINT('Ctrl Pts',(44.5198078063777,37.7366096870706,-41.3466901975235));
#248687=CARTESIAN_POINT('Ctrl Pts',(44.5998950713162,37.6809067185249,-41.3481305742695));
#248688=CARTESIAN_POINT('Ctrl Pts',(44.6766934223472,37.6218051869062,-41.3489863447338));
#248689=CARTESIAN_POINT('Ctrl Pts',(44.7329036980364,37.5785475734113,-41.3496127005485));
#248690=CARTESIAN_POINT('Ctrl Pts',(44.7873531091644,37.5334697910065,-41.3499258784558));
#248691=CARTESIAN_POINT('Ctrl Pts',(44.8399443096851,37.4867306678373,-41.3499258784558));
#248692=CARTESIAN_POINT('',(44.839944309685,37.4867306678373,-52.64995));
#248693=CARTESIAN_POINT('',(44.839944309685,37.4867306678373,235.35105));
#248694=CARTESIAN_POINT('Origin',(42.8470578959213,35.2443204150433,-52.64995));
#248695=CARTESIAN_POINT('Origin',(44.0630480057168,38.1666157975539,235.35105));
#248696=CARTESIAN_POINT('Ctrl Pts',(26.2992566779342,39.4087810931356,-39.1625636424987));
#248697=CARTESIAN_POINT('Ctrl Pts',(31.903874175502,39.0168680593679,-39.7153157040946));
#248698=CARTESIAN_POINT('Ctrl Pts',(37.4870209577723,38.6264564042711,-40.4393222961257));
#248699=CARTESIAN_POINT('Ctrl Pts',(43.0563273171537,38.2370125658228,-41.2737227474219));
#248700=CARTESIAN_POINT('',(44.0630480057168,38.166615797554,-52.64995));
#248701=CARTESIAN_POINT('Ctrl Pts',(44.839944309685,37.4867306678373,-41.3499258784558));
#248702=CARTESIAN_POINT('Ctrl Pts',(44.8399443096851,37.4867306678373,-40.1779974386957));
#248703=CARTESIAN_POINT('Ctrl Pts',(44.0845625322695,36.6367696109743,-39.8944822890418));
#248704=CARTESIAN_POINT('Ctrl Pts',(44.5912415343056,37.7077590820187,-41.3499258752894));
#248705=CARTESIAN_POINT('Ctrl Pts',(44.6149072014673,37.6867267800084,-40.1779974336417));
#248706=CARTESIAN_POINT('Ctrl Pts',(43.9595274298496,36.7478914351849,-39.8944822858058));
#248707=CARTESIAN_POINT('Ctrl Pts',(44.3136937213669,37.8823162857708,-41.343363404867));
#248708=CARTESIAN_POINT('Ctrl Pts',(44.3663746862182,37.849051706332,-40.1674920635188));
#248709=CARTESIAN_POINT('Ctrl Pts',(43.8200866324971,36.835758129222,-39.887919815423));
#248710=CARTESIAN_POINT('Ctrl Pts',(43.7019124427066,38.1390166965721,-41.3171961008681));
#248711=CARTESIAN_POINT('Ctrl Pts',(43.8196015906779,38.1008702319186,-40.1253788430241));
#248712=CARTESIAN_POINT('Ctrl Pts',(43.5128927223798,36.9652495181622,-39.8617525114841));
#248713=CARTESIAN_POINT('Ctrl Pts',(43.3844623592655,38.214067128441,-41.2983035466937));
#248714=CARTESIAN_POINT('Ctrl Pts',(43.5344232858197,38.1836802846001,-40.0946545134465));
#248715=CARTESIAN_POINT('Ctrl Pts',(43.3535628849498,37.0032968338361,-39.8428593266731));
#248716=CARTESIAN_POINT('Ctrl Pts',(43.0563273171537,38.2370125658228,-41.2737227474219));
#248717=CARTESIAN_POINT('Ctrl Pts',(43.23812030497,38.224300361751,-40.0543903140502));
#248718=CARTESIAN_POINT('Ctrl Pts',(43.1889493654704,37.0152446912691,-39.8182791580079));
#248719=CARTESIAN_POINT('',(43.1889493654704,37.0152446912691,-39.8182791580079));
#248720=CARTESIAN_POINT('Origin',(42.9516926065375,36.740666490433,-41.2737227474219));
#248721=CARTESIAN_POINT('',(44.0845625322695,36.6367696109743,-39.8944822890418));
#248722=CARTESIAN_POINT('Ctrl Pts',(44.0845625322695,36.6367696109743,-39.8944822890418));
#248723=CARTESIAN_POINT('Ctrl Pts',(43.9941797939515,36.7170950246707,-39.8944822890418));
#248724=CARTESIAN_POINT('Ctrl Pts',(43.8962901478094,36.7852564677658,-39.8910542505833));
#248725=CARTESIAN_POINT('Ctrl Pts',(43.7909432593811,36.8413335920204,-39.8842118316081));
#248726=CARTESIAN_POINT('Ctrl Pts',(43.7506303648273,36.862792519101,-39.8815934560798));
#248727=CARTESIAN_POINT('Ctrl Pts',(43.7092251907653,36.8824814307082,-39.8784749689682));
#248728=CARTESIAN_POINT('Ctrl Pts',(43.6667294913925,36.9004031219782,-39.8748566639276));
#248729=CARTESIAN_POINT('Ctrl Pts',(43.6666496039709,36.9004368128629,-39.8748498618967));
#248730=CARTESIAN_POINT('Ctrl Pts',(43.666569712705,36.9004704974973,-39.8748430581001));
#248731=CARTESIAN_POINT('Ctrl Pts',(43.6664898175948,36.9005041758817,-39.8748362525378));
#248732=CARTESIAN_POINT('Ctrl Pts',(43.5643771770591,36.9435479709188,-39.8661381741221));
#248733=CARTESIAN_POINT('Ctrl Pts',(43.4597085659155,36.9748052400739,-39.8548713027024));
#248734=CARTESIAN_POINT('Ctrl Pts',(43.3525514979871,36.9944348238144,-39.8410580051271));
#248735=CARTESIAN_POINT('Ctrl Pts',(43.2986448352407,37.0043097240054,-39.8341090582382));
#248736=CARTESIAN_POINT('Ctrl Pts',(43.2441082468328,37.0112411932519,-39.8265155089204));
#248737=CARTESIAN_POINT('Ctrl Pts',(43.1889493654704,37.0152446912691,-39.8182791580079));
#248738=CARTESIAN_POINT('Origin',(43.8435011028032,36.3655255414403,-41.3499258784558));
#248739=CARTESIAN_POINT('Origin',(0.,-12.9675000200282,235.35105));
#248740=CARTESIAN_POINT('Origin',(0.,-12.9675000200281,-41.3499258784557));
#248741=CARTESIAN_POINT('Origin',(0.,-12.9675000200281,-52.64995));
#248742=CARTESIAN_POINT('Ctrl Pts',(51.204512585851,30.0888272971254,-41.2737227474219));
#248743=CARTESIAN_POINT('Ctrl Pts',(51.1918003817794,30.2706202849417,-40.0543903140502));
#248744=CARTESIAN_POINT('Ctrl Pts',(49.9827447112974,30.221449345442,-39.8182791580079));
#248745=CARTESIAN_POINT('Ctrl Pts',(51.1815637992349,30.4170102355187,-41.298307134608));
#248746=CARTESIAN_POINT('Ctrl Pts',(51.1511744833359,30.5669657276558,-40.0946602834914));
#248747=CARTESIAN_POINT('Ctrl Pts',(49.970795119399,30.3860867600489,-39.8428628946809));
#248748=CARTESIAN_POINT('Ctrl Pts',(51.1065500370229,30.7342489164072,-41.3171858838447));
#248749=CARTESIAN_POINT('Ctrl Pts',(51.0684082345096,30.8519555741622,-40.125362313696));
#248750=CARTESIAN_POINT('Ctrl Pts',(49.9327664722994,30.5453106517579,-39.8617422945218));
#248751=CARTESIAN_POINT('Ctrl Pts',(50.8500106529935,31.3458145441506,-41.3433504080566));
#248752=CARTESIAN_POINT('Ctrl Pts',(50.8167365053657,31.3985364985707,-40.1674712617341));
#248753=CARTESIAN_POINT('Ctrl Pts',(49.8033560611762,30.8523961753476,-39.8879068185516));
#248754=CARTESIAN_POINT('Ctrl Pts',(50.6751042513768,31.6239157533749,-41.3499258753262));
#248755=CARTESIAN_POINT('Ctrl Pts',(50.6540845266547,31.6475672688382,-40.1779974337035));
#248756=CARTESIAN_POINT('Ctrl Pts',(49.715313604986,30.9921150076825,-39.8944822858423));
#248757=CARTESIAN_POINT('Ctrl Pts',(50.4542306878656,31.8724442896568,-41.3499258784558));
#248758=CARTESIAN_POINT('Ctrl Pts',(50.4542306878656,31.8724442896567,-40.1779974386957));
#248759=CARTESIAN_POINT('Ctrl Pts',(49.6042696310026,31.1170625122411,-39.8944822890418));
#248760=CARTESIAN_POINT('',(49.6042696310026,31.1170625122412,-39.8944822890418));
#248761=CARTESIAN_POINT('Origin',(49.3330255614686,30.8760010827748,-41.3499258784557));
#248762=CARTESIAN_POINT('',(49.9827447112974,30.221449345442,-39.8182791580079));
#248763=CARTESIAN_POINT('Ctrl Pts',(49.9827447112974,30.221449345442,-39.8182791580079));
#248764=CARTESIAN_POINT('Ctrl Pts',(49.9742478426489,30.3385164122227,-39.8357596691874));
#248765=CARTESIAN_POINT('Ctrl Pts',(49.9525777122479,30.4527365881464,-39.850340487351));
#248766=CARTESIAN_POINT('Ctrl Pts',(49.917564983954,30.5640807882657,-39.8620074889831));
#248767=CARTESIAN_POINT('Ctrl Pts',(49.9032876571132,30.6094842062339,-39.8667650044259));
#248768=CARTESIAN_POINT('Ctrl Pts',(49.8867911421677,30.6544092836466,-39.8710378812991));
#248769=CARTESIAN_POINT('Ctrl Pts',(49.8680615705257,30.6988535344112,-39.8748246333721));
#248770=CARTESIAN_POINT('Ctrl Pts',(49.8680277409604,30.6989338101224,-39.8748314730468));
#248771=CARTESIAN_POINT('Ctrl Pts',(49.8679939050223,30.699014082039,-39.8748383109414));
#248772=CARTESIAN_POINT('Ctrl Pts',(49.8679600627116,30.6990943501611,-39.8748451470561));
#248773=CARTESIAN_POINT('Ctrl Pts',(49.834210673313,30.7791420788835,-39.8816624916982));
#248774=CARTESIAN_POINT('Ctrl Pts',(49.7941455915938,30.8553753559226,-39.8867070324262));
#248775=CARTESIAN_POINT('Ctrl Pts',(49.7477894766075,30.9277322498077,-39.8899765761449));
#248776=CARTESIAN_POINT('Ctrl Pts',(49.7052516615016,30.9941291895563,-39.8929768113077));
#248777=CARTESIAN_POINT('Ctrl Pts',(49.6574159846453,31.0572618495019,-39.8944822890418));
#248778=CARTESIAN_POINT('Ctrl Pts',(49.6042696310026,31.1170625122411,-39.8944822890418));
#248779=CARTESIAN_POINT('Origin',(49.7081665104613,29.9841925865092,-41.2737227474219));
#248780=CARTESIAN_POINT('Origin',(51.1341158175823,31.0955479856884,235.35105));
#248781=CARTESIAN_POINT('Ctrl Pts',(51.2045125858511,30.0888272971254,-41.2737227474219));
#248782=CARTESIAN_POINT('Ctrl Pts',(51.5939564242993,24.519520937744,-40.4393222961257));
#248783=CARTESIAN_POINT('Ctrl Pts',(51.9843680793961,18.9363741554737,-39.7153157040947));
#248784=CARTESIAN_POINT('Ctrl Pts',(52.3762811131638,13.3317566579059,-39.1625636424987));
#248785=CARTESIAN_POINT('',(51.1341158175823,31.0955479856884,-52.64995));
#248786=CARTESIAN_POINT('Ctrl Pts',(51.202570601752,13.3932250805846,-37.7071200530847));
#248787=CARTESIAN_POINT('Ctrl Pts',(52.3681090731164,13.4486222752606,-37.971813107807));
#248788=CARTESIAN_POINT('Ctrl Pts',(52.3762811131638,13.3317566579059,-39.1625636424987));
#248789=CARTESIAN_POINT('Ctrl Pts',(51.243814149994,12.8221846817494,-37.6510924855238));
#248790=CARTESIAN_POINT('Ctrl Pts',(52.3823956057955,13.0329073967221,-37.9286345805849));
#248791=CARTESIAN_POINT('Ctrl Pts',(52.4027610669746,12.9530756759645,-39.1065428641427));
#248792=CARTESIAN_POINT('Ctrl Pts',(51.3887400699185,12.2740430086498,-37.6224808645841));
#248793=CARTESIAN_POINT('Ctrl Pts',(52.4810099507979,12.6258889587099,-37.9059960140017));
#248794=CARTESIAN_POINT('Ctrl Pts',(52.4983460113501,12.5896787161743,-39.0779244541051));
#248795=CARTESIAN_POINT('Ctrl Pts',(51.6374655590603,11.7545242974889,-37.6224808631404));
#248796=CARTESIAN_POINT('Ctrl Pts',(52.6630979669895,12.2455574854105,-37.9059960127943));
#248797=CARTESIAN_POINT('Ctrl Pts',(52.6630979669895,12.2455574854105,-39.0779244525544));
#248798=CARTESIAN_POINT('',(51.202570601752,13.3932250805846,-37.7071200530847));
#248799=CARTESIAN_POINT('Origin',(50.8799350377741,13.2271219472897,-39.1625636424987));
#248800=CARTESIAN_POINT('',(51.6374655590603,11.7545242974889,-37.6224808631404));
#248801=CARTESIAN_POINT('Ctrl Pts',(51.6374655590603,11.7545242974889,-37.6224808631404));
#248802=CARTESIAN_POINT('Ctrl Pts',(51.5683401737289,11.8989080967521,-37.6224808635416));
#248803=CARTESIAN_POINT('Ctrl Pts',(51.5073117137531,12.0453267862124,-37.6246896514879));
#248804=CARTESIAN_POINT('Ctrl Pts',(51.4542914421325,12.1937580895562,-37.629072347155));
#248805=CARTESIAN_POINT('Ctrl Pts',(51.401143473863,12.3425468822047,-37.6334655983234));
#248806=CARTESIAN_POINT('Ctrl Pts',(51.3560423053796,12.4933581163808,-37.6400432640145));
#248807=CARTESIAN_POINT('Ctrl Pts',(51.3189474852192,12.6461827680851,-37.6487836824747));
#248808=CARTESIAN_POINT('Ctrl Pts',(51.2817682244751,12.7993553013199,-37.6575439971369));
#248809=CARTESIAN_POINT('Ctrl Pts',(51.2526317828013,12.9545505495523,-37.668476942121));
#248810=CARTESIAN_POINT('Ctrl Pts',(51.2315467536769,13.1117710662234,-37.6815739017301));
#248811=CARTESIAN_POINT('Ctrl Pts',(51.2190600923228,13.2048778548357,-37.6893299877397));
#248812=CARTESIAN_POINT('Ctrl Pts',(51.2093980530995,13.2986951308912,-37.6978452571967));
#248813=CARTESIAN_POINT('Ctrl Pts',(51.202570601752,13.3932250805846,-37.7071200530847));
#248814=CARTESIAN_POINT('Origin',(51.3101603185126,11.5978231885467,-39.0779244525544));
#248815=CARTESIAN_POINT('Origin',(0.,-12.9675000200281,-55.24995));
#248816=CARTESIAN_POINT('Origin',(0.,-12.9675000200281,-52.64995));
#248817=CARTESIAN_POINT('Origin',(0.,-12.9675000200281,-39.0779244525544));
#248818=CARTESIAN_POINT('Ctrl Pts',(51.6374655590602,-37.6895243375453,
-37.6224808631404));
#248819=CARTESIAN_POINT('Ctrl Pts',(52.6630979669894,-38.180557525467,-37.9059960127944));
#248820=CARTESIAN_POINT('Ctrl Pts',(52.6630979669894,-38.1805575254669,
-39.0779244525544));
#248821=CARTESIAN_POINT('Ctrl Pts',(51.3887400699171,-38.2090430487116,
-37.6224808645844));
#248822=CARTESIAN_POINT('Ctrl Pts',(52.4810099507953,-38.5608889987718,
-37.9059960140155));
#248823=CARTESIAN_POINT('Ctrl Pts',(52.4983460113489,-38.5246787562331,
-39.077924454111));
#248824=CARTESIAN_POINT('Ctrl Pts',(51.2438141500031,-38.7571847218022,
-37.6510924855255));
#248825=CARTESIAN_POINT('Ctrl Pts',(52.3823956058033,-38.9679074367732,
-37.9286345805868));
#248826=CARTESIAN_POINT('Ctrl Pts',(52.4027610669748,-38.8880757160172,
-39.1065428641511));
#248827=CARTESIAN_POINT('Ctrl Pts',(51.2025706017519,-39.328225120641,-37.7071200530847));
#248828=CARTESIAN_POINT('Ctrl Pts',(52.3681090731163,-39.383622315317,-37.971813107807));
#248829=CARTESIAN_POINT('Ctrl Pts',(52.3762811131638,-39.2667566979623,
-39.1625636424987));
#248830=CARTESIAN_POINT('',(51.6374655590602,-37.6895243375453,-37.6224808631404));
#248831=CARTESIAN_POINT('Origin',(51.3101603185125,-37.532823228603,-39.0779244525544));
#248832=CARTESIAN_POINT('',(51.2025706017519,-39.328225120641,-37.7071200530847));
#248833=CARTESIAN_POINT('Ctrl Pts',(51.2025706017519,-39.328225120641,-37.7071200530847));
#248834=CARTESIAN_POINT('Ctrl Pts',(51.2140977238333,-39.1686255548923,
-37.6914609587884));
#248835=CARTESIAN_POINT('Ctrl Pts',(51.2337022263897,-39.0110569630202,
-37.6779662189121));
#248836=CARTESIAN_POINT('Ctrl Pts',(51.2613462375948,-38.8555107743848,
-37.6666367940901));
#248837=CARTESIAN_POINT('Ctrl Pts',(51.2889523169909,-38.7001780188965,
-37.6553229149708));
#248838=CARTESIAN_POINT('Ctrl Pts',(51.3245758784465,-38.5468619993575,
-37.646168392601));
#248839=CARTESIAN_POINT('Ctrl Pts',(51.3682283722045,-38.3955646680986,
-37.6391871085577));
#248840=CARTESIAN_POINT('Ctrl Pts',(51.4117275642993,-38.2447986726358,
-37.6322303418412));
#248841=CARTESIAN_POINT('Ctrl Pts',(51.4631994205721,-38.0960370947074,
-37.6274315577981));
#248842=CARTESIAN_POINT('Ctrl Pts',(51.5227037486505,-37.9492940589207,
-37.6248176146113));
#248843=CARTESIAN_POINT('Ctrl Pts',(51.558106523932,-37.8619876244502,-37.6232624194478));
#248844=CARTESIAN_POINT('Ctrl Pts',(51.5963535473405,-37.7753959521341,
-37.6224808633791));
#248845=CARTESIAN_POINT('Ctrl Pts',(51.6374655590602,-37.6895243375453,
-37.6224808631404));
#248846=CARTESIAN_POINT('Origin',(50.879935037774,-39.1621219873461,-39.1625636424987));
#248847=CARTESIAN_POINT('Origin',(42.8470578959211,-61.1793204550998,235.35105));
#248848=CARTESIAN_POINT('',(44.8399443096849,-63.4217307078938,-41.3499258784557));
#248849=CARTESIAN_POINT('',(44.8399443096849,-63.4217307078937,-52.64995));
#248850=CARTESIAN_POINT('',(44.8399443096849,-63.4217307078938,235.35105));
#248851=CARTESIAN_POINT('',(43.0563273171535,-64.1720126058792,-41.273722747422));
#248852=CARTESIAN_POINT('Ctrl Pts',(44.8399443096849,-63.4217307078938,
-41.3499258784558));
#248853=CARTESIAN_POINT('Ctrl Pts',(44.7680634760552,-63.4856130133605,
-41.3499258784558));
#248854=CARTESIAN_POINT('Ctrl Pts',(44.6927093993648,-63.5463912211525,
-41.3493408309145));
#248855=CARTESIAN_POINT('Ctrl Pts',(44.6141372863133,-63.6036616909928,
-41.3481707358316));
#248856=CARTESIAN_POINT('Ctrl Pts',(44.5362131291965,-63.6604598718826,
-41.3470102901017));
#248857=CARTESIAN_POINT('Ctrl Pts',(44.4551238575238,-63.7138075633975,
-41.3452744063959));
#248858=CARTESIAN_POINT('Ctrl Pts',(44.3711666486527,-63.763327519689,-41.3429630847143));
#248859=CARTESIAN_POINT('Ctrl Pts',(44.287892099677,-63.8124448269568,-41.3406705564948));
#248860=CARTESIAN_POINT('Ctrl Pts',(44.2017961674148,-63.8577960340032,
-41.3378119100798));
#248861=CARTESIAN_POINT('Ctrl Pts',(44.1132152276405,-63.8990347068794,
-41.3343871454693));
#248862=CARTESIAN_POINT('Ctrl Pts',(44.0256970544502,-63.9397786109757,
-41.3310034701203));
#248863=CARTESIAN_POINT('Ctrl Pts',(43.9357533160473,-63.9765077468977,
-41.3270671793065));
#248864=CARTESIAN_POINT('Ctrl Pts',(43.8437517984982,-64.0089142889505,
-41.3225782730279));
#248865=CARTESIAN_POINT('Ctrl Pts',(43.752377649904,-64.0410998470569,-41.3181199771188));
#248866=CARTESIAN_POINT('Ctrl Pts',(43.6589738622758,-64.0690212328289,
-41.3131165767453));
#248867=CARTESIAN_POINT('Ctrl Pts',(43.5639413031887,-64.0924078517263,
-41.3075680719073));
#248868=CARTESIAN_POINT('Ctrl Pts',(43.4698946871375,-64.1155518393166,
-41.3020771316531));
#248869=CARTESIAN_POINT('Ctrl Pts',(43.3742531488302,-64.1342543800497,
-41.2960523389522));
#248870=CARTESIAN_POINT('Ctrl Pts',(43.2774420575633,-64.1482882005304,
-41.2894936938049));
#248871=CARTESIAN_POINT('Ctrl Pts',(43.2043379083053,-64.1588854419587,
-41.2845411189758));
#248872=CARTESIAN_POINT('Ctrl Pts',(43.1305676449252,-64.1668212164406,
-41.2792841368482));
#248873=CARTESIAN_POINT('Ctrl Pts',(43.0563273171535,-64.1720126058793,
-41.2737227474219));
#248874=CARTESIAN_POINT('',(43.0563273171535,-64.1720126058792,-52.64995));
#248875=CARTESIAN_POINT('',(43.0563273171535,-64.1720126058792,235.35105));
#248876=CARTESIAN_POINT('Origin',(42.8470578959211,-61.1793204550997,-52.64995));
#248877=CARTESIAN_POINT('Origin',(48.2118204350714,-55.8145579159494,235.35105));
#248878=CARTESIAN_POINT('',(51.2045125858509,-56.0238273371818,-41.2737227474219));
#248879=CARTESIAN_POINT('',(51.2045125858509,-56.0238273371818,-52.64995));
#248880=CARTESIAN_POINT('',(51.2045125858509,-56.0238273371818,235.35105));
#248881=CARTESIAN_POINT('',(50.4542306878654,-57.8074443297132,-41.3499258784557));
#248882=CARTESIAN_POINT('Ctrl Pts',(51.2045125858509,-56.0238273371818,
-41.2737227474219));
#248883=CARTESIAN_POINT('Ctrl Pts',(51.1976386505577,-56.1221291916803,
-41.2810866008773));
#248884=CARTESIAN_POINT('Ctrl Pts',(51.1859516555336,-56.2196057177593,
-41.2879167524659));
#248885=CARTESIAN_POINT('Ctrl Pts',(51.1696491164396,-56.3158058502849,
-41.2942132021878));
#248886=CARTESIAN_POINT('Ctrl Pts',(51.1532218742289,-56.4127418471005,
-41.3005578153829));
#248887=CARTESIAN_POINT('Ctrl Pts',(51.1321085028996,-56.5083816032577,
-41.3063605305851));
#248888=CARTESIAN_POINT('Ctrl Pts',(51.1065507692525,-56.602299175737,-41.3116213477945));
#248889=CARTESIAN_POINT('Ctrl Pts',(51.0807947759837,-56.6969452972597,
-41.3169229748677));
#248890=CARTESIAN_POINT('Ctrl Pts',(51.0505255204564,-56.7898422016671,
-41.3216742639821));
#248891=CARTESIAN_POINT('Ctrl Pts',(51.0160259163275,-56.8805933838835,
-41.3258752151377));
#248892=CARTESIAN_POINT('Ctrl Pts',(50.9810986445782,-56.9724695454474,
-41.3301282425657));
#248893=CARTESIAN_POINT('Ctrl Pts',(50.9418358149772,-57.0621462483671,
-41.3338172031508));
#248894=CARTESIAN_POINT('Ctrl Pts',(50.8985623695729,-57.149255551143,-41.336942096893));
#248895=CARTESIAN_POINT('Ctrl Pts',(50.854994800732,-57.2369569234258,-41.3400882300923));
#248896=CARTESIAN_POINT('Ctrl Pts',(50.8073622790973,-57.3220557483516,
-41.3426626026266));
#248897=CARTESIAN_POINT('Ctrl Pts',(50.7560227497974,-57.4042228434554,
-41.3446652144958));
#248898=CARTESIAN_POINT('Ctrl Pts',(50.7041097070974,-57.4873078264078,
-41.3466901975235));
#248899=CARTESIAN_POINT('Ctrl Pts',(50.6484067385514,-57.5673950913467,
-41.3481305742695));
#248900=CARTESIAN_POINT('Ctrl Pts',(50.5893052069323,-57.644193442378,-41.3489863447338));
#248901=CARTESIAN_POINT('Ctrl Pts',(50.546047593438,-57.7004037180663,-41.3496127005485));
#248902=CARTESIAN_POINT('Ctrl Pts',(50.5009698110338,-57.7548531291934,
-41.3499258784558));
#248903=CARTESIAN_POINT('Ctrl Pts',(50.4542306878654,-57.8074443297132,
-41.3499258784558));
#248904=CARTESIAN_POINT('',(50.4542306878654,-57.8074443297132,-52.64995));
#248905=CARTESIAN_POINT('',(50.4542306878654,-57.8074443297133,235.35105));
#248906=CARTESIAN_POINT('Origin',(48.2118204350714,-55.8145579159494,-52.64995));
#248907=CARTESIAN_POINT('Origin',(51.1341158175821,-57.030548025745,235.35105));
#248908=CARTESIAN_POINT('Ctrl Pts',(52.3762811131638,-39.2667566979623,
-39.1625636424987));
#248909=CARTESIAN_POINT('Ctrl Pts',(51.984368079396,-44.8713741955301,-39.7153157040947));
#248910=CARTESIAN_POINT('Ctrl Pts',(51.5939564242992,-50.4545209778004,
-40.4393222961257));
#248911=CARTESIAN_POINT('Ctrl Pts',(51.2045125858509,-56.0238273371818,
-41.2737227474219));
#248912=CARTESIAN_POINT('',(51.1341158175821,-57.0305480257449,-52.64995));
#248913=CARTESIAN_POINT('Ctrl Pts',(50.4542306878654,-57.8074443297132,
-41.3499258784558));
#248914=CARTESIAN_POINT('Ctrl Pts',(50.4542306878655,-57.8074443297132,
-40.1779974386957));
#248915=CARTESIAN_POINT('Ctrl Pts',(49.6042696310024,-57.0520625522976,
-39.8944822890418));
#248916=CARTESIAN_POINT('Ctrl Pts',(50.6752591020463,-57.5587415543343,
-41.3499258752894));
#248917=CARTESIAN_POINT('Ctrl Pts',(50.6542268000352,-57.5824072214955,
-40.177997433644));
#248918=CARTESIAN_POINT('Ctrl Pts',(49.7153914552119,-56.9270274498771,
-39.8944822858055));
#248919=CARTESIAN_POINT('Ctrl Pts',(50.8498163057994,-57.2811937413941,
-41.3433634048676));
#248920=CARTESIAN_POINT('Ctrl Pts',(50.8165517263607,-57.3338747062451,
-40.1674920635201));
#248921=CARTESIAN_POINT('Ctrl Pts',(49.8032581492502,-56.7875866525247,
-39.887919815423));
#248922=CARTESIAN_POINT('Ctrl Pts',(51.1065167165998,-56.6694124627357,
-41.3171961008675));
#248923=CARTESIAN_POINT('Ctrl Pts',(51.0683702519462,-56.7871016107072,
-40.125378843023));
#248924=CARTESIAN_POINT('Ctrl Pts',(49.9327495381902,-56.4803927424085,
-39.8617525114842));
#248925=CARTESIAN_POINT('Ctrl Pts',(51.1815671484691,-56.351962379293,-41.2983035466914));
#248926=CARTESIAN_POINT('Ctrl Pts',(51.1511803046297,-56.5019233058474,
-40.094654513445));
#248927=CARTESIAN_POINT('Ctrl Pts',(49.9707968538638,-56.3210629049775,
-39.8428593266729));
#248928=CARTESIAN_POINT('Ctrl Pts',(51.2045125858509,-56.0238273371818,
-41.2737227474219));
#248929=CARTESIAN_POINT('Ctrl Pts',(51.1918003817792,-56.2056203249981,
-40.0543903140502));
#248930=CARTESIAN_POINT('Ctrl Pts',(49.9827447112972,-56.1564493854985,
-39.8182791580079));
#248931=CARTESIAN_POINT('',(49.9827447112972,-56.1564493854985,-39.8182791580079));
#248932=CARTESIAN_POINT('Origin',(49.7081665104611,-55.9191926265656,-41.2737227474219));
#248933=CARTESIAN_POINT('',(49.6042696310024,-57.0520625522976,-39.8944822890418));
#248934=CARTESIAN_POINT('Ctrl Pts',(49.6042696310024,-57.0520625522976,
-39.8944822890418));
#248935=CARTESIAN_POINT('Ctrl Pts',(49.6845950444281,-56.9616798142842,
-39.8944822890418));
#248936=CARTESIAN_POINT('Ctrl Pts',(49.7527564873346,-56.8637901684971,
-39.8910542506064));
#248937=CARTESIAN_POINT('Ctrl Pts',(49.8088336114817,-56.7584432804741,
-39.8842118316772));
#248938=CARTESIAN_POINT('Ctrl Pts',(49.8302925387824,-56.7181303855846,
-39.8815934561347));
#248939=CARTESIAN_POINT('Ctrl Pts',(49.8499814505784,-56.6767252111676,
-39.878474969));
#248940=CARTESIAN_POINT('Ctrl Pts',(49.8679031420063,-56.6342295114207,
-39.8748566639276));
#248941=CARTESIAN_POINT('Ctrl Pts',(49.867936832891,-56.6341496239991,-39.8748498618967));
#248942=CARTESIAN_POINT('Ctrl Pts',(49.8679705175255,-56.6340697327332,
-39.8748430581001));
#248943=CARTESIAN_POINT('Ctrl Pts',(49.8680041959098,-56.6339898376229,
-39.8748362525379));
#248944=CARTESIAN_POINT('Ctrl Pts',(49.9110479907903,-56.5318771974589,
-39.8661381741537));
#248945=CARTESIAN_POINT('Ctrl Pts',(49.9423052598744,-56.4272085867056,
-39.8548713027844));
#248946=CARTESIAN_POINT('Ctrl Pts',(49.9619348436282,-56.3200515191852,
-39.8410580052779));
#248947=CARTESIAN_POINT('Ctrl Pts',(49.9718097439332,-56.266144856058,-39.8341090583481));
#248948=CARTESIAN_POINT('Ctrl Pts',(49.9787412132511,-56.21160826726,-39.82651550898));
#248949=CARTESIAN_POINT('Ctrl Pts',(49.9827447112972,-56.1564493854985,
-39.8182791580079));
#248950=CARTESIAN_POINT('Origin',(49.3330255614684,-56.8110011228313,-41.3499258784558));
#248951=CARTESIAN_POINT('Origin',(0.,-12.9675000200282,235.35105));
#248952=CARTESIAN_POINT('Origin',(0.,-12.9675000200281,-41.3499258784557));
#248953=CARTESIAN_POINT('Origin',(0.,-12.9675000200281,-52.64995));
#248954=CARTESIAN_POINT('Ctrl Pts',(43.0563273171535,-64.1720126058792,
-41.2737227474219));
#248955=CARTESIAN_POINT('Ctrl Pts',(43.2381203049698,-64.1593004018075,
-40.0543903140503));
#248956=CARTESIAN_POINT('Ctrl Pts',(43.1889493654702,-62.9502447313255,
-39.8182791580079));
#248957=CARTESIAN_POINT('Ctrl Pts',(43.3845102555472,-64.1490638192631,
-41.2983071346081));
#248958=CARTESIAN_POINT('Ctrl Pts',(43.5344657476846,-64.1186745033647,
-40.0946602834885));
#248959=CARTESIAN_POINT('Ctrl Pts',(43.3535867800773,-62.9382951394238,
-39.8428628946803));
#248960=CARTESIAN_POINT('Ctrl Pts',(43.7017489364349,-64.0740500570513,
-41.3171858838442));
#248961=CARTESIAN_POINT('Ctrl Pts',(43.8194555941901,-64.0359082545366,
-40.1253623136954));
#248962=CARTESIAN_POINT('Ctrl Pts',(43.5128106717856,-62.900266492328,-39.8617422945218));
#248963=CARTESIAN_POINT('Ctrl Pts',(44.3133145641792,-63.8175106730215,
-41.3433504080572));
#248964=CARTESIAN_POINT('Ctrl Pts',(44.3660365185992,-63.784236525395,-40.1674712617347));
#248965=CARTESIAN_POINT('Ctrl Pts',(43.8198961953762,-62.7708560812039,
-39.8879068185516));
#248966=CARTESIAN_POINT('Ctrl Pts',(44.5914157734028,-63.6426042714052,
-41.3499258753244));
#248967=CARTESIAN_POINT('Ctrl Pts',(44.6150672888642,-63.6215845466798,
-40.1779974336972));
#248968=CARTESIAN_POINT('Ctrl Pts',(43.9596150277081,-62.6828136250119,
-39.8944822858415));
#248969=CARTESIAN_POINT('Ctrl Pts',(44.8399443096849,-63.4217307078937,
-41.3499258784558));
#248970=CARTESIAN_POINT('Ctrl Pts',(44.8399443096849,-63.4217307078938,
-40.1779974386957));
#248971=CARTESIAN_POINT('Ctrl Pts',(44.0845625322693,-62.5717696510307,
-39.8944822890418));
#248972=CARTESIAN_POINT('',(44.0845625322693,-62.5717696510307,-39.8944822890418));
#248973=CARTESIAN_POINT('Origin',(43.843501102803,-62.3005255814968,-41.3499258784557));
#248974=CARTESIAN_POINT('',(43.1889493654702,-62.9502447313255,-39.8182791580079));
#248975=CARTESIAN_POINT('Ctrl Pts',(43.1889493654702,-62.9502447313255,
-39.8182791580079));
#248976=CARTESIAN_POINT('Ctrl Pts',(43.3060164327881,-62.941747862638,-39.8357596692677));
#248977=CARTESIAN_POINT('Ctrl Pts',(43.4202366092234,-62.9200777320771,
-39.8503404874849));
#248978=CARTESIAN_POINT('Ctrl Pts',(43.5315808098271,-62.8850650035,-39.8620074891438));
#248979=CARTESIAN_POINT('Ctrl Pts',(43.5769842272734,-62.8707876767699,
-39.8667650045221));
#248980=CARTESIAN_POINT('Ctrl Pts',(43.6219093041749,-62.854291161985,-39.8710378813417));
#248981=CARTESIAN_POINT('Ctrl Pts',(43.6663535544392,-62.8355615905537,
-39.8748246333721));
#248982=CARTESIAN_POINT('Ctrl Pts',(43.6664338301504,-62.8355277609884,
-39.8748314730468));
#248983=CARTESIAN_POINT('Ctrl Pts',(43.6665141020671,-62.8354939250504,
-39.8748383109414));
#248984=CARTESIAN_POINT('Ctrl Pts',(43.6665943701892,-62.8354600827397,
-39.8748451470561));
#248985=CARTESIAN_POINT('Ctrl Pts',(43.7466420990542,-62.8017106932808,
-39.8816624917103));
#248986=CARTESIAN_POINT('Ctrl Pts',(43.8228753762223,-62.7616456114792,
-39.8867070324441));
#248987=CARTESIAN_POINT('Ctrl Pts',(43.8952322702226,-62.7152894963879,
-39.8899765761624));
#248988=CARTESIAN_POINT('Ctrl Pts',(43.9616292098295,-62.672751681344,-39.8929768113136));
#248989=CARTESIAN_POINT('Ctrl Pts',(44.0247618696462,-62.6249160045702,
-39.8944822890418));
#248990=CARTESIAN_POINT('Ctrl Pts',(44.0845625322693,-62.5717696510307,
-39.8944822890418));
#248991=CARTESIAN_POINT('Origin',(42.9516926065373,-62.6756665304895,-41.2737227474219));
#248992=CARTESIAN_POINT('Origin',(44.0630480057166,-64.1016158376104,235.35105));
#248993=CARTESIAN_POINT('Ctrl Pts',(43.0563273171535,-64.1720126058792,
-41.273722747422));
#248994=CARTESIAN_POINT('Ctrl Pts',(37.4870209577721,-64.5614564443275,
-40.4393222961258));
#248995=CARTESIAN_POINT('Ctrl Pts',(31.9038741755017,-64.9518680994243,
-39.7153157040947));
#248996=CARTESIAN_POINT('Ctrl Pts',(26.299256677934,-65.343781133192,-39.1625636424987));
#248997=CARTESIAN_POINT('',(44.0630480057166,-64.1016158376104,-52.64995));
#248998=CARTESIAN_POINT('Ctrl Pts',(26.3607251006126,-64.1700706217802,
-37.7071200530847));
#248999=CARTESIAN_POINT('Ctrl Pts',(26.4161222952887,-65.3356090931445,
-37.971813107807));
#249000=CARTESIAN_POINT('Ctrl Pts',(26.299256677934,-65.343781133192,-39.1625636424987));
#249001=CARTESIAN_POINT('Ctrl Pts',(25.7896847017718,-64.2113141700146,
-37.6510924855215));
#249002=CARTESIAN_POINT('Ctrl Pts',(26.0004074167582,-65.3498956258269,
-37.9286345805828));
#249003=CARTESIAN_POINT('Ctrl Pts',(25.9205756959923,-65.3702610870028,
-39.1065428641436));
#249004=CARTESIAN_POINT('Ctrl Pts',(25.2415430286856,-64.3562400899596,
-37.6224808645879));
#249005=CARTESIAN_POINT('Ctrl Pts',(25.5933889787265,-65.4485099708125,
-37.9059960140076));
#249006=CARTESIAN_POINT('Ctrl Pts',(25.5571787362025,-65.4658460313782,
-39.0779244541051));
#249007=CARTESIAN_POINT('Ctrl Pts',(24.722024317517,-64.6049655790884,-37.6224808631404));
#249008=CARTESIAN_POINT('Ctrl Pts',(25.2130575054386,-65.6305979870177,
-37.9059960127943));
#249009=CARTESIAN_POINT('Ctrl Pts',(25.2130575054386,-65.6305979870176,
-39.0779244525544));
#249010=CARTESIAN_POINT('',(26.3607251006126,-64.1700706217802,-37.7071200530847));
#249011=CARTESIAN_POINT('Origin',(26.1946219673178,-63.8474350578023,-39.1625636424987));
#249012=CARTESIAN_POINT('',(24.722024317517,-64.6049655790884,-37.6224808631404));
#249013=CARTESIAN_POINT('Ctrl Pts',(24.722024317517,-64.6049655790884,-37.6224808631404));
#249014=CARTESIAN_POINT('Ctrl Pts',(24.8664081169227,-64.5358401936933,
-37.6224808635427));
#249015=CARTESIAN_POINT('Ctrl Pts',(25.0128268065285,-64.4748117336668,
-37.6246896514935));
#249016=CARTESIAN_POINT('Ctrl Pts',(25.1612581100212,-64.4217914620098,
-37.629072347169));
#249017=CARTESIAN_POINT('Ctrl Pts',(25.3100469028066,-64.3686434937081,
-37.6334655983456));
#249018=CARTESIAN_POINT('Ctrl Pts',(25.4608581371227,-64.3235423252056,
-37.6400432640483));
#249019=CARTESIAN_POINT('Ctrl Pts',(25.6136827889703,-64.2864475050405,
-37.648783682524));
#249020=CARTESIAN_POINT('Ctrl Pts',(25.7668553223293,-64.2492682442964,
-37.6575439972006));
#249021=CARTESIAN_POINT('Ctrl Pts',(25.9220505706891,-64.2201318026351,
-37.6684769422025));
#249022=CARTESIAN_POINT('Ctrl Pts',(26.0792710874908,-64.1990467735369,
-37.6815739018329));
#249023=CARTESIAN_POINT('Ctrl Pts',(26.1723778756961,-64.1865601122634,
-37.6893299878148));
#249024=CARTESIAN_POINT('Ctrl Pts',(26.2661951513385,-64.1768980730961,
-37.6978452572376));
#249025=CARTESIAN_POINT('Ctrl Pts',(26.3607251006126,-64.1700706217802,
-37.7071200530847));
#249026=CARTESIAN_POINT('Origin',(24.5653232085747,-64.2776603385407,-39.0779244525544));
#249027=CARTESIAN_POINT('Origin',(0.,-12.9675000200281,-55.24995));
#249028=CARTESIAN_POINT('Origin',(0.,-12.9675000200281,-39.0779244525544));
#249029=CARTESIAN_POINT('Origin',(0.,-12.9675000200281,-52.64995));
#249030=CARTESIAN_POINT('Origin',(0.,-12.9675000200281,-39.0779244525544));
#249031=CARTESIAN_POINT('Origin',(0.,-12.9675000200281,-37.6224808631404));
#249032=CARTESIAN_POINT('Origin',(0.,-12.9675000200281,-36.0027343734933));
#249033=CARTESIAN_POINT('Origin',(0.,-12.9675000200281,-36.9730300997693));
#249034=CARTESIAN_POINT('Origin',(0.,-12.9675000200281,-36.0027343734933));
#249035=CARTESIAN_POINT('Origin',(0.,-12.9675000200281,-28.64995));
#249036=CARTESIAN_POINT('Origin',(0.,-12.9675000200281,-28.64995));
#249037=CARTESIAN_POINT('Origin',(0.,-12.9675000200281,-39.0779244525544));
#249038=CARTESIAN_POINT('Origin',(0.,-12.9675000200281,-37.6224808631404));
#249039=CARTESIAN_POINT('Origin',(0.,-12.9675000200281,-39.0779244525544));
#249040=CARTESIAN_POINT('Origin',(0.,-12.9675000200281,-37.6224808631404));
#249041=CARTESIAN_POINT('Ctrl Pts',(43.1889493654702,-62.9502447313255,
-39.8182791580079));
#249042=CARTESIAN_POINT('Ctrl Pts',(43.2381203049698,-64.1593004018075,
-40.0543903140503));
#249043=CARTESIAN_POINT('Ctrl Pts',(43.0563273171535,-64.1720126058792,
-41.2737227474219));
#249044=CARTESIAN_POINT('Ctrl Pts',(37.601037205815,-63.3558221234085,-38.9838894046597));
#249045=CARTESIAN_POINT('Ctrl Pts',(37.6737894092837,-64.5483963219802,
-39.2334583931343));
#249046=CARTESIAN_POINT('Ctrl Pts',(37.4870588216962,-64.561453796624,-40.4393279688782));
#249047=CARTESIAN_POINT('Ctrl Pts',(31.9944550772227,-63.7631729893641,
-38.2598728770263));
#249048=CARTESIAN_POINT('Ctrl Pts',(32.0660652327991,-64.9405265958656,
-38.5181051330294));
#249049=CARTESIAN_POINT('Ctrl Pts',(31.9038355290703,-64.951870801846,-39.7153118927587));
#249050=CARTESIAN_POINT('Ctrl Pts',(26.3607251006126,-64.1700706217802,
-37.7071200530847));
#249051=CARTESIAN_POINT('Ctrl Pts',(26.4161222952887,-65.3356090931446,
-37.971813107807));
#249052=CARTESIAN_POINT('Ctrl Pts',(26.299256677934,-65.343781133192,-39.1625636424987));
#249053=CARTESIAN_POINT('Ctrl Pts',(26.3607251006126,-64.1700706217802,
-37.7071200530847));
#249054=CARTESIAN_POINT('Ctrl Pts',(27.4631807689973,-64.0904454705621,
-37.8152873750011));
#249055=CARTESIAN_POINT('Ctrl Pts',(28.5708560659873,-64.0103508505359,
-37.9306225804214));
#249056=CARTESIAN_POINT('Ctrl Pts',(29.6856323200486,-63.9296692017906,
-38.0531029163005));
#249057=CARTESIAN_POINT('Ctrl Pts',(30.7751530506771,-63.8508154151505,
-38.1728084307914));
#249058=CARTESIAN_POINT('Ctrl Pts',(31.8714564875302,-63.7714008635034,
-38.2993400360045));
#249059=CARTESIAN_POINT('Ctrl Pts',(32.9762913921302,-63.6913171853042,
-38.4327189046099));
#249060=CARTESIAN_POINT('Ctrl Pts',(33.5084198852201,-63.6527459862737,
-38.4969589970124));
#249061=CARTESIAN_POINT('Ctrl Pts',(34.0425273518562,-63.614019591588,-38.5627880146862));
#249062=CARTESIAN_POINT('Ctrl Pts',(34.5788086790266,-63.5751260489737,
-38.6302108770047));
#249063=CARTESIAN_POINT('Ctrl Pts',(36.1448893682756,-63.4615468081186,
-38.8271031373561));
#249064=CARTESIAN_POINT('Ctrl Pts',(37.7294988066828,-63.3465421354812,
-39.0375887447045));
#249065=CARTESIAN_POINT('Ctrl Pts',(39.3360623391576,-63.2299236849227,
-39.2616214281767));
#249066=CARTESIAN_POINT('Ctrl Pts',(40.6060743557284,-63.1377350907157,
-39.4387225476549));
#249067=CARTESIAN_POINT('Ctrl Pts',(41.889805634289,-63.0445381474314,-39.6242903860922));
#249068=CARTESIAN_POINT('Ctrl Pts',(43.1889493654701,-62.9502447313255,
-39.8182791580079));
#249069=CARTESIAN_POINT('Origin',(0.,-12.9675000200281,-41.3499258784557));
#249070=CARTESIAN_POINT('Origin',(0.,-12.9675000200281,-39.8944822890418));
#249071=CARTESIAN_POINT('Ctrl Pts',(51.2025706017519,-39.328225120641,-37.7071200530847));
#249072=CARTESIAN_POINT('Ctrl Pts',(52.3681090731163,-39.383622315317,-37.971813107807));
#249073=CARTESIAN_POINT('Ctrl Pts',(52.3762811131638,-39.2667566979623,
-39.1625636424987));
#249074=CARTESIAN_POINT('Ctrl Pts',(50.7956729692978,-44.9619550972486,
-38.2598728770176));
#249075=CARTESIAN_POINT('Ctrl Pts',(51.9730265758272,-45.0335652528346,
-38.518105133122));
#249076=CARTESIAN_POINT('Ctrl Pts',(51.9843707818182,-44.8713355490926,
-39.7153118927877));
#249077=CARTESIAN_POINT('Ctrl Pts',(50.3883221033785,-50.568537225844,-38.9838894046595));
#249078=CARTESIAN_POINT('Ctrl Pts',(51.5808963019407,-50.6412894292773,
-39.2334583932555));
#249079=CARTESIAN_POINT('Ctrl Pts',(51.593953776595,-50.4545588417343,-40.439327968821));
#249080=CARTESIAN_POINT('Ctrl Pts',(49.9827447112972,-56.1564493854985,
-39.8182791580079));
#249081=CARTESIAN_POINT('Ctrl Pts',(51.1918003817792,-56.2056203249982,
-40.0543903140503));
#249082=CARTESIAN_POINT('Ctrl Pts',(51.2045125858509,-56.0238273371818,
-41.2737227474219));
#249083=CARTESIAN_POINT('Ctrl Pts',(49.9827447112972,-56.1564493854985,
-39.8182791580079));
#249084=CARTESIAN_POINT('Ctrl Pts',(50.0911214886949,-54.6632697259096,
-39.5953168471712));
#249085=CARTESIAN_POINT('Ctrl Pts',(50.1980496341728,-53.1904501707553,
-39.383479797693));
#249086=CARTESIAN_POINT('Ctrl Pts',(50.3036634881978,-51.7354201301719,
-39.1828342154937));
#249087=CARTESIAN_POINT('Ctrl Pts',(50.3810449553401,-50.6693444688322,
-39.0358246240957));
#249088=CARTESIAN_POINT('Ctrl Pts',(50.4577210805591,-49.6128188084273,
-38.8948211810747));
#249089=CARTESIAN_POINT('Ctrl Pts',(50.53374730462,-48.5648325682818,-38.7598376298278));
#249090=CARTESIAN_POINT('Ctrl Pts',(50.5689702478275,-48.0793006314427,
-38.6972997618981));
#249091=CARTESIAN_POINT('Ctrl Pts',(50.6040535531298,-47.5956039481458,
-38.6360542494831));
#249092=CARTESIAN_POINT('Ctrl Pts',(50.6390034272056,-47.1136342590436,
-38.5761013219299));
#249093=CARTESIAN_POINT('Ctrl Pts',(50.7295722452733,-45.8646619453888,
-38.4207397954076));
#249094=CARTESIAN_POINT('Ctrl Pts',(50.8192477956374,-44.6272466675281,
-38.2740493733813));
#249095=CARTESIAN_POINT('Ctrl Pts',(50.9081832836966,-43.3989068589922,
-38.1359863030349));
#249096=CARTESIAN_POINT('Ctrl Pts',(50.9891192449324,-42.281053173163,-38.0103416638308));
#249097=CARTESIAN_POINT('Ctrl Pts',(51.0694423684864,-41.1707157672133,
-37.8918417736258));
#249098=CARTESIAN_POINT('Ctrl Pts',(51.149269876778,-40.0660162000401,-37.7804979349991));
#249099=CARTESIAN_POINT('Ctrl Pts',(51.1670609623838,-39.8198127923561,
-37.7556828329486));
#249100=CARTESIAN_POINT('Ctrl Pts',(51.1848274355191,-39.573889384857,-37.7312233765221));
#249101=CARTESIAN_POINT('Ctrl Pts',(51.2025706017519,-39.328225120641,-37.7071200530847));
#249102=CARTESIAN_POINT('Ctrl Pts',(49.9827447112974,30.221449345442,-39.8182791580079));
#249103=CARTESIAN_POINT('Ctrl Pts',(51.1918003817794,30.2706202849417,-40.0543903140502));
#249104=CARTESIAN_POINT('Ctrl Pts',(51.2045125858511,30.0888272971254,-41.2737227474219));
#249105=CARTESIAN_POINT('Ctrl Pts',(50.3883221033964,24.6335371857877,-38.9838894046629));
#249106=CARTESIAN_POINT('Ctrl Pts',(51.5808963020367,24.7062893892444,-39.233458393181));
#249107=CARTESIAN_POINT('Ctrl Pts',(51.5939537765951,24.5195588016784,-40.4393279688242));
#249108=CARTESIAN_POINT('Ctrl Pts',(50.7956729693229,19.0269550571941,-38.2598728770233));
#249109=CARTESIAN_POINT('Ctrl Pts',(51.9730265758558,19.098565212774,-38.5181051331097));
#249110=CARTESIAN_POINT('Ctrl Pts',(51.9843707818182,18.9363355090369,-39.7153118927739));
#249111=CARTESIAN_POINT('Ctrl Pts',(51.202570601752,13.3932250805846,-37.7071200530847));
#249112=CARTESIAN_POINT('Ctrl Pts',(52.3681090731165,13.4486222752606,-37.971813107807));
#249113=CARTESIAN_POINT('Ctrl Pts',(52.3762811131638,13.3317566579059,-39.1625636424987));
#249114=CARTESIAN_POINT('Ctrl Pts',(51.202570601752,13.3932250805846,-37.7071200530847));
#249115=CARTESIAN_POINT('Ctrl Pts',(51.122945450528,14.4956807490165,-37.8152873750052));
#249116=CARTESIAN_POINT('Ctrl Pts',(51.0428508304973,15.6033560460543,-37.9306225804305));
#249117=CARTESIAN_POINT('Ctrl Pts',(50.9621691817486,16.7181323001641,-38.0531029163155));
#249118=CARTESIAN_POINT('Ctrl Pts',(50.8833153951093,17.8076530307813,-38.1728084308057));
#249119=CARTESIAN_POINT('Ctrl Pts',(50.803900843464,18.903956467623,-38.2993400360181));
#249120=CARTESIAN_POINT('Ctrl Pts',(50.723817165267,20.0087913722114,-38.4327189046227));
#249121=CARTESIAN_POINT('Ctrl Pts',(50.6852459662377,20.540919865293,-38.4969589970245));
#249122=CARTESIAN_POINT('Ctrl Pts',(50.6465195715533,21.0750273319207,-38.5627880146976));
#249123=CARTESIAN_POINT('Ctrl Pts',(50.6076260289403,21.6113086590827,-38.6302108770153));
#249124=CARTESIAN_POINT('Ctrl Pts',(50.4940467880895,23.1773893483014,-38.8271031373637));
#249125=CARTESIAN_POINT('Ctrl Pts',(50.3790421154564,24.7619987866776,-39.0375887447086));
#249126=CARTESIAN_POINT('Ctrl Pts',(50.2624236649002,26.3685623191205,-39.2616214281763));
#249127=CARTESIAN_POINT('Ctrl Pts',(50.170235070693,27.6385743356943,-39.438722547655));
#249128=CARTESIAN_POINT('Ctrl Pts',(50.0770381274072,28.9223056142579,-39.6242903860925));
#249129=CARTESIAN_POINT('Ctrl Pts',(49.9827447112974,30.221449345442,-39.8182791580079));
#249130=CARTESIAN_POINT('Origin',(0.,-12.9675000200281,-41.3499258784557));
#249131=CARTESIAN_POINT('Origin',(0.,-12.9675000200281,-39.8944822890418));
#249132=CARTESIAN_POINT('Ctrl Pts',(26.3607251006129,38.2350705817238,-37.7071200530847));
#249133=CARTESIAN_POINT('Ctrl Pts',(26.4161222952889,39.4006090530882,-37.971813107807));
#249134=CARTESIAN_POINT('Ctrl Pts',(26.2992566779342,39.4087810931356,-39.1625636424987));
#249135=CARTESIAN_POINT('Ctrl Pts',(31.994455077222,37.8281729492938,-38.2598728770231));
#249136=CARTESIAN_POINT('Ctrl Pts',(32.0660652328021,39.0055265558251,-38.5181051330933));
#249137=CARTESIAN_POINT('Ctrl Pts',(31.9038355290649,39.01687076179,-39.7153118927753));
#249138=CARTESIAN_POINT('Ctrl Pts',(37.6010372058154,37.4208220833505,-38.9838894046594));
#249139=CARTESIAN_POINT('Ctrl Pts',(37.6737894092744,38.6133962819915,-39.2334583931755));
#249140=CARTESIAN_POINT('Ctrl Pts',(37.4870588217073,38.6264537565668,-40.4393279688211));
#249141=CARTESIAN_POINT('Ctrl Pts',(43.1889493654704,37.015244691269,-39.8182791580079));
#249142=CARTESIAN_POINT('Ctrl Pts',(43.23812030497,38.224300361751,-40.0543903140502));
#249143=CARTESIAN_POINT('Ctrl Pts',(43.0563273171537,38.2370125658228,-41.2737227474219));
#249144=CARTESIAN_POINT('Ctrl Pts',(43.1889493654704,37.015244691269,-39.8182791580079));
#249145=CARTESIAN_POINT('Ctrl Pts',(41.6957697057964,37.123621468673,-39.5953168471585));
#249146=CARTESIAN_POINT('Ctrl Pts',(40.2229501505596,37.2305496141585,-39.3834797976693));
#249147=CARTESIAN_POINT('Ctrl Pts',(38.7679201098954,37.3361634681915,-39.1828342154603));
#249148=CARTESIAN_POINT('Ctrl Pts',(37.701844448578,37.4135449353336,-39.0358246240664));
#249149=CARTESIAN_POINT('Ctrl Pts',(36.6453187881949,37.4902210605526,-38.8948211810493));
#249150=CARTESIAN_POINT('Ctrl Pts',(35.5973325480708,37.5662472846133,-38.759837629806));
#249151=CARTESIAN_POINT('Ctrl Pts',(35.1118006112682,37.6014702278188,-38.6972997618815));
#249152=CARTESIAN_POINT('Ctrl Pts',(34.6281039280075,37.636553533119,-38.6360542494713));
#249153=CARTESIAN_POINT('Ctrl Pts',(34.1461342389413,37.6715034071926,-38.5761013219228));
#249154=CARTESIAN_POINT('Ctrl Pts',(32.897161925551,37.762072225242,-38.4207397954338));
#249155=CARTESIAN_POINT('Ctrl Pts',(31.6597466479497,37.8517477755866,-38.274049373437));
#249156=CARTESIAN_POINT('Ctrl Pts',(30.4314068396699,37.9406832636257,-38.1359863031161));
#249157=CARTESIAN_POINT('Ctrl Pts',(29.3135531539302,38.0216192248535,-38.010341663919));
#249158=CARTESIAN_POINT('Ctrl Pts',(28.2032157480691,38.1019423483989,-37.8918417737198));
#249159=CARTESIAN_POINT('Ctrl Pts',(27.098516180984,38.1817698566814,-37.7804979350974));
#249160=CARTESIAN_POINT('Ctrl Pts',(26.8523127729753,38.1995609423102,-37.7556828330132));
#249161=CARTESIAN_POINT('Ctrl Pts',(26.6063893651522,38.2173274154682,-37.731223376554));
#249162=CARTESIAN_POINT('Ctrl Pts',(26.3607251006129,38.2350705817238,-37.7071200530847));
#249163=CARTESIAN_POINT('Origin',(-55.3689732639432,-39.4760261191947,-55.24995));
#249164=CARTESIAN_POINT('',(-52.6630979669894,-38.1805575254669,-52.64995));
#249165=CARTESIAN_POINT('',(-52.6630979669894,-38.1805575254669,-55.24995));
#249166=CARTESIAN_POINT('Origin',(-55.3689732639432,-39.4760261191947,-52.64995));
#249167=CARTESIAN_POINT('Origin',(0.,-12.9675000200281,-55.24995));
#249168=CARTESIAN_POINT('Origin',(0.,-12.9675000200281,-39.0779244525544));
#249169=CARTESIAN_POINT('Origin',(0.,-12.9675000200281,-52.64995));
#249170=CARTESIAN_POINT('Origin',(0.,-12.9675000200281,-39.0779244525544));
#249171=CARTESIAN_POINT('Origin',(0.,-12.9675000200281,-37.6224808631404));
#249172=CARTESIAN_POINT('Ctrl Pts',(-52.1419834946474,-42.6173687451066,
-39.5132811674967));
#249173=CARTESIAN_POINT('Ctrl Pts',(-52.1327810050217,-42.7489704779756,
-38.3173126020845));
#249174=CARTESIAN_POINT('Ctrl Pts',(-50.9590827221993,-42.6955891686747,
-38.0578375780827));
#249175=CARTESIAN_POINT('Ctrl Pts',(-51.8286928526804,-47.0976336572277,
-40.0086902420288));
#249176=CARTESIAN_POINT('Ctrl Pts',(-51.817197900376,-47.2620191329047,
-38.806978691719));
#249177=CARTESIAN_POINT('Ctrl Pts',(-50.6332299575652,-47.1974014010278,
-38.5532483700491));
#249178=CARTESIAN_POINT('Ctrl Pts',(-51.5162900940338,-51.5652012463084,
-40.6057258043764));
#249179=CARTESIAN_POINT('Ctrl Pts',(-51.5035559922642,-51.7473073860814,
-39.3966344269474));
#249180=CARTESIAN_POINT('Ctrl Pts',(-50.307441595963,-51.6828823044661,
-39.1502839521633));
#249181=CARTESIAN_POINT('Ctrl Pts',(-51.2045125858509,-56.0238273371818,
-41.2737227474219));
#249182=CARTESIAN_POINT('Ctrl Pts',(-51.1918003817792,-56.2056203249982,
-40.0543903140503));
#249183=CARTESIAN_POINT('Ctrl Pts',(-49.9827447112972,-56.1564493854985,
-39.8182791580079));
#249184=CARTESIAN_POINT('Ctrl Pts',(-49.9827447112972,-56.1564493854985,
-39.8182791580079));
#249185=CARTESIAN_POINT('Ctrl Pts',(-50.2766098672488,-52.1076717408327,
-39.2137137167888));
#249186=CARTESIAN_POINT('Ctrl Pts',(-50.5713690581735,-48.0491354164006,
-38.6672717073897));
#249187=CARTESIAN_POINT('Ctrl Pts',(-50.8662592829545,-43.9775643489176,
-38.2016959289247));
#249188=CARTESIAN_POINT('Ctrl Pts',(46.6981266849492,30.7091523375488,-39.2904704603133));
#249189=CARTESIAN_POINT('Ctrl Pts',(46.6689684123063,30.6404043382273,-39.273452295095));
#249190=CARTESIAN_POINT('Ctrl Pts',(46.6043681216411,30.5066861069553,-39.238925705885));
#249191=CARTESIAN_POINT('Ctrl Pts',(46.5083209189471,30.3487389562033,-39.1945593129175));
#249192=CARTESIAN_POINT('Ctrl Pts',(46.4437937583117,30.2581216171786,-39.1673894861782));
#249193=CARTESIAN_POINT('Ctrl Pts',(46.3992224148768,30.1986447451181,-39.1491520227249));
#249194=CARTESIAN_POINT('Ctrl Pts',(46.3761748773305,30.1693908446446,-39.1399767764946));
#249195=CARTESIAN_POINT('Ctrl Pts',(46.3284414024809,30.1117648114071,-39.1214771434543));
#249196=CARTESIAN_POINT('Ctrl Pts',(46.3038983378397,30.083571828401,-39.112209259666));
#249197=CARTESIAN_POINT('Ctrl Pts',(46.253707387608,30.0286632749651,-39.0937226519629));
#249198=CARTESIAN_POINT('Ctrl Pts',(46.2280147026909,30.001893564456,-39.0844865568113));
#249199=CARTESIAN_POINT('Ctrl Pts',(46.1492148010453,29.9236586721517,-39.0568159196779));
#249200=CARTESIAN_POINT('Ctrl Pts',(46.0669347173688,29.8495134741745,-39.0292038481275));
#249201=CARTESIAN_POINT('Ctrl Pts',(45.9503410384262,29.7587889734315,-38.9925114043613));
#249202=CARTESIAN_POINT('Ctrl Pts',(45.8594191065401,29.6948377475824,-38.9650526418885));
#249203=CARTESIAN_POINT('Ctrl Pts',(45.7964751089327,29.6549785818455,-38.9467936623891));
#249204=CARTESIAN_POINT('Ctrl Pts',(45.748348603817,29.6261284949947,-38.9331097524421));
#249205=CARTESIAN_POINT('Ctrl Pts',(45.7321473284057,29.616684052073,-38.9285487676403));
#249206=CARTESIAN_POINT('Ctrl Pts',(45.6996106203311,29.5982459977232,-38.9194791520014));
#249207=CARTESIAN_POINT('Ctrl Pts',(45.683249044345,29.5892352448745,-38.9149628379356));
#249208=CARTESIAN_POINT('Ctrl Pts',(45.6010439155842,29.5452684013657,-38.8924942188443));
#249209=CARTESIAN_POINT('Ctrl Pts',(45.4667739830181,29.4816584171599,-38.8571935516581));
#249210=CARTESIAN_POINT('Ctrl Pts',(45.2922645146651,29.4187721922835,-38.8147007629208));
#249211=CARTESIAN_POINT('Ctrl Pts',(45.184512437616,29.3885937253944,-38.7899522655792));
#249212=CARTESIAN_POINT('Ctrl Pts',(45.1119891467798,29.3701842541612,-38.7736235920333));
#249213=CARTESIAN_POINT('Ctrl Pts',(45.0754052578815,29.3618381514785,-38.7655490803555));
#249214=CARTESIAN_POINT('Ctrl Pts',(45.0014447932705,29.3468760834356,-38.7495561846596));
#249215=CARTESIAN_POINT('Ctrl Pts',(44.964301863367,29.3403115562353,-38.7416890516424));
#249216=CARTESIAN_POINT('Ctrl Pts',(44.8900079594565,29.3290481892184,-38.726277749838));
#249217=CARTESIAN_POINT('Ctrl Pts',(44.8527936282157,29.324336495618,-38.7187198739728));
#249218=CARTESIAN_POINT('Ctrl Pts',(44.7410083373266,29.3129455735289,-38.6964994820139));
#249219=CARTESIAN_POINT('Ctrl Pts',(44.6662563757167,29.3089967422249,-38.6822807693139));
#249220=CARTESIAN_POINT('Ctrl Pts',(44.516312468428,29.3084067934202,-38.6550493453909));
#249221=CARTESIAN_POINT('Ctrl Pts',(44.441103189525,29.3117700143417,-38.6420342479066));
#249222=CARTESIAN_POINT('Ctrl Pts',(44.3468378615956,29.3206690055189,-38.6265520162729));
#249223=CARTESIAN_POINT('Ctrl Pts',(44.3279589148655,29.3226883315868,-38.6234933649988));
#249224=CARTESIAN_POINT('Ctrl Pts',(44.2901960653062,29.3271995080042,-38.6174591262491));
#249225=CARTESIAN_POINT('Ctrl Pts',(44.271274393292,29.329697893027,-38.614477863833));
#249226=CARTESIAN_POINT('Ctrl Pts',(44.2146592782019,29.3378915995821,-38.60568558559));
#249227=CARTESIAN_POINT('Ctrl Pts',(44.1772069502033,29.344266758826,-38.6000392683017));
#249228=CARTESIAN_POINT('Ctrl Pts',(44.0655444875092,29.3661148598052,-38.5837127379559));
#249229=CARTESIAN_POINT('Ctrl Pts',(43.9553791862171,29.3933792052515,-38.5686255047386));
#249230=CARTESIAN_POINT('Ctrl Pts',(43.8114622524781,29.4404829778103,-38.5509833019505));
#249231=CARTESIAN_POINT('Ctrl Pts',(43.705021834675,29.481230340464,-38.5390021142185));
#249232=CARTESIAN_POINT('Ctrl Pts',(43.6350719757086,29.512061063653,-38.5318621614261));
#249233=CARTESIAN_POINT('Ctrl Pts',(43.5656410085295,29.5447591316771,-38.525155654825));
#249234=CARTESIAN_POINT('Ctrl Pts',(43.5311320054746,29.5620794464364,-38.5220163122062));
#249235=CARTESIAN_POINT('Ctrl Pts',(43.4634866412134,29.5981758355574,-38.5162526847879));
#249236=CARTESIAN_POINT('Ctrl Pts',(43.4301834663392,29.6170276546,-38.5136117755133));
#249237=CARTESIAN_POINT('Ctrl Pts',(43.3647025891651,29.6562685687332,-38.5088155315793));
#249238=CARTESIAN_POINT('Ctrl Pts',(43.2681192378476,29.7174608121974,-38.5023448938576));
#249239=CARTESIAN_POINT('Ctrl Pts',(43.1764049274077,29.7855824582168,-38.4980286134812));
#249240=CARTESIAN_POINT('Ctrl Pts',(43.0584774180437,29.8826126224142,-38.4942050936184));
#249241=CARTESIAN_POINT('Ctrl Pts',(43.001681818637,29.9342392650769,-38.4932590761897));
#249242=CARTESIAN_POINT('Ctrl Pts',(42.8926599718677,30.0438904492243,-38.4933742455196));
#249243=CARTESIAN_POINT('Ctrl Pts',(42.8414047150844,30.1009342501745,-38.4944336470273));
#249244=CARTESIAN_POINT('Ctrl Pts',(42.7451036203247,30.2193471227021,-38.498479276642));
#249245=CARTESIAN_POINT('Ctrl Pts',(42.6550322643363,30.3420646399833,-38.5044516702661));
#249246=CARTESIAN_POINT('Ctrl Pts',(42.5773225406025,30.4733365238586,-38.5142428327574));
#249247=CARTESIAN_POINT('Ctrl Pts',(42.5326943378214,30.5580963840027,-38.5215739479982));
#249248=CARTESIAN_POINT('Ctrl Pts',(42.5239673850246,30.5751883092729,-38.5231018165939));
#249249=CARTESIAN_POINT('Ctrl Pts',(42.5069121510755,30.60964376351,-38.5262794637242));
#249250=CARTESIAN_POINT('Ctrl Pts',(42.4985805781952,30.627019094627,-38.5279307934181));
#249251=CARTESIAN_POINT('Ctrl Pts',(42.4743295471271,30.6792614198295,-38.5330409224498));
#249252=CARTESIAN_POINT('Ctrl Pts',(42.4438856226513,30.7493896366731,-38.5402834483744));
#249253=CARTESIAN_POINT('Ctrl Pts',(42.4037483179465,30.8560072598611,-38.5524071291592));
#249254=CARTESIAN_POINT('Ctrl Pts',(42.3690543371876,30.9640160484273,-38.5657659376104));
#249255=CARTESIAN_POINT('Ctrl Pts',(42.3397558527982,31.0734075527136,-38.5803463747351));
#249256=CARTESIAN_POINT('Ctrl Pts',(42.3238156343608,31.1472555030051,-38.5908775753381));
#249257=CARTESIAN_POINT('Ctrl Pts',(42.3096820427396,31.2215665449467,-38.6018154236264));
#249258=CARTESIAN_POINT('Ctrl Pts',(42.3035171869091,31.2589715314082,-38.6074906718877));
#249259=CARTESIAN_POINT('Ctrl Pts',(42.2930235524414,31.3341791410138,-38.6192399292287));
#249260=CARTESIAN_POINT('Ctrl Pts',(42.2886818075092,31.3721585359098,-38.6253436316658));
#249261=CARTESIAN_POINT('Ctrl Pts',(42.281930630611,31.4478003630713,-38.6378362101326));
#249262=CARTESIAN_POINT('Ctrl Pts',(42.277074994566,31.5232809912004,-38.6506356205751));
#249263=CARTESIAN_POINT('Ctrl Pts',(42.2747992363309,31.6735553614761,-38.6774229397946));
#249264=CARTESIAN_POINT('Ctrl Pts',(42.2834818483937,31.8228397562226,-38.7059581415094));
#249265=CARTESIAN_POINT('Ctrl Pts',(42.3030248127084,31.9711385758679,-38.7362097844166));
#249266=CARTESIAN_POINT('Ctrl Pts',(42.3164494406915,32.0449687602614,-38.7519128032936));
#249267=CARTESIAN_POINT('Ctrl Pts',(42.3317154579634,32.1186122141692,-38.7679009120377));
#249268=CARTESIAN_POINT('Ctrl Pts',(42.3402956643805,32.1554227583218,-38.7760569897633));
#249269=CARTESIAN_POINT('Ctrl Pts',(42.3591481714288,32.228169160774,-38.7925026060078));
#249270=CARTESIAN_POINT('Ctrl Pts',(42.3694448348212,32.2642362896146,-38.8008201507359));
#249271=CARTESIAN_POINT('Ctrl Pts',(42.4028917825415,32.3714169561226,-38.8260275044574));
#249272=CARTESIAN_POINT('Ctrl Pts',(42.428602574983,32.4415633880281,-38.8431823298655));
#249273=CARTESIAN_POINT('Ctrl Pts',(42.4722685042023,32.5448307979217,-38.8694323201497));
#249274=CARTESIAN_POINT('Ctrl Pts',(42.4876674804306,32.5789105800712,-38.8782643966373));
#249275=CARTESIAN_POINT('Ctrl Pts',(42.5202146590728,32.6464795812123,-38.8961197808447));
#249276=CARTESIAN_POINT('Ctrl Pts',(42.5373018269229,32.6798350022668,-38.9051083126545));
#249277=CARTESIAN_POINT('Ctrl Pts',(42.5906929412925,32.7780783962456,-38.9321048428364));
#249278=CARTESIAN_POINT('Ctrl Pts',(42.629225789877,32.8414173722334,-38.9502105255135));
#249279=CARTESIAN_POINT('Ctrl Pts',(42.7120000069194,32.9638220552461,-38.9866125955294));
#249280=CARTESIAN_POINT('Ctrl Pts',(42.7783647966162,33.0524402968179,-39.0140612314234));
#249281=CARTESIAN_POINT('Ctrl Pts',(42.8754380724448,33.1642175243331,-39.0509520337677));
#249282=CARTESIAN_POINT('Ctrl Pts',(42.9268673384212,33.2179450225078,-39.0694937486382));
#249283=CARTESIAN_POINT('Ctrl Pts',(42.9797817061918,33.2705900457306,-39.088089881442));
#249284=CARTESIAN_POINT('Ctrl Pts',(43.0069972096607,33.2963736994336,-39.097418269769));
#249285=CARTESIAN_POINT('Ctrl Pts',(43.0622936398443,33.3462615369726,-39.1159154063528));
#249286=CARTESIAN_POINT('Ctrl Pts',(43.0904949946047,33.3704876748183,-39.1251268688783));
#249287=CARTESIAN_POINT('Ctrl Pts',(43.176562606447,33.4408730143712,-39.1525915568785));
#249288=CARTESIAN_POINT('Ctrl Pts',(43.2360245534179,33.4848790444095,-39.1707230137558));
#249289=CARTESIAN_POINT('Ctrl Pts',(43.358992255749,33.5670176609587,-39.2066046432507));
#249290=CARTESIAN_POINT('Ctrl Pts',(43.4542745623933,33.6242424638975,-39.233238623837));
#249291=CARTESIAN_POINT('Ctrl Pts',(43.5542222374601,33.6747516510336,-39.2594493821381));
#249292=CARTESIAN_POINT('Ctrl Pts',(43.6219256430316,33.7069073870393,-39.2768314299875));
#249293=CARTESIAN_POINT('Ctrl Pts',(43.6563381479934,33.7222286468184,-39.2854811722856));
#249294=CARTESIAN_POINT('Ctrl Pts',(43.7254519170511,33.7509934760635,-39.3024907499371));
#249295=CARTESIAN_POINT('Ctrl Pts',(43.7602995448845,33.7645084608315,-39.3108885064059));
#249296=CARTESIAN_POINT('Ctrl Pts',(43.8304781084082,33.789780836939,-39.3274499785309));
#249297=CARTESIAN_POINT('Ctrl Pts',(43.9365171946568,33.8250735562425,-39.3519527568515));
#249298=CARTESIAN_POINT('Ctrl Pts',(44.0809642638621,33.8617420360433,-39.3832806139221));
#249299=CARTESIAN_POINT('Ctrl Pts',(44.1916183723467,33.8813683146414,-39.4057679385072));
#249300=CARTESIAN_POINT('Ctrl Pts',(44.2659122959159,33.8926702964892,-39.4205323411483));
#249301=CARTESIAN_POINT('Ctrl Pts',(44.3033049221432,33.8974288658374,-39.4277978831022));
#249302=CARTESIAN_POINT('Ctrl Pts',(44.3598453576919,33.9032050944765,-39.4385322478049));
#249303=CARTESIAN_POINT('Ctrl Pts',(44.3787527158677,33.9049006163346,-39.4420799976889));
#249304=CARTESIAN_POINT('Ctrl Pts',(44.4164967874688,33.9078161173588,-39.4490791780208));
#249305=CARTESIAN_POINT('Ctrl Pts',(44.4353708468856,33.9090400957878,-39.4525377314439));
#249306=CARTESIAN_POINT('Ctrl Pts',(44.4919347179527,33.9120095261765,-39.462779235967));
#249307=CARTESIAN_POINT('Ctrl Pts',(44.52962054914,33.9130584408517,-39.4694384189012));
#249308=CARTESIAN_POINT('Ctrl Pts',(44.6425299001817,33.9134342925821,-39.4889026473125));
#249309=CARTESIAN_POINT('Ctrl Pts',(44.7176656228988,33.9100023852834,-39.5012068570978));
#249310=CARTESIAN_POINT('Ctrl Pts',(44.867623327666,33.8957625538083,-39.524471978366));
#249311=CARTESIAN_POINT('Ctrl Pts',(44.9424659600731,33.8849485744664,-39.5354353652432));
#249312=CARTESIAN_POINT('Ctrl Pts',(45.0357885152669,33.8666999843662,-39.5482785606344));
#249313=CARTESIAN_POINT('Ctrl Pts',(45.0544546343785,33.8628074782943,-39.5508053225112));
#249314=CARTESIAN_POINT('Ctrl Pts',(45.091743102575,33.8545484160302,-39.5557691634051));
#249315=CARTESIAN_POINT('Ctrl Pts',(45.1104022544846,33.850171655015,-39.5582107864407));
#249316=CARTESIAN_POINT('Ctrl Pts',(45.1661672125598,33.8363538303533,-39.5653802281989));
#249317=CARTESIAN_POINT('Ctrl Pts',(45.2029511118778,33.8262578362557,-39.5699395109212));
#249318=CARTESIAN_POINT('Ctrl Pts',(45.312316831343,33.7933159380614,-39.582990524906));
#249319=CARTESIAN_POINT('Ctrl Pts',(45.4195983160475,33.7551076509549,-39.5947758536238));
#249320=CARTESIAN_POINT('Ctrl Pts',(45.5585113890164,33.6937328563153,-39.6079933748399));
#249321=CARTESIAN_POINT('Ctrl Pts',(45.6606150024606,33.6424505696195,-39.6166516297843));
#249322=CARTESIAN_POINT('Ctrl Pts',(45.7272860947277,33.6047101271221,-39.6215780075552));
#249323=CARTESIAN_POINT('Ctrl Pts',(45.7932287365117,33.5651705839516,-39.6260731428005));
#249324=CARTESIAN_POINT('Ctrl Pts',(45.8259059249178,33.5444453395394,-39.6281074988013));
#249325=CARTESIAN_POINT('Ctrl Pts',(45.8897275017006,33.5016881508368,-39.6316923737189));
#249326=CARTESIAN_POINT('Ctrl Pts',(45.9210297733036,33.4795651380848,-39.6332542688506));
#249327=CARTESIAN_POINT('Ctrl Pts',(45.9823424846244,33.4339088874735,-39.6359180193303));
#249328=CARTESIAN_POINT('Ctrl Pts',(46.0724202597563,33.3632801300718,-39.6392265347984));
#249329=CARTESIAN_POINT('Ctrl Pts',(46.1850394564173,33.2606222983665,-39.6409205727319));
#249330=CARTESIAN_POINT('Ctrl Pts',(46.2638636333332,33.1772336958075,-39.6401443034625));
#249331=CARTESIAN_POINT('Ctrl Pts',(46.3151397511292,33.1201974856456,-39.6391646017005));
#249332=CARTESIAN_POINT('Ctrl Pts',(46.3401349353408,33.0909661742941,-39.6384440851485));
#249333=CARTESIAN_POINT('Ctrl Pts',(46.3888523044997,33.0309971480077,-39.6365301000439));
#249334=CARTESIAN_POINT('Ctrl Pts',(46.4123735341802,33.0005036828642,-39.6353439924849));
#249335=CARTESIAN_POINT('Ctrl Pts',(46.4576879006691,32.9386388625828,-39.6325280276393));
#249336=CARTESIAN_POINT('Ctrl Pts',(46.52311576659,32.8444620833496,-39.6276360146217));
#249337=CARTESIAN_POINT('Ctrl Pts',(46.5810426872604,32.7462345994881,-39.6207752343847));
#249338=CARTESIAN_POINT('Ctrl Pts',(46.6516918187307,32.6117039458857,-39.6098936921283));
#249339=CARTESIAN_POINT('Ctrl Pts',(46.683723185051,32.5426422373878,-39.6035832967262));
#249340=CARTESIAN_POINT('Ctrl Pts',(46.7195635412788,32.4540883209461,-39.5945936116187));
#249341=CARTESIAN_POINT('Ctrl Pts',(46.7265235775841,32.4362514419463,-39.5927383889278));
#249342=CARTESIAN_POINT('Ctrl Pts',(46.7400123459627,32.4003742100513,-39.5889189813535));
#249343=CARTESIAN_POINT('Ctrl Pts',(46.7465535157541,32.3822946053341,-39.5869502184844));
#249344=CARTESIAN_POINT('Ctrl Pts',(46.7654644360989,32.3279072933142,-39.5808958427402));
#249345=CARTESIAN_POINT('Ctrl Pts',(46.7770937339888,32.2915493874551,-39.5766741707955));
#249346=CARTESIAN_POINT('Ctrl Pts',(46.8091770518909,32.182013131159,-39.5634457571489));
#249347=CARTESIAN_POINT('Ctrl Pts',(46.8444383818759,32.034891308334,-39.5443264312115));
#249348=CARTESIAN_POINT('Ctrl Pts',(46.8650708643864,31.8856621776612,-39.5223044891954));
#249349=CARTESIAN_POINT('Ctrl Pts',(46.8750487417844,31.7729724844591,-39.50469487268));
#249350=CARTESIAN_POINT('Ctrl Pts',(46.8774570362353,31.7352651712118,-39.4986397605723));
#249351=CARTESIAN_POINT('Ctrl Pts',(46.8796767940079,31.6785286095959,-39.4892824810203));
#249352=CARTESIAN_POINT('Ctrl Pts',(46.8801843407089,31.6595724593507,-39.4861150486293));
#249353=CARTESIAN_POINT('Ctrl Pts',(46.8807312344332,31.6216180949417,-39.479690628598));
#249354=CARTESIAN_POINT('Ctrl Pts',(46.8807699646674,31.6025797052015,-39.4764266299692));
#249355=CARTESIAN_POINT('Ctrl Pts',(46.8801790388754,31.5455906639181,-39.4665317368708));
#249356=CARTESIAN_POINT('Ctrl Pts',(46.8788490796135,31.5078273383739,-39.4598096545541));
#249357=CARTESIAN_POINT('Ctrl Pts',(46.874360617844,31.4326451774338,-39.4461013696832));
#249358=CARTESIAN_POINT('Ctrl Pts',(46.864884835636,31.320441459725,-39.4251517854185));
#249359=CARTESIAN_POINT('Ctrl Pts',(46.8414902947658,31.1730719473388,-39.3956936109857));
#249360=CARTESIAN_POINT('Ctrl Pts',(46.8074810934279,31.0279105813681,-39.364717848004));
#249361=CARTESIAN_POINT('Ctrl Pts',(46.7869180083019,30.9560697433081,-39.3487190247537));
#249362=CARTESIAN_POINT('Ctrl Pts',(46.7645577771926,30.884604709384,-39.332461491893));
#249363=CARTESIAN_POINT('Ctrl Pts',(46.7524740339114,30.8490466969583,-39.3242001683612));
#249364=CARTESIAN_POINT('Ctrl Pts',(46.7264943673172,30.7783632715819,-39.3074248425479));
#249365=CARTESIAN_POINT('Ctrl Pts',(46.7127058212706,30.7435263372096,-39.2989795429224));
#249366=CARTESIAN_POINT('Ctrl Pts',(46.6981266849492,30.7091523375488,-39.2904704603133));
#249367=CARTESIAN_POINT('Ctrl Pts',(44.7926621173534,30.9780510210195,-41.4731170634489));
#249368=CARTESIAN_POINT('Ctrl Pts',(44.7841183378731,30.958431594105,-41.4560988982307));
#249369=CARTESIAN_POINT('Ctrl Pts',(44.7652574387158,30.9202429989855,-41.4215723090211));
#249370=CARTESIAN_POINT('Ctrl Pts',(44.7373647422364,30.8750641226134,-41.3772059160528));
#249371=CARTESIAN_POINT('Ctrl Pts',(44.7186826069414,30.8491098680677,-41.3500360893141));
#249372=CARTESIAN_POINT('Ctrl Pts',(44.7057896374646,30.8320666178198,-41.3317986258606));
#249373=CARTESIAN_POINT('Ctrl Pts',(44.6991283043737,30.8236797190306,-41.3226233796301));
#249374=CARTESIAN_POINT('Ctrl Pts',(44.6853430526266,30.8071501195218,-41.3041237465898));
#249375=CARTESIAN_POINT('Ctrl Pts',(44.6782604199269,30.7990587859436,-41.2948558628018));
#249376=CARTESIAN_POINT('Ctrl Pts',(44.6637865272211,30.7832912649286,-41.2763692550984));
#249377=CARTESIAN_POINT('Ctrl Pts',(44.65638232911,30.7755995480316,-41.2671331599469));
#249378=CARTESIAN_POINT('Ctrl Pts',(44.6336879630273,30.7531065345255,-41.2394625228135));
#249379=CARTESIAN_POINT('Ctrl Pts',(44.6100194582072,30.7317609779911,-41.211850451263));
#249380=CARTESIAN_POINT('Ctrl Pts',(44.5765344835469,30.7055824366946,-41.1751580074971));
#249381=CARTESIAN_POINT('Ctrl Pts',(44.5504480754,30.6870962504203,-41.147699245024));
#249382=CARTESIAN_POINT('Ctrl Pts',(44.5324056777293,30.6755504391987,-41.1294402655247));
#249383=CARTESIAN_POINT('Ctrl Pts',(44.5186168522497,30.6671837862428,-41.1157563555777));
#249384=CARTESIAN_POINT('Ctrl Pts',(44.5139760207251,30.6644431539959,-41.1111953707762));
#249385=CARTESIAN_POINT('Ctrl Pts',(44.5046579712977,30.6590892493455,-41.102125755137));
#249386=CARTESIAN_POINT('Ctrl Pts',(44.4999732573772,30.6564710151932,-41.0976094410703));
#249387=CARTESIAN_POINT('Ctrl Pts',(44.4764410055871,30.6436866063214,-41.0751408219827));
#249388=CARTESIAN_POINT('Ctrl Pts',(44.4380363426647,30.6251318507397,-41.0398401547925));
#249389=CARTESIAN_POINT('Ctrl Pts',(44.3881999640401,30.6066279457426,-40.9973473660572));
#249390=CARTESIAN_POINT('Ctrl Pts',(44.3574626802754,30.5976558165788,-40.9725988687145));
#249391=CARTESIAN_POINT('Ctrl Pts',(44.3367823836873,30.5921565153947,-40.9562701951691));
#249392=CARTESIAN_POINT('Ctrl Pts',(44.3263541271388,30.5896491085923,-40.9481956834911));
#249393=CARTESIAN_POINT('Ctrl Pts',(44.3052793937559,30.5851218575581,-40.9322027877955));
#249394=CARTESIAN_POINT('Ctrl Pts',(44.2946995104909,30.5831174982377,-40.924335654778));
#249395=CARTESIAN_POINT('Ctrl Pts',(44.2735450602529,30.5796377993431,-40.9089243529734));
#249396=CARTESIAN_POINT('Ctrl Pts',(44.2629524396991,30.5781585711684,-40.9013664771085));
#249397=CARTESIAN_POINT('Ctrl Pts',(44.2311453972639,30.5744985086998,-40.8791460851492));
#249398=CARTESIAN_POINT('Ctrl Pts',(44.2098907431643,30.5730912421562,-40.8649273724495));
#249399=CARTESIAN_POINT('Ctrl Pts',(44.1672866942957,30.5723474200962,-40.8376959485268));
#249400=CARTESIAN_POINT('Ctrl Pts',(44.1459323927671,30.5730120277702,-40.8246808510428));
#249401=CARTESIAN_POINT('Ctrl Pts',(44.1191870166623,30.5751734135742,-40.8091986194082));
#249402=CARTESIAN_POINT('Ctrl Pts',(44.1138315874482,30.5756735271978,-40.806139968135));
#249403=CARTESIAN_POINT('Ctrl Pts',(44.1031212948485,30.5768077596639,-40.8001057293845));
#249404=CARTESIAN_POINT('Ctrl Pts',(44.0977557278508,30.5774435866632,-40.7971244669688));
#249405=CARTESIAN_POINT('Ctrl Pts',(44.0817045383335,30.5795497856634,-40.7883321887253));
#249406=CARTESIAN_POINT('Ctrl Pts',(44.0710902649836,30.5812139186595,-40.7826858714375));
#249407=CARTESIAN_POINT('Ctrl Pts',(44.0394561806682,30.5869813183234,-40.7663593410916));
#249408=CARTESIAN_POINT('Ctrl Pts',(44.0082701709188,30.5942909050994,-40.7512721078743));
#249409=CARTESIAN_POINT('Ctrl Pts',(43.9675777996734,30.6070988998346,-40.7336299050859));
#249410=CARTESIAN_POINT('Ctrl Pts',(43.9375066395073,30.6182485087226,-40.721648717354));
#249411=CARTESIAN_POINT('Ctrl Pts',(43.917761614853,30.626725808719,-40.7145087645619));
#249412=CARTESIAN_POINT('Ctrl Pts',(43.8981718083816,30.6357351147044,-40.7078022579606));
#249413=CARTESIAN_POINT('Ctrl Pts',(43.8884396229394,30.6405162381665,-40.7046629153417));
#249414=CARTESIAN_POINT('Ctrl Pts',(43.8693712864522,30.6504970769624,-40.6988992879235));
#249415=CARTESIAN_POINT('Ctrl Pts',(43.8599880575193,30.6557176389023,-40.6962583786489));
#249416=CARTESIAN_POINT('Ctrl Pts',(43.8415477166501,30.6665995934339,-40.6914621347147));
#249417=CARTESIAN_POINT('Ctrl Pts',(43.8143622090585,30.6835906587784,-40.6849914969931));
#249418=CARTESIAN_POINT('Ctrl Pts',(43.7885885365895,30.7025683103525,-40.6806752166169));
#249419=CARTESIAN_POINT('Ctrl Pts',(43.7554869731093,30.7296502406846,-40.676851696754));
#249420=CARTESIAN_POINT('Ctrl Pts',(43.7395647886014,30.744083456595,-40.6759056793254));
#249421=CARTESIAN_POINT('Ctrl Pts',(43.7090440489059,30.7747854825451,-40.6760208486551));
#249422=CARTESIAN_POINT('Ctrl Pts',(43.6947173014185,30.7907796762741,-40.6770802501629));
#249423=CARTESIAN_POINT('Ctrl Pts',(43.6678443418708,30.8240220908504,-40.6811258797777));
#249424=CARTESIAN_POINT('Ctrl Pts',(43.6427576069985,30.8585127548254,-40.687098273402));
#249425=CARTESIAN_POINT('Ctrl Pts',(43.6212142380078,30.8954846730083,-40.6968894358922));
#249426=CARTESIAN_POINT('Ctrl Pts',(43.6088787182641,30.9193798597989,-40.7042205511341));
#249427=CARTESIAN_POINT('Ctrl Pts',(43.6064685586478,30.9241994859948,-40.7057484197296));
#249428=CARTESIAN_POINT('Ctrl Pts',(43.6017624551859,30.9339175659931,-40.70892606686));
#249429=CARTESIAN_POINT('Ctrl Pts',(43.5994656231147,30.9388193592268,-40.7105773965538));
#249430=CARTESIAN_POINT('Ctrl Pts',(43.5927866482525,30.953560895212,-40.7156875255853));
#249431=CARTESIAN_POINT('Ctrl Pts',(43.5844198153918,30.9733582110501,-40.72293005151));
#249432=CARTESIAN_POINT('Ctrl Pts',(43.5734440082896,31.0034822735469,-40.7350537322951));
#249433=CARTESIAN_POINT('Ctrl Pts',(43.5640181327981,31.0340244080827,-40.7484125407461));
#249434=CARTESIAN_POINT('Ctrl Pts',(43.5561284133843,31.0649820306433,-40.7629929778707));
#249435=CARTESIAN_POINT('Ctrl Pts',(43.5518912037438,31.0858969805267,-40.7735241784737));
#249436=CARTESIAN_POINT('Ctrl Pts',(43.5481682579358,31.1069510729684,-40.7844620267622));
#249437=CARTESIAN_POINT('Ctrl Pts',(43.5465635963524,31.1175527760565,-40.7901372750232));
#249438=CARTESIAN_POINT('Ctrl Pts',(43.5438765944467,31.1388768366658,-40.8018865323646));
#249439=CARTESIAN_POINT('Ctrl Pts',(43.5427912565025,31.1496493641875,-40.8079902348016));
#249440=CARTESIAN_POINT('Ctrl Pts',(43.5411674088753,31.1711124235333,-40.8204828132684));
#249441=CARTESIAN_POINT('Ctrl Pts',(43.5400805588778,31.19253758885,-40.8332822237109));
#249442=CARTESIAN_POINT('Ctrl Pts',(43.5400129658238,31.2352236668913,-40.8600695429299));
#249443=CARTESIAN_POINT('Ctrl Pts',(43.5430492497798,31.2776738375434,-40.8886047446452));
#249444=CARTESIAN_POINT('Ctrl Pts',(43.5491614319672,31.3198884817001,-40.918856387552));
#249445=CARTESIAN_POINT('Ctrl Pts',(43.5532522131496,31.3409199794841,-40.9345594064291));
#249446=CARTESIAN_POINT('Ctrl Pts',(43.5578644352119,31.361905871423,-40.9505475151733));
#249447=CARTESIAN_POINT('Ctrl Pts',(43.560439098329,31.3723994717644,-40.9587035928991));
#249448=CARTESIAN_POINT('Ctrl Pts',(43.5660648897127,31.3931449423641,-40.9751492091434));
#249449=CARTESIAN_POINT('Ctrl Pts',(43.5691234314236,31.4034342087731,-40.9834667538713));
#249450=CARTESIAN_POINT('Ctrl Pts',(43.5790202279964,31.4340221767704,-41.0086741075936));
#249451=CARTESIAN_POINT('Ctrl Pts',(43.5865808644402,31.4540562960243,-41.0258289330007));
#249452=CARTESIAN_POINT('Ctrl Pts',(43.5993606039644,31.4835727602996,-41.0520789232858));
#249453=CARTESIAN_POINT('Ctrl Pts',(43.6038584649574,31.4933175175814,-41.0609109997729));
#249454=CARTESIAN_POINT('Ctrl Pts',(43.6133480280387,31.5126460303085,-41.0787663839806));
#249455=CARTESIAN_POINT('Ctrl Pts',(43.6183219077102,31.5221915251339,-41.0877549157913));
#249456=CARTESIAN_POINT('Ctrl Pts',(43.6338406007018,31.5503182102049,-41.1147514459697));
#249457=CARTESIAN_POINT('Ctrl Pts',(43.6450116757484,31.5684678157769,-41.13285712865));
#249458=CARTESIAN_POINT('Ctrl Pts',(43.6689569093208,31.6035742491305,-41.1692591986645));
#249459=CARTESIAN_POINT('Ctrl Pts',(43.6881189975485,31.6290150958394,-41.1967078345595));
#249460=CARTESIAN_POINT('Ctrl Pts',(43.7160805799803,31.6611548911343,-41.2335986369031));
#249461=CARTESIAN_POINT('Ctrl Pts',(43.7308739938731,31.6766212732249,-41.2521403517739));
#249462=CARTESIAN_POINT('Ctrl Pts',(43.7460847706871,31.6917854492915,-41.2707364845776));
#249463=CARTESIAN_POINT('Ctrl Pts',(43.7539033240721,31.6992171694526,-41.2800648729051));
#249464=CARTESIAN_POINT('Ctrl Pts',(43.7697797892606,31.7136063232936,-41.298562009488));
#249465=CARTESIAN_POINT('Ctrl Pts',(43.7778723272806,31.7205988773597,-41.3077734720143));
#249466=CARTESIAN_POINT('Ctrl Pts',(43.8025568401133,31.7409299545529,-41.3352381600133));
#249467=CARTESIAN_POINT('Ctrl Pts',(43.8195937300504,31.7536621581445,-41.353369616892));
#249468=CARTESIAN_POINT('Ctrl Pts',(43.8547939251157,31.7774712224987,-41.3892512463859));
#249469=CARTESIAN_POINT('Ctrl Pts',(43.8820456950658,31.7940939723408,-41.4158852269725));
#249470=CARTESIAN_POINT('Ctrl Pts',(43.9105977352555,31.8088239425505,-41.4420959852738));
#249471=CARTESIAN_POINT('Ctrl Pts',(43.9299312426308,31.8182163905263,-41.4594780331231));
#249472=CARTESIAN_POINT('Ctrl Pts',(43.9397545046832,31.8226994853967,-41.4681277754213));
#249473=CARTESIAN_POINT('Ctrl Pts',(43.959476379363,31.8311327029401,-41.4851373530728));
#249474=CARTESIAN_POINT('Ctrl Pts',(43.969416794615,31.835103670887,-41.4935351095415));
#249475=CARTESIAN_POINT('Ctrl Pts',(43.9894286782948,31.8425474915593,-41.5100965816665));
#249476=CARTESIAN_POINT('Ctrl Pts',(44.0196562937352,31.8529720625538,-41.5345993599874));
#249477=CARTESIAN_POINT('Ctrl Pts',(44.0607928561344,31.8639280327151,-41.5659272170578));
#249478=CARTESIAN_POINT('Ctrl Pts',(44.0922765794535,31.8699137146658,-41.5884145416429));
#249479=CARTESIAN_POINT('Ctrl Pts',(44.1134085621028,31.8733992175668,-41.6031789442838));
#249480=CARTESIAN_POINT('Ctrl Pts',(44.1240412545,31.8748890570172,-41.6104444862381));
#249481=CARTESIAN_POINT('Ctrl Pts',(44.1401138557838,31.8767382236783,-41.6211788509405));
#249482=CARTESIAN_POINT('Ctrl Pts',(44.1454877988083,31.8772894545129,-41.6247266008247));
#249483=CARTESIAN_POINT('Ctrl Pts',(44.1562140153048,31.878256418298,-41.6317257811562));
#249484=CARTESIAN_POINT('Ctrl Pts',(44.161576905651,31.8786734249769,-41.6351843345794));
#249485=CARTESIAN_POINT('Ctrl Pts',(44.1776466456902,31.8797244502982,-41.6454258391029));
#249486=CARTESIAN_POINT('Ctrl Pts',(44.1883500092183,31.8801603696231,-41.6520850220369));
#249487=CARTESIAN_POINT('Ctrl Pts',(44.2204087008324,31.8806796234647,-41.671549250448));
#249488=CARTESIAN_POINT('Ctrl Pts',(44.2417298059497,31.8799780982567,-41.6838534602333));
#249489=CARTESIAN_POINT('Ctrl Pts',(44.2842582084951,31.8764766164199,-41.7071185815018));
#249490=CARTESIAN_POINT('Ctrl Pts',(44.3054713486111,31.8736750129732,-41.7180819683776));
#249491=CARTESIAN_POINT('Ctrl Pts',(44.3319064277948,31.8688271235064,-41.7309251637703));
#249492=CARTESIAN_POINT('Ctrl Pts',(44.3371930873745,31.8677885276791,-41.7334519256467));
#249493=CARTESIAN_POINT('Ctrl Pts',(44.3477523920959,31.8655764110726,-41.7384157665409));
#249494=CARTESIAN_POINT('Ctrl Pts',(44.353035452149,31.8644001232798,-41.7408573895762));
#249495=CARTESIAN_POINT('Ctrl Pts',(44.368821997144,31.8606750365135,-41.7480268313348));
#249496=CARTESIAN_POINT('Ctrl Pts',(44.3792318927429,31.8579388865424,-41.752586114057));
#249497=CARTESIAN_POINT('Ctrl Pts',(44.4101727404,31.8489724804825,-41.7656371280416));
#249498=CARTESIAN_POINT('Ctrl Pts',(44.4405041748167,31.8385015328462,-41.7774224567595));
#249499=CARTESIAN_POINT('Ctrl Pts',(44.4797386522914,31.8215610256552,-41.7906399779756));
#249500=CARTESIAN_POINT('Ctrl Pts',(44.5085558494592,31.8073558935676,-41.7992982329201));
#249501=CARTESIAN_POINT('Ctrl Pts',(44.5273583247585,31.7968714183439,-41.8042246106906));
#249502=CARTESIAN_POINT('Ctrl Pts',(44.5459478308046,31.7858731708475,-41.8087197459362));
#249503=CARTESIAN_POINT('Ctrl Pts',(44.5551558111633,31.7801015230391,-41.8107541019367));
#249504=CARTESIAN_POINT('Ctrl Pts',(44.5731320510561,31.7681815367951,-41.814338976855));
#249505=CARTESIAN_POINT('Ctrl Pts',(44.5819448307914,31.7620078883687,-41.8159008719862));
#249506=CARTESIAN_POINT('Ctrl Pts',(44.5991987000126,31.7492554022398,-41.8185646224661));
#249507=CARTESIAN_POINT('Ctrl Pts',(44.6245350600795,31.7295108031857,-41.8218731379338));
#249508=CARTESIAN_POINT('Ctrl Pts',(44.6561620699444,31.7007477525095,-41.8235671758672));
#249509=CARTESIAN_POINT('Ctrl Pts',(44.6782580742923,31.6773394437008,-41.8227909065983));
#249510=CARTESIAN_POINT('Ctrl Pts',(44.6926220014235,31.6613194462407,-41.8218112048364));
#249511=CARTESIAN_POINT('Ctrl Pts',(44.6996188611148,31.6531046671394,-41.8210906882841));
#249512=CARTESIAN_POINT('Ctrl Pts',(44.7132456597446,31.6362429219073,-41.8191767031797));
#249513=CARTESIAN_POINT('Ctrl Pts',(44.7198193777268,31.627664624135,-41.8179905956202));
#249514=CARTESIAN_POINT('Ctrl Pts',(44.7324727845908,31.610252798272,-41.8151746307749));
#249515=CARTESIAN_POINT('Ctrl Pts',(44.7507253937504,31.5837345714901,-41.8102826177571));
#249516=CARTESIAN_POINT('Ctrl Pts',(44.7668325292565,31.5560404782777,-41.8034218375205));
#249517=CARTESIAN_POINT('Ctrl Pts',(44.7864242741839,31.5180816884312,-41.7925402952635));
#249518=CARTESIAN_POINT('Ctrl Pts',(44.7952779235527,31.4985810718442,-41.7862298998632));
#249519=CARTESIAN_POINT('Ctrl Pts',(44.8051436066325,31.4735589245645,-41.777240214754));
#249520=CARTESIAN_POINT('Ctrl Pts',(44.8070571630202,31.4685179927861,-41.7753849920635));
#249521=CARTESIAN_POINT('Ctrl Pts',(44.8107609555809,31.4583769076679,-41.7715655844892));
#249522=CARTESIAN_POINT('Ctrl Pts',(44.8125545845603,31.4532656516023,-41.76959682162));
#249523=CARTESIAN_POINT('Ctrl Pts',(44.8177323950795,31.4378873281915,-41.7635424458753));
#249524=CARTESIAN_POINT('Ctrl Pts',(44.8209059367305,31.4276035217402,-41.7593207739311));
#249525=CARTESIAN_POINT('Ctrl Pts',(44.8296276705658,31.3966113763671,-41.7460923602843));
#249526=CARTESIAN_POINT('Ctrl Pts',(44.8391161742293,31.3549585404116,-41.7269730343471));
#249527=CARTESIAN_POINT('Ctrl Pts',(44.8444380100638,31.312658433005,-41.7049510923314));
#249528=CARTESIAN_POINT('Ctrl Pts',(44.8468637082338,31.2806969121874,-41.6873414758157));
#249529=CARTESIAN_POINT('Ctrl Pts',(44.8474108190536,31.2699990859542,-41.6812863637077));
#249530=CARTESIAN_POINT('Ctrl Pts',(44.8478348231013,31.2538978106508,-41.671929084156));
#249531=CARTESIAN_POINT('Ctrl Pts',(44.8479099202363,31.2485174556463,-41.6687616517648));
#249532=CARTESIAN_POINT('Ctrl Pts',(44.8479268208064,31.2377432265879,-41.6623372317338));
#249533=CARTESIAN_POINT('Ctrl Pts',(44.8478683021095,31.2323379437313,-41.6590732331048));
#249534=CARTESIAN_POINT('Ctrl Pts',(44.8474921214824,31.2161555213209,-41.6491783400064));
#249535=CARTESIAN_POINT('Ctrl Pts',(44.8469759958029,31.2054292064128,-41.6424562576898));
#249536=CARTESIAN_POINT('Ctrl Pts',(44.8454249887827,31.1840681958411,-41.6287479728186));
#249537=CARTESIAN_POINT('Ctrl Pts',(44.8423204600693,31.1521790951542,-41.6077983885548));
#249538=CARTESIAN_POINT('Ctrl Pts',(44.8351290816859,31.1102584040656,-41.5783402141209));
#249539=CARTESIAN_POINT('Ctrl Pts',(44.8249268329474,31.0689281614894,-41.54736445114));
#249540=CARTESIAN_POINT('Ctrl Pts',(44.8188163283608,31.0484607830594,-41.5313656278891));
#249541=CARTESIAN_POINT('Ctrl Pts',(44.8121960627665,31.028093840338,-41.5151080950287));
#249542=CARTESIAN_POINT('Ctrl Pts',(44.808629563005,31.0179567656131,-41.5068467714969));
#249543=CARTESIAN_POINT('Ctrl Pts',(44.8009827391877,30.9977990758989,-41.4900714456835));
#249544=CARTESIAN_POINT('Ctrl Pts',(44.7969340070935,30.9878607344767,-41.4816261460579));
#249545=CARTESIAN_POINT('Ctrl Pts',(44.7926621173534,30.9780510210195,-41.4731170634489));
#249546=CARTESIAN_POINT('',(42.5465433949648,31.1494605775469,-38.9933921633854));
#249547=CARTESIAN_POINT('',(43.4124119497911,29.8671948678953,-38.9060746475284));
#249548=CARTESIAN_POINT('Ctrl Pts',(42.5465433949858,31.149460577658,-38.9933921633669));
#249549=CARTESIAN_POINT('Ctrl Pts',(42.5517121988544,31.1235309006459,-38.9890511466991));
#249550=CARTESIAN_POINT('Ctrl Pts',(42.5573895309802,31.0977319961209,-38.9848419481203));
#249551=CARTESIAN_POINT('Ctrl Pts',(42.5635729904876,31.072063191646,-38.9807642563972));
#249552=CARTESIAN_POINT('Ctrl Pts',(42.5712503905032,31.0401927347216,-38.9757013833469));
#249553=CARTESIAN_POINT('Ctrl Pts',(42.5797080333646,31.0085228392725,-38.9708412376922));
#249554=CARTESIAN_POINT('Ctrl Pts',(42.588946982225,30.9770538375888,-38.9661846968102));
#249555=CARTESIAN_POINT('Ctrl Pts',(42.598185929499,30.9455848413087,-38.9615281567277));
#249556=CARTESIAN_POINT('Ctrl Pts',(42.6082061579755,30.9143167308057,-38.9570752148634));
#249557=CARTESIAN_POINT('Ctrl Pts',(42.6190146688054,30.8832507585404,-38.9528281316886));
#249558=CARTESIAN_POINT('Ctrl Pts',(42.6298231763812,30.8521847956286,-38.9485810497924));
#249559=CARTESIAN_POINT('Ctrl Pts',(42.6414199451632,30.8213209708386,-38.9445397978418));
#249560=CARTESIAN_POINT('Ctrl Pts',(42.6538171837854,30.7906641657846,-38.9407085616));
#249561=CARTESIAN_POINT('Ctrl Pts',(42.6662144355469,30.760007328239,-38.9368773212977));
#249562=CARTESIAN_POINT('Ctrl Pts',(42.679412432567,30.7295576275844,-38.933256079272));
#249563=CARTESIAN_POINT('Ctrl Pts',(42.6934317597292,30.6993135470368,-38.929849324519));
#249564=CARTESIAN_POINT('Ctrl Pts',(42.7004414190611,30.6841915159301,-38.9281459481751));
#249565=CARTESIAN_POINT('Ctrl Pts',(42.7076664478388,30.6691033617142,-38.9264946184812));
#249566=CARTESIAN_POINT('Ctrl Pts',(42.7150618821773,30.6541435858172,-38.924905794916));
#249567=CARTESIAN_POINT('Ctrl Pts',(42.7224573165159,30.6391838099201,-38.9233169713508));
#249568=CARTESIAN_POINT('Ctrl Pts',(42.7300260074317,30.6243421619354,-38.9217891027553));
#249569=CARTESIAN_POINT('Ctrl Pts',(42.7377673957025,30.609622247504,-38.9203228797071));
#249570=CARTESIAN_POINT('Ctrl Pts',(42.7687329487861,30.5507425897785,-38.9144579875143));
#249571=CARTESIAN_POINT('Ctrl Pts',(42.8024375668609,30.4937516435998,-38.9095621141477));
#249572=CARTESIAN_POINT('Ctrl Pts',(42.8388299093084,30.438621888508,-38.9056211995292));
#249573=CARTESIAN_POINT('Ctrl Pts',(42.8752222517559,30.3834921334163,-38.9016802849107));
#249574=CARTESIAN_POINT('Ctrl Pts',(42.9142995039568,30.330221730441,-38.898694431399));
#249575=CARTESIAN_POINT('Ctrl Pts',(42.9560847992068,30.2788238207524,-38.8966716165917));
#249576=CARTESIAN_POINT('Ctrl Pts',(42.9978700944569,30.2274259110637,-38.8946488017843));
#249577=CARTESIAN_POINT('Ctrl Pts',(43.0423540539347,30.1779090615142,-38.8935894002766));
#249578=CARTESIAN_POINT('Ctrl Pts',(43.0896679045841,30.1303216200235,-38.8935318156116));
#249579=CARTESIAN_POINT('Ctrl Pts',(43.1369817552336,30.0827341785328,-38.8934742309466));
#249580=CARTESIAN_POINT('Ctrl Pts',(43.1862827102732,30.0379274090563,-38.8944202483754));
#249581=CARTESIAN_POINT('Ctrl Pts',(43.2374695236468,29.9958252623364,-38.8963320083068));
#249582=CARTESIAN_POINT('Ctrl Pts',(43.2886563370204,29.9537231156164,-38.8982437682382));
#249583=CARTESIAN_POINT('Ctrl Pts',(43.3417388904795,29.9143166390041,-38.9011209692255));
#249584=CARTESIAN_POINT('Ctrl Pts',(43.3967029760762,29.8775860305619,-38.9049562506722));
#249585=CARTESIAN_POINT('Ctrl Pts',(43.4019223133192,29.8740981269513,-38.9053204453472));
#249586=CARTESIAN_POINT('Ctrl Pts',(43.4071586307135,29.8706343666859,-38.9056932332283));
#249587=CARTESIAN_POINT('Ctrl Pts',(43.4124119245055,29.8671948319696,-38.9060746716112));
#249588=CARTESIAN_POINT('Ctrl Pts',(43.4124119916018,29.8671949277328,-38.9060746094712));
#249589=CARTESIAN_POINT('Ctrl Pts',(43.306953409283,29.9434764107567,-38.910152608303));
#249590=CARTESIAN_POINT('Ctrl Pts',(43.2083433673275,30.0286067508031,-38.9150790128273));
#249591=CARTESIAN_POINT('Ctrl Pts',(43.0323970922931,30.2092699147785,-38.926031267232));
#249592=CARTESIAN_POINT('Ctrl Pts',(42.9545167445323,30.303420598745,-38.9319503267308));
#249593=CARTESIAN_POINT('Ctrl Pts',(42.8824130593679,30.406577317803,-38.9385942614148));
#249594=CARTESIAN_POINT('Ctrl Pts',(42.8802160625943,30.4097376871659,-38.9387979558357));
#249595=CARTESIAN_POINT('Ctrl Pts',(42.873503757505,30.4194461821076,-38.9394241486516));
#249596=CARTESIAN_POINT('Ctrl Pts',(42.8690151216511,30.4260123314163,-38.9398482921576));
#249597=CARTESIAN_POINT('Ctrl Pts',(42.7974813182203,30.5318494929995,-38.9466952735419));
#249598=CARTESIAN_POINT('Ctrl Pts',(42.7379995399575,30.6368649182166,-38.953586864865));
#249599=CARTESIAN_POINT('Ctrl Pts',(42.627565466591,30.8761040070808,-38.9710040199756));
#249600=CARTESIAN_POINT('Ctrl Pts',(42.5804757556733,31.011029152592,-38.981657984184));
#249601=CARTESIAN_POINT('Ctrl Pts',(42.5465433948297,31.149460577507,-38.9933921634656));
#249602=CARTESIAN_POINT('Ctrl Pts',(44.5079524583208,33.2091977213449,-52.99995));
#249603=CARTESIAN_POINT('Ctrl Pts',(43.5445019199415,33.2091977213449,-52.9416166666667));
#249604=CARTESIAN_POINT('Ctrl Pts',(43.0627766507519,32.3748250798187,-52.8832833333334));
#249605=CARTESIAN_POINT('Ctrl Pts',(42.5810513815623,31.5404524382925,-52.82495));
#249606=CARTESIAN_POINT('Ctrl Pts',(43.0627766507519,30.7060797967663,-52.7666166666667));
#249607=CARTESIAN_POINT('Ctrl Pts',(43.5445019199415,29.87170715524,-52.7082833333333));
#249608=CARTESIAN_POINT('Ctrl Pts',(44.5079524583208,29.87170715524,-52.64995));
#249609=CARTESIAN_POINT('Ctrl Pts',(45.4714029967,29.87170715524,-52.5916166666666));
#249610=CARTESIAN_POINT('Ctrl Pts',(45.9531282658897,30.7060797967663,-52.5332833333334));
#249611=CARTESIAN_POINT('Ctrl Pts',(46.4348535350793,31.5404524382925,-52.4749500000001));
#249612=CARTESIAN_POINT('Ctrl Pts',(45.9531282658897,32.3748250798187,-52.4166166666667));
#249613=CARTESIAN_POINT('Ctrl Pts',(45.4714029967,33.2091977213449,-52.3582833333334));
#249614=CARTESIAN_POINT('Ctrl Pts',(44.5079524583208,33.2091977213449,-52.29995));
#249615=CARTESIAN_POINT('Ctrl Pts',(43.5445019199415,33.2091977213449,-52.2416166666667));
#249616=CARTESIAN_POINT('Ctrl Pts',(43.0627766507519,32.3748250798187,-52.1832833333333));
#249617=CARTESIAN_POINT('Ctrl Pts',(42.5810513815623,31.5404524382925,-52.12495));
#249618=CARTESIAN_POINT('Ctrl Pts',(43.0627766507519,30.7060797967663,-52.0666166666667));
#249619=CARTESIAN_POINT('Ctrl Pts',(43.5445019199415,29.87170715524,-52.0082833333333));
#249620=CARTESIAN_POINT('Ctrl Pts',(44.5079524583208,29.87170715524,-51.94995));
#249621=CARTESIAN_POINT('Ctrl Pts',(45.4714029967,29.87170715524,-51.8916166666667));
#249622=CARTESIAN_POINT('Ctrl Pts',(45.9531282658897,30.7060797967663,-51.8332833333333));
#249623=CARTESIAN_POINT('Ctrl Pts',(46.4348535350793,31.5404524382925,-51.77495));
#249624=CARTESIAN_POINT('Ctrl Pts',(45.9531282658897,32.3748250798187,-51.7166166666667));
#249625=CARTESIAN_POINT('Ctrl Pts',(45.4714029967,33.2091977213449,-51.6582833333333));
#249626=CARTESIAN_POINT('Ctrl Pts',(44.5079524583208,33.2091977213449,-51.59995));
#249627=CARTESIAN_POINT('Ctrl Pts',(43.5445019199415,33.2091977213449,-51.5416166666667));
#249628=CARTESIAN_POINT('Ctrl Pts',(43.0627766507519,32.3748250798187,-51.4832833333333));
#249629=CARTESIAN_POINT('Ctrl Pts',(42.5810513815623,31.5404524382925,-51.42495));
#249630=CARTESIAN_POINT('Ctrl Pts',(43.0627766507519,30.7060797967663,-51.3666166666667));
#249631=CARTESIAN_POINT('Ctrl Pts',(43.5445019199415,29.87170715524,-51.3082833333333));
#249632=CARTESIAN_POINT('Ctrl Pts',(44.5079524583208,29.87170715524,-51.24995));
#249633=CARTESIAN_POINT('Ctrl Pts',(45.4714029967,29.87170715524,-51.1916166666667));
#249634=CARTESIAN_POINT('Ctrl Pts',(45.9531282658897,30.7060797967663,-51.1332833333333));
#249635=CARTESIAN_POINT('Ctrl Pts',(46.4348535350793,31.5404524382925,-51.07495));
#249636=CARTESIAN_POINT('Ctrl Pts',(45.9531282658897,32.3748250798187,-51.0166166666667));
#249637=CARTESIAN_POINT('Ctrl Pts',(45.4714029967,33.2091977213449,-50.9582833333334));
#249638=CARTESIAN_POINT('Ctrl Pts',(44.5079524583208,33.2091977213449,-50.89995));
#249639=CARTESIAN_POINT('Ctrl Pts',(43.5445019199415,33.2091977213449,-50.8416166666667));
#249640=CARTESIAN_POINT('Ctrl Pts',(43.0627766507519,32.3748250798187,-50.7832833333333));
#249641=CARTESIAN_POINT('Ctrl Pts',(42.5810513815623,31.5404524382925,-50.72495));
#249642=CARTESIAN_POINT('Ctrl Pts',(43.0627766507519,30.7060797967663,-50.6666166666667));
#249643=CARTESIAN_POINT('Ctrl Pts',(43.5445019199415,29.87170715524,-50.6082833333334));
#249644=CARTESIAN_POINT('Ctrl Pts',(44.5079524583208,29.87170715524,-50.54995));
#249645=CARTESIAN_POINT('Ctrl Pts',(45.4714029967,29.87170715524,-50.4916166666667));
#249646=CARTESIAN_POINT('Ctrl Pts',(45.9531282658897,30.7060797967663,-50.4332833333333));
#249647=CARTESIAN_POINT('Ctrl Pts',(46.4348535350793,31.5404524382925,-50.37495));
#249648=CARTESIAN_POINT('Ctrl Pts',(45.9531282658897,32.3748250798187,-50.3166166666667));
#249649=CARTESIAN_POINT('Ctrl Pts',(45.4714029967,33.2091977213449,-50.2582833333334));
#249650=CARTESIAN_POINT('Ctrl Pts',(44.5079524583208,33.2091977213449,-50.19995));
#249651=CARTESIAN_POINT('Ctrl Pts',(43.5445019199415,33.2091977213449,-50.1416166666667));
#249652=CARTESIAN_POINT('Ctrl Pts',(43.0627766507519,32.3748250798187,-50.0832833333333));
#249653=CARTESIAN_POINT('Ctrl Pts',(42.5810513815623,31.5404524382925,-50.02495));
#249654=CARTESIAN_POINT('Ctrl Pts',(43.0627766507519,30.7060797967663,-49.9666166666667));
#249655=CARTESIAN_POINT('Ctrl Pts',(43.5445019199415,29.87170715524,-49.9082833333334));
#249656=CARTESIAN_POINT('Ctrl Pts',(44.5079524583208,29.87170715524,-49.84995));
#249657=CARTESIAN_POINT('Ctrl Pts',(45.4714029967,29.87170715524,-49.7916166666667));
#249658=CARTESIAN_POINT('Ctrl Pts',(45.9531282658897,30.7060797967663,-49.7332833333333));
#249659=CARTESIAN_POINT('Ctrl Pts',(46.4348535350793,31.5404524382925,-49.67495));
#249660=CARTESIAN_POINT('Ctrl Pts',(45.9531282658897,32.3748250798187,-49.6166166666667));
#249661=CARTESIAN_POINT('Ctrl Pts',(45.4714029967,33.2091977213449,-49.5582833333334));
#249662=CARTESIAN_POINT('Ctrl Pts',(44.5079524583208,33.2091977213449,-49.49995));
#249663=CARTESIAN_POINT('Ctrl Pts',(43.5445019199415,33.2091977213449,-49.4416166666667));
#249664=CARTESIAN_POINT('Ctrl Pts',(43.0627766507519,32.3748250798187,-49.3832833333334));
#249665=CARTESIAN_POINT('Ctrl Pts',(42.5810513815623,31.5404524382925,-49.32495));
#249666=CARTESIAN_POINT('Ctrl Pts',(43.0627766507519,30.7060797967663,-49.2666166666667));
#249667=CARTESIAN_POINT('Ctrl Pts',(43.5445019199415,29.87170715524,-49.2082833333334));
#249668=CARTESIAN_POINT('Ctrl Pts',(44.5079524583208,29.87170715524,-49.14995));
#249669=CARTESIAN_POINT('Ctrl Pts',(45.4714029967,29.87170715524,-49.0916166666667));
#249670=CARTESIAN_POINT('Ctrl Pts',(45.9531282658897,30.7060797967663,-49.0332833333333));
#249671=CARTESIAN_POINT('Ctrl Pts',(46.4348535350793,31.5404524382925,-48.97495));
#249672=CARTESIAN_POINT('Ctrl Pts',(45.9531282658897,32.3748250798187,-48.9166166666667));
#249673=CARTESIAN_POINT('Ctrl Pts',(45.4714029967,33.2091977213449,-48.8582833333333));
#249674=CARTESIAN_POINT('Ctrl Pts',(44.5079524583208,33.2091977213449,-48.79995));
#249675=CARTESIAN_POINT('Ctrl Pts',(43.5445019199415,33.2091977213449,-48.7416166666667));
#249676=CARTESIAN_POINT('Ctrl Pts',(43.0627766507519,32.3748250798187,-48.6832833333333));
#249677=CARTESIAN_POINT('Ctrl Pts',(42.5810513815623,31.5404524382925,-48.62495));
#249678=CARTESIAN_POINT('Ctrl Pts',(43.0627766507519,30.7060797967663,-48.5666166666667));
#249679=CARTESIAN_POINT('Ctrl Pts',(43.5445019199415,29.87170715524,-48.5082833333333));
#249680=CARTESIAN_POINT('Ctrl Pts',(44.5079524583208,29.87170715524,-48.44995));
#249681=CARTESIAN_POINT('Ctrl Pts',(45.4714029967,29.87170715524,-48.3916166666667));
#249682=CARTESIAN_POINT('Ctrl Pts',(45.9531282658897,30.7060797967663,-48.3332833333333));
#249683=CARTESIAN_POINT('Ctrl Pts',(46.4348535350793,31.5404524382925,-48.27495));
#249684=CARTESIAN_POINT('Ctrl Pts',(45.9531282658897,32.3748250798187,-48.2166166666667));
#249685=CARTESIAN_POINT('Ctrl Pts',(45.4714029967,33.2091977213449,-48.1582833333333));
#249686=CARTESIAN_POINT('Ctrl Pts',(44.5079524583208,33.2091977213449,-48.09995));
#249687=CARTESIAN_POINT('Ctrl Pts',(43.5445019199415,33.2091977213449,-48.0416166666667));
#249688=CARTESIAN_POINT('Ctrl Pts',(43.0627766507519,32.3748250798187,-47.9832833333334));
#249689=CARTESIAN_POINT('Ctrl Pts',(42.5810513815623,31.5404524382925,-47.92495));
#249690=CARTESIAN_POINT('Ctrl Pts',(43.0627766507519,30.7060797967663,-47.8666166666667));
#249691=CARTESIAN_POINT('Ctrl Pts',(43.5445019199415,29.87170715524,-47.8082833333333));
#249692=CARTESIAN_POINT('Ctrl Pts',(44.5079524583208,29.87170715524,-47.74995));
#249693=CARTESIAN_POINT('Ctrl Pts',(45.4714029967,29.87170715524,-47.6916166666667));
#249694=CARTESIAN_POINT('Ctrl Pts',(45.9531282658897,30.7060797967663,-47.6332833333333));
#249695=CARTESIAN_POINT('Ctrl Pts',(46.4348535350793,31.5404524382925,-47.57495));
#249696=CARTESIAN_POINT('Ctrl Pts',(45.9531282658897,32.3748250798187,-47.5166166666667));
#249697=CARTESIAN_POINT('Ctrl Pts',(45.4714029967,33.2091977213449,-47.4582833333333));
#249698=CARTESIAN_POINT('Ctrl Pts',(44.5079524583208,33.2091977213449,-47.39995));
#249699=CARTESIAN_POINT('Ctrl Pts',(43.5445019199415,33.2091977213449,-47.3416166666666));
#249700=CARTESIAN_POINT('Ctrl Pts',(43.0627766507519,32.3748250798187,-47.2832833333333));
#249701=CARTESIAN_POINT('Ctrl Pts',(42.5810513815623,31.5404524382925,-47.22495));
#249702=CARTESIAN_POINT('Ctrl Pts',(43.0627766507519,30.7060797967663,-47.1666166666667));
#249703=CARTESIAN_POINT('Ctrl Pts',(43.5445019199415,29.87170715524,-47.1082833333333));
#249704=CARTESIAN_POINT('Ctrl Pts',(44.5079524583208,29.87170715524,-47.04995));
#249705=CARTESIAN_POINT('Ctrl Pts',(45.4714029967,29.87170715524,-46.9916166666667));
#249706=CARTESIAN_POINT('Ctrl Pts',(45.9531282658897,30.7060797967663,-46.9332833333333));
#249707=CARTESIAN_POINT('Ctrl Pts',(46.4348535350793,31.5404524382925,-46.87495));
#249708=CARTESIAN_POINT('Ctrl Pts',(45.9531282658897,32.3748250798187,-46.8166166666667));
#249709=CARTESIAN_POINT('Ctrl Pts',(45.4714029967,33.2091977213449,-46.7582833333333));
#249710=CARTESIAN_POINT('Ctrl Pts',(44.5079524583208,33.2091977213449,-46.69995));
#249711=CARTESIAN_POINT('Ctrl Pts',(43.5445019199415,33.2091977213449,-46.6416166666666));
#249712=CARTESIAN_POINT('Ctrl Pts',(43.0627766507519,32.3748250798187,-46.5832833333334));
#249713=CARTESIAN_POINT('Ctrl Pts',(42.5810513815623,31.5404524382925,-46.52495));
#249714=CARTESIAN_POINT('Ctrl Pts',(43.0627766507519,30.7060797967663,-46.4666166666667));
#249715=CARTESIAN_POINT('Ctrl Pts',(43.5445019199415,29.87170715524,-46.4082833333333));
#249716=CARTESIAN_POINT('Ctrl Pts',(44.5079524583208,29.87170715524,-46.34995));
#249717=CARTESIAN_POINT('Ctrl Pts',(45.4714029967,29.87170715524,-46.2916166666667));
#249718=CARTESIAN_POINT('Ctrl Pts',(45.9531282658897,30.7060797967663,-46.2332833333334));
#249719=CARTESIAN_POINT('Ctrl Pts',(46.4348535350793,31.5404524382925,-46.17495));
#249720=CARTESIAN_POINT('Ctrl Pts',(45.9531282658897,32.3748250798187,-46.1166166666667));
#249721=CARTESIAN_POINT('Ctrl Pts',(45.4714029967,33.2091977213449,-46.0582833333333));
#249722=CARTESIAN_POINT('Ctrl Pts',(44.5079524583208,33.2091977213449,-45.99995));
#249723=CARTESIAN_POINT('Ctrl Pts',(43.5445019199415,33.2091977213449,-45.9416166666667));
#249724=CARTESIAN_POINT('Ctrl Pts',(43.0627766507519,32.3748250798187,-45.8832833333333));
#249725=CARTESIAN_POINT('Ctrl Pts',(42.5810513815623,31.5404524382925,-45.82495));
#249726=CARTESIAN_POINT('Ctrl Pts',(43.0627766507519,30.7060797967663,-45.7666166666667));
#249727=CARTESIAN_POINT('Ctrl Pts',(43.5445019199415,29.87170715524,-45.7082833333333));
#249728=CARTESIAN_POINT('Ctrl Pts',(44.5079524583208,29.87170715524,-45.64995));
#249729=CARTESIAN_POINT('Ctrl Pts',(45.4714029967,29.87170715524,-45.5916166666667));
#249730=CARTESIAN_POINT('Ctrl Pts',(45.9531282658897,30.7060797967663,-45.5332833333333));
#249731=CARTESIAN_POINT('Ctrl Pts',(46.4348535350793,31.5404524382925,-45.47495));
#249732=CARTESIAN_POINT('Ctrl Pts',(45.9531282658897,32.3748250798187,-45.4166166666667));
#249733=CARTESIAN_POINT('Ctrl Pts',(45.4714029967,33.2091977213449,-45.3582833333333));
#249734=CARTESIAN_POINT('Ctrl Pts',(44.5079524583208,33.2091977213449,-45.29995));
#249735=CARTESIAN_POINT('Ctrl Pts',(43.5445019199415,33.2091977213449,-45.2416166666667));
#249736=CARTESIAN_POINT('Ctrl Pts',(43.0627766507519,32.3748250798187,-45.1832833333333));
#249737=CARTESIAN_POINT('Ctrl Pts',(42.5810513815623,31.5404524382925,-45.12495));
#249738=CARTESIAN_POINT('Ctrl Pts',(43.0627766507519,30.7060797967663,-45.0666166666667));
#249739=CARTESIAN_POINT('Ctrl Pts',(43.5445019199415,29.87170715524,-45.0082833333334));
#249740=CARTESIAN_POINT('Ctrl Pts',(44.5079524583208,29.87170715524,-44.94995));
#249741=CARTESIAN_POINT('Ctrl Pts',(45.4714029967,29.87170715524,-44.8916166666667));
#249742=CARTESIAN_POINT('Ctrl Pts',(45.9531282658897,30.7060797967663,-44.8332833333334));
#249743=CARTESIAN_POINT('Ctrl Pts',(46.4348535350793,31.5404524382925,-44.77495));
#249744=CARTESIAN_POINT('Ctrl Pts',(45.9531282658897,32.3748250798187,-44.7166166666667));
#249745=CARTESIAN_POINT('Ctrl Pts',(45.4714029967,33.2091977213449,-44.6582833333333));
#249746=CARTESIAN_POINT('Ctrl Pts',(44.5079524583208,33.2091977213449,-44.59995));
#249747=CARTESIAN_POINT('Ctrl Pts',(43.5445019199415,33.2091977213449,-44.5416166666667));
#249748=CARTESIAN_POINT('Ctrl Pts',(43.0627766507519,32.3748250798187,-44.4832833333334));
#249749=CARTESIAN_POINT('Ctrl Pts',(42.5810513815623,31.5404524382925,-44.42495));
#249750=CARTESIAN_POINT('Ctrl Pts',(43.0627766507519,30.7060797967663,-44.3666166666667));
#249751=CARTESIAN_POINT('Ctrl Pts',(43.5445019199415,29.87170715524,-44.3082833333334));
#249752=CARTESIAN_POINT('Ctrl Pts',(44.5079524583208,29.87170715524,-44.24995));
#249753=CARTESIAN_POINT('Ctrl Pts',(45.4714029967,29.87170715524,-44.1916166666667));
#249754=CARTESIAN_POINT('Ctrl Pts',(45.9531282658897,30.7060797967663,-44.1332833333334));
#249755=CARTESIAN_POINT('Ctrl Pts',(46.4348535350793,31.5404524382925,-44.07495));
#249756=CARTESIAN_POINT('Ctrl Pts',(45.9531282658897,32.3748250798187,-44.0166166666667));
#249757=CARTESIAN_POINT('Ctrl Pts',(45.4714029967,33.2091977213449,-43.9582833333334));
#249758=CARTESIAN_POINT('Ctrl Pts',(44.5079524583208,33.2091977213449,-43.89995));
#249759=CARTESIAN_POINT('Ctrl Pts',(43.5445019199415,33.2091977213449,-43.8416166666667));
#249760=CARTESIAN_POINT('Ctrl Pts',(43.0627766507519,32.3748250798187,-43.7832833333334));
#249761=CARTESIAN_POINT('Ctrl Pts',(42.5810513815623,31.5404524382925,-43.72495));
#249762=CARTESIAN_POINT('Ctrl Pts',(43.0627766507519,30.7060797967663,-43.6666166666667));
#249763=CARTESIAN_POINT('Ctrl Pts',(43.5445019199415,29.87170715524,-43.6082833333333));
#249764=CARTESIAN_POINT('Ctrl Pts',(44.5079524583208,29.87170715524,-43.54995));
#249765=CARTESIAN_POINT('Ctrl Pts',(45.4714029967,29.87170715524,-43.4916166666667));
#249766=CARTESIAN_POINT('Ctrl Pts',(45.9531282658897,30.7060797967663,-43.4332833333333));
#249767=CARTESIAN_POINT('Ctrl Pts',(46.4348535350793,31.5404524382925,-43.37495));
#249768=CARTESIAN_POINT('Ctrl Pts',(45.9531282658897,32.3748250798187,-43.3166166666667));
#249769=CARTESIAN_POINT('Ctrl Pts',(45.4714029967,33.2091977213449,-43.2582833333333));
#249770=CARTESIAN_POINT('Ctrl Pts',(44.5079524583208,33.2091977213449,-43.19995));
#249771=CARTESIAN_POINT('Ctrl Pts',(43.5445019199415,33.2091977213449,-43.1416166666666));
#249772=CARTESIAN_POINT('Ctrl Pts',(43.0627766507519,32.3748250798187,-43.0832833333333));
#249773=CARTESIAN_POINT('Ctrl Pts',(42.5810513815623,31.5404524382925,-43.02495));
#249774=CARTESIAN_POINT('Ctrl Pts',(43.0627766507519,30.7060797967663,-42.9666166666667));
#249775=CARTESIAN_POINT('Ctrl Pts',(43.5445019199415,29.87170715524,-42.9082833333333));
#249776=CARTESIAN_POINT('Ctrl Pts',(44.5079524583208,29.87170715524,-42.84995));
#249777=CARTESIAN_POINT('Ctrl Pts',(45.4714029967,29.87170715524,-42.7916166666667));
#249778=CARTESIAN_POINT('Ctrl Pts',(45.9531282658897,30.7060797967663,-42.7332833333334));
#249779=CARTESIAN_POINT('Ctrl Pts',(46.4348535350793,31.5404524382925,-42.67495));
#249780=CARTESIAN_POINT('Ctrl Pts',(45.9531282658897,32.3748250798187,-42.6166166666667));
#249781=CARTESIAN_POINT('Ctrl Pts',(45.4714029967,33.2091977213449,-42.5582833333333));
#249782=CARTESIAN_POINT('Ctrl Pts',(44.5079524583208,33.2091977213449,-42.49995));
#249783=CARTESIAN_POINT('Ctrl Pts',(43.5445019199415,33.2091977213449,-42.4416166666667));
#249784=CARTESIAN_POINT('Ctrl Pts',(43.0627766507519,32.3748250798187,-42.3832833333333));
#249785=CARTESIAN_POINT('Ctrl Pts',(42.5810513815623,31.5404524382925,-42.32495));
#249786=CARTESIAN_POINT('Ctrl Pts',(43.0627766507519,30.7060797967663,-42.2666166666667));
#249787=CARTESIAN_POINT('Ctrl Pts',(43.5445019199415,29.87170715524,-42.2082833333333));
#249788=CARTESIAN_POINT('Ctrl Pts',(44.5079524583208,29.87170715524,-42.14995));
#249789=CARTESIAN_POINT('Ctrl Pts',(45.4714029967,29.87170715524,-42.0916166666667));
#249790=CARTESIAN_POINT('Ctrl Pts',(45.9531282658897,30.7060797967663,-42.0332833333334));
#249791=CARTESIAN_POINT('Ctrl Pts',(46.4348535350793,31.5404524382925,-41.97495));
#249792=CARTESIAN_POINT('Ctrl Pts',(45.9531282658897,32.3748250798187,-41.9166166666666));
#249793=CARTESIAN_POINT('Ctrl Pts',(45.4714029967,33.2091977213449,-41.8582833333333));
#249794=CARTESIAN_POINT('Ctrl Pts',(44.5079524583208,33.2091977213449,-41.79995));
#249795=CARTESIAN_POINT('Ctrl Pts',(43.5445019199415,33.2091977213449,-41.7416166666667));
#249796=CARTESIAN_POINT('Ctrl Pts',(43.0627766507519,32.3748250798187,-41.6832833333333));
#249797=CARTESIAN_POINT('Ctrl Pts',(42.5810513815623,31.5404524382925,-41.62495));
#249798=CARTESIAN_POINT('Ctrl Pts',(43.0627766507519,30.7060797967663,-41.5666166666667));
#249799=CARTESIAN_POINT('Ctrl Pts',(43.5445019199415,29.87170715524,-41.5082833333334));
#249800=CARTESIAN_POINT('Ctrl Pts',(44.5079524583208,29.87170715524,-41.44995));
#249801=CARTESIAN_POINT('Ctrl Pts',(45.4714029967,29.87170715524,-41.3916166666667));
#249802=CARTESIAN_POINT('Ctrl Pts',(45.9531282658897,30.7060797967663,-41.3332833333334));
#249803=CARTESIAN_POINT('Ctrl Pts',(46.4348535350793,31.5404524382925,-41.27495));
#249804=CARTESIAN_POINT('Ctrl Pts',(45.9531282658897,32.3748250798187,-41.2166166666667));
#249805=CARTESIAN_POINT('Ctrl Pts',(45.4714029967,33.2091977213449,-41.1582833333333));
#249806=CARTESIAN_POINT('Ctrl Pts',(44.5079524583208,33.2091977213449,-41.09995));
#249807=CARTESIAN_POINT('Ctrl Pts',(43.5445019199415,33.2091977213449,-41.0416166666667));
#249808=CARTESIAN_POINT('Ctrl Pts',(43.0627766507519,32.3748250798187,-40.9832833333333));
#249809=CARTESIAN_POINT('Ctrl Pts',(42.5810513815623,31.5404524382925,-40.92495));
#249810=CARTESIAN_POINT('Ctrl Pts',(43.0627766507519,30.7060797967663,-40.8666166666667));
#249811=CARTESIAN_POINT('Ctrl Pts',(43.5445019199415,29.87170715524,-40.8082833333334));
#249812=CARTESIAN_POINT('Ctrl Pts',(44.5079524583208,29.87170715524,-40.74995));
#249813=CARTESIAN_POINT('Ctrl Pts',(45.4714029967,29.87170715524,-40.6916166666667));
#249814=CARTESIAN_POINT('Ctrl Pts',(45.9531282658897,30.7060797967663,-40.6332833333334));
#249815=CARTESIAN_POINT('Ctrl Pts',(46.4348535350793,31.5404524382925,-40.57495));
#249816=CARTESIAN_POINT('Ctrl Pts',(45.9531282658897,32.3748250798187,-40.5166166666666));
#249817=CARTESIAN_POINT('Ctrl Pts',(45.4714029967,33.2091977213449,-40.4582833333333));
#249818=CARTESIAN_POINT('Ctrl Pts',(44.5079524583208,33.2091977213449,-40.39995));
#249819=CARTESIAN_POINT('Ctrl Pts',(43.5445019199415,33.2091977213449,-40.3416166666667));
#249820=CARTESIAN_POINT('Ctrl Pts',(43.0627766507519,32.3748250798187,-40.2832833333334));
#249821=CARTESIAN_POINT('Ctrl Pts',(42.5810513815623,31.5404524382925,-40.22495));
#249822=CARTESIAN_POINT('Ctrl Pts',(43.0627766507519,30.7060797967663,-40.1666166666667));
#249823=CARTESIAN_POINT('Ctrl Pts',(43.5445019199415,29.87170715524,-40.1082833333334));
#249824=CARTESIAN_POINT('Ctrl Pts',(44.5079524583208,29.87170715524,-40.04995));
#249825=CARTESIAN_POINT('Ctrl Pts',(45.4714029967,29.87170715524,-39.9916166666667));
#249826=CARTESIAN_POINT('Ctrl Pts',(45.9531282658897,30.7060797967663,-39.9332833333333));
#249827=CARTESIAN_POINT('Ctrl Pts',(46.4348535350793,31.5404524382925,-39.87495));
#249828=CARTESIAN_POINT('Ctrl Pts',(45.9531282658897,32.3748250798187,-39.8166166666667));
#249829=CARTESIAN_POINT('Ctrl Pts',(45.4714029967,33.2091977213449,-39.7582833333334));
#249830=CARTESIAN_POINT('Ctrl Pts',(44.5079524583208,33.2091977213449,-39.69995));
#249831=CARTESIAN_POINT('Ctrl Pts',(43.5445019199415,33.2091977213449,-39.6416166666667));
#249832=CARTESIAN_POINT('Ctrl Pts',(43.0627766507519,32.3748250798187,-39.5832833333333));
#249833=CARTESIAN_POINT('Ctrl Pts',(42.5810513815623,31.5404524382925,-39.52495));
#249834=CARTESIAN_POINT('Ctrl Pts',(43.0627766507519,30.7060797967663,-39.4666166666667));
#249835=CARTESIAN_POINT('Ctrl Pts',(43.5445019199415,29.87170715524,-39.4082833333333));
#249836=CARTESIAN_POINT('Ctrl Pts',(44.5079524583208,29.87170715524,-39.34995));
#249837=CARTESIAN_POINT('Ctrl Pts',(45.4714029967,29.87170715524,-39.2916166666667));
#249838=CARTESIAN_POINT('Ctrl Pts',(45.9531282658897,30.7060797967663,-39.2332833333333));
#249839=CARTESIAN_POINT('Ctrl Pts',(46.4348535350793,31.5404524382925,-39.17495));
#249840=CARTESIAN_POINT('Ctrl Pts',(45.9531282658897,32.3748250798187,-39.1166166666667));
#249841=CARTESIAN_POINT('Ctrl Pts',(45.4714029967,33.2091977213449,-39.0582833333333));
#249842=CARTESIAN_POINT('Ctrl Pts',(44.5079524583208,33.2091977213449,-38.99995));
#249843=CARTESIAN_POINT('Ctrl Pts',(43.5445019199415,33.2091977213449,-38.9416166666667));
#249844=CARTESIAN_POINT('Ctrl Pts',(43.0627766507519,32.3748250798187,-38.8832833333334));
#249845=CARTESIAN_POINT('Ctrl Pts',(42.5810513815623,31.5404524382925,-38.82495));
#249846=CARTESIAN_POINT('Ctrl Pts',(43.0627766507519,30.7060797967663,-38.7666166666667));
#249847=CARTESIAN_POINT('Ctrl Pts',(43.5445019199415,29.87170715524,-38.7082833333333));
#249848=CARTESIAN_POINT('Ctrl Pts',(44.5079524583208,29.87170715524,-38.64995));
#249849=CARTESIAN_POINT('Ctrl Pts',(45.4714029967,29.87170715524,-38.5916166666667));
#249850=CARTESIAN_POINT('Ctrl Pts',(45.9531282658897,30.7060797967663,-38.5332833333334));
#249851=CARTESIAN_POINT('Ctrl Pts',(46.4348535350793,31.5404524382925,-38.47495));
#249852=CARTESIAN_POINT('Ctrl Pts',(45.9531282658897,32.3748250798187,-38.4166166666667));
#249853=CARTESIAN_POINT('Ctrl Pts',(45.4714029967,33.2091977213449,-38.3582833333333));
#249854=CARTESIAN_POINT('Ctrl Pts',(44.5079524583208,33.2091977213449,-38.29995));
#249855=CARTESIAN_POINT('Ctrl Pts',(43.5445019199415,33.2091977213449,-38.2416166666667));
#249856=CARTESIAN_POINT('Ctrl Pts',(43.0627766507519,32.3748250798187,-38.1832833333333));
#249857=CARTESIAN_POINT('Ctrl Pts',(42.5810513815623,31.5404524382925,-38.12495));
#249858=CARTESIAN_POINT('Ctrl Pts',(43.0627766507519,30.7060797967663,-38.0666166666667));
#249859=CARTESIAN_POINT('Ctrl Pts',(43.5445019199415,29.87170715524,-38.0082833333333));
#249860=CARTESIAN_POINT('Ctrl Pts',(44.5079524583208,29.87170715524,-37.94995));
#249861=CARTESIAN_POINT('Ctrl Pts',(45.4714029967,29.87170715524,-37.8916166666667));
#249862=CARTESIAN_POINT('Ctrl Pts',(45.9531282658897,30.7060797967663,-37.8332833333334));
#249863=CARTESIAN_POINT('Ctrl Pts',(46.4348535350793,31.5404524382925,-37.77495));
#249864=CARTESIAN_POINT('Ctrl Pts',(45.9531282658897,32.3748250798187,-37.7166166666667));
#249865=CARTESIAN_POINT('Ctrl Pts',(45.4714029967,33.2091977213449,-37.6582833333333));
#249866=CARTESIAN_POINT('Ctrl Pts',(44.5079524583208,33.2091977213449,-37.59995));
#249867=CARTESIAN_POINT('Ctrl Pts',(43.5445019199415,33.2091977213449,-37.5416166666667));
#249868=CARTESIAN_POINT('Ctrl Pts',(43.0627766507519,32.3748250798187,-37.4832833333334));
#249869=CARTESIAN_POINT('Ctrl Pts',(42.5810513815623,31.5404524382925,-37.42495));
#249870=CARTESIAN_POINT('Ctrl Pts',(43.0627766507519,30.7060797967663,-37.3666166666667));
#249871=CARTESIAN_POINT('Ctrl Pts',(43.5445019199415,29.87170715524,-37.3082833333333));
#249872=CARTESIAN_POINT('Ctrl Pts',(44.5079524583208,29.87170715524,-37.24995));
#249873=CARTESIAN_POINT('Ctrl Pts',(45.4714029967,29.87170715524,-37.1916166666667));
#249874=CARTESIAN_POINT('Ctrl Pts',(45.9531282658897,30.7060797967663,-37.1332833333334));
#249875=CARTESIAN_POINT('Ctrl Pts',(46.4348535350793,31.5404524382925,-37.07495));
#249876=CARTESIAN_POINT('Ctrl Pts',(45.9531282658897,32.3748250798187,-37.0166166666667));
#249877=CARTESIAN_POINT('Ctrl Pts',(45.8905850977848,32.4831530246427,-37.0090431559831));
#249878=CARTESIAN_POINT('Ctrl Pts',(45.8125914103809,32.5809465634453,-37.0009024189827));
#249879=CARTESIAN_POINT('Ctrl Pts',(44.5079524583208,33.6091932047179,-53.2308875));
#249880=CARTESIAN_POINT('Ctrl Pts',(43.3135644199415,33.6091932047179,-53.1725541666667));
#249881=CARTESIAN_POINT('Ctrl Pts',(42.7163704007519,32.5748228215052,-53.1142208333334));
#249882=CARTESIAN_POINT('Ctrl Pts',(42.1191763815623,31.5404524382925,-53.0558875000001));
#249883=CARTESIAN_POINT('Ctrl Pts',(42.7163704007519,30.5060820550798,-52.9975541666667));
#249884=CARTESIAN_POINT('Ctrl Pts',(43.3135644199415,29.4717116718671,-52.9392208333334));
#249885=CARTESIAN_POINT('Ctrl Pts',(44.5079524583208,29.4717116718671,-52.8808875));
#249886=CARTESIAN_POINT('Ctrl Pts',(45.7023404967,29.4717116718671,-52.8225541666667));
#249887=CARTESIAN_POINT('Ctrl Pts',(46.2995345158897,30.5060820550798,-52.7642208333334));
#249888=CARTESIAN_POINT('Ctrl Pts',(46.8967285350793,31.5404524382925,-52.7058875));
#249889=CARTESIAN_POINT('Ctrl Pts',(46.2995345158897,32.5748228215052,-52.6475541666667));
#249890=CARTESIAN_POINT('Ctrl Pts',(45.7023404967,33.6091932047179,-52.5892208333333));
#249891=CARTESIAN_POINT('Ctrl Pts',(44.5079524583208,33.6091932047179,-52.5308875));
#249892=CARTESIAN_POINT('Ctrl Pts',(43.3135644199415,33.6091932047179,-52.4725541666667));
#249893=CARTESIAN_POINT('Ctrl Pts',(42.7163704007519,32.5748228215052,-52.4142208333333));
#249894=CARTESIAN_POINT('Ctrl Pts',(42.1191763815623,31.5404524382925,-52.3558875000001));
#249895=CARTESIAN_POINT('Ctrl Pts',(42.7163704007519,30.5060820550798,-52.2975541666667));
#249896=CARTESIAN_POINT('Ctrl Pts',(43.3135644199415,29.4717116718671,-52.2392208333334));
#249897=CARTESIAN_POINT('Ctrl Pts',(44.5079524583208,29.4717116718671,-52.1808875));
#249898=CARTESIAN_POINT('Ctrl Pts',(45.7023404967,29.4717116718671,-52.1225541666667));
#249899=CARTESIAN_POINT('Ctrl Pts',(46.2995345158897,30.5060820550798,-52.0642208333334));
#249900=CARTESIAN_POINT('Ctrl Pts',(46.8967285350793,31.5404524382925,-52.0058875));
#249901=CARTESIAN_POINT('Ctrl Pts',(46.2995345158897,32.5748228215052,-51.9475541666667));
#249902=CARTESIAN_POINT('Ctrl Pts',(45.7023404967,33.6091932047179,-51.8892208333334));
#249903=CARTESIAN_POINT('Ctrl Pts',(44.5079524583208,33.6091932047179,-51.8308875));
#249904=CARTESIAN_POINT('Ctrl Pts',(43.3135644199415,33.6091932047179,-51.7725541666667));
#249905=CARTESIAN_POINT('Ctrl Pts',(42.7163704007519,32.5748228215052,-51.7142208333334));
#249906=CARTESIAN_POINT('Ctrl Pts',(42.1191763815623,31.5404524382925,-51.6558875));
#249907=CARTESIAN_POINT('Ctrl Pts',(42.7163704007519,30.5060820550798,-51.5975541666667));
#249908=CARTESIAN_POINT('Ctrl Pts',(43.3135644199415,29.4717116718671,-51.5392208333333));
#249909=CARTESIAN_POINT('Ctrl Pts',(44.5079524583208,29.4717116718671,-51.4808875));
#249910=CARTESIAN_POINT('Ctrl Pts',(45.7023404967,29.4717116718671,-51.4225541666667));
#249911=CARTESIAN_POINT('Ctrl Pts',(46.2995345158897,30.5060820550798,-51.3642208333334));
#249912=CARTESIAN_POINT('Ctrl Pts',(46.8967285350793,31.5404524382925,-51.3058875));
#249913=CARTESIAN_POINT('Ctrl Pts',(46.2995345158897,32.5748228215052,-51.2475541666667));
#249914=CARTESIAN_POINT('Ctrl Pts',(45.7023404967,33.6091932047179,-51.1892208333333));
#249915=CARTESIAN_POINT('Ctrl Pts',(44.5079524583208,33.6091932047179,-51.1308875));
#249916=CARTESIAN_POINT('Ctrl Pts',(43.3135644199415,33.6091932047179,-51.0725541666667));
#249917=CARTESIAN_POINT('Ctrl Pts',(42.7163704007519,32.5748228215052,-51.0142208333334));
#249918=CARTESIAN_POINT('Ctrl Pts',(42.1191763815623,31.5404524382925,-50.9558875));
#249919=CARTESIAN_POINT('Ctrl Pts',(42.7163704007519,30.5060820550798,-50.8975541666667));
#249920=CARTESIAN_POINT('Ctrl Pts',(43.3135644199415,29.4717116718671,-50.8392208333333));
#249921=CARTESIAN_POINT('Ctrl Pts',(44.5079524583208,29.4717116718671,-50.7808875));
#249922=CARTESIAN_POINT('Ctrl Pts',(45.7023404967,29.4717116718671,-50.7225541666666));
#249923=CARTESIAN_POINT('Ctrl Pts',(46.2995345158897,30.5060820550798,-50.6642208333333));
#249924=CARTESIAN_POINT('Ctrl Pts',(46.8967285350793,31.5404524382925,-50.6058875));
#249925=CARTESIAN_POINT('Ctrl Pts',(46.2995345158897,32.5748228215052,-50.5475541666667));
#249926=CARTESIAN_POINT('Ctrl Pts',(45.7023404967,33.6091932047179,-50.4892208333333));
#249927=CARTESIAN_POINT('Ctrl Pts',(44.5079524583208,33.6091932047179,-50.4308875));
#249928=CARTESIAN_POINT('Ctrl Pts',(43.3135644199415,33.6091932047179,-50.3725541666667));
#249929=CARTESIAN_POINT('Ctrl Pts',(42.7163704007519,32.5748228215052,-50.3142208333334));
#249930=CARTESIAN_POINT('Ctrl Pts',(42.1191763815623,31.5404524382925,-50.2558875));
#249931=CARTESIAN_POINT('Ctrl Pts',(42.7163704007519,30.5060820550798,-50.1975541666667));
#249932=CARTESIAN_POINT('Ctrl Pts',(43.3135644199415,29.4717116718671,-50.1392208333333));
#249933=CARTESIAN_POINT('Ctrl Pts',(44.5079524583208,29.4717116718671,-50.0808875));
#249934=CARTESIAN_POINT('Ctrl Pts',(45.7023404967,29.4717116718671,-50.0225541666667));
#249935=CARTESIAN_POINT('Ctrl Pts',(46.2995345158897,30.5060820550798,-49.9642208333334));
#249936=CARTESIAN_POINT('Ctrl Pts',(46.8967285350793,31.5404524382925,-49.9058875));
#249937=CARTESIAN_POINT('Ctrl Pts',(46.2995345158897,32.5748228215052,-49.8475541666667));
#249938=CARTESIAN_POINT('Ctrl Pts',(45.7023404967,33.6091932047179,-49.7892208333333));
#249939=CARTESIAN_POINT('Ctrl Pts',(44.5079524583208,33.6091932047179,-49.7308875));
#249940=CARTESIAN_POINT('Ctrl Pts',(43.3135644199415,33.6091932047179,-49.6725541666667));
#249941=CARTESIAN_POINT('Ctrl Pts',(42.7163704007519,32.5748228215052,-49.6142208333334));
#249942=CARTESIAN_POINT('Ctrl Pts',(42.1191763815623,31.5404524382925,-49.5558875));
#249943=CARTESIAN_POINT('Ctrl Pts',(42.7163704007519,30.5060820550798,-49.4975541666667));
#249944=CARTESIAN_POINT('Ctrl Pts',(43.3135644199415,29.4717116718671,-49.4392208333333));
#249945=CARTESIAN_POINT('Ctrl Pts',(44.5079524583208,29.4717116718671,-49.3808875));
#249946=CARTESIAN_POINT('Ctrl Pts',(45.7023404967,29.4717116718671,-49.3225541666667));
#249947=CARTESIAN_POINT('Ctrl Pts',(46.2995345158897,30.5060820550798,-49.2642208333334));
#249948=CARTESIAN_POINT('Ctrl Pts',(46.8967285350793,31.5404524382925,-49.2058875));
#249949=CARTESIAN_POINT('Ctrl Pts',(46.2995345158897,32.5748228215052,-49.1475541666667));
#249950=CARTESIAN_POINT('Ctrl Pts',(45.7023404967,33.6091932047179,-49.0892208333333));
#249951=CARTESIAN_POINT('Ctrl Pts',(44.5079524583208,33.6091932047179,-49.0308875));
#249952=CARTESIAN_POINT('Ctrl Pts',(43.3135644199415,33.6091932047179,-48.9725541666667));
#249953=CARTESIAN_POINT('Ctrl Pts',(42.7163704007519,32.5748228215052,-48.9142208333333));
#249954=CARTESIAN_POINT('Ctrl Pts',(42.1191763815623,31.5404524382925,-48.8558875));
#249955=CARTESIAN_POINT('Ctrl Pts',(42.7163704007519,30.5060820550798,-48.7975541666667));
#249956=CARTESIAN_POINT('Ctrl Pts',(43.3135644199415,29.4717116718671,-48.7392208333334));
#249957=CARTESIAN_POINT('Ctrl Pts',(44.5079524583208,29.4717116718671,-48.6808875));
#249958=CARTESIAN_POINT('Ctrl Pts',(45.7023404967,29.4717116718671,-48.6225541666667));
#249959=CARTESIAN_POINT('Ctrl Pts',(46.2995345158897,30.5060820550798,-48.5642208333334));
#249960=CARTESIAN_POINT('Ctrl Pts',(46.8967285350793,31.5404524382925,-48.5058875));
#249961=CARTESIAN_POINT('Ctrl Pts',(46.2995345158897,32.5748228215052,-48.4475541666667));
#249962=CARTESIAN_POINT('Ctrl Pts',(45.7023404967,33.6091932047179,-48.3892208333334));
#249963=CARTESIAN_POINT('Ctrl Pts',(44.5079524583208,33.6091932047179,-48.3308875));
#249964=CARTESIAN_POINT('Ctrl Pts',(43.3135644199415,33.6091932047179,-48.2725541666667));
#249965=CARTESIAN_POINT('Ctrl Pts',(42.7163704007519,32.5748228215052,-48.2142208333334));
#249966=CARTESIAN_POINT('Ctrl Pts',(42.1191763815623,31.5404524382925,-48.1558875));
#249967=CARTESIAN_POINT('Ctrl Pts',(42.7163704007519,30.5060820550798,-48.0975541666667));
#249968=CARTESIAN_POINT('Ctrl Pts',(43.3135644199415,29.4717116718671,-48.0392208333334));
#249969=CARTESIAN_POINT('Ctrl Pts',(44.5079524583208,29.4717116718671,-47.9808875));
#249970=CARTESIAN_POINT('Ctrl Pts',(45.7023404967,29.4717116718671,-47.9225541666667));
#249971=CARTESIAN_POINT('Ctrl Pts',(46.2995345158897,30.5060820550798,-47.8642208333334));
#249972=CARTESIAN_POINT('Ctrl Pts',(46.8967285350793,31.5404524382925,-47.8058875000001));
#249973=CARTESIAN_POINT('Ctrl Pts',(46.2995345158897,32.5748228215052,-47.7475541666667));
#249974=CARTESIAN_POINT('Ctrl Pts',(45.7023404967,33.6091932047179,-47.6892208333334));
#249975=CARTESIAN_POINT('Ctrl Pts',(44.5079524583208,33.6091932047179,-47.6308875));
#249976=CARTESIAN_POINT('Ctrl Pts',(43.3135644199415,33.6091932047179,-47.5725541666667));
#249977=CARTESIAN_POINT('Ctrl Pts',(42.7163704007519,32.5748228215052,-47.5142208333333));
#249978=CARTESIAN_POINT('Ctrl Pts',(42.1191763815623,31.5404524382925,-47.4558875));
#249979=CARTESIAN_POINT('Ctrl Pts',(42.7163704007519,30.5060820550798,-47.3975541666667));
#249980=CARTESIAN_POINT('Ctrl Pts',(43.3135644199415,29.4717116718671,-47.3392208333333));
#249981=CARTESIAN_POINT('Ctrl Pts',(44.5079524583208,29.4717116718671,-47.2808875));
#249982=CARTESIAN_POINT('Ctrl Pts',(45.7023404967,29.4717116718671,-47.2225541666667));
#249983=CARTESIAN_POINT('Ctrl Pts',(46.2995345158897,30.5060820550798,-47.1642208333334));
#249984=CARTESIAN_POINT('Ctrl Pts',(46.8967285350793,31.5404524382925,-47.1058875));
#249985=CARTESIAN_POINT('Ctrl Pts',(46.2995345158897,32.5748228215052,-47.0475541666667));
#249986=CARTESIAN_POINT('Ctrl Pts',(45.7023404967,33.6091932047179,-46.9892208333334));
#249987=CARTESIAN_POINT('Ctrl Pts',(44.5079524583208,33.6091932047179,-46.9308875));
#249988=CARTESIAN_POINT('Ctrl Pts',(43.3135644199415,33.6091932047179,-46.8725541666667));
#249989=CARTESIAN_POINT('Ctrl Pts',(42.7163704007519,32.5748228215052,-46.8142208333334));
#249990=CARTESIAN_POINT('Ctrl Pts',(42.1191763815623,31.5404524382925,-46.7558875));
#249991=CARTESIAN_POINT('Ctrl Pts',(42.7163704007519,30.5060820550798,-46.6975541666667));
#249992=CARTESIAN_POINT('Ctrl Pts',(43.3135644199415,29.4717116718671,-46.6392208333333));
#249993=CARTESIAN_POINT('Ctrl Pts',(44.5079524583208,29.4717116718671,-46.5808875));
#249994=CARTESIAN_POINT('Ctrl Pts',(45.7023404967,29.4717116718671,-46.5225541666667));
#249995=CARTESIAN_POINT('Ctrl Pts',(46.2995345158897,30.5060820550798,-46.4642208333334));
#249996=CARTESIAN_POINT('Ctrl Pts',(46.8967285350793,31.5404524382925,-46.4058875));
#249997=CARTESIAN_POINT('Ctrl Pts',(46.2995345158897,32.5748228215052,-46.3475541666667));
#249998=CARTESIAN_POINT('Ctrl Pts',(45.7023404967,33.6091932047179,-46.2892208333334));
#249999=CARTESIAN_POINT('Ctrl Pts',(44.5079524583208,33.6091932047179,-46.2308875));
#250000=CARTESIAN_POINT('Ctrl Pts',(43.3135644199415,33.6091932047179,-46.1725541666667));
#250001=CARTESIAN_POINT('Ctrl Pts',(42.7163704007519,32.5748228215052,-46.1142208333334));
#250002=CARTESIAN_POINT('Ctrl Pts',(42.1191763815623,31.5404524382925,-46.0558875));
#250003=CARTESIAN_POINT('Ctrl Pts',(42.7163704007519,30.5060820550798,-45.9975541666667));
#250004=CARTESIAN_POINT('Ctrl Pts',(43.3135644199415,29.4717116718671,-45.9392208333333));
#250005=CARTESIAN_POINT('Ctrl Pts',(44.5079524583208,29.4717116718671,-45.8808875));
#250006=CARTESIAN_POINT('Ctrl Pts',(45.7023404967,29.4717116718671,-45.8225541666667));
#250007=CARTESIAN_POINT('Ctrl Pts',(46.2995345158897,30.5060820550798,-45.7642208333334));
#250008=CARTESIAN_POINT('Ctrl Pts',(46.8967285350793,31.5404524382925,-45.7058875));
#250009=CARTESIAN_POINT('Ctrl Pts',(46.2995345158897,32.5748228215052,-45.6475541666667));
#250010=CARTESIAN_POINT('Ctrl Pts',(45.7023404967,33.6091932047179,-45.5892208333333));
#250011=CARTESIAN_POINT('Ctrl Pts',(44.5079524583208,33.6091932047179,-45.5308875));
#250012=CARTESIAN_POINT('Ctrl Pts',(43.3135644199415,33.6091932047179,-45.4725541666667));
#250013=CARTESIAN_POINT('Ctrl Pts',(42.7163704007519,32.5748228215052,-45.4142208333334));
#250014=CARTESIAN_POINT('Ctrl Pts',(42.1191763815623,31.5404524382925,-45.3558875));
#250015=CARTESIAN_POINT('Ctrl Pts',(42.7163704007519,30.5060820550798,-45.2975541666667));
#250016=CARTESIAN_POINT('Ctrl Pts',(43.3135644199415,29.4717116718671,-45.2392208333333));
#250017=CARTESIAN_POINT('Ctrl Pts',(44.5079524583208,29.4717116718671,-45.1808875));
#250018=CARTESIAN_POINT('Ctrl Pts',(45.7023404967,29.4717116718671,-45.1225541666667));
#250019=CARTESIAN_POINT('Ctrl Pts',(46.2995345158897,30.5060820550798,-45.0642208333334));
#250020=CARTESIAN_POINT('Ctrl Pts',(46.8967285350793,31.5404524382925,-45.0058875));
#250021=CARTESIAN_POINT('Ctrl Pts',(46.2995345158897,32.5748228215052,-44.9475541666667));
#250022=CARTESIAN_POINT('Ctrl Pts',(45.7023404967,33.6091932047179,-44.8892208333333));
#250023=CARTESIAN_POINT('Ctrl Pts',(44.5079524583208,33.6091932047179,-44.8308875));
#250024=CARTESIAN_POINT('Ctrl Pts',(43.3135644199415,33.6091932047179,-44.7725541666666));
#250025=CARTESIAN_POINT('Ctrl Pts',(42.7163704007519,32.5748228215052,-44.7142208333334));
#250026=CARTESIAN_POINT('Ctrl Pts',(42.1191763815623,31.5404524382925,-44.6558875));
#250027=CARTESIAN_POINT('Ctrl Pts',(42.7163704007519,30.5060820550798,-44.5975541666667));
#250028=CARTESIAN_POINT('Ctrl Pts',(43.3135644199415,29.4717116718671,-44.5392208333333));
#250029=CARTESIAN_POINT('Ctrl Pts',(44.5079524583208,29.4717116718671,-44.4808875));
#250030=CARTESIAN_POINT('Ctrl Pts',(45.7023404967,29.4717116718671,-44.4225541666667));
#250031=CARTESIAN_POINT('Ctrl Pts',(46.2995345158897,30.5060820550798,-44.3642208333333));
#250032=CARTESIAN_POINT('Ctrl Pts',(46.8967285350793,31.5404524382925,-44.3058875));
#250033=CARTESIAN_POINT('Ctrl Pts',(46.2995345158897,32.5748228215052,-44.2475541666667));
#250034=CARTESIAN_POINT('Ctrl Pts',(45.7023404967,33.6091932047179,-44.1892208333334));
#250035=CARTESIAN_POINT('Ctrl Pts',(44.5079524583208,33.6091932047179,-44.1308875));
#250036=CARTESIAN_POINT('Ctrl Pts',(43.3135644199415,33.6091932047179,-44.0725541666667));
#250037=CARTESIAN_POINT('Ctrl Pts',(42.7163704007519,32.5748228215052,-44.0142208333334));
#250038=CARTESIAN_POINT('Ctrl Pts',(42.1191763815623,31.5404524382925,-43.9558875));
#250039=CARTESIAN_POINT('Ctrl Pts',(42.7163704007519,30.5060820550798,-43.8975541666667));
#250040=CARTESIAN_POINT('Ctrl Pts',(43.3135644199415,29.4717116718671,-43.8392208333333));
#250041=CARTESIAN_POINT('Ctrl Pts',(44.5079524583208,29.4717116718671,-43.7808875));
#250042=CARTESIAN_POINT('Ctrl Pts',(45.7023404967,29.4717116718671,-43.7225541666667));
#250043=CARTESIAN_POINT('Ctrl Pts',(46.2995345158897,30.5060820550798,-43.6642208333334));
#250044=CARTESIAN_POINT('Ctrl Pts',(46.8967285350793,31.5404524382925,-43.6058875));
#250045=CARTESIAN_POINT('Ctrl Pts',(46.2995345158897,32.5748228215052,-43.5475541666667));
#250046=CARTESIAN_POINT('Ctrl Pts',(45.7023404967,33.6091932047179,-43.4892208333333));
#250047=CARTESIAN_POINT('Ctrl Pts',(44.5079524583208,33.6091932047179,-43.4308875));
#250048=CARTESIAN_POINT('Ctrl Pts',(43.3135644199415,33.6091932047179,-43.3725541666667));
#250049=CARTESIAN_POINT('Ctrl Pts',(42.7163704007519,32.5748228215052,-43.3142208333334));
#250050=CARTESIAN_POINT('Ctrl Pts',(42.1191763815623,31.5404524382925,-43.2558875));
#250051=CARTESIAN_POINT('Ctrl Pts',(42.7163704007519,30.5060820550798,-43.1975541666667));
#250052=CARTESIAN_POINT('Ctrl Pts',(43.3135644199415,29.4717116718671,-43.1392208333334));
#250053=CARTESIAN_POINT('Ctrl Pts',(44.5079524583208,29.4717116718671,-43.0808875));
#250054=CARTESIAN_POINT('Ctrl Pts',(45.7023404967,29.4717116718671,-43.0225541666667));
#250055=CARTESIAN_POINT('Ctrl Pts',(46.2995345158897,30.5060820550798,-42.9642208333334));
#250056=CARTESIAN_POINT('Ctrl Pts',(46.8967285350793,31.5404524382925,-42.9058875));
#250057=CARTESIAN_POINT('Ctrl Pts',(46.2995345158897,32.5748228215052,-42.8475541666667));
#250058=CARTESIAN_POINT('Ctrl Pts',(45.7023404967,33.6091932047179,-42.7892208333334));
#250059=CARTESIAN_POINT('Ctrl Pts',(44.5079524583208,33.6091932047179,-42.7308875));
#250060=CARTESIAN_POINT('Ctrl Pts',(43.3135644199415,33.6091932047179,-42.6725541666667));
#250061=CARTESIAN_POINT('Ctrl Pts',(42.7163704007519,32.5748228215052,-42.6142208333334));
#250062=CARTESIAN_POINT('Ctrl Pts',(42.1191763815623,31.5404524382925,-42.5558875));
#250063=CARTESIAN_POINT('Ctrl Pts',(42.7163704007519,30.5060820550798,-42.4975541666667));
#250064=CARTESIAN_POINT('Ctrl Pts',(43.3135644199415,29.4717116718671,-42.4392208333334));
#250065=CARTESIAN_POINT('Ctrl Pts',(44.5079524583208,29.4717116718671,-42.3808875));
#250066=CARTESIAN_POINT('Ctrl Pts',(45.7023404967,29.4717116718671,-42.3225541666667));
#250067=CARTESIAN_POINT('Ctrl Pts',(46.2995345158897,30.5060820550798,-42.2642208333334));
#250068=CARTESIAN_POINT('Ctrl Pts',(46.8967285350793,31.5404524382925,-42.2058875));
#250069=CARTESIAN_POINT('Ctrl Pts',(46.2995345158897,32.5748228215052,-42.1475541666667));
#250070=CARTESIAN_POINT('Ctrl Pts',(45.7023404967,33.6091932047179,-42.0892208333333));
#250071=CARTESIAN_POINT('Ctrl Pts',(44.5079524583208,33.6091932047179,-42.0308875));
#250072=CARTESIAN_POINT('Ctrl Pts',(43.3135644199415,33.6091932047179,-41.9725541666667));
#250073=CARTESIAN_POINT('Ctrl Pts',(42.7163704007519,32.5748228215052,-41.9142208333334));
#250074=CARTESIAN_POINT('Ctrl Pts',(42.1191763815623,31.5404524382925,-41.8558875));
#250075=CARTESIAN_POINT('Ctrl Pts',(42.7163704007519,30.5060820550798,-41.7975541666667));
#250076=CARTESIAN_POINT('Ctrl Pts',(43.3135644199415,29.4717116718671,-41.7392208333333));
#250077=CARTESIAN_POINT('Ctrl Pts',(44.5079524583208,29.4717116718671,-41.6808875));
#250078=CARTESIAN_POINT('Ctrl Pts',(45.7023404967,29.4717116718671,-41.6225541666667));
#250079=CARTESIAN_POINT('Ctrl Pts',(46.2995345158897,30.5060820550798,-41.5642208333334));
#250080=CARTESIAN_POINT('Ctrl Pts',(46.8967285350793,31.5404524382925,-41.5058875));
#250081=CARTESIAN_POINT('Ctrl Pts',(46.2995345158897,32.5748228215052,-41.4475541666667));
#250082=CARTESIAN_POINT('Ctrl Pts',(45.7023404967,33.6091932047179,-41.3892208333333));
#250083=CARTESIAN_POINT('Ctrl Pts',(44.5079524583208,33.6091932047179,-41.3308875));
#250084=CARTESIAN_POINT('Ctrl Pts',(43.3135644199415,33.6091932047179,-41.2725541666667));
#250085=CARTESIAN_POINT('Ctrl Pts',(42.7163704007519,32.5748228215052,-41.2142208333333));
#250086=CARTESIAN_POINT('Ctrl Pts',(42.1191763815623,31.5404524382925,-41.1558875));
#250087=CARTESIAN_POINT('Ctrl Pts',(42.7163704007519,30.5060820550798,-41.0975541666667));
#250088=CARTESIAN_POINT('Ctrl Pts',(43.3135644199415,29.4717116718671,-41.0392208333333));
#250089=CARTESIAN_POINT('Ctrl Pts',(44.5079524583208,29.4717116718671,-40.9808875));
#250090=CARTESIAN_POINT('Ctrl Pts',(45.7023404967,29.4717116718671,-40.9225541666667));
#250091=CARTESIAN_POINT('Ctrl Pts',(46.2995345158897,30.5060820550798,-40.8642208333334));
#250092=CARTESIAN_POINT('Ctrl Pts',(46.8967285350793,31.5404524382925,-40.8058875));
#250093=CARTESIAN_POINT('Ctrl Pts',(46.2995345158897,32.5748228215052,-40.7475541666667));
#250094=CARTESIAN_POINT('Ctrl Pts',(45.7023404967,33.6091932047179,-40.6892208333333));
#250095=CARTESIAN_POINT('Ctrl Pts',(44.5079524583208,33.6091932047179,-40.6308875));
#250096=CARTESIAN_POINT('Ctrl Pts',(43.3135644199415,33.6091932047179,-40.5725541666667));
#250097=CARTESIAN_POINT('Ctrl Pts',(42.7163704007519,32.5748228215052,-40.5142208333333));
#250098=CARTESIAN_POINT('Ctrl Pts',(42.1191763815623,31.5404524382925,-40.4558875));
#250099=CARTESIAN_POINT('Ctrl Pts',(42.7163704007519,30.5060820550798,-40.3975541666667));
#250100=CARTESIAN_POINT('Ctrl Pts',(43.3135644199415,29.4717116718671,-40.3392208333333));
#250101=CARTESIAN_POINT('Ctrl Pts',(44.5079524583208,29.4717116718671,-40.2808875));
#250102=CARTESIAN_POINT('Ctrl Pts',(45.7023404967,29.4717116718671,-40.2225541666667));
#250103=CARTESIAN_POINT('Ctrl Pts',(46.2995345158897,30.5060820550798,-40.1642208333333));
#250104=CARTESIAN_POINT('Ctrl Pts',(46.8967285350793,31.5404524382925,-40.1058875));
#250105=CARTESIAN_POINT('Ctrl Pts',(46.2995345158897,32.5748228215052,-40.0475541666667));
#250106=CARTESIAN_POINT('Ctrl Pts',(45.7023404967,33.6091932047179,-39.9892208333333));
#250107=CARTESIAN_POINT('Ctrl Pts',(44.5079524583208,33.6091932047179,-39.9308875));
#250108=CARTESIAN_POINT('Ctrl Pts',(43.3135644199415,33.6091932047179,-39.8725541666667));
#250109=CARTESIAN_POINT('Ctrl Pts',(42.7163704007519,32.5748228215052,-39.8142208333334));
#250110=CARTESIAN_POINT('Ctrl Pts',(42.1191763815623,31.5404524382925,-39.7558875));
#250111=CARTESIAN_POINT('Ctrl Pts',(42.7163704007519,30.5060820550798,-39.6975541666667));
#250112=CARTESIAN_POINT('Ctrl Pts',(43.3135644199415,29.4717116718671,-39.6392208333334));
#250113=CARTESIAN_POINT('Ctrl Pts',(44.5079524583208,29.4717116718671,-39.5808875));
#250114=CARTESIAN_POINT('Ctrl Pts',(45.7023404967,29.4717116718671,-39.5225541666667));
#250115=CARTESIAN_POINT('Ctrl Pts',(46.2995345158897,30.5060820550798,-39.4642208333333));
#250116=CARTESIAN_POINT('Ctrl Pts',(46.8967285350793,31.5404524382925,-39.4058875));
#250117=CARTESIAN_POINT('Ctrl Pts',(46.2995345158897,32.5748228215052,-39.3475541666667));
#250118=CARTESIAN_POINT('Ctrl Pts',(45.7023404967,33.6091932047179,-39.2892208333334));
#250119=CARTESIAN_POINT('Ctrl Pts',(44.5079524583208,33.6091932047179,-39.2308875));
#250120=CARTESIAN_POINT('Ctrl Pts',(43.3135644199415,33.6091932047179,-39.1725541666667));
#250121=CARTESIAN_POINT('Ctrl Pts',(42.7163704007519,32.5748228215052,-39.1142208333333));
#250122=CARTESIAN_POINT('Ctrl Pts',(42.1191763815623,31.5404524382925,-39.0558875));
#250123=CARTESIAN_POINT('Ctrl Pts',(42.7163704007519,30.5060820550798,-38.9975541666667));
#250124=CARTESIAN_POINT('Ctrl Pts',(43.3135644199415,29.4717116718671,-38.9392208333334));
#250125=CARTESIAN_POINT('Ctrl Pts',(44.5079524583208,29.4717116718671,-38.8808875));
#250126=CARTESIAN_POINT('Ctrl Pts',(45.7023404967,29.4717116718671,-38.8225541666667));
#250127=CARTESIAN_POINT('Ctrl Pts',(46.2995345158897,30.5060820550798,-38.7642208333333));
#250128=CARTESIAN_POINT('Ctrl Pts',(46.8967285350793,31.5404524382925,-38.7058875));
#250129=CARTESIAN_POINT('Ctrl Pts',(46.2995345158897,32.5748228215052,-38.6475541666667));
#250130=CARTESIAN_POINT('Ctrl Pts',(45.7023404967,33.6091932047179,-38.5892208333334));
#250131=CARTESIAN_POINT('Ctrl Pts',(44.5079524583208,33.6091932047179,-38.5308875));
#250132=CARTESIAN_POINT('Ctrl Pts',(43.3135644199415,33.6091932047179,-38.4725541666667));
#250133=CARTESIAN_POINT('Ctrl Pts',(42.7163704007519,32.5748228215052,-38.4142208333334));
#250134=CARTESIAN_POINT('Ctrl Pts',(42.1191763815623,31.5404524382925,-38.3558875));
#250135=CARTESIAN_POINT('Ctrl Pts',(42.7163704007519,30.5060820550798,-38.2975541666667));
#250136=CARTESIAN_POINT('Ctrl Pts',(43.3135644199415,29.4717116718671,-38.2392208333333));
#250137=CARTESIAN_POINT('Ctrl Pts',(44.5079524583208,29.4717116718671,-38.1808875));
#250138=CARTESIAN_POINT('Ctrl Pts',(45.7023404967,29.4717116718671,-38.1225541666667));
#250139=CARTESIAN_POINT('Ctrl Pts',(46.2995345158897,30.5060820550798,-38.0642208333334));
#250140=CARTESIAN_POINT('Ctrl Pts',(46.8967285350793,31.5404524382925,-38.0058875));
#250141=CARTESIAN_POINT('Ctrl Pts',(46.2995345158897,32.5748228215052,-37.9475541666667));
#250142=CARTESIAN_POINT('Ctrl Pts',(45.7023404967,33.6091932047179,-37.8892208333334));
#250143=CARTESIAN_POINT('Ctrl Pts',(44.5079524583208,33.6091932047179,-37.8308875));
#250144=CARTESIAN_POINT('Ctrl Pts',(43.3135644199415,33.6091932047179,-37.7725541666667));
#250145=CARTESIAN_POINT('Ctrl Pts',(42.7163704007519,32.5748228215052,-37.7142208333333));
#250146=CARTESIAN_POINT('Ctrl Pts',(42.1191763815623,31.5404524382925,-37.6558875));
#250147=CARTESIAN_POINT('Ctrl Pts',(42.7163704007519,30.5060820550798,-37.5975541666667));
#250148=CARTESIAN_POINT('Ctrl Pts',(43.3135644199415,29.4717116718671,-37.5392208333334));
#250149=CARTESIAN_POINT('Ctrl Pts',(44.5079524583208,29.4717116718671,-37.4808875));
#250150=CARTESIAN_POINT('Ctrl Pts',(45.7023404967,29.4717116718671,-37.4225541666667));
#250151=CARTESIAN_POINT('Ctrl Pts',(46.2995345158897,30.5060820550798,-37.3642208333333));
#250152=CARTESIAN_POINT('Ctrl Pts',(46.8967285350793,31.5404524382925,-37.3058875));
#250153=CARTESIAN_POINT('Ctrl Pts',(46.2995345158897,32.5748228215052,-37.2475541666667));
#250154=CARTESIAN_POINT('Ctrl Pts',(46.2219998538691,32.7091167954726,-37.239980655983));
#250155=CARTESIAN_POINT('Ctrl Pts',(46.1253112086366,32.8303512837246,-37.2318399189827));
#250156=CARTESIAN_POINT('Ctrl Pts',(42.546543395006,31.1494605775565,-38.993392163361));
#250157=CARTESIAN_POINT('Ctrl Pts',(42.5576587142752,31.0937006569123,-38.9901394976073));
#250158=CARTESIAN_POINT('Ctrl Pts',(42.5711087182558,31.0386518233917,-38.9869283124078));
#250159=CARTESIAN_POINT('Ctrl Pts',(42.586750690162,30.9845892824225,-38.9837746614135));
#250160=CARTESIAN_POINT('Ctrl Pts',(42.602479569683,30.9302263671454,-38.9806034885691));
#250161=CARTESIAN_POINT('Ctrl Pts',(42.6204243147379,30.8768612681174,-38.977490522151));
#250162=CARTESIAN_POINT('Ctrl Pts',(42.6403992722336,30.8247394146376,-38.9744500788686));
#250163=CARTESIAN_POINT('Ctrl Pts',(42.6606375885134,30.7719303633021,-38.9713695490206));
#250164=CARTESIAN_POINT('Ctrl Pts',(42.6829593947816,30.7203979979648,-38.968363493014));
#250165=CARTESIAN_POINT('Ctrl Pts',(42.7071386920132,30.6703548651506,-38.9654443093952));
#250166=CARTESIAN_POINT('Ctrl Pts',(42.7286485792856,30.6258365263719,-38.9628474055247));
#250167=CARTESIAN_POINT('Ctrl Pts',(42.7516276640965,30.5824962164819,-38.9603192203944));
#250168=CARTESIAN_POINT('Ctrl Pts',(42.7759016507519,30.5404524382925,-38.9578666666667));
#250169=CARTESIAN_POINT('Ctrl Pts',(42.8032592290852,30.4930677226471,-38.9551025582541));
#250170=CARTESIAN_POINT('Ctrl Pts',(42.8328663425998,30.4462838661656,-38.9522423299495));
#250171=CARTESIAN_POINT('Ctrl Pts',(42.8646979426783,30.4004021978905,-38.9492960373434));
#250172=CARTESIAN_POINT('Ctrl Pts',(42.8962082750338,30.3549836008737,-38.9463794808711));
#250173=CARTESIAN_POINT('Ctrl Pts',(42.9298985291123,30.310449779292,-38.9433786035812));
#250174=CARTESIAN_POINT('Ctrl Pts',(42.9656935238546,30.2670957569757,-38.9403058097603));
#250175=CARTESIAN_POINT('Ctrl Pts',(43.0010929508448,30.2242208366478,-38.9372669731492));
#250176=CARTESIAN_POINT('Ctrl Pts',(43.0385507803684,30.1825004955475,-38.9341578253332));
#250177=CARTESIAN_POINT('Ctrl Pts',(43.0779440423292,30.1422122201699,-38.9309926733074));
#250178=CARTESIAN_POINT('Ctrl Pts',(43.1171238614532,30.1021422370424,-38.9278446708903));
#250179=CARTESIAN_POINT('Ctrl Pts',(43.1582179876216,30.0634895370743,-38.9246413003028));
#250180=CARTESIAN_POINT('Ctrl Pts',(43.2010575102137,30.026508792424,-38.9213985239789));
#250181=CARTESIAN_POINT('Ctrl Pts',(43.2436909155241,29.9897059762402,-38.9181713498887));
#250182=CARTESIAN_POINT('Ctrl Pts',(43.2880525876963,29.9545596919455,-38.914905185536));
#250183=CARTESIAN_POINT('Ctrl Pts',(43.3339328063802,29.9212928582627,-38.9116171288744));
#250184=CARTESIAN_POINT('Ctrl Pts',(43.3596308718016,29.9026597023435,-38.9097754485681));
#250185=CARTESIAN_POINT('Ctrl Pts',(43.3858045938695,29.8846156169163,-38.9079269216165));
#250186=CARTESIAN_POINT('Ctrl Pts',(43.4124119307855,29.8671948409963,-38.9060746707971));
#250187=CARTESIAN_POINT('Origin',(44.5079524583208,31.5404524382925,235.35105));
#250188=CARTESIAN_POINT('',(44.236619467102,29.5589435596493,-39.0141960675245));
#250189=CARTESIAN_POINT('Ctrl Pts',(43.4124119245055,29.8671948319696,-38.9060746716112));
#250190=CARTESIAN_POINT('Ctrl Pts',(43.4347318263428,29.8525811285912,-38.9076953057508));
#250191=CARTESIAN_POINT('Ctrl Pts',(43.4574472657287,29.8383464180801,-38.9094785669247));
#250192=CARTESIAN_POINT('Ctrl Pts',(43.4805657277221,29.8245047392673,-38.9114288083032));
#250193=CARTESIAN_POINT('Ctrl Pts',(43.5088609654949,29.807563577987,-38.913815755304));
#250194=CARTESIAN_POINT('Ctrl Pts',(43.5377748005682,29.7912042828046,-38.9164545150156));
#250195=CARTESIAN_POINT('Ctrl Pts',(43.5672796770166,29.7754780139697,-38.919349653254));
#250196=CARTESIAN_POINT('Ctrl Pts',(43.5965174949706,29.7598940888484,-38.922218586629));
#250197=CARTESIAN_POINT('Ctrl Pts',(43.6264809533112,29.7448658896409,-38.9253559403288));
#250198=CARTESIAN_POINT('Ctrl Pts',(43.6567606170124,29.7306258031448,-38.9287240628826));
#250199=CARTESIAN_POINT('Ctrl Pts',(43.6867773203878,29.7165093830744,-38.9320629353557));
#250200=CARTESIAN_POINT('Ctrl Pts',(43.7171486731233,29.7031357677765,-38.9356311637963));
#250201=CARTESIAN_POINT('Ctrl Pts',(43.74787091788,29.6905129658013,-38.9394291519851));
#250202=CARTESIAN_POINT('Ctrl Pts',(43.7783370856922,29.6779953777707,-38.9431954830728));
#250203=CARTESIAN_POINT('Ctrl Pts',(43.8091488314015,29.6662150049623,-38.9471876300055));
#250204=CARTESIAN_POINT('Ctrl Pts',(43.8403053963098,29.655181264008,-38.9514068723595));
#250205=CARTESIAN_POINT('Ctrl Pts',(43.8712126325087,29.6442358199631,-38.9555923504569));
#250206=CARTESIAN_POINT('Ctrl Pts',(43.9024591937255,29.6340251151907,-38.96000130694));
#250207=CARTESIAN_POINT('Ctrl Pts',(43.9340457277949,29.6245633327707,-38.9646362624899));
#250208=CARTESIAN_POINT('Ctrl Pts',(43.9653895268376,29.6151742619057,-38.9692355995052));
#250209=CARTESIAN_POINT('Ctrl Pts',(43.9970680900916,29.6065226347007,-38.9740574728663));
#250210=CARTESIAN_POINT('Ctrl Pts',(44.0290834665269,29.5986273975902,-38.9791056375968));
#250211=CARTESIAN_POINT('Ctrl Pts',(44.0608625364734,29.5907904354703,-38.9841165416665));
#250212=CARTESIAN_POINT('Ctrl Pts',(44.0929734563391,29.5836987046376,-38.9893504007192));
#250213=CARTESIAN_POINT('Ctrl Pts',(44.1254197237287,29.5773761007637,-38.9948122462768));
#250214=CARTESIAN_POINT('Ctrl Pts',(44.1576359403445,29.5710983254643,-39.000235366215));
#250215=CARTESIAN_POINT('Ctrl Pts',(44.1901665881168,29.5655813086992,-39.0058803943283));
#250216=CARTESIAN_POINT('Ctrl Pts',(44.2230652009806,29.5608466061619,-39.0117622591756));
#250217=CARTESIAN_POINT('Ctrl Pts',(44.2275783635669,29.5601970808328,-39.012569156794));
#250218=CARTESIAN_POINT('Ctrl Pts',(44.2320969536309,29.5595625845471,-39.0133802622792));
#250219=CARTESIAN_POINT('Ctrl Pts',(44.2366193326589,29.5589433410896,-39.0141952785063));
#250220=CARTESIAN_POINT('',(42.5996219947327,32.1390102378578,-39.2098645096971));
#250221=CARTESIAN_POINT('Ctrl Pts',(44.2366191251681,29.5589433654202,-39.0141965786228));
#250222=CARTESIAN_POINT('Ctrl Pts',(44.1816176782784,29.566474982975,-39.0171948894326));
#250223=CARTESIAN_POINT('Ctrl Pts',(44.1264789676119,29.5763621734674,-39.0202688267391));
#250224=CARTESIAN_POINT('Ctrl Pts',(44.0715029830857,29.588655665456,-39.0234047166939));
#250225=CARTESIAN_POINT('Ctrl Pts',(44.0169261942809,29.6008598910231,-39.0265178360905));
#250226=CARTESIAN_POINT('Ctrl Pts',(43.9625104680952,29.6154358140615,-39.0296919830407));
#250227=CARTESIAN_POINT('Ctrl Pts',(43.9085612350477,29.6323831987791,-39.0329117223836));
#250228=CARTESIAN_POINT('Ctrl Pts',(43.8548976765229,29.6492408429061,-39.0361144124109));
#250229=CARTESIAN_POINT('Ctrl Pts',(43.8016964116104,29.6684449522924,-39.039362178014));
#250230=CARTESIAN_POINT('Ctrl Pts',(43.7492592823951,29.6899437547989,-39.042638262187));
#250231=CARTESIAN_POINT('Ctrl Pts',(43.6969935738813,29.7113722761924,-39.045903636608));
#250232=CARTESIAN_POINT('Ctrl Pts',(43.6454877381092,29.7350803961258,-39.0491971047438));
#250233=CARTESIAN_POINT('Ctrl Pts',(43.595031006667,29.7609659628588,-39.0525010772784));
#250234=CARTESIAN_POINT('Ctrl Pts',(43.5446056724429,29.7868354220326,-39.0558029938822));
#250235=CARTESIAN_POINT('Ctrl Pts',(43.4952288227897,29.8148793433641,-39.0591153591484));
#250236=CARTESIAN_POINT('Ctrl Pts',(43.4471688705001,29.8449477707636,-39.0624202412502));
#250237=CARTESIAN_POINT('Ctrl Pts',(43.3990553382291,29.8750497201644,-39.0657288078234));
#250238=CARTESIAN_POINT('Ctrl Pts',(43.352262246232,29.9071802631789,-39.0690298314617));
#250239=CARTESIAN_POINT('Ctrl Pts',(43.3070288337395,29.9411461158919,-39.072305590473));
#250240=CARTESIAN_POINT('Ctrl Pts',(43.2616662391463,29.9752089716821,-39.0755907047243));
#250241=CARTESIAN_POINT('Ctrl Pts',(43.217872734279,30.011117076979,-39.0788503688593));
#250242=CARTESIAN_POINT('Ctrl Pts',(43.1758511046526,30.0486398807422,-39.0820676158819));
#250243=CARTESIAN_POINT('Ctrl Pts',(43.1334566861023,30.0864955627341,-39.0853134042549));
#250244=CARTESIAN_POINT('Ctrl Pts',(43.0928661024029,30.1259940743276,-39.0885159814558));
#250245=CARTESIAN_POINT('Ctrl Pts',(43.0542417580791,30.1668715695527,-39.0916594494718));
#250246=CARTESIAN_POINT('Ctrl Pts',(43.0153972412906,30.2079820810018,-39.0948208363708));
#250247=CARTESIAN_POINT('Ctrl Pts',(42.9785416250927,30.2504866150729,-39.097922407934));
#250248=CARTESIAN_POINT('Ctrl Pts',(42.9437897138948,30.2940999455835,-39.1009500473225));
#250249=CARTESIAN_POINT('Ctrl Pts',(42.9085853984175,30.3382810393245,-39.1040171008602));
#250250=CARTESIAN_POINT('Ctrl Pts',(42.8755399737454,30.3835992377108,-39.1070082600792));
#250251=CARTESIAN_POINT('Ctrl Pts',(42.844719305314,30.4297520295712,-39.109911376434));
#250252=CARTESIAN_POINT('Ctrl Pts',(42.8203919250237,30.4661813666424,-39.1122028652039));
#250253=CARTESIAN_POINT('Ctrl Pts',(42.7974495117931,30.5031304481747,-39.1144395505765));
#250254=CARTESIAN_POINT('Ctrl Pts',(42.7759016507519,30.5404524382925,-39.1166166666667));
#250255=CARTESIAN_POINT('Ctrl Pts',(42.7485193766326,30.587879928294,-39.1193832702501));
#250256=CARTESIAN_POINT('Ctrl Pts',(42.7227852103423,30.636958193604,-39.1222461931116));
#250257=CARTESIAN_POINT('Ctrl Pts',(42.6989482557022,30.6875143844291,-39.1251953452699));
#250258=CARTESIAN_POINT('Ctrl Pts',(42.6753689155071,30.7375241965227,-39.128112624892));
#250259=CARTESIAN_POINT('Ctrl Pts',(42.6536466666086,30.7889798985313,-39.1311142647052));
#250260=CARTESIAN_POINT('Ctrl Pts',(42.6339995109737,30.8416687077707,-39.1341878453422));
#250261=CARTESIAN_POINT('Ctrl Pts',(42.6145810606266,30.8937441860271,-39.1372256475614));
#250262=CARTESIAN_POINT('Ctrl Pts',(42.5971902480339,30.9470238046399,-39.1403337006506));
#250263=CARTESIAN_POINT('Ctrl Pts',(42.5820056476045,31.0012625948999,-39.143497707743));
#250264=CARTESIAN_POINT('Ctrl Pts',(42.5669082682819,31.0551898348266,-39.1466435406198));
#250265=CARTESIAN_POINT('Ctrl Pts',(42.5539923214714,31.1100647309391,-39.1498446557392));
#250266=CARTESIAN_POINT('Ctrl Pts',(42.5433935917014,31.1656142631698,-39.1530851197771));
#250267=CARTESIAN_POINT('Ctrl Pts',(42.5328373585439,31.2209410642817,-39.156312590867));
#250268=CARTESIAN_POINT('Ctrl Pts',(42.5245801588322,31.2769364683933,-39.159579058983));
#250269=CARTESIAN_POINT('Ctrl Pts',(42.5187102065973,31.3333073354667,-39.1628674169599));
#250270=CARTESIAN_POINT('Ctrl Pts',(42.5128535965813,31.3895500733124,-39.1661483006014));
#250271=CARTESIAN_POINT('Ctrl Pts',(42.5093736002375,31.4461658639795,-39.1694509335672));
#250272=CARTESIAN_POINT('Ctrl Pts',(42.5083077219769,31.502850275984,-39.172757549812));
#250273=CARTESIAN_POINT('Ctrl Pts',(42.5072408681143,31.5595865714247,-39.1760671926139));
#250274=CARTESIAN_POINT('Ctrl Pts',(42.5085926033184,31.6163908743015,-39.1793807828468));
#250275=CARTESIAN_POINT('Ctrl Pts',(42.512348305768,31.6729554658862,-39.1826803624361));
#250276=CARTESIAN_POINT('Ctrl Pts',(42.51610881692,31.7295924812843,-39.1859841667201));
#250277=CARTESIAN_POINT('Ctrl Pts',(42.522279319495,31.785988440723,-39.1892738818491));
#250278=CARTESIAN_POINT('Ctrl Pts',(42.5307934391592,31.841843081299,-39.1925319844119));
#250279=CARTESIAN_POINT('Ctrl Pts',(42.5393585830543,31.8980324529088,-39.1958096124435));
#250280=CARTESIAN_POINT('Ctrl Pts',(42.5502952384567,31.9536733046506,-39.1990552074192));
#250281=CARTESIAN_POINT('Ctrl Pts',(42.5634866283946,32.0084794812234,-39.202252068528));
#250282=CARTESIAN_POINT('Ctrl Pts',(42.5740999898522,32.0525747406936,-39.2048241585532));
#250283=CARTESIAN_POINT('Ctrl Pts',(42.5861718501526,32.0961299612849,-39.2073647175113));
#250284=CARTESIAN_POINT('Ctrl Pts',(42.5996208651864,32.1390094796345,-39.2098658272488));
#250285=CARTESIAN_POINT('Ctrl Pts',(42.5996211287169,32.1390103205417,-39.2098620634844));
#250286=CARTESIAN_POINT('Ctrl Pts',(42.5994572744447,32.1384879169033,-39.2097205819177));
#250287=CARTESIAN_POINT('Ctrl Pts',(42.5992936549467,32.1379655109967,-39.2095791463362));
#250288=CARTESIAN_POINT('Ctrl Pts',(42.599130270052,32.1374431028809,-39.2094377567205));
#250289=CARTESIAN_POINT('Ctrl Pts',(42.5893329175536,32.1061169728464,-39.2009593480741));
#250290=CARTESIAN_POINT('Ctrl Pts',(42.5803770676735,32.0747718601698,-39.1926435115987));
#250291=CARTESIAN_POINT('Ctrl Pts',(42.5722375892794,32.0434514998719,-39.184494909014));
#250292=CARTESIAN_POINT('Ctrl Pts',(42.563947246632,32.0115506204622,-39.1761952730602));
#250293=CARTESIAN_POINT('Ctrl Pts',(42.5564828395702,31.97956241044,-39.1680413954435));
#250294=CARTESIAN_POINT('Ctrl Pts',(42.5498886395242,31.9478668123839,-39.1601218550228));
#250295=CARTESIAN_POINT('Ctrl Pts',(42.5431680501022,31.9155637127605,-39.15205052276));
#250296=CARTESIAN_POINT('Ctrl Pts',(42.5373266000632,31.8834870424314,-39.1442015176493));
#250297=CARTESIAN_POINT('Ctrl Pts',(42.5323124691512,31.8516556037808,-39.1365690002841));
#250298=CARTESIAN_POINT('Ctrl Pts',(42.5271988370559,31.8191924971763,-39.128785022073));
#250299=CARTESIAN_POINT('Ctrl Pts',(42.5229439406764,31.7869791989586,-39.1212247661578));
#250300=CARTESIAN_POINT('Ctrl Pts',(42.5194951584437,31.7550189050201,-39.1138789650356));
#250301=CARTESIAN_POINT('Ctrl Pts',(42.5123805250403,31.6890867122931,-39.0987250125639));
#250302=CARTESIAN_POINT('Ctrl Pts',(42.508690420396,31.6242317713433,-39.0844826612156));
#250303=CARTESIAN_POINT('Ctrl Pts',(42.5080522085159,31.5604742687753,-39.0710861007614));
#250304=CARTESIAN_POINT('Ctrl Pts',(42.5077225703561,31.527543346495,-39.0641667411037));
#250305=CARTESIAN_POINT('Ctrl Pts',(42.5082086866532,31.4949050545532,-39.0574732885357));
#250306=CARTESIAN_POINT('Ctrl Pts',(42.5094692953678,31.4625612862931,-39.050998430158));
#250307=CARTESIAN_POINT('Ctrl Pts',(42.5107590556556,31.4294695684798,-39.0443738406978));
#250308=CARTESIAN_POINT('Ctrl Pts',(42.5128605944209,31.3966833301453,-39.0379776981527));
#250309=CARTESIAN_POINT('Ctrl Pts',(42.5157322592149,31.364212570118,-39.0318042712848));
#250310=CARTESIAN_POINT('Ctrl Pts',(42.518470838614,31.3332466458677,-39.0259169477791));
#250311=CARTESIAN_POINT('Ctrl Pts',(42.5219235433117,31.3025110976608,-39.0202232095696));
#250312=CARTESIAN_POINT('Ctrl Pts',(42.5259998070332,31.2723751844448,-39.0147819750659));
#250313=CARTESIAN_POINT('Ctrl Pts',(42.5263010222903,31.2701482929905,-39.0143798953768));
#250314=CARTESIAN_POINT('Ctrl Pts',(42.5266056457019,31.2679246529169,-39.013979190334));
#250315=CARTESIAN_POINT('Ctrl Pts',(42.5269136422624,31.2657044023431,-39.0135798817453));
#250316=CARTESIAN_POINT('Ctrl Pts',(42.5315025550251,31.2326243699617,-39.007630489726));
#250317=CARTESIAN_POINT('Ctrl Pts',(42.5368513500173,31.2001397627821,-39.0019606799009));
#250318=CARTESIAN_POINT('Ctrl Pts',(42.5428860222013,31.1682775284555,-38.9965615346981));
#250319=CARTESIAN_POINT('Ctrl Pts',(42.5440784696113,31.1619815710881,-38.9954946670181));
#250320=CARTESIAN_POINT('Ctrl Pts',(42.5452977554539,31.1557093015287,-38.9944382514666));
#250321=CARTESIAN_POINT('Ctrl Pts',(42.5465433949858,31.149460577658,-38.9933921633669));
#250322=CARTESIAN_POINT('Ctrl Pts',(46.6981266849492,30.7091523375488,-39.2904704603133));
#250323=CARTESIAN_POINT('Ctrl Pts',(46.6689684123063,30.6404043382273,-39.273452295095));
#250324=CARTESIAN_POINT('Ctrl Pts',(46.6043681216411,30.5066861069553,-39.238925705885));
#250325=CARTESIAN_POINT('Ctrl Pts',(46.5083209189471,30.3487389562033,-39.1945593129175));
#250326=CARTESIAN_POINT('Ctrl Pts',(46.4437937583117,30.2581216171786,-39.1673894861782));
#250327=CARTESIAN_POINT('Ctrl Pts',(46.3992224148768,30.1986447451181,-39.1491520227249));
#250328=CARTESIAN_POINT('Ctrl Pts',(46.3761748773305,30.1693908446446,-39.1399767764946));
#250329=CARTESIAN_POINT('Ctrl Pts',(46.3284414024809,30.1117648114071,-39.1214771434543));
#250330=CARTESIAN_POINT('Ctrl Pts',(46.3038983378397,30.083571828401,-39.112209259666));
#250331=CARTESIAN_POINT('Ctrl Pts',(46.253707387608,30.0286632749651,-39.0937226519629));
#250332=CARTESIAN_POINT('Ctrl Pts',(46.2280147026909,30.001893564456,-39.0844865568113));
#250333=CARTESIAN_POINT('Ctrl Pts',(46.1492148010453,29.9236586721517,-39.0568159196779));
#250334=CARTESIAN_POINT('Ctrl Pts',(46.0669347173688,29.8495134741745,-39.0292038481275));
#250335=CARTESIAN_POINT('Ctrl Pts',(45.9503410384262,29.7587889734315,-38.9925114043613));
#250336=CARTESIAN_POINT('Ctrl Pts',(45.8594191065401,29.6948377475824,-38.9650526418885));
#250337=CARTESIAN_POINT('Ctrl Pts',(45.7964751089327,29.6549785818455,-38.9467936623891));
#250338=CARTESIAN_POINT('Ctrl Pts',(45.748348603817,29.6261284949947,-38.9331097524421));
#250339=CARTESIAN_POINT('Ctrl Pts',(45.7321473284057,29.616684052073,-38.9285487676403));
#250340=CARTESIAN_POINT('Ctrl Pts',(45.6996106203311,29.5982459977232,-38.9194791520014));
#250341=CARTESIAN_POINT('Ctrl Pts',(45.683249044345,29.5892352448745,-38.9149628379356));
#250342=CARTESIAN_POINT('Ctrl Pts',(45.6010439155842,29.5452684013657,-38.8924942188443));
#250343=CARTESIAN_POINT('Ctrl Pts',(45.4667739830181,29.4816584171599,-38.8571935516581));
#250344=CARTESIAN_POINT('Ctrl Pts',(45.2922645146651,29.4187721922835,-38.8147007629208));
#250345=CARTESIAN_POINT('Ctrl Pts',(45.184512437616,29.3885937253944,-38.7899522655792));
#250346=CARTESIAN_POINT('Ctrl Pts',(45.1119891467798,29.3701842541612,-38.7736235920333));
#250347=CARTESIAN_POINT('Ctrl Pts',(45.0754052578815,29.3618381514785,-38.7655490803555));
#250348=CARTESIAN_POINT('Ctrl Pts',(45.0014447932705,29.3468760834356,-38.7495561846596));
#250349=CARTESIAN_POINT('Ctrl Pts',(44.964301863367,29.3403115562353,-38.7416890516424));
#250350=CARTESIAN_POINT('Ctrl Pts',(44.8900079594565,29.3290481892184,-38.726277749838));
#250351=CARTESIAN_POINT('Ctrl Pts',(44.8527936282157,29.324336495618,-38.7187198739728));
#250352=CARTESIAN_POINT('Ctrl Pts',(44.7410083373266,29.3129455735289,-38.6964994820139));
#250353=CARTESIAN_POINT('Ctrl Pts',(44.6662563757167,29.3089967422249,-38.6822807693139));
#250354=CARTESIAN_POINT('Ctrl Pts',(44.516312468428,29.3084067934202,-38.6550493453909));
#250355=CARTESIAN_POINT('Ctrl Pts',(44.441103189525,29.3117700143417,-38.6420342479066));
#250356=CARTESIAN_POINT('Ctrl Pts',(44.3468378615956,29.3206690055189,-38.6265520162729));
#250357=CARTESIAN_POINT('Ctrl Pts',(44.3279589148655,29.3226883315868,-38.6234933649988));
#250358=CARTESIAN_POINT('Ctrl Pts',(44.2901960653062,29.3271995080042,-38.6174591262491));
#250359=CARTESIAN_POINT('Ctrl Pts',(44.271274393292,29.329697893027,-38.614477863833));
#250360=CARTESIAN_POINT('Ctrl Pts',(44.2146592782019,29.3378915995821,-38.60568558559));
#250361=CARTESIAN_POINT('Ctrl Pts',(44.1772069502033,29.344266758826,-38.6000392683017));
#250362=CARTESIAN_POINT('Ctrl Pts',(44.0655444875092,29.3661148598052,-38.5837127379559));
#250363=CARTESIAN_POINT('Ctrl Pts',(43.9553791862171,29.3933792052515,-38.5686255047386));
#250364=CARTESIAN_POINT('Ctrl Pts',(43.8114622524781,29.4404829778103,-38.5509833019505));
#250365=CARTESIAN_POINT('Ctrl Pts',(43.705021834675,29.481230340464,-38.5390021142185));
#250366=CARTESIAN_POINT('Ctrl Pts',(43.6350719757086,29.512061063653,-38.5318621614261));
#250367=CARTESIAN_POINT('Ctrl Pts',(43.5656410085295,29.5447591316771,-38.525155654825));
#250368=CARTESIAN_POINT('Ctrl Pts',(43.5311320054746,29.5620794464364,-38.5220163122062));
#250369=CARTESIAN_POINT('Ctrl Pts',(43.4634866412134,29.5981758355574,-38.5162526847879));
#250370=CARTESIAN_POINT('Ctrl Pts',(43.4301834663392,29.6170276546,-38.5136117755133));
#250371=CARTESIAN_POINT('Ctrl Pts',(43.3647025891651,29.6562685687332,-38.5088155315793));
#250372=CARTESIAN_POINT('Ctrl Pts',(43.2681192378476,29.7174608121974,-38.5023448938576));
#250373=CARTESIAN_POINT('Ctrl Pts',(43.1764049274077,29.7855824582168,-38.4980286134812));
#250374=CARTESIAN_POINT('Ctrl Pts',(43.0584774180437,29.8826126224142,-38.4942050936184));
#250375=CARTESIAN_POINT('Ctrl Pts',(43.001681818637,29.9342392650769,-38.4932590761897));
#250376=CARTESIAN_POINT('Ctrl Pts',(42.8926599718677,30.0438904492243,-38.4933742455196));
#250377=CARTESIAN_POINT('Ctrl Pts',(42.8414047150844,30.1009342501745,-38.4944336470273));
#250378=CARTESIAN_POINT('Ctrl Pts',(42.7451036203247,30.2193471227021,-38.498479276642));
#250379=CARTESIAN_POINT('Ctrl Pts',(42.6550322643363,30.3420646399833,-38.5044516702661));
#250380=CARTESIAN_POINT('Ctrl Pts',(42.5773225406025,30.4733365238586,-38.5142428327574));
#250381=CARTESIAN_POINT('Ctrl Pts',(42.5326943378214,30.5580963840027,-38.5215739479982));
#250382=CARTESIAN_POINT('Ctrl Pts',(42.5239673850246,30.5751883092729,-38.5231018165939));
#250383=CARTESIAN_POINT('Ctrl Pts',(42.5069121510755,30.60964376351,-38.5262794637242));
#250384=CARTESIAN_POINT('Ctrl Pts',(42.4985805781952,30.627019094627,-38.5279307934181));
#250385=CARTESIAN_POINT('Ctrl Pts',(42.4743295471271,30.6792614198295,-38.5330409224498));
#250386=CARTESIAN_POINT('Ctrl Pts',(42.4438856226513,30.7493896366731,-38.5402834483744));
#250387=CARTESIAN_POINT('Ctrl Pts',(42.4037483179465,30.8560072598611,-38.5524071291592));
#250388=CARTESIAN_POINT('Ctrl Pts',(42.3690543371876,30.9640160484273,-38.5657659376104));
#250389=CARTESIAN_POINT('Ctrl Pts',(42.3397558527982,31.0734075527136,-38.5803463747351));
#250390=CARTESIAN_POINT('Ctrl Pts',(42.3238156343608,31.1472555030051,-38.5908775753381));
#250391=CARTESIAN_POINT('Ctrl Pts',(42.3096820427396,31.2215665449467,-38.6018154236264));
#250392=CARTESIAN_POINT('Ctrl Pts',(42.3035171869091,31.2589715314082,-38.6074906718877));
#250393=CARTESIAN_POINT('Ctrl Pts',(42.2930235524414,31.3341791410138,-38.6192399292287));
#250394=CARTESIAN_POINT('Ctrl Pts',(42.2886818075092,31.3721585359098,-38.6253436316658));
#250395=CARTESIAN_POINT('Ctrl Pts',(42.281930630611,31.4478003630713,-38.6378362101326));
#250396=CARTESIAN_POINT('Ctrl Pts',(42.277074994566,31.5232809912004,-38.6506356205751));
#250397=CARTESIAN_POINT('Ctrl Pts',(42.2747992363309,31.6735553614761,-38.6774229397946));
#250398=CARTESIAN_POINT('Ctrl Pts',(42.2834818483937,31.8228397562226,-38.7059581415094));
#250399=CARTESIAN_POINT('Ctrl Pts',(42.3030248127084,31.9711385758679,-38.7362097844166));
#250400=CARTESIAN_POINT('Ctrl Pts',(42.3164494406915,32.0449687602614,-38.7519128032936));
#250401=CARTESIAN_POINT('Ctrl Pts',(42.3317154579634,32.1186122141692,-38.7679009120377));
#250402=CARTESIAN_POINT('Ctrl Pts',(42.3402956643805,32.1554227583218,-38.7760569897633));
#250403=CARTESIAN_POINT('Ctrl Pts',(42.3591481714288,32.228169160774,-38.7925026060078));
#250404=CARTESIAN_POINT('Ctrl Pts',(42.3694448348212,32.2642362896146,-38.8008201507359));
#250405=CARTESIAN_POINT('Ctrl Pts',(42.4028917825415,32.3714169561226,-38.8260275044574));
#250406=CARTESIAN_POINT('Ctrl Pts',(42.428602574983,32.4415633880281,-38.8431823298655));
#250407=CARTESIAN_POINT('Ctrl Pts',(42.4722685042023,32.5448307979217,-38.8694323201497));
#250408=CARTESIAN_POINT('Ctrl Pts',(42.4876674804306,32.5789105800712,-38.8782643966373));
#250409=CARTESIAN_POINT('Ctrl Pts',(42.5202146590728,32.6464795812123,-38.8961197808447));
#250410=CARTESIAN_POINT('Ctrl Pts',(42.5373018269229,32.6798350022668,-38.9051083126545));
#250411=CARTESIAN_POINT('Ctrl Pts',(42.5906929412925,32.7780783962456,-38.9321048428364));
#250412=CARTESIAN_POINT('Ctrl Pts',(42.629225789877,32.8414173722334,-38.9502105255135));
#250413=CARTESIAN_POINT('Ctrl Pts',(42.7120000069194,32.9638220552461,-38.9866125955294));
#250414=CARTESIAN_POINT('Ctrl Pts',(42.7783647966162,33.0524402968179,-39.0140612314234));
#250415=CARTESIAN_POINT('Ctrl Pts',(42.8754380724448,33.1642175243331,-39.0509520337677));
#250416=CARTESIAN_POINT('Ctrl Pts',(42.9268673384212,33.2179450225078,-39.0694937486382));
#250417=CARTESIAN_POINT('Ctrl Pts',(42.9797817061918,33.2705900457306,-39.088089881442));
#250418=CARTESIAN_POINT('Ctrl Pts',(43.0069972096607,33.2963736994336,-39.097418269769));
#250419=CARTESIAN_POINT('Ctrl Pts',(43.0622936398443,33.3462615369726,-39.1159154063528));
#250420=CARTESIAN_POINT('Ctrl Pts',(43.0904949946047,33.3704876748183,-39.1251268688783));
#250421=CARTESIAN_POINT('Ctrl Pts',(43.176562606447,33.4408730143712,-39.1525915568785));
#250422=CARTESIAN_POINT('Ctrl Pts',(43.2360245534179,33.4848790444095,-39.1707230137558));
#250423=CARTESIAN_POINT('Ctrl Pts',(43.358992255749,33.5670176609587,-39.2066046432507));
#250424=CARTESIAN_POINT('Ctrl Pts',(43.4542745623933,33.6242424638975,-39.233238623837));
#250425=CARTESIAN_POINT('Ctrl Pts',(43.5542222374601,33.6747516510336,-39.2594493821381));
#250426=CARTESIAN_POINT('Ctrl Pts',(43.6219256430316,33.7069073870393,-39.2768314299875));
#250427=CARTESIAN_POINT('Ctrl Pts',(43.6563381479934,33.7222286468184,-39.2854811722856));
#250428=CARTESIAN_POINT('Ctrl Pts',(43.7254519170511,33.7509934760635,-39.3024907499371));
#250429=CARTESIAN_POINT('Ctrl Pts',(43.7602995448845,33.7645084608315,-39.3108885064059));
#250430=CARTESIAN_POINT('Ctrl Pts',(43.8304781084082,33.789780836939,-39.3274499785309));
#250431=CARTESIAN_POINT('Ctrl Pts',(43.9365171946568,33.8250735562425,-39.3519527568515));
#250432=CARTESIAN_POINT('Ctrl Pts',(44.0809642638621,33.8617420360433,-39.3832806139221));
#250433=CARTESIAN_POINT('Ctrl Pts',(44.1916183723467,33.8813683146414,-39.4057679385072));
#250434=CARTESIAN_POINT('Ctrl Pts',(44.2659122959159,33.8926702964892,-39.4205323411483));
#250435=CARTESIAN_POINT('Ctrl Pts',(44.3033049221432,33.8974288658374,-39.4277978831022));
#250436=CARTESIAN_POINT('Ctrl Pts',(44.3598453576919,33.9032050944765,-39.4385322478049));
#250437=CARTESIAN_POINT('Ctrl Pts',(44.3787527158677,33.9049006163346,-39.4420799976889));
#250438=CARTESIAN_POINT('Ctrl Pts',(44.4164967874688,33.9078161173588,-39.4490791780208));
#250439=CARTESIAN_POINT('Ctrl Pts',(44.4353708468856,33.9090400957878,-39.4525377314439));
#250440=CARTESIAN_POINT('Ctrl Pts',(44.4919347179527,33.9120095261765,-39.462779235967));
#250441=CARTESIAN_POINT('Ctrl Pts',(44.52962054914,33.9130584408517,-39.4694384189012));
#250442=CARTESIAN_POINT('Ctrl Pts',(44.6425299001817,33.9134342925821,-39.4889026473125));
#250443=CARTESIAN_POINT('Ctrl Pts',(44.7176656228988,33.9100023852834,-39.5012068570978));
#250444=CARTESIAN_POINT('Ctrl Pts',(44.867623327666,33.8957625538083,-39.524471978366));
#250445=CARTESIAN_POINT('Ctrl Pts',(44.9424659600731,33.8849485744664,-39.5354353652432));
#250446=CARTESIAN_POINT('Ctrl Pts',(45.0357885152669,33.8666999843662,-39.5482785606344));
#250447=CARTESIAN_POINT('Ctrl Pts',(45.0544546343785,33.8628074782943,-39.5508053225112));
#250448=CARTESIAN_POINT('Ctrl Pts',(45.091743102575,33.8545484160302,-39.5557691634051));
#250449=CARTESIAN_POINT('Ctrl Pts',(45.1104022544846,33.850171655015,-39.5582107864407));
#250450=CARTESIAN_POINT('Ctrl Pts',(45.1661672125598,33.8363538303533,-39.5653802281989));
#250451=CARTESIAN_POINT('Ctrl Pts',(45.2029511118778,33.8262578362557,-39.5699395109212));
#250452=CARTESIAN_POINT('Ctrl Pts',(45.312316831343,33.7933159380614,-39.582990524906));
#250453=CARTESIAN_POINT('Ctrl Pts',(45.4195983160475,33.7551076509549,-39.5947758536238));
#250454=CARTESIAN_POINT('Ctrl Pts',(45.5585113890164,33.6937328563153,-39.6079933748399));
#250455=CARTESIAN_POINT('Ctrl Pts',(45.6606150024606,33.6424505696195,-39.6166516297843));
#250456=CARTESIAN_POINT('Ctrl Pts',(45.7272860947277,33.6047101271221,-39.6215780075552));
#250457=CARTESIAN_POINT('Ctrl Pts',(45.7932287365117,33.5651705839516,-39.6260731428005));
#250458=CARTESIAN_POINT('Ctrl Pts',(45.8259059249178,33.5444453395394,-39.6281074988013));
#250459=CARTESIAN_POINT('Ctrl Pts',(45.8897275017006,33.5016881508368,-39.6316923737189));
#250460=CARTESIAN_POINT('Ctrl Pts',(45.9210297733036,33.4795651380848,-39.6332542688506));
#250461=CARTESIAN_POINT('Ctrl Pts',(45.9823424846244,33.4339088874735,-39.6359180193303));
#250462=CARTESIAN_POINT('Ctrl Pts',(46.0724202597563,33.3632801300718,-39.6392265347984));
#250463=CARTESIAN_POINT('Ctrl Pts',(46.1850394564173,33.2606222983665,-39.6409205727319));
#250464=CARTESIAN_POINT('Ctrl Pts',(46.2638636333332,33.1772336958075,-39.6401443034625));
#250465=CARTESIAN_POINT('Ctrl Pts',(46.3151397511292,33.1201974856456,-39.6391646017005));
#250466=CARTESIAN_POINT('Ctrl Pts',(46.3401349353408,33.0909661742941,-39.6384440851485));
#250467=CARTESIAN_POINT('Ctrl Pts',(46.3888523044997,33.0309971480077,-39.6365301000439));
#250468=CARTESIAN_POINT('Ctrl Pts',(46.4123735341802,33.0005036828642,-39.6353439924849));
#250469=CARTESIAN_POINT('Ctrl Pts',(46.4576879006691,32.9386388625828,-39.6325280276393));
#250470=CARTESIAN_POINT('Ctrl Pts',(46.52311576659,32.8444620833496,-39.6276360146217));
#250471=CARTESIAN_POINT('Ctrl Pts',(46.5810426872604,32.7462345994881,-39.6207752343847));
#250472=CARTESIAN_POINT('Ctrl Pts',(46.6516918187307,32.6117039458857,-39.6098936921283));
#250473=CARTESIAN_POINT('Ctrl Pts',(46.683723185051,32.5426422373878,-39.6035832967262));
#250474=CARTESIAN_POINT('Ctrl Pts',(46.7195635412788,32.4540883209461,-39.5945936116187));
#250475=CARTESIAN_POINT('Ctrl Pts',(46.7265235775841,32.4362514419463,-39.5927383889278));
#250476=CARTESIAN_POINT('Ctrl Pts',(46.7400123459627,32.4003742100513,-39.5889189813535));
#250477=CARTESIAN_POINT('Ctrl Pts',(46.7465535157541,32.3822946053341,-39.5869502184844));
#250478=CARTESIAN_POINT('Ctrl Pts',(46.7654644360989,32.3279072933142,-39.5808958427402));
#250479=CARTESIAN_POINT('Ctrl Pts',(46.7770937339888,32.2915493874551,-39.5766741707955));
#250480=CARTESIAN_POINT('Ctrl Pts',(46.8091770518909,32.182013131159,-39.5634457571489));
#250481=CARTESIAN_POINT('Ctrl Pts',(46.8444383818759,32.034891308334,-39.5443264312115));
#250482=CARTESIAN_POINT('Ctrl Pts',(46.8650708643864,31.8856621776612,-39.5223044891954));
#250483=CARTESIAN_POINT('Ctrl Pts',(46.8750487417844,31.7729724844591,-39.50469487268));
#250484=CARTESIAN_POINT('Ctrl Pts',(46.8774570362353,31.7352651712118,-39.4986397605723));
#250485=CARTESIAN_POINT('Ctrl Pts',(46.8796767940079,31.6785286095959,-39.4892824810203));
#250486=CARTESIAN_POINT('Ctrl Pts',(46.8801843407089,31.6595724593507,-39.4861150486293));
#250487=CARTESIAN_POINT('Ctrl Pts',(46.8807312344332,31.6216180949417,-39.479690628598));
#250488=CARTESIAN_POINT('Ctrl Pts',(46.8807699646674,31.6025797052015,-39.4764266299692));
#250489=CARTESIAN_POINT('Ctrl Pts',(46.8801790388754,31.5455906639181,-39.4665317368708));
#250490=CARTESIAN_POINT('Ctrl Pts',(46.8788490796135,31.5078273383739,-39.4598096545541));
#250491=CARTESIAN_POINT('Ctrl Pts',(46.874360617844,31.4326451774338,-39.4461013696832));
#250492=CARTESIAN_POINT('Ctrl Pts',(46.864884835636,31.320441459725,-39.4251517854185));
#250493=CARTESIAN_POINT('Ctrl Pts',(46.8414902947658,31.1730719473388,-39.3956936109857));
#250494=CARTESIAN_POINT('Ctrl Pts',(46.8074810934279,31.0279105813681,-39.364717848004));
#250495=CARTESIAN_POINT('Ctrl Pts',(46.7869180083019,30.9560697433081,-39.3487190247537));
#250496=CARTESIAN_POINT('Ctrl Pts',(46.7645577771926,30.884604709384,-39.332461491893));
#250497=CARTESIAN_POINT('Ctrl Pts',(46.7524740339114,30.8490466969583,-39.3242001683612));
#250498=CARTESIAN_POINT('Ctrl Pts',(46.7264943673172,30.7783632715819,-39.3074248425479));
#250499=CARTESIAN_POINT('Ctrl Pts',(46.7127058212706,30.7435263372096,-39.2989795429224));
#250500=CARTESIAN_POINT('Ctrl Pts',(46.6981266849492,30.7091523375488,-39.2904704603133));
#250501=CARTESIAN_POINT('Ctrl Pts',(44.7926621173534,30.9780510210195,-41.4731170634489));
#250502=CARTESIAN_POINT('Ctrl Pts',(44.7841183378731,30.958431594105,-41.4560988982307));
#250503=CARTESIAN_POINT('Ctrl Pts',(44.7652574387158,30.9202429989855,-41.4215723090211));
#250504=CARTESIAN_POINT('Ctrl Pts',(44.7373647422364,30.8750641226134,-41.3772059160528));
#250505=CARTESIAN_POINT('Ctrl Pts',(44.7186826069414,30.8491098680677,-41.3500360893141));
#250506=CARTESIAN_POINT('Ctrl Pts',(44.7057896374646,30.8320666178198,-41.3317986258606));
#250507=CARTESIAN_POINT('Ctrl Pts',(44.6991283043737,30.8236797190306,-41.3226233796301));
#250508=CARTESIAN_POINT('Ctrl Pts',(44.6853430526266,30.8071501195218,-41.3041237465898));
#250509=CARTESIAN_POINT('Ctrl Pts',(44.6782604199269,30.7990587859436,-41.2948558628018));
#250510=CARTESIAN_POINT('Ctrl Pts',(44.6637865272211,30.7832912649286,-41.2763692550984));
#250511=CARTESIAN_POINT('Ctrl Pts',(44.65638232911,30.7755995480316,-41.2671331599469));
#250512=CARTESIAN_POINT('Ctrl Pts',(44.6336879630273,30.7531065345255,-41.2394625228135));
#250513=CARTESIAN_POINT('Ctrl Pts',(44.6100194582072,30.7317609779911,-41.211850451263));
#250514=CARTESIAN_POINT('Ctrl Pts',(44.5765344835469,30.7055824366946,-41.1751580074971));
#250515=CARTESIAN_POINT('Ctrl Pts',(44.5504480754,30.6870962504203,-41.147699245024));
#250516=CARTESIAN_POINT('Ctrl Pts',(44.5324056777293,30.6755504391987,-41.1294402655247));
#250517=CARTESIAN_POINT('Ctrl Pts',(44.5186168522497,30.6671837862428,-41.1157563555777));
#250518=CARTESIAN_POINT('Ctrl Pts',(44.5139760207251,30.6644431539959,-41.1111953707762));
#250519=CARTESIAN_POINT('Ctrl Pts',(44.5046579712977,30.6590892493455,-41.102125755137));
#250520=CARTESIAN_POINT('Ctrl Pts',(44.4999732573772,30.6564710151932,-41.0976094410703));
#250521=CARTESIAN_POINT('Ctrl Pts',(44.4764410055871,30.6436866063214,-41.0751408219827));
#250522=CARTESIAN_POINT('Ctrl Pts',(44.4380363426647,30.6251318507397,-41.0398401547925));
#250523=CARTESIAN_POINT('Ctrl Pts',(44.3881999640401,30.6066279457426,-40.9973473660572));
#250524=CARTESIAN_POINT('Ctrl Pts',(44.3574626802754,30.5976558165788,-40.9725988687145));
#250525=CARTESIAN_POINT('Ctrl Pts',(44.3367823836873,30.5921565153947,-40.9562701951691));
#250526=CARTESIAN_POINT('Ctrl Pts',(44.3263541271388,30.5896491085923,-40.9481956834911));
#250527=CARTESIAN_POINT('Ctrl Pts',(44.3052793937559,30.5851218575581,-40.9322027877955));
#250528=CARTESIAN_POINT('Ctrl Pts',(44.2946995104909,30.5831174982377,-40.924335654778));
#250529=CARTESIAN_POINT('Ctrl Pts',(44.2735450602529,30.5796377993431,-40.9089243529734));
#250530=CARTESIAN_POINT('Ctrl Pts',(44.2629524396991,30.5781585711684,-40.9013664771085));
#250531=CARTESIAN_POINT('Ctrl Pts',(44.2311453972639,30.5744985086998,-40.8791460851492));
#250532=CARTESIAN_POINT('Ctrl Pts',(44.2098907431643,30.5730912421562,-40.8649273724495));
#250533=CARTESIAN_POINT('Ctrl Pts',(44.1672866942957,30.5723474200962,-40.8376959485268));
#250534=CARTESIAN_POINT('Ctrl Pts',(44.1459323927671,30.5730120277702,-40.8246808510428));
#250535=CARTESIAN_POINT('Ctrl Pts',(44.1191870166623,30.5751734135742,-40.8091986194082));
#250536=CARTESIAN_POINT('Ctrl Pts',(44.1138315874482,30.5756735271978,-40.806139968135));
#250537=CARTESIAN_POINT('Ctrl Pts',(44.1031212948485,30.5768077596639,-40.8001057293845));
#250538=CARTESIAN_POINT('Ctrl Pts',(44.0977557278508,30.5774435866632,-40.7971244669688));
#250539=CARTESIAN_POINT('Ctrl Pts',(44.0817045383335,30.5795497856634,-40.7883321887253));
#250540=CARTESIAN_POINT('Ctrl Pts',(44.0710902649836,30.5812139186595,-40.7826858714375));
#250541=CARTESIAN_POINT('Ctrl Pts',(44.0394561806682,30.5869813183234,-40.7663593410916));
#250542=CARTESIAN_POINT('Ctrl Pts',(44.0082701709188,30.5942909050994,-40.7512721078743));
#250543=CARTESIAN_POINT('Ctrl Pts',(43.9675777996734,30.6070988998346,-40.7336299050859));
#250544=CARTESIAN_POINT('Ctrl Pts',(43.9375066395073,30.6182485087226,-40.721648717354));
#250545=CARTESIAN_POINT('Ctrl Pts',(43.917761614853,30.626725808719,-40.7145087645619));
#250546=CARTESIAN_POINT('Ctrl Pts',(43.8981718083816,30.6357351147044,-40.7078022579606));
#250547=CARTESIAN_POINT('Ctrl Pts',(43.8884396229394,30.6405162381665,-40.7046629153417));
#250548=CARTESIAN_POINT('Ctrl Pts',(43.8693712864522,30.6504970769624,-40.6988992879235));
#250549=CARTESIAN_POINT('Ctrl Pts',(43.8599880575193,30.6557176389023,-40.6962583786489));
#250550=CARTESIAN_POINT('Ctrl Pts',(43.8415477166501,30.6665995934339,-40.6914621347147));
#250551=CARTESIAN_POINT('Ctrl Pts',(43.8143622090585,30.6835906587784,-40.6849914969931));
#250552=CARTESIAN_POINT('Ctrl Pts',(43.7885885365895,30.7025683103525,-40.6806752166169));
#250553=CARTESIAN_POINT('Ctrl Pts',(43.7554869731093,30.7296502406846,-40.676851696754));
#250554=CARTESIAN_POINT('Ctrl Pts',(43.7395647886014,30.744083456595,-40.6759056793254));
#250555=CARTESIAN_POINT('Ctrl Pts',(43.7090440489059,30.7747854825451,-40.6760208486551));
#250556=CARTESIAN_POINT('Ctrl Pts',(43.6947173014185,30.7907796762741,-40.6770802501629));
#250557=CARTESIAN_POINT('Ctrl Pts',(43.6678443418708,30.8240220908504,-40.6811258797777));
#250558=CARTESIAN_POINT('Ctrl Pts',(43.6427576069985,30.8585127548254,-40.687098273402));
#250559=CARTESIAN_POINT('Ctrl Pts',(43.6212142380078,30.8954846730083,-40.6968894358922));
#250560=CARTESIAN_POINT('Ctrl Pts',(43.6088787182641,30.9193798597989,-40.7042205511341));
#250561=CARTESIAN_POINT('Ctrl Pts',(43.6064685586478,30.9241994859948,-40.7057484197296));
#250562=CARTESIAN_POINT('Ctrl Pts',(43.6017624551859,30.9339175659931,-40.70892606686));
#250563=CARTESIAN_POINT('Ctrl Pts',(43.5994656231147,30.9388193592268,-40.7105773965538));
#250564=CARTESIAN_POINT('Ctrl Pts',(43.5927866482525,30.953560895212,-40.7156875255853));
#250565=CARTESIAN_POINT('Ctrl Pts',(43.5844198153918,30.9733582110501,-40.72293005151));
#250566=CARTESIAN_POINT('Ctrl Pts',(43.5734440082896,31.0034822735469,-40.7350537322951));
#250567=CARTESIAN_POINT('Ctrl Pts',(43.5640181327981,31.0340244080827,-40.7484125407461));
#250568=CARTESIAN_POINT('Ctrl Pts',(43.5561284133843,31.0649820306433,-40.7629929778707));
#250569=CARTESIAN_POINT('Ctrl Pts',(43.5518912037438,31.0858969805267,-40.7735241784737));
#250570=CARTESIAN_POINT('Ctrl Pts',(43.5481682579358,31.1069510729684,-40.7844620267622));
#250571=CARTESIAN_POINT('Ctrl Pts',(43.5465635963524,31.1175527760565,-40.7901372750232));
#250572=CARTESIAN_POINT('Ctrl Pts',(43.5438765944467,31.1388768366658,-40.8018865323646));
#250573=CARTESIAN_POINT('Ctrl Pts',(43.5427912565025,31.1496493641875,-40.8079902348016));
#250574=CARTESIAN_POINT('Ctrl Pts',(43.5411674088753,31.1711124235333,-40.8204828132684));
#250575=CARTESIAN_POINT('Ctrl Pts',(43.5400805588778,31.19253758885,-40.8332822237109));
#250576=CARTESIAN_POINT('Ctrl Pts',(43.5400129658238,31.2352236668913,-40.8600695429299));
#250577=CARTESIAN_POINT('Ctrl Pts',(43.5430492497798,31.2776738375434,-40.8886047446452));
#250578=CARTESIAN_POINT('Ctrl Pts',(43.5491614319672,31.3198884817001,-40.918856387552));
#250579=CARTESIAN_POINT('Ctrl Pts',(43.5532522131496,31.3409199794841,-40.9345594064291));
#250580=CARTESIAN_POINT('Ctrl Pts',(43.5578644352119,31.361905871423,-40.9505475151733));
#250581=CARTESIAN_POINT('Ctrl Pts',(43.560439098329,31.3723994717644,-40.9587035928991));
#250582=CARTESIAN_POINT('Ctrl Pts',(43.5660648897127,31.3931449423641,-40.9751492091434));
#250583=CARTESIAN_POINT('Ctrl Pts',(43.5691234314236,31.4034342087731,-40.9834667538713));
#250584=CARTESIAN_POINT('Ctrl Pts',(43.5790202279964,31.4340221767704,-41.0086741075936));
#250585=CARTESIAN_POINT('Ctrl Pts',(43.5865808644402,31.4540562960243,-41.0258289330007));
#250586=CARTESIAN_POINT('Ctrl Pts',(43.5993606039644,31.4835727602996,-41.0520789232858));
#250587=CARTESIAN_POINT('Ctrl Pts',(43.6038584649574,31.4933175175814,-41.0609109997729));
#250588=CARTESIAN_POINT('Ctrl Pts',(43.6133480280387,31.5126460303085,-41.0787663839806));
#250589=CARTESIAN_POINT('Ctrl Pts',(43.6183219077102,31.5221915251339,-41.0877549157913));
#250590=CARTESIAN_POINT('Ctrl Pts',(43.6338406007018,31.5503182102049,-41.1147514459697));
#250591=CARTESIAN_POINT('Ctrl Pts',(43.6450116757484,31.5684678157769,-41.13285712865));
#250592=CARTESIAN_POINT('Ctrl Pts',(43.6689569093208,31.6035742491305,-41.1692591986645));
#250593=CARTESIAN_POINT('Ctrl Pts',(43.6881189975485,31.6290150958394,-41.1967078345595));
#250594=CARTESIAN_POINT('Ctrl Pts',(43.7160805799803,31.6611548911343,-41.2335986369031));
#250595=CARTESIAN_POINT('Ctrl Pts',(43.7308739938731,31.6766212732249,-41.2521403517739));
#250596=CARTESIAN_POINT('Ctrl Pts',(43.7460847706871,31.6917854492915,-41.2707364845776));
#250597=CARTESIAN_POINT('Ctrl Pts',(43.7539033240721,31.6992171694526,-41.2800648729051));
#250598=CARTESIAN_POINT('Ctrl Pts',(43.7697797892606,31.7136063232936,-41.298562009488));
#250599=CARTESIAN_POINT('Ctrl Pts',(43.7778723272806,31.7205988773597,-41.3077734720143));
#250600=CARTESIAN_POINT('Ctrl Pts',(43.8025568401133,31.7409299545529,-41.3352381600133));
#250601=CARTESIAN_POINT('Ctrl Pts',(43.8195937300504,31.7536621581445,-41.353369616892));
#250602=CARTESIAN_POINT('Ctrl Pts',(43.8547939251157,31.7774712224987,-41.3892512463859));
#250603=CARTESIAN_POINT('Ctrl Pts',(43.8820456950658,31.7940939723408,-41.4158852269725));
#250604=CARTESIAN_POINT('Ctrl Pts',(43.9105977352555,31.8088239425505,-41.4420959852738));
#250605=CARTESIAN_POINT('Ctrl Pts',(43.9299312426308,31.8182163905263,-41.4594780331231));
#250606=CARTESIAN_POINT('Ctrl Pts',(43.9397545046832,31.8226994853967,-41.4681277754213));
#250607=CARTESIAN_POINT('Ctrl Pts',(43.959476379363,31.8311327029401,-41.4851373530728));
#250608=CARTESIAN_POINT('Ctrl Pts',(43.969416794615,31.835103670887,-41.4935351095415));
#250609=CARTESIAN_POINT('Ctrl Pts',(43.9894286782948,31.8425474915593,-41.5100965816665));
#250610=CARTESIAN_POINT('Ctrl Pts',(44.0196562937352,31.8529720625538,-41.5345993599874));
#250611=CARTESIAN_POINT('Ctrl Pts',(44.0607928561344,31.8639280327151,-41.5659272170578));
#250612=CARTESIAN_POINT('Ctrl Pts',(44.0922765794535,31.8699137146658,-41.5884145416429));
#250613=CARTESIAN_POINT('Ctrl Pts',(44.1134085621028,31.8733992175668,-41.6031789442838));
#250614=CARTESIAN_POINT('Ctrl Pts',(44.1240412545,31.8748890570172,-41.6104444862381));
#250615=CARTESIAN_POINT('Ctrl Pts',(44.1401138557838,31.8767382236783,-41.6211788509405));
#250616=CARTESIAN_POINT('Ctrl Pts',(44.1454877988083,31.8772894545129,-41.6247266008247));
#250617=CARTESIAN_POINT('Ctrl Pts',(44.1562140153048,31.878256418298,-41.6317257811562));
#250618=CARTESIAN_POINT('Ctrl Pts',(44.161576905651,31.8786734249769,-41.6351843345794));
#250619=CARTESIAN_POINT('Ctrl Pts',(44.1776466456902,31.8797244502982,-41.6454258391029));
#250620=CARTESIAN_POINT('Ctrl Pts',(44.1883500092183,31.8801603696231,-41.6520850220369));
#250621=CARTESIAN_POINT('Ctrl Pts',(44.2204087008324,31.8806796234647,-41.671549250448));
#250622=CARTESIAN_POINT('Ctrl Pts',(44.2417298059497,31.8799780982567,-41.6838534602333));
#250623=CARTESIAN_POINT('Ctrl Pts',(44.2842582084951,31.8764766164199,-41.7071185815018));
#250624=CARTESIAN_POINT('Ctrl Pts',(44.3054713486111,31.8736750129732,-41.7180819683776));
#250625=CARTESIAN_POINT('Ctrl Pts',(44.3319064277948,31.8688271235064,-41.7309251637703));
#250626=CARTESIAN_POINT('Ctrl Pts',(44.3371930873745,31.8677885276791,-41.7334519256467));
#250627=CARTESIAN_POINT('Ctrl Pts',(44.3477523920959,31.8655764110726,-41.7384157665409));
#250628=CARTESIAN_POINT('Ctrl Pts',(44.353035452149,31.8644001232798,-41.7408573895762));
#250629=CARTESIAN_POINT('Ctrl Pts',(44.368821997144,31.8606750365135,-41.7480268313348));
#250630=CARTESIAN_POINT('Ctrl Pts',(44.3792318927429,31.8579388865424,-41.752586114057));
#250631=CARTESIAN_POINT('Ctrl Pts',(44.4101727404,31.8489724804825,-41.7656371280416));
#250632=CARTESIAN_POINT('Ctrl Pts',(44.4405041748167,31.8385015328462,-41.7774224567595));
#250633=CARTESIAN_POINT('Ctrl Pts',(44.4797386522914,31.8215610256552,-41.7906399779756));
#250634=CARTESIAN_POINT('Ctrl Pts',(44.5085558494592,31.8073558935676,-41.7992982329201));
#250635=CARTESIAN_POINT('Ctrl Pts',(44.5273583247585,31.7968714183439,-41.8042246106906));
#250636=CARTESIAN_POINT('Ctrl Pts',(44.5459478308046,31.7858731708475,-41.8087197459362));
#250637=CARTESIAN_POINT('Ctrl Pts',(44.5551558111633,31.7801015230391,-41.8107541019367));
#250638=CARTESIAN_POINT('Ctrl Pts',(44.5731320510561,31.7681815367951,-41.814338976855));
#250639=CARTESIAN_POINT('Ctrl Pts',(44.5819448307914,31.7620078883687,-41.8159008719862));
#250640=CARTESIAN_POINT('Ctrl Pts',(44.5991987000126,31.7492554022398,-41.8185646224661));
#250641=CARTESIAN_POINT('Ctrl Pts',(44.6245350600795,31.7295108031857,-41.8218731379338));
#250642=CARTESIAN_POINT('Ctrl Pts',(44.6561620699444,31.7007477525095,-41.8235671758672));
#250643=CARTESIAN_POINT('Ctrl Pts',(44.6782580742923,31.6773394437008,-41.8227909065983));
#250644=CARTESIAN_POINT('Ctrl Pts',(44.6926220014235,31.6613194462407,-41.8218112048364));
#250645=CARTESIAN_POINT('Ctrl Pts',(44.6996188611148,31.6531046671394,-41.8210906882841));
#250646=CARTESIAN_POINT('Ctrl Pts',(44.7132456597446,31.6362429219073,-41.8191767031797));
#250647=CARTESIAN_POINT('Ctrl Pts',(44.7198193777268,31.627664624135,-41.8179905956202));
#250648=CARTESIAN_POINT('Ctrl Pts',(44.7324727845908,31.610252798272,-41.8151746307749));
#250649=CARTESIAN_POINT('Ctrl Pts',(44.7507253937504,31.5837345714901,-41.8102826177571));
#250650=CARTESIAN_POINT('Ctrl Pts',(44.7668325292565,31.5560404782777,-41.8034218375205));
#250651=CARTESIAN_POINT('Ctrl Pts',(44.7864242741839,31.5180816884312,-41.7925402952635));
#250652=CARTESIAN_POINT('Ctrl Pts',(44.7952779235527,31.4985810718442,-41.7862298998632));
#250653=CARTESIAN_POINT('Ctrl Pts',(44.8051436066325,31.4735589245645,-41.777240214754));
#250654=CARTESIAN_POINT('Ctrl Pts',(44.8070571630202,31.4685179927861,-41.7753849920635));
#250655=CARTESIAN_POINT('Ctrl Pts',(44.8107609555809,31.4583769076679,-41.7715655844892));
#250656=CARTESIAN_POINT('Ctrl Pts',(44.8125545845603,31.4532656516023,-41.76959682162));
#250657=CARTESIAN_POINT('Ctrl Pts',(44.8177323950795,31.4378873281915,-41.7635424458753));
#250658=CARTESIAN_POINT('Ctrl Pts',(44.8209059367305,31.4276035217402,-41.7593207739311));
#250659=CARTESIAN_POINT('Ctrl Pts',(44.8296276705658,31.3966113763671,-41.7460923602843));
#250660=CARTESIAN_POINT('Ctrl Pts',(44.8391161742293,31.3549585404116,-41.7269730343471));
#250661=CARTESIAN_POINT('Ctrl Pts',(44.8444380100638,31.312658433005,-41.7049510923314));
#250662=CARTESIAN_POINT('Ctrl Pts',(44.8468637082338,31.2806969121874,-41.6873414758157));
#250663=CARTESIAN_POINT('Ctrl Pts',(44.8474108190536,31.2699990859542,-41.6812863637077));
#250664=CARTESIAN_POINT('Ctrl Pts',(44.8478348231013,31.2538978106508,-41.671929084156));
#250665=CARTESIAN_POINT('Ctrl Pts',(44.8479099202363,31.2485174556463,-41.6687616517648));
#250666=CARTESIAN_POINT('Ctrl Pts',(44.8479268208064,31.2377432265879,-41.6623372317338));
#250667=CARTESIAN_POINT('Ctrl Pts',(44.8478683021095,31.2323379437313,-41.6590732331048));
#250668=CARTESIAN_POINT('Ctrl Pts',(44.8474921214824,31.2161555213209,-41.6491783400064));
#250669=CARTESIAN_POINT('Ctrl Pts',(44.8469759958029,31.2054292064128,-41.6424562576898));
#250670=CARTESIAN_POINT('Ctrl Pts',(44.8454249887827,31.1840681958411,-41.6287479728186));
#250671=CARTESIAN_POINT('Ctrl Pts',(44.8423204600693,31.1521790951542,-41.6077983885548));
#250672=CARTESIAN_POINT('Ctrl Pts',(44.8351290816859,31.1102584040656,-41.5783402141209));
#250673=CARTESIAN_POINT('Ctrl Pts',(44.8249268329474,31.0689281614894,-41.54736445114));
#250674=CARTESIAN_POINT('Ctrl Pts',(44.8188163283608,31.0484607830594,-41.5313656278891));
#250675=CARTESIAN_POINT('Ctrl Pts',(44.8121960627665,31.028093840338,-41.5151080950287));
#250676=CARTESIAN_POINT('Ctrl Pts',(44.808629563005,31.0179567656131,-41.5068467714969));
#250677=CARTESIAN_POINT('Ctrl Pts',(44.8009827391877,30.9977990758989,-41.4900714456835));
#250678=CARTESIAN_POINT('Ctrl Pts',(44.7969340070935,30.9878607344767,-41.4816261460579));
#250679=CARTESIAN_POINT('Ctrl Pts',(44.7926621173534,30.9780510210195,-41.4731170634489));
#250680=CARTESIAN_POINT('Ctrl Pts',(45.9506566843146,32.3790914166432,-40.3575678858382));
#250681=CARTESIAN_POINT('Ctrl Pts',(45.9241762187347,32.4857587342096,-40.3334357147994));
#250682=CARTESIAN_POINT('Ctrl Pts',(45.8833609513182,32.5889003369546,-40.3114654491246));
#250683=CARTESIAN_POINT('Ctrl Pts',(45.7741007712946,32.7781362580382,-40.2740055971064));
#250684=CARTESIAN_POINT('Ctrl Pts',(45.7072894462425,32.8634116806853,-40.2585741398382));
#250685=CARTESIAN_POINT('Ctrl Pts',(45.5743075775965,32.989444414025,-40.2380701272289));
#250686=CARTESIAN_POINT('Ctrl Pts',(45.5152506641723,33.0350940714751,-40.2313718283122));
#250687=CARTESIAN_POINT('Ctrl Pts',(45.4499236404499,33.0758951502756,-40.2260815011696));
#250688=CARTESIAN_POINT('Ctrl Pts',(45.4481230226174,33.0770127394939,-40.2259372093736));
#250689=CARTESIAN_POINT('Ctrl Pts',(45.4445215185278,33.0792340735076,-40.2256516559397));
#250690=CARTESIAN_POINT('Ctrl Pts',(45.4427204399715,33.0803379828413,-40.225510369052));
#250691=CARTESIAN_POINT('Ctrl Pts',(45.4373314986288,33.0836201423993,-40.2250921735013));
#250692=CARTESIAN_POINT('Ctrl Pts',(45.4337333703977,33.0857841424913,-40.2248189435083));
#250693=CARTESIAN_POINT('Ctrl Pts',(45.4263798098968,33.0901505597053,-40.2242729152289));
#250694=CARTESIAN_POINT('Ctrl Pts',(45.4226308321482,33.0923467584675,-40.2240011956117));
#250695=CARTESIAN_POINT('Ctrl Pts',(45.4112166580987,33.0989467358971,-40.2231924467728));
#250696=CARTESIAN_POINT('Ctrl Pts',(45.4034897677801,33.1032948476848,-40.2226706845611));
#250697=CARTESIAN_POINT('Ctrl Pts',(45.3208157329137,33.1485541094836,-40.2173576933466));
#250698=CARTESIAN_POINT('Ctrl Pts',(45.2416758433089,33.180918628968,-40.2146176874415));
#250699=CARTESIAN_POINT('Ctrl Pts',(44.998745313087,33.2510628523576,-40.2117974091292));
#250700=CARTESIAN_POINT('Ctrl Pts',(44.8303310441375,33.2631001270432,-40.2168378999613));
#250701=CARTESIAN_POINT('Ctrl Pts',(44.597970209409,33.2372616316389,-40.2297741904108));
#250702=CARTESIAN_POINT('Ctrl Pts',(44.5338416044383,33.2252555296773,-40.234170313172));
#250703=CARTESIAN_POINT('Ctrl Pts',(44.4689444465313,33.2087417401602,-40.238822271049));
#250704=CARTESIAN_POINT('Ctrl Pts',(46.6981266849492,30.7091523375488,-39.2904704603133));
#250705=CARTESIAN_POINT('Ctrl Pts',(46.6689684123063,30.6404043382273,-39.273452295095));
#250706=CARTESIAN_POINT('Ctrl Pts',(46.6043681216411,30.5066861069553,-39.238925705885));
#250707=CARTESIAN_POINT('Ctrl Pts',(46.5083209189471,30.3487389562033,-39.1945593129175));
#250708=CARTESIAN_POINT('Ctrl Pts',(46.4437937583117,30.2581216171786,-39.1673894861782));
#250709=CARTESIAN_POINT('Ctrl Pts',(46.3992224148768,30.1986447451181,-39.1491520227249));
#250710=CARTESIAN_POINT('Ctrl Pts',(46.3761748773305,30.1693908446446,-39.1399767764946));
#250711=CARTESIAN_POINT('Ctrl Pts',(46.3284414024809,30.1117648114071,-39.1214771434543));
#250712=CARTESIAN_POINT('Ctrl Pts',(46.3038983378397,30.083571828401,-39.112209259666));
#250713=CARTESIAN_POINT('Ctrl Pts',(46.253707387608,30.0286632749651,-39.0937226519629));
#250714=CARTESIAN_POINT('Ctrl Pts',(46.2280147026909,30.001893564456,-39.0844865568113));
#250715=CARTESIAN_POINT('Ctrl Pts',(46.1492148010453,29.9236586721517,-39.0568159196779));
#250716=CARTESIAN_POINT('Ctrl Pts',(46.0669347173688,29.8495134741745,-39.0292038481275));
#250717=CARTESIAN_POINT('Ctrl Pts',(45.9503410384262,29.7587889734315,-38.9925114043613));
#250718=CARTESIAN_POINT('Ctrl Pts',(45.8594191065401,29.6948377475824,-38.9650526418885));
#250719=CARTESIAN_POINT('Ctrl Pts',(45.7964751089327,29.6549785818455,-38.9467936623891));
#250720=CARTESIAN_POINT('Ctrl Pts',(45.748348603817,29.6261284949947,-38.9331097524421));
#250721=CARTESIAN_POINT('Ctrl Pts',(45.7321473284057,29.616684052073,-38.9285487676403));
#250722=CARTESIAN_POINT('Ctrl Pts',(45.6996106203311,29.5982459977232,-38.9194791520014));
#250723=CARTESIAN_POINT('Ctrl Pts',(45.683249044345,29.5892352448745,-38.9149628379356));
#250724=CARTESIAN_POINT('Ctrl Pts',(45.6010439155842,29.5452684013657,-38.8924942188443));
#250725=CARTESIAN_POINT('Ctrl Pts',(45.4667739830181,29.4816584171599,-38.8571935516581));
#250726=CARTESIAN_POINT('Ctrl Pts',(45.2922645146651,29.4187721922835,-38.8147007629208));
#250727=CARTESIAN_POINT('Ctrl Pts',(45.184512437616,29.3885937253944,-38.7899522655792));
#250728=CARTESIAN_POINT('Ctrl Pts',(45.1119891467798,29.3701842541612,-38.7736235920333));
#250729=CARTESIAN_POINT('Ctrl Pts',(45.0754052578815,29.3618381514785,-38.7655490803555));
#250730=CARTESIAN_POINT('Ctrl Pts',(45.0014447932705,29.3468760834356,-38.7495561846596));
#250731=CARTESIAN_POINT('Ctrl Pts',(44.964301863367,29.3403115562353,-38.7416890516424));
#250732=CARTESIAN_POINT('Ctrl Pts',(44.8900079594565,29.3290481892184,-38.726277749838));
#250733=CARTESIAN_POINT('Ctrl Pts',(44.8527936282157,29.324336495618,-38.7187198739728));
#250734=CARTESIAN_POINT('Ctrl Pts',(44.7410083373266,29.3129455735289,-38.6964994820139));
#250735=CARTESIAN_POINT('Ctrl Pts',(44.6662563757167,29.3089967422249,-38.6822807693139));
#250736=CARTESIAN_POINT('Ctrl Pts',(44.516312468428,29.3084067934202,-38.6550493453909));
#250737=CARTESIAN_POINT('Ctrl Pts',(44.441103189525,29.3117700143417,-38.6420342479066));
#250738=CARTESIAN_POINT('Ctrl Pts',(44.3468378615956,29.3206690055189,-38.6265520162729));
#250739=CARTESIAN_POINT('Ctrl Pts',(44.3279589148655,29.3226883315868,-38.6234933649988));
#250740=CARTESIAN_POINT('Ctrl Pts',(44.2901960653062,29.3271995080042,-38.6174591262491));
#250741=CARTESIAN_POINT('Ctrl Pts',(44.271274393292,29.329697893027,-38.614477863833));
#250742=CARTESIAN_POINT('Ctrl Pts',(44.2146592782019,29.3378915995821,-38.60568558559));
#250743=CARTESIAN_POINT('Ctrl Pts',(44.1772069502033,29.344266758826,-38.6000392683017));
#250744=CARTESIAN_POINT('Ctrl Pts',(44.0655444875092,29.3661148598052,-38.5837127379559));
#250745=CARTESIAN_POINT('Ctrl Pts',(43.9553791862171,29.3933792052515,-38.5686255047386));
#250746=CARTESIAN_POINT('Ctrl Pts',(43.8114622524781,29.4404829778103,-38.5509833019505));
#250747=CARTESIAN_POINT('Ctrl Pts',(43.705021834675,29.481230340464,-38.5390021142185));
#250748=CARTESIAN_POINT('Ctrl Pts',(43.6350719757086,29.512061063653,-38.5318621614261));
#250749=CARTESIAN_POINT('Ctrl Pts',(43.5656410085295,29.5447591316771,-38.525155654825));
#250750=CARTESIAN_POINT('Ctrl Pts',(43.5311320054746,29.5620794464364,-38.5220163122062));
#250751=CARTESIAN_POINT('Ctrl Pts',(43.4634866412134,29.5981758355574,-38.5162526847879));
#250752=CARTESIAN_POINT('Ctrl Pts',(43.4301834663392,29.6170276546,-38.5136117755133));
#250753=CARTESIAN_POINT('Ctrl Pts',(43.3647025891651,29.6562685687332,-38.5088155315793));
#250754=CARTESIAN_POINT('Ctrl Pts',(43.2681192378476,29.7174608121974,-38.5023448938576));
#250755=CARTESIAN_POINT('Ctrl Pts',(43.1764049274077,29.7855824582168,-38.4980286134812));
#250756=CARTESIAN_POINT('Ctrl Pts',(43.0584774180437,29.8826126224142,-38.4942050936184));
#250757=CARTESIAN_POINT('Ctrl Pts',(43.001681818637,29.9342392650769,-38.4932590761897));
#250758=CARTESIAN_POINT('Ctrl Pts',(42.8926599718677,30.0438904492243,-38.4933742455196));
#250759=CARTESIAN_POINT('Ctrl Pts',(42.8414047150844,30.1009342501745,-38.4944336470273));
#250760=CARTESIAN_POINT('Ctrl Pts',(42.7451036203247,30.2193471227021,-38.498479276642));
#250761=CARTESIAN_POINT('Ctrl Pts',(42.6550322643363,30.3420646399833,-38.5044516702661));
#250762=CARTESIAN_POINT('Ctrl Pts',(42.5773225406025,30.4733365238586,-38.5142428327574));
#250763=CARTESIAN_POINT('Ctrl Pts',(42.5326943378214,30.5580963840027,-38.5215739479982));
#250764=CARTESIAN_POINT('Ctrl Pts',(42.5239673850246,30.5751883092729,-38.5231018165939));
#250765=CARTESIAN_POINT('Ctrl Pts',(42.5069121510755,30.60964376351,-38.5262794637242));
#250766=CARTESIAN_POINT('Ctrl Pts',(42.4985805781952,30.627019094627,-38.5279307934181));
#250767=CARTESIAN_POINT('Ctrl Pts',(42.4743295471271,30.6792614198295,-38.5330409224498));
#250768=CARTESIAN_POINT('Ctrl Pts',(42.4438856226513,30.7493896366731,-38.5402834483744));
#250769=CARTESIAN_POINT('Ctrl Pts',(42.4037483179465,30.8560072598611,-38.5524071291592));
#250770=CARTESIAN_POINT('Ctrl Pts',(42.3690543371876,30.9640160484273,-38.5657659376104));
#250771=CARTESIAN_POINT('Ctrl Pts',(42.3397558527982,31.0734075527136,-38.5803463747351));
#250772=CARTESIAN_POINT('Ctrl Pts',(42.3238156343608,31.1472555030051,-38.5908775753381));
#250773=CARTESIAN_POINT('Ctrl Pts',(42.3096820427396,31.2215665449467,-38.6018154236264));
#250774=CARTESIAN_POINT('Ctrl Pts',(42.3035171869091,31.2589715314082,-38.6074906718877));
#250775=CARTESIAN_POINT('Ctrl Pts',(42.2930235524414,31.3341791410138,-38.6192399292287));
#250776=CARTESIAN_POINT('Ctrl Pts',(42.2886818075092,31.3721585359098,-38.6253436316658));
#250777=CARTESIAN_POINT('Ctrl Pts',(42.281930630611,31.4478003630713,-38.6378362101326));
#250778=CARTESIAN_POINT('Ctrl Pts',(42.277074994566,31.5232809912004,-38.6506356205751));
#250779=CARTESIAN_POINT('Ctrl Pts',(42.2747992363309,31.6735553614761,-38.6774229397946));
#250780=CARTESIAN_POINT('Ctrl Pts',(42.2834818483937,31.8228397562226,-38.7059581415094));
#250781=CARTESIAN_POINT('Ctrl Pts',(42.3030248127084,31.9711385758679,-38.7362097844166));
#250782=CARTESIAN_POINT('Ctrl Pts',(42.3164494406915,32.0449687602614,-38.7519128032936));
#250783=CARTESIAN_POINT('Ctrl Pts',(42.3317154579634,32.1186122141692,-38.7679009120377));
#250784=CARTESIAN_POINT('Ctrl Pts',(42.3402956643805,32.1554227583218,-38.7760569897633));
#250785=CARTESIAN_POINT('Ctrl Pts',(42.3591481714288,32.228169160774,-38.7925026060078));
#250786=CARTESIAN_POINT('Ctrl Pts',(42.3694448348212,32.2642362896146,-38.8008201507359));
#250787=CARTESIAN_POINT('Ctrl Pts',(42.4028917825415,32.3714169561226,-38.8260275044574));
#250788=CARTESIAN_POINT('Ctrl Pts',(42.428602574983,32.4415633880281,-38.8431823298655));
#250789=CARTESIAN_POINT('Ctrl Pts',(42.4722685042023,32.5448307979217,-38.8694323201497));
#250790=CARTESIAN_POINT('Ctrl Pts',(42.4876674804306,32.5789105800712,-38.8782643966373));
#250791=CARTESIAN_POINT('Ctrl Pts',(42.5202146590728,32.6464795812123,-38.8961197808447));
#250792=CARTESIAN_POINT('Ctrl Pts',(42.5373018269229,32.6798350022668,-38.9051083126545));
#250793=CARTESIAN_POINT('Ctrl Pts',(42.5906929412925,32.7780783962456,-38.9321048428364));
#250794=CARTESIAN_POINT('Ctrl Pts',(42.629225789877,32.8414173722334,-38.9502105255135));
#250795=CARTESIAN_POINT('Ctrl Pts',(42.7120000069194,32.9638220552461,-38.9866125955294));
#250796=CARTESIAN_POINT('Ctrl Pts',(42.7783647966162,33.0524402968179,-39.0140612314234));
#250797=CARTESIAN_POINT('Ctrl Pts',(42.8754380724448,33.1642175243331,-39.0509520337677));
#250798=CARTESIAN_POINT('Ctrl Pts',(42.9268673384212,33.2179450225078,-39.0694937486382));
#250799=CARTESIAN_POINT('Ctrl Pts',(42.9797817061918,33.2705900457306,-39.088089881442));
#250800=CARTESIAN_POINT('Ctrl Pts',(43.0069972096607,33.2963736994336,-39.097418269769));
#250801=CARTESIAN_POINT('Ctrl Pts',(43.0622936398443,33.3462615369726,-39.1159154063528));
#250802=CARTESIAN_POINT('Ctrl Pts',(43.0904949946047,33.3704876748183,-39.1251268688783));
#250803=CARTESIAN_POINT('Ctrl Pts',(43.176562606447,33.4408730143712,-39.1525915568785));
#250804=CARTESIAN_POINT('Ctrl Pts',(43.2360245534179,33.4848790444095,-39.1707230137558));
#250805=CARTESIAN_POINT('Ctrl Pts',(43.358992255749,33.5670176609587,-39.2066046432507));
#250806=CARTESIAN_POINT('Ctrl Pts',(43.4542745623933,33.6242424638975,-39.233238623837));
#250807=CARTESIAN_POINT('Ctrl Pts',(43.5542222374601,33.6747516510336,-39.2594493821381));
#250808=CARTESIAN_POINT('Ctrl Pts',(43.6219256430316,33.7069073870393,-39.2768314299875));
#250809=CARTESIAN_POINT('Ctrl Pts',(43.6563381479934,33.7222286468184,-39.2854811722856));
#250810=CARTESIAN_POINT('Ctrl Pts',(43.7254519170511,33.7509934760635,-39.3024907499371));
#250811=CARTESIAN_POINT('Ctrl Pts',(43.7602995448845,33.7645084608315,-39.3108885064059));
#250812=CARTESIAN_POINT('Ctrl Pts',(43.8304781084082,33.789780836939,-39.3274499785309));
#250813=CARTESIAN_POINT('Ctrl Pts',(43.9365171946568,33.8250735562425,-39.3519527568515));
#250814=CARTESIAN_POINT('Ctrl Pts',(44.0809642638621,33.8617420360433,-39.3832806139221));
#250815=CARTESIAN_POINT('Ctrl Pts',(44.1916183723467,33.8813683146414,-39.4057679385072));
#250816=CARTESIAN_POINT('Ctrl Pts',(44.2659122959159,33.8926702964892,-39.4205323411483));
#250817=CARTESIAN_POINT('Ctrl Pts',(44.3033049221432,33.8974288658374,-39.4277978831022));
#250818=CARTESIAN_POINT('Ctrl Pts',(44.3598453576919,33.9032050944765,-39.4385322478049));
#250819=CARTESIAN_POINT('Ctrl Pts',(44.3787527158677,33.9049006163346,-39.4420799976889));
#250820=CARTESIAN_POINT('Ctrl Pts',(44.4164967874688,33.9078161173588,-39.4490791780208));
#250821=CARTESIAN_POINT('Ctrl Pts',(44.4353708468856,33.9090400957878,-39.4525377314439));
#250822=CARTESIAN_POINT('Ctrl Pts',(44.4919347179527,33.9120095261765,-39.462779235967));
#250823=CARTESIAN_POINT('Ctrl Pts',(44.52962054914,33.9130584408517,-39.4694384189012));
#250824=CARTESIAN_POINT('Ctrl Pts',(44.6425299001817,33.9134342925821,-39.4889026473125));
#250825=CARTESIAN_POINT('Ctrl Pts',(44.7176656228988,33.9100023852834,-39.5012068570978));
#250826=CARTESIAN_POINT('Ctrl Pts',(44.867623327666,33.8957625538083,-39.524471978366));
#250827=CARTESIAN_POINT('Ctrl Pts',(44.9424659600731,33.8849485744664,-39.5354353652432));
#250828=CARTESIAN_POINT('Ctrl Pts',(45.0357885152669,33.8666999843662,-39.5482785606344));
#250829=CARTESIAN_POINT('Ctrl Pts',(45.0544546343785,33.8628074782943,-39.5508053225112));
#250830=CARTESIAN_POINT('Ctrl Pts',(45.091743102575,33.8545484160302,-39.5557691634051));
#250831=CARTESIAN_POINT('Ctrl Pts',(45.1104022544846,33.850171655015,-39.5582107864407));
#250832=CARTESIAN_POINT('Ctrl Pts',(45.1661672125598,33.8363538303533,-39.5653802281989));
#250833=CARTESIAN_POINT('Ctrl Pts',(45.2029511118778,33.8262578362557,-39.5699395109212));
#250834=CARTESIAN_POINT('Ctrl Pts',(45.312316831343,33.7933159380614,-39.582990524906));
#250835=CARTESIAN_POINT('Ctrl Pts',(45.4195983160475,33.7551076509549,-39.5947758536238));
#250836=CARTESIAN_POINT('Ctrl Pts',(45.5585113890164,33.6937328563153,-39.6079933748399));
#250837=CARTESIAN_POINT('Ctrl Pts',(45.6606150024606,33.6424505696195,-39.6166516297843));
#250838=CARTESIAN_POINT('Ctrl Pts',(45.7272860947277,33.6047101271221,-39.6215780075552));
#250839=CARTESIAN_POINT('Ctrl Pts',(45.7932287365117,33.5651705839516,-39.6260731428005));
#250840=CARTESIAN_POINT('Ctrl Pts',(45.8259059249178,33.5444453395394,-39.6281074988013));
#250841=CARTESIAN_POINT('Ctrl Pts',(45.8897275017006,33.5016881508368,-39.6316923737189));
#250842=CARTESIAN_POINT('Ctrl Pts',(45.9210297733036,33.4795651380848,-39.6332542688506));
#250843=CARTESIAN_POINT('Ctrl Pts',(45.9823424846244,33.4339088874735,-39.6359180193303));
#250844=CARTESIAN_POINT('Ctrl Pts',(46.0724202597563,33.3632801300718,-39.6392265347984));
#250845=CARTESIAN_POINT('Ctrl Pts',(46.1850394564173,33.2606222983665,-39.6409205727319));
#250846=CARTESIAN_POINT('Ctrl Pts',(46.2638636333332,33.1772336958075,-39.6401443034625));
#250847=CARTESIAN_POINT('Ctrl Pts',(46.3151397511292,33.1201974856456,-39.6391646017005));
#250848=CARTESIAN_POINT('Ctrl Pts',(46.3401349353408,33.0909661742941,-39.6384440851485));
#250849=CARTESIAN_POINT('Ctrl Pts',(46.3888523044997,33.0309971480077,-39.6365301000439));
#250850=CARTESIAN_POINT('Ctrl Pts',(46.4123735341802,33.0005036828642,-39.6353439924849));
#250851=CARTESIAN_POINT('Ctrl Pts',(46.4576879006691,32.9386388625828,-39.6325280276393));
#250852=CARTESIAN_POINT('Ctrl Pts',(46.52311576659,32.8444620833496,-39.6276360146217));
#250853=CARTESIAN_POINT('Ctrl Pts',(46.5810426872604,32.7462345994881,-39.6207752343847));
#250854=CARTESIAN_POINT('Ctrl Pts',(46.6516918187307,32.6117039458857,-39.6098936921283));
#250855=CARTESIAN_POINT('Ctrl Pts',(46.683723185051,32.5426422373878,-39.6035832967262));
#250856=CARTESIAN_POINT('Ctrl Pts',(46.7195635412788,32.4540883209461,-39.5945936116187));
#250857=CARTESIAN_POINT('Ctrl Pts',(46.7265235775841,32.4362514419463,-39.5927383889278));
#250858=CARTESIAN_POINT('Ctrl Pts',(46.7400123459627,32.4003742100513,-39.5889189813535));
#250859=CARTESIAN_POINT('Ctrl Pts',(46.7465535157541,32.3822946053341,-39.5869502184844));
#250860=CARTESIAN_POINT('Ctrl Pts',(46.7654644360989,32.3279072933142,-39.5808958427402));
#250861=CARTESIAN_POINT('Ctrl Pts',(46.7770937339888,32.2915493874551,-39.5766741707955));
#250862=CARTESIAN_POINT('Ctrl Pts',(46.8091770518909,32.182013131159,-39.5634457571489));
#250863=CARTESIAN_POINT('Ctrl Pts',(46.8444383818759,32.034891308334,-39.5443264312115));
#250864=CARTESIAN_POINT('Ctrl Pts',(46.8650708643864,31.8856621776612,-39.5223044891954));
#250865=CARTESIAN_POINT('Ctrl Pts',(46.8750487417844,31.7729724844591,-39.50469487268));
#250866=CARTESIAN_POINT('Ctrl Pts',(46.8774570362353,31.7352651712118,-39.4986397605723));
#250867=CARTESIAN_POINT('Ctrl Pts',(46.8796767940079,31.6785286095959,-39.4892824810203));
#250868=CARTESIAN_POINT('Ctrl Pts',(46.8801843407089,31.6595724593507,-39.4861150486293));
#250869=CARTESIAN_POINT('Ctrl Pts',(46.8807312344332,31.6216180949417,-39.479690628598));
#250870=CARTESIAN_POINT('Ctrl Pts',(46.8807699646674,31.6025797052015,-39.4764266299692));
#250871=CARTESIAN_POINT('Ctrl Pts',(46.8801790388754,31.5455906639181,-39.4665317368708));
#250872=CARTESIAN_POINT('Ctrl Pts',(46.8788490796135,31.5078273383739,-39.4598096545541));
#250873=CARTESIAN_POINT('Ctrl Pts',(46.874360617844,31.4326451774338,-39.4461013696832));
#250874=CARTESIAN_POINT('Ctrl Pts',(46.864884835636,31.320441459725,-39.4251517854185));
#250875=CARTESIAN_POINT('Ctrl Pts',(46.8414902947658,31.1730719473388,-39.3956936109857));
#250876=CARTESIAN_POINT('Ctrl Pts',(46.8074810934279,31.0279105813681,-39.364717848004));
#250877=CARTESIAN_POINT('Ctrl Pts',(46.7869180083019,30.9560697433081,-39.3487190247537));
#250878=CARTESIAN_POINT('Ctrl Pts',(46.7645577771926,30.884604709384,-39.332461491893));
#250879=CARTESIAN_POINT('Ctrl Pts',(46.7524740339114,30.8490466969583,-39.3242001683612));
#250880=CARTESIAN_POINT('Ctrl Pts',(46.7264943673172,30.7783632715819,-39.3074248425479));
#250881=CARTESIAN_POINT('Ctrl Pts',(46.7127058212706,30.7435263372096,-39.2989795429224));
#250882=CARTESIAN_POINT('Ctrl Pts',(46.6981266849492,30.7091523375488,-39.2904704603133));
#250883=CARTESIAN_POINT('Ctrl Pts',(44.7926621173534,30.9780510210195,-41.4731170634489));
#250884=CARTESIAN_POINT('Ctrl Pts',(44.7841183378731,30.958431594105,-41.4560988982307));
#250885=CARTESIAN_POINT('Ctrl Pts',(44.7652574387158,30.9202429989855,-41.4215723090211));
#250886=CARTESIAN_POINT('Ctrl Pts',(44.7373647422364,30.8750641226134,-41.3772059160528));
#250887=CARTESIAN_POINT('Ctrl Pts',(44.7186826069414,30.8491098680677,-41.3500360893141));
#250888=CARTESIAN_POINT('Ctrl Pts',(44.7057896374646,30.8320666178198,-41.3317986258606));
#250889=CARTESIAN_POINT('Ctrl Pts',(44.6991283043737,30.8236797190306,-41.3226233796301));
#250890=CARTESIAN_POINT('Ctrl Pts',(44.6853430526266,30.8071501195218,-41.3041237465898));
#250891=CARTESIAN_POINT('Ctrl Pts',(44.6782604199269,30.7990587859436,-41.2948558628018));
#250892=CARTESIAN_POINT('Ctrl Pts',(44.6637865272211,30.7832912649286,-41.2763692550984));
#250893=CARTESIAN_POINT('Ctrl Pts',(44.65638232911,30.7755995480316,-41.2671331599469));
#250894=CARTESIAN_POINT('Ctrl Pts',(44.6336879630273,30.7531065345255,-41.2394625228135));
#250895=CARTESIAN_POINT('Ctrl Pts',(44.6100194582072,30.7317609779911,-41.211850451263));
#250896=CARTESIAN_POINT('Ctrl Pts',(44.5765344835469,30.7055824366946,-41.1751580074971));
#250897=CARTESIAN_POINT('Ctrl Pts',(44.5504480754,30.6870962504203,-41.147699245024));
#250898=CARTESIAN_POINT('Ctrl Pts',(44.5324056777293,30.6755504391987,-41.1294402655247));
#250899=CARTESIAN_POINT('Ctrl Pts',(44.5186168522497,30.6671837862428,-41.1157563555777));
#250900=CARTESIAN_POINT('Ctrl Pts',(44.5139760207251,30.6644431539959,-41.1111953707762));
#250901=CARTESIAN_POINT('Ctrl Pts',(44.5046579712977,30.6590892493455,-41.102125755137));
#250902=CARTESIAN_POINT('Ctrl Pts',(44.4999732573772,30.6564710151932,-41.0976094410703));
#250903=CARTESIAN_POINT('Ctrl Pts',(44.4764410055871,30.6436866063214,-41.0751408219827));
#250904=CARTESIAN_POINT('Ctrl Pts',(44.4380363426647,30.6251318507397,-41.0398401547925));
#250905=CARTESIAN_POINT('Ctrl Pts',(44.3881999640401,30.6066279457426,-40.9973473660572));
#250906=CARTESIAN_POINT('Ctrl Pts',(44.3574626802754,30.5976558165788,-40.9725988687145));
#250907=CARTESIAN_POINT('Ctrl Pts',(44.3367823836873,30.5921565153947,-40.9562701951691));
#250908=CARTESIAN_POINT('Ctrl Pts',(44.3263541271388,30.5896491085923,-40.9481956834911));
#250909=CARTESIAN_POINT('Ctrl Pts',(44.3052793937559,30.5851218575581,-40.9322027877955));
#250910=CARTESIAN_POINT('Ctrl Pts',(44.2946995104909,30.5831174982377,-40.924335654778));
#250911=CARTESIAN_POINT('Ctrl Pts',(44.2735450602529,30.5796377993431,-40.9089243529734));
#250912=CARTESIAN_POINT('Ctrl Pts',(44.2629524396991,30.5781585711684,-40.9013664771085));
#250913=CARTESIAN_POINT('Ctrl Pts',(44.2311453972639,30.5744985086998,-40.8791460851492));
#250914=CARTESIAN_POINT('Ctrl Pts',(44.2098907431643,30.5730912421562,-40.8649273724495));
#250915=CARTESIAN_POINT('Ctrl Pts',(44.1672866942957,30.5723474200962,-40.8376959485268));
#250916=CARTESIAN_POINT('Ctrl Pts',(44.1459323927671,30.5730120277702,-40.8246808510428));
#250917=CARTESIAN_POINT('Ctrl Pts',(44.1191870166623,30.5751734135742,-40.8091986194082));
#250918=CARTESIAN_POINT('Ctrl Pts',(44.1138315874482,30.5756735271978,-40.806139968135));
#250919=CARTESIAN_POINT('Ctrl Pts',(44.1031212948485,30.5768077596639,-40.8001057293845));
#250920=CARTESIAN_POINT('Ctrl Pts',(44.0977557278508,30.5774435866632,-40.7971244669688));
#250921=CARTESIAN_POINT('Ctrl Pts',(44.0817045383335,30.5795497856634,-40.7883321887253));
#250922=CARTESIAN_POINT('Ctrl Pts',(44.0710902649836,30.5812139186595,-40.7826858714375));
#250923=CARTESIAN_POINT('Ctrl Pts',(44.0394561806682,30.5869813183234,-40.7663593410916));
#250924=CARTESIAN_POINT('Ctrl Pts',(44.0082701709188,30.5942909050994,-40.7512721078743));
#250925=CARTESIAN_POINT('Ctrl Pts',(43.9675777996734,30.6070988998346,-40.7336299050859));
#250926=CARTESIAN_POINT('Ctrl Pts',(43.9375066395073,30.6182485087226,-40.721648717354));
#250927=CARTESIAN_POINT('Ctrl Pts',(43.917761614853,30.626725808719,-40.7145087645619));
#250928=CARTESIAN_POINT('Ctrl Pts',(43.8981718083816,30.6357351147044,-40.7078022579606));
#250929=CARTESIAN_POINT('Ctrl Pts',(43.8884396229394,30.6405162381665,-40.7046629153417));
#250930=CARTESIAN_POINT('Ctrl Pts',(43.8693712864522,30.6504970769624,-40.6988992879235));
#250931=CARTESIAN_POINT('Ctrl Pts',(43.8599880575193,30.6557176389023,-40.6962583786489));
#250932=CARTESIAN_POINT('Ctrl Pts',(43.8415477166501,30.6665995934339,-40.6914621347147));
#250933=CARTESIAN_POINT('Ctrl Pts',(43.8143622090585,30.6835906587784,-40.6849914969931));
#250934=CARTESIAN_POINT('Ctrl Pts',(43.7885885365895,30.7025683103525,-40.6806752166169));
#250935=CARTESIAN_POINT('Ctrl Pts',(43.7554869731093,30.7296502406846,-40.676851696754));
#250936=CARTESIAN_POINT('Ctrl Pts',(43.7395647886014,30.744083456595,-40.6759056793254));
#250937=CARTESIAN_POINT('Ctrl Pts',(43.7090440489059,30.7747854825451,-40.6760208486551));
#250938=CARTESIAN_POINT('Ctrl Pts',(43.6947173014185,30.7907796762741,-40.6770802501629));
#250939=CARTESIAN_POINT('Ctrl Pts',(43.6678443418708,30.8240220908504,-40.6811258797777));
#250940=CARTESIAN_POINT('Ctrl Pts',(43.6427576069985,30.8585127548254,-40.687098273402));
#250941=CARTESIAN_POINT('Ctrl Pts',(43.6212142380078,30.8954846730083,-40.6968894358922));
#250942=CARTESIAN_POINT('Ctrl Pts',(43.6088787182641,30.9193798597989,-40.7042205511341));
#250943=CARTESIAN_POINT('Ctrl Pts',(43.6064685586478,30.9241994859948,-40.7057484197296));
#250944=CARTESIAN_POINT('Ctrl Pts',(43.6017624551859,30.9339175659931,-40.70892606686));
#250945=CARTESIAN_POINT('Ctrl Pts',(43.5994656231147,30.9388193592268,-40.7105773965538));
#250946=CARTESIAN_POINT('Ctrl Pts',(43.5927866482525,30.953560895212,-40.7156875255853));
#250947=CARTESIAN_POINT('Ctrl Pts',(43.5844198153918,30.9733582110501,-40.72293005151));
#250948=CARTESIAN_POINT('Ctrl Pts',(43.5734440082896,31.0034822735469,-40.7350537322951));
#250949=CARTESIAN_POINT('Ctrl Pts',(43.5640181327981,31.0340244080827,-40.7484125407461));
#250950=CARTESIAN_POINT('Ctrl Pts',(43.5561284133843,31.0649820306433,-40.7629929778707));
#250951=CARTESIAN_POINT('Ctrl Pts',(43.5518912037438,31.0858969805267,-40.7735241784737));
#250952=CARTESIAN_POINT('Ctrl Pts',(43.5481682579358,31.1069510729684,-40.7844620267622));
#250953=CARTESIAN_POINT('Ctrl Pts',(43.5465635963524,31.1175527760565,-40.7901372750232));
#250954=CARTESIAN_POINT('Ctrl Pts',(43.5438765944467,31.1388768366658,-40.8018865323646));
#250955=CARTESIAN_POINT('Ctrl Pts',(43.5427912565025,31.1496493641875,-40.8079902348016));
#250956=CARTESIAN_POINT('Ctrl Pts',(43.5411674088753,31.1711124235333,-40.8204828132684));
#250957=CARTESIAN_POINT('Ctrl Pts',(43.5400805588778,31.19253758885,-40.8332822237109));
#250958=CARTESIAN_POINT('Ctrl Pts',(43.5400129658238,31.2352236668913,-40.8600695429299));
#250959=CARTESIAN_POINT('Ctrl Pts',(43.5430492497798,31.2776738375434,-40.8886047446452));
#250960=CARTESIAN_POINT('Ctrl Pts',(43.5491614319672,31.3198884817001,-40.918856387552));
#250961=CARTESIAN_POINT('Ctrl Pts',(43.5532522131496,31.3409199794841,-40.9345594064291));
#250962=CARTESIAN_POINT('Ctrl Pts',(43.5578644352119,31.361905871423,-40.9505475151733));
#250963=CARTESIAN_POINT('Ctrl Pts',(43.560439098329,31.3723994717644,-40.9587035928991));
#250964=CARTESIAN_POINT('Ctrl Pts',(43.5660648897127,31.3931449423641,-40.9751492091434));
#250965=CARTESIAN_POINT('Ctrl Pts',(43.5691234314236,31.4034342087731,-40.9834667538713));
#250966=CARTESIAN_POINT('Ctrl Pts',(43.5790202279964,31.4340221767704,-41.0086741075936));
#250967=CARTESIAN_POINT('Ctrl Pts',(43.5865808644402,31.4540562960243,-41.0258289330007));
#250968=CARTESIAN_POINT('Ctrl Pts',(43.5993606039644,31.4835727602996,-41.0520789232858));
#250969=CARTESIAN_POINT('Ctrl Pts',(43.6038584649574,31.4933175175814,-41.0609109997729));
#250970=CARTESIAN_POINT('Ctrl Pts',(43.6133480280387,31.5126460303085,-41.0787663839806));
#250971=CARTESIAN_POINT('Ctrl Pts',(43.6183219077102,31.5221915251339,-41.0877549157913));
#250972=CARTESIAN_POINT('Ctrl Pts',(43.6338406007018,31.5503182102049,-41.1147514459697));
#250973=CARTESIAN_POINT('Ctrl Pts',(43.6450116757484,31.5684678157769,-41.13285712865));
#250974=CARTESIAN_POINT('Ctrl Pts',(43.6689569093208,31.6035742491305,-41.1692591986645));
#250975=CARTESIAN_POINT('Ctrl Pts',(43.6881189975485,31.6290150958394,-41.1967078345595));
#250976=CARTESIAN_POINT('Ctrl Pts',(43.7160805799803,31.6611548911343,-41.2335986369031));
#250977=CARTESIAN_POINT('Ctrl Pts',(43.7308739938731,31.6766212732249,-41.2521403517739));
#250978=CARTESIAN_POINT('Ctrl Pts',(43.7460847706871,31.6917854492915,-41.2707364845776));
#250979=CARTESIAN_POINT('Ctrl Pts',(43.7539033240721,31.6992171694526,-41.2800648729051));
#250980=CARTESIAN_POINT('Ctrl Pts',(43.7697797892606,31.7136063232936,-41.298562009488));
#250981=CARTESIAN_POINT('Ctrl Pts',(43.7778723272806,31.7205988773597,-41.3077734720143));
#250982=CARTESIAN_POINT('Ctrl Pts',(43.8025568401133,31.7409299545529,-41.3352381600133));
#250983=CARTESIAN_POINT('Ctrl Pts',(43.8195937300504,31.7536621581445,-41.353369616892));
#250984=CARTESIAN_POINT('Ctrl Pts',(43.8547939251157,31.7774712224987,-41.3892512463859));
#250985=CARTESIAN_POINT('Ctrl Pts',(43.8820456950658,31.7940939723408,-41.4158852269725));
#250986=CARTESIAN_POINT('Ctrl Pts',(43.9105977352555,31.8088239425505,-41.4420959852738));
#250987=CARTESIAN_POINT('Ctrl Pts',(43.9299312426308,31.8182163905263,-41.4594780331231));
#250988=CARTESIAN_POINT('Ctrl Pts',(43.9397545046832,31.8226994853967,-41.4681277754213));
#250989=CARTESIAN_POINT('Ctrl Pts',(43.959476379363,31.8311327029401,-41.4851373530728));
#250990=CARTESIAN_POINT('Ctrl Pts',(43.969416794615,31.835103670887,-41.4935351095415));
#250991=CARTESIAN_POINT('Ctrl Pts',(43.9894286782948,31.8425474915593,-41.5100965816665));
#250992=CARTESIAN_POINT('Ctrl Pts',(44.0196562937352,31.8529720625538,-41.5345993599874));
#250993=CARTESIAN_POINT('Ctrl Pts',(44.0607928561344,31.8639280327151,-41.5659272170578));
#250994=CARTESIAN_POINT('Ctrl Pts',(44.0922765794535,31.8699137146658,-41.5884145416429));
#250995=CARTESIAN_POINT('Ctrl Pts',(44.1134085621028,31.8733992175668,-41.6031789442838));
#250996=CARTESIAN_POINT('Ctrl Pts',(44.1240412545,31.8748890570172,-41.6104444862381));
#250997=CARTESIAN_POINT('Ctrl Pts',(44.1401138557838,31.8767382236783,-41.6211788509405));
#250998=CARTESIAN_POINT('Ctrl Pts',(44.1454877988083,31.8772894545129,-41.6247266008247));
#250999=CARTESIAN_POINT('Ctrl Pts',(44.1562140153048,31.878256418298,-41.6317257811562));
#251000=CARTESIAN_POINT('Ctrl Pts',(44.161576905651,31.8786734249769,-41.6351843345794));
#251001=CARTESIAN_POINT('Ctrl Pts',(44.1776466456902,31.8797244502982,-41.6454258391029));
#251002=CARTESIAN_POINT('Ctrl Pts',(44.1883500092183,31.8801603696231,-41.6520850220369));
#251003=CARTESIAN_POINT('Ctrl Pts',(44.2204087008324,31.8806796234647,-41.671549250448));
#251004=CARTESIAN_POINT('Ctrl Pts',(44.2417298059497,31.8799780982567,-41.6838534602333));
#251005=CARTESIAN_POINT('Ctrl Pts',(44.2842582084951,31.8764766164199,-41.7071185815018));
#251006=CARTESIAN_POINT('Ctrl Pts',(44.3054713486111,31.8736750129732,-41.7180819683776));
#251007=CARTESIAN_POINT('Ctrl Pts',(44.3319064277948,31.8688271235064,-41.7309251637703));
#251008=CARTESIAN_POINT('Ctrl Pts',(44.3371930873745,31.8677885276791,-41.7334519256467));
#251009=CARTESIAN_POINT('Ctrl Pts',(44.3477523920959,31.8655764110726,-41.7384157665409));
#251010=CARTESIAN_POINT('Ctrl Pts',(44.353035452149,31.8644001232798,-41.7408573895762));
#251011=CARTESIAN_POINT('Ctrl Pts',(44.368821997144,31.8606750365135,-41.7480268313348));
#251012=CARTESIAN_POINT('Ctrl Pts',(44.3792318927429,31.8579388865424,-41.752586114057));
#251013=CARTESIAN_POINT('Ctrl Pts',(44.4101727404,31.8489724804825,-41.7656371280416));
#251014=CARTESIAN_POINT('Ctrl Pts',(44.4405041748167,31.8385015328462,-41.7774224567595));
#251015=CARTESIAN_POINT('Ctrl Pts',(44.4797386522914,31.8215610256552,-41.7906399779756));
#251016=CARTESIAN_POINT('Ctrl Pts',(44.5085558494592,31.8073558935676,-41.7992982329201));
#251017=CARTESIAN_POINT('Ctrl Pts',(44.5273583247585,31.7968714183439,-41.8042246106906));
#251018=CARTESIAN_POINT('Ctrl Pts',(44.5459478308046,31.7858731708475,-41.8087197459362));
#251019=CARTESIAN_POINT('Ctrl Pts',(44.5551558111633,31.7801015230391,-41.8107541019367));
#251020=CARTESIAN_POINT('Ctrl Pts',(44.5731320510561,31.7681815367951,-41.814338976855));
#251021=CARTESIAN_POINT('Ctrl Pts',(44.5819448307914,31.7620078883687,-41.8159008719862));
#251022=CARTESIAN_POINT('Ctrl Pts',(44.5991987000126,31.7492554022398,-41.8185646224661));
#251023=CARTESIAN_POINT('Ctrl Pts',(44.6245350600795,31.7295108031857,-41.8218731379338));
#251024=CARTESIAN_POINT('Ctrl Pts',(44.6561620699444,31.7007477525095,-41.8235671758672));
#251025=CARTESIAN_POINT('Ctrl Pts',(44.6782580742923,31.6773394437008,-41.8227909065983));
#251026=CARTESIAN_POINT('Ctrl Pts',(44.6926220014235,31.6613194462407,-41.8218112048364));
#251027=CARTESIAN_POINT('Ctrl Pts',(44.6996188611148,31.6531046671394,-41.8210906882841));
#251028=CARTESIAN_POINT('Ctrl Pts',(44.7132456597446,31.6362429219073,-41.8191767031797));
#251029=CARTESIAN_POINT('Ctrl Pts',(44.7198193777268,31.627664624135,-41.8179905956202));
#251030=CARTESIAN_POINT('Ctrl Pts',(44.7324727845908,31.610252798272,-41.8151746307749));
#251031=CARTESIAN_POINT('Ctrl Pts',(44.7507253937504,31.5837345714901,-41.8102826177571));
#251032=CARTESIAN_POINT('Ctrl Pts',(44.7668325292565,31.5560404782777,-41.8034218375205));
#251033=CARTESIAN_POINT('Ctrl Pts',(44.7864242741839,31.5180816884312,-41.7925402952635));
#251034=CARTESIAN_POINT('Ctrl Pts',(44.7952779235527,31.4985810718442,-41.7862298998632));
#251035=CARTESIAN_POINT('Ctrl Pts',(44.8051436066325,31.4735589245645,-41.777240214754));
#251036=CARTESIAN_POINT('Ctrl Pts',(44.8070571630202,31.4685179927861,-41.7753849920635));
#251037=CARTESIAN_POINT('Ctrl Pts',(44.8107609555809,31.4583769076679,-41.7715655844892));
#251038=CARTESIAN_POINT('Ctrl Pts',(44.8125545845603,31.4532656516023,-41.76959682162));
#251039=CARTESIAN_POINT('Ctrl Pts',(44.8177323950795,31.4378873281915,-41.7635424458753));
#251040=CARTESIAN_POINT('Ctrl Pts',(44.8209059367305,31.4276035217402,-41.7593207739311));
#251041=CARTESIAN_POINT('Ctrl Pts',(44.8296276705658,31.3966113763671,-41.7460923602843));
#251042=CARTESIAN_POINT('Ctrl Pts',(44.8391161742293,31.3549585404116,-41.7269730343471));
#251043=CARTESIAN_POINT('Ctrl Pts',(44.8444380100638,31.312658433005,-41.7049510923314));
#251044=CARTESIAN_POINT('Ctrl Pts',(44.8468637082338,31.2806969121874,-41.6873414758157));
#251045=CARTESIAN_POINT('Ctrl Pts',(44.8474108190536,31.2699990859542,-41.6812863637077));
#251046=CARTESIAN_POINT('Ctrl Pts',(44.8478348231013,31.2538978106508,-41.671929084156));
#251047=CARTESIAN_POINT('Ctrl Pts',(44.8479099202363,31.2485174556463,-41.6687616517648));
#251048=CARTESIAN_POINT('Ctrl Pts',(44.8479268208064,31.2377432265879,-41.6623372317338));
#251049=CARTESIAN_POINT('Ctrl Pts',(44.8478683021095,31.2323379437313,-41.6590732331048));
#251050=CARTESIAN_POINT('Ctrl Pts',(44.8474921214824,31.2161555213209,-41.6491783400064));
#251051=CARTESIAN_POINT('Ctrl Pts',(44.8469759958029,31.2054292064128,-41.6424562576898));
#251052=CARTESIAN_POINT('Ctrl Pts',(44.8454249887827,31.1840681958411,-41.6287479728186));
#251053=CARTESIAN_POINT('Ctrl Pts',(44.8423204600693,31.1521790951542,-41.6077983885548));
#251054=CARTESIAN_POINT('Ctrl Pts',(44.8351290816859,31.1102584040656,-41.5783402141209));
#251055=CARTESIAN_POINT('Ctrl Pts',(44.8249268329474,31.0689281614894,-41.54736445114));
#251056=CARTESIAN_POINT('Ctrl Pts',(44.8188163283608,31.0484607830594,-41.5313656278891));
#251057=CARTESIAN_POINT('Ctrl Pts',(44.8121960627665,31.028093840338,-41.5151080950287));
#251058=CARTESIAN_POINT('Ctrl Pts',(44.808629563005,31.0179567656131,-41.5068467714969));
#251059=CARTESIAN_POINT('Ctrl Pts',(44.8009827391877,30.9977990758989,-41.4900714456835));
#251060=CARTESIAN_POINT('Ctrl Pts',(44.7969340070935,30.9878607344767,-41.4816261460579));
#251061=CARTESIAN_POINT('Ctrl Pts',(44.7926621173534,30.9780510210195,-41.4731170634489));
#251062=CARTESIAN_POINT('',(46.348736272544,30.7584582252104,-39.6906856150703));
#251063=CARTESIAN_POINT('',(46.0995611578475,30.7936217551105,-39.9761074628063));
#251064=CARTESIAN_POINT('',(46.348736272544,30.7584582252104,-39.6906856150703));
#251065=CARTESIAN_POINT('',(46.2910026132808,32.4463939541198,-40.0133525199849));
#251066=CARTESIAN_POINT('Ctrl Pts',(46.348736272544,30.7584582252104,-39.6906856150703));
#251067=CARTESIAN_POINT('Ctrl Pts',(46.3614254481729,30.7883280602527,-39.6991946976794));
#251068=CARTESIAN_POINT('Ctrl Pts',(46.3734280792928,30.8185995307445,-39.7076399973049));
#251069=CARTESIAN_POINT('Ctrl Pts',(46.3960461932204,30.8800184397817,-39.7244153231182));
#251070=CARTESIAN_POINT('Ctrl Pts',(46.4065681949313,30.9109152099792,-39.7326766466501));
#251071=CARTESIAN_POINT('Ctrl Pts',(46.4260423093758,30.9730107791217,-39.7489341795107));
#251072=CARTESIAN_POINT('Ctrl Pts',(46.4439553357389,31.0354316602054,-39.764933002761));
#251073=CARTESIAN_POINT('Ctrl Pts',(46.4735992389084,31.1615543100329,-39.7959087657426));
#251074=CARTESIAN_POINT('Ctrl Pts',(46.4940227302404,31.289588481428,-39.8253669401756));
#251075=CARTESIAN_POINT('Ctrl Pts',(46.5023302645975,31.3870655242667,-39.8463165244401));
#251076=CARTESIAN_POINT('Ctrl Pts',(46.506280107836,31.4523789139669,-39.8600248093111));
#251077=CARTESIAN_POINT('Ctrl Pts',(46.5074608406805,31.4851846703929,-39.8667468916278));
#251078=CARTESIAN_POINT('Ctrl Pts',(46.5080123902999,31.5346913151838,-39.8766417847262));
#251079=CARTESIAN_POINT('Ctrl Pts',(46.5079914918558,31.5512299067555,-39.879905783355));
#251080=CARTESIAN_POINT('Ctrl Pts',(46.5075417789082,31.5842004583658,-39.8863302033863));
#251081=CARTESIAN_POINT('Ctrl Pts',(46.5071135271648,31.6006673192385,-39.8894976357773));
#251082=CARTESIAN_POINT('Ctrl Pts',(46.5052230429695,31.6499529002985,-39.8988549153293));
#251083=CARTESIAN_POINT('Ctrl Pts',(46.5031560194756,31.6827076912229,-39.9049100274371));
#251084=CARTESIAN_POINT('Ctrl Pts',(46.494562927216,31.7805948790823,-39.9225196439524));
#251085=CARTESIAN_POINT('Ctrl Pts',(46.4767378404699,31.9102172554903,-39.9445415859684));
#251086=CARTESIAN_POINT('Ctrl Pts',(46.4462022758287,32.0380000397181,-39.9636609119059));
#251087=CARTESIAN_POINT('Ctrl Pts',(46.4184025922855,32.1331342652581,-39.9768893255524));
#251088=CARTESIAN_POINT('Ctrl Pts',(46.4083237615152,32.1647111636399,-39.9811109974971));
#251089=CARTESIAN_POINT('Ctrl Pts',(46.3919309761109,32.2119456968313,-39.9871653732414));
#251090=CARTESIAN_POINT('Ctrl Pts',(46.3862603264385,32.2276473949945,-39.9891341361105));
#251091=CARTESIAN_POINT('Ctrl Pts',(46.3745657539712,32.2588055871924,-39.9929535436847));
#251092=CARTESIAN_POINT('Ctrl Pts',(46.3685310519543,32.2742961715652,-39.9948087663756));
#251093=CARTESIAN_POINT('Ctrl Pts',(46.340730665806,32.3430910112799,-40.00285047101));
#251094=CARTESIAN_POINT('Ctrl Pts',(46.3169453252715,32.3953369342895,-40.0084299233149));
#251095=CARTESIAN_POINT('Ctrl Pts',(46.2910031870661,32.446394079709,-40.0133500693448));
#251096=CARTESIAN_POINT('Ctrl Pts',(46.2910021078285,32.4463936912103,-40.0133527637202));
#251097=CARTESIAN_POINT('Ctrl Pts',(46.3486217884263,32.3037296072064,-40.0136728648342));
#251098=CARTESIAN_POINT('Ctrl Pts',(46.386668413569,32.1539381754564,-40.0127279860568));
#251099=CARTESIAN_POINT('Ctrl Pts',(46.4200060593677,31.8665821327808,-40.0089408346456));
#251100=CARTESIAN_POINT('Ctrl Pts',(46.4197397558165,31.7306141336591,-40.0063483988712));
#251101=CARTESIAN_POINT('Ctrl Pts',(46.3858725160227,31.4446264987979,-39.999488756941));
#251102=CARTESIAN_POINT('Ctrl Pts',(46.3483278372589,31.2963700576375,-39.9950892255237));
#251103=CARTESIAN_POINT('Ctrl Pts',(46.2421281802311,31.027394804457,-39.9857972773175));
#251104=CARTESIAN_POINT('Ctrl Pts',(46.1774476182685,30.90637643183,-39.9810433254305));
#251105=CARTESIAN_POINT('Ctrl Pts',(46.0995611578475,30.7936217551105,-39.9761074628063));
#251106=CARTESIAN_POINT('Ctrl Pts',(46.6981266849492,30.7091523375488,-39.2904704603133));
#251107=CARTESIAN_POINT('Ctrl Pts',(46.6689684123063,30.6404043382273,-39.273452295095));
#251108=CARTESIAN_POINT('Ctrl Pts',(46.6043681216411,30.5066861069553,-39.238925705885));
#251109=CARTESIAN_POINT('Ctrl Pts',(46.5083209189471,30.3487389562033,-39.1945593129175));
#251110=CARTESIAN_POINT('Ctrl Pts',(46.4437937583117,30.2581216171786,-39.1673894861782));
#251111=CARTESIAN_POINT('Ctrl Pts',(46.3992224148768,30.1986447451181,-39.1491520227249));
#251112=CARTESIAN_POINT('Ctrl Pts',(46.3761748773305,30.1693908446446,-39.1399767764946));
#251113=CARTESIAN_POINT('Ctrl Pts',(46.3284414024809,30.1117648114071,-39.1214771434543));
#251114=CARTESIAN_POINT('Ctrl Pts',(46.3038983378397,30.083571828401,-39.112209259666));
#251115=CARTESIAN_POINT('Ctrl Pts',(46.253707387608,30.0286632749651,-39.0937226519629));
#251116=CARTESIAN_POINT('Ctrl Pts',(46.2280147026909,30.001893564456,-39.0844865568113));
#251117=CARTESIAN_POINT('Ctrl Pts',(46.1492148010453,29.9236586721517,-39.0568159196779));
#251118=CARTESIAN_POINT('Ctrl Pts',(46.0669347173688,29.8495134741745,-39.0292038481275));
#251119=CARTESIAN_POINT('Ctrl Pts',(45.9503410384262,29.7587889734315,-38.9925114043613));
#251120=CARTESIAN_POINT('Ctrl Pts',(45.8594191065401,29.6948377475824,-38.9650526418885));
#251121=CARTESIAN_POINT('Ctrl Pts',(45.7964751089327,29.6549785818455,-38.9467936623891));
#251122=CARTESIAN_POINT('Ctrl Pts',(45.748348603817,29.6261284949947,-38.9331097524421));
#251123=CARTESIAN_POINT('Ctrl Pts',(45.7321473284057,29.616684052073,-38.9285487676403));
#251124=CARTESIAN_POINT('Ctrl Pts',(45.6996106203311,29.5982459977232,-38.9194791520014));
#251125=CARTESIAN_POINT('Ctrl Pts',(45.683249044345,29.5892352448745,-38.9149628379356));
#251126=CARTESIAN_POINT('Ctrl Pts',(45.6010439155842,29.5452684013657,-38.8924942188443));
#251127=CARTESIAN_POINT('Ctrl Pts',(45.4667739830181,29.4816584171599,-38.8571935516581));
#251128=CARTESIAN_POINT('Ctrl Pts',(45.2922645146651,29.4187721922835,-38.8147007629208));
#251129=CARTESIAN_POINT('Ctrl Pts',(45.184512437616,29.3885937253944,-38.7899522655792));
#251130=CARTESIAN_POINT('Ctrl Pts',(45.1119891467798,29.3701842541612,-38.7736235920333));
#251131=CARTESIAN_POINT('Ctrl Pts',(45.0754052578815,29.3618381514785,-38.7655490803555));
#251132=CARTESIAN_POINT('Ctrl Pts',(45.0014447932705,29.3468760834356,-38.7495561846596));
#251133=CARTESIAN_POINT('Ctrl Pts',(44.964301863367,29.3403115562353,-38.7416890516424));
#251134=CARTESIAN_POINT('Ctrl Pts',(44.8900079594565,29.3290481892184,-38.726277749838));
#251135=CARTESIAN_POINT('Ctrl Pts',(44.8527936282157,29.324336495618,-38.7187198739728));
#251136=CARTESIAN_POINT('Ctrl Pts',(44.7410083373266,29.3129455735289,-38.6964994820139));
#251137=CARTESIAN_POINT('Ctrl Pts',(44.6662563757167,29.3089967422249,-38.6822807693139));
#251138=CARTESIAN_POINT('Ctrl Pts',(44.516312468428,29.3084067934202,-38.6550493453909));
#251139=CARTESIAN_POINT('Ctrl Pts',(44.441103189525,29.3117700143417,-38.6420342479066));
#251140=CARTESIAN_POINT('Ctrl Pts',(44.3468378615956,29.3206690055189,-38.6265520162729));
#251141=CARTESIAN_POINT('Ctrl Pts',(44.3279589148655,29.3226883315868,-38.6234933649988));
#251142=CARTESIAN_POINT('Ctrl Pts',(44.2901960653062,29.3271995080042,-38.6174591262491));
#251143=CARTESIAN_POINT('Ctrl Pts',(44.271274393292,29.329697893027,-38.614477863833));
#251144=CARTESIAN_POINT('Ctrl Pts',(44.2146592782019,29.3378915995821,-38.60568558559));
#251145=CARTESIAN_POINT('Ctrl Pts',(44.1772069502033,29.344266758826,-38.6000392683017));
#251146=CARTESIAN_POINT('Ctrl Pts',(44.0655444875092,29.3661148598052,-38.5837127379559));
#251147=CARTESIAN_POINT('Ctrl Pts',(43.9553791862171,29.3933792052515,-38.5686255047386));
#251148=CARTESIAN_POINT('Ctrl Pts',(43.8114622524781,29.4404829778103,-38.5509833019505));
#251149=CARTESIAN_POINT('Ctrl Pts',(43.705021834675,29.481230340464,-38.5390021142185));
#251150=CARTESIAN_POINT('Ctrl Pts',(43.6350719757086,29.512061063653,-38.5318621614261));
#251151=CARTESIAN_POINT('Ctrl Pts',(43.5656410085295,29.5447591316771,-38.525155654825));
#251152=CARTESIAN_POINT('Ctrl Pts',(43.5311320054746,29.5620794464364,-38.5220163122062));
#251153=CARTESIAN_POINT('Ctrl Pts',(43.4634866412134,29.5981758355574,-38.5162526847879));
#251154=CARTESIAN_POINT('Ctrl Pts',(43.4301834663392,29.6170276546,-38.5136117755133));
#251155=CARTESIAN_POINT('Ctrl Pts',(43.3647025891651,29.6562685687332,-38.5088155315793));
#251156=CARTESIAN_POINT('Ctrl Pts',(43.2681192378476,29.7174608121974,-38.5023448938576));
#251157=CARTESIAN_POINT('Ctrl Pts',(43.1764049274077,29.7855824582168,-38.4980286134812));
#251158=CARTESIAN_POINT('Ctrl Pts',(43.0584774180437,29.8826126224142,-38.4942050936184));
#251159=CARTESIAN_POINT('Ctrl Pts',(43.001681818637,29.9342392650769,-38.4932590761897));
#251160=CARTESIAN_POINT('Ctrl Pts',(42.8926599718677,30.0438904492243,-38.4933742455196));
#251161=CARTESIAN_POINT('Ctrl Pts',(42.8414047150844,30.1009342501745,-38.4944336470273));
#251162=CARTESIAN_POINT('Ctrl Pts',(42.7451036203247,30.2193471227021,-38.498479276642));
#251163=CARTESIAN_POINT('Ctrl Pts',(42.6550322643363,30.3420646399833,-38.5044516702661));
#251164=CARTESIAN_POINT('Ctrl Pts',(42.5773225406025,30.4733365238586,-38.5142428327574));
#251165=CARTESIAN_POINT('Ctrl Pts',(42.5326943378214,30.5580963840027,-38.5215739479982));
#251166=CARTESIAN_POINT('Ctrl Pts',(42.5239673850246,30.5751883092729,-38.5231018165939));
#251167=CARTESIAN_POINT('Ctrl Pts',(42.5069121510755,30.60964376351,-38.5262794637242));
#251168=CARTESIAN_POINT('Ctrl Pts',(42.4985805781952,30.627019094627,-38.5279307934181));
#251169=CARTESIAN_POINT('Ctrl Pts',(42.4743295471271,30.6792614198295,-38.5330409224498));
#251170=CARTESIAN_POINT('Ctrl Pts',(42.4438856226513,30.7493896366731,-38.5402834483744));
#251171=CARTESIAN_POINT('Ctrl Pts',(42.4037483179465,30.8560072598611,-38.5524071291592));
#251172=CARTESIAN_POINT('Ctrl Pts',(42.3690543371876,30.9640160484273,-38.5657659376104));
#251173=CARTESIAN_POINT('Ctrl Pts',(42.3397558527982,31.0734075527136,-38.5803463747351));
#251174=CARTESIAN_POINT('Ctrl Pts',(42.3238156343608,31.1472555030051,-38.5908775753381));
#251175=CARTESIAN_POINT('Ctrl Pts',(42.3096820427396,31.2215665449467,-38.6018154236264));
#251176=CARTESIAN_POINT('Ctrl Pts',(42.3035171869091,31.2589715314082,-38.6074906718877));
#251177=CARTESIAN_POINT('Ctrl Pts',(42.2930235524414,31.3341791410138,-38.6192399292287));
#251178=CARTESIAN_POINT('Ctrl Pts',(42.2886818075092,31.3721585359098,-38.6253436316658));
#251179=CARTESIAN_POINT('Ctrl Pts',(42.281930630611,31.4478003630713,-38.6378362101326));
#251180=CARTESIAN_POINT('Ctrl Pts',(42.277074994566,31.5232809912004,-38.6506356205751));
#251181=CARTESIAN_POINT('Ctrl Pts',(42.2747992363309,31.6735553614761,-38.6774229397946));
#251182=CARTESIAN_POINT('Ctrl Pts',(42.2834818483937,31.8228397562226,-38.7059581415094));
#251183=CARTESIAN_POINT('Ctrl Pts',(42.3030248127084,31.9711385758679,-38.7362097844166));
#251184=CARTESIAN_POINT('Ctrl Pts',(42.3164494406915,32.0449687602614,-38.7519128032936));
#251185=CARTESIAN_POINT('Ctrl Pts',(42.3317154579634,32.1186122141692,-38.7679009120377));
#251186=CARTESIAN_POINT('Ctrl Pts',(42.3402956643805,32.1554227583218,-38.7760569897633));
#251187=CARTESIAN_POINT('Ctrl Pts',(42.3591481714288,32.228169160774,-38.7925026060078));
#251188=CARTESIAN_POINT('Ctrl Pts',(42.3694448348212,32.2642362896146,-38.8008201507359));
#251189=CARTESIAN_POINT('Ctrl Pts',(42.4028917825415,32.3714169561226,-38.8260275044574));
#251190=CARTESIAN_POINT('Ctrl Pts',(42.428602574983,32.4415633880281,-38.8431823298655));
#251191=CARTESIAN_POINT('Ctrl Pts',(42.4722685042023,32.5448307979217,-38.8694323201497));
#251192=CARTESIAN_POINT('Ctrl Pts',(42.4876674804306,32.5789105800712,-38.8782643966373));
#251193=CARTESIAN_POINT('Ctrl Pts',(42.5202146590728,32.6464795812123,-38.8961197808447));
#251194=CARTESIAN_POINT('Ctrl Pts',(42.5373018269229,32.6798350022668,-38.9051083126545));
#251195=CARTESIAN_POINT('Ctrl Pts',(42.5906929412925,32.7780783962456,-38.9321048428364));
#251196=CARTESIAN_POINT('Ctrl Pts',(42.629225789877,32.8414173722334,-38.9502105255135));
#251197=CARTESIAN_POINT('Ctrl Pts',(42.7120000069194,32.9638220552461,-38.9866125955294));
#251198=CARTESIAN_POINT('Ctrl Pts',(42.7783647966162,33.0524402968179,-39.0140612314234));
#251199=CARTESIAN_POINT('Ctrl Pts',(42.8754380724448,33.1642175243331,-39.0509520337677));
#251200=CARTESIAN_POINT('Ctrl Pts',(42.9268673384212,33.2179450225078,-39.0694937486382));
#251201=CARTESIAN_POINT('Ctrl Pts',(42.9797817061918,33.2705900457306,-39.088089881442));
#251202=CARTESIAN_POINT('Ctrl Pts',(43.0069972096607,33.2963736994336,-39.097418269769));
#251203=CARTESIAN_POINT('Ctrl Pts',(43.0622936398443,33.3462615369726,-39.1159154063528));
#251204=CARTESIAN_POINT('Ctrl Pts',(43.0904949946047,33.3704876748183,-39.1251268688783));
#251205=CARTESIAN_POINT('Ctrl Pts',(43.176562606447,33.4408730143712,-39.1525915568785));
#251206=CARTESIAN_POINT('Ctrl Pts',(43.2360245534179,33.4848790444095,-39.1707230137558));
#251207=CARTESIAN_POINT('Ctrl Pts',(43.358992255749,33.5670176609587,-39.2066046432507));
#251208=CARTESIAN_POINT('Ctrl Pts',(43.4542745623933,33.6242424638975,-39.233238623837));
#251209=CARTESIAN_POINT('Ctrl Pts',(43.5542222374601,33.6747516510336,-39.2594493821381));
#251210=CARTESIAN_POINT('Ctrl Pts',(43.6219256430316,33.7069073870393,-39.2768314299875));
#251211=CARTESIAN_POINT('Ctrl Pts',(43.6563381479934,33.7222286468184,-39.2854811722856));
#251212=CARTESIAN_POINT('Ctrl Pts',(43.7254519170511,33.7509934760635,-39.3024907499371));
#251213=CARTESIAN_POINT('Ctrl Pts',(43.7602995448845,33.7645084608315,-39.3108885064059));
#251214=CARTESIAN_POINT('Ctrl Pts',(43.8304781084082,33.789780836939,-39.3274499785309));
#251215=CARTESIAN_POINT('Ctrl Pts',(43.9365171946568,33.8250735562425,-39.3519527568515));
#251216=CARTESIAN_POINT('Ctrl Pts',(44.0809642638621,33.8617420360433,-39.3832806139221));
#251217=CARTESIAN_POINT('Ctrl Pts',(44.1916183723467,33.8813683146414,-39.4057679385072));
#251218=CARTESIAN_POINT('Ctrl Pts',(44.2659122959159,33.8926702964892,-39.4205323411483));
#251219=CARTESIAN_POINT('Ctrl Pts',(44.3033049221432,33.8974288658374,-39.4277978831022));
#251220=CARTESIAN_POINT('Ctrl Pts',(44.3598453576919,33.9032050944765,-39.4385322478049));
#251221=CARTESIAN_POINT('Ctrl Pts',(44.3787527158677,33.9049006163346,-39.4420799976889));
#251222=CARTESIAN_POINT('Ctrl Pts',(44.4164967874688,33.9078161173588,-39.4490791780208));
#251223=CARTESIAN_POINT('Ctrl Pts',(44.4353708468856,33.9090400957878,-39.4525377314439));
#251224=CARTESIAN_POINT('Ctrl Pts',(44.4919347179527,33.9120095261765,-39.462779235967));
#251225=CARTESIAN_POINT('Ctrl Pts',(44.52962054914,33.9130584408517,-39.4694384189012));
#251226=CARTESIAN_POINT('Ctrl Pts',(44.6425299001817,33.9134342925821,-39.4889026473125));
#251227=CARTESIAN_POINT('Ctrl Pts',(44.7176656228988,33.9100023852834,-39.5012068570978));
#251228=CARTESIAN_POINT('Ctrl Pts',(44.867623327666,33.8957625538083,-39.524471978366));
#251229=CARTESIAN_POINT('Ctrl Pts',(44.9424659600731,33.8849485744664,-39.5354353652432));
#251230=CARTESIAN_POINT('Ctrl Pts',(45.0357885152669,33.8666999843662,-39.5482785606344));
#251231=CARTESIAN_POINT('Ctrl Pts',(45.0544546343785,33.8628074782943,-39.5508053225112));
#251232=CARTESIAN_POINT('Ctrl Pts',(45.091743102575,33.8545484160302,-39.5557691634051));
#251233=CARTESIAN_POINT('Ctrl Pts',(45.1104022544846,33.850171655015,-39.5582107864407));
#251234=CARTESIAN_POINT('Ctrl Pts',(45.1661672125598,33.8363538303533,-39.5653802281989));
#251235=CARTESIAN_POINT('Ctrl Pts',(45.2029511118778,33.8262578362557,-39.5699395109212));
#251236=CARTESIAN_POINT('Ctrl Pts',(45.312316831343,33.7933159380614,-39.582990524906));
#251237=CARTESIAN_POINT('Ctrl Pts',(45.4195983160475,33.7551076509549,-39.5947758536238));
#251238=CARTESIAN_POINT('Ctrl Pts',(45.5585113890164,33.6937328563153,-39.6079933748399));
#251239=CARTESIAN_POINT('Ctrl Pts',(45.6606150024606,33.6424505696195,-39.6166516297843));
#251240=CARTESIAN_POINT('Ctrl Pts',(45.7272860947277,33.6047101271221,-39.6215780075552));
#251241=CARTESIAN_POINT('Ctrl Pts',(45.7932287365117,33.5651705839516,-39.6260731428005));
#251242=CARTESIAN_POINT('Ctrl Pts',(45.8259059249178,33.5444453395394,-39.6281074988013));
#251243=CARTESIAN_POINT('Ctrl Pts',(45.8897275017006,33.5016881508368,-39.6316923737189));
#251244=CARTESIAN_POINT('Ctrl Pts',(45.9210297733036,33.4795651380848,-39.6332542688506));
#251245=CARTESIAN_POINT('Ctrl Pts',(45.9823424846244,33.4339088874735,-39.6359180193303));
#251246=CARTESIAN_POINT('Ctrl Pts',(46.0724202597563,33.3632801300718,-39.6392265347984));
#251247=CARTESIAN_POINT('Ctrl Pts',(46.1850394564173,33.2606222983665,-39.6409205727319));
#251248=CARTESIAN_POINT('Ctrl Pts',(46.2638636333332,33.1772336958075,-39.6401443034625));
#251249=CARTESIAN_POINT('Ctrl Pts',(46.3151397511292,33.1201974856456,-39.6391646017005));
#251250=CARTESIAN_POINT('Ctrl Pts',(46.3401349353408,33.0909661742941,-39.6384440851485));
#251251=CARTESIAN_POINT('Ctrl Pts',(46.3888523044997,33.0309971480077,-39.6365301000439));
#251252=CARTESIAN_POINT('Ctrl Pts',(46.4123735341802,33.0005036828642,-39.6353439924849));
#251253=CARTESIAN_POINT('Ctrl Pts',(46.4576879006691,32.9386388625828,-39.6325280276393));
#251254=CARTESIAN_POINT('Ctrl Pts',(46.52311576659,32.8444620833496,-39.6276360146217));
#251255=CARTESIAN_POINT('Ctrl Pts',(46.5810426872604,32.7462345994881,-39.6207752343847));
#251256=CARTESIAN_POINT('Ctrl Pts',(46.6516918187307,32.6117039458857,-39.6098936921283));
#251257=CARTESIAN_POINT('Ctrl Pts',(46.683723185051,32.5426422373878,-39.6035832967262));
#251258=CARTESIAN_POINT('Ctrl Pts',(46.7195635412788,32.4540883209461,-39.5945936116187));
#251259=CARTESIAN_POINT('Ctrl Pts',(46.7265235775841,32.4362514419463,-39.5927383889278));
#251260=CARTESIAN_POINT('Ctrl Pts',(46.7400123459627,32.4003742100513,-39.5889189813535));
#251261=CARTESIAN_POINT('Ctrl Pts',(46.7465535157541,32.3822946053341,-39.5869502184844));
#251262=CARTESIAN_POINT('Ctrl Pts',(46.7654644360989,32.3279072933142,-39.5808958427402));
#251263=CARTESIAN_POINT('Ctrl Pts',(46.7770937339888,32.2915493874551,-39.5766741707955));
#251264=CARTESIAN_POINT('Ctrl Pts',(46.8091770518909,32.182013131159,-39.5634457571489));
#251265=CARTESIAN_POINT('Ctrl Pts',(46.8444383818759,32.034891308334,-39.5443264312115));
#251266=CARTESIAN_POINT('Ctrl Pts',(46.8650708643864,31.8856621776612,-39.5223044891954));
#251267=CARTESIAN_POINT('Ctrl Pts',(46.8750487417844,31.7729724844591,-39.50469487268));
#251268=CARTESIAN_POINT('Ctrl Pts',(46.8774570362353,31.7352651712118,-39.4986397605723));
#251269=CARTESIAN_POINT('Ctrl Pts',(46.8796767940079,31.6785286095959,-39.4892824810203));
#251270=CARTESIAN_POINT('Ctrl Pts',(46.8801843407089,31.6595724593507,-39.4861150486293));
#251271=CARTESIAN_POINT('Ctrl Pts',(46.8807312344332,31.6216180949417,-39.479690628598));
#251272=CARTESIAN_POINT('Ctrl Pts',(46.8807699646674,31.6025797052015,-39.4764266299692));
#251273=CARTESIAN_POINT('Ctrl Pts',(46.8801790388754,31.5455906639181,-39.4665317368708));
#251274=CARTESIAN_POINT('Ctrl Pts',(46.8788490796135,31.5078273383739,-39.4598096545541));
#251275=CARTESIAN_POINT('Ctrl Pts',(46.874360617844,31.4326451774338,-39.4461013696832));
#251276=CARTESIAN_POINT('Ctrl Pts',(46.864884835636,31.320441459725,-39.4251517854185));
#251277=CARTESIAN_POINT('Ctrl Pts',(46.8414902947658,31.1730719473388,-39.3956936109857));
#251278=CARTESIAN_POINT('Ctrl Pts',(46.8074810934279,31.0279105813681,-39.364717848004));
#251279=CARTESIAN_POINT('Ctrl Pts',(46.7869180083019,30.9560697433081,-39.3487190247537));
#251280=CARTESIAN_POINT('Ctrl Pts',(46.7645577771926,30.884604709384,-39.332461491893));
#251281=CARTESIAN_POINT('Ctrl Pts',(46.7524740339114,30.8490466969583,-39.3242001683612));
#251282=CARTESIAN_POINT('Ctrl Pts',(46.7264943673172,30.7783632715819,-39.3074248425479));
#251283=CARTESIAN_POINT('Ctrl Pts',(46.7127058212706,30.7435263372096,-39.2989795429224));
#251284=CARTESIAN_POINT('Ctrl Pts',(46.6981266849492,30.7091523375488,-39.2904704603133));
#251285=CARTESIAN_POINT('Ctrl Pts',(44.7926621173534,30.9780510210195,-41.4731170634489));
#251286=CARTESIAN_POINT('Ctrl Pts',(44.7841183378731,30.958431594105,-41.4560988982307));
#251287=CARTESIAN_POINT('Ctrl Pts',(44.7652574387158,30.9202429989855,-41.4215723090211));
#251288=CARTESIAN_POINT('Ctrl Pts',(44.7373647422364,30.8750641226134,-41.3772059160528));
#251289=CARTESIAN_POINT('Ctrl Pts',(44.7186826069414,30.8491098680677,-41.3500360893141));
#251290=CARTESIAN_POINT('Ctrl Pts',(44.7057896374646,30.8320666178198,-41.3317986258606));
#251291=CARTESIAN_POINT('Ctrl Pts',(44.6991283043737,30.8236797190306,-41.3226233796301));
#251292=CARTESIAN_POINT('Ctrl Pts',(44.6853430526266,30.8071501195218,-41.3041237465898));
#251293=CARTESIAN_POINT('Ctrl Pts',(44.6782604199269,30.7990587859436,-41.2948558628018));
#251294=CARTESIAN_POINT('Ctrl Pts',(44.6637865272211,30.7832912649286,-41.2763692550984));
#251295=CARTESIAN_POINT('Ctrl Pts',(44.65638232911,30.7755995480316,-41.2671331599469));
#251296=CARTESIAN_POINT('Ctrl Pts',(44.6336879630273,30.7531065345255,-41.2394625228135));
#251297=CARTESIAN_POINT('Ctrl Pts',(44.6100194582072,30.7317609779911,-41.211850451263));
#251298=CARTESIAN_POINT('Ctrl Pts',(44.5765344835469,30.7055824366946,-41.1751580074971));
#251299=CARTESIAN_POINT('Ctrl Pts',(44.5504480754,30.6870962504203,-41.147699245024));
#251300=CARTESIAN_POINT('Ctrl Pts',(44.5324056777293,30.6755504391987,-41.1294402655247));
#251301=CARTESIAN_POINT('Ctrl Pts',(44.5186168522497,30.6671837862428,-41.1157563555777));
#251302=CARTESIAN_POINT('Ctrl Pts',(44.5139760207251,30.6644431539959,-41.1111953707762));
#251303=CARTESIAN_POINT('Ctrl Pts',(44.5046579712977,30.6590892493455,-41.102125755137));
#251304=CARTESIAN_POINT('Ctrl Pts',(44.4999732573772,30.6564710151932,-41.0976094410703));
#251305=CARTESIAN_POINT('Ctrl Pts',(44.4764410055871,30.6436866063214,-41.0751408219827));
#251306=CARTESIAN_POINT('Ctrl Pts',(44.4380363426647,30.6251318507397,-41.0398401547925));
#251307=CARTESIAN_POINT('Ctrl Pts',(44.3881999640401,30.6066279457426,-40.9973473660572));
#251308=CARTESIAN_POINT('Ctrl Pts',(44.3574626802754,30.5976558165788,-40.9725988687145));
#251309=CARTESIAN_POINT('Ctrl Pts',(44.3367823836873,30.5921565153947,-40.9562701951691));
#251310=CARTESIAN_POINT('Ctrl Pts',(44.3263541271388,30.5896491085923,-40.9481956834911));
#251311=CARTESIAN_POINT('Ctrl Pts',(44.3052793937559,30.5851218575581,-40.9322027877955));
#251312=CARTESIAN_POINT('Ctrl Pts',(44.2946995104909,30.5831174982377,-40.924335654778));
#251313=CARTESIAN_POINT('Ctrl Pts',(44.2735450602529,30.5796377993431,-40.9089243529734));
#251314=CARTESIAN_POINT('Ctrl Pts',(44.2629524396991,30.5781585711684,-40.9013664771085));
#251315=CARTESIAN_POINT('Ctrl Pts',(44.2311453972639,30.5744985086998,-40.8791460851492));
#251316=CARTESIAN_POINT('Ctrl Pts',(44.2098907431643,30.5730912421562,-40.8649273724495));
#251317=CARTESIAN_POINT('Ctrl Pts',(44.1672866942957,30.5723474200962,-40.8376959485268));
#251318=CARTESIAN_POINT('Ctrl Pts',(44.1459323927671,30.5730120277702,-40.8246808510428));
#251319=CARTESIAN_POINT('Ctrl Pts',(44.1191870166623,30.5751734135742,-40.8091986194082));
#251320=CARTESIAN_POINT('Ctrl Pts',(44.1138315874482,30.5756735271978,-40.806139968135));
#251321=CARTESIAN_POINT('Ctrl Pts',(44.1031212948485,30.5768077596639,-40.8001057293845));
#251322=CARTESIAN_POINT('Ctrl Pts',(44.0977557278508,30.5774435866632,-40.7971244669688));
#251323=CARTESIAN_POINT('Ctrl Pts',(44.0817045383335,30.5795497856634,-40.7883321887253));
#251324=CARTESIAN_POINT('Ctrl Pts',(44.0710902649836,30.5812139186595,-40.7826858714375));
#251325=CARTESIAN_POINT('Ctrl Pts',(44.0394561806682,30.5869813183234,-40.7663593410916));
#251326=CARTESIAN_POINT('Ctrl Pts',(44.0082701709188,30.5942909050994,-40.7512721078743));
#251327=CARTESIAN_POINT('Ctrl Pts',(43.9675777996734,30.6070988998346,-40.7336299050859));
#251328=CARTESIAN_POINT('Ctrl Pts',(43.9375066395073,30.6182485087226,-40.721648717354));
#251329=CARTESIAN_POINT('Ctrl Pts',(43.917761614853,30.626725808719,-40.7145087645619));
#251330=CARTESIAN_POINT('Ctrl Pts',(43.8981718083816,30.6357351147044,-40.7078022579606));
#251331=CARTESIAN_POINT('Ctrl Pts',(43.8884396229394,30.6405162381665,-40.7046629153417));
#251332=CARTESIAN_POINT('Ctrl Pts',(43.8693712864522,30.6504970769624,-40.6988992879235));
#251333=CARTESIAN_POINT('Ctrl Pts',(43.8599880575193,30.6557176389023,-40.6962583786489));
#251334=CARTESIAN_POINT('Ctrl Pts',(43.8415477166501,30.6665995934339,-40.6914621347147));
#251335=CARTESIAN_POINT('Ctrl Pts',(43.8143622090585,30.6835906587784,-40.6849914969931));
#251336=CARTESIAN_POINT('Ctrl Pts',(43.7885885365895,30.7025683103525,-40.6806752166169));
#251337=CARTESIAN_POINT('Ctrl Pts',(43.7554869731093,30.7296502406846,-40.676851696754));
#251338=CARTESIAN_POINT('Ctrl Pts',(43.7395647886014,30.744083456595,-40.6759056793254));
#251339=CARTESIAN_POINT('Ctrl Pts',(43.7090440489059,30.7747854825451,-40.6760208486551));
#251340=CARTESIAN_POINT('Ctrl Pts',(43.6947173014185,30.7907796762741,-40.6770802501629));
#251341=CARTESIAN_POINT('Ctrl Pts',(43.6678443418708,30.8240220908504,-40.6811258797777));
#251342=CARTESIAN_POINT('Ctrl Pts',(43.6427576069985,30.8585127548254,-40.687098273402));
#251343=CARTESIAN_POINT('Ctrl Pts',(43.6212142380078,30.8954846730083,-40.6968894358922));
#251344=CARTESIAN_POINT('Ctrl Pts',(43.6088787182641,30.9193798597989,-40.7042205511341));
#251345=CARTESIAN_POINT('Ctrl Pts',(43.6064685586478,30.9241994859948,-40.7057484197296));
#251346=CARTESIAN_POINT('Ctrl Pts',(43.6017624551859,30.9339175659931,-40.70892606686));
#251347=CARTESIAN_POINT('Ctrl Pts',(43.5994656231147,30.9388193592268,-40.7105773965538));
#251348=CARTESIAN_POINT('Ctrl Pts',(43.5927866482525,30.953560895212,-40.7156875255853));
#251349=CARTESIAN_POINT('Ctrl Pts',(43.5844198153918,30.9733582110501,-40.72293005151));
#251350=CARTESIAN_POINT('Ctrl Pts',(43.5734440082896,31.0034822735469,-40.7350537322951));
#251351=CARTESIAN_POINT('Ctrl Pts',(43.5640181327981,31.0340244080827,-40.7484125407461));
#251352=CARTESIAN_POINT('Ctrl Pts',(43.5561284133843,31.0649820306433,-40.7629929778707));
#251353=CARTESIAN_POINT('Ctrl Pts',(43.5518912037438,31.0858969805267,-40.7735241784737));
#251354=CARTESIAN_POINT('Ctrl Pts',(43.5481682579358,31.1069510729684,-40.7844620267622));
#251355=CARTESIAN_POINT('Ctrl Pts',(43.5465635963524,31.1175527760565,-40.7901372750232));
#251356=CARTESIAN_POINT('Ctrl Pts',(43.5438765944467,31.1388768366658,-40.8018865323646));
#251357=CARTESIAN_POINT('Ctrl Pts',(43.5427912565025,31.1496493641875,-40.8079902348016));
#251358=CARTESIAN_POINT('Ctrl Pts',(43.5411674088753,31.1711124235333,-40.8204828132684));
#251359=CARTESIAN_POINT('Ctrl Pts',(43.5400805588778,31.19253758885,-40.8332822237109));
#251360=CARTESIAN_POINT('Ctrl Pts',(43.5400129658238,31.2352236668913,-40.8600695429299));
#251361=CARTESIAN_POINT('Ctrl Pts',(43.5430492497798,31.2776738375434,-40.8886047446452));
#251362=CARTESIAN_POINT('Ctrl Pts',(43.5491614319672,31.3198884817001,-40.918856387552));
#251363=CARTESIAN_POINT('Ctrl Pts',(43.5532522131496,31.3409199794841,-40.9345594064291));
#251364=CARTESIAN_POINT('Ctrl Pts',(43.5578644352119,31.361905871423,-40.9505475151733));
#251365=CARTESIAN_POINT('Ctrl Pts',(43.560439098329,31.3723994717644,-40.9587035928991));
#251366=CARTESIAN_POINT('Ctrl Pts',(43.5660648897127,31.3931449423641,-40.9751492091434));
#251367=CARTESIAN_POINT('Ctrl Pts',(43.5691234314236,31.4034342087731,-40.9834667538713));
#251368=CARTESIAN_POINT('Ctrl Pts',(43.5790202279964,31.4340221767704,-41.0086741075936));
#251369=CARTESIAN_POINT('Ctrl Pts',(43.5865808644402,31.4540562960243,-41.0258289330007));
#251370=CARTESIAN_POINT('Ctrl Pts',(43.5993606039644,31.4835727602996,-41.0520789232858));
#251371=CARTESIAN_POINT('Ctrl Pts',(43.6038584649574,31.4933175175814,-41.0609109997729));
#251372=CARTESIAN_POINT('Ctrl Pts',(43.6133480280387,31.5126460303085,-41.0787663839806));
#251373=CARTESIAN_POINT('Ctrl Pts',(43.6183219077102,31.5221915251339,-41.0877549157913));
#251374=CARTESIAN_POINT('Ctrl Pts',(43.6338406007018,31.5503182102049,-41.1147514459697));
#251375=CARTESIAN_POINT('Ctrl Pts',(43.6450116757484,31.5684678157769,-41.13285712865));
#251376=CARTESIAN_POINT('Ctrl Pts',(43.6689569093208,31.6035742491305,-41.1692591986645));
#251377=CARTESIAN_POINT('Ctrl Pts',(43.6881189975485,31.6290150958394,-41.1967078345595));
#251378=CARTESIAN_POINT('Ctrl Pts',(43.7160805799803,31.6611548911343,-41.2335986369031));
#251379=CARTESIAN_POINT('Ctrl Pts',(43.7308739938731,31.6766212732249,-41.2521403517739));
#251380=CARTESIAN_POINT('Ctrl Pts',(43.7460847706871,31.6917854492915,-41.2707364845776));
#251381=CARTESIAN_POINT('Ctrl Pts',(43.7539033240721,31.6992171694526,-41.2800648729051));
#251382=CARTESIAN_POINT('Ctrl Pts',(43.7697797892606,31.7136063232936,-41.298562009488));
#251383=CARTESIAN_POINT('Ctrl Pts',(43.7778723272806,31.7205988773597,-41.3077734720143));
#251384=CARTESIAN_POINT('Ctrl Pts',(43.8025568401133,31.7409299545529,-41.3352381600133));
#251385=CARTESIAN_POINT('Ctrl Pts',(43.8195937300504,31.7536621581445,-41.353369616892));
#251386=CARTESIAN_POINT('Ctrl Pts',(43.8547939251157,31.7774712224987,-41.3892512463859));
#251387=CARTESIAN_POINT('Ctrl Pts',(43.8820456950658,31.7940939723408,-41.4158852269725));
#251388=CARTESIAN_POINT('Ctrl Pts',(43.9105977352555,31.8088239425505,-41.4420959852738));
#251389=CARTESIAN_POINT('Ctrl Pts',(43.9299312426308,31.8182163905263,-41.4594780331231));
#251390=CARTESIAN_POINT('Ctrl Pts',(43.9397545046832,31.8226994853967,-41.4681277754213));
#251391=CARTESIAN_POINT('Ctrl Pts',(43.959476379363,31.8311327029401,-41.4851373530728));
#251392=CARTESIAN_POINT('Ctrl Pts',(43.969416794615,31.835103670887,-41.4935351095415));
#251393=CARTESIAN_POINT('Ctrl Pts',(43.9894286782948,31.8425474915593,-41.5100965816665));
#251394=CARTESIAN_POINT('Ctrl Pts',(44.0196562937352,31.8529720625538,-41.5345993599874));
#251395=CARTESIAN_POINT('Ctrl Pts',(44.0607928561344,31.8639280327151,-41.5659272170578));
#251396=CARTESIAN_POINT('Ctrl Pts',(44.0922765794535,31.8699137146658,-41.5884145416429));
#251397=CARTESIAN_POINT('Ctrl Pts',(44.1134085621028,31.8733992175668,-41.6031789442838));
#251398=CARTESIAN_POINT('Ctrl Pts',(44.1240412545,31.8748890570172,-41.6104444862381));
#251399=CARTESIAN_POINT('Ctrl Pts',(44.1401138557838,31.8767382236783,-41.6211788509405));
#251400=CARTESIAN_POINT('Ctrl Pts',(44.1454877988083,31.8772894545129,-41.6247266008247));
#251401=CARTESIAN_POINT('Ctrl Pts',(44.1562140153048,31.878256418298,-41.6317257811562));
#251402=CARTESIAN_POINT('Ctrl Pts',(44.161576905651,31.8786734249769,-41.6351843345794));
#251403=CARTESIAN_POINT('Ctrl Pts',(44.1776466456902,31.8797244502982,-41.6454258391029));
#251404=CARTESIAN_POINT('Ctrl Pts',(44.1883500092183,31.8801603696231,-41.6520850220369));
#251405=CARTESIAN_POINT('Ctrl Pts',(44.2204087008324,31.8806796234647,-41.671549250448));
#251406=CARTESIAN_POINT('Ctrl Pts',(44.2417298059497,31.8799780982567,-41.6838534602333));
#251407=CARTESIAN_POINT('Ctrl Pts',(44.2842582084951,31.8764766164199,-41.7071185815018));
#251408=CARTESIAN_POINT('Ctrl Pts',(44.3054713486111,31.8736750129732,-41.7180819683776));
#251409=CARTESIAN_POINT('Ctrl Pts',(44.3319064277948,31.8688271235064,-41.7309251637703));
#251410=CARTESIAN_POINT('Ctrl Pts',(44.3371930873745,31.8677885276791,-41.7334519256467));
#251411=CARTESIAN_POINT('Ctrl Pts',(44.3477523920959,31.8655764110726,-41.7384157665409));
#251412=CARTESIAN_POINT('Ctrl Pts',(44.353035452149,31.8644001232798,-41.7408573895762));
#251413=CARTESIAN_POINT('Ctrl Pts',(44.368821997144,31.8606750365135,-41.7480268313348));
#251414=CARTESIAN_POINT('Ctrl Pts',(44.3792318927429,31.8579388865424,-41.752586114057));
#251415=CARTESIAN_POINT('Ctrl Pts',(44.4101727404,31.8489724804825,-41.7656371280416));
#251416=CARTESIAN_POINT('Ctrl Pts',(44.4405041748167,31.8385015328462,-41.7774224567595));
#251417=CARTESIAN_POINT('Ctrl Pts',(44.4797386522914,31.8215610256552,-41.7906399779756));
#251418=CARTESIAN_POINT('Ctrl Pts',(44.5085558494592,31.8073558935676,-41.7992982329201));
#251419=CARTESIAN_POINT('Ctrl Pts',(44.5273583247585,31.7968714183439,-41.8042246106906));
#251420=CARTESIAN_POINT('Ctrl Pts',(44.5459478308046,31.7858731708475,-41.8087197459362));
#251421=CARTESIAN_POINT('Ctrl Pts',(44.5551558111633,31.7801015230391,-41.8107541019367));
#251422=CARTESIAN_POINT('Ctrl Pts',(44.5731320510561,31.7681815367951,-41.814338976855));
#251423=CARTESIAN_POINT('Ctrl Pts',(44.5819448307914,31.7620078883687,-41.8159008719862));
#251424=CARTESIAN_POINT('Ctrl Pts',(44.5991987000126,31.7492554022398,-41.8185646224661));
#251425=CARTESIAN_POINT('Ctrl Pts',(44.6245350600795,31.7295108031857,-41.8218731379338));
#251426=CARTESIAN_POINT('Ctrl Pts',(44.6561620699444,31.7007477525095,-41.8235671758672));
#251427=CARTESIAN_POINT('Ctrl Pts',(44.6782580742923,31.6773394437008,-41.8227909065983));
#251428=CARTESIAN_POINT('Ctrl Pts',(44.6926220014235,31.6613194462407,-41.8218112048364));
#251429=CARTESIAN_POINT('Ctrl Pts',(44.6996188611148,31.6531046671394,-41.8210906882841));
#251430=CARTESIAN_POINT('Ctrl Pts',(44.7132456597446,31.6362429219073,-41.8191767031797));
#251431=CARTESIAN_POINT('Ctrl Pts',(44.7198193777268,31.627664624135,-41.8179905956202));
#251432=CARTESIAN_POINT('Ctrl Pts',(44.7324727845908,31.610252798272,-41.8151746307749));
#251433=CARTESIAN_POINT('Ctrl Pts',(44.7507253937504,31.5837345714901,-41.8102826177571));
#251434=CARTESIAN_POINT('Ctrl Pts',(44.7668325292565,31.5560404782777,-41.8034218375205));
#251435=CARTESIAN_POINT('Ctrl Pts',(44.7864242741839,31.5180816884312,-41.7925402952635));
#251436=CARTESIAN_POINT('Ctrl Pts',(44.7952779235527,31.4985810718442,-41.7862298998632));
#251437=CARTESIAN_POINT('Ctrl Pts',(44.8051436066325,31.4735589245645,-41.777240214754));
#251438=CARTESIAN_POINT('Ctrl Pts',(44.8070571630202,31.4685179927861,-41.7753849920635));
#251439=CARTESIAN_POINT('Ctrl Pts',(44.8107609555809,31.4583769076679,-41.7715655844892));
#251440=CARTESIAN_POINT('Ctrl Pts',(44.8125545845603,31.4532656516023,-41.76959682162));
#251441=CARTESIAN_POINT('Ctrl Pts',(44.8177323950795,31.4378873281915,-41.7635424458753));
#251442=CARTESIAN_POINT('Ctrl Pts',(44.8209059367305,31.4276035217402,-41.7593207739311));
#251443=CARTESIAN_POINT('Ctrl Pts',(44.8296276705658,31.3966113763671,-41.7460923602843));
#251444=CARTESIAN_POINT('Ctrl Pts',(44.8391161742293,31.3549585404116,-41.7269730343471));
#251445=CARTESIAN_POINT('Ctrl Pts',(44.8444380100638,31.312658433005,-41.7049510923314));
#251446=CARTESIAN_POINT('Ctrl Pts',(44.8468637082338,31.2806969121874,-41.6873414758157));
#251447=CARTESIAN_POINT('Ctrl Pts',(44.8474108190536,31.2699990859542,-41.6812863637077));
#251448=CARTESIAN_POINT('Ctrl Pts',(44.8478348231013,31.2538978106508,-41.671929084156));
#251449=CARTESIAN_POINT('Ctrl Pts',(44.8479099202363,31.2485174556463,-41.6687616517648));
#251450=CARTESIAN_POINT('Ctrl Pts',(44.8479268208064,31.2377432265879,-41.6623372317338));
#251451=CARTESIAN_POINT('Ctrl Pts',(44.8478683021095,31.2323379437313,-41.6590732331048));
#251452=CARTESIAN_POINT('Ctrl Pts',(44.8474921214824,31.2161555213209,-41.6491783400064));
#251453=CARTESIAN_POINT('Ctrl Pts',(44.8469759958029,31.2054292064128,-41.6424562576898));
#251454=CARTESIAN_POINT('Ctrl Pts',(44.8454249887827,31.1840681958411,-41.6287479728186));
#251455=CARTESIAN_POINT('Ctrl Pts',(44.8423204600693,31.1521790951542,-41.6077983885548));
#251456=CARTESIAN_POINT('Ctrl Pts',(44.8351290816859,31.1102584040656,-41.5783402141209));
#251457=CARTESIAN_POINT('Ctrl Pts',(44.8249268329474,31.0689281614894,-41.54736445114));
#251458=CARTESIAN_POINT('Ctrl Pts',(44.8188163283608,31.0484607830594,-41.5313656278891));
#251459=CARTESIAN_POINT('Ctrl Pts',(44.8121960627665,31.028093840338,-41.5151080950287));
#251460=CARTESIAN_POINT('Ctrl Pts',(44.808629563005,31.0179567656131,-41.5068467714969));
#251461=CARTESIAN_POINT('Ctrl Pts',(44.8009827391877,30.9977990758989,-41.4900714456835));
#251462=CARTESIAN_POINT('Ctrl Pts',(44.7969340070935,30.9878607344767,-41.4816261460579));
#251463=CARTESIAN_POINT('Ctrl Pts',(44.7926621173534,30.9780510210195,-41.4731170634489));
#251464=CARTESIAN_POINT('',(42.6662672096693,32.3203213022045,-39.2608974781454));
#251465=CARTESIAN_POINT('',(42.8533186609869,32.1498328366219,-39.6198492128429));
#251466=CARTESIAN_POINT('',(42.6662672096693,32.3203213022045,-39.2608974781454));
#251467=CARTESIAN_POINT('Origin',(44.5948075437535,31.4456508901469,-39.4587542606758));
#251468=CARTESIAN_POINT('Ctrl Pts',(42.5996246294394,32.1390101092634,-39.2098678882799));
#251469=CARTESIAN_POINT('Ctrl Pts',(42.5778854323284,31.9533222655754,-39.2197530981027));
#251470=CARTESIAN_POINT('Ctrl Pts',(42.5749625469443,31.7663344672666,-39.2248889570454));
#251471=CARTESIAN_POINT('Ctrl Pts',(42.6153194208193,31.3447914220134,-39.227652546232));
#251472=CARTESIAN_POINT('Ctrl Pts',(42.6710207843962,31.1137099758597,-39.2229144237327));
#251473=CARTESIAN_POINT('Ctrl Pts',(42.8122767959315,30.7727304789194,-39.2094810818855));
#251474=CARTESIAN_POINT('Ctrl Pts',(42.8730213773354,30.6564231621241,-39.2038964044379));
#251475=CARTESIAN_POINT('Ctrl Pts',(42.9570024701842,30.5246587771562,-39.1952391038725));
#251476=CARTESIAN_POINT('Ctrl Pts',(42.9703798319536,30.5043770417005,-39.1938226714298));
#251477=CARTESIAN_POINT('Ctrl Pts',(42.9857295783759,30.4818787161795,-39.1921578967565));
#251478=CARTESIAN_POINT('Ctrl Pts',(42.9874048472462,30.4794333222496,-39.1919756969673));
#251479=CARTESIAN_POINT('Ctrl Pts',(43.0478538286388,30.3915574743341,-39.1853833703606));
#251480=CARTESIAN_POINT('Ctrl Pts',(43.1120893711745,30.3104168174511,-39.1777786535206));
#251481=CARTESIAN_POINT('Ctrl Pts',(43.2866950275929,30.1179734855588,-39.1559135146894));
#251482=CARTESIAN_POINT('Ctrl Pts',(43.4026330192994,30.0137306736984,-39.1404076188054));
#251483=CARTESIAN_POINT('Ctrl Pts',(43.7432241441741,29.7628250133007,-39.0923982295612));
#251484=CARTESIAN_POINT('Ctrl Pts',(43.9830229737115,29.6420959083149,-39.0560763077533));
#251485=CARTESIAN_POINT('Ctrl Pts',(44.236619853131,29.5589442208509,-39.0141970922745));
#251486=CARTESIAN_POINT('Ctrl Pts',(44.2366195673479,29.558943308954,-39.0141953208016));
#251487=CARTESIAN_POINT('Ctrl Pts',(44.2485133712811,29.5573147073404,-39.016338804237));
#251488=CARTESIAN_POINT('Ctrl Pts',(44.2604132202835,29.5557943338693,-39.0185056969943));
#251489=CARTESIAN_POINT('Ctrl Pts',(44.2722948154515,29.5543845957057,-39.0206914003809));
#251490=CARTESIAN_POINT('Ctrl Pts',(44.288696030367,29.5524386096434,-39.0237085197559));
#251491=CARTESIAN_POINT('Ctrl Pts',(44.3050952734897,29.5506978499007,-39.0267671710297));
#251492=CARTESIAN_POINT('Ctrl Pts',(44.3214722160119,29.5491651362618,-39.0298636173565));
#251493=CARTESIAN_POINT('Ctrl Pts',(44.386979986101,29.5430342817064,-39.0422494026637));
#251494=CARTESIAN_POINT('Ctrl Pts',(44.4523142911657,29.540165884783,-39.055264500148));
#251495=CARTESIAN_POINT('Ctrl Pts',(44.5174452018332,29.5404749664642,-39.0688802121094));
#251496=CARTESIAN_POINT('Ctrl Pts',(44.5825761125008,29.5407840481455,-39.0824959240709));
#251497=CARTESIAN_POINT('Ctrl Pts',(44.64751868345,29.5442668522271,-39.0967146367708));
#251498=CARTESIAN_POINT('Ctrl Pts',(44.7122655456777,29.5509157680261,-39.1115282314101));
#251499=CARTESIAN_POINT('Ctrl Pts',(44.7446389767916,29.5542402259256,-39.1189350287298));
#251500=CARTESIAN_POINT('Ctrl Pts',(44.7769718892781,29.5583592071516,-39.126492904595));
#251501=CARTESIAN_POINT('Ctrl Pts',(44.8092469543587,29.5632772749199,-39.1341985554972));
#251502=CARTESIAN_POINT('Ctrl Pts',(44.8415220194394,29.5681953426883,-39.1419042063993));
#251503=CARTESIAN_POINT('Ctrl Pts',(44.8737942873649,29.5739237069059,-39.1497713394166));
#251504=CARTESIAN_POINT('Ctrl Pts',(44.9059258943645,29.5804480647761,-39.1577677872645));
#251505=CARTESIAN_POINT('Ctrl Pts',(44.938057501364,29.5869724226462,-39.1657642351124));
#251506=CARTESIAN_POINT('Ctrl Pts',(44.9698454327154,29.5942479284802,-39.1738387467903));
#251507=CARTESIAN_POINT('Ctrl Pts',(45.0013540521658,29.6022690447017,-39.1820030835632));
#251508=CARTESIAN_POINT('Ctrl Pts',(45.0328626716162,29.6102901609231,-39.1901674203362));
#251509=CARTESIAN_POINT('Ctrl Pts',(45.0640729757577,29.6190530375165,-39.1984168566288));
#251510=CARTESIAN_POINT('Ctrl Pts',(45.0949896013656,29.6285455570274,-39.2067492398949));
#251511=CARTESIAN_POINT('Ctrl Pts',(45.156822852581,29.6475305960497,-39.2234140064273));
#251512=CARTESIAN_POINT('Ctrl Pts',(45.2174823675629,29.6694301295854,-39.2404109353306));
#251513=CARTESIAN_POINT('Ctrl Pts',(45.2769854784582,29.6942159135793,-39.2577349344145));
#251514=CARTESIAN_POINT('Ctrl Pts',(45.3364885893535,29.7190016975732,-39.2750589334985));
#251515=CARTESIAN_POINT('Ctrl Pts',(45.394834111845,29.7466769167217,-39.2927093736018));
#251516=CARTESIAN_POINT('Ctrl Pts',(45.4519914987675,29.7772762445693,-39.3106842688742));
#251517=CARTESIAN_POINT('Ctrl Pts',(45.4662808454981,29.7849260765312,-39.3151779926924));
#251518=CARTESIAN_POINT('Ctrl Pts',(45.4805013249128,29.7927646822922,-39.3196943067583));
#251519=CARTESIAN_POINT('Ctrl Pts',(45.4946409653392,29.8007841394154,-39.3242291145778));
#251520=CARTESIAN_POINT('Ctrl Pts',(45.5087806057656,29.8088035965387,-39.3287639223973));
#251521=CARTESIAN_POINT('Ctrl Pts',(45.5228621313133,29.8170188131519,-39.333324907199));
#251522=CARTESIAN_POINT('Ctrl Pts',(45.5368055540997,29.8253835454178,-39.3378862105147));
#251523=CARTESIAN_POINT('Ctrl Pts',(45.5646923996724,29.8421130099497,-39.3470088171461));
#251524=CARTESIAN_POINT('Ctrl Pts',(45.592047766323,29.8594467945522,-39.3561383047734));
#251525=CARTESIAN_POINT('Ctrl Pts',(45.6188977087295,29.8773827904181,-39.3652795111332));
#251526=CARTESIAN_POINT('Ctrl Pts',(45.645747651136,29.8953187862839,-39.3744207174929));
#251527=CARTESIAN_POINT('Ctrl Pts',(45.6720921468082,29.913857035864,-39.3835736164339));
#251528=CARTESIAN_POINT('Ctrl Pts',(45.6979337955271,29.9329872123234,-39.3927366395782));
#251529=CARTESIAN_POINT('Ctrl Pts',(45.723775444246,29.9521173887828,-39.4018996627226));
#251530=CARTESIAN_POINT('Ctrl Pts',(45.7491143076062,29.9718394539443,-39.4110727653601));
#251531=CARTESIAN_POINT('Ctrl Pts',(45.7739546683399,29.9921505677002,-39.4202560992287));
#251532=CARTESIAN_POINT('Ctrl Pts',(45.8068346095582,30.0190353715716,-39.4324116182663));
#251533=CARTESIAN_POINT('Ctrl Pts',(45.8388420879535,30.0469508662714,-39.4445853507697));
#251534=CARTESIAN_POINT('Ctrl Pts',(45.8699706488795,30.0759012064987,-39.4567766090453));
#251535=CARTESIAN_POINT('Ctrl Pts',(45.8699705802672,30.0759010588502,-39.4567767210169));
#251536=CARTESIAN_POINT('Ctrl Pts',(45.7207779205447,29.9782872881653,-39.4493772126299));
#251537=CARTESIAN_POINT('Ctrl Pts',(45.5599480087114,29.8999062682101,-39.443153002748));
#251538=CARTESIAN_POINT('Ctrl Pts',(45.2312083411652,29.7880737938443,-39.4337065378474));
#251539=CARTESIAN_POINT('Ctrl Pts',(45.0639383024835,29.7527249035763,-39.4303654026819));
#251540=CARTESIAN_POINT('Ctrl Pts',(44.7172828005758,29.7227187429158,-39.4261204619104));
#251541=CARTESIAN_POINT('Ctrl Pts',(44.4580078817622,29.7223780036854,-39.4233297449024));
#251542=CARTESIAN_POINT('Ctrl Pts',(43.9688200623754,29.8616791617328,-39.4312638039626));
#251543=CARTESIAN_POINT('Ctrl Pts',(43.7845565914904,29.9464353434952,-39.4372490396889));
#251544=CARTESIAN_POINT('Ctrl Pts',(43.4833583146081,30.1477786147003,-39.451636962852));
#251545=CARTESIAN_POINT('Ctrl Pts',(43.3618510615377,30.253415997476,-39.4592126441986));
#251546=CARTESIAN_POINT('Ctrl Pts',(43.2339064911603,30.3970340532892,-39.4692641092024));
#251547=CARTESIAN_POINT('Ctrl Pts',(43.2133112308633,30.4213696846452,-39.4709597499161));
#251548=CARTESIAN_POINT('Ctrl Pts',(43.1834134449199,30.4585680431386,-39.4735415640413));
#251549=CARTESIAN_POINT('Ctrl Pts',(43.1736501665408,30.4710326685332,-39.4744052149167));
#251550=CARTESIAN_POINT('Ctrl Pts',(43.1592837513826,30.4898576355279,-39.4757067642036));
#251551=CARTESIAN_POINT('Ctrl Pts',(43.1545612559406,30.4961264783958,-39.4761397377086));
#251552=CARTESIAN_POINT('Ctrl Pts',(43.1475388808391,30.5055703919114,-39.476791296143));
#251553=CARTESIAN_POINT('Ctrl Pts',(43.1452096879129,30.5087232484512,-39.4770087021575));
#251554=CARTESIAN_POINT('Ctrl Pts',(43.0728360470021,30.6073319480963,-39.4838046000217));
#251555=CARTESIAN_POINT('Ctrl Pts',(42.9826289996721,30.7481521195083,-39.4928576045613));
#251556=CARTESIAN_POINT('Ctrl Pts',(42.8339657780202,31.1281625580106,-39.5216333315955));
#251557=CARTESIAN_POINT('Ctrl Pts',(42.791434110928,31.331147172449,-39.5386487817205));
#251558=CARTESIAN_POINT('Ctrl Pts',(42.7726932000113,31.7434993189507,-39.5768149205341));
#251559=CARTESIAN_POINT('Ctrl Pts',(42.7969939924394,31.9505108240015,-39.5977725133492));
#251560=CARTESIAN_POINT('Ctrl Pts',(42.8533186609868,32.1498328366219,-39.6198492128429));
#251561=CARTESIAN_POINT('Ctrl Pts',(46.6981267205988,30.7091523325179,-39.2904704194778));
#251562=CARTESIAN_POINT('Ctrl Pts',(46.6835475840845,30.6747783323977,-39.2819613368687));
#251563=CARTESIAN_POINT('Ctrl Pts',(46.6681815313185,30.6408774203964,-39.2733908710118));
#251564=CARTESIAN_POINT('Ctrl Pts',(46.6359019577837,30.5740061471226,-39.2561284474008));
#251565=CARTESIAN_POINT('Ctrl Pts',(46.6189883510676,30.5410358371774,-39.2474364841832));
#251566=CARTESIAN_POINT('Ctrl Pts',(46.5659489722029,30.4435074198558,-39.2211790841066));
#251567=CARTESIAN_POINT('Ctrl Pts',(46.5275294727818,30.380328928234,-39.2034324856053));
#251568=CARTESIAN_POINT('Ctrl Pts',(46.4653032277899,30.2883271564893,-39.1764460813684));
#251569=CARTESIAN_POINT('Ctrl Pts',(46.4437937905871,30.2581216061217,-39.1673894453427));
#251570=CARTESIAN_POINT('Ctrl Pts',(46.3992224465595,30.1986447332673,-39.1491519818895));
#251571=CARTESIAN_POINT('Ctrl Pts',(46.3761749087066,30.1693908324035,-39.1399767356591));
#251572=CARTESIAN_POINT('Ctrl Pts',(46.3284414332219,30.1117647983971,-39.1214771026188));
#251573=CARTESIAN_POINT('Ctrl Pts',(46.303898368254,30.0835718150149,-39.1122092188305));
#251574=CARTESIAN_POINT('Ctrl Pts',(46.2537074173542,30.0286632608467,-39.0937226111275));
#251575=CARTESIAN_POINT('Ctrl Pts',(46.2280147320948,30.0018935499806,-39.0844865159759));
#251576=CARTESIAN_POINT('Ctrl Pts',(46.1492148293995,29.9236586566334,-39.0568158788424));
#251577=CARTESIAN_POINT('Ctrl Pts',(46.0943604073998,29.8742287721887,-39.0384076932709));
#251578=CARTESIAN_POINT('Ctrl Pts',(46.0086385620827,29.8041510367818,-39.0108576711398));
#251579=CARTESIAN_POINT('Ctrl Pts',(45.9794896966975,29.7814700124874,-39.0016844996603));
#251580=CARTESIAN_POINT('Ctrl Pts',(45.9200349383669,29.7374728126538,-38.9833588188378));
#251581=CARTESIAN_POINT('Ctrl Pts',(45.8897290958639,29.7161565779658,-38.9742063077404));
#251582=CARTESIAN_POINT('Ctrl Pts',(45.8279451414554,29.674906815849,-38.9559225219059));
#251583=CARTESIAN_POINT('Ctrl Pts',(45.7964751325824,29.6549785627515,-38.9467936215536));
#251584=CARTESIAN_POINT('Ctrl Pts',(45.7483486268243,29.6261284755174,-38.9331097116066));
#251585=CARTESIAN_POINT('Ctrl Pts',(45.7321473511967,29.6166840324703,-38.9285487268047));
#251586=CARTESIAN_POINT('Ctrl Pts',(45.6996106426877,29.5982459778757,-38.9194791111659));
#251587=CARTESIAN_POINT('Ctrl Pts',(45.6832490664831,29.5892352249074,-38.9149627971));
#251588=CARTESIAN_POINT('Ctrl Pts',(45.6010439366246,29.5452683808152,-38.8924941780088));
#251589=CARTESIAN_POINT('Ctrl Pts',(45.533907519743,29.5134615094348,-38.8748432564238));
#251590=CARTESIAN_POINT('Ctrl Pts',(45.3969716065162,29.4565064723111,-38.8401970944675));
#251591=CARTESIAN_POINT('Ctrl Pts',(45.3271663113639,29.4313507911438,-38.8231995021285));
#251592=CARTESIAN_POINT('Ctrl Pts',(45.220429860233,29.3986526185597,-38.7982016312344));
#251593=CARTESIAN_POINT('Ctrl Pts',(45.1845124530894,29.3885937027738,-38.7899522247438));
#251594=CARTESIAN_POINT('Ctrl Pts',(45.1119891612833,29.3701842312991,-38.7736235511978));
#251595=CARTESIAN_POINT('Ctrl Pts',(45.0754052718956,29.3618381285072,-38.76554903952));
#251596=CARTESIAN_POINT('Ctrl Pts',(45.0014448062951,29.346876060269,-38.7495561438242));
#251597=CARTESIAN_POINT('Ctrl Pts',(44.9643018758947,29.3403115329834,-38.7416890108069));
#251598=CARTESIAN_POINT('Ctrl Pts',(44.89000797099,29.3290481658209,-38.7262777090026));
#251599=CARTESIAN_POINT('Ctrl Pts',(44.8527936392512,29.32433647216,-38.7187198331373));
#251600=CARTESIAN_POINT('Ctrl Pts',(44.7410083468657,29.3129455499263,-38.6964994411784));
#251601=CARTESIAN_POINT('Ctrl Pts',(44.6662563842549,29.3089967185748,-38.6822807284784));
#251602=CARTESIAN_POINT('Ctrl Pts',(44.516312474958,29.3084067697729,-38.6550493045554));
#251603=CARTESIAN_POINT('Ctrl Pts',(44.4411031950474,29.3117699907449,-38.6420342070711));
#251604=CARTESIAN_POINT('Ctrl Pts',(44.3468378658548,29.3206689820482,-38.6265519754374));
#251605=CARTESIAN_POINT('Ctrl Pts',(44.3279589188716,29.3226883081445,-38.6234933241634));
#251606=CARTESIAN_POINT('Ctrl Pts',(44.2901960688061,29.327199484625,-38.6174590854136));
#251607=CARTESIAN_POINT('Ctrl Pts',(44.2712743965384,29.3296978696828,-38.6144778229975));
#251608=CARTESIAN_POINT('Ctrl Pts',(44.2146592806893,29.3378915763517,-38.6056855447545));
#251609=CARTESIAN_POINT('Ctrl Pts',(44.1772069521887,29.3442667356837,-38.6000392274662));
#251610=CARTESIAN_POINT('Ctrl Pts',(44.1027653093944,29.3588321365371,-38.5891548739024));
#251611=CARTESIAN_POINT('Ctrl Pts',(44.0657945493931,29.367019473238,-38.5839196795321));
#251612=CARTESIAN_POINT('Ctrl Pts',(43.9923490651605,29.3851891795989,-38.5738612044767));
#251613=CARTESIAN_POINT('Ctrl Pts',(43.9558743453872,29.3951715650289,-38.5690379266201));
#251614=CARTESIAN_POINT('Ctrl Pts',(43.8834205256851,29.4169303775312,-38.5598042071748));
#251615=CARTESIAN_POINT('Ctrl Pts',(43.8474414227296,29.4287067933557,-38.5553937623361));
#251616=CARTESIAN_POINT('Ctrl Pts',(43.7759820552624,29.4540657978905,-38.546989591198));
#251617=CARTESIAN_POINT('Ctrl Pts',(43.7405017799738,29.4676483473598,-38.542995855313));
#251618=CARTESIAN_POINT('Ctrl Pts',(43.6700470429442,29.4966453190668,-38.5354320574723));
#251619=CARTESIAN_POINT('Ctrl Pts',(43.6350719704198,29.5120610427986,-38.5318621205907));
#251620=CARTESIAN_POINT('Ctrl Pts',(43.5656410023081,29.5447591112658,-38.5251556139896));
#251621=CARTESIAN_POINT('Ctrl Pts',(43.5311319987896,29.5620794262597,-38.5220162713707));
#251622=CARTESIAN_POINT('Ctrl Pts',(43.4634866336197,29.5981758158694,-38.5162526439524));
#251623=CARTESIAN_POINT('Ctrl Pts',(43.4301834582978,29.617027635167,-38.5136117346778));
#251624=CARTESIAN_POINT('Ctrl Pts',(43.3647025802437,29.6562685498308,-38.5088154907438));
#251625=CARTESIAN_POINT('Ctrl Pts',(43.3325078138225,29.6766655352735,-38.5066584800714));
#251626=CARTESIAN_POINT('Ctrl Pts',(43.2375484215017,29.7401688684101,-38.5009063557603));
#251627=CARTESIAN_POINT('Ctrl Pts',(43.1764049159542,29.7855824410607,-38.4980285726457));
#251628=CARTESIAN_POINT('Ctrl Pts',(43.0584774050032,29.8826126065668,-38.494205052783));
#251629=CARTESIAN_POINT('Ctrl Pts',(43.0016818048319,29.9342392499254,-38.4932590353542));
#251630=CARTESIAN_POINT('Ctrl Pts',(42.8926599565938,30.0438904355498,-38.4933742046842));
#251631=CARTESIAN_POINT('Ctrl Pts',(42.8414046991196,30.1009342372681,-38.4944336061919));
#251632=CARTESIAN_POINT('Ctrl Pts',(42.745103603061,30.2193471113892,-38.4984792358066));
#251633=CARTESIAN_POINT('Ctrl Pts',(42.7000683931882,30.2807072512537,-38.5014657717858));
#251634=CARTESIAN_POINT('Ctrl Pts',(42.6161769147351,30.4076991927421,-38.509346871509));
#251635=CARTESIAN_POINT('Ctrl Pts',(42.5773225210722,30.4733365159606,-38.5142427919219));
#251636=CARTESIAN_POINT('Ctrl Pts',(42.5326943176869,30.5580963772433,-38.5215739071627));
#251637=CARTESIAN_POINT('Ctrl Pts',(42.5239673647719,30.5751883027432,-38.5231017757584));
#251638=CARTESIAN_POINT('Ctrl Pts',(42.5069121305918,30.6096437574431,-38.5262794228887));
#251639=CARTESIAN_POINT('Ctrl Pts',(42.4985805575985,30.6270190887935,-38.5279307525826));
#251640=CARTESIAN_POINT('Ctrl Pts',(42.4743295262018,30.6792614146976,-38.5330408816144));
#251641=CARTESIAN_POINT('Ctrl Pts',(42.4591077838217,30.7143247126095,-38.5366620368727));
#251642=CARTESIAN_POINT('Ctrl Pts',(42.4305062506586,30.7849297888302,-38.5443247619881));
#251643=CARTESIAN_POINT('Ctrl Pts',(42.4171273401332,30.8204683232161,-38.5483659010294));
#251644=CARTESIAN_POINT('Ctrl Pts',(42.3921836892083,30.892009947854,-38.5568599906005));
#251645=CARTESIAN_POINT('Ctrl Pts',(42.380618995835,30.9280130500868,-38.5613129523282));
#251646=CARTESIAN_POINT('Ctrl Pts',(42.3592881338188,31.0004799406419,-38.5706260495541));
#251647=CARTESIAN_POINT('Ctrl Pts',(42.3495219836973,31.036943733628,-38.5754861898888));
#251648=CARTESIAN_POINT('Ctrl Pts',(42.3317857266679,31.110331516506,-38.585611932928));
#251649=CARTESIAN_POINT('Ctrl Pts',(42.3238156113846,31.147255504153,-38.5908775345026));
#251650=CARTESIAN_POINT('Ctrl Pts',(42.3096820195686,31.2215665470911,-38.6018153827909));
#251651=CARTESIAN_POINT('Ctrl Pts',(42.3035171636528,31.258971534054,-38.6074906310522));
#251652=CARTESIAN_POINT('Ctrl Pts',(42.293023529039,31.3341791446678,-38.6192398883933));
#251653=CARTESIAN_POINT('Ctrl Pts',(42.2886817840459,31.3721585400728,-38.6253435908304));
#251654=CARTESIAN_POINT('Ctrl Pts',(42.2819306070517,31.4478003682479,-38.6378361692971));
#251655=CARTESIAN_POINT('Ctrl Pts',(42.2795025001241,31.4855415035392,-38.6442359720864));
#251656=CARTESIAN_POINT('Ctrl Pts',(42.2765060406855,31.560848596424,-38.6573322314144));
#251657=CARTESIAN_POINT('Ctrl Pts',(42.2759365326951,31.5984178369017,-38.664029078225));
#251658=CARTESIAN_POINT('Ctrl Pts',(42.2769710380182,31.7108769251965,-38.6845569897124));
#251659=CARTESIAN_POINT('Ctrl Pts',(42.2813124523233,31.7855186497121,-38.6988245267215));
#251660=CARTESIAN_POINT('Ctrl Pts',(42.2932530869353,31.8969906246886,-38.721084142073));
#251661=CARTESIAN_POINT('Ctrl Pts',(42.2981395716803,31.9340660421392,-38.7286473137566));
#251662=CARTESIAN_POINT('Ctrl Pts',(42.3097367545214,32.0080522410799,-38.744060932418));
#251663=CARTESIAN_POINT('Ctrl Pts',(42.316449417552,32.0449687734335,-38.7519127624581));
#251664=CARTESIAN_POINT('Ctrl Pts',(42.3317154350232,32.1186122283265,-38.7679008712022));
#251665=CARTESIAN_POINT('Ctrl Pts',(42.3402956415526,32.1554227729715,-38.7760569489278));
#251666=CARTESIAN_POINT('Ctrl Pts',(42.3591481488484,32.2281691763966,-38.7925025651723));
#251667=CARTESIAN_POINT('Ctrl Pts',(42.3694448123762,32.2642363057195,-38.8008201099004));
#251668=CARTESIAN_POINT('Ctrl Pts',(42.3917427778168,32.3356900843468,-38.8176250123815));
#251669=CARTESIAN_POINT('Ctrl Pts',(42.4037464930944,32.3710895501939,-38.8261151112762));
#251670=CARTESIAN_POINT('Ctrl Pts',(42.4294540323857,32.4412374478768,-38.8432687473174));
#251671=CARTESIAN_POINT('Ctrl Pts',(42.4431578632506,32.4759858769281,-38.8519322857914));
#251672=CARTESIAN_POINT('Ctrl Pts',(42.4722684831154,32.544830817777,-38.8694322793142));
#251673=CARTESIAN_POINT('Ctrl Pts',(42.4876674595477,32.5789106003817,-38.8782643558018));
#251674=CARTESIAN_POINT('Ctrl Pts',(42.5202146386211,32.6464796024254,-38.8961197400092));
#251675=CARTESIAN_POINT('Ctrl Pts',(42.5373018066979,32.6798350239254,-38.905108271819));
#251676=CARTESIAN_POINT('Ctrl Pts',(42.5906929217761,32.7780784192159,-38.9321048020009));
#251677=CARTESIAN_POINT('Ctrl Pts',(42.6292257708725,32.8414173960492,-38.950210484678));
#251678=CARTESIAN_POINT('Ctrl Pts',(42.7119999890155,32.9638220806952,-38.986612554694));
#251679=CARTESIAN_POINT('Ctrl Pts',(42.7562439154297,33.0229003618273,-39.004911678637));
#251680=CARTESIAN_POINT('Ctrl Pts',(42.826900203736,33.1083283039828,-39.0325062641257));
#251681=CARTESIAN_POINT('Ctrl Pts',(42.851168465327,33.1362718837218,-39.041728825905));
#251682=CARTESIAN_POINT('Ctrl Pts',(42.9011535381211,33.1910822095534,-39.0602231613282));
#251683=CARTESIAN_POINT('Ctrl Pts',(42.926867323379,33.2179450513447,-39.0694937078027));
#251684=CARTESIAN_POINT('Ctrl Pts',(42.9797816918549,33.2705900752688,-39.0880898406065));
#251685=CARTESIAN_POINT('Ctrl Pts',(43.0069971956867,33.2963737293151,-39.0974182289335));
#251686=CARTESIAN_POINT('Ctrl Pts',(43.0622936266078,33.3462615675182,-39.1159153655173));
#251687=CARTESIAN_POINT('Ctrl Pts',(43.0904949817445,33.3704877056864,-39.1251268280428));
#251688=CARTESIAN_POINT('Ctrl Pts',(43.1765625947351,33.4408730461757,-39.1525915160431));
#251689=CARTESIAN_POINT('Ctrl Pts',(43.2360245424999,33.4848790767991,-39.1707229729204));
#251690=CARTESIAN_POINT('Ctrl Pts',(43.3282503204797,33.5464830400295,-39.1976341950415));
#251691=CARTESIAN_POINT('Ctrl Pts',(43.359502217261,33.566285970248,-39.206558164691));
#251692=CARTESIAN_POINT('Ctrl Pts',(43.4230323912785,33.6044189036262,-39.2243131706243));
#251693=CARTESIAN_POINT('Ctrl Pts',(43.4553106240002,33.6227489710991,-39.2331442099428));
#251694=CARTESIAN_POINT('Ctrl Pts',(43.5209070176006,33.65791645796,-39.2507127455309));
#251695=CARTESIAN_POINT('Ctrl Pts',(43.5542222307926,33.6747516859435,-39.2594493413026));
#251696=CARTESIAN_POINT('Ctrl Pts',(43.6219256372691,33.706907422375,-39.276831389152));
#251697=CARTESIAN_POINT('Ctrl Pts',(43.6563381426909,33.722228682357,-39.2854811314501));
#251698=CARTESIAN_POINT('Ctrl Pts',(43.7254519126727,33.7509935119824,-39.3024907091016));
#251699=CARTESIAN_POINT('Ctrl Pts',(43.7602995409721,33.764508496929,-39.3108884655704));
#251700=CARTESIAN_POINT('Ctrl Pts',(43.8304781054344,33.7897808733701,-39.3274499376954));
#251701=CARTESIAN_POINT('Ctrl Pts',(43.8658243260975,33.8015455969846,-39.3356175899088));
#251702=CARTESIAN_POINT('Ctrl Pts',(43.9726293596981,33.8342393544862,-39.3597845122642));
#251703=CARTESIAN_POINT('Ctrl Pts',(44.0448528415367,33.8525737793304,-39.3754484613995));
#251704=CARTESIAN_POINT('Ctrl Pts',(44.1547335175137,33.8748267811095,-39.3982721883298));
#251705=CARTESIAN_POINT('Ctrl Pts',(44.1916183742053,33.881368352274,-39.4057678976717));
#251706=CARTESIAN_POINT('Ctrl Pts',(44.265912298769,33.8926703342681,-39.4205323003128));
#251707=CARTESIAN_POINT('Ctrl Pts',(44.3033049254971,33.8974289036774,-39.4277978422667));
#251708=CARTESIAN_POINT('Ctrl Pts',(44.3598453618029,33.90320513239,-39.4385322069694));
#251709=CARTESIAN_POINT('Ctrl Pts',(44.3787527202319,33.9049006542695,-39.4420799568534));
#251710=CARTESIAN_POINT('Ctrl Pts',(44.4164967923385,33.9078161553301,-39.4490791371853));
#251711=CARTESIAN_POINT('Ctrl Pts',(44.4353708520081,33.9090401337743,-39.4525376906084));
#251712=CARTESIAN_POINT('Ctrl Pts',(44.4919347238328,33.9120095641989,-39.4627791951316));
#251713=CARTESIAN_POINT('Ctrl Pts',(44.5296205555248,33.9130584788855,-39.4694383780658));
#251714=CARTESIAN_POINT('Ctrl Pts',(44.6425299080792,33.9134343306132,-39.4889026064771));
#251715=CARTESIAN_POINT('Ctrl Pts',(44.7176656318032,33.9100024232635,-39.5012068162623));
#251716=CARTESIAN_POINT('Ctrl Pts',(44.8676233385802,33.8957625915874,-39.5244719375305));
#251717=CARTESIAN_POINT('Ctrl Pts',(44.9424659719907,33.8849486120956,-39.5354353244078));
#251718=CARTESIAN_POINT('Ctrl Pts',(45.0357885284359,33.8667000217447,-39.5482785197989));
#251719=CARTESIAN_POINT('Ctrl Pts',(45.0544546477979,33.8628075156194,-39.5508052816758));
#251720=CARTESIAN_POINT('Ctrl Pts',(45.0917431164945,33.8545484532422,-39.5557691225697));
#251721=CARTESIAN_POINT('Ctrl Pts',(45.1104022686543,33.850171692167,-39.5582107456052));
#251722=CARTESIAN_POINT('Ctrl Pts',(45.1661672274775,33.8363538673165,-39.5653801873635));
#251723=CARTESIAN_POINT('Ctrl Pts',(45.2029511272889,33.8262578730812,-39.5699394700858));
#251724=CARTESIAN_POINT('Ctrl Pts',(45.2758616079105,33.8042966073194,-39.5786401460756));
#251725=CARTESIAN_POINT('Ctrl Pts',(45.311968730411,33.7924363563062,-39.5827790715619));
#251726=CARTESIAN_POINT('Ctrl Pts',(45.3834929256923,33.7669724612522,-39.590638826668));
#251727=CARTESIAN_POINT('Ctrl Pts',(45.4189099909314,33.7533687979858,-39.5943596509345));
#251728=CARTESIAN_POINT('Ctrl Pts',(45.4890551389974,33.724420965446,-39.6013847400349));
#251729=CARTESIAN_POINT('Ctrl Pts',(45.523783224749,33.7090768034382,-39.6046890060346));
#251730=CARTESIAN_POINT('Ctrl Pts',(45.5925464395182,33.676638101801,-39.6108793832571));
#251731=CARTESIAN_POINT('Ctrl Pts',(45.6265815821811,33.6595435965646,-39.6137655022888));
#251732=CARTESIAN_POINT('Ctrl Pts',(45.6939497482673,33.6235812098373,-39.6191147790932));
#251733=CARTESIAN_POINT('Ctrl Pts',(45.7272861171773,33.6047101609453,-39.6215779667197));
#251734=CARTESIAN_POINT('Ctrl Pts',(45.7932287598473,33.5651706172408,-39.626073101965));
#251735=CARTESIAN_POINT('Ctrl Pts',(45.8259059486925,33.5444453725487,-39.6281074579657));
#251736=CARTESIAN_POINT('Ctrl Pts',(45.889727526333,33.5016881832693,-39.6316923328834));
#251737=CARTESIAN_POINT('Ctrl Pts',(45.9210297983567,33.4795651702188,-39.6332542280151));
#251738=CARTESIAN_POINT('Ctrl Pts',(45.9823425105019,33.4339089189919,-39.6359179784948));
#251739=CARTESIAN_POINT('Ctrl Pts',(46.0123687882815,33.4103663991699,-39.6370209490844));
#251740=CARTESIAN_POINT('Ctrl Pts',(46.1005740843723,33.3376145658878,-39.6396496275905));
#251741=CARTESIAN_POINT('Ctrl Pts',(46.1568837934186,33.2862857741618,-39.6404966874468));
#251742=CARTESIAN_POINT('Ctrl Pts',(46.2375893334767,33.2050303747233,-39.640403167924));
#251743=CARTESIAN_POINT('Ctrl Pts',(46.2638636629985,33.1772337238693,-39.6401442626271));
#251744=CARTESIAN_POINT('Ctrl Pts',(46.3151397814851,33.1201975129399,-39.639164560865));
#251745=CARTESIAN_POINT('Ctrl Pts',(46.3401349660335,33.0909662011952,-39.6384440443131));
#251746=CARTESIAN_POINT('Ctrl Pts',(46.3888523358489,33.0309971741023,-39.6365300592084));
#251747=CARTESIAN_POINT('Ctrl Pts',(46.4123735658465,33.0005037085489,-39.6353439516494));
#251748=CARTESIAN_POINT('Ctrl Pts',(46.4576879329464,32.9386388874358,-39.6325279868037));
#251749=CARTESIAN_POINT('Ctrl Pts',(46.4794980193706,32.9072464072476,-39.63089741826));
#251750=CARTESIAN_POINT('Ctrl Pts',(46.5424231785881,32.8117200519201,-39.6253488421165));
#251751=CARTESIAN_POINT('Ctrl Pts',(46.5810427212027,32.7462346217556,-39.6207751935492));
#251752=CARTESIAN_POINT('Ctrl Pts',(46.6516918536282,32.6117039663465,-39.6098936512928));
#251753=CARTESIAN_POINT('Ctrl Pts',(46.6837232203822,32.5426422569213,-39.6035832558907));
#251754=CARTESIAN_POINT('Ctrl Pts',(46.719563577096,32.4540883392911,-39.5945935707833));
#251755=CARTESIAN_POINT('Ctrl Pts',(46.7265236134956,32.4362514600518,-39.5927383480922));
#251756=CARTESIAN_POINT('Ctrl Pts',(46.7400123820574,32.4003742276752,-39.588918940518));
#251757=CARTESIAN_POINT('Ctrl Pts',(46.7465535519376,32.3822946227154,-39.5869501776489));
#251758=CARTESIAN_POINT('Ctrl Pts',(46.7654644725393,32.3279073099657,-39.5808958019048));
#251759=CARTESIAN_POINT('Ctrl Pts',(46.7770937705874,32.2915494036189,-39.57667412996));
#251760=CARTESIAN_POINT('Ctrl Pts',(46.7984826494802,32.2185252317751,-39.5678551875289));
#251761=CARTESIAN_POINT('Ctrl Pts',(46.8082357339547,32.1818782773392,-39.5632601045207));
#251762=CARTESIAN_POINT('Ctrl Pts',(46.8258916494835,32.1083194173387,-39.5537041356314));
#251763=CARTESIAN_POINT('Ctrl Pts',(46.8337943715014,32.0714074960361,-39.548743229206));
#251764=CARTESIAN_POINT('Ctrl Pts',(46.854754879426,31.9602784901863,-39.533315750657));
#251765=CARTESIAN_POINT('Ctrl Pts',(46.8650709021906,31.8856621883816,-39.5223044483599));
#251766=CARTESIAN_POINT('Ctrl Pts',(46.87504877973,31.7729724936691,-39.5046948318446));
#251767=CARTESIAN_POINT('Ctrl Pts',(46.8774570742158,31.7352651799165,-39.4986397197368));
#251768=CARTESIAN_POINT('Ctrl Pts',(46.879676832022,31.6785286175404,-39.4892824401848));
#251769=CARTESIAN_POINT('Ctrl Pts',(46.880184378731,31.6595724670412,-39.4861150077938));
#251770=CARTESIAN_POINT('Ctrl Pts',(46.8807312724654,31.6216181021237,-39.4796905877625));
#251771=CARTESIAN_POINT('Ctrl Pts',(46.8807700027013,31.6025797121284,-39.4764265891337));
#251772=CARTESIAN_POINT('Ctrl Pts',(46.8801790769053,31.5455906700815,-39.4665316960354));
#251773=CARTESIAN_POINT('Ctrl Pts',(46.8788491176281,31.5078273440315,-39.4598096137186));
#251774=CARTESIAN_POINT('Ctrl Pts',(46.8743606558037,31.4326451820844,-39.4461013288477));
#251775=CARTESIAN_POINT('Ctrl Pts',(46.8712025098556,31.3952438492793,-39.4391181973417));
#251776=CARTESIAN_POINT('Ctrl Pts',(46.8590349081897,31.2835993602235,-39.4177870145467));
#251777=CARTESIAN_POINT('Ctrl Pts',(46.8473376665826,31.2099145965172,-39.4030579339673));
#251778=CARTESIAN_POINT('Ctrl Pts',(46.8244864324902,31.1004910083645,-39.380205766645));
#251779=CARTESIAN_POINT('Ctrl Pts',(46.8159836152412,31.0642007178987,-39.3724617450316));
#251780=CARTESIAN_POINT('Ctrl Pts',(46.7971994649713,30.9919902975437,-39.356718397465));
#251781=CARTESIAN_POINT('Ctrl Pts',(46.7869180451234,30.9560697415795,-39.3487189839183));
#251782=CARTESIAN_POINT('Ctrl Pts',(46.7645578137196,30.8846047066995,-39.3324614510575));
#251783=CARTESIAN_POINT('Ctrl Pts',(46.7524740702791,30.8490466937981,-39.3242001275257));
#251784=CARTESIAN_POINT('Ctrl Pts',(46.7264944033419,30.7783632674765,-39.3074248017124));
#251785=CARTESIAN_POINT('Ctrl Pts',(46.7127058571131,30.7435263326383,-39.298979502087));
#251786=CARTESIAN_POINT('Ctrl Pts',(46.6981267205988,30.7091523325179,-39.2904704194778));
#251787=CARTESIAN_POINT('Ctrl Pts',(46.3487357027272,30.7584583056228,-39.6906862677766));
#251788=CARTESIAN_POINT('Ctrl Pts',(46.3360465301806,30.7285884779263,-39.6821771851674));
#251789=CARTESIAN_POINT('Ctrl Pts',(46.322674012045,30.6991291081308,-39.6736067193105));
#251790=CARTESIAN_POINT('Ctrl Pts',(46.2945851820176,30.641017718271,-39.6563442956996));
#251791=CARTESIAN_POINT('Ctrl Pts',(46.2798687954904,30.612365742748,-39.6476523324819));
#251792=CARTESIAN_POINT('Ctrl Pts',(46.2337236139186,30.5276092756908,-39.6213949324054));
#251793=CARTESIAN_POINT('Ctrl Pts',(46.2003029919731,30.4727017306776,-39.603648333904));
#251794=CARTESIAN_POINT('Ctrl Pts',(46.1461801500453,30.3927400894707,-39.5766619296672));
#251795=CARTESIAN_POINT('Ctrl Pts',(46.1274728516574,30.3664867733569,-39.5676052936415));
#251796=CARTESIAN_POINT('Ctrl Pts',(46.0887101379817,30.3147906415192,-39.5493678301882));
#251797=CARTESIAN_POINT('Ctrl Pts',(46.0686672178747,30.2893629692206,-39.5401925839578));
#251798=CARTESIAN_POINT('Ctrl Pts',(46.0271585782785,30.2392724858907,-39.5216929509175));
#251799=CARTESIAN_POINT('Ctrl Pts',(46.0058171042466,30.2147653940616,-39.5124250671292));
#251800=CARTESIAN_POINT('Ctrl Pts',(45.9621753273889,30.1670338430194,-39.4939384594262));
#251801=CARTESIAN_POINT('Ctrl Pts',(45.9398360673935,30.1437623234713,-39.4847023642746));
#251802=CARTESIAN_POINT('Ctrl Pts',(45.8713238239452,30.0757484083058,-39.4570317271412));
#251803=CARTESIAN_POINT('Ctrl Pts',(45.8236343202356,30.0327728117785,-39.4386235415696));
#251804=CARTESIAN_POINT('Ctrl Pts',(45.7491141599547,29.9718399517963,-39.4110735194385));
#251805=CARTESIAN_POINT('Ctrl Pts',(45.7237751109832,29.9521177433449,-39.401900347959));
#251806=CARTESIAN_POINT('Ctrl Pts',(45.672092787902,29.9138581053763,-39.3835746671366));
#251807=CARTESIAN_POINT('Ctrl Pts',(45.6457495575596,29.8953206245202,-39.3744221560391));
#251808=CARTESIAN_POINT('Ctrl Pts',(45.5920456528258,29.8594459358056,-39.3561383702047));
#251809=CARTESIAN_POINT('Ctrl Pts',(45.5646920216606,29.842113315145,-39.3470094698523));
#251810=CARTESIAN_POINT('Ctrl Pts',(45.52286176357,29.8170191244728,-39.3333255599053));
#251811=CARTESIAN_POINT('Ctrl Pts',(45.5087802414794,29.8088039098643,-39.3287645751035));
#251812=CARTESIAN_POINT('Ctrl Pts',(45.48050096757,29.7927649995304,-39.3196949594646));
#251813=CARTESIAN_POINT('Ctrl Pts',(45.4662804916472,29.7849263956811,-39.3151786453986));
#251814=CARTESIAN_POINT('Ctrl Pts',(45.3948337755398,29.7466772451965,-39.2927100263081));
#251815=CARTESIAN_POINT('Ctrl Pts',(45.3364866021309,29.7190013424949,-39.2750591047224));
#251816=CARTESIAN_POINT('Ctrl Pts',(45.2174835285277,29.6694316700735,-39.2404129427663));
#251817=CARTESIAN_POINT('Ctrl Pts',(45.156822585129,29.6475313681073,-39.2234153504273));
#251818=CARTESIAN_POINT('Ctrl Pts',(45.0640726127793,29.6190533635405,-39.1984174795332));
#251819=CARTESIAN_POINT('Ctrl Pts',(45.0328624242923,29.6102905224853,-39.1901680730424));
#251820=CARTESIAN_POINT('Ctrl Pts',(44.9698452008949,29.594248293903,-39.1738393994966));
#251821=CARTESIAN_POINT('Ctrl Pts',(44.9380572773652,29.5869727898151,-39.1657648878187));
#251822=CARTESIAN_POINT('Ctrl Pts',(44.8737940791812,29.5739240771953,-39.1497719921229));
#251823=CARTESIAN_POINT('Ctrl Pts',(44.8415218191992,29.5681957143413,-39.1419048591056));
#251824=CARTESIAN_POINT('Ctrl Pts',(44.7769717049288,29.5583595811323,-39.1264935573013));
#251825=CARTESIAN_POINT('Ctrl Pts',(44.7446388004034,29.554240600873,-39.118935681436));
#251826=CARTESIAN_POINT('Ctrl Pts',(44.6475185309788,29.5442672294863,-39.0967152894771));
#251827=CARTESIAN_POINT('Ctrl Pts',(44.5825759760276,29.5407844261647,-39.0824965767772));
#251828=CARTESIAN_POINT('Ctrl Pts',(44.4523141867918,29.5401662627562,-39.0552651528542));
#251829=CARTESIAN_POINT('Ctrl Pts',(44.3869798978321,29.5430346588726,-39.0422500553699));
#251830=CARTESIAN_POINT('Ctrl Pts',(44.3050952054121,29.5506982250521,-39.026767823736));
#251831=CARTESIAN_POINT('Ctrl Pts',(44.2886959663336,29.5524389843404,-39.0237091724622));
#251832=CARTESIAN_POINT('Ctrl Pts',(44.2558935445924,29.5563309554553,-39.0176749337123));
#251833=CARTESIAN_POINT('Ctrl Pts',(44.2394575555595,29.5584878169524,-39.0146936712963));
#251834=CARTESIAN_POINT('Ctrl Pts',(44.1902803482843,29.5655653021513,-39.0059013930531));
#251835=CARTESIAN_POINT('Ctrl Pts',(44.1577491163975,29.5710766352626,-39.000255075765));
#251836=CARTESIAN_POINT('Ctrl Pts',(44.0930902835475,29.5836763028609,-38.9893707222011));
#251837=CARTESIAN_POINT('Ctrl Pts',(44.0609787991037,29.5907621271768,-38.9841355278308));
#251838=CARTESIAN_POINT('Ctrl Pts',(43.9971881339881,29.6064933938242,-38.9740770527754));
#251839=CARTESIAN_POINT('Ctrl Pts',(43.9655089572005,29.6151388498521,-38.9692537749189));
#251840=CARTESIAN_POINT('Ctrl Pts',(43.9025825453534,29.6339885284277,-38.9600200554735));
#251841=CARTESIAN_POINT('Ctrl Pts',(43.8713353076576,29.6441927411959,-38.9556096106348));
#251842=CARTESIAN_POINT('Ctrl Pts',(43.8092755782281,29.6661704841714,-38.9472054394967));
#251843=CARTESIAN_POINT('Ctrl Pts',(43.7784630771063,29.6779439802752,-38.9432117036118));
#251844=CARTESIAN_POINT('Ctrl Pts',(43.717278897594,29.7030826309711,-38.935647905771));
#251845=CARTESIAN_POINT('Ctrl Pts',(43.6869066895965,29.7164489157022,-38.9320779688894));
#251846=CARTESIAN_POINT('Ctrl Pts',(43.626614728406,29.7448033501699,-38.9253714622882));
#251847=CARTESIAN_POINT('Ctrl Pts',(43.5966488676322,29.7598244459156,-38.9222321196694));
#251848=CARTESIAN_POINT('Ctrl Pts',(43.5379107146287,29.7911322192132,-38.9164684922511));
#251849=CARTESIAN_POINT('Ctrl Pts',(43.5089935637976,29.807484575191,-38.9138275829765));
#251850=CARTESIAN_POINT('Ctrl Pts',(43.4521381627742,29.8415255160901,-38.9090313390425));
#251851=CARTESIAN_POINT('Ctrl Pts',(43.4241850948297,29.8592209427306,-38.9068743283701));
#251852=CARTESIAN_POINT('Ctrl Pts',(43.3417392436055,29.9143171533634,-38.901122204059));
#251853=CARTESIAN_POINT('Ctrl Pts',(43.2886565200899,29.9537233898351,-38.8982444209444));
#251854=CARTESIAN_POINT('Ctrl Pts',(43.1862829187094,30.0379276623574,-38.8944209010817));
#251855=CARTESIAN_POINT('Ctrl Pts',(43.1369819758927,30.0827344207114,-38.8934748836529));
#251856=CARTESIAN_POINT('Ctrl Pts',(43.042354298069,30.1779092800836,-38.8935900529829));
#251857=CARTESIAN_POINT('Ctrl Pts',(42.9978703496345,30.2274261173575,-38.8946494544906));
#251858=CARTESIAN_POINT('Ctrl Pts',(42.9142997798964,30.3302219112651,-38.8986950841053));
#251859=CARTESIAN_POINT('Ctrl Pts',(42.8752223854268,30.3834931157852,-38.9016816200845));
#251860=CARTESIAN_POINT('Ctrl Pts',(42.8024383095261,30.4937511191122,-38.9095627198077));
#251861=CARTESIAN_POINT('Ctrl Pts',(42.7687332609551,30.5507427160192,-38.9144586402205));
#251862=CARTESIAN_POINT('Ctrl Pts',(42.7300263292576,30.6243422699748,-38.9217897554615));
#251863=CARTESIAN_POINT('Ctrl Pts',(42.7224576402308,30.6391839142897,-38.9233176240571));
#251864=CARTESIAN_POINT('Ctrl Pts',(42.7076667752466,30.6691034586862,-38.9264952711875));
#251865=CARTESIAN_POINT('Ctrl Pts',(42.7004417482736,30.6841916091719,-38.9281466008814));
#251866=CARTESIAN_POINT('Ctrl Pts',(42.6794127755329,30.7295576912778,-38.9332567299131));
#251867=CARTESIAN_POINT('Ctrl Pts',(42.6662150606011,30.7600066923132,-38.9368778851714));
#251868=CARTESIAN_POINT('Ctrl Pts',(42.6414200236241,30.8213217799634,-38.9445406102868));
#251869=CARTESIAN_POINT('Ctrl Pts',(42.629823463925,30.8521850491422,-38.9485817493281));
#251870=CARTESIAN_POINT('Ctrl Pts',(42.6082065832887,30.9143165573564,-38.9570758388993));
#251871=CARTESIAN_POINT('Ctrl Pts',(42.5981863032189,30.9455848068317,-38.961528800627));
#251872=CARTESIAN_POINT('Ctrl Pts',(42.5797083779644,31.0085229028534,-38.9708418978528));
#251873=CARTESIAN_POINT('Ctrl Pts',(42.571250748879,31.0401927534638,-38.9757020381876));
#251874=CARTESIAN_POINT('Ctrl Pts',(42.5558959598811,31.103933624688,-38.9858277812267));
#251875=CARTESIAN_POINT('Ctrl Pts',(42.5489987926973,31.1360046433454,-38.9910933828013));
#251876=CARTESIAN_POINT('Ctrl Pts',(42.5367741244054,31.2005503513038,-39.0020312310896));
#251877=CARTESIAN_POINT('Ctrl Pts',(42.531445437756,31.2330406174058,-39.0077064793509));
#251878=CARTESIAN_POINT('Ctrl Pts',(42.5223832479161,31.2983679981005,-39.0194557366921));
#251879=CARTESIAN_POINT('Ctrl Pts',(42.5186386063126,31.3313586704159,-39.0255594391291));
#251880=CARTESIAN_POINT('Ctrl Pts',(42.5128275899613,31.3970661365692,-39.0380520175959));
#251881=CARTESIAN_POINT('Ctrl Pts',(42.5107450488446,31.4298512876605,-39.0444518203851));
#251882=CARTESIAN_POINT('Ctrl Pts',(42.5081952999573,31.495270824389,-39.0575480797132));
#251883=CARTESIAN_POINT('Ctrl Pts',(42.507727090815,31.5279080610915,-39.0642449265238));
#251884=CARTESIAN_POINT('Ctrl Pts',(42.5087049855303,31.625605856974,-39.084772838011));
#251885=CARTESIAN_POINT('Ctrl Pts',(42.5125287224658,31.6904529409863,-39.0990403750203));
#251886=CARTESIAN_POINT('Ctrl Pts',(42.5229793717988,31.7873014338719,-39.1212999903717));
#251887=CARTESIAN_POINT('Ctrl Pts',(42.527250083485,31.8195137897082,-39.1288631620553));
#251888=CARTESIAN_POINT('Ctrl Pts',(42.5373759630957,31.8837968383997,-39.1442767807167));
#251889=CARTESIAN_POINT('Ctrl Pts',(42.5432328418803,31.9158725287012,-39.1521286107568));
#251890=CARTESIAN_POINT('Ctrl Pts',(42.5565453513116,31.979860553896,-39.1681167195009));
#251891=CARTESIAN_POINT('Ctrl Pts',(42.5640243655532,32.0118455541873,-39.1762727972266));
#251892=CARTESIAN_POINT('Ctrl Pts',(42.5804515873162,32.0750569293471,-39.192718413471));
#251893=CARTESIAN_POINT('Ctrl Pts',(42.5894210497274,32.1063973617025,-39.2010359581991));
#251894=CARTESIAN_POINT('Ctrl Pts',(42.6088402032077,32.1684883139446,-39.2178408606802));
#251895=CARTESIAN_POINT('Ctrl Pts',(42.619291999646,32.1992499698161,-39.2263309595749));
#251896=CARTESIAN_POINT('Ctrl Pts',(42.6416719105595,32.2602089363087,-39.2434845956161));
#251897=CARTESIAN_POINT('Ctrl Pts',(42.6536000309827,32.2904062445222,-39.2521481340902));
#251898=CARTESIAN_POINT('Ctrl Pts',(42.6789350686126,32.3502357398653,-39.269648127613));
#251899=CARTESIAN_POINT('Ctrl Pts',(42.6923351877516,32.3798533880106,-39.2784802041006));
#251900=CARTESIAN_POINT('Ctrl Pts',(42.7206544615113,32.438576886634,-39.296335588308));
#251901=CARTESIAN_POINT('Ctrl Pts',(42.735520505061,32.4675664571484,-39.305324120118));
#251902=CARTESIAN_POINT('Ctrl Pts',(42.781967232886,32.5529530674262,-39.3323206502992));
#251903=CARTESIAN_POINT('Ctrl Pts',(42.8154829548893,32.6080060018973,-39.3504263329769));
#251904=CARTESIAN_POINT('Ctrl Pts',(42.8874701351811,32.7144034488201,-39.3868284029926));
#251905=CARTESIAN_POINT('Ctrl Pts',(42.9259438236345,32.7657588863051,-39.4051275269359));
#251906=CARTESIAN_POINT('Ctrl Pts',(42.9873790455293,32.8400241153901,-39.4327221124244));
#251907=CARTESIAN_POINT('Ctrl Pts',(43.0084791885273,32.8643171580889,-39.4419446742037));
#251908=CARTESIAN_POINT('Ctrl Pts',(43.0519370354341,32.9119687254291,-39.4604390096269));
#251909=CARTESIAN_POINT('Ctrl Pts',(43.0742921081275,32.9353238560783,-39.4697095561015));
#251910=CARTESIAN_POINT('Ctrl Pts',(43.1202930465425,32.9810962928332,-39.4883056889052));
#251911=CARTESIAN_POINT('Ctrl Pts',(43.1439518743549,33.0035148878545,-39.4976340772323));
#251912=CARTESIAN_POINT('Ctrl Pts',(43.1920201563362,33.0468935936175,-39.516131213816));
#251913=CARTESIAN_POINT('Ctrl Pts',(43.2165343057023,33.067959736328,-39.5253426763416));
#251914=CARTESIAN_POINT('Ctrl Pts',(43.2913465514678,33.1291669950141,-39.5528073643416));
#251915=CARTESIAN_POINT('Ctrl Pts',(43.3430293286761,33.1674385741862,-39.5709388212192));
#251916=CARTESIAN_POINT('Ctrl Pts',(43.4231851451275,33.2210209418068,-39.5978500433402));
#251917=CARTESIAN_POINT('Ctrl Pts',(43.4503462651464,33.2382463679058,-39.6067740129897));
#251918=CARTESIAN_POINT('Ctrl Pts',(43.5055591314263,33.2714182581268,-39.624529018923));
#251919=CARTESIAN_POINT('Ctrl Pts',(43.5336108390501,33.2873647780958,-39.6333600582416));
#251920=CARTESIAN_POINT('Ctrl Pts',(43.5906166462187,33.3179617274633,-39.6509285938296));
#251921=CARTESIAN_POINT('Ctrl Pts',(43.6195681837097,33.332610251026,-39.6596651896014));
#251922=CARTESIAN_POINT('Ctrl Pts',(43.6784023578464,33.3605920508175,-39.6770472374507));
#251923=CARTESIAN_POINT('Ctrl Pts',(43.7083061147169,33.3739259962444,-39.6856969797488));
#251924=CARTESIAN_POINT('Ctrl Pts',(43.7683632564387,33.3989627678266,-39.7027065574003));
#251925=CARTESIAN_POINT('Ctrl Pts',(43.7986438324276,33.4107277366309,-39.7111043138692));
#251926=CARTESIAN_POINT('Ctrl Pts',(43.8596237019195,33.4327310220396,-39.7276657859941));
#251927=CARTESIAN_POINT('Ctrl Pts',(43.890336277669,33.4429757189306,-39.7358334382075));
#251928=CARTESIAN_POINT('Ctrl Pts',(43.9831380894244,33.4714511139933,-39.7600003605629));
#251929=CARTESIAN_POINT('Ctrl Pts',(44.0458899346709,33.4874281577014,-39.7756643096983));
#251930=CARTESIAN_POINT('Ctrl Pts',(44.1413569280506,33.506834807521,-39.7984880366286));
#251931=CARTESIAN_POINT('Ctrl Pts',(44.1734028005723,33.5125427220107,-39.8059837459705));
#251932=CARTESIAN_POINT('Ctrl Pts',(44.2379488111806,33.5224114537718,-39.8207481486115));
#251933=CARTESIAN_POINT('Ctrl Pts',(44.2704346657345,33.5265706602302,-39.8280136905655));
#251934=CARTESIAN_POINT('Ctrl Pts',(44.3195548130225,33.5316268124821,-39.8387480552682));
#251935=CARTESIAN_POINT('Ctrl Pts',(44.3359806486903,33.533112514136,-39.8422958051522));
#251936=CARTESIAN_POINT('Ctrl Pts',(44.3687706554964,33.5356707262599,-39.849294985484));
#251937=CARTESIAN_POINT('Ctrl Pts',(44.385167271505,33.5367467362316,-39.8527535389071));
#251938=CARTESIAN_POINT('Ctrl Pts',(44.4343060324679,33.5393644028343,-39.8629950434304));
#251939=CARTESIAN_POINT('Ctrl Pts',(44.4670442875949,33.5403009170737,-39.8696542263645));
#251940=CARTESIAN_POINT('Ctrl Pts',(44.5651286496071,33.5407030633914,-39.8891184547758));
#251941=CARTESIAN_POINT('Ctrl Pts',(44.6303967828551,33.5377718061163,-39.901422664561));
#251942=CARTESIAN_POINT('Ctrl Pts',(44.7606559689193,33.5255009866035,-39.9246877858293));
#251943=CARTESIAN_POINT('Ctrl Pts',(44.8256649569195,33.5161561775268,-39.9356511727063));
#251944=CARTESIAN_POINT('Ctrl Pts',(44.9067228490285,33.5003647750523,-39.9484943680977));
#251945=CARTESIAN_POINT('Ctrl Pts',(44.9229356753385,33.4969955694502,-39.9510211299745));
#251946=CARTESIAN_POINT('Ctrl Pts',(44.9553230139946,33.4898452910065,-39.9559849708684));
#251947=CARTESIAN_POINT('Ctrl Pts',(44.9715294906083,33.4860553771579,-39.9584265939039));
#251948=CARTESIAN_POINT('Ctrl Pts',(45.0199639019752,33.4740881833957,-39.9655960356623));
#251949=CARTESIAN_POINT('Ctrl Pts',(45.0519117947774,33.4653417096262,-39.9701553183846));
#251950=CARTESIAN_POINT('Ctrl Pts',(45.1152354809225,33.446311250256,-39.9788559943743));
#251951=CARTESIAN_POINT('Ctrl Pts',(45.1465943739562,33.4360316133009,-39.9829949198606));
#251952=CARTESIAN_POINT('Ctrl Pts',(45.2087116410455,33.4139573018935,-39.9908546749667));
#251953=CARTESIAN_POINT('Ctrl Pts',(45.2394700085385,33.4021626107272,-39.9945754992332));
#251954=CARTESIAN_POINT('Ctrl Pts',(45.3003871502801,33.3770607090048,-40.0016005883336));
#251955=CARTESIAN_POINT('Ctrl Pts',(45.3305459270765,33.3637535047555,-40.0049048543333));
#251956=CARTESIAN_POINT('Ctrl Pts',(45.3902604247426,33.3356180078757,-40.0110952315559));
#251957=CARTESIAN_POINT('Ctrl Pts',(45.4198161574923,33.320789745125,-40.0139813505875));
#251958=CARTESIAN_POINT('Ctrl Pts',(45.4783165883616,33.2895921551583,-40.0193306273919));
#251959=CARTESIAN_POINT('Ctrl Pts',(45.5072641907393,33.2732200785006,-40.0217938150184));
#251960=CARTESIAN_POINT('Ctrl Pts',(45.5645240373204,33.2389139421848,-40.0262889502638));
#251961=CARTESIAN_POINT('Ctrl Pts',(45.5928978501659,33.2209306284775,-40.0283233062644));
#251962=CARTESIAN_POINT('Ctrl Pts',(45.6483131056985,33.1838278301212,-40.0319081811822));
#251963=CARTESIAN_POINT('Ctrl Pts',(45.67549164507,33.164629334656,-40.0334700763139));
#251964=CARTESIAN_POINT('Ctrl Pts',(45.7287256115122,33.1250064046253,-40.0361338267936));
#251965=CARTESIAN_POINT('Ctrl Pts',(45.7547947910058,33.1045739171436,-40.0372367973831));
#251966=CARTESIAN_POINT('Ctrl Pts',(45.8313734238719,33.0414298393551,-40.0398654758892));
#251967=CARTESIAN_POINT('Ctrl Pts',(45.8802576479033,32.9968758024409,-40.0407125357455));
#251968=CARTESIAN_POINT('Ctrl Pts',(45.9503157326903,32.9263396943911,-40.0406190162228));
#251969=CARTESIAN_POINT('Ctrl Pts',(45.9731228380904,32.9022091506732,-40.0403601109258));
#251970=CARTESIAN_POINT('Ctrl Pts',(46.0176306397645,32.8526937808809,-40.0393804091637));
#251971=CARTESIAN_POINT('Ctrl Pts',(46.0393256039723,32.827316116021,-40.0386598926118));
#251972=CARTESIAN_POINT('Ctrl Pts',(46.0816086740566,32.7752513538834,-40.0367459075072));
#251973=CARTESIAN_POINT('Ctrl Pts',(46.1020223635294,32.748776311325,-40.0355597999481));
#251974=CARTESIAN_POINT('Ctrl Pts',(46.1413479307733,32.6950625087254,-40.0327438351025));
#251975=CARTESIAN_POINT('Ctrl Pts',(46.1602745191316,32.667805408264,-40.0311132665587));
#251976=CARTESIAN_POINT('Ctrl Pts',(46.2148771442285,32.5848607282983,-40.0255646904152));
#251977=CARTESIAN_POINT('Ctrl Pts',(46.2483843529929,32.5279974828729,-40.020991041848));
#251978=CARTESIAN_POINT('Ctrl Pts',(46.3096714681144,32.4111744995713,-40.0101094995915));
#251979=CARTESIAN_POINT('Ctrl Pts',(46.3374529074462,32.3512004429127,-40.0037991041897));
#251980=CARTESIAN_POINT('Ctrl Pts',(46.3685304794595,32.2742958783444,-39.9948094190819));
#251981=CARTESIAN_POINT('Ctrl Pts',(46.3745651799673,32.258805297798,-39.992954196391));
#251982=CARTESIAN_POINT('Ctrl Pts',(46.3862597495084,32.2276471132964,-39.9891347888168));
#251983=CARTESIAN_POINT('Ctrl Pts',(46.3919303977612,32.2119454190112,-39.9871660259476));
#251984=CARTESIAN_POINT('Ctrl Pts',(46.4083231790586,32.1647108974852,-39.9811116502034));
#251985=CARTESIAN_POINT('Ctrl Pts',(46.4184020073002,32.1331340069007,-39.9768899782587));
#251986=CARTESIAN_POINT('Ctrl Pts',(46.436935125005,32.0697112055328,-39.9680710358276));
#251987=CARTESIAN_POINT('Ctrl Pts',(46.445383783564,32.0378820662313,-39.9634759528194));
#251988=CARTESIAN_POINT('Ctrl Pts',(46.4606734917644,31.9739924890849,-39.9539199839301));
#251989=CARTESIAN_POINT('Ctrl Pts',(46.4675144466818,31.9419320374959,-39.9489590775047));
#251990=CARTESIAN_POINT('Ctrl Pts',(46.4856499729356,31.845407387683,-39.9335315989557));
#251991=CARTESIAN_POINT('Ctrl Pts',(46.4945623229588,31.7805947077293,-39.9225202966587));
#251992=CARTESIAN_POINT('Ctrl Pts',(46.50315541296,31.682707544011,-39.9049106801433));
#251993=CARTESIAN_POINT('Ctrl Pts',(46.5052224358974,31.6499527611637,-39.8988555680355));
#251994=CARTESIAN_POINT('Ctrl Pts',(46.5071129195558,31.6006671922554,-39.8894982884836));
#251995=CARTESIAN_POINT('Ctrl Pts',(46.5075411711697,31.5842003354425,-39.8863308560925));
#251996=CARTESIAN_POINT('Ctrl Pts',(46.5079908839588,31.5512297919602,-39.8799064360613));
#251997=CARTESIAN_POINT('Ctrl Pts',(46.5080117823738,31.5346912044655,-39.8766424374324));
#251998=CARTESIAN_POINT('Ctrl Pts',(46.5074602328187,31.4851845718774,-39.8667475443341));
#251999=CARTESIAN_POINT('Ctrl Pts',(46.5062795002176,31.4523788235367,-39.8600254620174));
#252000=CARTESIAN_POINT('Ctrl Pts',(46.5023296578576,31.3870654499314,-39.8463171771464));
#252001=CARTESIAN_POINT('Ctrl Pts',(46.4995608696366,31.3545730297871,-39.8393340456404));
#252002=CARTESIAN_POINT('Ctrl Pts',(46.4889150985814,31.2575801349411,-39.8180028628456));
#252003=CARTESIAN_POINT('Ctrl Pts',(46.4787033805107,31.1935630593794,-39.8032737822661));
#252004=CARTESIAN_POINT('Ctrl Pts',(46.4587772997576,31.0984927597808,-39.7804216149437));
#252005=CARTESIAN_POINT('Ctrl Pts',(46.4513658768236,31.0669621494902,-39.7726775933303));
#252006=CARTESIAN_POINT('Ctrl Pts',(46.4349981252203,31.0042213580613,-39.7569342457637));
#252007=CARTESIAN_POINT('Ctrl Pts',(46.4260417208278,30.9730108067506,-39.748934832217));
#252008=CARTESIAN_POINT('Ctrl Pts',(46.4065676110902,30.9109152528886,-39.7326772993563));
#252009=CARTESIAN_POINT('Ctrl Pts',(46.3960456119263,30.8800184902932,-39.7244159758245));
#252010=CARTESIAN_POINT('Ctrl Pts',(46.3734275034811,30.8185995963653,-39.7076406500112));
#252011=CARTESIAN_POINT('Ctrl Pts',(46.3614248752738,30.7883281333193,-39.6991953503857));
#252012=CARTESIAN_POINT('Ctrl Pts',(46.3487357027272,30.7584583056228,-39.6906862677766));
#252013=CARTESIAN_POINT('',(42.4577131940165,32.5104083281549,-38.8606823233484));
#252014=CARTESIAN_POINT('',(42.4577131944622,32.5104083279563,-38.8606823233881));
#252015=CARTESIAN_POINT('',(46.6981266849484,30.7091523375492,-39.2904704603132));
#252016=CARTESIAN_POINT('Ctrl Pts',(46.6981266849492,30.7091523375488,-39.2904704603133));
#252017=CARTESIAN_POINT('Ctrl Pts',(46.5797439954818,30.4300352196549,-39.2213766504479));
#252018=CARTESIAN_POINT('Ctrl Pts',(46.4077912398568,30.1779725313306,-39.1472063538299));
#252019=CARTESIAN_POINT('Ctrl Pts',(45.9737831093239,29.752035876432,-38.9956460041782));
#252020=CARTESIAN_POINT('Ctrl Pts',(45.7147235512157,29.5834083339364,-38.9196908388693));
#252021=CARTESIAN_POINT('Ctrl Pts',(45.1527139049587,29.3607146626067,-38.7793910205612));
#252022=CARTESIAN_POINT('Ctrl Pts',(44.8561434351563,29.3053774688171,-38.7159976418443));
#252023=CARTESIAN_POINT('Ctrl Pts',(44.2653011709016,29.3121801855873,-38.6103011000027));
#252024=CARTESIAN_POINT('Ctrl Pts',(43.9766018912819,29.3704766749623,-38.5683428118836));
#252025=CARTESIAN_POINT('Ctrl Pts',(43.4335518958791,29.5939796223262,-38.5100427719152));
#252026=CARTESIAN_POINT('Ctrl Pts',(43.1848178911664,29.7570960269132,-38.4943558284383));
#252027=CARTESIAN_POINT('Ctrl Pts',(42.7660055088704,30.1651877888254,-38.4923938387362));
#252028=CARTESIAN_POINT('Ctrl Pts',(42.5990769824729,30.4036630363023,-38.5055049887944));
#252029=CARTESIAN_POINT('Ctrl Pts',(42.3602851983405,30.9324943875122,-38.5584474017113));
#252030=CARTESIAN_POINT('Ctrl Pts',(42.292408067155,31.2174998265278,-38.5980179340525));
#252031=CARTESIAN_POINT('Ctrl Pts',(42.270619938325,31.6778293530179,-38.6774582907849));
#252032=CARTESIAN_POINT('Ctrl Pts',(42.2818103158114,31.8495778784957,-38.7105098844616));
#252033=CARTESIAN_POINT('Ctrl Pts',(42.3419700050574,32.1874945526906,-38.7821575613242));
#252034=CARTESIAN_POINT('Ctrl Pts',(42.39095049389,32.3525183831361,-38.8205475941614));
#252035=CARTESIAN_POINT('Ctrl Pts',(42.4577131944621,32.5104083279563,-38.8606823233881));
#252036=CARTESIAN_POINT('',(46.6981266849484,30.7091523375492,-39.2904704603132));
#252037=CARTESIAN_POINT('Origin',(44.4157001211388,31.6455025209913,-39.4611695540092));
#252038=CARTESIAN_POINT('Origin',(44.5079524583208,31.5404524382925,-52.920575));
#252039=CARTESIAN_POINT('Ctrl Pts',(44.5079524583208,29.87170715524,-52.4912));
#252040=CARTESIAN_POINT('Ctrl Pts',(45.4714029967,29.87170715524,-52.4328666666667));
#252041=CARTESIAN_POINT('Ctrl Pts',(45.9531282658897,30.7060797967663,-52.3745333333334));
#252042=CARTESIAN_POINT('Ctrl Pts',(46.4348535350793,31.5404524382925,-52.3162000000001));
#252043=CARTESIAN_POINT('Ctrl Pts',(45.9531282658897,32.3748250798187,-52.2578666666667));
#252044=CARTESIAN_POINT('Ctrl Pts',(45.4714029967,33.2091977213449,-52.1995333333334));
#252045=CARTESIAN_POINT('Ctrl Pts',(44.5079524583208,33.2091977213449,-52.1412));
#252046=CARTESIAN_POINT('Ctrl Pts',(43.5445019199415,33.2091977213449,-52.0828666666667));
#252047=CARTESIAN_POINT('Ctrl Pts',(43.0627766507519,32.3748250798187,-52.0245333333333));
#252048=CARTESIAN_POINT('Ctrl Pts',(42.5810513815623,31.5404524382925,-51.9662));
#252049=CARTESIAN_POINT('Ctrl Pts',(43.0627766507519,30.7060797967663,-51.9078666666667));
#252050=CARTESIAN_POINT('Ctrl Pts',(43.5445019199415,29.87170715524,-51.8495333333334));
#252051=CARTESIAN_POINT('Ctrl Pts',(44.5079524583208,29.87170715524,-51.7912));
#252052=CARTESIAN_POINT('Ctrl Pts',(44.5079524583208,29.87170715524,-52.64995));
#252053=CARTESIAN_POINT('Ctrl Pts',(45.4714029967001,29.8717071552401,-52.5916166666667));
#252054=CARTESIAN_POINT('Ctrl Pts',(45.9531282658897,30.7060797967663,-52.5332833333334));
#252055=CARTESIAN_POINT('Ctrl Pts',(46.4348535350793,31.5404524382925,-52.47495));
#252056=CARTESIAN_POINT('Ctrl Pts',(45.9531282658897,32.3748250798187,-52.4166166666667));
#252057=CARTESIAN_POINT('Ctrl Pts',(45.4714029967,33.2091977213449,-52.3582833333334));
#252058=CARTESIAN_POINT('Ctrl Pts',(44.5079524583208,33.2091977213449,-52.29995));
#252059=CARTESIAN_POINT('Ctrl Pts',(43.5445019199415,33.2091977213449,-52.2416166666667));
#252060=CARTESIAN_POINT('Ctrl Pts',(43.0627766507519,32.3748250798187,-52.1832833333333));
#252061=CARTESIAN_POINT('Ctrl Pts',(42.5810513815623,31.5404524382925,-52.12495));
#252062=CARTESIAN_POINT('Ctrl Pts',(43.0627766507519,30.7060797967663,-52.0666166666667));
#252063=CARTESIAN_POINT('Ctrl Pts',(43.5445019199415,29.87170715524,-52.0082833333333));
#252064=CARTESIAN_POINT('Ctrl Pts',(44.5079524583208,29.87170715524,-51.94995));
#252065=CARTESIAN_POINT('Ctrl Pts',(44.5079524583208,33.6091932047179,-52.6102625));
#252066=CARTESIAN_POINT('Ctrl Pts',(43.3135644199415,33.6091932047179,-52.5519291666666));
#252067=CARTESIAN_POINT('Ctrl Pts',(42.7163704007519,32.5748228215052,-52.4935958333333));
#252068=CARTESIAN_POINT('Ctrl Pts',(42.1191763815623,31.5404524382925,-52.4352625));
#252069=CARTESIAN_POINT('Ctrl Pts',(42.7163704007519,30.5060820550798,-52.3769291666667));
#252070=CARTESIAN_POINT('Ctrl Pts',(43.3135644199415,29.4717116718671,-52.3185958333334));
#252071=CARTESIAN_POINT('Ctrl Pts',(44.5079524583208,29.4717116718671,-52.2602625));
#252072=CARTESIAN_POINT('Ctrl Pts',(45.7023404967,29.4717116718671,-52.2019291666667));
#252073=CARTESIAN_POINT('Ctrl Pts',(46.2995345158897,30.5060820550798,-52.1435958333333));
#252074=CARTESIAN_POINT('Ctrl Pts',(46.8967285350793,31.5404524382925,-52.0852625));
#252075=CARTESIAN_POINT('Ctrl Pts',(46.2995345158897,32.5748228215052,-52.0269291666667));
#252076=CARTESIAN_POINT('Ctrl Pts',(45.7023404967,33.6091932047179,-51.9685958333333));
#252077=CARTESIAN_POINT('Ctrl Pts',(44.5079524583208,33.6091932047179,-51.9102625));
#252078=CARTESIAN_POINT('Ctrl Pts',(43.3135644199415,33.6091932047179,-51.8519291666667));
#252079=CARTESIAN_POINT('Ctrl Pts',(42.7163704007519,32.5748228215052,-51.7935958333333));
#252080=CARTESIAN_POINT('Ctrl Pts',(42.1191763815623,31.5404524382925,-51.7352625));
#252081=CARTESIAN_POINT('Ctrl Pts',(42.7163704007519,30.5060820550798,-51.6769291666667));
#252082=CARTESIAN_POINT('Ctrl Pts',(43.3135644199415,29.4717116718671,-51.6185958333333));
#252083=CARTESIAN_POINT('Ctrl Pts',(44.5079524583208,29.4717116718671,-51.5602625));
#252084=CARTESIAN_POINT('Ctrl Pts',(45.7023404967,29.4717116718671,-51.5019291666666));
#252085=CARTESIAN_POINT('Ctrl Pts',(46.2995345158897,30.5060820550798,-51.4435958333333));
#252086=CARTESIAN_POINT('Ctrl Pts',(46.8967285350793,31.5404524382925,-51.3852625));
#252087=CARTESIAN_POINT('Ctrl Pts',(46.2995345158897,32.5748228215052,-51.3269291666667));
#252088=CARTESIAN_POINT('Ctrl Pts',(45.7023404967,33.6091932047179,-51.2685958333333));
#252089=CARTESIAN_POINT('Ctrl Pts',(44.5079524583208,33.6091932047179,-51.2102625));
#252090=CARTESIAN_POINT('Ctrl Pts',(43.3135644199415,33.6091932047179,-51.1519291666666));
#252091=CARTESIAN_POINT('Ctrl Pts',(42.7163704007519,32.5748228215052,-51.0935958333334));
#252092=CARTESIAN_POINT('Ctrl Pts',(42.1191763815623,31.5404524382925,-51.0352625));
#252093=CARTESIAN_POINT('Ctrl Pts',(42.7163704007519,30.5060820550798,-50.9769291666667));
#252094=CARTESIAN_POINT('Ctrl Pts',(43.3135644199415,29.4717116718671,-50.9185958333333));
#252095=CARTESIAN_POINT('Ctrl Pts',(44.5079524583208,29.4717116718671,-50.8602625));
#252096=CARTESIAN_POINT('Ctrl Pts',(45.7023404967,29.4717116718671,-50.8019291666667));
#252097=CARTESIAN_POINT('Ctrl Pts',(46.2995345158897,30.5060820550798,-50.7435958333333));
#252098=CARTESIAN_POINT('Ctrl Pts',(46.8967285350793,31.5404524382925,-50.6852625));
#252099=CARTESIAN_POINT('Ctrl Pts',(46.2995345158897,32.5748228215052,-50.6269291666667));
#252100=CARTESIAN_POINT('Ctrl Pts',(45.7023404967,33.6091932047179,-50.5685958333333));
#252101=CARTESIAN_POINT('Ctrl Pts',(44.5079524583208,33.6091932047179,-50.5102625));
#252102=CARTESIAN_POINT('Ctrl Pts',(43.3135644199415,33.6091932047179,-50.4519291666667));
#252103=CARTESIAN_POINT('Ctrl Pts',(42.7163704007519,32.5748228215052,-50.3935958333333));
#252104=CARTESIAN_POINT('Ctrl Pts',(42.1191763815623,31.5404524382925,-50.3352625));
#252105=CARTESIAN_POINT('Ctrl Pts',(42.7163704007519,30.5060820550798,-50.2769291666667));
#252106=CARTESIAN_POINT('Ctrl Pts',(43.3135644199415,29.4717116718671,-50.2185958333333));
#252107=CARTESIAN_POINT('Ctrl Pts',(44.5079524583208,29.4717116718671,-50.1602625));
#252108=CARTESIAN_POINT('Ctrl Pts',(45.7023404967,29.4717116718671,-50.1019291666667));
#252109=CARTESIAN_POINT('Ctrl Pts',(46.2995345158897,30.5060820550798,-50.0435958333333));
#252110=CARTESIAN_POINT('Ctrl Pts',(46.8967285350793,31.5404524382925,-49.9852625));
#252111=CARTESIAN_POINT('Ctrl Pts',(46.2995345158897,32.5748228215052,-49.9269291666667));
#252112=CARTESIAN_POINT('Ctrl Pts',(45.7023404967,33.6091932047179,-49.8685958333333));
#252113=CARTESIAN_POINT('Ctrl Pts',(44.5079524583208,33.6091932047179,-49.8102625));
#252114=CARTESIAN_POINT('Ctrl Pts',(43.3135644199415,33.6091932047179,-49.7519291666667));
#252115=CARTESIAN_POINT('Ctrl Pts',(42.7163704007519,32.5748228215052,-49.6935958333334));
#252116=CARTESIAN_POINT('Ctrl Pts',(42.1191763815623,31.5404524382925,-49.6352625));
#252117=CARTESIAN_POINT('Ctrl Pts',(42.7163704007519,30.5060820550798,-49.5769291666667));
#252118=CARTESIAN_POINT('Ctrl Pts',(43.3135644199415,29.4717116718671,-49.5185958333334));
#252119=CARTESIAN_POINT('Ctrl Pts',(44.5079524583208,29.4717116718671,-49.4602625));
#252120=CARTESIAN_POINT('Ctrl Pts',(45.7023404967,29.4717116718671,-49.4019291666667));
#252121=CARTESIAN_POINT('Ctrl Pts',(46.2995345158897,30.5060820550798,-49.3435958333333));
#252122=CARTESIAN_POINT('Ctrl Pts',(46.8967285350793,31.5404524382925,-49.2852625));
#252123=CARTESIAN_POINT('Ctrl Pts',(46.2995345158897,32.5748228215052,-49.2269291666667));
#252124=CARTESIAN_POINT('Ctrl Pts',(45.7023404967,33.6091932047179,-49.1685958333334));
#252125=CARTESIAN_POINT('Ctrl Pts',(44.5079524583208,33.6091932047179,-49.1102625));
#252126=CARTESIAN_POINT('Ctrl Pts',(43.3135644199415,33.6091932047179,-49.0519291666667));
#252127=CARTESIAN_POINT('Ctrl Pts',(42.7163704007519,32.5748228215052,-48.9935958333333));
#252128=CARTESIAN_POINT('Ctrl Pts',(42.1191763815623,31.5404524382925,-48.9352625));
#252129=CARTESIAN_POINT('Ctrl Pts',(42.7163704007519,30.5060820550798,-48.8769291666667));
#252130=CARTESIAN_POINT('Ctrl Pts',(43.3135644199415,29.4717116718671,-48.8185958333333));
#252131=CARTESIAN_POINT('Ctrl Pts',(44.5079524583208,29.4717116718671,-48.7602625));
#252132=CARTESIAN_POINT('Ctrl Pts',(45.7023404967,29.4717116718671,-48.7019291666667));
#252133=CARTESIAN_POINT('Ctrl Pts',(46.2995345158897,30.5060820550798,-48.6435958333333));
#252134=CARTESIAN_POINT('Ctrl Pts',(46.8967285350793,31.5404524382925,-48.5852625));
#252135=CARTESIAN_POINT('Ctrl Pts',(46.2995345158897,32.5748228215052,-48.5269291666667));
#252136=CARTESIAN_POINT('Ctrl Pts',(45.7023404967,33.6091932047179,-48.4685958333333));
#252137=CARTESIAN_POINT('Ctrl Pts',(44.5079524583208,33.6091932047179,-48.4102625));
#252138=CARTESIAN_POINT('Ctrl Pts',(43.3135644199415,33.6091932047179,-48.3519291666667));
#252139=CARTESIAN_POINT('Ctrl Pts',(42.7163704007519,32.5748228215052,-48.2935958333333));
#252140=CARTESIAN_POINT('Ctrl Pts',(42.1191763815623,31.5404524382925,-48.2352625));
#252141=CARTESIAN_POINT('Ctrl Pts',(42.7163704007519,30.5060820550798,-48.1769291666667));
#252142=CARTESIAN_POINT('Ctrl Pts',(43.3135644199415,29.4717116718671,-48.1185958333334));
#252143=CARTESIAN_POINT('Ctrl Pts',(44.5079524583208,29.4717116718671,-48.0602625));
#252144=CARTESIAN_POINT('Ctrl Pts',(45.7023404967,29.4717116718671,-48.0019291666667));
#252145=CARTESIAN_POINT('Ctrl Pts',(46.2995345158897,30.5060820550798,-47.9435958333334));
#252146=CARTESIAN_POINT('Ctrl Pts',(46.8967285350793,31.5404524382925,-47.8852625));
#252147=CARTESIAN_POINT('Ctrl Pts',(46.2995345158897,32.5748228215052,-47.8269291666667));
#252148=CARTESIAN_POINT('Ctrl Pts',(45.7023404967,33.6091932047179,-47.7685958333333));
#252149=CARTESIAN_POINT('Ctrl Pts',(44.5079524583208,33.6091932047179,-47.7102625));
#252150=CARTESIAN_POINT('Ctrl Pts',(43.3135644199415,33.6091932047179,-47.6519291666667));
#252151=CARTESIAN_POINT('Ctrl Pts',(42.7163704007519,32.5748228215052,-47.5935958333333));
#252152=CARTESIAN_POINT('Ctrl Pts',(42.1191763815623,31.5404524382925,-47.5352625));
#252153=CARTESIAN_POINT('Ctrl Pts',(42.7163704007519,30.5060820550798,-47.4769291666667));
#252154=CARTESIAN_POINT('Ctrl Pts',(43.3135644199415,29.4717116718671,-47.4185958333333));
#252155=CARTESIAN_POINT('Ctrl Pts',(44.5079524583208,29.4717116718671,-47.3602625));
#252156=CARTESIAN_POINT('Ctrl Pts',(45.7023404967,29.4717116718671,-47.3019291666666));
#252157=CARTESIAN_POINT('Ctrl Pts',(46.2995345158897,30.5060820550798,-47.2435958333333));
#252158=CARTESIAN_POINT('Ctrl Pts',(46.8967285350793,31.5404524382925,-47.1852625));
#252159=CARTESIAN_POINT('Ctrl Pts',(46.2995345158897,32.5748228215052,-47.1269291666667));
#252160=CARTESIAN_POINT('Ctrl Pts',(45.7023404967,33.6091932047179,-47.0685958333333));
#252161=CARTESIAN_POINT('Ctrl Pts',(44.5079524583208,33.6091932047179,-47.0102625));
#252162=CARTESIAN_POINT('Ctrl Pts',(43.3135644199415,33.6091932047179,-46.9519291666667));
#252163=CARTESIAN_POINT('Ctrl Pts',(42.7163704007519,32.5748228215052,-46.8935958333333));
#252164=CARTESIAN_POINT('Ctrl Pts',(42.1191763815623,31.5404524382925,-46.8352625));
#252165=CARTESIAN_POINT('Ctrl Pts',(42.7163704007519,30.5060820550798,-46.7769291666667));
#252166=CARTESIAN_POINT('Ctrl Pts',(43.3135644199415,29.4717116718671,-46.7185958333333));
#252167=CARTESIAN_POINT('Ctrl Pts',(44.5079524583208,29.4717116718671,-46.6602625));
#252168=CARTESIAN_POINT('Ctrl Pts',(45.7023404967,29.4717116718671,-46.6019291666667));
#252169=CARTESIAN_POINT('Ctrl Pts',(46.2995345158897,30.5060820550798,-46.5435958333334));
#252170=CARTESIAN_POINT('Ctrl Pts',(46.8967285350793,31.5404524382925,-46.4852625));
#252171=CARTESIAN_POINT('Ctrl Pts',(46.2995345158897,32.5748228215052,-46.4269291666667));
#252172=CARTESIAN_POINT('Ctrl Pts',(45.7023404967,33.6091932047179,-46.3685958333333));
#252173=CARTESIAN_POINT('Ctrl Pts',(44.5079524583208,33.6091932047179,-46.3102625));
#252174=CARTESIAN_POINT('Ctrl Pts',(43.3135644199415,33.6091932047179,-46.2519291666667));
#252175=CARTESIAN_POINT('Ctrl Pts',(42.7163704007519,32.5748228215052,-46.1935958333333));
#252176=CARTESIAN_POINT('Ctrl Pts',(42.1191763815623,31.5404524382925,-46.1352625));
#252177=CARTESIAN_POINT('Ctrl Pts',(42.7163704007519,30.5060820550798,-46.0769291666667));
#252178=CARTESIAN_POINT('Ctrl Pts',(43.3135644199415,29.4717116718671,-46.0185958333334));
#252179=CARTESIAN_POINT('Ctrl Pts',(44.5079524583208,29.4717116718671,-45.9602625));
#252180=CARTESIAN_POINT('Ctrl Pts',(45.7023404967,29.4717116718671,-45.9019291666667));
#252181=CARTESIAN_POINT('Ctrl Pts',(46.2995345158897,30.5060820550798,-45.8435958333333));
#252182=CARTESIAN_POINT('Ctrl Pts',(46.8967285350793,31.5404524382925,-45.7852625));
#252183=CARTESIAN_POINT('Ctrl Pts',(46.2995345158897,32.5748228215052,-45.7269291666667));
#252184=CARTESIAN_POINT('Ctrl Pts',(45.7023404967,33.6091932047179,-45.6685958333334));
#252185=CARTESIAN_POINT('Ctrl Pts',(44.5079524583208,33.6091932047179,-45.6102625));
#252186=CARTESIAN_POINT('Ctrl Pts',(43.3135644199415,33.6091932047179,-45.5519291666667));
#252187=CARTESIAN_POINT('Ctrl Pts',(42.7163704007519,32.5748228215052,-45.4935958333333));
#252188=CARTESIAN_POINT('Ctrl Pts',(42.1191763815623,31.5404524382925,-45.4352625));
#252189=CARTESIAN_POINT('Ctrl Pts',(42.7163704007519,30.5060820550798,-45.3769291666667));
#252190=CARTESIAN_POINT('Ctrl Pts',(43.3135644199415,29.4717116718671,-45.3185958333333));
#252191=CARTESIAN_POINT('Ctrl Pts',(44.5079524583208,29.4717116718671,-45.2602625));
#252192=CARTESIAN_POINT('Ctrl Pts',(45.7023404967,29.4717116718671,-45.2019291666667));
#252193=CARTESIAN_POINT('Ctrl Pts',(46.2995345158897,30.5060820550798,-45.1435958333333));
#252194=CARTESIAN_POINT('Ctrl Pts',(46.8967285350793,31.5404524382925,-45.0852625));
#252195=CARTESIAN_POINT('Ctrl Pts',(46.2995345158897,32.5748228215052,-45.0269291666667));
#252196=CARTESIAN_POINT('Ctrl Pts',(45.7023404967,33.6091932047179,-44.9685958333334));
#252197=CARTESIAN_POINT('Ctrl Pts',(44.5079524583208,33.6091932047179,-44.9102625));
#252198=CARTESIAN_POINT('Ctrl Pts',(43.3135644199415,33.6091932047179,-44.8519291666667));
#252199=CARTESIAN_POINT('Ctrl Pts',(42.7163704007519,32.5748228215052,-44.7935958333333));
#252200=CARTESIAN_POINT('Ctrl Pts',(42.1191763815623,31.5404524382925,-44.7352625));
#252201=CARTESIAN_POINT('Ctrl Pts',(42.7163704007519,30.5060820550798,-44.6769291666667));
#252202=CARTESIAN_POINT('Ctrl Pts',(43.3135644199415,29.4717116718671,-44.6185958333334));
#252203=CARTESIAN_POINT('Ctrl Pts',(44.5079524583208,29.4717116718671,-44.5602625));
#252204=CARTESIAN_POINT('Ctrl Pts',(45.7023404967,29.4717116718671,-44.5019291666667));
#252205=CARTESIAN_POINT('Ctrl Pts',(46.2995345158897,30.5060820550798,-44.4435958333333));
#252206=CARTESIAN_POINT('Ctrl Pts',(46.8967285350793,31.5404524382925,-44.3852625));
#252207=CARTESIAN_POINT('Ctrl Pts',(46.2995345158897,32.5748228215052,-44.3269291666667));
#252208=CARTESIAN_POINT('Ctrl Pts',(45.7023404967,33.6091932047179,-44.2685958333334));
#252209=CARTESIAN_POINT('Ctrl Pts',(44.5079524583208,33.6091932047179,-44.2102625));
#252210=CARTESIAN_POINT('Ctrl Pts',(43.3135644199415,33.6091932047179,-44.1519291666667));
#252211=CARTESIAN_POINT('Ctrl Pts',(42.7163704007519,32.5748228215052,-44.0935958333334));
#252212=CARTESIAN_POINT('Ctrl Pts',(42.1191763815623,31.5404524382925,-44.0352625));
#252213=CARTESIAN_POINT('Ctrl Pts',(42.7163704007519,30.5060820550798,-43.9769291666667));
#252214=CARTESIAN_POINT('Ctrl Pts',(43.3135644199415,29.4717116718671,-43.9185958333333));
#252215=CARTESIAN_POINT('Ctrl Pts',(44.5079524583208,29.4717116718671,-43.8602625));
#252216=CARTESIAN_POINT('Ctrl Pts',(45.7023404967,29.4717116718671,-43.8019291666667));
#252217=CARTESIAN_POINT('Ctrl Pts',(46.2995345158897,30.5060820550798,-43.7435958333334));
#252218=CARTESIAN_POINT('Ctrl Pts',(46.8967285350793,31.5404524382925,-43.6852625));
#252219=CARTESIAN_POINT('Ctrl Pts',(46.2995345158897,32.5748228215052,-43.6269291666667));
#252220=CARTESIAN_POINT('Ctrl Pts',(45.7023404967,33.6091932047179,-43.5685958333333));
#252221=CARTESIAN_POINT('Ctrl Pts',(44.5079524583208,33.6091932047179,-43.5102625));
#252222=CARTESIAN_POINT('Ctrl Pts',(43.3135644199415,33.6091932047179,-43.4519291666667));
#252223=CARTESIAN_POINT('Ctrl Pts',(42.7163704007519,32.5748228215052,-43.3935958333334));
#252224=CARTESIAN_POINT('Ctrl Pts',(42.1191763815623,31.5404524382925,-43.3352625));
#252225=CARTESIAN_POINT('Ctrl Pts',(42.7163704007519,30.5060820550798,-43.2769291666667));
#252226=CARTESIAN_POINT('Ctrl Pts',(43.3135644199415,29.4717116718671,-43.2185958333333));
#252227=CARTESIAN_POINT('Ctrl Pts',(44.5079524583208,29.4717116718671,-43.1602625));
#252228=CARTESIAN_POINT('Ctrl Pts',(45.7023404967,29.4717116718671,-43.1019291666667));
#252229=CARTESIAN_POINT('Ctrl Pts',(46.2995345158897,30.5060820550798,-43.0435958333334));
#252230=CARTESIAN_POINT('Ctrl Pts',(46.8967285350793,31.5404524382925,-42.9852625));
#252231=CARTESIAN_POINT('Ctrl Pts',(46.2995345158897,32.5748228215052,-42.9269291666667));
#252232=CARTESIAN_POINT('Ctrl Pts',(45.7023404967,33.6091932047179,-42.8685958333333));
#252233=CARTESIAN_POINT('Ctrl Pts',(44.5079524583208,33.6091932047179,-42.8102625));
#252234=CARTESIAN_POINT('Ctrl Pts',(43.3135644199415,33.6091932047179,-42.7519291666666));
#252235=CARTESIAN_POINT('Ctrl Pts',(42.7163704007519,32.5748228215052,-42.6935958333333));
#252236=CARTESIAN_POINT('Ctrl Pts',(42.1191763815623,31.5404524382925,-42.6352625));
#252237=CARTESIAN_POINT('Ctrl Pts',(42.7163704007519,30.5060820550798,-42.5769291666667));
#252238=CARTESIAN_POINT('Ctrl Pts',(43.3135644199415,29.4717116718671,-42.5185958333333));
#252239=CARTESIAN_POINT('Ctrl Pts',(44.5079524583208,29.4717116718671,-42.4602625));
#252240=CARTESIAN_POINT('Ctrl Pts',(45.7023404967,29.4717116718671,-42.4019291666666));
#252241=CARTESIAN_POINT('Ctrl Pts',(46.2995345158897,30.5060820550798,-42.3435958333334));
#252242=CARTESIAN_POINT('Ctrl Pts',(46.8967285350793,31.5404524382925,-42.2852625));
#252243=CARTESIAN_POINT('Ctrl Pts',(46.2995345158897,32.5748228215052,-42.2269291666667));
#252244=CARTESIAN_POINT('Ctrl Pts',(45.7023404967,33.6091932047179,-42.1685958333333));
#252245=CARTESIAN_POINT('Ctrl Pts',(44.5079524583208,33.6091932047179,-42.1102625));
#252246=CARTESIAN_POINT('Ctrl Pts',(43.3135644199415,33.6091932047179,-42.0519291666666));
#252247=CARTESIAN_POINT('Ctrl Pts',(42.7163704007519,32.5748228215052,-41.9935958333334));
#252248=CARTESIAN_POINT('Ctrl Pts',(42.1191763815623,31.5404524382925,-41.9352625));
#252249=CARTESIAN_POINT('Ctrl Pts',(42.7163704007519,30.5060820550798,-41.8769291666667));
#252250=CARTESIAN_POINT('Ctrl Pts',(43.3135644199415,29.4717116718671,-41.8185958333333));
#252251=CARTESIAN_POINT('Ctrl Pts',(44.5079524583208,29.4717116718671,-41.7602625));
#252252=CARTESIAN_POINT('Ctrl Pts',(45.7023404967,29.4717116718671,-41.7019291666666));
#252253=CARTESIAN_POINT('Ctrl Pts',(46.2995345158897,30.5060820550798,-41.6435958333334));
#252254=CARTESIAN_POINT('Ctrl Pts',(46.8967285350793,31.5404524382925,-41.5852625));
#252255=CARTESIAN_POINT('Ctrl Pts',(46.2995345158897,32.5748228215052,-41.5269291666667));
#252256=CARTESIAN_POINT('Ctrl Pts',(45.7023404967,33.6091932047179,-41.4685958333333));
#252257=CARTESIAN_POINT('Ctrl Pts',(44.5079524583208,33.6091932047179,-41.4102625));
#252258=CARTESIAN_POINT('Ctrl Pts',(43.3135644199415,33.6091932047179,-41.3519291666666));
#252259=CARTESIAN_POINT('Ctrl Pts',(42.7163704007519,32.5748228215052,-41.2935958333334));
#252260=CARTESIAN_POINT('Ctrl Pts',(42.1191763815623,31.5404524382925,-41.2352625));
#252261=CARTESIAN_POINT('Ctrl Pts',(42.7163704007519,30.5060820550798,-41.1769291666667));
#252262=CARTESIAN_POINT('Ctrl Pts',(43.3135644199415,29.4717116718671,-41.1185958333333));
#252263=CARTESIAN_POINT('Ctrl Pts',(44.5079524583208,29.4717116718671,-41.0602625));
#252264=CARTESIAN_POINT('Ctrl Pts',(45.7023404967,29.4717116718671,-41.0019291666666));
#252265=CARTESIAN_POINT('Ctrl Pts',(46.2995345158897,30.5060820550798,-40.9435958333334));
#252266=CARTESIAN_POINT('Ctrl Pts',(46.8967285350793,31.5404524382925,-40.8852625));
#252267=CARTESIAN_POINT('Ctrl Pts',(46.2995345158897,32.5748228215052,-40.8269291666667));
#252268=CARTESIAN_POINT('Ctrl Pts',(45.7023404967,33.6091932047179,-40.7685958333333));
#252269=CARTESIAN_POINT('Ctrl Pts',(44.5079524583208,33.6091932047179,-40.7102625));
#252270=CARTESIAN_POINT('Ctrl Pts',(43.3135644199415,33.6091932047179,-40.6519291666667));
#252271=CARTESIAN_POINT('Ctrl Pts',(42.7163704007519,32.5748228215052,-40.5935958333334));
#252272=CARTESIAN_POINT('Ctrl Pts',(42.1191763815623,31.5404524382925,-40.5352625));
#252273=CARTESIAN_POINT('Ctrl Pts',(42.7163704007519,30.5060820550798,-40.4769291666667));
#252274=CARTESIAN_POINT('Ctrl Pts',(43.3135644199415,29.4717116718671,-40.4185958333333));
#252275=CARTESIAN_POINT('Ctrl Pts',(44.5079524583208,29.4717116718671,-40.3602625));
#252276=CARTESIAN_POINT('Ctrl Pts',(45.7023404967,29.4717116718671,-40.3019291666667));
#252277=CARTESIAN_POINT('Ctrl Pts',(46.2995345158897,30.5060820550798,-40.2435958333334));
#252278=CARTESIAN_POINT('Ctrl Pts',(46.8967285350793,31.5404524382925,-40.1852625));
#252279=CARTESIAN_POINT('Ctrl Pts',(46.2995345158897,32.5748228215052,-40.1269291666666));
#252280=CARTESIAN_POINT('Ctrl Pts',(45.7023404967,33.6091932047179,-40.0685958333333));
#252281=CARTESIAN_POINT('Ctrl Pts',(44.5079524583208,33.6091932047179,-40.0102625));
#252282=CARTESIAN_POINT('Ctrl Pts',(43.3135644199415,33.6091932047179,-39.9519291666667));
#252283=CARTESIAN_POINT('Ctrl Pts',(42.7163704007519,32.5748228215052,-39.8935958333334));
#252284=CARTESIAN_POINT('Ctrl Pts',(42.1191763815623,31.5404524382925,-39.8352625));
#252285=CARTESIAN_POINT('Ctrl Pts',(42.7163704007519,30.5060820550798,-39.7769291666666));
#252286=CARTESIAN_POINT('Ctrl Pts',(43.3135644199415,29.4717116718671,-39.7185958333334));
#252287=CARTESIAN_POINT('Ctrl Pts',(44.5079524583208,29.4717116718671,-39.6602625));
#252288=CARTESIAN_POINT('Ctrl Pts',(45.7023404967,29.4717116718671,-39.6019291666667));
#252289=CARTESIAN_POINT('Ctrl Pts',(46.2995345158897,30.5060820550798,-39.5435958333333));
#252290=CARTESIAN_POINT('Ctrl Pts',(46.8967285350793,31.5404524382925,-39.4852625));
#252291=CARTESIAN_POINT('Ctrl Pts',(46.2995345158897,32.5748228215052,-39.4269291666667));
#252292=CARTESIAN_POINT('Ctrl Pts',(45.7023404967,33.6091932047179,-39.3685958333334));
#252293=CARTESIAN_POINT('Ctrl Pts',(44.5079524583208,33.6091932047179,-39.3102625));
#252294=CARTESIAN_POINT('Ctrl Pts',(43.3135644199415,33.6091932047179,-39.2519291666667));
#252295=CARTESIAN_POINT('Ctrl Pts',(42.7163704007519,32.5748228215052,-39.1935958333334));
#252296=CARTESIAN_POINT('Ctrl Pts',(42.1191763815623,31.5404524382925,-39.1352625));
#252297=CARTESIAN_POINT('Ctrl Pts',(42.7163704007519,30.5060820550798,-39.0769291666667));
#252298=CARTESIAN_POINT('Ctrl Pts',(43.3135644199415,29.4717116718671,-39.0185958333333));
#252299=CARTESIAN_POINT('Ctrl Pts',(44.5079524583208,29.4717116718671,-38.9602625));
#252300=CARTESIAN_POINT('Ctrl Pts',(45.7023404967,29.4717116718671,-38.9019291666667));
#252301=CARTESIAN_POINT('Ctrl Pts',(46.2995345158897,30.5060820550798,-38.8435958333333));
#252302=CARTESIAN_POINT('Ctrl Pts',(46.8967285350793,31.5404524382925,-38.7852625));
#252303=CARTESIAN_POINT('Ctrl Pts',(46.2995345158897,32.5748228215052,-38.7269291666667));
#252304=CARTESIAN_POINT('Ctrl Pts',(45.7023404967,33.6091932047179,-38.6685958333334));
#252305=CARTESIAN_POINT('Ctrl Pts',(44.5079524583208,33.6091932047179,-38.6102625));
#252306=CARTESIAN_POINT('Ctrl Pts',(43.3135644199415,33.6091932047179,-38.5519291666667));
#252307=CARTESIAN_POINT('Ctrl Pts',(42.7163704007519,32.5748228215052,-38.4935958333334));
#252308=CARTESIAN_POINT('Ctrl Pts',(42.1191763815623,31.5404524382925,-38.4352625));
#252309=CARTESIAN_POINT('Ctrl Pts',(42.7163704007519,30.5060820550798,-38.3769291666666));
#252310=CARTESIAN_POINT('Ctrl Pts',(43.3135644199415,29.4717116718671,-38.3185958333333));
#252311=CARTESIAN_POINT('Ctrl Pts',(44.5079524583208,29.4717116718671,-38.2602625));
#252312=CARTESIAN_POINT('Ctrl Pts',(45.7023404967,29.4717116718671,-38.2019291666667));
#252313=CARTESIAN_POINT('Ctrl Pts',(46.2995345158897,30.5060820550798,-38.1435958333334));
#252314=CARTESIAN_POINT('Ctrl Pts',(46.8967285350793,31.5404524382925,-38.0852625));
#252315=CARTESIAN_POINT('Ctrl Pts',(46.2995345158897,32.5748228215052,-38.0269291666667));
#252316=CARTESIAN_POINT('Ctrl Pts',(45.7023404967,33.6091932047179,-37.9685958333333));
#252317=CARTESIAN_POINT('Ctrl Pts',(44.5079524583208,33.6091932047179,-37.9102625));
#252318=CARTESIAN_POINT('Ctrl Pts',(43.3135644199415,33.6091932047179,-37.8519291666667));
#252319=CARTESIAN_POINT('Ctrl Pts',(42.7163704007519,32.5748228215052,-37.7935958333334));
#252320=CARTESIAN_POINT('Ctrl Pts',(42.1191763815623,31.5404524382925,-37.7352625));
#252321=CARTESIAN_POINT('Ctrl Pts',(42.7163704007519,30.5060820550798,-37.6769291666667));
#252322=CARTESIAN_POINT('Ctrl Pts',(43.3135644199415,29.4717116718671,-37.6185958333333));
#252323=CARTESIAN_POINT('Ctrl Pts',(44.5079524583208,29.4717116718671,-37.5602625));
#252324=CARTESIAN_POINT('Ctrl Pts',(45.7023404967,29.4717116718671,-37.5019291666666));
#252325=CARTESIAN_POINT('Ctrl Pts',(46.2995345158897,30.5060820550798,-37.4435958333333));
#252326=CARTESIAN_POINT('Ctrl Pts',(46.8967285350793,31.5404524382925,-37.3852625));
#252327=CARTESIAN_POINT('Ctrl Pts',(46.2995345158897,32.5748228215052,-37.3269291666667));
#252328=CARTESIAN_POINT('Ctrl Pts',(45.7023404967,33.6091932047179,-37.2685958333333));
#252329=CARTESIAN_POINT('Ctrl Pts',(44.5079524583208,33.6091932047179,-37.2102625));
#252330=CARTESIAN_POINT('Ctrl Pts',(43.3135644199415,33.6091932047179,-37.1519291666667));
#252331=CARTESIAN_POINT('Ctrl Pts',(42.7163704007519,32.5748228215052,-37.0935958333333));
#252332=CARTESIAN_POINT('Ctrl Pts',(42.1191763815623,31.5404524382925,-37.0352625));
#252333=CARTESIAN_POINT('Ctrl Pts',(42.7163704007519,30.5060820550798,-36.9769291666667));
#252334=CARTESIAN_POINT('Ctrl Pts',(43.3135644199415,29.4717116718671,-36.9185958333333));
#252335=CARTESIAN_POINT('Ctrl Pts',(44.5079524583208,29.4717116718671,-36.8602625));
#252336=CARTESIAN_POINT('Ctrl Pts',(45.7023404967,29.4717116718671,-36.8019291666666));
#252337=CARTESIAN_POINT('Ctrl Pts',(46.2995345158897,30.5060820550798,-36.7435958333334));
#252338=CARTESIAN_POINT('Ctrl Pts',(46.8967285350793,31.5404524382925,-36.6852625));
#252339=CARTESIAN_POINT('Ctrl Pts',(46.2995345158897,32.5748228215052,-36.6269291666666));
#252340=CARTESIAN_POINT('Ctrl Pts',(46.222006582932,32.7091051403937,-36.6193563132714));
#252341=CARTESIAN_POINT('Ctrl Pts',(46.1253278975281,32.8303303578336,-36.611216324118));
#252342=CARTESIAN_POINT('Ctrl Pts',(44.5079524583208,33.2091977213449,-52.8412));
#252343=CARTESIAN_POINT('Ctrl Pts',(43.5445019199415,33.2091977213449,-52.7828666666667));
#252344=CARTESIAN_POINT('Ctrl Pts',(43.0627766507519,32.3748250798187,-52.7245333333334));
#252345=CARTESIAN_POINT('Ctrl Pts',(42.5810513815623,31.5404524382925,-52.6662));
#252346=CARTESIAN_POINT('Ctrl Pts',(43.0627766507519,30.7060797967663,-52.6078666666667));
#252347=CARTESIAN_POINT('Ctrl Pts',(43.5445019199415,29.87170715524,-52.5495333333333));
#252348=CARTESIAN_POINT('Ctrl Pts',(44.5079524583208,29.87170715524,-52.4912));
#252349=CARTESIAN_POINT('Ctrl Pts',(45.4714029967,29.87170715524,-52.4328666666667));
#252350=CARTESIAN_POINT('Ctrl Pts',(45.9531282658897,30.7060797967663,-52.3745333333334));
#252351=CARTESIAN_POINT('Ctrl Pts',(46.4348535350793,31.5404524382925,-52.3162000000001));
#252352=CARTESIAN_POINT('Ctrl Pts',(45.9531282658897,32.3748250798187,-52.2578666666667));
#252353=CARTESIAN_POINT('Ctrl Pts',(45.4714029967,33.2091977213449,-52.1995333333334));
#252354=CARTESIAN_POINT('Ctrl Pts',(44.5079524583208,33.2091977213449,-52.1412));
#252355=CARTESIAN_POINT('Ctrl Pts',(43.5445019199415,33.2091977213449,-52.0828666666667));
#252356=CARTESIAN_POINT('Ctrl Pts',(43.0627766507519,32.3748250798187,-52.0245333333333));
#252357=CARTESIAN_POINT('Ctrl Pts',(42.5810513815623,31.5404524382925,-51.9662));
#252358=CARTESIAN_POINT('Ctrl Pts',(43.0627766507519,30.7060797967663,-51.9078666666667));
#252359=CARTESIAN_POINT('Ctrl Pts',(43.5445019199415,29.87170715524,-51.8495333333334));
#252360=CARTESIAN_POINT('Ctrl Pts',(44.5079524583208,29.87170715524,-51.7912));
#252361=CARTESIAN_POINT('Ctrl Pts',(45.4714029967,29.87170715524,-51.7328666666667));
#252362=CARTESIAN_POINT('Ctrl Pts',(45.9531282658897,30.7060797967663,-51.6745333333333));
#252363=CARTESIAN_POINT('Ctrl Pts',(46.4348535350793,31.5404524382925,-51.6162));
#252364=CARTESIAN_POINT('Ctrl Pts',(45.9531282658897,32.3748250798187,-51.5578666666667));
#252365=CARTESIAN_POINT('Ctrl Pts',(45.4714029967,33.2091977213449,-51.4995333333333));
#252366=CARTESIAN_POINT('Ctrl Pts',(44.5079524583208,33.2091977213449,-51.4412));
#252367=CARTESIAN_POINT('Ctrl Pts',(43.5445019199415,33.2091977213449,-51.3828666666667));
#252368=CARTESIAN_POINT('Ctrl Pts',(43.0627766507519,32.3748250798187,-51.3245333333334));
#252369=CARTESIAN_POINT('Ctrl Pts',(42.5810513815623,31.5404524382925,-51.2662));
#252370=CARTESIAN_POINT('Ctrl Pts',(43.0627766507519,30.7060797967663,-51.2078666666667));
#252371=CARTESIAN_POINT('Ctrl Pts',(43.5445019199415,29.87170715524,-51.1495333333333));
#252372=CARTESIAN_POINT('Ctrl Pts',(44.5079524583208,29.87170715524,-51.0912));
#252373=CARTESIAN_POINT('Ctrl Pts',(45.4714029967,29.87170715524,-51.0328666666667));
#252374=CARTESIAN_POINT('Ctrl Pts',(45.9531282658897,30.7060797967663,-50.9745333333333));
#252375=CARTESIAN_POINT('Ctrl Pts',(46.4348535350793,31.5404524382925,-50.9162));
#252376=CARTESIAN_POINT('Ctrl Pts',(45.9531282658897,32.3748250798187,-50.8578666666667));
#252377=CARTESIAN_POINT('Ctrl Pts',(45.4714029967,33.2091977213449,-50.7995333333333));
#252378=CARTESIAN_POINT('Ctrl Pts',(44.5079524583208,33.2091977213449,-50.7412));
#252379=CARTESIAN_POINT('Ctrl Pts',(43.5445019199415,33.2091977213449,-50.6828666666667));
#252380=CARTESIAN_POINT('Ctrl Pts',(43.0627766507519,32.3748250798187,-50.6245333333333));
#252381=CARTESIAN_POINT('Ctrl Pts',(42.5810513815623,31.5404524382925,-50.5662));
#252382=CARTESIAN_POINT('Ctrl Pts',(43.0627766507519,30.7060797967663,-50.5078666666667));
#252383=CARTESIAN_POINT('Ctrl Pts',(43.5445019199415,29.87170715524,-50.4495333333333));
#252384=CARTESIAN_POINT('Ctrl Pts',(44.5079524583208,29.87170715524,-50.3912));
#252385=CARTESIAN_POINT('Ctrl Pts',(45.4714029967,29.87170715524,-50.3328666666666));
#252386=CARTESIAN_POINT('Ctrl Pts',(45.9531282658897,30.7060797967663,-50.2745333333333));
#252387=CARTESIAN_POINT('Ctrl Pts',(46.4348535350793,31.5404524382925,-50.2162));
#252388=CARTESIAN_POINT('Ctrl Pts',(45.9531282658897,32.3748250798187,-50.1578666666667));
#252389=CARTESIAN_POINT('Ctrl Pts',(45.4714029967,33.2091977213449,-50.0995333333333));
#252390=CARTESIAN_POINT('Ctrl Pts',(44.5079524583208,33.2091977213449,-50.0412));
#252391=CARTESIAN_POINT('Ctrl Pts',(43.5445019199415,33.2091977213449,-49.9828666666667));
#252392=CARTESIAN_POINT('Ctrl Pts',(43.0627766507519,32.3748250798187,-49.9245333333334));
#252393=CARTESIAN_POINT('Ctrl Pts',(42.5810513815623,31.5404524382925,-49.8662));
#252394=CARTESIAN_POINT('Ctrl Pts',(43.0627766507519,30.7060797967663,-49.8078666666667));
#252395=CARTESIAN_POINT('Ctrl Pts',(43.5445019199415,29.87170715524,-49.7495333333333));
#252396=CARTESIAN_POINT('Ctrl Pts',(44.5079524583208,29.87170715524,-49.6912));
#252397=CARTESIAN_POINT('Ctrl Pts',(45.4714029967,29.87170715524,-49.6328666666667));
#252398=CARTESIAN_POINT('Ctrl Pts',(45.9531282658897,30.7060797967663,-49.5745333333333));
#252399=CARTESIAN_POINT('Ctrl Pts',(46.4348535350793,31.5404524382925,-49.5162));
#252400=CARTESIAN_POINT('Ctrl Pts',(45.9531282658897,32.3748250798187,-49.4578666666667));
#252401=CARTESIAN_POINT('Ctrl Pts',(45.4714029967,33.2091977213449,-49.3995333333333));
#252402=CARTESIAN_POINT('Ctrl Pts',(44.5079524583208,33.2091977213449,-49.3412));
#252403=CARTESIAN_POINT('Ctrl Pts',(43.5445019199415,33.2091977213449,-49.2828666666666));
#252404=CARTESIAN_POINT('Ctrl Pts',(43.0627766507519,32.3748250798187,-49.2245333333333));
#252405=CARTESIAN_POINT('Ctrl Pts',(42.5810513815623,31.5404524382925,-49.1662));
#252406=CARTESIAN_POINT('Ctrl Pts',(43.0627766507519,30.7060797967663,-49.1078666666667));
#252407=CARTESIAN_POINT('Ctrl Pts',(43.5445019199415,29.87170715524,-49.0495333333334));
#252408=CARTESIAN_POINT('Ctrl Pts',(44.5079524583208,29.87170715524,-48.9912));
#252409=CARTESIAN_POINT('Ctrl Pts',(45.4714029967,29.87170715524,-48.9328666666667));
#252410=CARTESIAN_POINT('Ctrl Pts',(45.9531282658897,30.7060797967663,-48.8745333333333));
#252411=CARTESIAN_POINT('Ctrl Pts',(46.4348535350793,31.5404524382925,-48.8162));
#252412=CARTESIAN_POINT('Ctrl Pts',(45.9531282658897,32.3748250798187,-48.7578666666667));
#252413=CARTESIAN_POINT('Ctrl Pts',(45.4714029967,33.2091977213449,-48.6995333333334));
#252414=CARTESIAN_POINT('Ctrl Pts',(44.5079524583208,33.2091977213449,-48.6412));
#252415=CARTESIAN_POINT('Ctrl Pts',(43.5445019199415,33.2091977213449,-48.5828666666667));
#252416=CARTESIAN_POINT('Ctrl Pts',(43.0627766507519,32.3748250798187,-48.5245333333333));
#252417=CARTESIAN_POINT('Ctrl Pts',(42.5810513815623,31.5404524382925,-48.4662));
#252418=CARTESIAN_POINT('Ctrl Pts',(43.0627766507519,30.7060797967663,-48.4078666666667));
#252419=CARTESIAN_POINT('Ctrl Pts',(43.5445019199415,29.87170715524,-48.3495333333333));
#252420=CARTESIAN_POINT('Ctrl Pts',(44.5079524583208,29.87170715524,-48.2912));
#252421=CARTESIAN_POINT('Ctrl Pts',(45.4714029967,29.87170715524,-48.2328666666667));
#252422=CARTESIAN_POINT('Ctrl Pts',(45.9531282658897,30.7060797967663,-48.1745333333334));
#252423=CARTESIAN_POINT('Ctrl Pts',(46.4348535350793,31.5404524382925,-48.1162));
#252424=CARTESIAN_POINT('Ctrl Pts',(45.9531282658897,32.3748250798187,-48.0578666666667));
#252425=CARTESIAN_POINT('Ctrl Pts',(45.4714029967,33.2091977213449,-47.9995333333334));
#252426=CARTESIAN_POINT('Ctrl Pts',(44.5079524583208,33.2091977213449,-47.9412));
#252427=CARTESIAN_POINT('Ctrl Pts',(43.5445019199415,33.2091977213449,-47.8828666666667));
#252428=CARTESIAN_POINT('Ctrl Pts',(43.0627766507519,32.3748250798187,-47.8245333333333));
#252429=CARTESIAN_POINT('Ctrl Pts',(42.5810513815623,31.5404524382925,-47.7662));
#252430=CARTESIAN_POINT('Ctrl Pts',(43.0627766507519,30.7060797967663,-47.7078666666667));
#252431=CARTESIAN_POINT('Ctrl Pts',(43.5445019199415,29.87170715524,-47.6495333333334));
#252432=CARTESIAN_POINT('Ctrl Pts',(44.5079524583208,29.87170715524,-47.5912));
#252433=CARTESIAN_POINT('Ctrl Pts',(45.4714029967,29.87170715524,-47.5328666666667));
#252434=CARTESIAN_POINT('Ctrl Pts',(45.9531282658897,30.7060797967663,-47.4745333333334));
#252435=CARTESIAN_POINT('Ctrl Pts',(46.4348535350793,31.5404524382925,-47.4162));
#252436=CARTESIAN_POINT('Ctrl Pts',(45.9531282658897,32.3748250798187,-47.3578666666667));
#252437=CARTESIAN_POINT('Ctrl Pts',(45.4714029967,33.2091977213449,-47.2995333333334));
#252438=CARTESIAN_POINT('Ctrl Pts',(44.5079524583208,33.2091977213449,-47.2412));
#252439=CARTESIAN_POINT('Ctrl Pts',(43.5445019199415,33.2091977213449,-47.1828666666667));
#252440=CARTESIAN_POINT('Ctrl Pts',(43.0627766507519,32.3748250798187,-47.1245333333333));
#252441=CARTESIAN_POINT('Ctrl Pts',(42.5810513815623,31.5404524382925,-47.0662));
#252442=CARTESIAN_POINT('Ctrl Pts',(43.0627766507519,30.7060797967663,-47.0078666666667));
#252443=CARTESIAN_POINT('Ctrl Pts',(43.5445019199415,29.87170715524,-46.9495333333334));
#252444=CARTESIAN_POINT('Ctrl Pts',(44.5079524583208,29.87170715524,-46.8912));
#252445=CARTESIAN_POINT('Ctrl Pts',(45.4714029967,29.87170715524,-46.8328666666667));
#252446=CARTESIAN_POINT('Ctrl Pts',(45.9531282658897,30.7060797967663,-46.7745333333333));
#252447=CARTESIAN_POINT('Ctrl Pts',(46.4348535350793,31.5404524382925,-46.7162));
#252448=CARTESIAN_POINT('Ctrl Pts',(45.9531282658897,32.3748250798187,-46.6578666666667));
#252449=CARTESIAN_POINT('Ctrl Pts',(45.4714029967,33.2091977213449,-46.5995333333333));
#252450=CARTESIAN_POINT('Ctrl Pts',(44.5079524583208,33.2091977213449,-46.5412));
#252451=CARTESIAN_POINT('Ctrl Pts',(43.5445019199415,33.2091977213449,-46.4828666666667));
#252452=CARTESIAN_POINT('Ctrl Pts',(43.0627766507519,32.3748250798187,-46.4245333333333));
#252453=CARTESIAN_POINT('Ctrl Pts',(42.5810513815623,31.5404524382925,-46.3662));
#252454=CARTESIAN_POINT('Ctrl Pts',(43.0627766507519,30.7060797967663,-46.3078666666667));
#252455=CARTESIAN_POINT('Ctrl Pts',(43.5445019199415,29.87170715524,-46.2495333333334));
#252456=CARTESIAN_POINT('Ctrl Pts',(44.5079524583208,29.87170715524,-46.1912));
#252457=CARTESIAN_POINT('Ctrl Pts',(45.4714029967,29.87170715524,-46.1328666666667));
#252458=CARTESIAN_POINT('Ctrl Pts',(45.9531282658897,30.7060797967663,-46.0745333333334));
#252459=CARTESIAN_POINT('Ctrl Pts',(46.4348535350793,31.5404524382925,-46.0162));
#252460=CARTESIAN_POINT('Ctrl Pts',(45.9531282658897,32.3748250798187,-45.9578666666667));
#252461=CARTESIAN_POINT('Ctrl Pts',(45.4714029967,33.2091977213449,-45.8995333333333));
#252462=CARTESIAN_POINT('Ctrl Pts',(44.5079524583208,33.2091977213449,-45.8412));
#252463=CARTESIAN_POINT('Ctrl Pts',(43.5445019199415,33.2091977213449,-45.7828666666667));
#252464=CARTESIAN_POINT('Ctrl Pts',(43.0627766507519,32.3748250798187,-45.7245333333333));
#252465=CARTESIAN_POINT('Ctrl Pts',(42.5810513815623,31.5404524382925,-45.6662));
#252466=CARTESIAN_POINT('Ctrl Pts',(43.0627766507519,30.7060797967663,-45.6078666666667));
#252467=CARTESIAN_POINT('Ctrl Pts',(43.5445019199415,29.87170715524,-45.5495333333333));
#252468=CARTESIAN_POINT('Ctrl Pts',(44.5079524583208,29.87170715524,-45.4912));
#252469=CARTESIAN_POINT('Ctrl Pts',(45.4714029967,29.87170715524,-45.4328666666666));
#252470=CARTESIAN_POINT('Ctrl Pts',(45.9531282658897,30.7060797967663,-45.3745333333333));
#252471=CARTESIAN_POINT('Ctrl Pts',(46.4348535350793,31.5404524382925,-45.3162));
#252472=CARTESIAN_POINT('Ctrl Pts',(45.9531282658897,32.3748250798187,-45.2578666666667));
#252473=CARTESIAN_POINT('Ctrl Pts',(45.4714029967,33.2091977213449,-45.1995333333333));
#252474=CARTESIAN_POINT('Ctrl Pts',(44.5079524583208,33.2091977213449,-45.1412));
#252475=CARTESIAN_POINT('Ctrl Pts',(43.5445019199415,33.2091977213449,-45.0828666666667));
#252476=CARTESIAN_POINT('Ctrl Pts',(43.0627766507519,32.3748250798187,-45.0245333333333));
#252477=CARTESIAN_POINT('Ctrl Pts',(42.5810513815623,31.5404524382925,-44.9662));
#252478=CARTESIAN_POINT('Ctrl Pts',(43.0627766507519,30.7060797967663,-44.9078666666666));
#252479=CARTESIAN_POINT('Ctrl Pts',(43.5445019199415,29.87170715524,-44.8495333333333));
#252480=CARTESIAN_POINT('Ctrl Pts',(44.5079524583208,29.87170715524,-44.7912));
#252481=CARTESIAN_POINT('Ctrl Pts',(45.4714029967,29.87170715524,-44.7328666666666));
#252482=CARTESIAN_POINT('Ctrl Pts',(45.9531282658897,30.7060797967663,-44.6745333333334));
#252483=CARTESIAN_POINT('Ctrl Pts',(46.4348535350793,31.5404524382925,-44.6162));
#252484=CARTESIAN_POINT('Ctrl Pts',(45.9531282658897,32.3748250798187,-44.5578666666667));
#252485=CARTESIAN_POINT('Ctrl Pts',(45.4714029967,33.2091977213449,-44.4995333333333));
#252486=CARTESIAN_POINT('Ctrl Pts',(44.5079524583208,33.2091977213449,-44.4412));
#252487=CARTESIAN_POINT('Ctrl Pts',(43.5445019199415,33.2091977213449,-44.3828666666667));
#252488=CARTESIAN_POINT('Ctrl Pts',(43.0627766507519,32.3748250798187,-44.3245333333334));
#252489=CARTESIAN_POINT('Ctrl Pts',(42.5810513815623,31.5404524382925,-44.2662));
#252490=CARTESIAN_POINT('Ctrl Pts',(43.0627766507519,30.7060797967663,-44.2078666666667));
#252491=CARTESIAN_POINT('Ctrl Pts',(43.5445019199415,29.87170715524,-44.1495333333334));
#252492=CARTESIAN_POINT('Ctrl Pts',(44.5079524583208,29.87170715524,-44.0912));
#252493=CARTESIAN_POINT('Ctrl Pts',(45.4714029967,29.87170715524,-44.0328666666667));
#252494=CARTESIAN_POINT('Ctrl Pts',(45.9531282658897,30.7060797967663,-43.9745333333333));
#252495=CARTESIAN_POINT('Ctrl Pts',(46.4348535350793,31.5404524382925,-43.9162));
#252496=CARTESIAN_POINT('Ctrl Pts',(45.9531282658897,32.3748250798187,-43.8578666666667));
#252497=CARTESIAN_POINT('Ctrl Pts',(45.4714029967,33.2091977213449,-43.7995333333334));
#252498=CARTESIAN_POINT('Ctrl Pts',(44.5079524583208,33.2091977213449,-43.7412));
#252499=CARTESIAN_POINT('Ctrl Pts',(43.5445019199415,33.2091977213449,-43.6828666666667));
#252500=CARTESIAN_POINT('Ctrl Pts',(43.0627766507519,32.3748250798187,-43.6245333333333));
#252501=CARTESIAN_POINT('Ctrl Pts',(42.5810513815623,31.5404524382925,-43.5662));
#252502=CARTESIAN_POINT('Ctrl Pts',(43.0627766507519,30.7060797967663,-43.5078666666667));
#252503=CARTESIAN_POINT('Ctrl Pts',(43.5445019199415,29.87170715524,-43.4495333333334));
#252504=CARTESIAN_POINT('Ctrl Pts',(44.5079524583208,29.87170715524,-43.3912));
#252505=CARTESIAN_POINT('Ctrl Pts',(45.4714029967,29.87170715524,-43.3328666666667));
#252506=CARTESIAN_POINT('Ctrl Pts',(45.9531282658897,30.7060797967663,-43.2745333333334));
#252507=CARTESIAN_POINT('Ctrl Pts',(46.4348535350793,31.5404524382925,-43.2162));
#252508=CARTESIAN_POINT('Ctrl Pts',(45.9531282658897,32.3748250798187,-43.1578666666667));
#252509=CARTESIAN_POINT('Ctrl Pts',(45.4714029967,33.2091977213449,-43.0995333333334));
#252510=CARTESIAN_POINT('Ctrl Pts',(44.5079524583208,33.2091977213449,-43.0412));
#252511=CARTESIAN_POINT('Ctrl Pts',(43.5445019199415,33.2091977213449,-42.9828666666667));
#252512=CARTESIAN_POINT('Ctrl Pts',(43.0627766507519,32.3748250798187,-42.9245333333334));
#252513=CARTESIAN_POINT('Ctrl Pts',(42.5810513815623,31.5404524382925,-42.8662));
#252514=CARTESIAN_POINT('Ctrl Pts',(43.0627766507519,30.7060797967663,-42.8078666666667));
#252515=CARTESIAN_POINT('Ctrl Pts',(43.5445019199415,29.87170715524,-42.7495333333334));
#252516=CARTESIAN_POINT('Ctrl Pts',(44.5079524583208,29.87170715524,-42.6912));
#252517=CARTESIAN_POINT('Ctrl Pts',(45.4714029967,29.87170715524,-42.6328666666667));
#252518=CARTESIAN_POINT('Ctrl Pts',(45.9531282658897,30.7060797967663,-42.5745333333333));
#252519=CARTESIAN_POINT('Ctrl Pts',(46.4348535350793,31.5404524382925,-42.5162));
#252520=CARTESIAN_POINT('Ctrl Pts',(45.9531282658897,32.3748250798187,-42.4578666666667));
#252521=CARTESIAN_POINT('Ctrl Pts',(45.4714029967,33.2091977213449,-42.3995333333334));
#252522=CARTESIAN_POINT('Ctrl Pts',(44.5079524583208,33.2091977213449,-42.3412));
#252523=CARTESIAN_POINT('Ctrl Pts',(43.5445019199415,33.2091977213449,-42.2828666666667));
#252524=CARTESIAN_POINT('Ctrl Pts',(43.0627766507519,32.3748250798187,-42.2245333333333));
#252525=CARTESIAN_POINT('Ctrl Pts',(42.5810513815623,31.5404524382925,-42.1662));
#252526=CARTESIAN_POINT('Ctrl Pts',(43.0627766507519,30.7060797967663,-42.1078666666667));
#252527=CARTESIAN_POINT('Ctrl Pts',(43.5445019199415,29.87170715524,-42.0495333333334));
#252528=CARTESIAN_POINT('Ctrl Pts',(44.5079524583208,29.87170715524,-41.9912));
#252529=CARTESIAN_POINT('Ctrl Pts',(45.4714029967,29.87170715524,-41.9328666666667));
#252530=CARTESIAN_POINT('Ctrl Pts',(45.9531282658897,30.7060797967663,-41.8745333333334));
#252531=CARTESIAN_POINT('Ctrl Pts',(46.4348535350793,31.5404524382925,-41.8162));
#252532=CARTESIAN_POINT('Ctrl Pts',(45.9531282658897,32.3748250798187,-41.7578666666667));
#252533=CARTESIAN_POINT('Ctrl Pts',(45.4714029967,33.2091977213449,-41.6995333333333));
#252534=CARTESIAN_POINT('Ctrl Pts',(44.5079524583208,33.2091977213449,-41.6412));
#252535=CARTESIAN_POINT('Ctrl Pts',(43.5445019199415,33.2091977213449,-41.5828666666667));
#252536=CARTESIAN_POINT('Ctrl Pts',(43.0627766507519,32.3748250798187,-41.5245333333334));
#252537=CARTESIAN_POINT('Ctrl Pts',(42.5810513815623,31.5404524382925,-41.4662));
#252538=CARTESIAN_POINT('Ctrl Pts',(43.0627766507519,30.7060797967663,-41.4078666666667));
#252539=CARTESIAN_POINT('Ctrl Pts',(43.5445019199415,29.87170715524,-41.3495333333333));
#252540=CARTESIAN_POINT('Ctrl Pts',(44.5079524583208,29.87170715524,-41.2912));
#252541=CARTESIAN_POINT('Ctrl Pts',(45.4714029967,29.87170715524,-41.2328666666667));
#252542=CARTESIAN_POINT('Ctrl Pts',(45.9531282658897,30.7060797967663,-41.1745333333334));
#252543=CARTESIAN_POINT('Ctrl Pts',(46.4348535350793,31.5404524382925,-41.1162));
#252544=CARTESIAN_POINT('Ctrl Pts',(45.9531282658897,32.3748250798187,-41.0578666666667));
#252545=CARTESIAN_POINT('Ctrl Pts',(45.4714029967,33.2091977213449,-40.9995333333333));
#252546=CARTESIAN_POINT('Ctrl Pts',(44.5079524583208,33.2091977213449,-40.9412));
#252547=CARTESIAN_POINT('Ctrl Pts',(43.5445019199415,33.2091977213449,-40.8828666666667));
#252548=CARTESIAN_POINT('Ctrl Pts',(43.0627766507519,32.3748250798187,-40.8245333333333));
#252549=CARTESIAN_POINT('Ctrl Pts',(42.5810513815623,31.5404524382925,-40.7662));
#252550=CARTESIAN_POINT('Ctrl Pts',(43.0627766507519,30.7060797967663,-40.7078666666667));
#252551=CARTESIAN_POINT('Ctrl Pts',(43.5445019199415,29.87170715524,-40.6495333333333));
#252552=CARTESIAN_POINT('Ctrl Pts',(44.5079524583208,29.87170715524,-40.5912));
#252553=CARTESIAN_POINT('Ctrl Pts',(45.4714029967,29.87170715524,-40.5328666666667));
#252554=CARTESIAN_POINT('Ctrl Pts',(45.9531282658897,30.7060797967663,-40.4745333333334));
#252555=CARTESIAN_POINT('Ctrl Pts',(46.4348535350793,31.5404524382925,-40.4162));
#252556=CARTESIAN_POINT('Ctrl Pts',(45.9531282658897,32.3748250798187,-40.3578666666667));
#252557=CARTESIAN_POINT('Ctrl Pts',(45.4714029967,33.2091977213449,-40.2995333333333));
#252558=CARTESIAN_POINT('Ctrl Pts',(44.5079524583208,33.2091977213449,-40.2412));
#252559=CARTESIAN_POINT('Ctrl Pts',(43.5445019199415,33.2091977213449,-40.1828666666667));
#252560=CARTESIAN_POINT('Ctrl Pts',(43.0627766507519,32.3748250798187,-40.1245333333334));
#252561=CARTESIAN_POINT('Ctrl Pts',(42.5810513815623,31.5404524382925,-40.0662));
#252562=CARTESIAN_POINT('Ctrl Pts',(43.0627766507519,30.7060797967663,-40.0078666666667));
#252563=CARTESIAN_POINT('Ctrl Pts',(43.5445019199415,29.87170715524,-39.9495333333333));
#252564=CARTESIAN_POINT('Ctrl Pts',(44.5079524583208,29.87170715524,-39.8912));
#252565=CARTESIAN_POINT('Ctrl Pts',(45.4714029967,29.87170715524,-39.8328666666666));
#252566=CARTESIAN_POINT('Ctrl Pts',(45.9531282658897,30.7060797967663,-39.7745333333334));
#252567=CARTESIAN_POINT('Ctrl Pts',(46.4348535350793,31.5404524382925,-39.7162));
#252568=CARTESIAN_POINT('Ctrl Pts',(45.9531282658897,32.3748250798187,-39.6578666666667));
#252569=CARTESIAN_POINT('Ctrl Pts',(45.4714029967,33.2091977213449,-39.5995333333333));
#252570=CARTESIAN_POINT('Ctrl Pts',(44.5079524583208,33.2091977213449,-39.5412));
#252571=CARTESIAN_POINT('Ctrl Pts',(43.5445019199415,33.2091977213449,-39.4828666666666));
#252572=CARTESIAN_POINT('Ctrl Pts',(43.0627766507519,32.3748250798187,-39.4245333333334));
#252573=CARTESIAN_POINT('Ctrl Pts',(42.5810513815623,31.5404524382925,-39.3662));
#252574=CARTESIAN_POINT('Ctrl Pts',(43.0627766507519,30.7060797967663,-39.3078666666666));
#252575=CARTESIAN_POINT('Ctrl Pts',(43.5445019199415,29.87170715524,-39.2495333333333));
#252576=CARTESIAN_POINT('Ctrl Pts',(44.5079524583208,29.87170715524,-39.1912));
#252577=CARTESIAN_POINT('Ctrl Pts',(45.4714029967,29.87170715524,-39.1328666666667));
#252578=CARTESIAN_POINT('Ctrl Pts',(45.9531282658897,30.7060797967663,-39.0745333333333));
#252579=CARTESIAN_POINT('Ctrl Pts',(46.4348535350793,31.5404524382925,-39.0162));
#252580=CARTESIAN_POINT('Ctrl Pts',(45.9531282658897,32.3748250798187,-38.9578666666667));
#252581=CARTESIAN_POINT('Ctrl Pts',(45.4714029967,33.2091977213449,-38.8995333333334));
#252582=CARTESIAN_POINT('Ctrl Pts',(44.5079524583208,33.2091977213449,-38.8412));
#252583=CARTESIAN_POINT('Ctrl Pts',(43.5445019199415,33.2091977213449,-38.7828666666667));
#252584=CARTESIAN_POINT('Ctrl Pts',(43.0627766507519,32.3748250798187,-38.7245333333334));
#252585=CARTESIAN_POINT('Ctrl Pts',(42.5810513815623,31.5404524382925,-38.6662));
#252586=CARTESIAN_POINT('Ctrl Pts',(43.0627766507519,30.7060797967663,-38.6078666666667));
#252587=CARTESIAN_POINT('Ctrl Pts',(43.5445019199415,29.87170715524,-38.5495333333334));
#252588=CARTESIAN_POINT('Ctrl Pts',(44.5079524583208,29.87170715524,-38.4912));
#252589=CARTESIAN_POINT('Ctrl Pts',(45.4714029967,29.87170715524,-38.4328666666667));
#252590=CARTESIAN_POINT('Ctrl Pts',(45.9531282658897,30.7060797967663,-38.3745333333333));
#252591=CARTESIAN_POINT('Ctrl Pts',(46.4348535350793,31.5404524382925,-38.3162));
#252592=CARTESIAN_POINT('Ctrl Pts',(45.9531282658897,32.3748250798187,-38.2578666666667));
#252593=CARTESIAN_POINT('Ctrl Pts',(45.4714029967,33.2091977213449,-38.1995333333333));
#252594=CARTESIAN_POINT('Ctrl Pts',(44.5079524583208,33.2091977213449,-38.1412));
#252595=CARTESIAN_POINT('Ctrl Pts',(43.5445019199415,33.2091977213449,-38.0828666666667));
#252596=CARTESIAN_POINT('Ctrl Pts',(43.0627766507519,32.3748250798187,-38.0245333333334));
#252597=CARTESIAN_POINT('Ctrl Pts',(42.5810513815623,31.5404524382925,-37.9662));
#252598=CARTESIAN_POINT('Ctrl Pts',(43.0627766507519,30.7060797967663,-37.9078666666667));
#252599=CARTESIAN_POINT('Ctrl Pts',(43.5445019199415,29.87170715524,-37.8495333333334));
#252600=CARTESIAN_POINT('Ctrl Pts',(44.5079524583208,29.87170715524,-37.7912));
#252601=CARTESIAN_POINT('Ctrl Pts',(45.4714029967,29.87170715524,-37.7328666666667));
#252602=CARTESIAN_POINT('Ctrl Pts',(45.9531282658897,30.7060797967663,-37.6745333333334));
#252603=CARTESIAN_POINT('Ctrl Pts',(46.4348535350793,31.5404524382925,-37.6162));
#252604=CARTESIAN_POINT('Ctrl Pts',(45.9531282658897,32.3748250798187,-37.5578666666667));
#252605=CARTESIAN_POINT('Ctrl Pts',(45.4714029967,33.2091977213449,-37.4995333333334));
#252606=CARTESIAN_POINT('Ctrl Pts',(44.5079524583208,33.2091977213449,-37.4412));
#252607=CARTESIAN_POINT('Ctrl Pts',(43.5445019199415,33.2091977213449,-37.3828666666667));
#252608=CARTESIAN_POINT('Ctrl Pts',(43.0627766507519,32.3748250798187,-37.3245333333333));
#252609=CARTESIAN_POINT('Ctrl Pts',(42.5810513815623,31.5404524382925,-37.2662));
#252610=CARTESIAN_POINT('Ctrl Pts',(43.0627766507519,30.7060797967663,-37.2078666666667));
#252611=CARTESIAN_POINT('Ctrl Pts',(43.5445019199415,29.87170715524,-37.1495333333334));
#252612=CARTESIAN_POINT('Ctrl Pts',(44.5079524583208,29.87170715524,-37.0912));
#252613=CARTESIAN_POINT('Ctrl Pts',(45.4714029967,29.87170715524,-37.0328666666667));
#252614=CARTESIAN_POINT('Ctrl Pts',(45.9531282658897,30.7060797967663,-36.9745333333333));
#252615=CARTESIAN_POINT('Ctrl Pts',(46.4348535350793,31.5404524382925,-36.9162));
#252616=CARTESIAN_POINT('Ctrl Pts',(45.9531282658897,32.3748250798187,-36.8578666666667));
#252617=CARTESIAN_POINT('Ctrl Pts',(45.8905905257689,32.4831436230984,-36.8502938132714));
#252618=CARTESIAN_POINT('Ctrl Pts',(45.8126048724392,32.5809296836203,-36.8421538241181));
#252619=CARTESIAN_POINT('Ctrl Pts',(44.5079524583208,33.6091932047179,-52.6102625));
#252620=CARTESIAN_POINT('Ctrl Pts',(43.3135644199415,33.6091932047179,-52.5519291666666));
#252621=CARTESIAN_POINT('Ctrl Pts',(42.7163704007519,32.5748228215052,-52.4935958333333));
#252622=CARTESIAN_POINT('Ctrl Pts',(42.1191763815623,31.5404524382925,-52.4352625));
#252623=CARTESIAN_POINT('Ctrl Pts',(42.7163704007519,30.5060820550798,-52.3769291666667));
#252624=CARTESIAN_POINT('Ctrl Pts',(43.3135644199415,29.4717116718671,-52.3185958333334));
#252625=CARTESIAN_POINT('Ctrl Pts',(44.5079524583208,29.4717116718671,-52.2602625));
#252626=CARTESIAN_POINT('Ctrl Pts',(45.7023404967,29.4717116718671,-52.2019291666667));
#252627=CARTESIAN_POINT('Ctrl Pts',(46.2995345158897,30.5060820550798,-52.1435958333333));
#252628=CARTESIAN_POINT('Ctrl Pts',(46.8967285350793,31.5404524382925,-52.0852625));
#252629=CARTESIAN_POINT('Ctrl Pts',(46.2995345158897,32.5748228215052,-52.0269291666667));
#252630=CARTESIAN_POINT('Ctrl Pts',(45.7023404967,33.6091932047179,-51.9685958333333));
#252631=CARTESIAN_POINT('Ctrl Pts',(44.5079524583208,33.6091932047179,-51.9102625));
#252632=CARTESIAN_POINT('Ctrl Pts',(43.3135644199415,33.6091932047179,-51.8519291666667));
#252633=CARTESIAN_POINT('Ctrl Pts',(42.7163704007519,32.5748228215052,-51.7935958333333));
#252634=CARTESIAN_POINT('Ctrl Pts',(42.1191763815623,31.5404524382925,-51.7352625));
#252635=CARTESIAN_POINT('Ctrl Pts',(42.7163704007519,30.5060820550798,-51.6769291666667));
#252636=CARTESIAN_POINT('Ctrl Pts',(43.3135644199415,29.4717116718671,-51.6185958333333));
#252637=CARTESIAN_POINT('Ctrl Pts',(44.5079524583208,29.4717116718671,-51.5602625));
#252638=CARTESIAN_POINT('Ctrl Pts',(45.7023404967,29.4717116718671,-51.5019291666666));
#252639=CARTESIAN_POINT('Ctrl Pts',(46.2995345158897,30.5060820550798,-51.4435958333333));
#252640=CARTESIAN_POINT('Ctrl Pts',(46.8967285350793,31.5404524382925,-51.3852625));
#252641=CARTESIAN_POINT('Ctrl Pts',(46.2995345158897,32.5748228215052,-51.3269291666667));
#252642=CARTESIAN_POINT('Ctrl Pts',(45.7023404967,33.6091932047179,-51.2685958333333));
#252643=CARTESIAN_POINT('Ctrl Pts',(44.5079524583208,33.6091932047179,-51.2102625));
#252644=CARTESIAN_POINT('Ctrl Pts',(43.3135644199415,33.6091932047179,-51.1519291666666));
#252645=CARTESIAN_POINT('Ctrl Pts',(42.7163704007519,32.5748228215052,-51.0935958333334));
#252646=CARTESIAN_POINT('Ctrl Pts',(42.1191763815623,31.5404524382925,-51.0352625));
#252647=CARTESIAN_POINT('Ctrl Pts',(42.7163704007519,30.5060820550798,-50.9769291666667));
#252648=CARTESIAN_POINT('Ctrl Pts',(43.3135644199415,29.4717116718671,-50.9185958333333));
#252649=CARTESIAN_POINT('Ctrl Pts',(44.5079524583208,29.4717116718671,-50.8602625));
#252650=CARTESIAN_POINT('Ctrl Pts',(45.7023404967,29.4717116718671,-50.8019291666667));
#252651=CARTESIAN_POINT('Ctrl Pts',(46.2995345158897,30.5060820550798,-50.7435958333333));
#252652=CARTESIAN_POINT('Ctrl Pts',(46.8967285350793,31.5404524382925,-50.6852625));
#252653=CARTESIAN_POINT('Ctrl Pts',(46.2995345158897,32.5748228215052,-50.6269291666667));
#252654=CARTESIAN_POINT('Ctrl Pts',(45.7023404967,33.6091932047179,-50.5685958333333));
#252655=CARTESIAN_POINT('Ctrl Pts',(44.5079524583208,33.6091932047179,-50.5102625));
#252656=CARTESIAN_POINT('Ctrl Pts',(43.3135644199415,33.6091932047179,-50.4519291666667));
#252657=CARTESIAN_POINT('Ctrl Pts',(42.7163704007519,32.5748228215052,-50.3935958333333));
#252658=CARTESIAN_POINT('Ctrl Pts',(42.1191763815623,31.5404524382925,-50.3352625));
#252659=CARTESIAN_POINT('Ctrl Pts',(42.7163704007519,30.5060820550798,-50.2769291666667));
#252660=CARTESIAN_POINT('Ctrl Pts',(43.3135644199415,29.4717116718671,-50.2185958333333));
#252661=CARTESIAN_POINT('Ctrl Pts',(44.5079524583208,29.4717116718671,-50.1602625));
#252662=CARTESIAN_POINT('Ctrl Pts',(45.7023404967,29.4717116718671,-50.1019291666667));
#252663=CARTESIAN_POINT('Ctrl Pts',(46.2995345158897,30.5060820550798,-50.0435958333333));
#252664=CARTESIAN_POINT('Ctrl Pts',(46.8967285350793,31.5404524382925,-49.9852625));
#252665=CARTESIAN_POINT('Ctrl Pts',(46.2995345158897,32.5748228215052,-49.9269291666667));
#252666=CARTESIAN_POINT('Ctrl Pts',(45.7023404967,33.6091932047179,-49.8685958333333));
#252667=CARTESIAN_POINT('Ctrl Pts',(44.5079524583208,33.6091932047179,-49.8102625));
#252668=CARTESIAN_POINT('Ctrl Pts',(43.3135644199415,33.6091932047179,-49.7519291666667));
#252669=CARTESIAN_POINT('Ctrl Pts',(42.7163704007519,32.5748228215052,-49.6935958333334));
#252670=CARTESIAN_POINT('Ctrl Pts',(42.1191763815623,31.5404524382925,-49.6352625));
#252671=CARTESIAN_POINT('Ctrl Pts',(42.7163704007519,30.5060820550798,-49.5769291666667));
#252672=CARTESIAN_POINT('Ctrl Pts',(43.3135644199415,29.4717116718671,-49.5185958333334));
#252673=CARTESIAN_POINT('Ctrl Pts',(44.5079524583208,29.4717116718671,-49.4602625));
#252674=CARTESIAN_POINT('Ctrl Pts',(45.7023404967,29.4717116718671,-49.4019291666667));
#252675=CARTESIAN_POINT('Ctrl Pts',(46.2995345158897,30.5060820550798,-49.3435958333333));
#252676=CARTESIAN_POINT('Ctrl Pts',(46.8967285350793,31.5404524382925,-49.2852625));
#252677=CARTESIAN_POINT('Ctrl Pts',(46.2995345158897,32.5748228215052,-49.2269291666667));
#252678=CARTESIAN_POINT('Ctrl Pts',(45.7023404967,33.6091932047179,-49.1685958333334));
#252679=CARTESIAN_POINT('Ctrl Pts',(44.5079524583208,33.6091932047179,-49.1102625));
#252680=CARTESIAN_POINT('Ctrl Pts',(43.3135644199415,33.6091932047179,-49.0519291666667));
#252681=CARTESIAN_POINT('Ctrl Pts',(42.7163704007519,32.5748228215052,-48.9935958333333));
#252682=CARTESIAN_POINT('Ctrl Pts',(42.1191763815623,31.5404524382925,-48.9352625));
#252683=CARTESIAN_POINT('Ctrl Pts',(42.7163704007519,30.5060820550798,-48.8769291666667));
#252684=CARTESIAN_POINT('Ctrl Pts',(43.3135644199415,29.4717116718671,-48.8185958333333));
#252685=CARTESIAN_POINT('Ctrl Pts',(44.5079524583208,29.4717116718671,-48.7602625));
#252686=CARTESIAN_POINT('Ctrl Pts',(45.7023404967,29.4717116718671,-48.7019291666667));
#252687=CARTESIAN_POINT('Ctrl Pts',(46.2995345158897,30.5060820550798,-48.6435958333333));
#252688=CARTESIAN_POINT('Ctrl Pts',(46.8967285350793,31.5404524382925,-48.5852625));
#252689=CARTESIAN_POINT('Ctrl Pts',(46.2995345158897,32.5748228215052,-48.5269291666667));
#252690=CARTESIAN_POINT('Ctrl Pts',(45.7023404967,33.6091932047179,-48.4685958333333));
#252691=CARTESIAN_POINT('Ctrl Pts',(44.5079524583208,33.6091932047179,-48.4102625));
#252692=CARTESIAN_POINT('Ctrl Pts',(43.3135644199415,33.6091932047179,-48.3519291666667));
#252693=CARTESIAN_POINT('Ctrl Pts',(42.7163704007519,32.5748228215052,-48.2935958333333));
#252694=CARTESIAN_POINT('Ctrl Pts',(42.1191763815623,31.5404524382925,-48.2352625));
#252695=CARTESIAN_POINT('Ctrl Pts',(42.7163704007519,30.5060820550798,-48.1769291666667));
#252696=CARTESIAN_POINT('Ctrl Pts',(43.3135644199415,29.4717116718671,-48.1185958333334));
#252697=CARTESIAN_POINT('Ctrl Pts',(44.5079524583208,29.4717116718671,-48.0602625));
#252698=CARTESIAN_POINT('Ctrl Pts',(45.7023404967,29.4717116718671,-48.0019291666667));
#252699=CARTESIAN_POINT('Ctrl Pts',(46.2995345158897,30.5060820550798,-47.9435958333334));
#252700=CARTESIAN_POINT('Ctrl Pts',(46.8967285350793,31.5404524382925,-47.8852625));
#252701=CARTESIAN_POINT('Ctrl Pts',(46.2995345158897,32.5748228215052,-47.8269291666667));
#252702=CARTESIAN_POINT('Ctrl Pts',(45.7023404967,33.6091932047179,-47.7685958333333));
#252703=CARTESIAN_POINT('Ctrl Pts',(44.5079524583208,33.6091932047179,-47.7102625));
#252704=CARTESIAN_POINT('Ctrl Pts',(43.3135644199415,33.6091932047179,-47.6519291666667));
#252705=CARTESIAN_POINT('Ctrl Pts',(42.7163704007519,32.5748228215052,-47.5935958333333));
#252706=CARTESIAN_POINT('Ctrl Pts',(42.1191763815623,31.5404524382925,-47.5352625));
#252707=CARTESIAN_POINT('Ctrl Pts',(42.7163704007519,30.5060820550798,-47.4769291666667));
#252708=CARTESIAN_POINT('Ctrl Pts',(43.3135644199415,29.4717116718671,-47.4185958333333));
#252709=CARTESIAN_POINT('Ctrl Pts',(44.5079524583208,29.4717116718671,-47.3602625));
#252710=CARTESIAN_POINT('Ctrl Pts',(45.7023404967,29.4717116718671,-47.3019291666666));
#252711=CARTESIAN_POINT('Ctrl Pts',(46.2995345158897,30.5060820550798,-47.2435958333333));
#252712=CARTESIAN_POINT('Ctrl Pts',(46.8967285350793,31.5404524382925,-47.1852625));
#252713=CARTESIAN_POINT('Ctrl Pts',(46.2995345158897,32.5748228215052,-47.1269291666667));
#252714=CARTESIAN_POINT('Ctrl Pts',(45.7023404967,33.6091932047179,-47.0685958333333));
#252715=CARTESIAN_POINT('Ctrl Pts',(44.5079524583208,33.6091932047179,-47.0102625));
#252716=CARTESIAN_POINT('Ctrl Pts',(43.3135644199415,33.6091932047179,-46.9519291666667));
#252717=CARTESIAN_POINT('Ctrl Pts',(42.7163704007519,32.5748228215052,-46.8935958333333));
#252718=CARTESIAN_POINT('Ctrl Pts',(42.1191763815623,31.5404524382925,-46.8352625));
#252719=CARTESIAN_POINT('Ctrl Pts',(42.7163704007519,30.5060820550798,-46.7769291666667));
#252720=CARTESIAN_POINT('Ctrl Pts',(43.3135644199415,29.4717116718671,-46.7185958333333));
#252721=CARTESIAN_POINT('Ctrl Pts',(44.5079524583208,29.4717116718671,-46.6602625));
#252722=CARTESIAN_POINT('Ctrl Pts',(45.7023404967,29.4717116718671,-46.6019291666667));
#252723=CARTESIAN_POINT('Ctrl Pts',(46.2995345158897,30.5060820550798,-46.5435958333334));
#252724=CARTESIAN_POINT('Ctrl Pts',(46.8967285350793,31.5404524382925,-46.4852625));
#252725=CARTESIAN_POINT('Ctrl Pts',(46.2995345158897,32.5748228215052,-46.4269291666667));
#252726=CARTESIAN_POINT('Ctrl Pts',(45.7023404967,33.6091932047179,-46.3685958333333));
#252727=CARTESIAN_POINT('Ctrl Pts',(44.5079524583208,33.6091932047179,-46.3102625));
#252728=CARTESIAN_POINT('Ctrl Pts',(43.3135644199415,33.6091932047179,-46.2519291666667));
#252729=CARTESIAN_POINT('Ctrl Pts',(42.7163704007519,32.5748228215052,-46.1935958333333));
#252730=CARTESIAN_POINT('Ctrl Pts',(42.1191763815623,31.5404524382925,-46.1352625));
#252731=CARTESIAN_POINT('Ctrl Pts',(42.7163704007519,30.5060820550798,-46.0769291666667));
#252732=CARTESIAN_POINT('Ctrl Pts',(43.3135644199415,29.4717116718671,-46.0185958333334));
#252733=CARTESIAN_POINT('Ctrl Pts',(44.5079524583208,29.4717116718671,-45.9602625));
#252734=CARTESIAN_POINT('Ctrl Pts',(45.7023404967,29.4717116718671,-45.9019291666667));
#252735=CARTESIAN_POINT('Ctrl Pts',(46.2995345158897,30.5060820550798,-45.8435958333333));
#252736=CARTESIAN_POINT('Ctrl Pts',(46.8967285350793,31.5404524382925,-45.7852625));
#252737=CARTESIAN_POINT('Ctrl Pts',(46.2995345158897,32.5748228215052,-45.7269291666667));
#252738=CARTESIAN_POINT('Ctrl Pts',(45.7023404967,33.6091932047179,-45.6685958333334));
#252739=CARTESIAN_POINT('Ctrl Pts',(44.5079524583208,33.6091932047179,-45.6102625));
#252740=CARTESIAN_POINT('Ctrl Pts',(43.3135644199415,33.6091932047179,-45.5519291666667));
#252741=CARTESIAN_POINT('Ctrl Pts',(42.7163704007519,32.5748228215052,-45.4935958333333));
#252742=CARTESIAN_POINT('Ctrl Pts',(42.1191763815623,31.5404524382925,-45.4352625));
#252743=CARTESIAN_POINT('Ctrl Pts',(42.7163704007519,30.5060820550798,-45.3769291666667));
#252744=CARTESIAN_POINT('Ctrl Pts',(43.3135644199415,29.4717116718671,-45.3185958333333));
#252745=CARTESIAN_POINT('Ctrl Pts',(44.5079524583208,29.4717116718671,-45.2602625));
#252746=CARTESIAN_POINT('Ctrl Pts',(45.7023404967,29.4717116718671,-45.2019291666667));
#252747=CARTESIAN_POINT('Ctrl Pts',(46.2995345158897,30.5060820550798,-45.1435958333333));
#252748=CARTESIAN_POINT('Ctrl Pts',(46.8967285350793,31.5404524382925,-45.0852625));
#252749=CARTESIAN_POINT('Ctrl Pts',(46.2995345158897,32.5748228215052,-45.0269291666667));
#252750=CARTESIAN_POINT('Ctrl Pts',(45.7023404967,33.6091932047179,-44.9685958333334));
#252751=CARTESIAN_POINT('Ctrl Pts',(44.5079524583208,33.6091932047179,-44.9102625));
#252752=CARTESIAN_POINT('Ctrl Pts',(43.3135644199415,33.6091932047179,-44.8519291666667));
#252753=CARTESIAN_POINT('Ctrl Pts',(42.7163704007519,32.5748228215052,-44.7935958333333));
#252754=CARTESIAN_POINT('Ctrl Pts',(42.1191763815623,31.5404524382925,-44.7352625));
#252755=CARTESIAN_POINT('Ctrl Pts',(42.7163704007519,30.5060820550798,-44.6769291666667));
#252756=CARTESIAN_POINT('Ctrl Pts',(43.3135644199415,29.4717116718671,-44.6185958333334));
#252757=CARTESIAN_POINT('Ctrl Pts',(44.5079524583208,29.4717116718671,-44.5602625));
#252758=CARTESIAN_POINT('Ctrl Pts',(45.7023404967,29.4717116718671,-44.5019291666667));
#252759=CARTESIAN_POINT('Ctrl Pts',(46.2995345158897,30.5060820550798,-44.4435958333333));
#252760=CARTESIAN_POINT('Ctrl Pts',(46.8967285350793,31.5404524382925,-44.3852625));
#252761=CARTESIAN_POINT('Ctrl Pts',(46.2995345158897,32.5748228215052,-44.3269291666667));
#252762=CARTESIAN_POINT('Ctrl Pts',(45.7023404967,33.6091932047179,-44.2685958333334));
#252763=CARTESIAN_POINT('Ctrl Pts',(44.5079524583208,33.6091932047179,-44.2102625));
#252764=CARTESIAN_POINT('Ctrl Pts',(43.3135644199415,33.6091932047179,-44.1519291666667));
#252765=CARTESIAN_POINT('Ctrl Pts',(42.7163704007519,32.5748228215052,-44.0935958333334));
#252766=CARTESIAN_POINT('Ctrl Pts',(42.1191763815623,31.5404524382925,-44.0352625));
#252767=CARTESIAN_POINT('Ctrl Pts',(42.7163704007519,30.5060820550798,-43.9769291666667));
#252768=CARTESIAN_POINT('Ctrl Pts',(43.3135644199415,29.4717116718671,-43.9185958333333));
#252769=CARTESIAN_POINT('Ctrl Pts',(44.5079524583208,29.4717116718671,-43.8602625));
#252770=CARTESIAN_POINT('Ctrl Pts',(45.7023404967,29.4717116718671,-43.8019291666667));
#252771=CARTESIAN_POINT('Ctrl Pts',(46.2995345158897,30.5060820550798,-43.7435958333334));
#252772=CARTESIAN_POINT('Ctrl Pts',(46.8967285350793,31.5404524382925,-43.6852625));
#252773=CARTESIAN_POINT('Ctrl Pts',(46.2995345158897,32.5748228215052,-43.6269291666667));
#252774=CARTESIAN_POINT('Ctrl Pts',(45.7023404967,33.6091932047179,-43.5685958333333));
#252775=CARTESIAN_POINT('Ctrl Pts',(44.5079524583208,33.6091932047179,-43.5102625));
#252776=CARTESIAN_POINT('Ctrl Pts',(43.3135644199415,33.6091932047179,-43.4519291666667));
#252777=CARTESIAN_POINT('Ctrl Pts',(42.7163704007519,32.5748228215052,-43.3935958333334));
#252778=CARTESIAN_POINT('Ctrl Pts',(42.1191763815623,31.5404524382925,-43.3352625));
#252779=CARTESIAN_POINT('Ctrl Pts',(42.7163704007519,30.5060820550798,-43.2769291666667));
#252780=CARTESIAN_POINT('Ctrl Pts',(43.3135644199415,29.4717116718671,-43.2185958333333));
#252781=CARTESIAN_POINT('Ctrl Pts',(44.5079524583208,29.4717116718671,-43.1602625));
#252782=CARTESIAN_POINT('Ctrl Pts',(45.7023404967,29.4717116718671,-43.1019291666667));
#252783=CARTESIAN_POINT('Ctrl Pts',(46.2995345158897,30.5060820550798,-43.0435958333334));
#252784=CARTESIAN_POINT('Ctrl Pts',(46.8967285350793,31.5404524382925,-42.9852625));
#252785=CARTESIAN_POINT('Ctrl Pts',(46.2995345158897,32.5748228215052,-42.9269291666667));
#252786=CARTESIAN_POINT('Ctrl Pts',(45.7023404967,33.6091932047179,-42.8685958333333));
#252787=CARTESIAN_POINT('Ctrl Pts',(44.5079524583208,33.6091932047179,-42.8102625));
#252788=CARTESIAN_POINT('Ctrl Pts',(43.3135644199415,33.6091932047179,-42.7519291666666));
#252789=CARTESIAN_POINT('Ctrl Pts',(42.7163704007519,32.5748228215052,-42.6935958333333));
#252790=CARTESIAN_POINT('Ctrl Pts',(42.1191763815623,31.5404524382925,-42.6352625));
#252791=CARTESIAN_POINT('Ctrl Pts',(42.7163704007519,30.5060820550798,-42.5769291666667));
#252792=CARTESIAN_POINT('Ctrl Pts',(43.3135644199415,29.4717116718671,-42.5185958333333));
#252793=CARTESIAN_POINT('Ctrl Pts',(44.5079524583208,29.4717116718671,-42.4602625));
#252794=CARTESIAN_POINT('Ctrl Pts',(45.7023404967,29.4717116718671,-42.4019291666666));
#252795=CARTESIAN_POINT('Ctrl Pts',(46.2995345158897,30.5060820550798,-42.3435958333334));
#252796=CARTESIAN_POINT('Ctrl Pts',(46.8967285350793,31.5404524382925,-42.2852625));
#252797=CARTESIAN_POINT('Ctrl Pts',(46.2995345158897,32.5748228215052,-42.2269291666667));
#252798=CARTESIAN_POINT('Ctrl Pts',(45.7023404967,33.6091932047179,-42.1685958333333));
#252799=CARTESIAN_POINT('Ctrl Pts',(44.5079524583208,33.6091932047179,-42.1102625));
#252800=CARTESIAN_POINT('Ctrl Pts',(43.3135644199415,33.6091932047179,-42.0519291666666));
#252801=CARTESIAN_POINT('Ctrl Pts',(42.7163704007519,32.5748228215052,-41.9935958333334));
#252802=CARTESIAN_POINT('Ctrl Pts',(42.1191763815623,31.5404524382925,-41.9352625));
#252803=CARTESIAN_POINT('Ctrl Pts',(42.7163704007519,30.5060820550798,-41.8769291666667));
#252804=CARTESIAN_POINT('Ctrl Pts',(43.3135644199415,29.4717116718671,-41.8185958333333));
#252805=CARTESIAN_POINT('Ctrl Pts',(44.5079524583208,29.4717116718671,-41.7602625));
#252806=CARTESIAN_POINT('Ctrl Pts',(45.7023404967,29.4717116718671,-41.7019291666666));
#252807=CARTESIAN_POINT('Ctrl Pts',(46.2995345158897,30.5060820550798,-41.6435958333334));
#252808=CARTESIAN_POINT('Ctrl Pts',(46.8967285350793,31.5404524382925,-41.5852625));
#252809=CARTESIAN_POINT('Ctrl Pts',(46.2995345158897,32.5748228215052,-41.5269291666667));
#252810=CARTESIAN_POINT('Ctrl Pts',(45.7023404967,33.6091932047179,-41.4685958333333));
#252811=CARTESIAN_POINT('Ctrl Pts',(44.5079524583208,33.6091932047179,-41.4102625));
#252812=CARTESIAN_POINT('Ctrl Pts',(43.3135644199415,33.6091932047179,-41.3519291666666));
#252813=CARTESIAN_POINT('Ctrl Pts',(42.7163704007519,32.5748228215052,-41.2935958333334));
#252814=CARTESIAN_POINT('Ctrl Pts',(42.1191763815623,31.5404524382925,-41.2352625));
#252815=CARTESIAN_POINT('Ctrl Pts',(42.7163704007519,30.5060820550798,-41.1769291666667));
#252816=CARTESIAN_POINT('Ctrl Pts',(43.3135644199415,29.4717116718671,-41.1185958333333));
#252817=CARTESIAN_POINT('Ctrl Pts',(44.5079524583208,29.4717116718671,-41.0602625));
#252818=CARTESIAN_POINT('Ctrl Pts',(45.7023404967,29.4717116718671,-41.0019291666666));
#252819=CARTESIAN_POINT('Ctrl Pts',(46.2995345158897,30.5060820550798,-40.9435958333334));
#252820=CARTESIAN_POINT('Ctrl Pts',(46.8967285350793,31.5404524382925,-40.8852625));
#252821=CARTESIAN_POINT('Ctrl Pts',(46.2995345158897,32.5748228215052,-40.8269291666667));
#252822=CARTESIAN_POINT('Ctrl Pts',(45.7023404967,33.6091932047179,-40.7685958333333));
#252823=CARTESIAN_POINT('Ctrl Pts',(44.5079524583208,33.6091932047179,-40.7102625));
#252824=CARTESIAN_POINT('Ctrl Pts',(43.3135644199415,33.6091932047179,-40.6519291666667));
#252825=CARTESIAN_POINT('Ctrl Pts',(42.7163704007519,32.5748228215052,-40.5935958333334));
#252826=CARTESIAN_POINT('Ctrl Pts',(42.1191763815623,31.5404524382925,-40.5352625));
#252827=CARTESIAN_POINT('Ctrl Pts',(42.7163704007519,30.5060820550798,-40.4769291666667));
#252828=CARTESIAN_POINT('Ctrl Pts',(43.3135644199415,29.4717116718671,-40.4185958333333));
#252829=CARTESIAN_POINT('Ctrl Pts',(44.5079524583208,29.4717116718671,-40.3602625));
#252830=CARTESIAN_POINT('Ctrl Pts',(45.7023404967,29.4717116718671,-40.3019291666667));
#252831=CARTESIAN_POINT('Ctrl Pts',(46.2995345158897,30.5060820550798,-40.2435958333334));
#252832=CARTESIAN_POINT('Ctrl Pts',(46.8967285350793,31.5404524382925,-40.1852625));
#252833=CARTESIAN_POINT('Ctrl Pts',(46.2995345158897,32.5748228215052,-40.1269291666666));
#252834=CARTESIAN_POINT('Ctrl Pts',(45.7023404967,33.6091932047179,-40.0685958333333));
#252835=CARTESIAN_POINT('Ctrl Pts',(44.5079524583208,33.6091932047179,-40.0102625));
#252836=CARTESIAN_POINT('Ctrl Pts',(43.3135644199415,33.6091932047179,-39.9519291666667));
#252837=CARTESIAN_POINT('Ctrl Pts',(42.7163704007519,32.5748228215052,-39.8935958333334));
#252838=CARTESIAN_POINT('Ctrl Pts',(42.1191763815623,31.5404524382925,-39.8352625));
#252839=CARTESIAN_POINT('Ctrl Pts',(42.7163704007519,30.5060820550798,-39.7769291666666));
#252840=CARTESIAN_POINT('Ctrl Pts',(43.3135644199415,29.4717116718671,-39.7185958333334));
#252841=CARTESIAN_POINT('Ctrl Pts',(44.5079524583208,29.4717116718671,-39.6602625));
#252842=CARTESIAN_POINT('Ctrl Pts',(45.7023404967,29.4717116718671,-39.6019291666667));
#252843=CARTESIAN_POINT('Ctrl Pts',(46.2995345158897,30.5060820550798,-39.5435958333333));
#252844=CARTESIAN_POINT('Ctrl Pts',(46.8967285350793,31.5404524382925,-39.4852625));
#252845=CARTESIAN_POINT('Ctrl Pts',(46.2995345158897,32.5748228215052,-39.4269291666667));
#252846=CARTESIAN_POINT('Ctrl Pts',(45.7023404967,33.6091932047179,-39.3685958333334));
#252847=CARTESIAN_POINT('Ctrl Pts',(44.5079524583208,33.6091932047179,-39.3102625));
#252848=CARTESIAN_POINT('Ctrl Pts',(43.3135644199415,33.6091932047179,-39.2519291666667));
#252849=CARTESIAN_POINT('Ctrl Pts',(42.7163704007519,32.5748228215052,-39.1935958333334));
#252850=CARTESIAN_POINT('Ctrl Pts',(42.1191763815623,31.5404524382925,-39.1352625));
#252851=CARTESIAN_POINT('Ctrl Pts',(42.7163704007519,30.5060820550798,-39.0769291666667));
#252852=CARTESIAN_POINT('Ctrl Pts',(43.3135644199415,29.4717116718671,-39.0185958333333));
#252853=CARTESIAN_POINT('Ctrl Pts',(44.5079524583208,29.4717116718671,-38.9602625));
#252854=CARTESIAN_POINT('Ctrl Pts',(45.7023404967,29.4717116718671,-38.9019291666667));
#252855=CARTESIAN_POINT('Ctrl Pts',(46.2995345158897,30.5060820550798,-38.8435958333333));
#252856=CARTESIAN_POINT('Ctrl Pts',(46.8967285350793,31.5404524382925,-38.7852625));
#252857=CARTESIAN_POINT('Ctrl Pts',(46.2995345158897,32.5748228215052,-38.7269291666667));
#252858=CARTESIAN_POINT('Ctrl Pts',(45.7023404967,33.6091932047179,-38.6685958333334));
#252859=CARTESIAN_POINT('Ctrl Pts',(44.5079524583208,33.6091932047179,-38.6102625));
#252860=CARTESIAN_POINT('Ctrl Pts',(43.3135644199415,33.6091932047179,-38.5519291666667));
#252861=CARTESIAN_POINT('Ctrl Pts',(42.7163704007519,32.5748228215052,-38.4935958333334));
#252862=CARTESIAN_POINT('Ctrl Pts',(42.1191763815623,31.5404524382925,-38.4352625));
#252863=CARTESIAN_POINT('Ctrl Pts',(42.7163704007519,30.5060820550798,-38.3769291666666));
#252864=CARTESIAN_POINT('Ctrl Pts',(43.3135644199415,29.4717116718671,-38.3185958333333));
#252865=CARTESIAN_POINT('Ctrl Pts',(44.5079524583208,29.4717116718671,-38.2602625));
#252866=CARTESIAN_POINT('Ctrl Pts',(45.7023404967,29.4717116718671,-38.2019291666667));
#252867=CARTESIAN_POINT('Ctrl Pts',(46.2995345158897,30.5060820550798,-38.1435958333334));
#252868=CARTESIAN_POINT('Ctrl Pts',(46.8967285350793,31.5404524382925,-38.0852625));
#252869=CARTESIAN_POINT('Ctrl Pts',(46.2995345158897,32.5748228215052,-38.0269291666667));
#252870=CARTESIAN_POINT('Ctrl Pts',(45.7023404967,33.6091932047179,-37.9685958333333));
#252871=CARTESIAN_POINT('Ctrl Pts',(44.5079524583208,33.6091932047179,-37.9102625));
#252872=CARTESIAN_POINT('Ctrl Pts',(43.3135644199415,33.6091932047179,-37.8519291666667));
#252873=CARTESIAN_POINT('Ctrl Pts',(42.7163704007519,32.5748228215052,-37.7935958333334));
#252874=CARTESIAN_POINT('Ctrl Pts',(42.1191763815623,31.5404524382925,-37.7352625));
#252875=CARTESIAN_POINT('Ctrl Pts',(42.7163704007519,30.5060820550798,-37.6769291666667));
#252876=CARTESIAN_POINT('Ctrl Pts',(43.3135644199415,29.4717116718671,-37.6185958333333));
#252877=CARTESIAN_POINT('Ctrl Pts',(44.5079524583208,29.4717116718671,-37.5602625));
#252878=CARTESIAN_POINT('Ctrl Pts',(45.7023404967,29.4717116718671,-37.5019291666666));
#252879=CARTESIAN_POINT('Ctrl Pts',(46.2995345158897,30.5060820550798,-37.4435958333333));
#252880=CARTESIAN_POINT('Ctrl Pts',(46.8967285350793,31.5404524382925,-37.3852625));
#252881=CARTESIAN_POINT('Ctrl Pts',(46.2995345158897,32.5748228215052,-37.3269291666667));
#252882=CARTESIAN_POINT('Ctrl Pts',(45.7023404967,33.6091932047179,-37.2685958333333));
#252883=CARTESIAN_POINT('Ctrl Pts',(44.5079524583208,33.6091932047179,-37.2102625));
#252884=CARTESIAN_POINT('Ctrl Pts',(43.3135644199415,33.6091932047179,-37.1519291666667));
#252885=CARTESIAN_POINT('Ctrl Pts',(42.7163704007519,32.5748228215052,-37.0935958333333));
#252886=CARTESIAN_POINT('Ctrl Pts',(42.1191763815623,31.5404524382925,-37.0352625));
#252887=CARTESIAN_POINT('Ctrl Pts',(42.7163704007519,30.5060820550798,-36.9769291666667));
#252888=CARTESIAN_POINT('Ctrl Pts',(43.3135644199415,29.4717116718671,-36.9185958333333));
#252889=CARTESIAN_POINT('Ctrl Pts',(44.5079524583208,29.4717116718671,-36.8602625));
#252890=CARTESIAN_POINT('Ctrl Pts',(45.7023404967,29.4717116718671,-36.8019291666666));
#252891=CARTESIAN_POINT('Ctrl Pts',(46.2995345158897,30.5060820550798,-36.7435958333334));
#252892=CARTESIAN_POINT('Ctrl Pts',(46.8967285350793,31.5404524382925,-36.6852625));
#252893=CARTESIAN_POINT('Ctrl Pts',(46.2995345158897,32.5748228215052,-36.6269291666666));
#252894=CARTESIAN_POINT('Ctrl Pts',(46.222006582932,32.7091051403937,-36.6193563132714));
#252895=CARTESIAN_POINT('Ctrl Pts',(46.1253278975281,32.8303303578336,-36.611216324118));
#252896=CARTESIAN_POINT('Ctrl Pts',(44.5079524583208,33.2091975287062,-52.84120011122));
#252897=CARTESIAN_POINT('Ctrl Pts',(43.5445020311616,33.2091975287062,-52.7828667778867));
#252898=CARTESIAN_POINT('Ctrl Pts',(43.0627768175819,32.3748249834993,-52.7245334445534));
#252899=CARTESIAN_POINT('Ctrl Pts',(42.5810516040023,31.5404524382925,-52.66620011122));
#252900=CARTESIAN_POINT('Ctrl Pts',(43.0627768175819,30.7060798930856,-52.6078667778867));
#252901=CARTESIAN_POINT('Ctrl Pts',(43.5445020311616,29.8717073478788,-52.5495334445533));
#252902=CARTESIAN_POINT('Ctrl Pts',(44.5079524583208,29.8717073478787,-52.49120011122));
#252903=CARTESIAN_POINT('Ctrl Pts',(45.47140288548,29.8717073478788,-52.4328667778868));
#252904=CARTESIAN_POINT('Ctrl Pts',(45.9531280990597,30.7060798930856,-52.3745334445534));
#252905=CARTESIAN_POINT('Ctrl Pts',(46.4348533126392,31.5404524382925,-52.3162001112201));
#252906=CARTESIAN_POINT('Ctrl Pts',(45.9531280990597,32.3748249834993,-52.2578667778867));
#252907=CARTESIAN_POINT('Ctrl Pts',(45.47140288548,33.2091975287062,-52.1995334445534));
#252908=CARTESIAN_POINT('Ctrl Pts',(44.5079524583208,33.2091975287062,-52.14120011122));
#252909=CARTESIAN_POINT('Ctrl Pts',(43.5445020311616,33.2091975287062,-52.0828667778867));
#252910=CARTESIAN_POINT('Ctrl Pts',(43.0627768175819,32.3748249834993,-52.0245334445533));
#252911=CARTESIAN_POINT('Ctrl Pts',(42.5810516040023,31.5404524382925,-51.96620011122));
#252912=CARTESIAN_POINT('Ctrl Pts',(43.0627768175819,30.7060798930856,-51.9078667778867));
#252913=CARTESIAN_POINT('Ctrl Pts',(43.5445020311616,29.8717073478788,-51.8495334445534));
#252914=CARTESIAN_POINT('Ctrl Pts',(44.5079524583208,29.8717073478787,-51.79120011122));
#252915=CARTESIAN_POINT('Ctrl Pts',(45.47140288548,29.8717073478788,-51.7328667778867));
#252916=CARTESIAN_POINT('Ctrl Pts',(45.9531280990597,30.7060798930856,-51.6745334445533));
#252917=CARTESIAN_POINT('Ctrl Pts',(46.4348533126392,31.5404524382925,-51.61620011122));
#252918=CARTESIAN_POINT('Ctrl Pts',(45.9531280990597,32.3748249834993,-51.5578667778867));
#252919=CARTESIAN_POINT('Ctrl Pts',(45.47140288548,33.2091975287062,-51.4995334445534));
#252920=CARTESIAN_POINT('Ctrl Pts',(44.5079524583208,33.2091975287062,-51.44120011122));
#252921=CARTESIAN_POINT('Ctrl Pts',(43.5445020311616,33.2091975287062,-51.3828667778867));
#252922=CARTESIAN_POINT('Ctrl Pts',(43.0627768175819,32.3748249834993,-51.3245334445534));
#252923=CARTESIAN_POINT('Ctrl Pts',(42.5810516040023,31.5404524382925,-51.26620011122));
#252924=CARTESIAN_POINT('Ctrl Pts',(43.0627768175819,30.7060798930856,-51.2078667778867));
#252925=CARTESIAN_POINT('Ctrl Pts',(43.5445020311616,29.8717073478788,-51.1495334445534));
#252926=CARTESIAN_POINT('Ctrl Pts',(44.5079524583208,29.8717073478787,-51.09120011122));
#252927=CARTESIAN_POINT('Ctrl Pts',(45.47140288548,29.8717073478788,-51.0328667778867));
#252928=CARTESIAN_POINT('Ctrl Pts',(45.9531280990597,30.7060798930856,-50.9745334445533));
#252929=CARTESIAN_POINT('Ctrl Pts',(46.4348533126392,31.5404524382925,-50.91620011122));
#252930=CARTESIAN_POINT('Ctrl Pts',(45.9531280990597,32.3748249834993,-50.8578667778867));
#252931=CARTESIAN_POINT('Ctrl Pts',(45.47140288548,33.2091975287062,-50.7995334445533));
#252932=CARTESIAN_POINT('Ctrl Pts',(44.5079524583208,33.2091975287062,-50.74120011122));
#252933=CARTESIAN_POINT('Ctrl Pts',(43.5445020311616,33.2091975287062,-50.6828667778867));
#252934=CARTESIAN_POINT('Ctrl Pts',(43.0627768175819,32.3748249834993,-50.6245334445533));
#252935=CARTESIAN_POINT('Ctrl Pts',(42.5810516040023,31.5404524382925,-50.56620011122));
#252936=CARTESIAN_POINT('Ctrl Pts',(43.0627768175819,30.7060798930856,-50.5078667778867));
#252937=CARTESIAN_POINT('Ctrl Pts',(43.5445020311616,29.8717073478788,-50.4495334445534));
#252938=CARTESIAN_POINT('Ctrl Pts',(44.5079524583208,29.8717073478787,-50.39120011122));
#252939=CARTESIAN_POINT('Ctrl Pts',(45.47140288548,29.8717073478788,-50.3328667778867));
#252940=CARTESIAN_POINT('Ctrl Pts',(45.9531280990597,30.7060798930856,-50.2745334445533));
#252941=CARTESIAN_POINT('Ctrl Pts',(46.4348533126392,31.5404524382925,-50.21620011122));
#252942=CARTESIAN_POINT('Ctrl Pts',(45.9531280990597,32.3748249834993,-50.1578667778867));
#252943=CARTESIAN_POINT('Ctrl Pts',(45.47140288548,33.2091975287062,-50.0995334445534));
#252944=CARTESIAN_POINT('Ctrl Pts',(44.5079524583208,33.2091975287062,-50.04120011122));
#252945=CARTESIAN_POINT('Ctrl Pts',(43.5445020311616,33.2091975287062,-49.9828667778867));
#252946=CARTESIAN_POINT('Ctrl Pts',(43.0627768175819,32.3748249834993,-49.9245334445534));
#252947=CARTESIAN_POINT('Ctrl Pts',(42.5810516040023,31.5404524382925,-49.8662001112201));
#252948=CARTESIAN_POINT('Ctrl Pts',(43.0627768175819,30.7060798930856,-49.8078667778867));
#252949=CARTESIAN_POINT('Ctrl Pts',(43.5445020311616,29.8717073478788,-49.7495334445534));
#252950=CARTESIAN_POINT('Ctrl Pts',(44.5079524583208,29.8717073478787,-49.69120011122));
#252951=CARTESIAN_POINT('Ctrl Pts',(45.47140288548,29.8717073478788,-49.6328667778867));
#252952=CARTESIAN_POINT('Ctrl Pts',(45.9531280990597,30.7060798930856,-49.5745334445533));
#252953=CARTESIAN_POINT('Ctrl Pts',(46.4348533126392,31.5404524382925,-49.51620011122));
#252954=CARTESIAN_POINT('Ctrl Pts',(45.9531280990597,32.3748249834993,-49.4578667778867));
#252955=CARTESIAN_POINT('Ctrl Pts',(45.47140288548,33.2091975287062,-49.3995334445534));
#252956=CARTESIAN_POINT('Ctrl Pts',(44.5079524583208,33.2091975287062,-49.34120011122));
#252957=CARTESIAN_POINT('Ctrl Pts',(43.5445020311616,33.2091975287062,-49.2828667778867));
#252958=CARTESIAN_POINT('Ctrl Pts',(43.0627768175819,32.3748249834993,-49.2245334445533));
#252959=CARTESIAN_POINT('Ctrl Pts',(42.5810516040023,31.5404524382925,-49.16620011122));
#252960=CARTESIAN_POINT('Ctrl Pts',(43.0627768175819,30.7060798930856,-49.1078667778867));
#252961=CARTESIAN_POINT('Ctrl Pts',(43.5445020311616,29.8717073478788,-49.0495334445534));
#252962=CARTESIAN_POINT('Ctrl Pts',(44.5079524583208,29.8717073478787,-48.99120011122));
#252963=CARTESIAN_POINT('Ctrl Pts',(45.47140288548,29.8717073478788,-48.9328667778867));
#252964=CARTESIAN_POINT('Ctrl Pts',(45.9531280990597,30.7060798930856,-48.8745334445533));
#252965=CARTESIAN_POINT('Ctrl Pts',(46.4348533126392,31.5404524382925,-48.81620011122));
#252966=CARTESIAN_POINT('Ctrl Pts',(45.9531280990597,32.3748249834993,-48.7578667778867));
#252967=CARTESIAN_POINT('Ctrl Pts',(45.47140288548,33.2091975287062,-48.6995334445534));
#252968=CARTESIAN_POINT('Ctrl Pts',(44.5079524583208,33.2091975287062,-48.64120011122));
#252969=CARTESIAN_POINT('Ctrl Pts',(43.5445020311616,33.2091975287062,-48.5828667778867));
#252970=CARTESIAN_POINT('Ctrl Pts',(43.0627768175819,32.3748249834993,-48.5245334445533));
#252971=CARTESIAN_POINT('Ctrl Pts',(42.5810516040023,31.5404524382925,-48.46620011122));
#252972=CARTESIAN_POINT('Ctrl Pts',(43.0627768175819,30.7060798930856,-48.4078667778867));
#252973=CARTESIAN_POINT('Ctrl Pts',(43.5445020311616,29.8717073478788,-48.3495334445534));
#252974=CARTESIAN_POINT('Ctrl Pts',(44.5079524583208,29.8717073478787,-48.29120011122));
#252975=CARTESIAN_POINT('Ctrl Pts',(45.47140288548,29.8717073478788,-48.2328667778867));
#252976=CARTESIAN_POINT('Ctrl Pts',(45.9531280990597,30.7060798930856,-48.1745334445534));
#252977=CARTESIAN_POINT('Ctrl Pts',(46.4348533126392,31.5404524382925,-48.11620011122));
#252978=CARTESIAN_POINT('Ctrl Pts',(45.9531280990597,32.3748249834993,-48.0578667778867));
#252979=CARTESIAN_POINT('Ctrl Pts',(45.47140288548,33.2091975287062,-47.9995334445534));
#252980=CARTESIAN_POINT('Ctrl Pts',(44.5079524583208,33.2091975287062,-47.94120011122));
#252981=CARTESIAN_POINT('Ctrl Pts',(43.5445020311616,33.2091975287062,-47.8828667778867));
#252982=CARTESIAN_POINT('Ctrl Pts',(43.0627768175819,32.3748249834993,-47.8245334445533));
#252983=CARTESIAN_POINT('Ctrl Pts',(42.5810516040023,31.5404524382925,-47.76620011122));
#252984=CARTESIAN_POINT('Ctrl Pts',(43.0627768175819,30.7060798930856,-47.7078667778867));
#252985=CARTESIAN_POINT('Ctrl Pts',(43.5445020311616,29.8717073478788,-47.6495334445534));
#252986=CARTESIAN_POINT('Ctrl Pts',(44.5079524583208,29.8717073478787,-47.59120011122));
#252987=CARTESIAN_POINT('Ctrl Pts',(45.47140288548,29.8717073478788,-47.5328667778867));
#252988=CARTESIAN_POINT('Ctrl Pts',(45.9531280990597,30.7060798930856,-47.4745334445534));
#252989=CARTESIAN_POINT('Ctrl Pts',(46.4348533126392,31.5404524382925,-47.41620011122));
#252990=CARTESIAN_POINT('Ctrl Pts',(45.9531280990597,32.3748249834993,-47.3578667778867));
#252991=CARTESIAN_POINT('Ctrl Pts',(45.47140288548,33.2091975287062,-47.2995334445534));
#252992=CARTESIAN_POINT('Ctrl Pts',(44.5079524583208,33.2091975287062,-47.24120011122));
#252993=CARTESIAN_POINT('Ctrl Pts',(43.5445020311616,33.2091975287062,-47.1828667778867));
#252994=CARTESIAN_POINT('Ctrl Pts',(43.0627768175819,32.3748249834993,-47.1245334445533));
#252995=CARTESIAN_POINT('Ctrl Pts',(42.5810516040023,31.5404524382925,-47.06620011122));
#252996=CARTESIAN_POINT('Ctrl Pts',(43.0627768175819,30.7060798930856,-47.0078667778867));
#252997=CARTESIAN_POINT('Ctrl Pts',(43.5445020311616,29.8717073478788,-46.9495334445534));
#252998=CARTESIAN_POINT('Ctrl Pts',(44.5079524583208,29.8717073478787,-46.89120011122));
#252999=CARTESIAN_POINT('Ctrl Pts',(45.47140288548,29.8717073478788,-46.8328667778867));
#253000=CARTESIAN_POINT('Ctrl Pts',(45.9531280990597,30.7060798930856,-46.7745334445533));
#253001=CARTESIAN_POINT('Ctrl Pts',(46.4348533126392,31.5404524382925,-46.71620011122));
#253002=CARTESIAN_POINT('Ctrl Pts',(45.9531280990597,32.3748249834993,-46.6578667778867));
#253003=CARTESIAN_POINT('Ctrl Pts',(45.47140288548,33.2091975287062,-46.5995334445534));
#253004=CARTESIAN_POINT('Ctrl Pts',(44.5079524583208,33.2091975287062,-46.54120011122));
#253005=CARTESIAN_POINT('Ctrl Pts',(43.5445020311616,33.2091975287062,-46.4828667778867));
#253006=CARTESIAN_POINT('Ctrl Pts',(43.0627768175819,32.3748249834993,-46.4245334445533));
#253007=CARTESIAN_POINT('Ctrl Pts',(42.5810516040023,31.5404524382925,-46.36620011122));
#253008=CARTESIAN_POINT('Ctrl Pts',(43.0627768175819,30.7060798930856,-46.3078667778867));
#253009=CARTESIAN_POINT('Ctrl Pts',(43.5445020311616,29.8717073478788,-46.2495334445534));
#253010=CARTESIAN_POINT('Ctrl Pts',(44.5079524583208,29.8717073478787,-46.19120011122));
#253011=CARTESIAN_POINT('Ctrl Pts',(45.47140288548,29.8717073478788,-46.1328667778867));
#253012=CARTESIAN_POINT('Ctrl Pts',(45.9531280990597,30.7060798930856,-46.0745334445534));
#253013=CARTESIAN_POINT('Ctrl Pts',(46.4348533126392,31.5404524382925,-46.01620011122));
#253014=CARTESIAN_POINT('Ctrl Pts',(45.9531280990597,32.3748249834993,-45.9578667778867));
#253015=CARTESIAN_POINT('Ctrl Pts',(45.47140288548,33.2091975287062,-45.8995334445533));
#253016=CARTESIAN_POINT('Ctrl Pts',(44.5079524583208,33.2091975287062,-45.84120011122));
#253017=CARTESIAN_POINT('Ctrl Pts',(43.5445020311616,33.2091975287062,-45.7828667778867));
#253018=CARTESIAN_POINT('Ctrl Pts',(43.0627768175819,32.3748249834993,-45.7245334445533));
#253019=CARTESIAN_POINT('Ctrl Pts',(42.5810516040023,31.5404524382925,-45.66620011122));
#253020=CARTESIAN_POINT('Ctrl Pts',(43.0627768175819,30.7060798930856,-45.6078667778867));
#253021=CARTESIAN_POINT('Ctrl Pts',(43.5445020311616,29.8717073478788,-45.5495334445534));
#253022=CARTESIAN_POINT('Ctrl Pts',(44.5079524583208,29.8717073478787,-45.49120011122));
#253023=CARTESIAN_POINT('Ctrl Pts',(45.47140288548,29.8717073478788,-45.4328667778867));
#253024=CARTESIAN_POINT('Ctrl Pts',(45.9531280990597,30.7060798930856,-45.3745334445533));
#253025=CARTESIAN_POINT('Ctrl Pts',(46.4348533126392,31.5404524382925,-45.31620011122));
#253026=CARTESIAN_POINT('Ctrl Pts',(45.9531280990597,32.3748249834993,-45.2578667778867));
#253027=CARTESIAN_POINT('Ctrl Pts',(45.47140288548,33.2091975287062,-45.1995334445534));
#253028=CARTESIAN_POINT('Ctrl Pts',(44.5079524583208,33.2091975287062,-45.14120011122));
#253029=CARTESIAN_POINT('Ctrl Pts',(43.5445020311616,33.2091975287062,-45.0828667778867));
#253030=CARTESIAN_POINT('Ctrl Pts',(43.0627768175819,32.3748249834993,-45.0245334445533));
#253031=CARTESIAN_POINT('Ctrl Pts',(42.5810516040023,31.5404524382925,-44.9662001112201));
#253032=CARTESIAN_POINT('Ctrl Pts',(43.0627768175819,30.7060798930856,-44.9078667778867));
#253033=CARTESIAN_POINT('Ctrl Pts',(43.5445020311616,29.8717073478788,-44.8495334445534));
#253034=CARTESIAN_POINT('Ctrl Pts',(44.5079524583208,29.8717073478787,-44.79120011122));
#253035=CARTESIAN_POINT('Ctrl Pts',(45.47140288548,29.8717073478788,-44.7328667778867));
#253036=CARTESIAN_POINT('Ctrl Pts',(45.9531280990597,30.7060798930856,-44.6745334445534));
#253037=CARTESIAN_POINT('Ctrl Pts',(46.4348533126392,31.5404524382925,-44.6162001112201));
#253038=CARTESIAN_POINT('Ctrl Pts',(45.9531280990597,32.3748249834993,-44.5578667778867));
#253039=CARTESIAN_POINT('Ctrl Pts',(45.47140288548,33.2091975287062,-44.4995334445534));
#253040=CARTESIAN_POINT('Ctrl Pts',(44.5079524583208,33.2091975287062,-44.44120011122));
#253041=CARTESIAN_POINT('Ctrl Pts',(43.5445020311616,33.2091975287062,-44.3828667778867));
#253042=CARTESIAN_POINT('Ctrl Pts',(43.0627768175819,32.3748249834993,-44.3245334445534));
#253043=CARTESIAN_POINT('Ctrl Pts',(42.5810516040023,31.5404524382925,-44.26620011122));
#253044=CARTESIAN_POINT('Ctrl Pts',(43.0627768175819,30.7060798930856,-44.2078667778867));
#253045=CARTESIAN_POINT('Ctrl Pts',(43.5445020311616,29.8717073478788,-44.1495334445534));
#253046=CARTESIAN_POINT('Ctrl Pts',(44.5079524583208,29.8717073478787,-44.09120011122));
#253047=CARTESIAN_POINT('Ctrl Pts',(45.47140288548,29.8717073478788,-44.0328667778867));
#253048=CARTESIAN_POINT('Ctrl Pts',(45.9531280990597,30.7060798930856,-43.9745334445534));
#253049=CARTESIAN_POINT('Ctrl Pts',(46.4348533126392,31.5404524382925,-43.9162001112201));
#253050=CARTESIAN_POINT('Ctrl Pts',(45.9531280990597,32.3748249834993,-43.8578667778867));
#253051=CARTESIAN_POINT('Ctrl Pts',(45.47140288548,33.2091975287062,-43.7995334445534));
#253052=CARTESIAN_POINT('Ctrl Pts',(44.5079524583208,33.2091975287062,-43.74120011122));
#253053=CARTESIAN_POINT('Ctrl Pts',(43.5445020311616,33.2091975287062,-43.6828667778867));
#253054=CARTESIAN_POINT('Ctrl Pts',(43.0627768175819,32.3748249834993,-43.6245334445534));
#253055=CARTESIAN_POINT('Ctrl Pts',(42.5810516040023,31.5404524382925,-43.5662001112201));
#253056=CARTESIAN_POINT('Ctrl Pts',(43.0627768175819,30.7060798930856,-43.5078667778867));
#253057=CARTESIAN_POINT('Ctrl Pts',(43.5445020311616,29.8717073478788,-43.4495334445534));
#253058=CARTESIAN_POINT('Ctrl Pts',(44.5079524583208,29.8717073478787,-43.39120011122));
#253059=CARTESIAN_POINT('Ctrl Pts',(45.47140288548,29.8717073478788,-43.3328667778867));
#253060=CARTESIAN_POINT('Ctrl Pts',(45.9531280990597,30.7060798930856,-43.2745334445534));
#253061=CARTESIAN_POINT('Ctrl Pts',(46.4348533126392,31.5404524382925,-43.21620011122));
#253062=CARTESIAN_POINT('Ctrl Pts',(45.9531280990597,32.3748249834993,-43.1578667778867));
#253063=CARTESIAN_POINT('Ctrl Pts',(45.47140288548,33.2091975287062,-43.0995334445534));
#253064=CARTESIAN_POINT('Ctrl Pts',(44.5079524583208,33.2091975287062,-43.04120011122));
#253065=CARTESIAN_POINT('Ctrl Pts',(43.5445020311616,33.2091975287062,-42.9828667778867));
#253066=CARTESIAN_POINT('Ctrl Pts',(43.0627768175819,32.3748249834993,-42.9245334445534));
#253067=CARTESIAN_POINT('Ctrl Pts',(42.5810516040023,31.5404524382925,-42.86620011122));
#253068=CARTESIAN_POINT('Ctrl Pts',(43.0627768175819,30.7060798930856,-42.8078667778867));
#253069=CARTESIAN_POINT('Ctrl Pts',(43.5445020311616,29.8717073478788,-42.7495334445534));
#253070=CARTESIAN_POINT('Ctrl Pts',(44.5079524583208,29.8717073478787,-42.69120011122));
#253071=CARTESIAN_POINT('Ctrl Pts',(45.47140288548,29.8717073478788,-42.6328667778867));
#253072=CARTESIAN_POINT('Ctrl Pts',(45.9531280990597,30.7060798930856,-42.5745334445534));
#253073=CARTESIAN_POINT('Ctrl Pts',(46.4348533126392,31.5404524382925,-42.51620011122));
#253074=CARTESIAN_POINT('Ctrl Pts',(45.9531280990597,32.3748249834993,-42.4578667778867));
#253075=CARTESIAN_POINT('Ctrl Pts',(45.47140288548,33.2091975287062,-42.3995334445534));
#253076=CARTESIAN_POINT('Ctrl Pts',(44.5079524583208,33.2091975287062,-42.34120011122));
#253077=CARTESIAN_POINT('Ctrl Pts',(43.5445020311616,33.2091975287062,-42.2828667778867));
#253078=CARTESIAN_POINT('Ctrl Pts',(43.0627768175819,32.3748249834993,-42.2245334445534));
#253079=CARTESIAN_POINT('Ctrl Pts',(42.5810516040023,31.5404524382925,-42.16620011122));
#253080=CARTESIAN_POINT('Ctrl Pts',(43.0627768175819,30.7060798930856,-42.1078667778867));
#253081=CARTESIAN_POINT('Ctrl Pts',(43.5445020311616,29.8717073478788,-42.0495334445534));
#253082=CARTESIAN_POINT('Ctrl Pts',(44.5079524583208,29.8717073478787,-41.99120011122));
#253083=CARTESIAN_POINT('Ctrl Pts',(45.47140288548,29.8717073478788,-41.9328667778867));
#253084=CARTESIAN_POINT('Ctrl Pts',(45.9531280990597,30.7060798930856,-41.8745334445534));
#253085=CARTESIAN_POINT('Ctrl Pts',(46.4348533126392,31.5404524382925,-41.81620011122));
#253086=CARTESIAN_POINT('Ctrl Pts',(45.9531280990597,32.3748249834993,-41.7578667778867));
#253087=CARTESIAN_POINT('Ctrl Pts',(45.47140288548,33.2091975287062,-41.6995334445533));
#253088=CARTESIAN_POINT('Ctrl Pts',(44.5079524583208,33.2091975287062,-41.64120011122));
#253089=CARTESIAN_POINT('Ctrl Pts',(43.5445020311616,33.2091975287062,-41.5828667778867));
#253090=CARTESIAN_POINT('Ctrl Pts',(43.0627768175819,32.3748249834993,-41.5245334445534));
#253091=CARTESIAN_POINT('Ctrl Pts',(42.5810516040023,31.5404524382925,-41.46620011122));
#253092=CARTESIAN_POINT('Ctrl Pts',(43.0627768175819,30.7060798930856,-41.4078667778867));
#253093=CARTESIAN_POINT('Ctrl Pts',(43.5445020311616,29.8717073478788,-41.3495334445533));
#253094=CARTESIAN_POINT('Ctrl Pts',(44.5079524583208,29.8717073478787,-41.29120011122));
#253095=CARTESIAN_POINT('Ctrl Pts',(45.47140288548,29.8717073478788,-41.2328667778867));
#253096=CARTESIAN_POINT('Ctrl Pts',(45.9531280990597,30.7060798930856,-41.1745334445534));
#253097=CARTESIAN_POINT('Ctrl Pts',(46.4348533126392,31.5404524382925,-41.11620011122));
#253098=CARTESIAN_POINT('Ctrl Pts',(45.9531280990597,32.3748249834993,-41.0578667778867));
#253099=CARTESIAN_POINT('Ctrl Pts',(45.47140288548,33.2091975287062,-40.9995334445534));
#253100=CARTESIAN_POINT('Ctrl Pts',(44.5079524583208,33.2091975287062,-40.94120011122));
#253101=CARTESIAN_POINT('Ctrl Pts',(43.5445020311616,33.2091975287062,-40.8828667778867));
#253102=CARTESIAN_POINT('Ctrl Pts',(43.0627768175819,32.3748249834993,-40.8245334445534));
#253103=CARTESIAN_POINT('Ctrl Pts',(42.5810516040023,31.5404524382925,-40.76620011122));
#253104=CARTESIAN_POINT('Ctrl Pts',(43.0627768175819,30.7060798930856,-40.7078667778867));
#253105=CARTESIAN_POINT('Ctrl Pts',(43.5445020311616,29.8717073478788,-40.6495334445533));
#253106=CARTESIAN_POINT('Ctrl Pts',(44.5079524583208,29.8717073478787,-40.59120011122));
#253107=CARTESIAN_POINT('Ctrl Pts',(45.47140288548,29.8717073478788,-40.5328667778867));
#253108=CARTESIAN_POINT('Ctrl Pts',(45.9531280990597,30.7060798930856,-40.4745334445534));
#253109=CARTESIAN_POINT('Ctrl Pts',(46.4348533126392,31.5404524382925,-40.41620011122));
#253110=CARTESIAN_POINT('Ctrl Pts',(45.9531280990597,32.3748249834993,-40.3578667778867));
#253111=CARTESIAN_POINT('Ctrl Pts',(45.47140288548,33.2091975287062,-40.2995334445534));
#253112=CARTESIAN_POINT('Ctrl Pts',(44.5079524583208,33.2091975287062,-40.24120011122));
#253113=CARTESIAN_POINT('Ctrl Pts',(43.5445020311616,33.2091975287062,-40.1828667778867));
#253114=CARTESIAN_POINT('Ctrl Pts',(43.0627768175819,32.3748249834993,-40.1245334445534));
#253115=CARTESIAN_POINT('Ctrl Pts',(42.5810516040023,31.5404524382925,-40.0662001112201));
#253116=CARTESIAN_POINT('Ctrl Pts',(43.0627768175819,30.7060798930856,-40.0078667778867));
#253117=CARTESIAN_POINT('Ctrl Pts',(43.5445020311616,29.8717073478788,-39.9495334445534));
#253118=CARTESIAN_POINT('Ctrl Pts',(44.5079524583208,29.8717073478787,-39.89120011122));
#253119=CARTESIAN_POINT('Ctrl Pts',(45.47140288548,29.8717073478788,-39.8328667778867));
#253120=CARTESIAN_POINT('Ctrl Pts',(45.9531280990597,30.7060798930856,-39.7745334445534));
#253121=CARTESIAN_POINT('Ctrl Pts',(46.4348533126392,31.5404524382925,-39.7162001112201));
#253122=CARTESIAN_POINT('Ctrl Pts',(45.9531280990597,32.3748249834993,-39.6578667778867));
#253123=CARTESIAN_POINT('Ctrl Pts',(45.47140288548,33.2091975287062,-39.5995334445534));
#253124=CARTESIAN_POINT('Ctrl Pts',(44.5079524583208,33.2091975287062,-39.54120011122));
#253125=CARTESIAN_POINT('Ctrl Pts',(43.5445020311616,33.2091975287062,-39.4828667778867));
#253126=CARTESIAN_POINT('Ctrl Pts',(43.0627768175819,32.3748249834993,-39.4245334445534));
#253127=CARTESIAN_POINT('Ctrl Pts',(42.5810516040023,31.5404524382925,-39.36620011122));
#253128=CARTESIAN_POINT('Ctrl Pts',(43.0627768175819,30.7060798930856,-39.3078667778867));
#253129=CARTESIAN_POINT('Ctrl Pts',(43.5445020311616,29.8717073478788,-39.2495334445534));
#253130=CARTESIAN_POINT('Ctrl Pts',(44.5079524583208,29.8717073478787,-39.19120011122));
#253131=CARTESIAN_POINT('Ctrl Pts',(45.47140288548,29.8717073478788,-39.1328667778867));
#253132=CARTESIAN_POINT('Ctrl Pts',(45.9531280990597,30.7060798930856,-39.0745334445534));
#253133=CARTESIAN_POINT('Ctrl Pts',(46.4348533126392,31.5404524382925,-39.0162001112201));
#253134=CARTESIAN_POINT('Ctrl Pts',(45.9531280990597,32.3748249834993,-38.9578667778867));
#253135=CARTESIAN_POINT('Ctrl Pts',(45.47140288548,33.2091975287062,-38.8995334445534));
#253136=CARTESIAN_POINT('Ctrl Pts',(44.5079524583208,33.2091975287062,-38.84120011122));
#253137=CARTESIAN_POINT('Ctrl Pts',(43.5445020311616,33.2091975287062,-38.7828667778867));
#253138=CARTESIAN_POINT('Ctrl Pts',(43.0627768175819,32.3748249834993,-38.7245334445534));
#253139=CARTESIAN_POINT('Ctrl Pts',(42.5810516040023,31.5404524382925,-38.66620011122));
#253140=CARTESIAN_POINT('Ctrl Pts',(43.0627768175819,30.7060798930856,-38.6078667778867));
#253141=CARTESIAN_POINT('Ctrl Pts',(43.5445020311616,29.8717073478788,-38.5495334445534));
#253142=CARTESIAN_POINT('Ctrl Pts',(44.5079524583208,29.8717073478787,-38.49120011122));
#253143=CARTESIAN_POINT('Ctrl Pts',(45.47140288548,29.8717073478788,-38.4328667778867));
#253144=CARTESIAN_POINT('Ctrl Pts',(45.9531280990597,30.7060798930856,-38.3745334445534));
#253145=CARTESIAN_POINT('Ctrl Pts',(46.4348533126392,31.5404524382925,-38.31620011122));
#253146=CARTESIAN_POINT('Ctrl Pts',(45.9531280990597,32.3748249834993,-38.2578667778867));
#253147=CARTESIAN_POINT('Ctrl Pts',(45.47140288548,33.2091975287062,-38.1995334445534));
#253148=CARTESIAN_POINT('Ctrl Pts',(44.5079524583208,33.2091975287062,-38.14120011122));
#253149=CARTESIAN_POINT('Ctrl Pts',(43.5445020311616,33.2091975287062,-38.0828667778867));
#253150=CARTESIAN_POINT('Ctrl Pts',(43.0627768175819,32.3748249834993,-38.0245334445534));
#253151=CARTESIAN_POINT('Ctrl Pts',(42.5810516040023,31.5404524382925,-37.96620011122));
#253152=CARTESIAN_POINT('Ctrl Pts',(43.0627768175819,30.7060798930856,-37.9078667778867));
#253153=CARTESIAN_POINT('Ctrl Pts',(43.5445020311616,29.8717073478788,-37.8495334445534));
#253154=CARTESIAN_POINT('Ctrl Pts',(44.5079524583208,29.8717073478787,-37.79120011122));
#253155=CARTESIAN_POINT('Ctrl Pts',(45.47140288548,29.8717073478788,-37.7328667778867));
#253156=CARTESIAN_POINT('Ctrl Pts',(45.9531280990597,30.7060798930856,-37.6745334445534));
#253157=CARTESIAN_POINT('Ctrl Pts',(46.4348533126392,31.5404524382925,-37.61620011122));
#253158=CARTESIAN_POINT('Ctrl Pts',(45.9531280990597,32.3748249834993,-37.5578667778867));
#253159=CARTESIAN_POINT('Ctrl Pts',(45.47140288548,33.2091975287062,-37.4995334445534));
#253160=CARTESIAN_POINT('Ctrl Pts',(44.5079524583208,33.2091975287062,-37.44120011122));
#253161=CARTESIAN_POINT('Ctrl Pts',(43.5445020311616,33.2091975287062,-37.3828667778867));
#253162=CARTESIAN_POINT('Ctrl Pts',(43.0627768175819,32.3748249834993,-37.3245334445534));
#253163=CARTESIAN_POINT('Ctrl Pts',(42.5810516040023,31.5404524382925,-37.26620011122));
#253164=CARTESIAN_POINT('Ctrl Pts',(43.0627768175819,30.7060798930856,-37.2078667778867));
#253165=CARTESIAN_POINT('Ctrl Pts',(43.5445020311616,29.8717073478788,-37.1495334445534));
#253166=CARTESIAN_POINT('Ctrl Pts',(44.5079524583208,29.8717073478787,-37.09120011122));
#253167=CARTESIAN_POINT('Ctrl Pts',(45.47140288548,29.8717073478788,-37.0328667778867));
#253168=CARTESIAN_POINT('Ctrl Pts',(45.9531280990597,30.7060798930856,-36.9745334445534));
#253169=CARTESIAN_POINT('Ctrl Pts',(46.4348533126392,31.5404524382925,-36.91620011122));
#253170=CARTESIAN_POINT('Ctrl Pts',(45.9531280990597,32.3748249834993,-36.8578667778867));
#253171=CARTESIAN_POINT('Ctrl Pts',(45.8905903661582,32.4831435142748,-36.8502939244914));
#253172=CARTESIAN_POINT('Ctrl Pts',(45.812604721831,32.5809295635084,-36.8421539353381));
#253173=CARTESIAN_POINT('Ctrl Pts',(45.3258959266108,30.0859149508445,-39.8341886424312));
#253174=CARTESIAN_POINT('Ctrl Pts',(45.4766887394293,30.1176683184879,-39.7972186137753));
#253175=CARTESIAN_POINT('Ctrl Pts',(45.6240618430092,30.1634775829848,-39.7576376985697));
#253176=CARTESIAN_POINT('Ctrl Pts',(45.9073780736838,30.2797207149013,-39.6755711641234));
#253177=CARTESIAN_POINT('Ctrl Pts',(46.0435967979149,30.3502619798024,-39.6330190481983));
#253178=CARTESIAN_POINT('Ctrl Pts',(46.1726018521413,30.4318752072269,-39.5898550147568));
#253179=CARTESIAN_POINT('Ctrl Pts',(44.5079524583208,33.5404524382925,-52.64995));
#253180=CARTESIAN_POINT('Ctrl Pts',(44.3600617863363,33.5275120044939,-52.64995));
#253181=CARTESIAN_POINT('Ctrl Pts',(44.2142042532552,33.4972658634834,-52.64995));
#253182=CARTESIAN_POINT('Ctrl Pts',(43.9445256487737,33.4073033028498,-52.64995));
#253183=CARTESIAN_POINT('Ctrl Pts',(43.8206799356498,33.3505752618931,-52.64995));
#253184=CARTESIAN_POINT('Ctrl Pts',(43.4951040594958,33.1566199207942,-52.64995));
#253185=CARTESIAN_POINT('Ctrl Pts',(43.3122546189713,32.993061702941,-52.6499500000001));
#253186=CARTESIAN_POINT('Ctrl Pts',(43.0527600317385,32.6506630729424,-52.6499500000001));
#253187=CARTESIAN_POINT('Ctrl Pts',(42.923716913873,32.4362244619228,-52.6499500000282));
#253188=CARTESIAN_POINT('Ctrl Pts',(42.815884786658,32.0187869403626,-52.6499500000282));
#253189=CARTESIAN_POINT('Ctrl Pts',(42.7978378140676,31.8711017322126,-52.64995));
#253190=CARTESIAN_POINT('Ctrl Pts',(42.8007193914761,31.5828389853602,-52.64995));
#253191=CARTESIAN_POINT('Ctrl Pts',(42.8195756983132,31.4434642093936,-52.64995));
#253192=CARTESIAN_POINT('Ctrl Pts',(42.8554737113965,31.3080200595814,-52.64995));
#253193=CARTESIAN_POINT('Ctrl Pts',(44.5079524583206,29.5404524382925,-40.39995));
#253194=CARTESIAN_POINT('Ctrl Pts',(44.6726735707786,29.5404524382924,-40.3916285943709));
#253195=CARTESIAN_POINT('Ctrl Pts',(44.8370885939324,29.560796052526,-40.3827292963916));
#253196=CARTESIAN_POINT('Ctrl Pts',(45.2540545582999,29.6660593396596,-40.3585947686536));
#253197=CARTESIAN_POINT('Ctrl Pts',(45.4952144476034,29.781100880629,-40.3430564392622));
#253198=CARTESIAN_POINT('Ctrl Pts',(45.9107928369525,30.0923892617563,-40.3129829440037));
#253199=CARTESIAN_POINT('Ctrl Pts',(46.0836233502634,30.2826150347246,-40.298703614746));
#253200=CARTESIAN_POINT('Ctrl Pts',(46.3539827028743,30.7265592826002,-40.2720971869114));
#253201=CARTESIAN_POINT('Ctrl Pts',(46.4455209456663,30.9781639989288,-40.257750158963));
#253202=CARTESIAN_POINT('Ctrl Pts',(46.5245281260493,31.498788220226,-40.2273804127207));
#253203=CARTESIAN_POINT('Ctrl Pts',(46.51271142587,31.7624037383698,-40.2120028408289));
#253204=CARTESIAN_POINT('Ctrl Pts',(46.390237568377,32.2624037194517,-40.1828361752658));
#253205=CARTESIAN_POINT('Ctrl Pts',(46.2837494529182,32.4947747783608,-40.1701589081232));
#253206=CARTESIAN_POINT('Ctrl Pts',(45.9828009175854,32.9171053148226,-40.1426375713279));
#253207=CARTESIAN_POINT('Ctrl Pts',(45.7874580424598,33.1003170079869,-40.1274255365594));
#253208=CARTESIAN_POINT('Ctrl Pts',(45.3425464845978,33.3762658448928,-40.0969009206428));
#253209=CARTESIAN_POINT('Ctrl Pts',(45.0986295415486,33.4686341292234,-40.0818846133193));
#253210=CARTESIAN_POINT('Ctrl Pts',(44.5906612810477,33.5551825985649,-40.0536986669188));
#253211=CARTESIAN_POINT('Ctrl Pts',(44.3315471104784,33.5491493054718,-40.0412919870582));
#253212=CARTESIAN_POINT('Ctrl Pts',(43.8212908135486,33.4375447334715,-40.0122596502992));
#253213=CARTESIAN_POINT('Ctrl Pts',(43.5758589971117,33.3297668085751,-39.9967173665271));
#253214=CARTESIAN_POINT('Ctrl Pts',(43.1496219859757,33.0304761630696,-39.9664553513854));
#253215=CARTESIAN_POINT('Ctrl Pts',(42.9706008156226,32.8449923244166,-39.9520015880131));
#253216=CARTESIAN_POINT('Ctrl Pts',(42.6865838608895,32.4082610549434,-39.9249155819424));
#253217=CARTESIAN_POINT('Ctrl Pts',(42.5875791924248,32.1590797911578,-39.911036595584));
#253218=CARTESIAN_POINT('Ctrl Pts',(42.4933024988169,31.6398809877825,-39.8807499987204));
#253219=CARTESIAN_POINT('Ctrl Pts',(42.4976238199733,31.375279663566,-39.8653149214744));
#253220=CARTESIAN_POINT('Ctrl Pts',(42.6062198512718,30.8714461891254,-39.8359246354654));
#253221=CARTESIAN_POINT('Ctrl Pts',(42.7061181645385,30.63629095421,-39.8229372892375));
#253222=CARTESIAN_POINT('Ctrl Pts',(42.9949839972762,30.2058136577985,-39.7957887343751));
#253223=CARTESIAN_POINT('Ctrl Pts',(43.1850710842596,30.0172073370075,-39.7806848689869));
#253224=CARTESIAN_POINT('Ctrl Pts',(43.6225900977621,29.7284769831686,-39.7501609164806));
#253225=CARTESIAN_POINT('Ctrl Pts',(43.8645262589039,29.6291319201338,-39.7350411852129));
#253226=CARTESIAN_POINT('Ctrl Pts',(44.2471843430749,29.553202963529,-39.7134954127037));
#253227=CARTESIAN_POINT('Ctrl Pts',(44.3775512255878,29.5404524382925,-39.7065376288468));
#253228=CARTESIAN_POINT('Ctrl Pts',(44.5079524583208,29.5404524382925,-39.69995));
#253229=CARTESIAN_POINT('Ctrl Pts',(44.5079524583208,33.2091977213449,-52.99995));
#253230=CARTESIAN_POINT('Ctrl Pts',(43.5445019199415,33.2091977213449,-52.9416166666667));
#253231=CARTESIAN_POINT('Ctrl Pts',(43.0627766507519,32.3748250798187,-52.8832833333334));
#253232=CARTESIAN_POINT('Ctrl Pts',(42.5810513815623,31.5404524382925,-52.82495));
#253233=CARTESIAN_POINT('Ctrl Pts',(43.0627766507519,30.7060797967663,-52.7666166666667));
#253234=CARTESIAN_POINT('Ctrl Pts',(43.5445019199415,29.87170715524,-52.7082833333333));
#253235=CARTESIAN_POINT('Ctrl Pts',(44.5079524583208,29.87170715524,-52.64995));
#253236=CARTESIAN_POINT('Ctrl Pts',(45.4714029967,29.87170715524,-52.5916166666666));
#253237=CARTESIAN_POINT('Ctrl Pts',(45.9531282658897,30.7060797967663,-52.5332833333334));
#253238=CARTESIAN_POINT('Ctrl Pts',(46.4348535350793,31.5404524382925,-52.4749500000001));
#253239=CARTESIAN_POINT('Ctrl Pts',(45.9531282658897,32.3748250798187,-52.4166166666667));
#253240=CARTESIAN_POINT('Ctrl Pts',(45.4714029967,33.2091977213449,-52.3582833333334));
#253241=CARTESIAN_POINT('Ctrl Pts',(44.5079524583208,33.2091977213449,-52.29995));
#253242=CARTESIAN_POINT('Ctrl Pts',(43.5445019199415,33.2091977213449,-52.2416166666667));
#253243=CARTESIAN_POINT('Ctrl Pts',(43.0627766507519,32.3748250798187,-52.1832833333333));
#253244=CARTESIAN_POINT('Ctrl Pts',(42.5810513815623,31.5404524382925,-52.12495));
#253245=CARTESIAN_POINT('Ctrl Pts',(43.0627766507519,30.7060797967663,-52.0666166666667));
#253246=CARTESIAN_POINT('Ctrl Pts',(43.5445019199415,29.87170715524,-52.0082833333333));
#253247=CARTESIAN_POINT('Ctrl Pts',(44.5079524583208,29.87170715524,-51.94995));
#253248=CARTESIAN_POINT('Ctrl Pts',(45.4714029967,29.87170715524,-51.8916166666667));
#253249=CARTESIAN_POINT('Ctrl Pts',(45.9531282658897,30.7060797967663,-51.8332833333333));
#253250=CARTESIAN_POINT('Ctrl Pts',(46.4348535350793,31.5404524382925,-51.77495));
#253251=CARTESIAN_POINT('Ctrl Pts',(45.9531282658897,32.3748250798187,-51.7166166666667));
#253252=CARTESIAN_POINT('Ctrl Pts',(45.4714029967,33.2091977213449,-51.6582833333333));
#253253=CARTESIAN_POINT('Ctrl Pts',(44.5079524583208,33.2091977213449,-51.59995));
#253254=CARTESIAN_POINT('Ctrl Pts',(43.5445019199415,33.2091977213449,-51.5416166666667));
#253255=CARTESIAN_POINT('Ctrl Pts',(43.0627766507519,32.3748250798187,-51.4832833333333));
#253256=CARTESIAN_POINT('Ctrl Pts',(42.5810513815623,31.5404524382925,-51.42495));
#253257=CARTESIAN_POINT('Ctrl Pts',(43.0627766507519,30.7060797967663,-51.3666166666667));
#253258=CARTESIAN_POINT('Ctrl Pts',(43.5445019199415,29.87170715524,-51.3082833333333));
#253259=CARTESIAN_POINT('Ctrl Pts',(44.5079524583208,29.87170715524,-51.24995));
#253260=CARTESIAN_POINT('Ctrl Pts',(45.4714029967,29.87170715524,-51.1916166666667));
#253261=CARTESIAN_POINT('Ctrl Pts',(45.9531282658897,30.7060797967663,-51.1332833333333));
#253262=CARTESIAN_POINT('Ctrl Pts',(46.4348535350793,31.5404524382925,-51.07495));
#253263=CARTESIAN_POINT('Ctrl Pts',(45.9531282658897,32.3748250798187,-51.0166166666667));
#253264=CARTESIAN_POINT('Ctrl Pts',(45.4714029967,33.2091977213449,-50.9582833333334));
#253265=CARTESIAN_POINT('Ctrl Pts',(44.5079524583208,33.2091977213449,-50.89995));
#253266=CARTESIAN_POINT('Ctrl Pts',(43.5445019199415,33.2091977213449,-50.8416166666667));
#253267=CARTESIAN_POINT('Ctrl Pts',(43.0627766507519,32.3748250798187,-50.7832833333333));
#253268=CARTESIAN_POINT('Ctrl Pts',(42.5810513815623,31.5404524382925,-50.72495));
#253269=CARTESIAN_POINT('Ctrl Pts',(43.0627766507519,30.7060797967663,-50.6666166666667));
#253270=CARTESIAN_POINT('Ctrl Pts',(43.5445019199415,29.87170715524,-50.6082833333334));
#253271=CARTESIAN_POINT('Ctrl Pts',(44.5079524583208,29.87170715524,-50.54995));
#253272=CARTESIAN_POINT('Ctrl Pts',(45.4714029967,29.87170715524,-50.4916166666667));
#253273=CARTESIAN_POINT('Ctrl Pts',(45.9531282658897,30.7060797967663,-50.4332833333333));
#253274=CARTESIAN_POINT('Ctrl Pts',(46.4348535350793,31.5404524382925,-50.37495));
#253275=CARTESIAN_POINT('Ctrl Pts',(45.9531282658897,32.3748250798187,-50.3166166666667));
#253276=CARTESIAN_POINT('Ctrl Pts',(45.4714029967,33.2091977213449,-50.2582833333334));
#253277=CARTESIAN_POINT('Ctrl Pts',(44.5079524583208,33.2091977213449,-50.19995));
#253278=CARTESIAN_POINT('Ctrl Pts',(43.5445019199415,33.2091977213449,-50.1416166666667));
#253279=CARTESIAN_POINT('Ctrl Pts',(43.0627766507519,32.3748250798187,-50.0832833333333));
#253280=CARTESIAN_POINT('Ctrl Pts',(42.5810513815623,31.5404524382925,-50.02495));
#253281=CARTESIAN_POINT('Ctrl Pts',(43.0627766507519,30.7060797967663,-49.9666166666667));
#253282=CARTESIAN_POINT('Ctrl Pts',(43.5445019199415,29.87170715524,-49.9082833333334));
#253283=CARTESIAN_POINT('Ctrl Pts',(44.5079524583208,29.87170715524,-49.84995));
#253284=CARTESIAN_POINT('Ctrl Pts',(45.4714029967,29.87170715524,-49.7916166666667));
#253285=CARTESIAN_POINT('Ctrl Pts',(45.9531282658897,30.7060797967663,-49.7332833333333));
#253286=CARTESIAN_POINT('Ctrl Pts',(46.4348535350793,31.5404524382925,-49.67495));
#253287=CARTESIAN_POINT('Ctrl Pts',(45.9531282658897,32.3748250798187,-49.6166166666667));
#253288=CARTESIAN_POINT('Ctrl Pts',(45.4714029967,33.2091977213449,-49.5582833333334));
#253289=CARTESIAN_POINT('Ctrl Pts',(44.5079524583208,33.2091977213449,-49.49995));
#253290=CARTESIAN_POINT('Ctrl Pts',(43.5445019199415,33.2091977213449,-49.4416166666667));
#253291=CARTESIAN_POINT('Ctrl Pts',(43.0627766507519,32.3748250798187,-49.3832833333334));
#253292=CARTESIAN_POINT('Ctrl Pts',(42.5810513815623,31.5404524382925,-49.32495));
#253293=CARTESIAN_POINT('Ctrl Pts',(43.0627766507519,30.7060797967663,-49.2666166666667));
#253294=CARTESIAN_POINT('Ctrl Pts',(43.5445019199415,29.87170715524,-49.2082833333334));
#253295=CARTESIAN_POINT('Ctrl Pts',(44.5079524583208,29.87170715524,-49.14995));
#253296=CARTESIAN_POINT('Ctrl Pts',(45.4714029967,29.87170715524,-49.0916166666667));
#253297=CARTESIAN_POINT('Ctrl Pts',(45.9531282658897,30.7060797967663,-49.0332833333333));
#253298=CARTESIAN_POINT('Ctrl Pts',(46.4348535350793,31.5404524382925,-48.97495));
#253299=CARTESIAN_POINT('Ctrl Pts',(45.9531282658897,32.3748250798187,-48.9166166666667));
#253300=CARTESIAN_POINT('Ctrl Pts',(45.4714029967,33.2091977213449,-48.8582833333333));
#253301=CARTESIAN_POINT('Ctrl Pts',(44.5079524583208,33.2091977213449,-48.79995));
#253302=CARTESIAN_POINT('Ctrl Pts',(43.5445019199415,33.2091977213449,-48.7416166666667));
#253303=CARTESIAN_POINT('Ctrl Pts',(43.0627766507519,32.3748250798187,-48.6832833333333));
#253304=CARTESIAN_POINT('Ctrl Pts',(42.5810513815623,31.5404524382925,-48.62495));
#253305=CARTESIAN_POINT('Ctrl Pts',(43.0627766507519,30.7060797967663,-48.5666166666667));
#253306=CARTESIAN_POINT('Ctrl Pts',(43.5445019199415,29.87170715524,-48.5082833333333));
#253307=CARTESIAN_POINT('Ctrl Pts',(44.5079524583208,29.87170715524,-48.44995));
#253308=CARTESIAN_POINT('Ctrl Pts',(45.4714029967,29.87170715524,-48.3916166666667));
#253309=CARTESIAN_POINT('Ctrl Pts',(45.9531282658897,30.7060797967663,-48.3332833333333));
#253310=CARTESIAN_POINT('Ctrl Pts',(46.4348535350793,31.5404524382925,-48.27495));
#253311=CARTESIAN_POINT('Ctrl Pts',(45.9531282658897,32.3748250798187,-48.2166166666667));
#253312=CARTESIAN_POINT('Ctrl Pts',(45.4714029967,33.2091977213449,-48.1582833333333));
#253313=CARTESIAN_POINT('Ctrl Pts',(44.5079524583208,33.2091977213449,-48.09995));
#253314=CARTESIAN_POINT('Ctrl Pts',(43.5445019199415,33.2091977213449,-48.0416166666667));
#253315=CARTESIAN_POINT('Ctrl Pts',(43.0627766507519,32.3748250798187,-47.9832833333334));
#253316=CARTESIAN_POINT('Ctrl Pts',(42.5810513815623,31.5404524382925,-47.92495));
#253317=CARTESIAN_POINT('Ctrl Pts',(43.0627766507519,30.7060797967663,-47.8666166666667));
#253318=CARTESIAN_POINT('Ctrl Pts',(43.5445019199415,29.87170715524,-47.8082833333333));
#253319=CARTESIAN_POINT('Ctrl Pts',(44.5079524583208,29.87170715524,-47.74995));
#253320=CARTESIAN_POINT('Ctrl Pts',(45.4714029967,29.87170715524,-47.6916166666667));
#253321=CARTESIAN_POINT('Ctrl Pts',(45.9531282658897,30.7060797967663,-47.6332833333333));
#253322=CARTESIAN_POINT('Ctrl Pts',(46.4348535350793,31.5404524382925,-47.57495));
#253323=CARTESIAN_POINT('Ctrl Pts',(45.9531282658897,32.3748250798187,-47.5166166666667));
#253324=CARTESIAN_POINT('Ctrl Pts',(45.4714029967,33.2091977213449,-47.4582833333333));
#253325=CARTESIAN_POINT('Ctrl Pts',(44.5079524583208,33.2091977213449,-47.39995));
#253326=CARTESIAN_POINT('Ctrl Pts',(43.5445019199415,33.2091977213449,-47.3416166666666));
#253327=CARTESIAN_POINT('Ctrl Pts',(43.0627766507519,32.3748250798187,-47.2832833333333));
#253328=CARTESIAN_POINT('Ctrl Pts',(42.5810513815623,31.5404524382925,-47.22495));
#253329=CARTESIAN_POINT('Ctrl Pts',(43.0627766507519,30.7060797967663,-47.1666166666667));
#253330=CARTESIAN_POINT('Ctrl Pts',(43.5445019199415,29.87170715524,-47.1082833333333));
#253331=CARTESIAN_POINT('Ctrl Pts',(44.5079524583208,29.87170715524,-47.04995));
#253332=CARTESIAN_POINT('Ctrl Pts',(45.4714029967,29.87170715524,-46.9916166666667));
#253333=CARTESIAN_POINT('Ctrl Pts',(45.9531282658897,30.7060797967663,-46.9332833333333));
#253334=CARTESIAN_POINT('Ctrl Pts',(46.4348535350793,31.5404524382925,-46.87495));
#253335=CARTESIAN_POINT('Ctrl Pts',(45.9531282658897,32.3748250798187,-46.8166166666667));
#253336=CARTESIAN_POINT('Ctrl Pts',(45.4714029967,33.2091977213449,-46.7582833333333));
#253337=CARTESIAN_POINT('Ctrl Pts',(44.5079524583208,33.2091977213449,-46.69995));
#253338=CARTESIAN_POINT('Ctrl Pts',(43.5445019199415,33.2091977213449,-46.6416166666666));
#253339=CARTESIAN_POINT('Ctrl Pts',(43.0627766507519,32.3748250798187,-46.5832833333334));
#253340=CARTESIAN_POINT('Ctrl Pts',(42.5810513815623,31.5404524382925,-46.52495));
#253341=CARTESIAN_POINT('Ctrl Pts',(43.0627766507519,30.7060797967663,-46.4666166666667));
#253342=CARTESIAN_POINT('Ctrl Pts',(43.5445019199415,29.87170715524,-46.4082833333333));
#253343=CARTESIAN_POINT('Ctrl Pts',(44.5079524583208,29.87170715524,-46.34995));
#253344=CARTESIAN_POINT('Ctrl Pts',(45.4714029967,29.87170715524,-46.2916166666667));
#253345=CARTESIAN_POINT('Ctrl Pts',(45.9531282658897,30.7060797967663,-46.2332833333334));
#253346=CARTESIAN_POINT('Ctrl Pts',(46.4348535350793,31.5404524382925,-46.17495));
#253347=CARTESIAN_POINT('Ctrl Pts',(45.9531282658897,32.3748250798187,-46.1166166666667));
#253348=CARTESIAN_POINT('Ctrl Pts',(45.4714029967,33.2091977213449,-46.0582833333333));
#253349=CARTESIAN_POINT('Ctrl Pts',(44.5079524583208,33.2091977213449,-45.99995));
#253350=CARTESIAN_POINT('Ctrl Pts',(43.5445019199415,33.2091977213449,-45.9416166666667));
#253351=CARTESIAN_POINT('Ctrl Pts',(43.0627766507519,32.3748250798187,-45.8832833333333));
#253352=CARTESIAN_POINT('Ctrl Pts',(42.5810513815623,31.5404524382925,-45.82495));
#253353=CARTESIAN_POINT('Ctrl Pts',(43.0627766507519,30.7060797967663,-45.7666166666667));
#253354=CARTESIAN_POINT('Ctrl Pts',(43.5445019199415,29.87170715524,-45.7082833333333));
#253355=CARTESIAN_POINT('Ctrl Pts',(44.5079524583208,29.87170715524,-45.64995));
#253356=CARTESIAN_POINT('Ctrl Pts',(45.4714029967,29.87170715524,-45.5916166666667));
#253357=CARTESIAN_POINT('Ctrl Pts',(45.9531282658897,30.7060797967663,-45.5332833333333));
#253358=CARTESIAN_POINT('Ctrl Pts',(46.4348535350793,31.5404524382925,-45.47495));
#253359=CARTESIAN_POINT('Ctrl Pts',(45.9531282658897,32.3748250798187,-45.4166166666667));
#253360=CARTESIAN_POINT('Ctrl Pts',(45.4714029967,33.2091977213449,-45.3582833333333));
#253361=CARTESIAN_POINT('Ctrl Pts',(44.5079524583208,33.2091977213449,-45.29995));
#253362=CARTESIAN_POINT('Ctrl Pts',(43.5445019199415,33.2091977213449,-45.2416166666667));
#253363=CARTESIAN_POINT('Ctrl Pts',(43.0627766507519,32.3748250798187,-45.1832833333333));
#253364=CARTESIAN_POINT('Ctrl Pts',(42.5810513815623,31.5404524382925,-45.12495));
#253365=CARTESIAN_POINT('Ctrl Pts',(43.0627766507519,30.7060797967663,-45.0666166666667));
#253366=CARTESIAN_POINT('Ctrl Pts',(43.5445019199415,29.87170715524,-45.0082833333334));
#253367=CARTESIAN_POINT('Ctrl Pts',(44.5079524583208,29.87170715524,-44.94995));
#253368=CARTESIAN_POINT('Ctrl Pts',(45.4714029967,29.87170715524,-44.8916166666667));
#253369=CARTESIAN_POINT('Ctrl Pts',(45.9531282658897,30.7060797967663,-44.8332833333334));
#253370=CARTESIAN_POINT('Ctrl Pts',(46.4348535350793,31.5404524382925,-44.77495));
#253371=CARTESIAN_POINT('Ctrl Pts',(45.9531282658897,32.3748250798187,-44.7166166666667));
#253372=CARTESIAN_POINT('Ctrl Pts',(45.4714029967,33.2091977213449,-44.6582833333333));
#253373=CARTESIAN_POINT('Ctrl Pts',(44.5079524583208,33.2091977213449,-44.59995));
#253374=CARTESIAN_POINT('Ctrl Pts',(43.5445019199415,33.2091977213449,-44.5416166666667));
#253375=CARTESIAN_POINT('Ctrl Pts',(43.0627766507519,32.3748250798187,-44.4832833333334));
#253376=CARTESIAN_POINT('Ctrl Pts',(42.5810513815623,31.5404524382925,-44.42495));
#253377=CARTESIAN_POINT('Ctrl Pts',(43.0627766507519,30.7060797967663,-44.3666166666667));
#253378=CARTESIAN_POINT('Ctrl Pts',(43.5445019199415,29.87170715524,-44.3082833333334));
#253379=CARTESIAN_POINT('Ctrl Pts',(44.5079524583208,29.87170715524,-44.24995));
#253380=CARTESIAN_POINT('Ctrl Pts',(45.4714029967,29.87170715524,-44.1916166666667));
#253381=CARTESIAN_POINT('Ctrl Pts',(45.9531282658897,30.7060797967663,-44.1332833333334));
#253382=CARTESIAN_POINT('Ctrl Pts',(46.4348535350793,31.5404524382925,-44.07495));
#253383=CARTESIAN_POINT('Ctrl Pts',(45.9531282658897,32.3748250798187,-44.0166166666667));
#253384=CARTESIAN_POINT('Ctrl Pts',(45.4714029967,33.2091977213449,-43.9582833333334));
#253385=CARTESIAN_POINT('Ctrl Pts',(44.5079524583208,33.2091977213449,-43.89995));
#253386=CARTESIAN_POINT('Ctrl Pts',(43.5445019199415,33.2091977213449,-43.8416166666667));
#253387=CARTESIAN_POINT('Ctrl Pts',(43.0627766507519,32.3748250798187,-43.7832833333334));
#253388=CARTESIAN_POINT('Ctrl Pts',(42.5810513815623,31.5404524382925,-43.72495));
#253389=CARTESIAN_POINT('Ctrl Pts',(43.0627766507519,30.7060797967663,-43.6666166666667));
#253390=CARTESIAN_POINT('Ctrl Pts',(43.5445019199415,29.87170715524,-43.6082833333333));
#253391=CARTESIAN_POINT('Ctrl Pts',(44.5079524583208,29.87170715524,-43.54995));
#253392=CARTESIAN_POINT('Ctrl Pts',(45.4714029967,29.87170715524,-43.4916166666667));
#253393=CARTESIAN_POINT('Ctrl Pts',(45.9531282658897,30.7060797967663,-43.4332833333333));
#253394=CARTESIAN_POINT('Ctrl Pts',(46.4348535350793,31.5404524382925,-43.37495));
#253395=CARTESIAN_POINT('Ctrl Pts',(45.9531282658897,32.3748250798187,-43.3166166666667));
#253396=CARTESIAN_POINT('Ctrl Pts',(45.4714029967,33.2091977213449,-43.2582833333333));
#253397=CARTESIAN_POINT('Ctrl Pts',(44.5079524583208,33.2091977213449,-43.19995));
#253398=CARTESIAN_POINT('Ctrl Pts',(43.5445019199415,33.2091977213449,-43.1416166666666));
#253399=CARTESIAN_POINT('Ctrl Pts',(43.0627766507519,32.3748250798187,-43.0832833333333));
#253400=CARTESIAN_POINT('Ctrl Pts',(42.5810513815623,31.5404524382925,-43.02495));
#253401=CARTESIAN_POINT('Ctrl Pts',(43.0627766507519,30.7060797967663,-42.9666166666667));
#253402=CARTESIAN_POINT('Ctrl Pts',(43.5445019199415,29.87170715524,-42.9082833333333));
#253403=CARTESIAN_POINT('Ctrl Pts',(44.5079524583208,29.87170715524,-42.84995));
#253404=CARTESIAN_POINT('Ctrl Pts',(45.4714029967,29.87170715524,-42.7916166666667));
#253405=CARTESIAN_POINT('Ctrl Pts',(45.9531282658897,30.7060797967663,-42.7332833333334));
#253406=CARTESIAN_POINT('Ctrl Pts',(46.4348535350793,31.5404524382925,-42.67495));
#253407=CARTESIAN_POINT('Ctrl Pts',(45.9531282658897,32.3748250798187,-42.6166166666667));
#253408=CARTESIAN_POINT('Ctrl Pts',(45.4714029967,33.2091977213449,-42.5582833333333));
#253409=CARTESIAN_POINT('Ctrl Pts',(44.5079524583208,33.2091977213449,-42.49995));
#253410=CARTESIAN_POINT('Ctrl Pts',(43.5445019199415,33.2091977213449,-42.4416166666667));
#253411=CARTESIAN_POINT('Ctrl Pts',(43.0627766507519,32.3748250798187,-42.3832833333333));
#253412=CARTESIAN_POINT('Ctrl Pts',(42.5810513815623,31.5404524382925,-42.32495));
#253413=CARTESIAN_POINT('Ctrl Pts',(43.0627766507519,30.7060797967663,-42.2666166666667));
#253414=CARTESIAN_POINT('Ctrl Pts',(43.5445019199415,29.87170715524,-42.2082833333333));
#253415=CARTESIAN_POINT('Ctrl Pts',(44.5079524583208,29.87170715524,-42.14995));
#253416=CARTESIAN_POINT('Ctrl Pts',(45.4714029967,29.87170715524,-42.0916166666667));
#253417=CARTESIAN_POINT('Ctrl Pts',(45.9531282658897,30.7060797967663,-42.0332833333334));
#253418=CARTESIAN_POINT('Ctrl Pts',(46.4348535350793,31.5404524382925,-41.97495));
#253419=CARTESIAN_POINT('Ctrl Pts',(45.9531282658897,32.3748250798187,-41.9166166666666));
#253420=CARTESIAN_POINT('Ctrl Pts',(45.4714029967,33.2091977213449,-41.8582833333333));
#253421=CARTESIAN_POINT('Ctrl Pts',(44.5079524583208,33.2091977213449,-41.79995));
#253422=CARTESIAN_POINT('Ctrl Pts',(43.5445019199415,33.2091977213449,-41.7416166666667));
#253423=CARTESIAN_POINT('Ctrl Pts',(43.0627766507519,32.3748250798187,-41.6832833333333));
#253424=CARTESIAN_POINT('Ctrl Pts',(42.5810513815623,31.5404524382925,-41.62495));
#253425=CARTESIAN_POINT('Ctrl Pts',(43.0627766507519,30.7060797967663,-41.5666166666667));
#253426=CARTESIAN_POINT('Ctrl Pts',(43.5445019199415,29.87170715524,-41.5082833333334));
#253427=CARTESIAN_POINT('Ctrl Pts',(44.5079524583208,29.87170715524,-41.44995));
#253428=CARTESIAN_POINT('Ctrl Pts',(45.4714029967,29.87170715524,-41.3916166666667));
#253429=CARTESIAN_POINT('Ctrl Pts',(45.9531282658897,30.7060797967663,-41.3332833333334));
#253430=CARTESIAN_POINT('Ctrl Pts',(46.4348535350793,31.5404524382925,-41.27495));
#253431=CARTESIAN_POINT('Ctrl Pts',(45.9531282658897,32.3748250798187,-41.2166166666667));
#253432=CARTESIAN_POINT('Ctrl Pts',(45.4714029967,33.2091977213449,-41.1582833333333));
#253433=CARTESIAN_POINT('Ctrl Pts',(44.5079524583208,33.2091977213449,-41.09995));
#253434=CARTESIAN_POINT('Ctrl Pts',(43.5445019199415,33.2091977213449,-41.0416166666667));
#253435=CARTESIAN_POINT('Ctrl Pts',(43.0627766507519,32.3748250798187,-40.9832833333333));
#253436=CARTESIAN_POINT('Ctrl Pts',(42.5810513815623,31.5404524382925,-40.92495));
#253437=CARTESIAN_POINT('Ctrl Pts',(43.0627766507519,30.7060797967663,-40.8666166666667));
#253438=CARTESIAN_POINT('Ctrl Pts',(43.5445019199415,29.87170715524,-40.8082833333334));
#253439=CARTESIAN_POINT('Ctrl Pts',(44.5079524583208,29.87170715524,-40.74995));
#253440=CARTESIAN_POINT('Ctrl Pts',(45.4714029967,29.87170715524,-40.6916166666667));
#253441=CARTESIAN_POINT('Ctrl Pts',(45.9531282658897,30.7060797967663,-40.6332833333334));
#253442=CARTESIAN_POINT('Ctrl Pts',(46.4348535350793,31.5404524382925,-40.57495));
#253443=CARTESIAN_POINT('Ctrl Pts',(45.9531282658897,32.3748250798187,-40.5166166666666));
#253444=CARTESIAN_POINT('Ctrl Pts',(45.4714029967,33.2091977213449,-40.4582833333333));
#253445=CARTESIAN_POINT('Ctrl Pts',(44.5079524583208,33.2091977213449,-40.39995));
#253446=CARTESIAN_POINT('Ctrl Pts',(43.5445019199415,33.2091977213449,-40.3416166666667));
#253447=CARTESIAN_POINT('Ctrl Pts',(43.0627766507519,32.3748250798187,-40.2832833333334));
#253448=CARTESIAN_POINT('Ctrl Pts',(42.5810513815623,31.5404524382925,-40.22495));
#253449=CARTESIAN_POINT('Ctrl Pts',(43.0627766507519,30.7060797967663,-40.1666166666667));
#253450=CARTESIAN_POINT('Ctrl Pts',(43.5445019199415,29.87170715524,-40.1082833333334));
#253451=CARTESIAN_POINT('Ctrl Pts',(44.5079524583208,29.87170715524,-40.04995));
#253452=CARTESIAN_POINT('Ctrl Pts',(45.4714029967,29.87170715524,-39.9916166666667));
#253453=CARTESIAN_POINT('Ctrl Pts',(45.9531282658897,30.7060797967663,-39.9332833333333));
#253454=CARTESIAN_POINT('Ctrl Pts',(46.4348535350793,31.5404524382925,-39.87495));
#253455=CARTESIAN_POINT('Ctrl Pts',(45.9531282658897,32.3748250798187,-39.8166166666667));
#253456=CARTESIAN_POINT('Ctrl Pts',(45.4714029967,33.2091977213449,-39.7582833333334));
#253457=CARTESIAN_POINT('Ctrl Pts',(44.5079524583208,33.2091977213449,-39.69995));
#253458=CARTESIAN_POINT('Ctrl Pts',(43.5445019199415,33.2091977213449,-39.6416166666667));
#253459=CARTESIAN_POINT('Ctrl Pts',(43.0627766507519,32.3748250798187,-39.5832833333333));
#253460=CARTESIAN_POINT('Ctrl Pts',(42.5810513815623,31.5404524382925,-39.52495));
#253461=CARTESIAN_POINT('Ctrl Pts',(43.0627766507519,30.7060797967663,-39.4666166666667));
#253462=CARTESIAN_POINT('Ctrl Pts',(43.5445019199415,29.87170715524,-39.4082833333333));
#253463=CARTESIAN_POINT('Ctrl Pts',(44.5079524583208,29.87170715524,-39.34995));
#253464=CARTESIAN_POINT('Ctrl Pts',(45.4714029967,29.87170715524,-39.2916166666667));
#253465=CARTESIAN_POINT('Ctrl Pts',(45.9531282658897,30.7060797967663,-39.2332833333333));
#253466=CARTESIAN_POINT('Ctrl Pts',(46.4348535350793,31.5404524382925,-39.17495));
#253467=CARTESIAN_POINT('Ctrl Pts',(45.9531282658897,32.3748250798187,-39.1166166666667));
#253468=CARTESIAN_POINT('Ctrl Pts',(45.4714029967,33.2091977213449,-39.0582833333333));
#253469=CARTESIAN_POINT('Ctrl Pts',(44.5079524583208,33.2091977213449,-38.99995));
#253470=CARTESIAN_POINT('Ctrl Pts',(43.5445019199415,33.2091977213449,-38.9416166666667));
#253471=CARTESIAN_POINT('Ctrl Pts',(43.0627766507519,32.3748250798187,-38.8832833333334));
#253472=CARTESIAN_POINT('Ctrl Pts',(42.5810513815623,31.5404524382925,-38.82495));
#253473=CARTESIAN_POINT('Ctrl Pts',(43.0627766507519,30.7060797967663,-38.7666166666667));
#253474=CARTESIAN_POINT('Ctrl Pts',(43.5445019199415,29.87170715524,-38.7082833333333));
#253475=CARTESIAN_POINT('Ctrl Pts',(44.5079524583208,29.87170715524,-38.64995));
#253476=CARTESIAN_POINT('Ctrl Pts',(45.4714029967,29.87170715524,-38.5916166666667));
#253477=CARTESIAN_POINT('Ctrl Pts',(45.9531282658897,30.7060797967663,-38.5332833333334));
#253478=CARTESIAN_POINT('Ctrl Pts',(46.4348535350793,31.5404524382925,-38.47495));
#253479=CARTESIAN_POINT('Ctrl Pts',(45.9531282658897,32.3748250798187,-38.4166166666667));
#253480=CARTESIAN_POINT('Ctrl Pts',(45.4714029967,33.2091977213449,-38.3582833333333));
#253481=CARTESIAN_POINT('Ctrl Pts',(44.5079524583208,33.2091977213449,-38.29995));
#253482=CARTESIAN_POINT('Ctrl Pts',(43.5445019199415,33.2091977213449,-38.2416166666667));
#253483=CARTESIAN_POINT('Ctrl Pts',(43.0627766507519,32.3748250798187,-38.1832833333333));
#253484=CARTESIAN_POINT('Ctrl Pts',(42.5810513815623,31.5404524382925,-38.12495));
#253485=CARTESIAN_POINT('Ctrl Pts',(43.0627766507519,30.7060797967663,-38.0666166666667));
#253486=CARTESIAN_POINT('Ctrl Pts',(43.5445019199415,29.87170715524,-38.0082833333333));
#253487=CARTESIAN_POINT('Ctrl Pts',(44.5079524583208,29.87170715524,-37.94995));
#253488=CARTESIAN_POINT('Ctrl Pts',(45.4714029967,29.87170715524,-37.8916166666667));
#253489=CARTESIAN_POINT('Ctrl Pts',(45.9531282658897,30.7060797967663,-37.8332833333334));
#253490=CARTESIAN_POINT('Ctrl Pts',(46.4348535350793,31.5404524382925,-37.77495));
#253491=CARTESIAN_POINT('Ctrl Pts',(45.9531282658897,32.3748250798187,-37.7166166666667));
#253492=CARTESIAN_POINT('Ctrl Pts',(45.4714029967,33.2091977213449,-37.6582833333333));
#253493=CARTESIAN_POINT('Ctrl Pts',(44.5079524583208,33.2091977213449,-37.59995));
#253494=CARTESIAN_POINT('Ctrl Pts',(43.5445019199415,33.2091977213449,-37.5416166666667));
#253495=CARTESIAN_POINT('Ctrl Pts',(43.0627766507519,32.3748250798187,-37.4832833333334));
#253496=CARTESIAN_POINT('Ctrl Pts',(42.5810513815623,31.5404524382925,-37.42495));
#253497=CARTESIAN_POINT('Ctrl Pts',(43.0627766507519,30.7060797967663,-37.3666166666667));
#253498=CARTESIAN_POINT('Ctrl Pts',(43.5445019199415,29.87170715524,-37.3082833333333));
#253499=CARTESIAN_POINT('Ctrl Pts',(44.5079524583208,29.87170715524,-37.24995));
#253500=CARTESIAN_POINT('Ctrl Pts',(45.4714029967,29.87170715524,-37.1916166666667));
#253501=CARTESIAN_POINT('Ctrl Pts',(45.9531282658897,30.7060797967663,-37.1332833333334));
#253502=CARTESIAN_POINT('Ctrl Pts',(46.4348535350793,31.5404524382925,-37.07495));
#253503=CARTESIAN_POINT('Ctrl Pts',(45.9531282658897,32.3748250798187,-37.0166166666667));
#253504=CARTESIAN_POINT('Ctrl Pts',(45.8905850977848,32.4831530246427,-37.0090431559831));
#253505=CARTESIAN_POINT('Ctrl Pts',(45.8125914103809,32.5809465634453,-37.0009024189827));
#253506=CARTESIAN_POINT('Ctrl Pts',(44.5079524583208,33.6091932047179,-53.2308875));
#253507=CARTESIAN_POINT('Ctrl Pts',(43.3135644199415,33.6091932047179,-53.1725541666667));
#253508=CARTESIAN_POINT('Ctrl Pts',(42.7163704007519,32.5748228215052,-53.1142208333334));
#253509=CARTESIAN_POINT('Ctrl Pts',(42.1191763815623,31.5404524382925,-53.0558875000001));
#253510=CARTESIAN_POINT('Ctrl Pts',(42.7163704007519,30.5060820550798,-52.9975541666667));
#253511=CARTESIAN_POINT('Ctrl Pts',(43.3135644199415,29.4717116718671,-52.9392208333334));
#253512=CARTESIAN_POINT('Ctrl Pts',(44.5079524583208,29.4717116718671,-52.8808875));
#253513=CARTESIAN_POINT('Ctrl Pts',(45.7023404967,29.4717116718671,-52.8225541666667));
#253514=CARTESIAN_POINT('Ctrl Pts',(46.2995345158897,30.5060820550798,-52.7642208333334));
#253515=CARTESIAN_POINT('Ctrl Pts',(46.8967285350793,31.5404524382925,-52.7058875));
#253516=CARTESIAN_POINT('Ctrl Pts',(46.2995345158897,32.5748228215052,-52.6475541666667));
#253517=CARTESIAN_POINT('Ctrl Pts',(45.7023404967,33.6091932047179,-52.5892208333333));
#253518=CARTESIAN_POINT('Ctrl Pts',(44.5079524583208,33.6091932047179,-52.5308875));
#253519=CARTESIAN_POINT('Ctrl Pts',(43.3135644199415,33.6091932047179,-52.4725541666667));
#253520=CARTESIAN_POINT('Ctrl Pts',(42.7163704007519,32.5748228215052,-52.4142208333333));
#253521=CARTESIAN_POINT('Ctrl Pts',(42.1191763815623,31.5404524382925,-52.3558875000001));
#253522=CARTESIAN_POINT('Ctrl Pts',(42.7163704007519,30.5060820550798,-52.2975541666667));
#253523=CARTESIAN_POINT('Ctrl Pts',(43.3135644199415,29.4717116718671,-52.2392208333334));
#253524=CARTESIAN_POINT('Ctrl Pts',(44.5079524583208,29.4717116718671,-52.1808875));
#253525=CARTESIAN_POINT('Ctrl Pts',(45.7023404967,29.4717116718671,-52.1225541666667));
#253526=CARTESIAN_POINT('Ctrl Pts',(46.2995345158897,30.5060820550798,-52.0642208333334));
#253527=CARTESIAN_POINT('Ctrl Pts',(46.8967285350793,31.5404524382925,-52.0058875));
#253528=CARTESIAN_POINT('Ctrl Pts',(46.2995345158897,32.5748228215052,-51.9475541666667));
#253529=CARTESIAN_POINT('Ctrl Pts',(45.7023404967,33.6091932047179,-51.8892208333334));
#253530=CARTESIAN_POINT('Ctrl Pts',(44.5079524583208,33.6091932047179,-51.8308875));
#253531=CARTESIAN_POINT('Ctrl Pts',(43.3135644199415,33.6091932047179,-51.7725541666667));
#253532=CARTESIAN_POINT('Ctrl Pts',(42.7163704007519,32.5748228215052,-51.7142208333334));
#253533=CARTESIAN_POINT('Ctrl Pts',(42.1191763815623,31.5404524382925,-51.6558875));
#253534=CARTESIAN_POINT('Ctrl Pts',(42.7163704007519,30.5060820550798,-51.5975541666667));
#253535=CARTESIAN_POINT('Ctrl Pts',(43.3135644199415,29.4717116718671,-51.5392208333333));
#253536=CARTESIAN_POINT('Ctrl Pts',(44.5079524583208,29.4717116718671,-51.4808875));
#253537=CARTESIAN_POINT('Ctrl Pts',(45.7023404967,29.4717116718671,-51.4225541666667));
#253538=CARTESIAN_POINT('Ctrl Pts',(46.2995345158897,30.5060820550798,-51.3642208333334));
#253539=CARTESIAN_POINT('Ctrl Pts',(46.8967285350793,31.5404524382925,-51.3058875));
#253540=CARTESIAN_POINT('Ctrl Pts',(46.2995345158897,32.5748228215052,-51.2475541666667));
#253541=CARTESIAN_POINT('Ctrl Pts',(45.7023404967,33.6091932047179,-51.1892208333333));
#253542=CARTESIAN_POINT('Ctrl Pts',(44.5079524583208,33.6091932047179,-51.1308875));
#253543=CARTESIAN_POINT('Ctrl Pts',(43.3135644199415,33.6091932047179,-51.0725541666667));
#253544=CARTESIAN_POINT('Ctrl Pts',(42.7163704007519,32.5748228215052,-51.0142208333334));
#253545=CARTESIAN_POINT('Ctrl Pts',(42.1191763815623,31.5404524382925,-50.9558875));
#253546=CARTESIAN_POINT('Ctrl Pts',(42.7163704007519,30.5060820550798,-50.8975541666667));
#253547=CARTESIAN_POINT('Ctrl Pts',(43.3135644199415,29.4717116718671,-50.8392208333333));
#253548=CARTESIAN_POINT('Ctrl Pts',(44.5079524583208,29.4717116718671,-50.7808875));
#253549=CARTESIAN_POINT('Ctrl Pts',(45.7023404967,29.4717116718671,-50.7225541666666));
#253550=CARTESIAN_POINT('Ctrl Pts',(46.2995345158897,30.5060820550798,-50.6642208333333));
#253551=CARTESIAN_POINT('Ctrl Pts',(46.8967285350793,31.5404524382925,-50.6058875));
#253552=CARTESIAN_POINT('Ctrl Pts',(46.2995345158897,32.5748228215052,-50.5475541666667));
#253553=CARTESIAN_POINT('Ctrl Pts',(45.7023404967,33.6091932047179,-50.4892208333333));
#253554=CARTESIAN_POINT('Ctrl Pts',(44.5079524583208,33.6091932047179,-50.4308875));
#253555=CARTESIAN_POINT('Ctrl Pts',(43.3135644199415,33.6091932047179,-50.3725541666667));
#253556=CARTESIAN_POINT('Ctrl Pts',(42.7163704007519,32.5748228215052,-50.3142208333334));
#253557=CARTESIAN_POINT('Ctrl Pts',(42.1191763815623,31.5404524382925,-50.2558875));
#253558=CARTESIAN_POINT('Ctrl Pts',(42.7163704007519,30.5060820550798,-50.1975541666667));
#253559=CARTESIAN_POINT('Ctrl Pts',(43.3135644199415,29.4717116718671,-50.1392208333333));
#253560=CARTESIAN_POINT('Ctrl Pts',(44.5079524583208,29.4717116718671,-50.0808875));
#253561=CARTESIAN_POINT('Ctrl Pts',(45.7023404967,29.4717116718671,-50.0225541666667));
#253562=CARTESIAN_POINT('Ctrl Pts',(46.2995345158897,30.5060820550798,-49.9642208333334));
#253563=CARTESIAN_POINT('Ctrl Pts',(46.8967285350793,31.5404524382925,-49.9058875));
#253564=CARTESIAN_POINT('Ctrl Pts',(46.2995345158897,32.5748228215052,-49.8475541666667));
#253565=CARTESIAN_POINT('Ctrl Pts',(45.7023404967,33.6091932047179,-49.7892208333333));
#253566=CARTESIAN_POINT('Ctrl Pts',(44.5079524583208,33.6091932047179,-49.7308875));
#253567=CARTESIAN_POINT('Ctrl Pts',(43.3135644199415,33.6091932047179,-49.6725541666667));
#253568=CARTESIAN_POINT('Ctrl Pts',(42.7163704007519,32.5748228215052,-49.6142208333334));
#253569=CARTESIAN_POINT('Ctrl Pts',(42.1191763815623,31.5404524382925,-49.5558875));
#253570=CARTESIAN_POINT('Ctrl Pts',(42.7163704007519,30.5060820550798,-49.4975541666667));
#253571=CARTESIAN_POINT('Ctrl Pts',(43.3135644199415,29.4717116718671,-49.4392208333333));
#253572=CARTESIAN_POINT('Ctrl Pts',(44.5079524583208,29.4717116718671,-49.3808875));
#253573=CARTESIAN_POINT('Ctrl Pts',(45.7023404967,29.4717116718671,-49.3225541666667));
#253574=CARTESIAN_POINT('Ctrl Pts',(46.2995345158897,30.5060820550798,-49.2642208333334));
#253575=CARTESIAN_POINT('Ctrl Pts',(46.8967285350793,31.5404524382925,-49.2058875));
#253576=CARTESIAN_POINT('Ctrl Pts',(46.2995345158897,32.5748228215052,-49.1475541666667));
#253577=CARTESIAN_POINT('Ctrl Pts',(45.7023404967,33.6091932047179,-49.0892208333333));
#253578=CARTESIAN_POINT('Ctrl Pts',(44.5079524583208,33.6091932047179,-49.0308875));
#253579=CARTESIAN_POINT('Ctrl Pts',(43.3135644199415,33.6091932047179,-48.9725541666667));
#253580=CARTESIAN_POINT('Ctrl Pts',(42.7163704007519,32.5748228215052,-48.9142208333333));
#253581=CARTESIAN_POINT('Ctrl Pts',(42.1191763815623,31.5404524382925,-48.8558875));
#253582=CARTESIAN_POINT('Ctrl Pts',(42.7163704007519,30.5060820550798,-48.7975541666667));
#253583=CARTESIAN_POINT('Ctrl Pts',(43.3135644199415,29.4717116718671,-48.7392208333334));
#253584=CARTESIAN_POINT('Ctrl Pts',(44.5079524583208,29.4717116718671,-48.6808875));
#253585=CARTESIAN_POINT('Ctrl Pts',(45.7023404967,29.4717116718671,-48.6225541666667));
#253586=CARTESIAN_POINT('Ctrl Pts',(46.2995345158897,30.5060820550798,-48.5642208333334));
#253587=CARTESIAN_POINT('Ctrl Pts',(46.8967285350793,31.5404524382925,-48.5058875));
#253588=CARTESIAN_POINT('Ctrl Pts',(46.2995345158897,32.5748228215052,-48.4475541666667));
#253589=CARTESIAN_POINT('Ctrl Pts',(45.7023404967,33.6091932047179,-48.3892208333334));
#253590=CARTESIAN_POINT('Ctrl Pts',(44.5079524583208,33.6091932047179,-48.3308875));
#253591=CARTESIAN_POINT('Ctrl Pts',(43.3135644199415,33.6091932047179,-48.2725541666667));
#253592=CARTESIAN_POINT('Ctrl Pts',(42.7163704007519,32.5748228215052,-48.2142208333334));
#253593=CARTESIAN_POINT('Ctrl Pts',(42.1191763815623,31.5404524382925,-48.1558875));
#253594=CARTESIAN_POINT('Ctrl Pts',(42.7163704007519,30.5060820550798,-48.0975541666667));
#253595=CARTESIAN_POINT('Ctrl Pts',(43.3135644199415,29.4717116718671,-48.0392208333334));
#253596=CARTESIAN_POINT('Ctrl Pts',(44.5079524583208,29.4717116718671,-47.9808875));
#253597=CARTESIAN_POINT('Ctrl Pts',(45.7023404967,29.4717116718671,-47.9225541666667));
#253598=CARTESIAN_POINT('Ctrl Pts',(46.2995345158897,30.5060820550798,-47.8642208333334));
#253599=CARTESIAN_POINT('Ctrl Pts',(46.8967285350793,31.5404524382925,-47.8058875000001));
#253600=CARTESIAN_POINT('Ctrl Pts',(46.2995345158897,32.5748228215052,-47.7475541666667));
#253601=CARTESIAN_POINT('Ctrl Pts',(45.7023404967,33.6091932047179,-47.6892208333334));
#253602=CARTESIAN_POINT('Ctrl Pts',(44.5079524583208,33.6091932047179,-47.6308875));
#253603=CARTESIAN_POINT('Ctrl Pts',(43.3135644199415,33.6091932047179,-47.5725541666667));
#253604=CARTESIAN_POINT('Ctrl Pts',(42.7163704007519,32.5748228215052,-47.5142208333333));
#253605=CARTESIAN_POINT('Ctrl Pts',(42.1191763815623,31.5404524382925,-47.4558875));
#253606=CARTESIAN_POINT('Ctrl Pts',(42.7163704007519,30.5060820550798,-47.3975541666667));
#253607=CARTESIAN_POINT('Ctrl Pts',(43.3135644199415,29.4717116718671,-47.3392208333333));
#253608=CARTESIAN_POINT('Ctrl Pts',(44.5079524583208,29.4717116718671,-47.2808875));
#253609=CARTESIAN_POINT('Ctrl Pts',(45.7023404967,29.4717116718671,-47.2225541666667));
#253610=CARTESIAN_POINT('Ctrl Pts',(46.2995345158897,30.5060820550798,-47.1642208333334));
#253611=CARTESIAN_POINT('Ctrl Pts',(46.8967285350793,31.5404524382925,-47.1058875));
#253612=CARTESIAN_POINT('Ctrl Pts',(46.2995345158897,32.5748228215052,-47.0475541666667));
#253613=CARTESIAN_POINT('Ctrl Pts',(45.7023404967,33.6091932047179,-46.9892208333334));
#253614=CARTESIAN_POINT('Ctrl Pts',(44.5079524583208,33.6091932047179,-46.9308875));
#253615=CARTESIAN_POINT('Ctrl Pts',(43.3135644199415,33.6091932047179,-46.8725541666667));
#253616=CARTESIAN_POINT('Ctrl Pts',(42.7163704007519,32.5748228215052,-46.8142208333334));
#253617=CARTESIAN_POINT('Ctrl Pts',(42.1191763815623,31.5404524382925,-46.7558875));
#253618=CARTESIAN_POINT('Ctrl Pts',(42.7163704007519,30.5060820550798,-46.6975541666667));
#253619=CARTESIAN_POINT('Ctrl Pts',(43.3135644199415,29.4717116718671,-46.6392208333333));
#253620=CARTESIAN_POINT('Ctrl Pts',(44.5079524583208,29.4717116718671,-46.5808875));
#253621=CARTESIAN_POINT('Ctrl Pts',(45.7023404967,29.4717116718671,-46.5225541666667));
#253622=CARTESIAN_POINT('Ctrl Pts',(46.2995345158897,30.5060820550798,-46.4642208333334));
#253623=CARTESIAN_POINT('Ctrl Pts',(46.8967285350793,31.5404524382925,-46.4058875));
#253624=CARTESIAN_POINT('Ctrl Pts',(46.2995345158897,32.5748228215052,-46.3475541666667));
#253625=CARTESIAN_POINT('Ctrl Pts',(45.7023404967,33.6091932047179,-46.2892208333334));
#253626=CARTESIAN_POINT('Ctrl Pts',(44.5079524583208,33.6091932047179,-46.2308875));
#253627=CARTESIAN_POINT('Ctrl Pts',(43.3135644199415,33.6091932047179,-46.1725541666667));
#253628=CARTESIAN_POINT('Ctrl Pts',(42.7163704007519,32.5748228215052,-46.1142208333334));
#253629=CARTESIAN_POINT('Ctrl Pts',(42.1191763815623,31.5404524382925,-46.0558875));
#253630=CARTESIAN_POINT('Ctrl Pts',(42.7163704007519,30.5060820550798,-45.9975541666667));
#253631=CARTESIAN_POINT('Ctrl Pts',(43.3135644199415,29.4717116718671,-45.9392208333333));
#253632=CARTESIAN_POINT('Ctrl Pts',(44.5079524583208,29.4717116718671,-45.8808875));
#253633=CARTESIAN_POINT('Ctrl Pts',(45.7023404967,29.4717116718671,-45.8225541666667));
#253634=CARTESIAN_POINT('Ctrl Pts',(46.2995345158897,30.5060820550798,-45.7642208333334));
#253635=CARTESIAN_POINT('Ctrl Pts',(46.8967285350793,31.5404524382925,-45.7058875));
#253636=CARTESIAN_POINT('Ctrl Pts',(46.2995345158897,32.5748228215052,-45.6475541666667));
#253637=CARTESIAN_POINT('Ctrl Pts',(45.7023404967,33.6091932047179,-45.5892208333333));
#253638=CARTESIAN_POINT('Ctrl Pts',(44.5079524583208,33.6091932047179,-45.5308875));
#253639=CARTESIAN_POINT('Ctrl Pts',(43.3135644199415,33.6091932047179,-45.4725541666667));
#253640=CARTESIAN_POINT('Ctrl Pts',(42.7163704007519,32.5748228215052,-45.4142208333334));
#253641=CARTESIAN_POINT('Ctrl Pts',(42.1191763815623,31.5404524382925,-45.3558875));
#253642=CARTESIAN_POINT('Ctrl Pts',(42.7163704007519,30.5060820550798,-45.2975541666667));
#253643=CARTESIAN_POINT('Ctrl Pts',(43.3135644199415,29.4717116718671,-45.2392208333333));
#253644=CARTESIAN_POINT('Ctrl Pts',(44.5079524583208,29.4717116718671,-45.1808875));
#253645=CARTESIAN_POINT('Ctrl Pts',(45.7023404967,29.4717116718671,-45.1225541666667));
#253646=CARTESIAN_POINT('Ctrl Pts',(46.2995345158897,30.5060820550798,-45.0642208333334));
#253647=CARTESIAN_POINT('Ctrl Pts',(46.8967285350793,31.5404524382925,-45.0058875));
#253648=CARTESIAN_POINT('Ctrl Pts',(46.2995345158897,32.5748228215052,-44.9475541666667));
#253649=CARTESIAN_POINT('Ctrl Pts',(45.7023404967,33.6091932047179,-44.8892208333333));
#253650=CARTESIAN_POINT('Ctrl Pts',(44.5079524583208,33.6091932047179,-44.8308875));
#253651=CARTESIAN_POINT('Ctrl Pts',(43.3135644199415,33.6091932047179,-44.7725541666666));
#253652=CARTESIAN_POINT('Ctrl Pts',(42.7163704007519,32.5748228215052,-44.7142208333334));
#253653=CARTESIAN_POINT('Ctrl Pts',(42.1191763815623,31.5404524382925,-44.6558875));
#253654=CARTESIAN_POINT('Ctrl Pts',(42.7163704007519,30.5060820550798,-44.5975541666667));
#253655=CARTESIAN_POINT('Ctrl Pts',(43.3135644199415,29.4717116718671,-44.5392208333333));
#253656=CARTESIAN_POINT('Ctrl Pts',(44.5079524583208,29.4717116718671,-44.4808875));
#253657=CARTESIAN_POINT('Ctrl Pts',(45.7023404967,29.4717116718671,-44.4225541666667));
#253658=CARTESIAN_POINT('Ctrl Pts',(46.2995345158897,30.5060820550798,-44.3642208333333));
#253659=CARTESIAN_POINT('Ctrl Pts',(46.8967285350793,31.5404524382925,-44.3058875));
#253660=CARTESIAN_POINT('Ctrl Pts',(46.2995345158897,32.5748228215052,-44.2475541666667));
#253661=CARTESIAN_POINT('Ctrl Pts',(45.7023404967,33.6091932047179,-44.1892208333334));
#253662=CARTESIAN_POINT('Ctrl Pts',(44.5079524583208,33.6091932047179,-44.1308875));
#253663=CARTESIAN_POINT('Ctrl Pts',(43.3135644199415,33.6091932047179,-44.0725541666667));
#253664=CARTESIAN_POINT('Ctrl Pts',(42.7163704007519,32.5748228215052,-44.0142208333334));
#253665=CARTESIAN_POINT('Ctrl Pts',(42.1191763815623,31.5404524382925,-43.9558875));
#253666=CARTESIAN_POINT('Ctrl Pts',(42.7163704007519,30.5060820550798,-43.8975541666667));
#253667=CARTESIAN_POINT('Ctrl Pts',(43.3135644199415,29.4717116718671,-43.8392208333333));
#253668=CARTESIAN_POINT('Ctrl Pts',(44.5079524583208,29.4717116718671,-43.7808875));
#253669=CARTESIAN_POINT('Ctrl Pts',(45.7023404967,29.4717116718671,-43.7225541666667));
#253670=CARTESIAN_POINT('Ctrl Pts',(46.2995345158897,30.5060820550798,-43.6642208333334));
#253671=CARTESIAN_POINT('Ctrl Pts',(46.8967285350793,31.5404524382925,-43.6058875));
#253672=CARTESIAN_POINT('Ctrl Pts',(46.2995345158897,32.5748228215052,-43.5475541666667));
#253673=CARTESIAN_POINT('Ctrl Pts',(45.7023404967,33.6091932047179,-43.4892208333333));
#253674=CARTESIAN_POINT('Ctrl Pts',(44.5079524583208,33.6091932047179,-43.4308875));
#253675=CARTESIAN_POINT('Ctrl Pts',(43.3135644199415,33.6091932047179,-43.3725541666667));
#253676=CARTESIAN_POINT('Ctrl Pts',(42.7163704007519,32.5748228215052,-43.3142208333334));
#253677=CARTESIAN_POINT('Ctrl Pts',(42.1191763815623,31.5404524382925,-43.2558875));
#253678=CARTESIAN_POINT('Ctrl Pts',(42.7163704007519,30.5060820550798,-43.1975541666667));
#253679=CARTESIAN_POINT('Ctrl Pts',(43.3135644199415,29.4717116718671,-43.1392208333334));
#253680=CARTESIAN_POINT('Ctrl Pts',(44.5079524583208,29.4717116718671,-43.0808875));
#253681=CARTESIAN_POINT('Ctrl Pts',(45.7023404967,29.4717116718671,-43.0225541666667));
#253682=CARTESIAN_POINT('Ctrl Pts',(46.2995345158897,30.5060820550798,-42.9642208333334));
#253683=CARTESIAN_POINT('Ctrl Pts',(46.8967285350793,31.5404524382925,-42.9058875));
#253684=CARTESIAN_POINT('Ctrl Pts',(46.2995345158897,32.5748228215052,-42.8475541666667));
#253685=CARTESIAN_POINT('Ctrl Pts',(45.7023404967,33.6091932047179,-42.7892208333334));
#253686=CARTESIAN_POINT('Ctrl Pts',(44.5079524583208,33.6091932047179,-42.7308875));
#253687=CARTESIAN_POINT('Ctrl Pts',(43.3135644199415,33.6091932047179,-42.6725541666667));
#253688=CARTESIAN_POINT('Ctrl Pts',(42.7163704007519,32.5748228215052,-42.6142208333334));
#253689=CARTESIAN_POINT('Ctrl Pts',(42.1191763815623,31.5404524382925,-42.5558875));
#253690=CARTESIAN_POINT('Ctrl Pts',(42.7163704007519,30.5060820550798,-42.4975541666667));
#253691=CARTESIAN_POINT('Ctrl Pts',(43.3135644199415,29.4717116718671,-42.4392208333334));
#253692=CARTESIAN_POINT('Ctrl Pts',(44.5079524583208,29.4717116718671,-42.3808875));
#253693=CARTESIAN_POINT('Ctrl Pts',(45.7023404967,29.4717116718671,-42.3225541666667));
#253694=CARTESIAN_POINT('Ctrl Pts',(46.2995345158897,30.5060820550798,-42.2642208333334));
#253695=CARTESIAN_POINT('Ctrl Pts',(46.8967285350793,31.5404524382925,-42.2058875));
#253696=CARTESIAN_POINT('Ctrl Pts',(46.2995345158897,32.5748228215052,-42.1475541666667));
#253697=CARTESIAN_POINT('Ctrl Pts',(45.7023404967,33.6091932047179,-42.0892208333333));
#253698=CARTESIAN_POINT('Ctrl Pts',(44.5079524583208,33.6091932047179,-42.0308875));
#253699=CARTESIAN_POINT('Ctrl Pts',(43.3135644199415,33.6091932047179,-41.9725541666667));
#253700=CARTESIAN_POINT('Ctrl Pts',(42.7163704007519,32.5748228215052,-41.9142208333334));
#253701=CARTESIAN_POINT('Ctrl Pts',(42.1191763815623,31.5404524382925,-41.8558875));
#253702=CARTESIAN_POINT('Ctrl Pts',(42.7163704007519,30.5060820550798,-41.7975541666667));
#253703=CARTESIAN_POINT('Ctrl Pts',(43.3135644199415,29.4717116718671,-41.7392208333333));
#253704=CARTESIAN_POINT('Ctrl Pts',(44.5079524583208,29.4717116718671,-41.6808875));
#253705=CARTESIAN_POINT('Ctrl Pts',(45.7023404967,29.4717116718671,-41.6225541666667));
#253706=CARTESIAN_POINT('Ctrl Pts',(46.2995345158897,30.5060820550798,-41.5642208333334));
#253707=CARTESIAN_POINT('Ctrl Pts',(46.8967285350793,31.5404524382925,-41.5058875));
#253708=CARTESIAN_POINT('Ctrl Pts',(46.2995345158897,32.5748228215052,-41.4475541666667));
#253709=CARTESIAN_POINT('Ctrl Pts',(45.7023404967,33.6091932047179,-41.3892208333333));
#253710=CARTESIAN_POINT('Ctrl Pts',(44.5079524583208,33.6091932047179,-41.3308875));
#253711=CARTESIAN_POINT('Ctrl Pts',(43.3135644199415,33.6091932047179,-41.2725541666667));
#253712=CARTESIAN_POINT('Ctrl Pts',(42.7163704007519,32.5748228215052,-41.2142208333333));
#253713=CARTESIAN_POINT('Ctrl Pts',(42.1191763815623,31.5404524382925,-41.1558875));
#253714=CARTESIAN_POINT('Ctrl Pts',(42.7163704007519,30.5060820550798,-41.0975541666667));
#253715=CARTESIAN_POINT('Ctrl Pts',(43.3135644199415,29.4717116718671,-41.0392208333333));
#253716=CARTESIAN_POINT('Ctrl Pts',(44.5079524583208,29.4717116718671,-40.9808875));
#253717=CARTESIAN_POINT('Ctrl Pts',(45.7023404967,29.4717116718671,-40.9225541666667));
#253718=CARTESIAN_POINT('Ctrl Pts',(46.2995345158897,30.5060820550798,-40.8642208333334));
#253719=CARTESIAN_POINT('Ctrl Pts',(46.8967285350793,31.5404524382925,-40.8058875));
#253720=CARTESIAN_POINT('Ctrl Pts',(46.2995345158897,32.5748228215052,-40.7475541666667));
#253721=CARTESIAN_POINT('Ctrl Pts',(45.7023404967,33.6091932047179,-40.6892208333333));
#253722=CARTESIAN_POINT('Ctrl Pts',(44.5079524583208,33.6091932047179,-40.6308875));
#253723=CARTESIAN_POINT('Ctrl Pts',(43.3135644199415,33.6091932047179,-40.5725541666667));
#253724=CARTESIAN_POINT('Ctrl Pts',(42.7163704007519,32.5748228215052,-40.5142208333333));
#253725=CARTESIAN_POINT('Ctrl Pts',(42.1191763815623,31.5404524382925,-40.4558875));
#253726=CARTESIAN_POINT('Ctrl Pts',(42.7163704007519,30.5060820550798,-40.3975541666667));
#253727=CARTESIAN_POINT('Ctrl Pts',(43.3135644199415,29.4717116718671,-40.3392208333333));
#253728=CARTESIAN_POINT('Ctrl Pts',(44.5079524583208,29.4717116718671,-40.2808875));
#253729=CARTESIAN_POINT('Ctrl Pts',(45.7023404967,29.4717116718671,-40.2225541666667));
#253730=CARTESIAN_POINT('Ctrl Pts',(46.2995345158897,30.5060820550798,-40.1642208333333));
#253731=CARTESIAN_POINT('Ctrl Pts',(46.8967285350793,31.5404524382925,-40.1058875));
#253732=CARTESIAN_POINT('Ctrl Pts',(46.2995345158897,32.5748228215052,-40.0475541666667));
#253733=CARTESIAN_POINT('Ctrl Pts',(45.7023404967,33.6091932047179,-39.9892208333333));
#253734=CARTESIAN_POINT('Ctrl Pts',(44.5079524583208,33.6091932047179,-39.9308875));
#253735=CARTESIAN_POINT('Ctrl Pts',(43.3135644199415,33.6091932047179,-39.8725541666667));
#253736=CARTESIAN_POINT('Ctrl Pts',(42.7163704007519,32.5748228215052,-39.8142208333334));
#253737=CARTESIAN_POINT('Ctrl Pts',(42.1191763815623,31.5404524382925,-39.7558875));
#253738=CARTESIAN_POINT('Ctrl Pts',(42.7163704007519,30.5060820550798,-39.6975541666667));
#253739=CARTESIAN_POINT('Ctrl Pts',(43.3135644199415,29.4717116718671,-39.6392208333334));
#253740=CARTESIAN_POINT('Ctrl Pts',(44.5079524583208,29.4717116718671,-39.5808875));
#253741=CARTESIAN_POINT('Ctrl Pts',(45.7023404967,29.4717116718671,-39.5225541666667));
#253742=CARTESIAN_POINT('Ctrl Pts',(46.2995345158897,30.5060820550798,-39.4642208333333));
#253743=CARTESIAN_POINT('Ctrl Pts',(46.8967285350793,31.5404524382925,-39.4058875));
#253744=CARTESIAN_POINT('Ctrl Pts',(46.2995345158897,32.5748228215052,-39.3475541666667));
#253745=CARTESIAN_POINT('Ctrl Pts',(45.7023404967,33.6091932047179,-39.2892208333334));
#253746=CARTESIAN_POINT('Ctrl Pts',(44.5079524583208,33.6091932047179,-39.2308875));
#253747=CARTESIAN_POINT('Ctrl Pts',(43.3135644199415,33.6091932047179,-39.1725541666667));
#253748=CARTESIAN_POINT('Ctrl Pts',(42.7163704007519,32.5748228215052,-39.1142208333333));
#253749=CARTESIAN_POINT('Ctrl Pts',(42.1191763815623,31.5404524382925,-39.0558875));
#253750=CARTESIAN_POINT('Ctrl Pts',(42.7163704007519,30.5060820550798,-38.9975541666667));
#253751=CARTESIAN_POINT('Ctrl Pts',(43.3135644199415,29.4717116718671,-38.9392208333334));
#253752=CARTESIAN_POINT('Ctrl Pts',(44.5079524583208,29.4717116718671,-38.8808875));
#253753=CARTESIAN_POINT('Ctrl Pts',(45.7023404967,29.4717116718671,-38.8225541666667));
#253754=CARTESIAN_POINT('Ctrl Pts',(46.2995345158897,30.5060820550798,-38.7642208333333));
#253755=CARTESIAN_POINT('Ctrl Pts',(46.8967285350793,31.5404524382925,-38.7058875));
#253756=CARTESIAN_POINT('Ctrl Pts',(46.2995345158897,32.5748228215052,-38.6475541666667));
#253757=CARTESIAN_POINT('Ctrl Pts',(45.7023404967,33.6091932047179,-38.5892208333334));
#253758=CARTESIAN_POINT('Ctrl Pts',(44.5079524583208,33.6091932047179,-38.5308875));
#253759=CARTESIAN_POINT('Ctrl Pts',(43.3135644199415,33.6091932047179,-38.4725541666667));
#253760=CARTESIAN_POINT('Ctrl Pts',(42.7163704007519,32.5748228215052,-38.4142208333334));
#253761=CARTESIAN_POINT('Ctrl Pts',(42.1191763815623,31.5404524382925,-38.3558875));
#253762=CARTESIAN_POINT('Ctrl Pts',(42.7163704007519,30.5060820550798,-38.2975541666667));
#253763=CARTESIAN_POINT('Ctrl Pts',(43.3135644199415,29.4717116718671,-38.2392208333333));
#253764=CARTESIAN_POINT('Ctrl Pts',(44.5079524583208,29.4717116718671,-38.1808875));
#253765=CARTESIAN_POINT('Ctrl Pts',(45.7023404967,29.4717116718671,-38.1225541666667));
#253766=CARTESIAN_POINT('Ctrl Pts',(46.2995345158897,30.5060820550798,-38.0642208333334));
#253767=CARTESIAN_POINT('Ctrl Pts',(46.8967285350793,31.5404524382925,-38.0058875));
#253768=CARTESIAN_POINT('Ctrl Pts',(46.2995345158897,32.5748228215052,-37.9475541666667));
#253769=CARTESIAN_POINT('Ctrl Pts',(45.7023404967,33.6091932047179,-37.8892208333334));
#253770=CARTESIAN_POINT('Ctrl Pts',(44.5079524583208,33.6091932047179,-37.8308875));
#253771=CARTESIAN_POINT('Ctrl Pts',(43.3135644199415,33.6091932047179,-37.7725541666667));
#253772=CARTESIAN_POINT('Ctrl Pts',(42.7163704007519,32.5748228215052,-37.7142208333333));
#253773=CARTESIAN_POINT('Ctrl Pts',(42.1191763815623,31.5404524382925,-37.6558875));
#253774=CARTESIAN_POINT('Ctrl Pts',(42.7163704007519,30.5060820550798,-37.5975541666667));
#253775=CARTESIAN_POINT('Ctrl Pts',(43.3135644199415,29.4717116718671,-37.5392208333334));
#253776=CARTESIAN_POINT('Ctrl Pts',(44.5079524583208,29.4717116718671,-37.4808875));
#253777=CARTESIAN_POINT('Ctrl Pts',(45.7023404967,29.4717116718671,-37.4225541666667));
#253778=CARTESIAN_POINT('Ctrl Pts',(46.2995345158897,30.5060820550798,-37.3642208333333));
#253779=CARTESIAN_POINT('Ctrl Pts',(46.8967285350793,31.5404524382925,-37.3058875));
#253780=CARTESIAN_POINT('Ctrl Pts',(46.2995345158897,32.5748228215052,-37.2475541666667));
#253781=CARTESIAN_POINT('Ctrl Pts',(46.2219998538691,32.7091167954726,-37.239980655983));
#253782=CARTESIAN_POINT('Ctrl Pts',(46.1253112086366,32.8303512837246,-37.2318399189827));
#253783=CARTESIAN_POINT('',(44.6028101950443,33.5382023184728,-39.8960584192517));
#253784=CARTESIAN_POINT('Ctrl Pts',(44.5079524583207,29.5404524382925,-39.5412));
#253785=CARTESIAN_POINT('Ctrl Pts',(44.4819640599349,29.5404524382925,-39.5425128857704));
#253786=CARTESIAN_POINT('Ctrl Pts',(44.4559582185953,29.5409589821351,-39.5438414269218));
#253787=CARTESIAN_POINT('Ctrl Pts',(44.1649835932381,29.5523160589081,-39.5588721743436));
#253788=CARTESIAN_POINT('Ctrl Pts',(43.9047498818082,29.6152478208572,-39.5738542093599));
#253789=CARTESIAN_POINT('Ctrl Pts',(43.4288502962916,29.8366243048529,-39.6043525894344));
#253790=CARTESIAN_POINT('Ctrl Pts',(43.2168722113724,29.9910586609984,-39.6195656652062));
#253791=CARTESIAN_POINT('Ctrl Pts',(42.8673886165607,30.3685431738061,-39.648230894323));
#253792=CARTESIAN_POINT('Ctrl Pts',(42.7317086737687,30.5866318895618,-39.6605604679907));
#253793=CARTESIAN_POINT('Ctrl Pts',(42.5449531333681,31.0736341008157,-39.6889689303139));
#253794=CARTESIAN_POINT('Ctrl Pts',(42.5002450908835,31.3395359025595,-39.7044798687489));
#253795=CARTESIAN_POINT('Ctrl Pts',(42.5174955965406,31.8629669597781,-39.7350133470867));
#253796=CARTESIAN_POINT('Ctrl Pts',(42.5752997723599,32.1156243266577,-39.749751693488));
#253797=CARTESIAN_POINT('Ctrl Pts',(42.7849619712644,32.5889458204941,-39.7773621139617));
#253798=CARTESIAN_POINT('Ctrl Pts',(42.9362187959742,32.8044575732572,-39.7903324084612));
#253799=CARTESIAN_POINT('Ctrl Pts',(43.3150542526911,33.1672635258398,-39.8200523146249));
#253800=CARTESIAN_POINT('Ctrl Pts',(43.5396719441365,33.3101828782814,-39.8355680656421));
#253801=CARTESIAN_POINT('Ctrl Pts',(43.917558345171,33.4565640653462,-39.8589276382755));
#253802=CARTESIAN_POINT('Ctrl Pts',(44.0546632593971,33.4935486751892,-39.8669326424869));
#253803=CARTESIAN_POINT('Ctrl Pts',(44.3295436040989,33.5371640157393,-39.8820912026746));
#253804=CARTESIAN_POINT('Ctrl Pts',(44.4663202768198,33.5446825305706,-39.8889734415788));
#253805=CARTESIAN_POINT('Ctrl Pts',(44.602810202553,33.5382016738972,-39.8960576849095));
#253806=CARTESIAN_POINT('Ctrl Pts',(42.8533186609868,32.1498328366219,-39.6198492128429));
#253807=CARTESIAN_POINT('Ctrl Pts',(42.9050935173468,32.3330539516136,-39.6401425936059));
#253808=CARTESIAN_POINT('Ctrl Pts',(42.982691066735,32.5080524772143,-39.6607364267285));
#253809=CARTESIAN_POINT('Ctrl Pts',(43.2002172353721,32.8455798638486,-39.7078850703729));
#253810=CARTESIAN_POINT('Ctrl Pts',(43.3395359031206,32.9998044792065,-39.7334291314113));
#253811=CARTESIAN_POINT('Ctrl Pts',(43.648144630106,33.246187293655,-39.7824493941379));
#253812=CARTESIAN_POINT('Ctrl Pts',(43.812496663251,33.3413573589809,-39.8056860731073));
#253813=CARTESIAN_POINT('Ctrl Pts',(44.1843827211634,33.4874274508034,-39.8525699812779));
#253814=CARTESIAN_POINT('Ctrl Pts',(44.3929618843463,33.5311592418717,-39.8754000806208));
#253815=CARTESIAN_POINT('Ctrl Pts',(44.6028101816435,33.5382028669661,-39.8960583683639));
#253816=CARTESIAN_POINT('Ctrl Pts',(44.5079524583208,33.2091977213449,-52.99995));
#253817=CARTESIAN_POINT('Ctrl Pts',(43.5445019199415,33.2091977213449,-52.9416166666667));
#253818=CARTESIAN_POINT('Ctrl Pts',(43.0627766507519,32.3748250798187,-52.8832833333334));
#253819=CARTESIAN_POINT('Ctrl Pts',(42.5810513815623,31.5404524382925,-52.82495));
#253820=CARTESIAN_POINT('Ctrl Pts',(43.0627766507519,30.7060797967663,-52.7666166666667));
#253821=CARTESIAN_POINT('Ctrl Pts',(43.5445019199415,29.87170715524,-52.7082833333333));
#253822=CARTESIAN_POINT('Ctrl Pts',(44.5079524583208,29.87170715524,-52.64995));
#253823=CARTESIAN_POINT('Ctrl Pts',(45.4714029967,29.87170715524,-52.5916166666666));
#253824=CARTESIAN_POINT('Ctrl Pts',(45.9531282658897,30.7060797967663,-52.5332833333334));
#253825=CARTESIAN_POINT('Ctrl Pts',(46.4348535350793,31.5404524382925,-52.4749500000001));
#253826=CARTESIAN_POINT('Ctrl Pts',(45.9531282658897,32.3748250798187,-52.4166166666667));
#253827=CARTESIAN_POINT('Ctrl Pts',(45.4714029967,33.2091977213449,-52.3582833333334));
#253828=CARTESIAN_POINT('Ctrl Pts',(44.5079524583208,33.2091977213449,-52.29995));
#253829=CARTESIAN_POINT('Ctrl Pts',(43.5445019199415,33.2091977213449,-52.2416166666667));
#253830=CARTESIAN_POINT('Ctrl Pts',(43.0627766507519,32.3748250798187,-52.1832833333333));
#253831=CARTESIAN_POINT('Ctrl Pts',(42.5810513815623,31.5404524382925,-52.12495));
#253832=CARTESIAN_POINT('Ctrl Pts',(43.0627766507519,30.7060797967663,-52.0666166666667));
#253833=CARTESIAN_POINT('Ctrl Pts',(43.5445019199415,29.87170715524,-52.0082833333333));
#253834=CARTESIAN_POINT('Ctrl Pts',(44.5079524583208,29.87170715524,-51.94995));
#253835=CARTESIAN_POINT('Ctrl Pts',(45.4714029967,29.87170715524,-51.8916166666667));
#253836=CARTESIAN_POINT('Ctrl Pts',(45.9531282658897,30.7060797967663,-51.8332833333333));
#253837=CARTESIAN_POINT('Ctrl Pts',(46.4348535350793,31.5404524382925,-51.77495));
#253838=CARTESIAN_POINT('Ctrl Pts',(45.9531282658897,32.3748250798187,-51.7166166666667));
#253839=CARTESIAN_POINT('Ctrl Pts',(45.4714029967,33.2091977213449,-51.6582833333333));
#253840=CARTESIAN_POINT('Ctrl Pts',(44.5079524583208,33.2091977213449,-51.59995));
#253841=CARTESIAN_POINT('Ctrl Pts',(43.5445019199415,33.2091977213449,-51.5416166666667));
#253842=CARTESIAN_POINT('Ctrl Pts',(43.0627766507519,32.3748250798187,-51.4832833333333));
#253843=CARTESIAN_POINT('Ctrl Pts',(42.5810513815623,31.5404524382925,-51.42495));
#253844=CARTESIAN_POINT('Ctrl Pts',(43.0627766507519,30.7060797967663,-51.3666166666667));
#253845=CARTESIAN_POINT('Ctrl Pts',(43.5445019199415,29.87170715524,-51.3082833333333));
#253846=CARTESIAN_POINT('Ctrl Pts',(44.5079524583208,29.87170715524,-51.24995));
#253847=CARTESIAN_POINT('Ctrl Pts',(45.4714029967,29.87170715524,-51.1916166666667));
#253848=CARTESIAN_POINT('Ctrl Pts',(45.9531282658897,30.7060797967663,-51.1332833333333));
#253849=CARTESIAN_POINT('Ctrl Pts',(46.4348535350793,31.5404524382925,-51.07495));
#253850=CARTESIAN_POINT('Ctrl Pts',(45.9531282658897,32.3748250798187,-51.0166166666667));
#253851=CARTESIAN_POINT('Ctrl Pts',(45.4714029967,33.2091977213449,-50.9582833333334));
#253852=CARTESIAN_POINT('Ctrl Pts',(44.5079524583208,33.2091977213449,-50.89995));
#253853=CARTESIAN_POINT('Ctrl Pts',(43.5445019199415,33.2091977213449,-50.8416166666667));
#253854=CARTESIAN_POINT('Ctrl Pts',(43.0627766507519,32.3748250798187,-50.7832833333333));
#253855=CARTESIAN_POINT('Ctrl Pts',(42.5810513815623,31.5404524382925,-50.72495));
#253856=CARTESIAN_POINT('Ctrl Pts',(43.0627766507519,30.7060797967663,-50.6666166666667));
#253857=CARTESIAN_POINT('Ctrl Pts',(43.5445019199415,29.87170715524,-50.6082833333334));
#253858=CARTESIAN_POINT('Ctrl Pts',(44.5079524583208,29.87170715524,-50.54995));
#253859=CARTESIAN_POINT('Ctrl Pts',(45.4714029967,29.87170715524,-50.4916166666667));
#253860=CARTESIAN_POINT('Ctrl Pts',(45.9531282658897,30.7060797967663,-50.4332833333333));
#253861=CARTESIAN_POINT('Ctrl Pts',(46.4348535350793,31.5404524382925,-50.37495));
#253862=CARTESIAN_POINT('Ctrl Pts',(45.9531282658897,32.3748250798187,-50.3166166666667));
#253863=CARTESIAN_POINT('Ctrl Pts',(45.4714029967,33.2091977213449,-50.2582833333334));
#253864=CARTESIAN_POINT('Ctrl Pts',(44.5079524583208,33.2091977213449,-50.19995));
#253865=CARTESIAN_POINT('Ctrl Pts',(43.5445019199415,33.2091977213449,-50.1416166666667));
#253866=CARTESIAN_POINT('Ctrl Pts',(43.0627766507519,32.3748250798187,-50.0832833333333));
#253867=CARTESIAN_POINT('Ctrl Pts',(42.5810513815623,31.5404524382925,-50.02495));
#253868=CARTESIAN_POINT('Ctrl Pts',(43.0627766507519,30.7060797967663,-49.9666166666667));
#253869=CARTESIAN_POINT('Ctrl Pts',(43.5445019199415,29.87170715524,-49.9082833333334));
#253870=CARTESIAN_POINT('Ctrl Pts',(44.5079524583208,29.87170715524,-49.84995));
#253871=CARTESIAN_POINT('Ctrl Pts',(45.4714029967,29.87170715524,-49.7916166666667));
#253872=CARTESIAN_POINT('Ctrl Pts',(45.9531282658897,30.7060797967663,-49.7332833333333));
#253873=CARTESIAN_POINT('Ctrl Pts',(46.4348535350793,31.5404524382925,-49.67495));
#253874=CARTESIAN_POINT('Ctrl Pts',(45.9531282658897,32.3748250798187,-49.6166166666667));
#253875=CARTESIAN_POINT('Ctrl Pts',(45.4714029967,33.2091977213449,-49.5582833333334));
#253876=CARTESIAN_POINT('Ctrl Pts',(44.5079524583208,33.2091977213449,-49.49995));
#253877=CARTESIAN_POINT('Ctrl Pts',(43.5445019199415,33.2091977213449,-49.4416166666667));
#253878=CARTESIAN_POINT('Ctrl Pts',(43.0627766507519,32.3748250798187,-49.3832833333334));
#253879=CARTESIAN_POINT('Ctrl Pts',(42.5810513815623,31.5404524382925,-49.32495));
#253880=CARTESIAN_POINT('Ctrl Pts',(43.0627766507519,30.7060797967663,-49.2666166666667));
#253881=CARTESIAN_POINT('Ctrl Pts',(43.5445019199415,29.87170715524,-49.2082833333334));
#253882=CARTESIAN_POINT('Ctrl Pts',(44.5079524583208,29.87170715524,-49.14995));
#253883=CARTESIAN_POINT('Ctrl Pts',(45.4714029967,29.87170715524,-49.0916166666667));
#253884=CARTESIAN_POINT('Ctrl Pts',(45.9531282658897,30.7060797967663,-49.0332833333333));
#253885=CARTESIAN_POINT('Ctrl Pts',(46.4348535350793,31.5404524382925,-48.97495));
#253886=CARTESIAN_POINT('Ctrl Pts',(45.9531282658897,32.3748250798187,-48.9166166666667));
#253887=CARTESIAN_POINT('Ctrl Pts',(45.4714029967,33.2091977213449,-48.8582833333333));
#253888=CARTESIAN_POINT('Ctrl Pts',(44.5079524583208,33.2091977213449,-48.79995));
#253889=CARTESIAN_POINT('Ctrl Pts',(43.5445019199415,33.2091977213449,-48.7416166666667));
#253890=CARTESIAN_POINT('Ctrl Pts',(43.0627766507519,32.3748250798187,-48.6832833333333));
#253891=CARTESIAN_POINT('Ctrl Pts',(42.5810513815623,31.5404524382925,-48.62495));
#253892=CARTESIAN_POINT('Ctrl Pts',(43.0627766507519,30.7060797967663,-48.5666166666667));
#253893=CARTESIAN_POINT('Ctrl Pts',(43.5445019199415,29.87170715524,-48.5082833333333));
#253894=CARTESIAN_POINT('Ctrl Pts',(44.5079524583208,29.87170715524,-48.44995));
#253895=CARTESIAN_POINT('Ctrl Pts',(45.4714029967,29.87170715524,-48.3916166666667));
#253896=CARTESIAN_POINT('Ctrl Pts',(45.9531282658897,30.7060797967663,-48.3332833333333));
#253897=CARTESIAN_POINT('Ctrl Pts',(46.4348535350793,31.5404524382925,-48.27495));
#253898=CARTESIAN_POINT('Ctrl Pts',(45.9531282658897,32.3748250798187,-48.2166166666667));
#253899=CARTESIAN_POINT('Ctrl Pts',(45.4714029967,33.2091977213449,-48.1582833333333));
#253900=CARTESIAN_POINT('Ctrl Pts',(44.5079524583208,33.2091977213449,-48.09995));
#253901=CARTESIAN_POINT('Ctrl Pts',(43.5445019199415,33.2091977213449,-48.0416166666667));
#253902=CARTESIAN_POINT('Ctrl Pts',(43.0627766507519,32.3748250798187,-47.9832833333334));
#253903=CARTESIAN_POINT('Ctrl Pts',(42.5810513815623,31.5404524382925,-47.92495));
#253904=CARTESIAN_POINT('Ctrl Pts',(43.0627766507519,30.7060797967663,-47.8666166666667));
#253905=CARTESIAN_POINT('Ctrl Pts',(43.5445019199415,29.87170715524,-47.8082833333333));
#253906=CARTESIAN_POINT('Ctrl Pts',(44.5079524583208,29.87170715524,-47.74995));
#253907=CARTESIAN_POINT('Ctrl Pts',(45.4714029967,29.87170715524,-47.6916166666667));
#253908=CARTESIAN_POINT('Ctrl Pts',(45.9531282658897,30.7060797967663,-47.6332833333333));
#253909=CARTESIAN_POINT('Ctrl Pts',(46.4348535350793,31.5404524382925,-47.57495));
#253910=CARTESIAN_POINT('Ctrl Pts',(45.9531282658897,32.3748250798187,-47.5166166666667));
#253911=CARTESIAN_POINT('Ctrl Pts',(45.4714029967,33.2091977213449,-47.4582833333333));
#253912=CARTESIAN_POINT('Ctrl Pts',(44.5079524583208,33.2091977213449,-47.39995));
#253913=CARTESIAN_POINT('Ctrl Pts',(43.5445019199415,33.2091977213449,-47.3416166666666));
#253914=CARTESIAN_POINT('Ctrl Pts',(43.0627766507519,32.3748250798187,-47.2832833333333));
#253915=CARTESIAN_POINT('Ctrl Pts',(42.5810513815623,31.5404524382925,-47.22495));
#253916=CARTESIAN_POINT('Ctrl Pts',(43.0627766507519,30.7060797967663,-47.1666166666667));
#253917=CARTESIAN_POINT('Ctrl Pts',(43.5445019199415,29.87170715524,-47.1082833333333));
#253918=CARTESIAN_POINT('Ctrl Pts',(44.5079524583208,29.87170715524,-47.04995));
#253919=CARTESIAN_POINT('Ctrl Pts',(45.4714029967,29.87170715524,-46.9916166666667));
#253920=CARTESIAN_POINT('Ctrl Pts',(45.9531282658897,30.7060797967663,-46.9332833333333));
#253921=CARTESIAN_POINT('Ctrl Pts',(46.4348535350793,31.5404524382925,-46.87495));
#253922=CARTESIAN_POINT('Ctrl Pts',(45.9531282658897,32.3748250798187,-46.8166166666667));
#253923=CARTESIAN_POINT('Ctrl Pts',(45.4714029967,33.2091977213449,-46.7582833333333));
#253924=CARTESIAN_POINT('Ctrl Pts',(44.5079524583208,33.2091977213449,-46.69995));
#253925=CARTESIAN_POINT('Ctrl Pts',(43.5445019199415,33.2091977213449,-46.6416166666666));
#253926=CARTESIAN_POINT('Ctrl Pts',(43.0627766507519,32.3748250798187,-46.5832833333334));
#253927=CARTESIAN_POINT('Ctrl Pts',(42.5810513815623,31.5404524382925,-46.52495));
#253928=CARTESIAN_POINT('Ctrl Pts',(43.0627766507519,30.7060797967663,-46.4666166666667));
#253929=CARTESIAN_POINT('Ctrl Pts',(43.5445019199415,29.87170715524,-46.4082833333333));
#253930=CARTESIAN_POINT('Ctrl Pts',(44.5079524583208,29.87170715524,-46.34995));
#253931=CARTESIAN_POINT('Ctrl Pts',(45.4714029967,29.87170715524,-46.2916166666667));
#253932=CARTESIAN_POINT('Ctrl Pts',(45.9531282658897,30.7060797967663,-46.2332833333334));
#253933=CARTESIAN_POINT('Ctrl Pts',(46.4348535350793,31.5404524382925,-46.17495));
#253934=CARTESIAN_POINT('Ctrl Pts',(45.9531282658897,32.3748250798187,-46.1166166666667));
#253935=CARTESIAN_POINT('Ctrl Pts',(45.4714029967,33.2091977213449,-46.0582833333333));
#253936=CARTESIAN_POINT('Ctrl Pts',(44.5079524583208,33.2091977213449,-45.99995));
#253937=CARTESIAN_POINT('Ctrl Pts',(43.5445019199415,33.2091977213449,-45.9416166666667));
#253938=CARTESIAN_POINT('Ctrl Pts',(43.0627766507519,32.3748250798187,-45.8832833333333));
#253939=CARTESIAN_POINT('Ctrl Pts',(42.5810513815623,31.5404524382925,-45.82495));
#253940=CARTESIAN_POINT('Ctrl Pts',(43.0627766507519,30.7060797967663,-45.7666166666667));
#253941=CARTESIAN_POINT('Ctrl Pts',(43.5445019199415,29.87170715524,-45.7082833333333));
#253942=CARTESIAN_POINT('Ctrl Pts',(44.5079524583208,29.87170715524,-45.64995));
#253943=CARTESIAN_POINT('Ctrl Pts',(45.4714029967,29.87170715524,-45.5916166666667));
#253944=CARTESIAN_POINT('Ctrl Pts',(45.9531282658897,30.7060797967663,-45.5332833333333));
#253945=CARTESIAN_POINT('Ctrl Pts',(46.4348535350793,31.5404524382925,-45.47495));
#253946=CARTESIAN_POINT('Ctrl Pts',(45.9531282658897,32.3748250798187,-45.4166166666667));
#253947=CARTESIAN_POINT('Ctrl Pts',(45.4714029967,33.2091977213449,-45.3582833333333));
#253948=CARTESIAN_POINT('Ctrl Pts',(44.5079524583208,33.2091977213449,-45.29995));
#253949=CARTESIAN_POINT('Ctrl Pts',(43.5445019199415,33.2091977213449,-45.2416166666667));
#253950=CARTESIAN_POINT('Ctrl Pts',(43.0627766507519,32.3748250798187,-45.1832833333333));
#253951=CARTESIAN_POINT('Ctrl Pts',(42.5810513815623,31.5404524382925,-45.12495));
#253952=CARTESIAN_POINT('Ctrl Pts',(43.0627766507519,30.7060797967663,-45.0666166666667));
#253953=CARTESIAN_POINT('Ctrl Pts',(43.5445019199415,29.87170715524,-45.0082833333334));
#253954=CARTESIAN_POINT('Ctrl Pts',(44.5079524583208,29.87170715524,-44.94995));
#253955=CARTESIAN_POINT('Ctrl Pts',(45.4714029967,29.87170715524,-44.8916166666667));
#253956=CARTESIAN_POINT('Ctrl Pts',(45.9531282658897,30.7060797967663,-44.8332833333334));
#253957=CARTESIAN_POINT('Ctrl Pts',(46.4348535350793,31.5404524382925,-44.77495));
#253958=CARTESIAN_POINT('Ctrl Pts',(45.9531282658897,32.3748250798187,-44.7166166666667));
#253959=CARTESIAN_POINT('Ctrl Pts',(45.4714029967,33.2091977213449,-44.6582833333333));
#253960=CARTESIAN_POINT('Ctrl Pts',(44.5079524583208,33.2091977213449,-44.59995));
#253961=CARTESIAN_POINT('Ctrl Pts',(43.5445019199415,33.2091977213449,-44.5416166666667));
#253962=CARTESIAN_POINT('Ctrl Pts',(43.0627766507519,32.3748250798187,-44.4832833333334));
#253963=CARTESIAN_POINT('Ctrl Pts',(42.5810513815623,31.5404524382925,-44.42495));
#253964=CARTESIAN_POINT('Ctrl Pts',(43.0627766507519,30.7060797967663,-44.3666166666667));
#253965=CARTESIAN_POINT('Ctrl Pts',(43.5445019199415,29.87170715524,-44.3082833333334));
#253966=CARTESIAN_POINT('Ctrl Pts',(44.5079524583208,29.87170715524,-44.24995));
#253967=CARTESIAN_POINT('Ctrl Pts',(45.4714029967,29.87170715524,-44.1916166666667));
#253968=CARTESIAN_POINT('Ctrl Pts',(45.9531282658897,30.7060797967663,-44.1332833333334));
#253969=CARTESIAN_POINT('Ctrl Pts',(46.4348535350793,31.5404524382925,-44.07495));
#253970=CARTESIAN_POINT('Ctrl Pts',(45.9531282658897,32.3748250798187,-44.0166166666667));
#253971=CARTESIAN_POINT('Ctrl Pts',(45.4714029967,33.2091977213449,-43.9582833333334));
#253972=CARTESIAN_POINT('Ctrl Pts',(44.5079524583208,33.2091977213449,-43.89995));
#253973=CARTESIAN_POINT('Ctrl Pts',(43.5445019199415,33.2091977213449,-43.8416166666667));
#253974=CARTESIAN_POINT('Ctrl Pts',(43.0627766507519,32.3748250798187,-43.7832833333334));
#253975=CARTESIAN_POINT('Ctrl Pts',(42.5810513815623,31.5404524382925,-43.72495));
#253976=CARTESIAN_POINT('Ctrl Pts',(43.0627766507519,30.7060797967663,-43.6666166666667));
#253977=CARTESIAN_POINT('Ctrl Pts',(43.5445019199415,29.87170715524,-43.6082833333333));
#253978=CARTESIAN_POINT('Ctrl Pts',(44.5079524583208,29.87170715524,-43.54995));
#253979=CARTESIAN_POINT('Ctrl Pts',(45.4714029967,29.87170715524,-43.4916166666667));
#253980=CARTESIAN_POINT('Ctrl Pts',(45.9531282658897,30.7060797967663,-43.4332833333333));
#253981=CARTESIAN_POINT('Ctrl Pts',(46.4348535350793,31.5404524382925,-43.37495));
#253982=CARTESIAN_POINT('Ctrl Pts',(45.9531282658897,32.3748250798187,-43.3166166666667));
#253983=CARTESIAN_POINT('Ctrl Pts',(45.4714029967,33.2091977213449,-43.2582833333333));
#253984=CARTESIAN_POINT('Ctrl Pts',(44.5079524583208,33.2091977213449,-43.19995));
#253985=CARTESIAN_POINT('Ctrl Pts',(43.5445019199415,33.2091977213449,-43.1416166666666));
#253986=CARTESIAN_POINT('Ctrl Pts',(43.0627766507519,32.3748250798187,-43.0832833333333));
#253987=CARTESIAN_POINT('Ctrl Pts',(42.5810513815623,31.5404524382925,-43.02495));
#253988=CARTESIAN_POINT('Ctrl Pts',(43.0627766507519,30.7060797967663,-42.9666166666667));
#253989=CARTESIAN_POINT('Ctrl Pts',(43.5445019199415,29.87170715524,-42.9082833333333));
#253990=CARTESIAN_POINT('Ctrl Pts',(44.5079524583208,29.87170715524,-42.84995));
#253991=CARTESIAN_POINT('Ctrl Pts',(45.4714029967,29.87170715524,-42.7916166666667));
#253992=CARTESIAN_POINT('Ctrl Pts',(45.9531282658897,30.7060797967663,-42.7332833333334));
#253993=CARTESIAN_POINT('Ctrl Pts',(46.4348535350793,31.5404524382925,-42.67495));
#253994=CARTESIAN_POINT('Ctrl Pts',(45.9531282658897,32.3748250798187,-42.6166166666667));
#253995=CARTESIAN_POINT('Ctrl Pts',(45.4714029967,33.2091977213449,-42.5582833333333));
#253996=CARTESIAN_POINT('Ctrl Pts',(44.5079524583208,33.2091977213449,-42.49995));
#253997=CARTESIAN_POINT('Ctrl Pts',(43.5445019199415,33.2091977213449,-42.4416166666667));
#253998=CARTESIAN_POINT('Ctrl Pts',(43.0627766507519,32.3748250798187,-42.3832833333333));
#253999=CARTESIAN_POINT('Ctrl Pts',(42.5810513815623,31.5404524382925,-42.32495));
#254000=CARTESIAN_POINT('Ctrl Pts',(43.0627766507519,30.7060797967663,-42.2666166666667));
#254001=CARTESIAN_POINT('Ctrl Pts',(43.5445019199415,29.87170715524,-42.2082833333333));
#254002=CARTESIAN_POINT('Ctrl Pts',(44.5079524583208,29.87170715524,-42.14995));
#254003=CARTESIAN_POINT('Ctrl Pts',(45.4714029967,29.87170715524,-42.0916166666667));
#254004=CARTESIAN_POINT('Ctrl Pts',(45.9531282658897,30.7060797967663,-42.0332833333334));
#254005=CARTESIAN_POINT('Ctrl Pts',(46.4348535350793,31.5404524382925,-41.97495));
#254006=CARTESIAN_POINT('Ctrl Pts',(45.9531282658897,32.3748250798187,-41.9166166666666));
#254007=CARTESIAN_POINT('Ctrl Pts',(45.4714029967,33.2091977213449,-41.8582833333333));
#254008=CARTESIAN_POINT('Ctrl Pts',(44.5079524583208,33.2091977213449,-41.79995));
#254009=CARTESIAN_POINT('Ctrl Pts',(43.5445019199415,33.2091977213449,-41.7416166666667));
#254010=CARTESIAN_POINT('Ctrl Pts',(43.0627766507519,32.3748250798187,-41.6832833333333));
#254011=CARTESIAN_POINT('Ctrl Pts',(42.5810513815623,31.5404524382925,-41.62495));
#254012=CARTESIAN_POINT('Ctrl Pts',(43.0627766507519,30.7060797967663,-41.5666166666667));
#254013=CARTESIAN_POINT('Ctrl Pts',(43.5445019199415,29.87170715524,-41.5082833333334));
#254014=CARTESIAN_POINT('Ctrl Pts',(44.5079524583208,29.87170715524,-41.44995));
#254015=CARTESIAN_POINT('Ctrl Pts',(45.4714029967,29.87170715524,-41.3916166666667));
#254016=CARTESIAN_POINT('Ctrl Pts',(45.9531282658897,30.7060797967663,-41.3332833333334));
#254017=CARTESIAN_POINT('Ctrl Pts',(46.4348535350793,31.5404524382925,-41.27495));
#254018=CARTESIAN_POINT('Ctrl Pts',(45.9531282658897,32.3748250798187,-41.2166166666667));
#254019=CARTESIAN_POINT('Ctrl Pts',(45.4714029967,33.2091977213449,-41.1582833333333));
#254020=CARTESIAN_POINT('Ctrl Pts',(44.5079524583208,33.2091977213449,-41.09995));
#254021=CARTESIAN_POINT('Ctrl Pts',(43.5445019199415,33.2091977213449,-41.0416166666667));
#254022=CARTESIAN_POINT('Ctrl Pts',(43.0627766507519,32.3748250798187,-40.9832833333333));
#254023=CARTESIAN_POINT('Ctrl Pts',(42.5810513815623,31.5404524382925,-40.92495));
#254024=CARTESIAN_POINT('Ctrl Pts',(43.0627766507519,30.7060797967663,-40.8666166666667));
#254025=CARTESIAN_POINT('Ctrl Pts',(43.5445019199415,29.87170715524,-40.8082833333334));
#254026=CARTESIAN_POINT('Ctrl Pts',(44.5079524583208,29.87170715524,-40.74995));
#254027=CARTESIAN_POINT('Ctrl Pts',(45.4714029967,29.87170715524,-40.6916166666667));
#254028=CARTESIAN_POINT('Ctrl Pts',(45.9531282658897,30.7060797967663,-40.6332833333334));
#254029=CARTESIAN_POINT('Ctrl Pts',(46.4348535350793,31.5404524382925,-40.57495));
#254030=CARTESIAN_POINT('Ctrl Pts',(45.9531282658897,32.3748250798187,-40.5166166666666));
#254031=CARTESIAN_POINT('Ctrl Pts',(45.4714029967,33.2091977213449,-40.4582833333333));
#254032=CARTESIAN_POINT('Ctrl Pts',(44.5079524583208,33.2091977213449,-40.39995));
#254033=CARTESIAN_POINT('Ctrl Pts',(43.5445019199415,33.2091977213449,-40.3416166666667));
#254034=CARTESIAN_POINT('Ctrl Pts',(43.0627766507519,32.3748250798187,-40.2832833333334));
#254035=CARTESIAN_POINT('Ctrl Pts',(42.5810513815623,31.5404524382925,-40.22495));
#254036=CARTESIAN_POINT('Ctrl Pts',(43.0627766507519,30.7060797967663,-40.1666166666667));
#254037=CARTESIAN_POINT('Ctrl Pts',(43.5445019199415,29.87170715524,-40.1082833333334));
#254038=CARTESIAN_POINT('Ctrl Pts',(44.5079524583208,29.87170715524,-40.04995));
#254039=CARTESIAN_POINT('Ctrl Pts',(45.4714029967,29.87170715524,-39.9916166666667));
#254040=CARTESIAN_POINT('Ctrl Pts',(45.9531282658897,30.7060797967663,-39.9332833333333));
#254041=CARTESIAN_POINT('Ctrl Pts',(46.4348535350793,31.5404524382925,-39.87495));
#254042=CARTESIAN_POINT('Ctrl Pts',(45.9531282658897,32.3748250798187,-39.8166166666667));
#254043=CARTESIAN_POINT('Ctrl Pts',(45.4714029967,33.2091977213449,-39.7582833333334));
#254044=CARTESIAN_POINT('Ctrl Pts',(44.5079524583208,33.2091977213449,-39.69995));
#254045=CARTESIAN_POINT('Ctrl Pts',(43.5445019199415,33.2091977213449,-39.6416166666667));
#254046=CARTESIAN_POINT('Ctrl Pts',(43.0627766507519,32.3748250798187,-39.5832833333333));
#254047=CARTESIAN_POINT('Ctrl Pts',(42.5810513815623,31.5404524382925,-39.52495));
#254048=CARTESIAN_POINT('Ctrl Pts',(43.0627766507519,30.7060797967663,-39.4666166666667));
#254049=CARTESIAN_POINT('Ctrl Pts',(43.5445019199415,29.87170715524,-39.4082833333333));
#254050=CARTESIAN_POINT('Ctrl Pts',(44.5079524583208,29.87170715524,-39.34995));
#254051=CARTESIAN_POINT('Ctrl Pts',(45.4714029967,29.87170715524,-39.2916166666667));
#254052=CARTESIAN_POINT('Ctrl Pts',(45.9531282658897,30.7060797967663,-39.2332833333333));
#254053=CARTESIAN_POINT('Ctrl Pts',(46.4348535350793,31.5404524382925,-39.17495));
#254054=CARTESIAN_POINT('Ctrl Pts',(45.9531282658897,32.3748250798187,-39.1166166666667));
#254055=CARTESIAN_POINT('Ctrl Pts',(45.4714029967,33.2091977213449,-39.0582833333333));
#254056=CARTESIAN_POINT('Ctrl Pts',(44.5079524583208,33.2091977213449,-38.99995));
#254057=CARTESIAN_POINT('Ctrl Pts',(43.5445019199415,33.2091977213449,-38.9416166666667));
#254058=CARTESIAN_POINT('Ctrl Pts',(43.0627766507519,32.3748250798187,-38.8832833333334));
#254059=CARTESIAN_POINT('Ctrl Pts',(42.5810513815623,31.5404524382925,-38.82495));
#254060=CARTESIAN_POINT('Ctrl Pts',(43.0627766507519,30.7060797967663,-38.7666166666667));
#254061=CARTESIAN_POINT('Ctrl Pts',(43.5445019199415,29.87170715524,-38.7082833333333));
#254062=CARTESIAN_POINT('Ctrl Pts',(44.5079524583208,29.87170715524,-38.64995));
#254063=CARTESIAN_POINT('Ctrl Pts',(45.4714029967,29.87170715524,-38.5916166666667));
#254064=CARTESIAN_POINT('Ctrl Pts',(45.9531282658897,30.7060797967663,-38.5332833333334));
#254065=CARTESIAN_POINT('Ctrl Pts',(46.4348535350793,31.5404524382925,-38.47495));
#254066=CARTESIAN_POINT('Ctrl Pts',(45.9531282658897,32.3748250798187,-38.4166166666667));
#254067=CARTESIAN_POINT('Ctrl Pts',(45.4714029967,33.2091977213449,-38.3582833333333));
#254068=CARTESIAN_POINT('Ctrl Pts',(44.5079524583208,33.2091977213449,-38.29995));
#254069=CARTESIAN_POINT('Ctrl Pts',(43.5445019199415,33.2091977213449,-38.2416166666667));
#254070=CARTESIAN_POINT('Ctrl Pts',(43.0627766507519,32.3748250798187,-38.1832833333333));
#254071=CARTESIAN_POINT('Ctrl Pts',(42.5810513815623,31.5404524382925,-38.12495));
#254072=CARTESIAN_POINT('Ctrl Pts',(43.0627766507519,30.7060797967663,-38.0666166666667));
#254073=CARTESIAN_POINT('Ctrl Pts',(43.5445019199415,29.87170715524,-38.0082833333333));
#254074=CARTESIAN_POINT('Ctrl Pts',(44.5079524583208,29.87170715524,-37.94995));
#254075=CARTESIAN_POINT('Ctrl Pts',(45.4714029967,29.87170715524,-37.8916166666667));
#254076=CARTESIAN_POINT('Ctrl Pts',(45.9531282658897,30.7060797967663,-37.8332833333334));
#254077=CARTESIAN_POINT('Ctrl Pts',(46.4348535350793,31.5404524382925,-37.77495));
#254078=CARTESIAN_POINT('Ctrl Pts',(45.9531282658897,32.3748250798187,-37.7166166666667));
#254079=CARTESIAN_POINT('Ctrl Pts',(45.4714029967,33.2091977213449,-37.6582833333333));
#254080=CARTESIAN_POINT('Ctrl Pts',(44.5079524583208,33.2091977213449,-37.59995));
#254081=CARTESIAN_POINT('Ctrl Pts',(43.5445019199415,33.2091977213449,-37.5416166666667));
#254082=CARTESIAN_POINT('Ctrl Pts',(43.0627766507519,32.3748250798187,-37.4832833333334));
#254083=CARTESIAN_POINT('Ctrl Pts',(42.5810513815623,31.5404524382925,-37.42495));
#254084=CARTESIAN_POINT('Ctrl Pts',(43.0627766507519,30.7060797967663,-37.3666166666667));
#254085=CARTESIAN_POINT('Ctrl Pts',(43.5445019199415,29.87170715524,-37.3082833333333));
#254086=CARTESIAN_POINT('Ctrl Pts',(44.5079524583208,29.87170715524,-37.24995));
#254087=CARTESIAN_POINT('Ctrl Pts',(45.4714029967,29.87170715524,-37.1916166666667));
#254088=CARTESIAN_POINT('Ctrl Pts',(45.9531282658897,30.7060797967663,-37.1332833333334));
#254089=CARTESIAN_POINT('Ctrl Pts',(46.4348535350793,31.5404524382925,-37.07495));
#254090=CARTESIAN_POINT('Ctrl Pts',(45.9531282658897,32.3748250798187,-37.0166166666667));
#254091=CARTESIAN_POINT('Ctrl Pts',(45.8905850977848,32.4831530246427,-37.0090431559831));
#254092=CARTESIAN_POINT('Ctrl Pts',(45.8125914103809,32.5809465634453,-37.0009024189827));
#254093=CARTESIAN_POINT('Ctrl Pts',(44.5079524583208,33.6091932047179,-53.2308875));
#254094=CARTESIAN_POINT('Ctrl Pts',(43.3135644199415,33.6091932047179,-53.1725541666667));
#254095=CARTESIAN_POINT('Ctrl Pts',(42.7163704007519,32.5748228215052,-53.1142208333334));
#254096=CARTESIAN_POINT('Ctrl Pts',(42.1191763815623,31.5404524382925,-53.0558875000001));
#254097=CARTESIAN_POINT('Ctrl Pts',(42.7163704007519,30.5060820550798,-52.9975541666667));
#254098=CARTESIAN_POINT('Ctrl Pts',(43.3135644199415,29.4717116718671,-52.9392208333334));
#254099=CARTESIAN_POINT('Ctrl Pts',(44.5079524583208,29.4717116718671,-52.8808875));
#254100=CARTESIAN_POINT('Ctrl Pts',(45.7023404967,29.4717116718671,-52.8225541666667));
#254101=CARTESIAN_POINT('Ctrl Pts',(46.2995345158897,30.5060820550798,-52.7642208333334));
#254102=CARTESIAN_POINT('Ctrl Pts',(46.8967285350793,31.5404524382925,-52.7058875));
#254103=CARTESIAN_POINT('Ctrl Pts',(46.2995345158897,32.5748228215052,-52.6475541666667));
#254104=CARTESIAN_POINT('Ctrl Pts',(45.7023404967,33.6091932047179,-52.5892208333333));
#254105=CARTESIAN_POINT('Ctrl Pts',(44.5079524583208,33.6091932047179,-52.5308875));
#254106=CARTESIAN_POINT('Ctrl Pts',(43.3135644199415,33.6091932047179,-52.4725541666667));
#254107=CARTESIAN_POINT('Ctrl Pts',(42.7163704007519,32.5748228215052,-52.4142208333333));
#254108=CARTESIAN_POINT('Ctrl Pts',(42.1191763815623,31.5404524382925,-52.3558875000001));
#254109=CARTESIAN_POINT('Ctrl Pts',(42.7163704007519,30.5060820550798,-52.2975541666667));
#254110=CARTESIAN_POINT('Ctrl Pts',(43.3135644199415,29.4717116718671,-52.2392208333334));
#254111=CARTESIAN_POINT('Ctrl Pts',(44.5079524583208,29.4717116718671,-52.1808875));
#254112=CARTESIAN_POINT('Ctrl Pts',(45.7023404967,29.4717116718671,-52.1225541666667));
#254113=CARTESIAN_POINT('Ctrl Pts',(46.2995345158897,30.5060820550798,-52.0642208333334));
#254114=CARTESIAN_POINT('Ctrl Pts',(46.8967285350793,31.5404524382925,-52.0058875));
#254115=CARTESIAN_POINT('Ctrl Pts',(46.2995345158897,32.5748228215052,-51.9475541666667));
#254116=CARTESIAN_POINT('Ctrl Pts',(45.7023404967,33.6091932047179,-51.8892208333334));
#254117=CARTESIAN_POINT('Ctrl Pts',(44.5079524583208,33.6091932047179,-51.8308875));
#254118=CARTESIAN_POINT('Ctrl Pts',(43.3135644199415,33.6091932047179,-51.7725541666667));
#254119=CARTESIAN_POINT('Ctrl Pts',(42.7163704007519,32.5748228215052,-51.7142208333334));
#254120=CARTESIAN_POINT('Ctrl Pts',(42.1191763815623,31.5404524382925,-51.6558875));
#254121=CARTESIAN_POINT('Ctrl Pts',(42.7163704007519,30.5060820550798,-51.5975541666667));
#254122=CARTESIAN_POINT('Ctrl Pts',(43.3135644199415,29.4717116718671,-51.5392208333333));
#254123=CARTESIAN_POINT('Ctrl Pts',(44.5079524583208,29.4717116718671,-51.4808875));
#254124=CARTESIAN_POINT('Ctrl Pts',(45.7023404967,29.4717116718671,-51.4225541666667));
#254125=CARTESIAN_POINT('Ctrl Pts',(46.2995345158897,30.5060820550798,-51.3642208333334));
#254126=CARTESIAN_POINT('Ctrl Pts',(46.8967285350793,31.5404524382925,-51.3058875));
#254127=CARTESIAN_POINT('Ctrl Pts',(46.2995345158897,32.5748228215052,-51.2475541666667));
#254128=CARTESIAN_POINT('Ctrl Pts',(45.7023404967,33.6091932047179,-51.1892208333333));
#254129=CARTESIAN_POINT('Ctrl Pts',(44.5079524583208,33.6091932047179,-51.1308875));
#254130=CARTESIAN_POINT('Ctrl Pts',(43.3135644199415,33.6091932047179,-51.0725541666667));
#254131=CARTESIAN_POINT('Ctrl Pts',(42.7163704007519,32.5748228215052,-51.0142208333334));
#254132=CARTESIAN_POINT('Ctrl Pts',(42.1191763815623,31.5404524382925,-50.9558875));
#254133=CARTESIAN_POINT('Ctrl Pts',(42.7163704007519,30.5060820550798,-50.8975541666667));
#254134=CARTESIAN_POINT('Ctrl Pts',(43.3135644199415,29.4717116718671,-50.8392208333333));
#254135=CARTESIAN_POINT('Ctrl Pts',(44.5079524583208,29.4717116718671,-50.7808875));
#254136=CARTESIAN_POINT('Ctrl Pts',(45.7023404967,29.4717116718671,-50.7225541666666));
#254137=CARTESIAN_POINT('Ctrl Pts',(46.2995345158897,30.5060820550798,-50.6642208333333));
#254138=CARTESIAN_POINT('Ctrl Pts',(46.8967285350793,31.5404524382925,-50.6058875));
#254139=CARTESIAN_POINT('Ctrl Pts',(46.2995345158897,32.5748228215052,-50.5475541666667));
#254140=CARTESIAN_POINT('Ctrl Pts',(45.7023404967,33.6091932047179,-50.4892208333333));
#254141=CARTESIAN_POINT('Ctrl Pts',(44.5079524583208,33.6091932047179,-50.4308875));
#254142=CARTESIAN_POINT('Ctrl Pts',(43.3135644199415,33.6091932047179,-50.3725541666667));
#254143=CARTESIAN_POINT('Ctrl Pts',(42.7163704007519,32.5748228215052,-50.3142208333334));
#254144=CARTESIAN_POINT('Ctrl Pts',(42.1191763815623,31.5404524382925,-50.2558875));
#254145=CARTESIAN_POINT('Ctrl Pts',(42.7163704007519,30.5060820550798,-50.1975541666667));
#254146=CARTESIAN_POINT('Ctrl Pts',(43.3135644199415,29.4717116718671,-50.1392208333333));
#254147=CARTESIAN_POINT('Ctrl Pts',(44.5079524583208,29.4717116718671,-50.0808875));
#254148=CARTESIAN_POINT('Ctrl Pts',(45.7023404967,29.4717116718671,-50.0225541666667));
#254149=CARTESIAN_POINT('Ctrl Pts',(46.2995345158897,30.5060820550798,-49.9642208333334));
#254150=CARTESIAN_POINT('Ctrl Pts',(46.8967285350793,31.5404524382925,-49.9058875));
#254151=CARTESIAN_POINT('Ctrl Pts',(46.2995345158897,32.5748228215052,-49.8475541666667));
#254152=CARTESIAN_POINT('Ctrl Pts',(45.7023404967,33.6091932047179,-49.7892208333333));
#254153=CARTESIAN_POINT('Ctrl Pts',(44.5079524583208,33.6091932047179,-49.7308875));
#254154=CARTESIAN_POINT('Ctrl Pts',(43.3135644199415,33.6091932047179,-49.6725541666667));
#254155=CARTESIAN_POINT('Ctrl Pts',(42.7163704007519,32.5748228215052,-49.6142208333334));
#254156=CARTESIAN_POINT('Ctrl Pts',(42.1191763815623,31.5404524382925,-49.5558875));
#254157=CARTESIAN_POINT('Ctrl Pts',(42.7163704007519,30.5060820550798,-49.4975541666667));
#254158=CARTESIAN_POINT('Ctrl Pts',(43.3135644199415,29.4717116718671,-49.4392208333333));
#254159=CARTESIAN_POINT('Ctrl Pts',(44.5079524583208,29.4717116718671,-49.3808875));
#254160=CARTESIAN_POINT('Ctrl Pts',(45.7023404967,29.4717116718671,-49.3225541666667));
#254161=CARTESIAN_POINT('Ctrl Pts',(46.2995345158897,30.5060820550798,-49.2642208333334));
#254162=CARTESIAN_POINT('Ctrl Pts',(46.8967285350793,31.5404524382925,-49.2058875));
#254163=CARTESIAN_POINT('Ctrl Pts',(46.2995345158897,32.5748228215052,-49.1475541666667));
#254164=CARTESIAN_POINT('Ctrl Pts',(45.7023404967,33.6091932047179,-49.0892208333333));
#254165=CARTESIAN_POINT('Ctrl Pts',(44.5079524583208,33.6091932047179,-49.0308875));
#254166=CARTESIAN_POINT('Ctrl Pts',(43.3135644199415,33.6091932047179,-48.9725541666667));
#254167=CARTESIAN_POINT('Ctrl Pts',(42.7163704007519,32.5748228215052,-48.9142208333333));
#254168=CARTESIAN_POINT('Ctrl Pts',(42.1191763815623,31.5404524382925,-48.8558875));
#254169=CARTESIAN_POINT('Ctrl Pts',(42.7163704007519,30.5060820550798,-48.7975541666667));
#254170=CARTESIAN_POINT('Ctrl Pts',(43.3135644199415,29.4717116718671,-48.7392208333334));
#254171=CARTESIAN_POINT('Ctrl Pts',(44.5079524583208,29.4717116718671,-48.6808875));
#254172=CARTESIAN_POINT('Ctrl Pts',(45.7023404967,29.4717116718671,-48.6225541666667));
#254173=CARTESIAN_POINT('Ctrl Pts',(46.2995345158897,30.5060820550798,-48.5642208333334));
#254174=CARTESIAN_POINT('Ctrl Pts',(46.8967285350793,31.5404524382925,-48.5058875));
#254175=CARTESIAN_POINT('Ctrl Pts',(46.2995345158897,32.5748228215052,-48.4475541666667));
#254176=CARTESIAN_POINT('Ctrl Pts',(45.7023404967,33.6091932047179,-48.3892208333334));
#254177=CARTESIAN_POINT('Ctrl Pts',(44.5079524583208,33.6091932047179,-48.3308875));
#254178=CARTESIAN_POINT('Ctrl Pts',(43.3135644199415,33.6091932047179,-48.2725541666667));
#254179=CARTESIAN_POINT('Ctrl Pts',(42.7163704007519,32.5748228215052,-48.2142208333334));
#254180=CARTESIAN_POINT('Ctrl Pts',(42.1191763815623,31.5404524382925,-48.1558875));
#254181=CARTESIAN_POINT('Ctrl Pts',(42.7163704007519,30.5060820550798,-48.0975541666667));
#254182=CARTESIAN_POINT('Ctrl Pts',(43.3135644199415,29.4717116718671,-48.0392208333334));
#254183=CARTESIAN_POINT('Ctrl Pts',(44.5079524583208,29.4717116718671,-47.9808875));
#254184=CARTESIAN_POINT('Ctrl Pts',(45.7023404967,29.4717116718671,-47.9225541666667));
#254185=CARTESIAN_POINT('Ctrl Pts',(46.2995345158897,30.5060820550798,-47.8642208333334));
#254186=CARTESIAN_POINT('Ctrl Pts',(46.8967285350793,31.5404524382925,-47.8058875000001));
#254187=CARTESIAN_POINT('Ctrl Pts',(46.2995345158897,32.5748228215052,-47.7475541666667));
#254188=CARTESIAN_POINT('Ctrl Pts',(45.7023404967,33.6091932047179,-47.6892208333334));
#254189=CARTESIAN_POINT('Ctrl Pts',(44.5079524583208,33.6091932047179,-47.6308875));
#254190=CARTESIAN_POINT('Ctrl Pts',(43.3135644199415,33.6091932047179,-47.5725541666667));
#254191=CARTESIAN_POINT('Ctrl Pts',(42.7163704007519,32.5748228215052,-47.5142208333333));
#254192=CARTESIAN_POINT('Ctrl Pts',(42.1191763815623,31.5404524382925,-47.4558875));
#254193=CARTESIAN_POINT('Ctrl Pts',(42.7163704007519,30.5060820550798,-47.3975541666667));
#254194=CARTESIAN_POINT('Ctrl Pts',(43.3135644199415,29.4717116718671,-47.3392208333333));
#254195=CARTESIAN_POINT('Ctrl Pts',(44.5079524583208,29.4717116718671,-47.2808875));
#254196=CARTESIAN_POINT('Ctrl Pts',(45.7023404967,29.4717116718671,-47.2225541666667));
#254197=CARTESIAN_POINT('Ctrl Pts',(46.2995345158897,30.5060820550798,-47.1642208333334));
#254198=CARTESIAN_POINT('Ctrl Pts',(46.8967285350793,31.5404524382925,-47.1058875));
#254199=CARTESIAN_POINT('Ctrl Pts',(46.2995345158897,32.5748228215052,-47.0475541666667));
#254200=CARTESIAN_POINT('Ctrl Pts',(45.7023404967,33.6091932047179,-46.9892208333334));
#254201=CARTESIAN_POINT('Ctrl Pts',(44.5079524583208,33.6091932047179,-46.9308875));
#254202=CARTESIAN_POINT('Ctrl Pts',(43.3135644199415,33.6091932047179,-46.8725541666667));
#254203=CARTESIAN_POINT('Ctrl Pts',(42.7163704007519,32.5748228215052,-46.8142208333334));
#254204=CARTESIAN_POINT('Ctrl Pts',(42.1191763815623,31.5404524382925,-46.7558875));
#254205=CARTESIAN_POINT('Ctrl Pts',(42.7163704007519,30.5060820550798,-46.6975541666667));
#254206=CARTESIAN_POINT('Ctrl Pts',(43.3135644199415,29.4717116718671,-46.6392208333333));
#254207=CARTESIAN_POINT('Ctrl Pts',(44.5079524583208,29.4717116718671,-46.5808875));
#254208=CARTESIAN_POINT('Ctrl Pts',(45.7023404967,29.4717116718671,-46.5225541666667));
#254209=CARTESIAN_POINT('Ctrl Pts',(46.2995345158897,30.5060820550798,-46.4642208333334));
#254210=CARTESIAN_POINT('Ctrl Pts',(46.8967285350793,31.5404524382925,-46.4058875));
#254211=CARTESIAN_POINT('Ctrl Pts',(46.2995345158897,32.5748228215052,-46.3475541666667));
#254212=CARTESIAN_POINT('Ctrl Pts',(45.7023404967,33.6091932047179,-46.2892208333334));
#254213=CARTESIAN_POINT('Ctrl Pts',(44.5079524583208,33.6091932047179,-46.2308875));
#254214=CARTESIAN_POINT('Ctrl Pts',(43.3135644199415,33.6091932047179,-46.1725541666667));
#254215=CARTESIAN_POINT('Ctrl Pts',(42.7163704007519,32.5748228215052,-46.1142208333334));
#254216=CARTESIAN_POINT('Ctrl Pts',(42.1191763815623,31.5404524382925,-46.0558875));
#254217=CARTESIAN_POINT('Ctrl Pts',(42.7163704007519,30.5060820550798,-45.9975541666667));
#254218=CARTESIAN_POINT('Ctrl Pts',(43.3135644199415,29.4717116718671,-45.9392208333333));
#254219=CARTESIAN_POINT('Ctrl Pts',(44.5079524583208,29.4717116718671,-45.8808875));
#254220=CARTESIAN_POINT('Ctrl Pts',(45.7023404967,29.4717116718671,-45.8225541666667));
#254221=CARTESIAN_POINT('Ctrl Pts',(46.2995345158897,30.5060820550798,-45.7642208333334));
#254222=CARTESIAN_POINT('Ctrl Pts',(46.8967285350793,31.5404524382925,-45.7058875));
#254223=CARTESIAN_POINT('Ctrl Pts',(46.2995345158897,32.5748228215052,-45.6475541666667));
#254224=CARTESIAN_POINT('Ctrl Pts',(45.7023404967,33.6091932047179,-45.5892208333333));
#254225=CARTESIAN_POINT('Ctrl Pts',(44.5079524583208,33.6091932047179,-45.5308875));
#254226=CARTESIAN_POINT('Ctrl Pts',(43.3135644199415,33.6091932047179,-45.4725541666667));
#254227=CARTESIAN_POINT('Ctrl Pts',(42.7163704007519,32.5748228215052,-45.4142208333334));
#254228=CARTESIAN_POINT('Ctrl Pts',(42.1191763815623,31.5404524382925,-45.3558875));
#254229=CARTESIAN_POINT('Ctrl Pts',(42.7163704007519,30.5060820550798,-45.2975541666667));
#254230=CARTESIAN_POINT('Ctrl Pts',(43.3135644199415,29.4717116718671,-45.2392208333333));
#254231=CARTESIAN_POINT('Ctrl Pts',(44.5079524583208,29.4717116718671,-45.1808875));
#254232=CARTESIAN_POINT('Ctrl Pts',(45.7023404967,29.4717116718671,-45.1225541666667));
#254233=CARTESIAN_POINT('Ctrl Pts',(46.2995345158897,30.5060820550798,-45.0642208333334));
#254234=CARTESIAN_POINT('Ctrl Pts',(46.8967285350793,31.5404524382925,-45.0058875));
#254235=CARTESIAN_POINT('Ctrl Pts',(46.2995345158897,32.5748228215052,-44.9475541666667));
#254236=CARTESIAN_POINT('Ctrl Pts',(45.7023404967,33.6091932047179,-44.8892208333333));
#254237=CARTESIAN_POINT('Ctrl Pts',(44.5079524583208,33.6091932047179,-44.8308875));
#254238=CARTESIAN_POINT('Ctrl Pts',(43.3135644199415,33.6091932047179,-44.7725541666666));
#254239=CARTESIAN_POINT('Ctrl Pts',(42.7163704007519,32.5748228215052,-44.7142208333334));
#254240=CARTESIAN_POINT('Ctrl Pts',(42.1191763815623,31.5404524382925,-44.6558875));
#254241=CARTESIAN_POINT('Ctrl Pts',(42.7163704007519,30.5060820550798,-44.5975541666667));
#254242=CARTESIAN_POINT('Ctrl Pts',(43.3135644199415,29.4717116718671,-44.5392208333333));
#254243=CARTESIAN_POINT('Ctrl Pts',(44.5079524583208,29.4717116718671,-44.4808875));
#254244=CARTESIAN_POINT('Ctrl Pts',(45.7023404967,29.4717116718671,-44.4225541666667));
#254245=CARTESIAN_POINT('Ctrl Pts',(46.2995345158897,30.5060820550798,-44.3642208333333));
#254246=CARTESIAN_POINT('Ctrl Pts',(46.8967285350793,31.5404524382925,-44.3058875));
#254247=CARTESIAN_POINT('Ctrl Pts',(46.2995345158897,32.5748228215052,-44.2475541666667));
#254248=CARTESIAN_POINT('Ctrl Pts',(45.7023404967,33.6091932047179,-44.1892208333334));
#254249=CARTESIAN_POINT('Ctrl Pts',(44.5079524583208,33.6091932047179,-44.1308875));
#254250=CARTESIAN_POINT('Ctrl Pts',(43.3135644199415,33.6091932047179,-44.0725541666667));
#254251=CARTESIAN_POINT('Ctrl Pts',(42.7163704007519,32.5748228215052,-44.0142208333334));
#254252=CARTESIAN_POINT('Ctrl Pts',(42.1191763815623,31.5404524382925,-43.9558875));
#254253=CARTESIAN_POINT('Ctrl Pts',(42.7163704007519,30.5060820550798,-43.8975541666667));
#254254=CARTESIAN_POINT('Ctrl Pts',(43.3135644199415,29.4717116718671,-43.8392208333333));
#254255=CARTESIAN_POINT('Ctrl Pts',(44.5079524583208,29.4717116718671,-43.7808875));
#254256=CARTESIAN_POINT('Ctrl Pts',(45.7023404967,29.4717116718671,-43.7225541666667));
#254257=CARTESIAN_POINT('Ctrl Pts',(46.2995345158897,30.5060820550798,-43.6642208333334));
#254258=CARTESIAN_POINT('Ctrl Pts',(46.8967285350793,31.5404524382925,-43.6058875));
#254259=CARTESIAN_POINT('Ctrl Pts',(46.2995345158897,32.5748228215052,-43.5475541666667));
#254260=CARTESIAN_POINT('Ctrl Pts',(45.7023404967,33.6091932047179,-43.4892208333333));
#254261=CARTESIAN_POINT('Ctrl Pts',(44.5079524583208,33.6091932047179,-43.4308875));
#254262=CARTESIAN_POINT('Ctrl Pts',(43.3135644199415,33.6091932047179,-43.3725541666667));
#254263=CARTESIAN_POINT('Ctrl Pts',(42.7163704007519,32.5748228215052,-43.3142208333334));
#254264=CARTESIAN_POINT('Ctrl Pts',(42.1191763815623,31.5404524382925,-43.2558875));
#254265=CARTESIAN_POINT('Ctrl Pts',(42.7163704007519,30.5060820550798,-43.1975541666667));
#254266=CARTESIAN_POINT('Ctrl Pts',(43.3135644199415,29.4717116718671,-43.1392208333334));
#254267=CARTESIAN_POINT('Ctrl Pts',(44.5079524583208,29.4717116718671,-43.0808875));
#254268=CARTESIAN_POINT('Ctrl Pts',(45.7023404967,29.4717116718671,-43.0225541666667));
#254269=CARTESIAN_POINT('Ctrl Pts',(46.2995345158897,30.5060820550798,-42.9642208333334));
#254270=CARTESIAN_POINT('Ctrl Pts',(46.8967285350793,31.5404524382925,-42.9058875));
#254271=CARTESIAN_POINT('Ctrl Pts',(46.2995345158897,32.5748228215052,-42.8475541666667));
#254272=CARTESIAN_POINT('Ctrl Pts',(45.7023404967,33.6091932047179,-42.7892208333334));
#254273=CARTESIAN_POINT('Ctrl Pts',(44.5079524583208,33.6091932047179,-42.7308875));
#254274=CARTESIAN_POINT('Ctrl Pts',(43.3135644199415,33.6091932047179,-42.6725541666667));
#254275=CARTESIAN_POINT('Ctrl Pts',(42.7163704007519,32.5748228215052,-42.6142208333334));
#254276=CARTESIAN_POINT('Ctrl Pts',(42.1191763815623,31.5404524382925,-42.5558875));
#254277=CARTESIAN_POINT('Ctrl Pts',(42.7163704007519,30.5060820550798,-42.4975541666667));
#254278=CARTESIAN_POINT('Ctrl Pts',(43.3135644199415,29.4717116718671,-42.4392208333334));
#254279=CARTESIAN_POINT('Ctrl Pts',(44.5079524583208,29.4717116718671,-42.3808875));
#254280=CARTESIAN_POINT('Ctrl Pts',(45.7023404967,29.4717116718671,-42.3225541666667));
#254281=CARTESIAN_POINT('Ctrl Pts',(46.2995345158897,30.5060820550798,-42.2642208333334));
#254282=CARTESIAN_POINT('Ctrl Pts',(46.8967285350793,31.5404524382925,-42.2058875));
#254283=CARTESIAN_POINT('Ctrl Pts',(46.2995345158897,32.5748228215052,-42.1475541666667));
#254284=CARTESIAN_POINT('Ctrl Pts',(45.7023404967,33.6091932047179,-42.0892208333333));
#254285=CARTESIAN_POINT('Ctrl Pts',(44.5079524583208,33.6091932047179,-42.0308875));
#254286=CARTESIAN_POINT('Ctrl Pts',(43.3135644199415,33.6091932047179,-41.9725541666667));
#254287=CARTESIAN_POINT('Ctrl Pts',(42.7163704007519,32.5748228215052,-41.9142208333334));
#254288=CARTESIAN_POINT('Ctrl Pts',(42.1191763815623,31.5404524382925,-41.8558875));
#254289=CARTESIAN_POINT('Ctrl Pts',(42.7163704007519,30.5060820550798,-41.7975541666667));
#254290=CARTESIAN_POINT('Ctrl Pts',(43.3135644199415,29.4717116718671,-41.7392208333333));
#254291=CARTESIAN_POINT('Ctrl Pts',(44.5079524583208,29.4717116718671,-41.6808875));
#254292=CARTESIAN_POINT('Ctrl Pts',(45.7023404967,29.4717116718671,-41.6225541666667));
#254293=CARTESIAN_POINT('Ctrl Pts',(46.2995345158897,30.5060820550798,-41.5642208333334));
#254294=CARTESIAN_POINT('Ctrl Pts',(46.8967285350793,31.5404524382925,-41.5058875));
#254295=CARTESIAN_POINT('Ctrl Pts',(46.2995345158897,32.5748228215052,-41.4475541666667));
#254296=CARTESIAN_POINT('Ctrl Pts',(45.7023404967,33.6091932047179,-41.3892208333333));
#254297=CARTESIAN_POINT('Ctrl Pts',(44.5079524583208,33.6091932047179,-41.3308875));
#254298=CARTESIAN_POINT('Ctrl Pts',(43.3135644199415,33.6091932047179,-41.2725541666667));
#254299=CARTESIAN_POINT('Ctrl Pts',(42.7163704007519,32.5748228215052,-41.2142208333333));
#254300=CARTESIAN_POINT('Ctrl Pts',(42.1191763815623,31.5404524382925,-41.1558875));
#254301=CARTESIAN_POINT('Ctrl Pts',(42.7163704007519,30.5060820550798,-41.0975541666667));
#254302=CARTESIAN_POINT('Ctrl Pts',(43.3135644199415,29.4717116718671,-41.0392208333333));
#254303=CARTESIAN_POINT('Ctrl Pts',(44.5079524583208,29.4717116718671,-40.9808875));
#254304=CARTESIAN_POINT('Ctrl Pts',(45.7023404967,29.4717116718671,-40.9225541666667));
#254305=CARTESIAN_POINT('Ctrl Pts',(46.2995345158897,30.5060820550798,-40.8642208333334));
#254306=CARTESIAN_POINT('Ctrl Pts',(46.8967285350793,31.5404524382925,-40.8058875));
#254307=CARTESIAN_POINT('Ctrl Pts',(46.2995345158897,32.5748228215052,-40.7475541666667));
#254308=CARTESIAN_POINT('Ctrl Pts',(45.7023404967,33.6091932047179,-40.6892208333333));
#254309=CARTESIAN_POINT('Ctrl Pts',(44.5079524583208,33.6091932047179,-40.6308875));
#254310=CARTESIAN_POINT('Ctrl Pts',(43.3135644199415,33.6091932047179,-40.5725541666667));
#254311=CARTESIAN_POINT('Ctrl Pts',(42.7163704007519,32.5748228215052,-40.5142208333333));
#254312=CARTESIAN_POINT('Ctrl Pts',(42.1191763815623,31.5404524382925,-40.4558875));
#254313=CARTESIAN_POINT('Ctrl Pts',(42.7163704007519,30.5060820550798,-40.3975541666667));
#254314=CARTESIAN_POINT('Ctrl Pts',(43.3135644199415,29.4717116718671,-40.3392208333333));
#254315=CARTESIAN_POINT('Ctrl Pts',(44.5079524583208,29.4717116718671,-40.2808875));
#254316=CARTESIAN_POINT('Ctrl Pts',(45.7023404967,29.4717116718671,-40.2225541666667));
#254317=CARTESIAN_POINT('Ctrl Pts',(46.2995345158897,30.5060820550798,-40.1642208333333));
#254318=CARTESIAN_POINT('Ctrl Pts',(46.8967285350793,31.5404524382925,-40.1058875));
#254319=CARTESIAN_POINT('Ctrl Pts',(46.2995345158897,32.5748228215052,-40.0475541666667));
#254320=CARTESIAN_POINT('Ctrl Pts',(45.7023404967,33.6091932047179,-39.9892208333333));
#254321=CARTESIAN_POINT('Ctrl Pts',(44.5079524583208,33.6091932047179,-39.9308875));
#254322=CARTESIAN_POINT('Ctrl Pts',(43.3135644199415,33.6091932047179,-39.8725541666667));
#254323=CARTESIAN_POINT('Ctrl Pts',(42.7163704007519,32.5748228215052,-39.8142208333334));
#254324=CARTESIAN_POINT('Ctrl Pts',(42.1191763815623,31.5404524382925,-39.7558875));
#254325=CARTESIAN_POINT('Ctrl Pts',(42.7163704007519,30.5060820550798,-39.6975541666667));
#254326=CARTESIAN_POINT('Ctrl Pts',(43.3135644199415,29.4717116718671,-39.6392208333334));
#254327=CARTESIAN_POINT('Ctrl Pts',(44.5079524583208,29.4717116718671,-39.5808875));
#254328=CARTESIAN_POINT('Ctrl Pts',(45.7023404967,29.4717116718671,-39.5225541666667));
#254329=CARTESIAN_POINT('Ctrl Pts',(46.2995345158897,30.5060820550798,-39.4642208333333));
#254330=CARTESIAN_POINT('Ctrl Pts',(46.8967285350793,31.5404524382925,-39.4058875));
#254331=CARTESIAN_POINT('Ctrl Pts',(46.2995345158897,32.5748228215052,-39.3475541666667));
#254332=CARTESIAN_POINT('Ctrl Pts',(45.7023404967,33.6091932047179,-39.2892208333334));
#254333=CARTESIAN_POINT('Ctrl Pts',(44.5079524583208,33.6091932047179,-39.2308875));
#254334=CARTESIAN_POINT('Ctrl Pts',(43.3135644199415,33.6091932047179,-39.1725541666667));
#254335=CARTESIAN_POINT('Ctrl Pts',(42.7163704007519,32.5748228215052,-39.1142208333333));
#254336=CARTESIAN_POINT('Ctrl Pts',(42.1191763815623,31.5404524382925,-39.0558875));
#254337=CARTESIAN_POINT('Ctrl Pts',(42.7163704007519,30.5060820550798,-38.9975541666667));
#254338=CARTESIAN_POINT('Ctrl Pts',(43.3135644199415,29.4717116718671,-38.9392208333334));
#254339=CARTESIAN_POINT('Ctrl Pts',(44.5079524583208,29.4717116718671,-38.8808875));
#254340=CARTESIAN_POINT('Ctrl Pts',(45.7023404967,29.4717116718671,-38.8225541666667));
#254341=CARTESIAN_POINT('Ctrl Pts',(46.2995345158897,30.5060820550798,-38.7642208333333));
#254342=CARTESIAN_POINT('Ctrl Pts',(46.8967285350793,31.5404524382925,-38.7058875));
#254343=CARTESIAN_POINT('Ctrl Pts',(46.2995345158897,32.5748228215052,-38.6475541666667));
#254344=CARTESIAN_POINT('Ctrl Pts',(45.7023404967,33.6091932047179,-38.5892208333334));
#254345=CARTESIAN_POINT('Ctrl Pts',(44.5079524583208,33.6091932047179,-38.5308875));
#254346=CARTESIAN_POINT('Ctrl Pts',(43.3135644199415,33.6091932047179,-38.4725541666667));
#254347=CARTESIAN_POINT('Ctrl Pts',(42.7163704007519,32.5748228215052,-38.4142208333334));
#254348=CARTESIAN_POINT('Ctrl Pts',(42.1191763815623,31.5404524382925,-38.3558875));
#254349=CARTESIAN_POINT('Ctrl Pts',(42.7163704007519,30.5060820550798,-38.2975541666667));
#254350=CARTESIAN_POINT('Ctrl Pts',(43.3135644199415,29.4717116718671,-38.2392208333333));
#254351=CARTESIAN_POINT('Ctrl Pts',(44.5079524583208,29.4717116718671,-38.1808875));
#254352=CARTESIAN_POINT('Ctrl Pts',(45.7023404967,29.4717116718671,-38.1225541666667));
#254353=CARTESIAN_POINT('Ctrl Pts',(46.2995345158897,30.5060820550798,-38.0642208333334));
#254354=CARTESIAN_POINT('Ctrl Pts',(46.8967285350793,31.5404524382925,-38.0058875));
#254355=CARTESIAN_POINT('Ctrl Pts',(46.2995345158897,32.5748228215052,-37.9475541666667));
#254356=CARTESIAN_POINT('Ctrl Pts',(45.7023404967,33.6091932047179,-37.8892208333334));
#254357=CARTESIAN_POINT('Ctrl Pts',(44.5079524583208,33.6091932047179,-37.8308875));
#254358=CARTESIAN_POINT('Ctrl Pts',(43.3135644199415,33.6091932047179,-37.7725541666667));
#254359=CARTESIAN_POINT('Ctrl Pts',(42.7163704007519,32.5748228215052,-37.7142208333333));
#254360=CARTESIAN_POINT('Ctrl Pts',(42.1191763815623,31.5404524382925,-37.6558875));
#254361=CARTESIAN_POINT('Ctrl Pts',(42.7163704007519,30.5060820550798,-37.5975541666667));
#254362=CARTESIAN_POINT('Ctrl Pts',(43.3135644199415,29.4717116718671,-37.5392208333334));
#254363=CARTESIAN_POINT('Ctrl Pts',(44.5079524583208,29.4717116718671,-37.4808875));
#254364=CARTESIAN_POINT('Ctrl Pts',(45.7023404967,29.4717116718671,-37.4225541666667));
#254365=CARTESIAN_POINT('Ctrl Pts',(46.2995345158897,30.5060820550798,-37.3642208333333));
#254366=CARTESIAN_POINT('Ctrl Pts',(46.8967285350793,31.5404524382925,-37.3058875));
#254367=CARTESIAN_POINT('Ctrl Pts',(46.2995345158897,32.5748228215052,-37.2475541666667));
#254368=CARTESIAN_POINT('Ctrl Pts',(46.2219998538691,32.7091167954726,-37.239980655983));
#254369=CARTESIAN_POINT('Ctrl Pts',(46.1253112086366,32.8303512837246,-37.2318399189827));
#254370=CARTESIAN_POINT('Ctrl Pts',(44.5079524583208,29.87170715524,-52.64995));
#254371=CARTESIAN_POINT('Ctrl Pts',(44.6656844499377,29.8551659258425,-52.64995));
#254372=CARTESIAN_POINT('Ctrl Pts',(44.8248930522266,29.859971256401,-52.64995));
#254373=CARTESIAN_POINT('Ctrl Pts',(45.1318235221548,29.9111573974697,-52.64995));
#254374=CARTESIAN_POINT('Ctrl Pts',(45.2783921862532,29.9557286678636,-52.64995));
#254375=CARTESIAN_POINT('Ctrl Pts',(45.6136601602179,30.1075367973101,-52.64995));
#254376=CARTESIAN_POINT('Ctrl Pts',(45.7919027673363,30.2317049318369,-52.64995));
#254377=CARTESIAN_POINT('Ctrl Pts',(46.142958313814,30.586793325784,-52.64995));
#254378=CARTESIAN_POINT('Ctrl Pts',(46.263796418765,30.8067269086716,-52.64995));
#254379=CARTESIAN_POINT('Ctrl Pts',(46.3921330992279,31.1120088134361,-52.64995));
#254380=CARTESIAN_POINT('Ctrl Pts',(46.4329712831975,31.2494771622503,-52.64995));
#254381=CARTESIAN_POINT('Ctrl Pts',(46.4841685595433,31.5316010230531,-52.64995));
#254382=CARTESIAN_POINT('Ctrl Pts',(46.4942078616458,31.6754009245257,-52.64995));
#254383=CARTESIAN_POINT('Ctrl Pts',(46.4884569292028,31.8190238668641,-52.64995));
#254384=CARTESIAN_POINT('Ctrl Pts',(46.0995611578475,30.7936217551105,-39.9761074628063));
#254385=CARTESIAN_POINT('Ctrl Pts',(46.0446831314069,30.7141759297788,-39.9726297030245));
#254386=CARTESIAN_POINT('Ctrl Pts',(45.9828153631749,30.6382127772846,-39.9689296509816));
#254387=CARTESIAN_POINT('Ctrl Pts',(45.8549789121757,30.5059161072079,-39.9628399295649));
#254388=CARTESIAN_POINT('Ctrl Pts',(45.7905370337022,30.4483633401059,-39.9602898047892));
#254389=CARTESIAN_POINT('Ctrl Pts',(45.7222548898542,30.3958213079794,-39.958107375254));
#254390=CARTESIAN_POINT('Ctrl Pts',(46.2910030640114,32.4463942341858,-40.0133533952396));
#254391=CARTESIAN_POINT('Ctrl Pts',(46.3764819107672,32.2781570359765,-40.0231672318018));
#254392=CARTESIAN_POINT('Ctrl Pts',(46.4377090636024,32.0986904899845,-40.0336361136513));
#254393=CARTESIAN_POINT('Ctrl Pts',(46.5090199982574,31.7229223169541,-40.0555559237447));
#254394=CARTESIAN_POINT('Ctrl Pts',(46.5172843967059,31.5282582026595,-40.0669113304119));
#254395=CARTESIAN_POINT('Ctrl Pts',(46.4702537911306,31.0718097984373,-40.0935374873249));
#254396=CARTESIAN_POINT('Ctrl Pts',(46.3909400941642,30.8161183615257,-40.1084528211447));
#254397=CARTESIAN_POINT('Ctrl Pts',(46.1427211482668,30.3607052140246,-40.1350185880823));
#254398=CARTESIAN_POINT('Ctrl Pts',(45.9801328439062,30.1631221897528,-40.1486669714983));
#254399=CARTESIAN_POINT('Ctrl Pts',(45.582272314324,29.8330739088149,-40.1783925570296));
#254400=CARTESIAN_POINT('Ctrl Pts',(45.3484458708397,29.7066366803743,-40.1938927885336));
#254401=CARTESIAN_POINT('Ctrl Pts',(44.9057198187658,29.5702291161657,-40.2202370429571));
#254402=CARTESIAN_POINT('Ctrl Pts',(44.707236793135,29.5404524382924,-40.2311325243694));
#254403=CARTESIAN_POINT('Ctrl Pts',(44.5079524583204,29.5404524382925,-40.2412));
#254404=CARTESIAN_POINT('Origin',(-44.5079524583208,31.5404524382925,235.35105));
#254405=CARTESIAN_POINT('',(-42.526443553871,31.2691191501876,-39.0141960261087));
#254406=CARTESIAN_POINT('',(-45.1065106637223,29.6321218916505,-39.2098644727505));
#254407=CARTESIAN_POINT('Ctrl Pts',(-42.5264433182785,31.2691190101349,
-39.0141952067154));
#254408=CARTESIAN_POINT('Ctrl Pts',(-42.5265992442052,31.2679804248256,
-39.013990016886));
#254409=CARTESIAN_POINT('Ctrl Pts',(-42.5267561298879,31.2668421931591,
-39.0137850971281));
#254410=CARTESIAN_POINT('Ctrl Pts',(-42.5269139699439,31.2657043581003,
-39.0135804553152));
#254411=CARTESIAN_POINT('Ctrl Pts',(-42.5314450660311,31.2330406596962,
-39.0077058266447));
#254412=CARTESIAN_POINT('Ctrl Pts',(-42.5367737540441,31.2005503855788,
-39.0020305783833));
#254413=CARTESIAN_POINT('Ctrl Pts',(-42.5428860897467,31.1682775236366,
-38.9965616542392));
#254414=CARTESIAN_POINT('Ctrl Pts',(-42.5489984254493,31.1360046616943,
-38.991092730095));
#254415=CARTESIAN_POINT('Ctrl Pts',(-42.555895594383,31.1039336351222,-38.9858271285204));
#254416=CARTESIAN_POINT('Ctrl Pts',(-42.5635729908238,31.0720631916436,
-38.9807642570009));
#254417=CARTESIAN_POINT('Ctrl Pts',(-42.5712503872647,31.040192748165,-38.9757013854813));
#254418=CARTESIAN_POINT('Ctrl Pts',(-42.5797080184842,31.0085228897363,
-38.9708412451465));
#254419=CARTESIAN_POINT('Ctrl Pts',(-42.5889469834378,30.9770538339552,
-38.9661846965336));
#254420=CARTESIAN_POINT('Ctrl Pts',(-42.5981859483915,30.9455847781742,
-38.9615281479207));
#254421=CARTESIAN_POINT('Ctrl Pts',(-42.60820623098,30.9143165209769,-38.957075186193));
#254422=CARTESIAN_POINT('Ctrl Pts',(-42.619014674011,30.8832507591964,-38.9528281414074));
#254423=CARTESIAN_POINT('Ctrl Pts',(-42.6298231170419,30.8521849974158,
-38.9485810966219));
#254424=CARTESIAN_POINT('Ctrl Pts',(-42.6414196796478,30.8213217206122,
-38.9445399575805));
#254425=CARTESIAN_POINT('Ctrl Pts',(-42.6538172012403,30.7906641692117,
-38.9407085950228));
#254426=CARTESIAN_POINT('Ctrl Pts',(-42.6662147228328,30.7600066178112,
-38.9368772324651));
#254427=CARTESIAN_POINT('Ctrl Pts',(-42.6794124410656,30.7295576092503,
-38.9332560772068));
#254428=CARTESIAN_POINT('Ctrl Pts',(-42.6934317597292,30.6993135470368,
-38.929849324519));
#254429=CARTESIAN_POINT('Ctrl Pts',(-42.700441419061,30.6841915159301,-38.9281459481751));
#254430=CARTESIAN_POINT('Ctrl Pts',(-42.7076664478387,30.6691033617142,
-38.9264946184812));
#254431=CARTESIAN_POINT('Ctrl Pts',(-42.7150618821773,30.6541435858172,
-38.924905794916));
#254432=CARTESIAN_POINT('Ctrl Pts',(-42.7224573165159,30.6391838099201,
-38.9233169713508));
#254433=CARTESIAN_POINT('Ctrl Pts',(-42.7300260074317,30.6243421619354,
-38.9217891027552));
#254434=CARTESIAN_POINT('Ctrl Pts',(-42.7377673957025,30.609622247504,-38.920322879707));
#254435=CARTESIAN_POINT('Ctrl Pts',(-42.768732948786,30.5507425897785,-38.9144579875142));
#254436=CARTESIAN_POINT('Ctrl Pts',(-42.802438005755,30.4937509787714,-38.9095620671014));
#254437=CARTESIAN_POINT('Ctrl Pts',(-42.8388300527629,30.4386219634623,
-38.9056215172398));
#254438=CARTESIAN_POINT('Ctrl Pts',(-42.8752220997707,30.3834929481532,
-38.9016809673782));
#254439=CARTESIAN_POINT('Ctrl Pts',(-42.9142995039568,30.330221730441,-38.898694431399));
#254440=CARTESIAN_POINT('Ctrl Pts',(-42.9560847992068,30.2788238207523,
-38.8966716165916));
#254441=CARTESIAN_POINT('Ctrl Pts',(-42.9978700944569,30.2274259110637,
-38.8946488017843));
#254442=CARTESIAN_POINT('Ctrl Pts',(-43.0423540539347,30.1779090615142,
-38.8935894002766));
#254443=CARTESIAN_POINT('Ctrl Pts',(-43.0896679045841,30.1303216200235,
-38.8935318156116));
#254444=CARTESIAN_POINT('Ctrl Pts',(-43.1369817552336,30.0827341785328,
-38.8934742309467));
#254445=CARTESIAN_POINT('Ctrl Pts',(-43.1862827102732,30.0379274090563,
-38.8944202483754));
#254446=CARTESIAN_POINT('Ctrl Pts',(-43.2374695236468,29.9958252623364,
-38.8963320083068));
#254447=CARTESIAN_POINT('Ctrl Pts',(-43.2886563370204,29.9537231156165,
-38.8982437682382));
#254448=CARTESIAN_POINT('Ctrl Pts',(-43.3417390736822,29.9143168693475,
-38.9011215513527));
#254449=CARTESIAN_POINT('Ctrl Pts',(-43.3967029881038,29.8775860531183,
-38.9049563008935));
#254450=CARTESIAN_POINT('Ctrl Pts',(-43.4241849453145,29.8592206450036,
-38.9068736756638));
#254451=CARTESIAN_POINT('Ctrl Pts',(-43.4521380201768,29.8415252139572,
-38.9090306863362));
#254452=CARTESIAN_POINT('Ctrl Pts',(-43.4805657277221,29.8245047392673,
-38.9114288083032));
#254453=CARTESIAN_POINT('Ctrl Pts',(-43.5089934352673,29.8074842645775,
-38.9138269302702));
#254454=CARTESIAN_POINT('Ctrl Pts',(-43.5379105932515,29.7911319045234,
-38.9164678395448));
#254455=CARTESIAN_POINT('Ctrl Pts',(-43.5672796770166,29.7754780139697,
-38.919349653254));
#254456=CARTESIAN_POINT('Ctrl Pts',(-43.5966487607817,29.7598241234161,
-38.9222314669631));
#254457=CARTESIAN_POINT('Ctrl Pts',(-43.6266146289649,29.7448030239206,
-38.9253708095819));
#254458=CARTESIAN_POINT('Ctrl Pts',(-43.6567606170124,29.7306258031448,
-38.9287240628825));
#254459=CARTESIAN_POINT('Ctrl Pts',(-43.68690660506,29.7164485823689,-38.9320773161831));
#254460=CARTESIAN_POINT('Ctrl Pts',(-43.7172788205642,29.7030822942954,
-38.9356472530647));
#254461=CARTESIAN_POINT('Ctrl Pts',(-43.74787091788,29.6905129658013,-38.9394291519851));
#254462=CARTESIAN_POINT('Ctrl Pts',(-43.7784630151957,29.6779436373071,
-38.9432110509055));
#254463=CARTESIAN_POINT('Ctrl Pts',(-43.8092755239302,29.666170138253,-38.9472047867905));
#254464=CARTESIAN_POINT('Ctrl Pts',(-43.8403053963098,29.655181264008,-38.9514068723595));
#254465=CARTESIAN_POINT('Ctrl Pts',(-43.8713352686894,29.644192389763,-38.9556089579285));
#254466=CARTESIAN_POINT('Ctrl Pts',(-43.9025825141023,29.6339881744307,
-38.9600194027673));
#254467=CARTESIAN_POINT('Ctrl Pts',(-43.9340457277949,29.6245633327707,
-38.9646362624899));
#254468=CARTESIAN_POINT('Ctrl Pts',(-43.9655089414875,29.6151384911106,
-38.9692531222126));
#254469=CARTESIAN_POINT('Ctrl Pts',(-43.9971881260961,29.6064930329024,
-38.9740764000692));
#254470=CARTESIAN_POINT('Ctrl Pts',(-44.0290834665269,29.5986273975902,
-38.9791056375968));
#254471=CARTESIAN_POINT('Ctrl Pts',(-44.0609788069577,29.5907617622781,
-38.9841348751245));
#254472=CARTESIAN_POINT('Ctrl Pts',(-44.0930902993264,29.5836759361658,
-38.9893700694948));
#254473=CARTESIAN_POINT('Ctrl Pts',(-44.1254197237287,29.5773761007637,
-38.9948122462768));
#254474=CARTESIAN_POINT('Ctrl Pts',(-44.157749148131,29.5710762653616,-39.0002544230587));
#254475=CARTESIAN_POINT('Ctrl Pts',(-44.1902803880436,29.5655649308414,
-39.0059007403469));
#254476=CARTESIAN_POINT('Ctrl Pts',(-44.2230652009806,29.5608466061619,
-39.0117622591756));
#254477=CARTESIAN_POINT('Ctrl Pts',(-44.2394576074491,29.5584874438222,
-39.01469301859));
#254478=CARTESIAN_POINT('Ctrl Pts',(-44.2558936005359,29.556330581768,-39.017674281006));
#254479=CARTESIAN_POINT('Ctrl Pts',(-44.2722948154515,29.5543845957057,
-39.0206914003809));
#254480=CARTESIAN_POINT('Ctrl Pts',(-44.288696030367,29.5524386096434,-39.0237085197559));
#254481=CARTESIAN_POINT('Ctrl Pts',(-44.3050952734896,29.5506978499007,
-39.0267671710297));
#254482=CARTESIAN_POINT('Ctrl Pts',(-44.3214722160119,29.5491651362618,
-39.0298636173565));
#254483=CARTESIAN_POINT('Ctrl Pts',(-44.386979986101,29.5430342817064,-39.0422494026637));
#254484=CARTESIAN_POINT('Ctrl Pts',(-44.4523142911657,29.5401658847829,
-39.0552645001479));
#254485=CARTESIAN_POINT('Ctrl Pts',(-44.5174452018332,29.5404749664642,
-39.0688802121094));
#254486=CARTESIAN_POINT('Ctrl Pts',(-44.5825761125008,29.5407840481454,
-39.0824959240709));
#254487=CARTESIAN_POINT('Ctrl Pts',(-44.64751868345,29.5442668522271,-39.0967146367708));
#254488=CARTESIAN_POINT('Ctrl Pts',(-44.7122655456777,29.5509157680261,
-39.1115282314101));
#254489=CARTESIAN_POINT('Ctrl Pts',(-44.7446389767916,29.5542402259256,
-39.1189350287298));
#254490=CARTESIAN_POINT('Ctrl Pts',(-44.7769718892781,29.5583592071516,
-39.126492904595));
#254491=CARTESIAN_POINT('Ctrl Pts',(-44.8092469543588,29.5632772749199,
-39.1341985554971));
#254492=CARTESIAN_POINT('Ctrl Pts',(-44.8415220194395,29.5681953426883,
-39.1419042063993));
#254493=CARTESIAN_POINT('Ctrl Pts',(-44.873794287365,29.5739237069059,-39.1497713394166));
#254494=CARTESIAN_POINT('Ctrl Pts',(-44.9059258943645,29.580448064776,-39.1577677872645));
#254495=CARTESIAN_POINT('Ctrl Pts',(-44.938057501364,29.5869724226462,-39.1657642351124));
#254496=CARTESIAN_POINT('Ctrl Pts',(-44.9698454327154,29.5942479284801,
-39.1738387467903));
#254497=CARTESIAN_POINT('Ctrl Pts',(-45.0013540521658,29.6022690447016,
-39.1820030835632));
#254498=CARTESIAN_POINT('Ctrl Pts',(-45.0328626716162,29.6102901609231,
-39.1901674203362));
#254499=CARTESIAN_POINT('Ctrl Pts',(-45.0640728677801,29.6190530040921,
-39.1984168268269));
#254500=CARTESIAN_POINT('Ctrl Pts',(-45.0949895328334,29.6285456745752,
-39.2067494504582));
#254501=CARTESIAN_POINT('Ctrl Pts',(-45.0988345002,29.6297262355499,-39.207785741594));
#254502=CARTESIAN_POINT('Ctrl Pts',(-45.1026749334513,29.630918067705,-39.2088233175957));
#254503=CARTESIAN_POINT('Ctrl Pts',(-45.1065107582268,29.6321211388928,
-39.2098621557269));
#254504=CARTESIAN_POINT('Ctrl Pts',(-42.5264433853035,31.2691187985001,
-39.0141965709288));
#254505=CARTESIAN_POINT('Ctrl Pts',(-42.533975017942,31.2141173491589,-39.0171948856712));
#254506=CARTESIAN_POINT('Ctrl Pts',(-42.5438622229547,31.1589786372441,
-39.0202688264213));
#254507=CARTESIAN_POINT('Ctrl Pts',(-42.5561557287987,31.1040026525962,
-39.023404719375));
#254508=CARTESIAN_POINT('Ctrl Pts',(-42.5683599682557,31.0494258630668,
-39.0265178417832));
#254509=CARTESIAN_POINT('Ctrl Pts',(-42.5829359045809,30.9950101372705,
-39.0296919913082));
#254510=CARTESIAN_POINT('Ctrl Pts',(-42.5998833018802,30.9410609056468,
-39.0329117328335));
#254511=CARTESIAN_POINT('Ctrl Pts',(-42.6167409587158,30.8873973479218,
-39.0361144250685));
#254512=CARTESIAN_POINT('Ctrl Pts',(-42.6359450801664,30.834196084843,-39.0393621924919));
#254513=CARTESIAN_POINT('Ctrl Pts',(-42.6574438939907,30.7817589584099,
-39.0426382781429));
#254514=CARTESIAN_POINT('Ctrl Pts',(-42.6788724270608,30.7294932517034,
-39.0459036540975));
#254515=CARTESIAN_POINT('Ctrl Pts',(-42.7025805580132,30.6779874187089,
-39.0491971234277));
#254516=CARTESIAN_POINT('Ctrl Pts',(-42.7284661350043,30.6275306909273,
-39.0525010968636));
#254517=CARTESIAN_POINT('Ctrl Pts',(-42.7543356047292,30.5771053597781,
-39.0558030144063));
#254518=CARTESIAN_POINT('Ctrl Pts',(-42.7823795359021,30.5277285141059,
-39.0591153803188));
#254519=CARTESIAN_POINT('Ctrl Pts',(-42.8124479723331,30.4796685666064,
-39.0624202628221));
#254520=CARTESIAN_POINT('Ctrl Pts',(-42.8425499311369,30.4315550385532,
-39.065728829837));
#254521=CARTESIAN_POINT('Ctrl Pts',(-42.8746804827911,30.3847619516162,
-39.0690298536715));
#254522=CARTESIAN_POINT('Ctrl Pts',(-42.9086463432861,30.3395285449195,
-39.072305612684));
#254523=CARTESIAN_POINT('Ctrl Pts',(-42.9427092073028,30.2941659555764,
-39.0755907269772));
#254524=CARTESIAN_POINT('Ctrl Pts',(-42.978617320009,30.2503724567378,-39.0788503909572));
#254525=CARTESIAN_POINT('Ctrl Pts',(-43.0161401302784,30.2083508338029,
-39.0820676376815));
#254526=CARTESIAN_POINT('Ctrl Pts',(-43.0539958194939,30.1659564212647,
-39.0853134258101));
#254527=CARTESIAN_POINT('Ctrl Pts',(-43.0934943374488,30.1253658443146,
-39.088516002619));
#254528=CARTESIAN_POINT('Ctrl Pts',(-43.1343718380936,30.0867415073552,
-39.0916594701529));
#254529=CARTESIAN_POINT('Ctrl Pts',(-43.1754823554595,30.0478969975327,
-39.0948208566027));
#254530=CARTESIAN_POINT('Ctrl Pts',(-43.2179868945264,30.0110413889675,
-39.0979224276242));
#254531=CARTESIAN_POINT('Ctrl Pts',(-43.2616002290463,29.9762894859414,
-39.1009500664389));
#254532=CARTESIAN_POINT('Ctrl Pts',(-43.3057813273405,29.9410851783504,
-39.1040171194296));
#254533=CARTESIAN_POINT('Ctrl Pts',(-43.3510995292929,29.9080397621653,
-39.107008278067));
#254534=CARTESIAN_POINT('Ctrl Pts',(-43.3972523236822,29.8772191026902,
-39.109911393871));
#254535=CARTESIAN_POINT('Ctrl Pts',(-43.4336815722595,29.852891789898,-39.1122028765141));
#254536=CARTESIAN_POINT('Ctrl Pts',(-43.4706305620717,29.8299494375692,
-39.1144395560518));
#254537=CARTESIAN_POINT('Ctrl Pts',(-43.5079524583199,29.8084016307237,
-39.1166166666663));
#254538=CARTESIAN_POINT('Ctrl Pts',(-43.5553799427766,29.7810193598056,
-39.1193832699262));
#254539=CARTESIAN_POINT('Ctrl Pts',(-43.6044581995708,29.7552851959446,
-39.1222461913981));
#254540=CARTESIAN_POINT('Ctrl Pts',(-43.6550143791165,29.7314482427253,
-39.1251953413445));
#254541=CARTESIAN_POINT('Ctrl Pts',(-43.7050241825406,29.7078689027626,
-39.1281126189239));
#254542=CARTESIAN_POINT('Ctrl Pts',(-43.756479873319,29.6861466532943,-39.1311142558983));
#254543=CARTESIAN_POINT('Ctrl Pts',(-43.8091686689389,29.6664994960942,
-39.1341878331413));
#254544=CARTESIAN_POINT('Ctrl Pts',(-43.8612441375445,29.6470810427793,
-39.1372256322283));
#254545=CARTESIAN_POINT('Ctrl Pts',(-43.9145237443489,29.6296902265431,
-39.1403336816531));
#254546=CARTESIAN_POINT('Ctrl Pts',(-43.9687625207563,29.61450562165,-39.1434976847857));
#254547=CARTESIAN_POINT('Ctrl Pts',(-44.0226897493758,29.5994082371991,
-39.1466435138693));
#254548=CARTESIAN_POINT('Ctrl Pts',(-44.0775646322468,29.5864922846488,
-39.1498446249087));
#254549=CARTESIAN_POINT('Ctrl Pts',(-44.1331141493744,29.5758935484052,
-39.1530850848182));
#254550=CARTESIAN_POINT('Ctrl Pts',(-44.1884409379484,29.565337308322,-39.1563125519425));
#254551=CARTESIAN_POINT('Ctrl Pts',(-44.244436327736,29.5570801011644,-39.1595790160483));
#254552=CARTESIAN_POINT('Ctrl Pts',(-44.3008071787297,29.5512101408557,
-39.1628673702128));
#254553=CARTESIAN_POINT('Ctrl Pts',(-44.3570499030541,29.5453535225217,
-39.1661482501976));
#254554=CARTESIAN_POINT('Ctrl Pts',(-44.4136656784857,29.5418735174476,
-39.1694508797056));
#254555=CARTESIAN_POINT('Ctrl Pts',(-44.4703500735278,29.540807629945,-39.1727574929379));
#254556=CARTESIAN_POINT('Ctrl Pts',(-44.5270863560613,29.5397407667554,
-39.1760671329622));
#254557=CARTESIAN_POINT('Ctrl Pts',(-44.5838906443107,29.5410924924669,
-39.1793807208643));
#254558=CARTESIAN_POINT('Ctrl Pts',(-44.6404552194646,29.5448481851576,
-39.1826802988214));
#254559=CARTESIAN_POINT('Ctrl Pts',(-44.6970922205564,29.5486086866808,
-39.1859841015965));
#254560=CARTESIAN_POINT('Ctrl Pts',(-44.7534881638628,29.5547791795424,
-39.1892738159161));
#254561=CARTESIAN_POINT('Ctrl Pts',(-44.8093427863577,29.5632932892976,
-39.1925319186275));
#254562=CARTESIAN_POINT('Ctrl Pts',(-44.8655321438493,29.5718584238448,
-39.1958095470461));
#254563=CARTESIAN_POINT('Ctrl Pts',(-44.9211729794212,29.5827950700452,
-39.1990551433739));
#254564=CARTESIAN_POINT('Ctrl Pts',(-44.9759791375788,29.5959864507854,
-39.2022520070656));
#254565=CARTESIAN_POINT('Ctrl Pts',(-45.0200746694849,29.6065998739822,
-39.2048241159244));
#254566=CARTESIAN_POINT('Ctrl Pts',(-45.0636301540079,29.6186718150447,
-39.2073646941016));
#254567=CARTESIAN_POINT('Ctrl Pts',(-45.1065099250746,29.6321209281423,
-39.2098658234324));
#254568=CARTESIAN_POINT('Ctrl Pts',(-46.6981266849492,30.7091523375488,
-39.2904704603133));
#254569=CARTESIAN_POINT('Ctrl Pts',(-46.6689684123063,30.6404043382273,
-39.273452295095));
#254570=CARTESIAN_POINT('Ctrl Pts',(-46.6043681216411,30.5066861069553,
-39.238925705885));
#254571=CARTESIAN_POINT('Ctrl Pts',(-46.5083209189471,30.3487389562033,
-39.1945593129175));
#254572=CARTESIAN_POINT('Ctrl Pts',(-46.4437937583117,30.2581216171786,
-39.1673894861782));
#254573=CARTESIAN_POINT('Ctrl Pts',(-46.3992224148768,30.1986447451181,
-39.1491520227249));
#254574=CARTESIAN_POINT('Ctrl Pts',(-46.3761748773305,30.1693908446446,
-39.1399767764946));
#254575=CARTESIAN_POINT('Ctrl Pts',(-46.3284414024809,30.1117648114071,
-39.1214771434543));
#254576=CARTESIAN_POINT('Ctrl Pts',(-46.3038983378397,30.083571828401,-39.112209259666));
#254577=CARTESIAN_POINT('Ctrl Pts',(-46.253707387608,30.0286632749651,-39.0937226519629));
#254578=CARTESIAN_POINT('Ctrl Pts',(-46.2280147026909,30.001893564456,-39.0844865568113));
#254579=CARTESIAN_POINT('Ctrl Pts',(-46.1492148010453,29.9236586721517,
-39.0568159196779));
#254580=CARTESIAN_POINT('Ctrl Pts',(-46.0669347173688,29.8495134741745,
-39.0292038481275));
#254581=CARTESIAN_POINT('Ctrl Pts',(-45.9503410384262,29.7587889734315,
-38.9925114043613));
#254582=CARTESIAN_POINT('Ctrl Pts',(-45.8594191065401,29.6948377475824,
-38.9650526418885));
#254583=CARTESIAN_POINT('Ctrl Pts',(-45.7964751089327,29.6549785818455,
-38.9467936623891));
#254584=CARTESIAN_POINT('Ctrl Pts',(-45.748348603817,29.6261284949947,-38.9331097524421));
#254585=CARTESIAN_POINT('Ctrl Pts',(-45.7321473284057,29.616684052073,-38.9285487676403));
#254586=CARTESIAN_POINT('Ctrl Pts',(-45.6996106203311,29.5982459977232,
-38.9194791520014));
#254587=CARTESIAN_POINT('Ctrl Pts',(-45.683249044345,29.5892352448745,-38.9149628379356));
#254588=CARTESIAN_POINT('Ctrl Pts',(-45.6010439155842,29.5452684013657,
-38.8924942188443));
#254589=CARTESIAN_POINT('Ctrl Pts',(-45.4667739830181,29.4816584171599,
-38.8571935516581));
#254590=CARTESIAN_POINT('Ctrl Pts',(-45.2922645146651,29.4187721922835,
-38.8147007629208));
#254591=CARTESIAN_POINT('Ctrl Pts',(-45.184512437616,29.3885937253944,-38.7899522655792));
#254592=CARTESIAN_POINT('Ctrl Pts',(-45.1119891467798,29.3701842541612,
-38.7736235920333));
#254593=CARTESIAN_POINT('Ctrl Pts',(-45.0754052578815,29.3618381514785,
-38.7655490803555));
#254594=CARTESIAN_POINT('Ctrl Pts',(-45.0014447932705,29.3468760834356,
-38.7495561846596));
#254595=CARTESIAN_POINT('Ctrl Pts',(-44.964301863367,29.3403115562353,-38.7416890516424));
#254596=CARTESIAN_POINT('Ctrl Pts',(-44.8900079594565,29.3290481892184,
-38.726277749838));
#254597=CARTESIAN_POINT('Ctrl Pts',(-44.8527936282157,29.324336495618,-38.7187198739728));
#254598=CARTESIAN_POINT('Ctrl Pts',(-44.7410083373266,29.3129455735289,
-38.6964994820139));
#254599=CARTESIAN_POINT('Ctrl Pts',(-44.6662563757167,29.3089967422249,
-38.6822807693139));
#254600=CARTESIAN_POINT('Ctrl Pts',(-44.516312468428,29.3084067934202,-38.6550493453909));
#254601=CARTESIAN_POINT('Ctrl Pts',(-44.441103189525,29.3117700143417,-38.6420342479066));
#254602=CARTESIAN_POINT('Ctrl Pts',(-44.3468378615956,29.3206690055189,
-38.6265520162729));
#254603=CARTESIAN_POINT('Ctrl Pts',(-44.3279589148655,29.3226883315868,
-38.6234933649988));
#254604=CARTESIAN_POINT('Ctrl Pts',(-44.2901960653062,29.3271995080042,
-38.6174591262491));
#254605=CARTESIAN_POINT('Ctrl Pts',(-44.271274393292,29.329697893027,-38.614477863833));
#254606=CARTESIAN_POINT('Ctrl Pts',(-44.2146592782019,29.3378915995821,
-38.60568558559));
#254607=CARTESIAN_POINT('Ctrl Pts',(-44.1772069502033,29.344266758826,-38.6000392683017));
#254608=CARTESIAN_POINT('Ctrl Pts',(-44.0655444875092,29.3661148598052,
-38.5837127379559));
#254609=CARTESIAN_POINT('Ctrl Pts',(-43.9553791862171,29.3933792052515,
-38.5686255047386));
#254610=CARTESIAN_POINT('Ctrl Pts',(-43.8114622524781,29.4404829778103,
-38.5509833019505));
#254611=CARTESIAN_POINT('Ctrl Pts',(-43.705021834675,29.481230340464,-38.5390021142185));
#254612=CARTESIAN_POINT('Ctrl Pts',(-43.6350719757086,29.512061063653,-38.5318621614261));
#254613=CARTESIAN_POINT('Ctrl Pts',(-43.5656410085295,29.5447591316771,
-38.525155654825));
#254614=CARTESIAN_POINT('Ctrl Pts',(-43.5311320054746,29.5620794464364,
-38.5220163122062));
#254615=CARTESIAN_POINT('Ctrl Pts',(-43.4634866412134,29.5981758355574,
-38.5162526847879));
#254616=CARTESIAN_POINT('Ctrl Pts',(-43.4301834663392,29.6170276546,-38.5136117755133));
#254617=CARTESIAN_POINT('Ctrl Pts',(-43.3647025891651,29.6562685687332,
-38.5088155315793));
#254618=CARTESIAN_POINT('Ctrl Pts',(-43.2681192378476,29.7174608121974,
-38.5023448938576));
#254619=CARTESIAN_POINT('Ctrl Pts',(-43.1764049274077,29.7855824582168,
-38.4980286134812));
#254620=CARTESIAN_POINT('Ctrl Pts',(-43.0584774180437,29.8826126224142,
-38.4942050936184));
#254621=CARTESIAN_POINT('Ctrl Pts',(-43.001681818637,29.9342392650769,-38.4932590761897));
#254622=CARTESIAN_POINT('Ctrl Pts',(-42.8926599718677,30.0438904492243,
-38.4933742455196));
#254623=CARTESIAN_POINT('Ctrl Pts',(-42.8414047150844,30.1009342501745,
-38.4944336470273));
#254624=CARTESIAN_POINT('Ctrl Pts',(-42.7451036203247,30.2193471227021,
-38.498479276642));
#254625=CARTESIAN_POINT('Ctrl Pts',(-42.6550322643363,30.3420646399833,
-38.5044516702661));
#254626=CARTESIAN_POINT('Ctrl Pts',(-42.5773225406025,30.4733365238586,
-38.5142428327574));
#254627=CARTESIAN_POINT('Ctrl Pts',(-42.5326943378214,30.5580963840027,
-38.5215739479982));
#254628=CARTESIAN_POINT('Ctrl Pts',(-42.5239673850246,30.5751883092729,
-38.5231018165939));
#254629=CARTESIAN_POINT('Ctrl Pts',(-42.5069121510755,30.60964376351,-38.5262794637242));
#254630=CARTESIAN_POINT('Ctrl Pts',(-42.4985805781952,30.627019094627,-38.5279307934181));
#254631=CARTESIAN_POINT('Ctrl Pts',(-42.4743295471271,30.6792614198295,
-38.5330409224498));
#254632=CARTESIAN_POINT('Ctrl Pts',(-42.4438856226513,30.7493896366731,
-38.5402834483744));
#254633=CARTESIAN_POINT('Ctrl Pts',(-42.4037483179465,30.8560072598611,
-38.5524071291592));
#254634=CARTESIAN_POINT('Ctrl Pts',(-42.3690543371876,30.9640160484273,
-38.5657659376104));
#254635=CARTESIAN_POINT('Ctrl Pts',(-42.3397558527982,31.0734075527136,
-38.5803463747351));
#254636=CARTESIAN_POINT('Ctrl Pts',(-42.3238156343608,31.1472555030051,
-38.5908775753381));
#254637=CARTESIAN_POINT('Ctrl Pts',(-42.3096820427396,31.2215665449467,
-38.6018154236264));
#254638=CARTESIAN_POINT('Ctrl Pts',(-42.3035171869091,31.2589715314082,
-38.6074906718877));
#254639=CARTESIAN_POINT('Ctrl Pts',(-42.2930235524414,31.3341791410138,
-38.6192399292287));
#254640=CARTESIAN_POINT('Ctrl Pts',(-42.2886818075092,31.3721585359098,
-38.6253436316658));
#254641=CARTESIAN_POINT('Ctrl Pts',(-42.281930630611,31.4478003630713,-38.6378362101326));
#254642=CARTESIAN_POINT('Ctrl Pts',(-42.277074994566,31.5232809912004,-38.6506356205751));
#254643=CARTESIAN_POINT('Ctrl Pts',(-42.2747992363309,31.6735553614761,
-38.6774229397946));
#254644=CARTESIAN_POINT('Ctrl Pts',(-42.2834818483937,31.8228397562226,
-38.7059581415094));
#254645=CARTESIAN_POINT('Ctrl Pts',(-42.3030248127084,31.9711385758679,
-38.7362097844166));
#254646=CARTESIAN_POINT('Ctrl Pts',(-42.3164494406915,32.0449687602614,
-38.7519128032936));
#254647=CARTESIAN_POINT('Ctrl Pts',(-42.3317154579634,32.1186122141692,
-38.7679009120377));
#254648=CARTESIAN_POINT('Ctrl Pts',(-42.3402956643805,32.1554227583218,
-38.7760569897633));
#254649=CARTESIAN_POINT('Ctrl Pts',(-42.3591481714288,32.228169160774,-38.7925026060078));
#254650=CARTESIAN_POINT('Ctrl Pts',(-42.3694448348212,32.2642362896146,
-38.8008201507359));
#254651=CARTESIAN_POINT('Ctrl Pts',(-42.4028917825415,32.3714169561226,
-38.8260275044574));
#254652=CARTESIAN_POINT('Ctrl Pts',(-42.428602574983,32.4415633880281,-38.8431823298655));
#254653=CARTESIAN_POINT('Ctrl Pts',(-42.4722685042023,32.5448307979217,
-38.8694323201497));
#254654=CARTESIAN_POINT('Ctrl Pts',(-42.4876674804306,32.5789105800712,
-38.8782643966373));
#254655=CARTESIAN_POINT('Ctrl Pts',(-42.5202146590728,32.6464795812123,
-38.8961197808447));
#254656=CARTESIAN_POINT('Ctrl Pts',(-42.5373018269229,32.6798350022668,
-38.9051083126545));
#254657=CARTESIAN_POINT('Ctrl Pts',(-42.5906929412925,32.7780783962456,
-38.9321048428364));
#254658=CARTESIAN_POINT('Ctrl Pts',(-42.629225789877,32.8414173722334,-38.9502105255135));
#254659=CARTESIAN_POINT('Ctrl Pts',(-42.7120000069194,32.9638220552461,
-38.9866125955294));
#254660=CARTESIAN_POINT('Ctrl Pts',(-42.7783647966162,33.0524402968179,
-39.0140612314234));
#254661=CARTESIAN_POINT('Ctrl Pts',(-42.8754380724448,33.1642175243331,
-39.0509520337677));
#254662=CARTESIAN_POINT('Ctrl Pts',(-42.9268673384212,33.2179450225078,
-39.0694937486382));
#254663=CARTESIAN_POINT('Ctrl Pts',(-42.9797817061918,33.2705900457306,
-39.088089881442));
#254664=CARTESIAN_POINT('Ctrl Pts',(-43.0069972096607,33.2963736994336,
-39.097418269769));
#254665=CARTESIAN_POINT('Ctrl Pts',(-43.0622936398443,33.3462615369726,
-39.1159154063528));
#254666=CARTESIAN_POINT('Ctrl Pts',(-43.0904949946047,33.3704876748183,
-39.1251268688783));
#254667=CARTESIAN_POINT('Ctrl Pts',(-43.176562606447,33.4408730143712,-39.1525915568785));
#254668=CARTESIAN_POINT('Ctrl Pts',(-43.2360245534179,33.4848790444095,
-39.1707230137558));
#254669=CARTESIAN_POINT('Ctrl Pts',(-43.358992255749,33.5670176609587,-39.2066046432507));
#254670=CARTESIAN_POINT('Ctrl Pts',(-43.4542745623933,33.6242424638975,
-39.233238623837));
#254671=CARTESIAN_POINT('Ctrl Pts',(-43.5542222374601,33.6747516510336,
-39.2594493821381));
#254672=CARTESIAN_POINT('Ctrl Pts',(-43.6219256430316,33.7069073870393,
-39.2768314299875));
#254673=CARTESIAN_POINT('Ctrl Pts',(-43.6563381479934,33.7222286468184,
-39.2854811722856));
#254674=CARTESIAN_POINT('Ctrl Pts',(-43.7254519170511,33.7509934760635,
-39.3024907499371));
#254675=CARTESIAN_POINT('Ctrl Pts',(-43.7602995448845,33.7645084608315,
-39.3108885064059));
#254676=CARTESIAN_POINT('Ctrl Pts',(-43.8304781084082,33.789780836939,-39.3274499785309));
#254677=CARTESIAN_POINT('Ctrl Pts',(-43.9365171946568,33.8250735562425,
-39.3519527568515));
#254678=CARTESIAN_POINT('Ctrl Pts',(-44.0809642638621,33.8617420360433,
-39.3832806139221));
#254679=CARTESIAN_POINT('Ctrl Pts',(-44.1916183723467,33.8813683146414,
-39.4057679385072));
#254680=CARTESIAN_POINT('Ctrl Pts',(-44.2659122959159,33.8926702964892,
-39.4205323411483));
#254681=CARTESIAN_POINT('Ctrl Pts',(-44.3033049221432,33.8974288658374,
-39.4277978831022));
#254682=CARTESIAN_POINT('Ctrl Pts',(-44.3598453576919,33.9032050944765,
-39.4385322478049));
#254683=CARTESIAN_POINT('Ctrl Pts',(-44.3787527158677,33.9049006163346,
-39.4420799976889));
#254684=CARTESIAN_POINT('Ctrl Pts',(-44.4164967874688,33.9078161173588,
-39.4490791780208));
#254685=CARTESIAN_POINT('Ctrl Pts',(-44.4353708468856,33.9090400957878,
-39.4525377314439));
#254686=CARTESIAN_POINT('Ctrl Pts',(-44.4919347179527,33.9120095261765,
-39.462779235967));
#254687=CARTESIAN_POINT('Ctrl Pts',(-44.52962054914,33.9130584408517,-39.4694384189012));
#254688=CARTESIAN_POINT('Ctrl Pts',(-44.6425299001817,33.9134342925821,
-39.4889026473125));
#254689=CARTESIAN_POINT('Ctrl Pts',(-44.7176656228988,33.9100023852834,
-39.5012068570978));
#254690=CARTESIAN_POINT('Ctrl Pts',(-44.867623327666,33.8957625538083,-39.524471978366));
#254691=CARTESIAN_POINT('Ctrl Pts',(-44.9424659600731,33.8849485744664,
-39.5354353652432));
#254692=CARTESIAN_POINT('Ctrl Pts',(-45.0357885152669,33.8666999843662,
-39.5482785606344));
#254693=CARTESIAN_POINT('Ctrl Pts',(-45.0544546343785,33.8628074782943,
-39.5508053225112));
#254694=CARTESIAN_POINT('Ctrl Pts',(-45.091743102575,33.8545484160302,-39.5557691634051));
#254695=CARTESIAN_POINT('Ctrl Pts',(-45.1104022544846,33.850171655015,-39.5582107864407));
#254696=CARTESIAN_POINT('Ctrl Pts',(-45.1661672125598,33.8363538303533,
-39.5653802281989));
#254697=CARTESIAN_POINT('Ctrl Pts',(-45.2029511118778,33.8262578362557,
-39.5699395109212));
#254698=CARTESIAN_POINT('Ctrl Pts',(-45.312316831343,33.7933159380614,-39.582990524906));
#254699=CARTESIAN_POINT('Ctrl Pts',(-45.4195983160475,33.7551076509549,
-39.5947758536238));
#254700=CARTESIAN_POINT('Ctrl Pts',(-45.5585113890164,33.6937328563153,
-39.6079933748399));
#254701=CARTESIAN_POINT('Ctrl Pts',(-45.6606150024606,33.6424505696195,
-39.6166516297843));
#254702=CARTESIAN_POINT('Ctrl Pts',(-45.7272860947277,33.6047101271221,
-39.6215780075552));
#254703=CARTESIAN_POINT('Ctrl Pts',(-45.7932287365117,33.5651705839516,
-39.6260731428005));
#254704=CARTESIAN_POINT('Ctrl Pts',(-45.8259059249178,33.5444453395394,
-39.6281074988013));
#254705=CARTESIAN_POINT('Ctrl Pts',(-45.8897275017006,33.5016881508368,
-39.6316923737189));
#254706=CARTESIAN_POINT('Ctrl Pts',(-45.9210297733036,33.4795651380848,
-39.6332542688506));
#254707=CARTESIAN_POINT('Ctrl Pts',(-45.9823424846244,33.4339088874735,
-39.6359180193303));
#254708=CARTESIAN_POINT('Ctrl Pts',(-46.0724202597563,33.3632801300718,
-39.6392265347984));
#254709=CARTESIAN_POINT('Ctrl Pts',(-46.1850394564173,33.2606222983665,
-39.6409205727319));
#254710=CARTESIAN_POINT('Ctrl Pts',(-46.2638636333332,33.1772336958075,
-39.6401443034625));
#254711=CARTESIAN_POINT('Ctrl Pts',(-46.3151397511292,33.1201974856456,
-39.6391646017005));
#254712=CARTESIAN_POINT('Ctrl Pts',(-46.3401349353408,33.0909661742941,
-39.6384440851485));
#254713=CARTESIAN_POINT('Ctrl Pts',(-46.3888523044997,33.0309971480077,
-39.6365301000439));
#254714=CARTESIAN_POINT('Ctrl Pts',(-46.4123735341802,33.0005036828642,
-39.6353439924849));
#254715=CARTESIAN_POINT('Ctrl Pts',(-46.4576879006691,32.9386388625828,
-39.6325280276393));
#254716=CARTESIAN_POINT('Ctrl Pts',(-46.52311576659,32.8444620833496,-39.6276360146217));
#254717=CARTESIAN_POINT('Ctrl Pts',(-46.5810426872604,32.7462345994881,
-39.6207752343847));
#254718=CARTESIAN_POINT('Ctrl Pts',(-46.6516918187307,32.6117039458857,
-39.6098936921283));
#254719=CARTESIAN_POINT('Ctrl Pts',(-46.683723185051,32.5426422373878,-39.6035832967262));
#254720=CARTESIAN_POINT('Ctrl Pts',(-46.7195635412788,32.4540883209461,
-39.5945936116187));
#254721=CARTESIAN_POINT('Ctrl Pts',(-46.7265235775841,32.4362514419463,
-39.5927383889278));
#254722=CARTESIAN_POINT('Ctrl Pts',(-46.7400123459627,32.4003742100513,
-39.5889189813535));
#254723=CARTESIAN_POINT('Ctrl Pts',(-46.7465535157541,32.3822946053341,
-39.5869502184844));
#254724=CARTESIAN_POINT('Ctrl Pts',(-46.7654644360989,32.3279072933142,
-39.5808958427402));
#254725=CARTESIAN_POINT('Ctrl Pts',(-46.7770937339888,32.2915493874551,
-39.5766741707955));
#254726=CARTESIAN_POINT('Ctrl Pts',(-46.8091770518909,32.182013131159,-39.5634457571489));
#254727=CARTESIAN_POINT('Ctrl Pts',(-46.8444383818759,32.034891308334,-39.5443264312115));
#254728=CARTESIAN_POINT('Ctrl Pts',(-46.8650708643864,31.8856621776612,
-39.5223044891954));
#254729=CARTESIAN_POINT('Ctrl Pts',(-46.8750487417844,31.7729724844591,
-39.50469487268));
#254730=CARTESIAN_POINT('Ctrl Pts',(-46.8774570362353,31.7352651712118,
-39.4986397605723));
#254731=CARTESIAN_POINT('Ctrl Pts',(-46.8796767940079,31.6785286095959,
-39.4892824810203));
#254732=CARTESIAN_POINT('Ctrl Pts',(-46.8801843407089,31.6595724593507,
-39.4861150486293));
#254733=CARTESIAN_POINT('Ctrl Pts',(-46.8807312344332,31.6216180949417,
-39.479690628598));
#254734=CARTESIAN_POINT('Ctrl Pts',(-46.8807699646674,31.6025797052015,
-39.4764266299692));
#254735=CARTESIAN_POINT('Ctrl Pts',(-46.8801790388754,31.5455906639181,
-39.4665317368708));
#254736=CARTESIAN_POINT('Ctrl Pts',(-46.8788490796135,31.5078273383739,
-39.4598096545541));
#254737=CARTESIAN_POINT('Ctrl Pts',(-46.874360617844,31.4326451774338,-39.4461013696832));
#254738=CARTESIAN_POINT('Ctrl Pts',(-46.864884835636,31.320441459725,-39.4251517854185));
#254739=CARTESIAN_POINT('Ctrl Pts',(-46.8414902947658,31.1730719473388,
-39.3956936109857));
#254740=CARTESIAN_POINT('Ctrl Pts',(-46.8074810934279,31.0279105813681,
-39.364717848004));
#254741=CARTESIAN_POINT('Ctrl Pts',(-46.7869180083019,30.9560697433081,
-39.3487190247537));
#254742=CARTESIAN_POINT('Ctrl Pts',(-46.7645577771926,30.884604709384,-39.332461491893));
#254743=CARTESIAN_POINT('Ctrl Pts',(-46.7524740339114,30.8490466969583,
-39.3242001683612));
#254744=CARTESIAN_POINT('Ctrl Pts',(-46.7264943673172,30.7783632715819,
-39.3074248425479));
#254745=CARTESIAN_POINT('Ctrl Pts',(-46.7127058212706,30.7435263372096,
-39.2989795429224));
#254746=CARTESIAN_POINT('Ctrl Pts',(-46.6981266849492,30.7091523375488,
-39.2904704603133));
#254747=CARTESIAN_POINT('Ctrl Pts',(-45.0394875320819,30.9432190801919,
-41.190386719266));
#254748=CARTESIAN_POINT('Ctrl Pts',(-45.0282734427409,30.91723575627,-41.1733685540478));
#254749=CARTESIAN_POINT('Ctrl Pts',(-45.0034876660128,30.8666726764904,
-41.1388419648381));
#254750=CARTESIAN_POINT('Ctrl Pts',(-44.9667665375866,30.8068862988478,
-41.09447557187));
#254751=CARTESIAN_POINT('Ctrl Pts',(-44.9421458413835,30.7725558756156,
-41.0673057451311));
#254752=CARTESIAN_POINT('Ctrl Pts',(-44.9251493960809,30.7500159625169,
-41.0490682816776));
#254753=CARTESIAN_POINT('Ctrl Pts',(-44.9163654668634,30.7389260450349,
-41.0398930354472));
#254754=CARTESIAN_POINT('Ctrl Pts',(-44.8981827131164,30.7170729960788,
-41.0213934024069));
#254755=CARTESIAN_POINT('Ctrl Pts',(-44.888838333634,30.7063777841388,-41.0121255186188));
#254756=CARTESIAN_POINT('Ctrl Pts',(-44.8697378119757,30.6855401076749,
-40.9936389109155));
#254757=CARTESIAN_POINT('Ctrl Pts',(-44.8599646045333,30.6753771122426,
-40.984402815764));
#254758=CARTESIAN_POINT('Ctrl Pts',(-44.8300025766326,30.6456635434001,
-40.9567321786306));
#254759=CARTESIAN_POINT('Ctrl Pts',(-44.7987417882795,30.6174785558847,
-40.9291201070801));
#254760=CARTESIAN_POINT('Ctrl Pts',(-44.7544912812914,30.5829390177582,
-40.8924276633141));
#254761=CARTESIAN_POINT('Ctrl Pts',(-44.7200063674423,30.5585634922437,
-40.8649689008411));
#254762=CARTESIAN_POINT('Ctrl Pts',(-44.6961476159991,30.5433500948652,
-40.8467099213417));
#254763=CARTESIAN_POINT('Ctrl Pts',(-44.6779108400504,30.5323301088838,
-40.8330260113948));
#254764=CARTESIAN_POINT('Ctrl Pts',(-44.6717725199842,30.5287210947847,
-40.8284650265932));
#254765=CARTESIAN_POINT('Ctrl Pts',(-44.6594468286685,30.521672327511,-40.8193954109541));
#254766=CARTESIAN_POINT('Ctrl Pts',(-44.6532495459125,30.5182260348866,
-40.8148790968875));
#254767=CARTESIAN_POINT('Ctrl Pts',(-44.6221170703041,30.5014023919654,
-40.7924104777995));
#254768=CARTESIAN_POINT('Ctrl Pts',(-44.5712944462502,30.4770113822335,
-40.7571098106096));
#254769=CARTESIAN_POINT('Ctrl Pts',(-44.5053084694641,30.4527583886953,
-40.7146170218743));
#254770=CARTESIAN_POINT('Ctrl Pts',(-44.4645950315289,30.4410392847555,
-40.6898685245315));
#254771=CARTESIAN_POINT('Ctrl Pts',(-44.4371992237873,30.4338676574989,
-40.6735398509862));
#254772=CARTESIAN_POINT('Ctrl Pts',(-44.4233828828253,30.4306039319716,
-40.6654653393082));
#254773=CARTESIAN_POINT('Ctrl Pts',(-44.395457566773,30.4247250011004,-40.6494724436125));
#254774=CARTESIAN_POINT('Ctrl Pts',(-44.3814368244576,30.4221299378924,
-40.6416053105951));
#254775=CARTESIAN_POINT('Ctrl Pts',(-44.353398925472,30.4176419772095,-40.6261940087904));
#254776=CARTESIAN_POINT('Ctrl Pts',(-44.3393578467875,30.4157440298243,
-40.6186361329255));
#254777=CARTESIAN_POINT('Ctrl Pts',(-44.2971907773647,30.4110825461462,
-40.5964157409664));
#254778=CARTESIAN_POINT('Ctrl Pts',(-44.2690063197214,30.4093460565949,
-40.5821970282665));
#254779=CARTESIAN_POINT('Ctrl Pts',(-44.212497942469,30.4086221665927,-40.5549656043439));
#254780=CARTESIAN_POINT('Ctrl Pts',(-44.1841675064314,30.4096363406377,
-40.5419505068598));
#254781=CARTESIAN_POINT('Ctrl Pts',(-44.1486758957365,30.4126704859088,
-40.5264682752254));
#254782=CARTESIAN_POINT('Ctrl Pts',(-44.141568690144,30.4133673915631,-40.5234096239519));
#254783=CARTESIAN_POINT('Ctrl Pts',(-44.1273541295014,30.414939058346,-40.5173753852017));
#254784=CARTESIAN_POINT('Ctrl Pts',(-44.1202325648852,30.4158161528369,
-40.5143941227858));
#254785=CARTESIAN_POINT('Ctrl Pts',(-44.0989269046614,30.418710900521,-40.5056018445424));
#254786=CARTESIAN_POINT('Ctrl Pts',(-44.0848361489451,30.4209852789275,
-40.4999555272545));
#254787=CARTESIAN_POINT('Ctrl Pts',(-44.0428355440345,30.4288357011986,
-40.4836289969086));
#254788=CARTESIAN_POINT('Ctrl Pts',(-44.001418907738,30.4387301387603,-40.4685417636913));
#254789=CARTESIAN_POINT('Ctrl Pts',(-43.9473552852602,30.4559806561897,
-40.4508995609031));
#254790=CARTESIAN_POINT('Ctrl Pts',(-43.9073915907435,30.4709642266074,
-40.4389183731711));
#254791=CARTESIAN_POINT('Ctrl Pts',(-43.8811432548962,30.4823370897352,
-40.4317784203789));
#254792=CARTESIAN_POINT('Ctrl Pts',(-43.8550972458946,30.4944149327137,
-40.4250719137776));
#254793=CARTESIAN_POINT('Ctrl Pts',(-43.8421555815742,30.5008203273088,
-40.4219325711588));
#254794=CARTESIAN_POINT('Ctrl Pts',(-43.8167947927211,30.5141840584711,
-40.4161689437405));
#254795=CARTESIAN_POINT('Ctrl Pts',(-43.8043130802594,30.5211703528968,
-40.413528034466));
#254796=CARTESIAN_POINT('Ctrl Pts',(-43.7797793173031,30.5357258010655,
-40.4087317905317));
#254797=CARTESIAN_POINT('Ctrl Pts',(-43.7436043213473,30.5584424906522,
-40.4022611528103));
#254798=CARTESIAN_POINT('Ctrl Pts',(-43.7092889915882,30.583786036936,-40.397944872434));
#254799=CARTESIAN_POINT('Ctrl Pts',(-43.6651994519323,30.6199287507259,
-40.394121352571));
#254800=CARTESIAN_POINT('Ctrl Pts',(-43.6439827068456,30.6391798378995,
-40.3931753351425));
#254801=CARTESIAN_POINT('Ctrl Pts',(-43.6032932824946,30.680108587057,-40.3932905044721));
#254802=CARTESIAN_POINT('Ctrl Pts',(-43.5841829799745,30.7014201645355,
-40.3943499059801));
#254803=CARTESIAN_POINT('Ctrl Pts',(-43.5483166082379,30.7456951818503,
-40.3983955355947));
#254804=CARTESIAN_POINT('Ctrl Pts',(-43.5148120542517,30.7916143604394,
-40.4043679292189));
#254805=CARTESIAN_POINT('Ctrl Pts',(-43.4859931451963,30.8408014772341,
-40.4141590917094));
#254806=CARTESIAN_POINT('Ctrl Pts',(-43.469474574758,30.8725808034089,-40.4214902069511));
#254807=CARTESIAN_POINT('Ctrl Pts',(-43.4662461658165,30.8789901287051,
-40.4230180755467));
#254808=CARTESIAN_POINT('Ctrl Pts',(-43.4599404108544,30.8919125782622,
-40.4261957226772));
#254809=CARTESIAN_POINT('Ctrl Pts',(-43.4568618652692,30.8984301381776,
-40.4278470523708));
#254810=CARTESIAN_POINT('Ctrl Pts',(-43.4479066843131,30.9180293597941,
-40.4329571814025));
#254811=CARTESIAN_POINT('Ctrl Pts',(-43.4366800830858,30.9443463169446,
-40.440199707327));
#254812=CARTESIAN_POINT('Ctrl Pts',(-43.4219268251392,30.9843790154574,
-40.4523233881121));
#254813=CARTESIAN_POINT('Ctrl Pts',(-43.4092278315493,31.0249558361973,
-40.4656821965631));
#254814=CARTESIAN_POINT('Ctrl Pts',(-43.3985649158327,31.0660734353404,
-40.4802626336878));
#254815=CARTESIAN_POINT('Ctrl Pts',(-43.3928117504253,31.0938450909326,
-40.4907938342908));
#254816=CARTESIAN_POINT('Ctrl Pts',(-43.3877402558097,31.1217978520093,
-40.5017316825792));
#254817=CARTESIAN_POINT('Ctrl Pts',(-43.3855448869231,31.1358715333473,
-40.5074069308404));
#254818=CARTESIAN_POINT('Ctrl Pts',(-43.3818466485176,31.1641754295066,
-40.5191561881817));
#254819=CARTESIAN_POINT('Ctrl Pts',(-43.3803394900793,31.1784722137567,
-40.5252598906186));
#254820=CARTESIAN_POINT('Ctrl Pts',(-43.3780514709974,31.2069533499868,
-40.5377524690855));
#254821=CARTESIAN_POINT('Ctrl Pts',(-43.3764764291988,31.2353806198054,
-40.5505518795279));
#254822=CARTESIAN_POINT('Ctrl Pts',(-43.3761228002374,31.292003207243,-40.577339198747));
#254823=CARTESIAN_POINT('Ctrl Pts',(-43.3798904844517,31.3482922086547,
-40.6058744004623));
#254824=CARTESIAN_POINT('Ctrl Pts',(-43.3877424304871,31.4042485256067,
-40.6361260433691));
#254825=CARTESIAN_POINT('Ctrl Pts',(-43.393042276717,31.4321193306868,-40.6518290622461));
#254826=CARTESIAN_POINT('Ctrl Pts',(-43.3990345440792,31.4599262492628,
-40.6678171709904));
#254827=CARTESIAN_POINT('Ctrl Pts',(-43.4023871385948,31.4738288295879,
-40.6759732487162));
#254828=CARTESIAN_POINT('Ctrl Pts',(-43.4097262599636,31.5013102698765,
-40.6924188649606));
#254829=CARTESIAN_POINT('Ctrl Pts',(-43.4137223958007,31.5149386860624,
-40.7007364096885));
#254830=CARTESIAN_POINT('Ctrl Pts',(-43.4266697743275,31.5554481319482,
-40.7259437634106));
#254831=CARTESIAN_POINT('Ctrl Pts',(-43.4365815013438,31.5819735775504,
-40.743098588818));
#254832=CARTESIAN_POINT('Ctrl Pts',(-43.453362100664,31.6210434116697,-40.7693485791028));
#254833=CARTESIAN_POINT('Ctrl Pts',(-43.4592720436944,31.6339404199602,
-40.77818065559));
#254834=CARTESIAN_POINT('Ctrl Pts',(-43.471748387858,31.6595177912398,-40.7960360397975));
#254835=CARTESIAN_POINT('Ctrl Pts',(-43.4782913690647,31.6721475181291,
-40.8050245716083));
#254836=CARTESIAN_POINT('Ctrl Pts',(-43.4987158872668,31.7093568101663,
-40.832021101787));
#254837=CARTESIAN_POINT('Ctrl Pts',(-43.5134312848982,31.7333600460206,
-40.8501267844669));
#254838=CARTESIAN_POINT('Ctrl Pts',(-43.5449969636312,31.7797747067972,
-40.8865288544817));
#254839=CARTESIAN_POINT('Ctrl Pts',(-43.570273480101,31.8133992725601,-40.9139774903764));
#254840=CARTESIAN_POINT('Ctrl Pts',(-43.6071874842548,31.8558549470217,
-40.9508682927202));
#254841=CARTESIAN_POINT('Ctrl Pts',(-43.6267265436653,31.8762775041081,
-40.9694100075909));
#254842=CARTESIAN_POINT('Ctrl Pts',(-43.6468212761471,31.8962967826001,
-40.9880061403947));
#254843=CARTESIAN_POINT('Ctrl Pts',(-43.6571524242715,31.9061057307006,
-40.997334528722));
#254844=CARTESIAN_POINT('Ctrl Pts',(-43.6781351765956,31.9250932263188,
-41.0158316653051));
#254845=CARTESIAN_POINT('Ctrl Pts',(-43.6888325213991,31.9343181422645,
-41.0250431278314));
#254846=CARTESIAN_POINT('Ctrl Pts',(-43.7214683281725,31.961133026229,-41.0525078158304));
#254847=CARTESIAN_POINT('Ctrl Pts',(-43.744000771517,31.977916302359,-41.070639272709));
#254848=CARTESIAN_POINT('Ctrl Pts',(-43.7905699795511,32.0092811177654,
-41.106520902203));
#254849=CARTESIAN_POINT('Ctrl Pts',(-43.8266341229871,32.0311632771839,
-41.1331548827895));
#254850=CARTESIAN_POINT('Ctrl Pts',(-43.8644344365312,32.050527928199,-41.1593656410909));
#254851=CARTESIAN_POINT('Ctrl Pts',(-43.8900335656271,32.0628690313763,
-41.1767476889401));
#254852=CARTESIAN_POINT('Ctrl Pts',(-43.903042008964,32.0687560539784,-41.1853974312384));
#254853=CARTESIAN_POINT('Ctrl Pts',(-43.9291618902095,32.0798229381751,
-41.2024070088898));
#254854=CARTESIAN_POINT('Ctrl Pts',(-43.9423286751247,32.0850301956599,
-41.2108047653586));
#254855=CARTESIAN_POINT('Ctrl Pts',(-43.9688389276373,32.0947834481969,
-41.2273662374836));
#254856=CARTESIAN_POINT('Ctrl Pts',(-44.0088868242005,32.1084293286422,
-41.2518690158044));
#254857=CARTESIAN_POINT('Ctrl Pts',(-44.0634057706764,32.1227159830699,
-41.2831968728749));
#254858=CARTESIAN_POINT('Ctrl Pts',(-44.1051448739617,32.1304686073096,
-41.30568419746));
#254859=CARTESIAN_POINT('Ctrl Pts',(-44.1331632182567,32.1349666221674,
-41.3204486001008));
#254860=CARTESIAN_POINT('Ctrl Pts',(-44.1472622735965,32.1368798783668,
-41.3277141420552));
#254861=CARTESIAN_POINT('Ctrl Pts',(-44.1685768983456,32.1392377391899,
-41.3384485067576));
#254862=CARTESIAN_POINT('Ctrl Pts',(-44.1757038998442,32.1399371964,-41.3419962566417));
#254863=CARTESIAN_POINT('Ctrl Pts',(-44.1899298892594,32.1411565650423,
-41.3489954369734));
#254864=CARTESIAN_POINT('Ctrl Pts',(-44.1970429564213,32.1416781032566,
-41.3524539903966));
#254865=CARTESIAN_POINT('Ctrl Pts',(-44.2183581262916,32.1429776302475,
-41.3626954949199));
#254866=CARTESIAN_POINT('Ctrl Pts',(-44.232556678806,32.1434929542666,-41.3693546778539));
#254867=CARTESIAN_POINT('Ctrl Pts',(-44.2750884056492,32.1439936324359,
-41.3888189062651));
#254868=CARTESIAN_POINT('Ctrl Pts',(-44.3033804172497,32.1429384256622,
-41.4011231160504));
#254869=CARTESIAN_POINT('Ctrl Pts',(-44.3598247343314,32.13804594572,-41.4243882373187));
#254870=CARTESIAN_POINT('Ctrl Pts',(-44.3879848006206,32.1342064546963,
-41.4353516241949));
#254871=CARTESIAN_POINT('Ctrl Pts',(-44.4230841862873,32.1276226980045,
-41.4481948195873));
#254872=CARTESIAN_POINT('Ctrl Pts',(-44.4301039616143,32.126214419323,-41.4507215814638));
#254873=CARTESIAN_POINT('Ctrl Pts',(-44.4441256434231,32.1232190082407,
-41.455685422358));
#254874=CARTESIAN_POINT('Ctrl Pts',(-44.4511413829898,32.1216281453652,
-41.4581270453932));
#254875=CARTESIAN_POINT('Ctrl Pts',(-44.472106554004,32.1165956901708,-41.4652964871519));
#254876=CARTESIAN_POINT('Ctrl Pts',(-44.4859328208737,32.1129061786889,
-41.4698557698741));
#254877=CARTESIAN_POINT('Ctrl Pts',(-44.5270324780087,32.1008340938932,
-41.4829067838587));
#254878=CARTESIAN_POINT('Ctrl Pts',(-44.5673316800757,32.08677017453,-41.4946921125766));
#254879=CARTESIAN_POINT('Ctrl Pts',(-44.6194780799712,32.0640738471498,
-41.5079096337926));
#254880=CARTESIAN_POINT('Ctrl Pts',(-44.6577884739158,32.045065905176,-41.5165678887371));
#254881=CARTESIAN_POINT('Ctrl Pts',(-44.6827916371924,32.031050813041,-41.5214942665077));
#254882=CARTESIAN_POINT('Ctrl Pts',(-44.7075150580676,32.0163554529027,
-41.5259894017533));
#254883=CARTESIAN_POINT('Ctrl Pts',(-44.7197631353705,32.0086467826241,
-41.5280237577537));
#254884=CARTESIAN_POINT('Ctrl Pts',(-44.7436779765282,31.9927322821733,
-41.5316086326721));
#254885=CARTESIAN_POINT('Ctrl Pts',(-44.7554039451266,31.9844926239501,
-41.5331705278033));
#254886=CARTESIAN_POINT('Ctrl Pts',(-44.7783650010144,31.9674779303508,
-41.5358342782831));
#254887=CARTESIAN_POINT('Ctrl Pts',(-44.8120876763637,31.941142023486,-41.5391427937509));
#254888=CARTESIAN_POINT('Ctrl Pts',(-44.8542060542843,31.9028069711657,
-41.5408368316843));
#254889=CARTESIAN_POINT('Ctrl Pts',(-44.883650374082,31.8716290815775,-41.5400605624154));
#254890=CARTESIAN_POINT('Ctrl Pts',(-44.9027957424029,31.8502960261458,
-41.5390808606534));
#254891=CARTESIAN_POINT('Ctrl Pts',(-44.912124025092,31.8393588588263,-41.5383603441012));
#254892=CARTESIAN_POINT('Ctrl Pts',(-44.9302963003321,31.816913187918,-41.5364463589967));
#254893=CARTESIAN_POINT('Ctrl Pts',(-44.9390653236876,31.8054960967264,
-41.5352602514373));
#254894=CARTESIAN_POINT('Ctrl Pts',(-44.9559494861592,31.7823260274566,
-41.532444286592));
#254895=CARTESIAN_POINT('Ctrl Pts',(-44.9803129684955,31.7470436123751,
-41.5275522735743));
#254896=CARTESIAN_POINT('Ctrl Pts',(-45.00183725318,31.7102129370948,-41.5206914933375));
#254897=CARTESIAN_POINT('Ctrl Pts',(-45.0280427451288,31.6597446570548,
-41.5098099510806));
#254898=CARTESIAN_POINT('Ctrl Pts',(-45.0398987329805,31.6338241168053,
-41.5034995556801));
#254899=CARTESIAN_POINT('Ctrl Pts',(-45.0531290598229,31.6005723463994,
-41.4945098705711));
#254900=CARTESIAN_POINT('Ctrl Pts',(-45.0556963147994,31.5938738844661,
-41.4926546478805));
#254901=CARTESIAN_POINT('Ctrl Pts',(-45.0606676096559,31.5803990532317,
-41.4888352403062));
#254902=CARTESIAN_POINT('Ctrl Pts',(-45.0630762139805,31.5736079348959,
-41.4868664774371));
#254903=CARTESIAN_POINT('Ctrl Pts',(-45.0700329505347,31.5531765604049,
-41.4808121016924));
#254904=CARTESIAN_POINT('Ctrl Pts',(-45.0743018132827,31.5395152309552,
-41.4765904297482));
#254905=CARTESIAN_POINT('Ctrl Pts',(-45.0860497029301,31.4983488303989,
-41.4633620161014));
#254906=CARTESIAN_POINT('Ctrl Pts',(-45.0988767040151,31.4430340104486,
-41.4442426901641));
#254907=CARTESIAN_POINT('Ctrl Pts',(-45.1061818129997,31.386882792419,-41.4222207481485));
#254908=CARTESIAN_POINT('Ctrl Pts',(-45.1095857869151,31.3444641027996,
-41.4046111316328));
#254909=CARTESIAN_POINT('Ctrl Pts',(-45.1103739871937,31.3302675876129,
-41.3985560195248));
#254910=CARTESIAN_POINT('Ctrl Pts',(-45.1110306052012,31.30890259785,-41.3891987399731));
#254911=CARTESIAN_POINT('Ctrl Pts',(-45.1111617199316,31.3017636946428,
-41.3860313075819));
#254912=CARTESIAN_POINT('Ctrl Pts',(-45.1112472734604,31.2874686716035,
-41.3796068875509));
#254913=CARTESIAN_POINT('Ctrl Pts',(-45.111201351958,31.2802974166487,-41.3763428889219));
#254914=CARTESIAN_POINT('Ctrl Pts',(-45.1107973541963,31.25882908612,-41.3664479958234));
#254915=CARTESIAN_POINT('Ctrl Pts',(-45.11017580813,31.2446005169708,-41.3597259135069));
#254916=CARTESIAN_POINT('Ctrl Pts',(-45.1082442962718,31.2162677536902,
-41.3460176286356));
#254917=CARTESIAN_POINT('Ctrl Pts',(-45.104314463686,31.1739750543259,-41.3250680443717));
#254918=CARTESIAN_POINT('Ctrl Pts',(-45.0950241996196,31.1183949914011,
-41.295609869938));
#254919=CARTESIAN_POINT('Ctrl Pts',(-45.0817381040079,31.0636149263882,
-41.264634106957));
#254920=CARTESIAN_POINT('Ctrl Pts',(-45.0737554763462,31.0364928582332,
-41.2486352837062));
#254921=CARTESIAN_POINT('Ctrl Pts',(-45.0650963255467,31.0095068957897,
-41.2323777508457));
#254922=CARTESIAN_POINT('Ctrl Pts',(-45.0604265398991,30.996076905732,-41.224116427314));
#254923=CARTESIAN_POINT('Ctrl Pts',(-45.0504049610752,30.9693743366894,
-41.2073411015006));
#254924=CARTESIAN_POINT('Ctrl Pts',(-45.0450945767524,30.9562107421528,
-41.1988958018751));
#254925=CARTESIAN_POINT('Ctrl Pts',(-45.0394875320819,30.9432190801919,
-41.190386719266));
#254926=CARTESIAN_POINT('Ctrl Pts',(-45.3466072487201,32.9831474726814,
-40.3575667765884));
#254927=CARTESIAN_POINT('Ctrl Pts',(-45.4775804476444,32.9506416230843,
-40.3279308140717));
#254928=CARTESIAN_POINT('Ctrl Pts',(-45.6018489459591,32.8970303670972,
-40.3018706355002));
#254929=CARTESIAN_POINT('Ctrl Pts',(-45.7930510520033,32.7694772175728,
-40.2654024161569));
#254930=CARTESIAN_POINT('Ctrl Pts',(-45.8648371032935,32.7073974754499,
-40.2528314281289));
#254931=CARTESIAN_POINT('Ctrl Pts',(-45.9708819323183,32.5885937141489,
-40.236033098347));
#254932=CARTESIAN_POINT('Ctrl Pts',(-46.0094601394925,32.5369923640417,
-40.2304669096557));
#254933=CARTESIAN_POINT('Ctrl Pts',(-46.0443914997218,32.4808275965294,
-40.2259504969968));
#254934=CARTESIAN_POINT('Ctrl Pts',(-46.0453687463461,32.4792476132019,
-40.2258246312621));
#254935=CARTESIAN_POINT('Ctrl Pts',(-46.0482994498696,32.4744830235869,
-40.2254486323447));
#254936=CARTESIAN_POINT('Ctrl Pts',(-46.0502410390434,32.4712910039402,
-40.2252015084794));
#254937=CARTESIAN_POINT('Ctrl Pts',(-46.0560808750791,32.4615817586325,
-40.22446420935));
#254938=CARTESIAN_POINT('Ctrl Pts',(-46.0599292529414,32.455034611037,-40.2239865664018));
#254939=CARTESIAN_POINT('Ctrl Pts',(-46.0675639706264,32.4417408317884,
-40.2230555504732));
#254940=CARTESIAN_POINT('Ctrl Pts',(-46.0713470910329,32.4349941460753,
-40.222602877568));
#254941=CARTESIAN_POINT('Ctrl Pts',(-46.110523107097,32.3634224247021,-40.218006074707));
#254942=CARTESIAN_POINT('Ctrl Pts',(-46.1395815298695,32.2953942994941,
-40.2153865540286));
#254943=CARTESIAN_POINT('Ctrl Pts',(-46.2069461227329,32.0848150750412,
-40.2116780528921));
#254944=CARTESIAN_POINT('Ctrl Pts',(-46.2252178127257,31.9383772329122,
-40.2146552898855));
#254945=CARTESIAN_POINT('Ctrl Pts',(-46.2146419207919,31.6745946451145,
-40.2265788965334));
#254946=CARTESIAN_POINT('Ctrl Pts',(-46.1952499881773,31.576162819291,-40.2334689298899));
#254947=CARTESIAN_POINT('Ctrl Pts',(-46.1762418209585,31.5014470256211,
-40.2388224305403));
#254948=CARTESIAN_POINT('Ctrl Pts',(-46.6981266849492,30.7091523375488,
-39.2904704603133));
#254949=CARTESIAN_POINT('Ctrl Pts',(-46.6689684123063,30.6404043382273,
-39.273452295095));
#254950=CARTESIAN_POINT('Ctrl Pts',(-46.6043681216411,30.5066861069553,
-39.238925705885));
#254951=CARTESIAN_POINT('Ctrl Pts',(-46.5083209189471,30.3487389562033,
-39.1945593129175));
#254952=CARTESIAN_POINT('Ctrl Pts',(-46.4437937583117,30.2581216171786,
-39.1673894861782));
#254953=CARTESIAN_POINT('Ctrl Pts',(-46.3992224148768,30.1986447451181,
-39.1491520227249));
#254954=CARTESIAN_POINT('Ctrl Pts',(-46.3761748773305,30.1693908446446,
-39.1399767764946));
#254955=CARTESIAN_POINT('Ctrl Pts',(-46.3284414024809,30.1117648114071,
-39.1214771434543));
#254956=CARTESIAN_POINT('Ctrl Pts',(-46.3038983378397,30.083571828401,-39.112209259666));
#254957=CARTESIAN_POINT('Ctrl Pts',(-46.253707387608,30.0286632749651,-39.0937226519629));
#254958=CARTESIAN_POINT('Ctrl Pts',(-46.2280147026909,30.001893564456,-39.0844865568113));
#254959=CARTESIAN_POINT('Ctrl Pts',(-46.1492148010453,29.9236586721517,
-39.0568159196779));
#254960=CARTESIAN_POINT('Ctrl Pts',(-46.0669347173688,29.8495134741745,
-39.0292038481275));
#254961=CARTESIAN_POINT('Ctrl Pts',(-45.9503410384262,29.7587889734315,
-38.9925114043613));
#254962=CARTESIAN_POINT('Ctrl Pts',(-45.8594191065401,29.6948377475824,
-38.9650526418885));
#254963=CARTESIAN_POINT('Ctrl Pts',(-45.7964751089327,29.6549785818455,
-38.9467936623891));
#254964=CARTESIAN_POINT('Ctrl Pts',(-45.748348603817,29.6261284949947,-38.9331097524421));
#254965=CARTESIAN_POINT('Ctrl Pts',(-45.7321473284057,29.616684052073,-38.9285487676403));
#254966=CARTESIAN_POINT('Ctrl Pts',(-45.6996106203311,29.5982459977232,
-38.9194791520014));
#254967=CARTESIAN_POINT('Ctrl Pts',(-45.683249044345,29.5892352448745,-38.9149628379356));
#254968=CARTESIAN_POINT('Ctrl Pts',(-45.6010439155842,29.5452684013657,
-38.8924942188443));
#254969=CARTESIAN_POINT('Ctrl Pts',(-45.4667739830181,29.4816584171599,
-38.8571935516581));
#254970=CARTESIAN_POINT('Ctrl Pts',(-45.2922645146651,29.4187721922835,
-38.8147007629208));
#254971=CARTESIAN_POINT('Ctrl Pts',(-45.184512437616,29.3885937253944,-38.7899522655792));
#254972=CARTESIAN_POINT('Ctrl Pts',(-45.1119891467798,29.3701842541612,
-38.7736235920333));
#254973=CARTESIAN_POINT('Ctrl Pts',(-45.0754052578815,29.3618381514785,
-38.7655490803555));
#254974=CARTESIAN_POINT('Ctrl Pts',(-45.0014447932705,29.3468760834356,
-38.7495561846596));
#254975=CARTESIAN_POINT('Ctrl Pts',(-44.964301863367,29.3403115562353,-38.7416890516424));
#254976=CARTESIAN_POINT('Ctrl Pts',(-44.8900079594565,29.3290481892184,
-38.726277749838));
#254977=CARTESIAN_POINT('Ctrl Pts',(-44.8527936282157,29.324336495618,-38.7187198739728));
#254978=CARTESIAN_POINT('Ctrl Pts',(-44.7410083373266,29.3129455735289,
-38.6964994820139));
#254979=CARTESIAN_POINT('Ctrl Pts',(-44.6662563757167,29.3089967422249,
-38.6822807693139));
#254980=CARTESIAN_POINT('Ctrl Pts',(-44.516312468428,29.3084067934202,-38.6550493453909));
#254981=CARTESIAN_POINT('Ctrl Pts',(-44.441103189525,29.3117700143417,-38.6420342479066));
#254982=CARTESIAN_POINT('Ctrl Pts',(-44.3468378615956,29.3206690055189,
-38.6265520162729));
#254983=CARTESIAN_POINT('Ctrl Pts',(-44.3279589148655,29.3226883315868,
-38.6234933649988));
#254984=CARTESIAN_POINT('Ctrl Pts',(-44.2901960653062,29.3271995080042,
-38.6174591262491));
#254985=CARTESIAN_POINT('Ctrl Pts',(-44.271274393292,29.329697893027,-38.614477863833));
#254986=CARTESIAN_POINT('Ctrl Pts',(-44.2146592782019,29.3378915995821,
-38.60568558559));
#254987=CARTESIAN_POINT('Ctrl Pts',(-44.1772069502033,29.344266758826,-38.6000392683017));
#254988=CARTESIAN_POINT('Ctrl Pts',(-44.0655444875092,29.3661148598052,
-38.5837127379559));
#254989=CARTESIAN_POINT('Ctrl Pts',(-43.9553791862171,29.3933792052515,
-38.5686255047386));
#254990=CARTESIAN_POINT('Ctrl Pts',(-43.8114622524781,29.4404829778103,
-38.5509833019505));
#254991=CARTESIAN_POINT('Ctrl Pts',(-43.705021834675,29.481230340464,-38.5390021142185));
#254992=CARTESIAN_POINT('Ctrl Pts',(-43.6350719757086,29.512061063653,-38.5318621614261));
#254993=CARTESIAN_POINT('Ctrl Pts',(-43.5656410085295,29.5447591316771,
-38.525155654825));
#254994=CARTESIAN_POINT('Ctrl Pts',(-43.5311320054746,29.5620794464364,
-38.5220163122062));
#254995=CARTESIAN_POINT('Ctrl Pts',(-43.4634866412134,29.5981758355574,
-38.5162526847879));
#254996=CARTESIAN_POINT('Ctrl Pts',(-43.4301834663392,29.6170276546,-38.5136117755133));
#254997=CARTESIAN_POINT('Ctrl Pts',(-43.3647025891651,29.6562685687332,
-38.5088155315793));
#254998=CARTESIAN_POINT('Ctrl Pts',(-43.2681192378476,29.7174608121974,
-38.5023448938576));
#254999=CARTESIAN_POINT('Ctrl Pts',(-43.1764049274077,29.7855824582168,
-38.4980286134812));
#255000=CARTESIAN_POINT('Ctrl Pts',(-43.0584774180437,29.8826126224142,
-38.4942050936184));
#255001=CARTESIAN_POINT('Ctrl Pts',(-43.001681818637,29.9342392650769,-38.4932590761897));
#255002=CARTESIAN_POINT('Ctrl Pts',(-42.8926599718677,30.0438904492243,
-38.4933742455196));
#255003=CARTESIAN_POINT('Ctrl Pts',(-42.8414047150844,30.1009342501745,
-38.4944336470273));
#255004=CARTESIAN_POINT('Ctrl Pts',(-42.7451036203247,30.2193471227021,
-38.498479276642));
#255005=CARTESIAN_POINT('Ctrl Pts',(-42.6550322643363,30.3420646399833,
-38.5044516702661));
#255006=CARTESIAN_POINT('Ctrl Pts',(-42.5773225406025,30.4733365238586,
-38.5142428327574));
#255007=CARTESIAN_POINT('Ctrl Pts',(-42.5326943378214,30.5580963840027,
-38.5215739479982));
#255008=CARTESIAN_POINT('Ctrl Pts',(-42.5239673850246,30.5751883092729,
-38.5231018165939));
#255009=CARTESIAN_POINT('Ctrl Pts',(-42.5069121510755,30.60964376351,-38.5262794637242));
#255010=CARTESIAN_POINT('Ctrl Pts',(-42.4985805781952,30.627019094627,-38.5279307934181));
#255011=CARTESIAN_POINT('Ctrl Pts',(-42.4743295471271,30.6792614198295,
-38.5330409224498));
#255012=CARTESIAN_POINT('Ctrl Pts',(-42.4438856226513,30.7493896366731,
-38.5402834483744));
#255013=CARTESIAN_POINT('Ctrl Pts',(-42.4037483179465,30.8560072598611,
-38.5524071291592));
#255014=CARTESIAN_POINT('Ctrl Pts',(-42.3690543371876,30.9640160484273,
-38.5657659376104));
#255015=CARTESIAN_POINT('Ctrl Pts',(-42.3397558527982,31.0734075527136,
-38.5803463747351));
#255016=CARTESIAN_POINT('Ctrl Pts',(-42.3238156343608,31.1472555030051,
-38.5908775753381));
#255017=CARTESIAN_POINT('Ctrl Pts',(-42.3096820427396,31.2215665449467,
-38.6018154236264));
#255018=CARTESIAN_POINT('Ctrl Pts',(-42.3035171869091,31.2589715314082,
-38.6074906718877));
#255019=CARTESIAN_POINT('Ctrl Pts',(-42.2930235524414,31.3341791410138,
-38.6192399292287));
#255020=CARTESIAN_POINT('Ctrl Pts',(-42.2886818075092,31.3721585359098,
-38.6253436316658));
#255021=CARTESIAN_POINT('Ctrl Pts',(-42.281930630611,31.4478003630713,-38.6378362101326));
#255022=CARTESIAN_POINT('Ctrl Pts',(-42.277074994566,31.5232809912004,-38.6506356205751));
#255023=CARTESIAN_POINT('Ctrl Pts',(-42.2747992363309,31.6735553614761,
-38.6774229397946));
#255024=CARTESIAN_POINT('Ctrl Pts',(-42.2834818483937,31.8228397562226,
-38.7059581415094));
#255025=CARTESIAN_POINT('Ctrl Pts',(-42.3030248127084,31.9711385758679,
-38.7362097844166));
#255026=CARTESIAN_POINT('Ctrl Pts',(-42.3164494406915,32.0449687602614,
-38.7519128032936));
#255027=CARTESIAN_POINT('Ctrl Pts',(-42.3317154579634,32.1186122141692,
-38.7679009120377));
#255028=CARTESIAN_POINT('Ctrl Pts',(-42.3402956643805,32.1554227583218,
-38.7760569897633));
#255029=CARTESIAN_POINT('Ctrl Pts',(-42.3591481714288,32.228169160774,-38.7925026060078));
#255030=CARTESIAN_POINT('Ctrl Pts',(-42.3694448348212,32.2642362896146,
-38.8008201507359));
#255031=CARTESIAN_POINT('Ctrl Pts',(-42.4028917825415,32.3714169561226,
-38.8260275044574));
#255032=CARTESIAN_POINT('Ctrl Pts',(-42.428602574983,32.4415633880281,-38.8431823298655));
#255033=CARTESIAN_POINT('Ctrl Pts',(-42.4722685042023,32.5448307979217,
-38.8694323201497));
#255034=CARTESIAN_POINT('Ctrl Pts',(-42.4876674804306,32.5789105800712,
-38.8782643966373));
#255035=CARTESIAN_POINT('Ctrl Pts',(-42.5202146590728,32.6464795812123,
-38.8961197808447));
#255036=CARTESIAN_POINT('Ctrl Pts',(-42.5373018269229,32.6798350022668,
-38.9051083126545));
#255037=CARTESIAN_POINT('Ctrl Pts',(-42.5906929412925,32.7780783962456,
-38.9321048428364));
#255038=CARTESIAN_POINT('Ctrl Pts',(-42.629225789877,32.8414173722334,-38.9502105255135));
#255039=CARTESIAN_POINT('Ctrl Pts',(-42.7120000069194,32.9638220552461,
-38.9866125955294));
#255040=CARTESIAN_POINT('Ctrl Pts',(-42.7783647966162,33.0524402968179,
-39.0140612314234));
#255041=CARTESIAN_POINT('Ctrl Pts',(-42.8754380724448,33.1642175243331,
-39.0509520337677));
#255042=CARTESIAN_POINT('Ctrl Pts',(-42.9268673384212,33.2179450225078,
-39.0694937486382));
#255043=CARTESIAN_POINT('Ctrl Pts',(-42.9797817061918,33.2705900457306,
-39.088089881442));
#255044=CARTESIAN_POINT('Ctrl Pts',(-43.0069972096607,33.2963736994336,
-39.097418269769));
#255045=CARTESIAN_POINT('Ctrl Pts',(-43.0622936398443,33.3462615369726,
-39.1159154063528));
#255046=CARTESIAN_POINT('Ctrl Pts',(-43.0904949946047,33.3704876748183,
-39.1251268688783));
#255047=CARTESIAN_POINT('Ctrl Pts',(-43.176562606447,33.4408730143712,-39.1525915568785));
#255048=CARTESIAN_POINT('Ctrl Pts',(-43.2360245534179,33.4848790444095,
-39.1707230137558));
#255049=CARTESIAN_POINT('Ctrl Pts',(-43.358992255749,33.5670176609587,-39.2066046432507));
#255050=CARTESIAN_POINT('Ctrl Pts',(-43.4542745623933,33.6242424638975,
-39.233238623837));
#255051=CARTESIAN_POINT('Ctrl Pts',(-43.5542222374601,33.6747516510336,
-39.2594493821381));
#255052=CARTESIAN_POINT('Ctrl Pts',(-43.6219256430316,33.7069073870393,
-39.2768314299875));
#255053=CARTESIAN_POINT('Ctrl Pts',(-43.6563381479934,33.7222286468184,
-39.2854811722856));
#255054=CARTESIAN_POINT('Ctrl Pts',(-43.7254519170511,33.7509934760635,
-39.3024907499371));
#255055=CARTESIAN_POINT('Ctrl Pts',(-43.7602995448845,33.7645084608315,
-39.3108885064059));
#255056=CARTESIAN_POINT('Ctrl Pts',(-43.8304781084082,33.789780836939,-39.3274499785309));
#255057=CARTESIAN_POINT('Ctrl Pts',(-43.9365171946568,33.8250735562425,
-39.3519527568515));
#255058=CARTESIAN_POINT('Ctrl Pts',(-44.0809642638621,33.8617420360433,
-39.3832806139221));
#255059=CARTESIAN_POINT('Ctrl Pts',(-44.1916183723467,33.8813683146414,
-39.4057679385072));
#255060=CARTESIAN_POINT('Ctrl Pts',(-44.2659122959159,33.8926702964892,
-39.4205323411483));
#255061=CARTESIAN_POINT('Ctrl Pts',(-44.3033049221432,33.8974288658374,
-39.4277978831022));
#255062=CARTESIAN_POINT('Ctrl Pts',(-44.3598453576919,33.9032050944765,
-39.4385322478049));
#255063=CARTESIAN_POINT('Ctrl Pts',(-44.3787527158677,33.9049006163346,
-39.4420799976889));
#255064=CARTESIAN_POINT('Ctrl Pts',(-44.4164967874688,33.9078161173588,
-39.4490791780208));
#255065=CARTESIAN_POINT('Ctrl Pts',(-44.4353708468856,33.9090400957878,
-39.4525377314439));
#255066=CARTESIAN_POINT('Ctrl Pts',(-44.4919347179527,33.9120095261765,
-39.462779235967));
#255067=CARTESIAN_POINT('Ctrl Pts',(-44.52962054914,33.9130584408517,-39.4694384189012));
#255068=CARTESIAN_POINT('Ctrl Pts',(-44.6425299001817,33.9134342925821,
-39.4889026473125));
#255069=CARTESIAN_POINT('Ctrl Pts',(-44.7176656228988,33.9100023852834,
-39.5012068570978));
#255070=CARTESIAN_POINT('Ctrl Pts',(-44.867623327666,33.8957625538083,-39.524471978366));
#255071=CARTESIAN_POINT('Ctrl Pts',(-44.9424659600731,33.8849485744664,
-39.5354353652432));
#255072=CARTESIAN_POINT('Ctrl Pts',(-45.0357885152669,33.8666999843662,
-39.5482785606344));
#255073=CARTESIAN_POINT('Ctrl Pts',(-45.0544546343785,33.8628074782943,
-39.5508053225112));
#255074=CARTESIAN_POINT('Ctrl Pts',(-45.091743102575,33.8545484160302,-39.5557691634051));
#255075=CARTESIAN_POINT('Ctrl Pts',(-45.1104022544846,33.850171655015,-39.5582107864407));
#255076=CARTESIAN_POINT('Ctrl Pts',(-45.1661672125598,33.8363538303533,
-39.5653802281989));
#255077=CARTESIAN_POINT('Ctrl Pts',(-45.2029511118778,33.8262578362557,
-39.5699395109212));
#255078=CARTESIAN_POINT('Ctrl Pts',(-45.312316831343,33.7933159380614,-39.582990524906));
#255079=CARTESIAN_POINT('Ctrl Pts',(-45.4195983160475,33.7551076509549,
-39.5947758536238));
#255080=CARTESIAN_POINT('Ctrl Pts',(-45.5585113890164,33.6937328563153,
-39.6079933748399));
#255081=CARTESIAN_POINT('Ctrl Pts',(-45.6606150024606,33.6424505696195,
-39.6166516297843));
#255082=CARTESIAN_POINT('Ctrl Pts',(-45.7272860947277,33.6047101271221,
-39.6215780075552));
#255083=CARTESIAN_POINT('Ctrl Pts',(-45.7932287365117,33.5651705839516,
-39.6260731428005));
#255084=CARTESIAN_POINT('Ctrl Pts',(-45.8259059249178,33.5444453395394,
-39.6281074988013));
#255085=CARTESIAN_POINT('Ctrl Pts',(-45.8897275017006,33.5016881508368,
-39.6316923737189));
#255086=CARTESIAN_POINT('Ctrl Pts',(-45.9210297733036,33.4795651380848,
-39.6332542688506));
#255087=CARTESIAN_POINT('Ctrl Pts',(-45.9823424846244,33.4339088874735,
-39.6359180193303));
#255088=CARTESIAN_POINT('Ctrl Pts',(-46.0724202597563,33.3632801300718,
-39.6392265347984));
#255089=CARTESIAN_POINT('Ctrl Pts',(-46.1850394564173,33.2606222983665,
-39.6409205727319));
#255090=CARTESIAN_POINT('Ctrl Pts',(-46.2638636333332,33.1772336958075,
-39.6401443034625));
#255091=CARTESIAN_POINT('Ctrl Pts',(-46.3151397511292,33.1201974856456,
-39.6391646017005));
#255092=CARTESIAN_POINT('Ctrl Pts',(-46.3401349353408,33.0909661742941,
-39.6384440851485));
#255093=CARTESIAN_POINT('Ctrl Pts',(-46.3888523044997,33.0309971480077,
-39.6365301000439));
#255094=CARTESIAN_POINT('Ctrl Pts',(-46.4123735341802,33.0005036828642,
-39.6353439924849));
#255095=CARTESIAN_POINT('Ctrl Pts',(-46.4576879006691,32.9386388625828,
-39.6325280276393));
#255096=CARTESIAN_POINT('Ctrl Pts',(-46.52311576659,32.8444620833496,-39.6276360146217));
#255097=CARTESIAN_POINT('Ctrl Pts',(-46.5810426872604,32.7462345994881,
-39.6207752343847));
#255098=CARTESIAN_POINT('Ctrl Pts',(-46.6516918187307,32.6117039458857,
-39.6098936921283));
#255099=CARTESIAN_POINT('Ctrl Pts',(-46.683723185051,32.5426422373878,-39.6035832967262));
#255100=CARTESIAN_POINT('Ctrl Pts',(-46.7195635412788,32.4540883209461,
-39.5945936116187));
#255101=CARTESIAN_POINT('Ctrl Pts',(-46.7265235775841,32.4362514419463,
-39.5927383889278));
#255102=CARTESIAN_POINT('Ctrl Pts',(-46.7400123459627,32.4003742100513,
-39.5889189813535));
#255103=CARTESIAN_POINT('Ctrl Pts',(-46.7465535157541,32.3822946053341,
-39.5869502184844));
#255104=CARTESIAN_POINT('Ctrl Pts',(-46.7654644360989,32.3279072933142,
-39.5808958427402));
#255105=CARTESIAN_POINT('Ctrl Pts',(-46.7770937339888,32.2915493874551,
-39.5766741707955));
#255106=CARTESIAN_POINT('Ctrl Pts',(-46.8091770518909,32.182013131159,-39.5634457571489));
#255107=CARTESIAN_POINT('Ctrl Pts',(-46.8444383818759,32.034891308334,-39.5443264312115));
#255108=CARTESIAN_POINT('Ctrl Pts',(-46.8650708643864,31.8856621776612,
-39.5223044891954));
#255109=CARTESIAN_POINT('Ctrl Pts',(-46.8750487417844,31.7729724844591,
-39.50469487268));
#255110=CARTESIAN_POINT('Ctrl Pts',(-46.8774570362353,31.7352651712118,
-39.4986397605723));
#255111=CARTESIAN_POINT('Ctrl Pts',(-46.8796767940079,31.6785286095959,
-39.4892824810203));
#255112=CARTESIAN_POINT('Ctrl Pts',(-46.8801843407089,31.6595724593507,
-39.4861150486293));
#255113=CARTESIAN_POINT('Ctrl Pts',(-46.8807312344332,31.6216180949417,
-39.479690628598));
#255114=CARTESIAN_POINT('Ctrl Pts',(-46.8807699646674,31.6025797052015,
-39.4764266299692));
#255115=CARTESIAN_POINT('Ctrl Pts',(-46.8801790388754,31.5455906639181,
-39.4665317368708));
#255116=CARTESIAN_POINT('Ctrl Pts',(-46.8788490796135,31.5078273383739,
-39.4598096545541));
#255117=CARTESIAN_POINT('Ctrl Pts',(-46.874360617844,31.4326451774338,-39.4461013696832));
#255118=CARTESIAN_POINT('Ctrl Pts',(-46.864884835636,31.320441459725,-39.4251517854185));
#255119=CARTESIAN_POINT('Ctrl Pts',(-46.8414902947658,31.1730719473388,
-39.3956936109857));
#255120=CARTESIAN_POINT('Ctrl Pts',(-46.8074810934279,31.0279105813681,
-39.364717848004));
#255121=CARTESIAN_POINT('Ctrl Pts',(-46.7869180083019,30.9560697433081,
-39.3487190247537));
#255122=CARTESIAN_POINT('Ctrl Pts',(-46.7645577771926,30.884604709384,-39.332461491893));
#255123=CARTESIAN_POINT('Ctrl Pts',(-46.7524740339114,30.8490466969583,
-39.3242001683612));
#255124=CARTESIAN_POINT('Ctrl Pts',(-46.7264943673172,30.7783632715819,
-39.3074248425479));
#255125=CARTESIAN_POINT('Ctrl Pts',(-46.7127058212706,30.7435263372096,
-39.2989795429224));
#255126=CARTESIAN_POINT('Ctrl Pts',(-46.6981266849492,30.7091523375488,
-39.2904704603133));
#255127=CARTESIAN_POINT('Ctrl Pts',(-45.0394875320819,30.9432190801919,
-41.190386719266));
#255128=CARTESIAN_POINT('Ctrl Pts',(-45.0282734427409,30.91723575627,-41.1733685540478));
#255129=CARTESIAN_POINT('Ctrl Pts',(-45.0034876660128,30.8666726764904,
-41.1388419648381));
#255130=CARTESIAN_POINT('Ctrl Pts',(-44.9667665375866,30.8068862988478,
-41.09447557187));
#255131=CARTESIAN_POINT('Ctrl Pts',(-44.9421458413835,30.7725558756156,
-41.0673057451311));
#255132=CARTESIAN_POINT('Ctrl Pts',(-44.9251493960809,30.7500159625169,
-41.0490682816776));
#255133=CARTESIAN_POINT('Ctrl Pts',(-44.9163654668634,30.7389260450349,
-41.0398930354472));
#255134=CARTESIAN_POINT('Ctrl Pts',(-44.8981827131164,30.7170729960788,
-41.0213934024069));
#255135=CARTESIAN_POINT('Ctrl Pts',(-44.888838333634,30.7063777841388,-41.0121255186188));
#255136=CARTESIAN_POINT('Ctrl Pts',(-44.8697378119757,30.6855401076749,
-40.9936389109155));
#255137=CARTESIAN_POINT('Ctrl Pts',(-44.8599646045333,30.6753771122426,
-40.984402815764));
#255138=CARTESIAN_POINT('Ctrl Pts',(-44.8300025766326,30.6456635434001,
-40.9567321786306));
#255139=CARTESIAN_POINT('Ctrl Pts',(-44.7987417882795,30.6174785558847,
-40.9291201070801));
#255140=CARTESIAN_POINT('Ctrl Pts',(-44.7544912812914,30.5829390177582,
-40.8924276633141));
#255141=CARTESIAN_POINT('Ctrl Pts',(-44.7200063674423,30.5585634922437,
-40.8649689008411));
#255142=CARTESIAN_POINT('Ctrl Pts',(-44.6961476159991,30.5433500948652,
-40.8467099213417));
#255143=CARTESIAN_POINT('Ctrl Pts',(-44.6779108400504,30.5323301088838,
-40.8330260113948));
#255144=CARTESIAN_POINT('Ctrl Pts',(-44.6717725199842,30.5287210947847,
-40.8284650265932));
#255145=CARTESIAN_POINT('Ctrl Pts',(-44.6594468286685,30.521672327511,-40.8193954109541));
#255146=CARTESIAN_POINT('Ctrl Pts',(-44.6532495459125,30.5182260348866,
-40.8148790968875));
#255147=CARTESIAN_POINT('Ctrl Pts',(-44.6221170703041,30.5014023919654,
-40.7924104777995));
#255148=CARTESIAN_POINT('Ctrl Pts',(-44.5712944462502,30.4770113822335,
-40.7571098106096));
#255149=CARTESIAN_POINT('Ctrl Pts',(-44.5053084694641,30.4527583886953,
-40.7146170218743));
#255150=CARTESIAN_POINT('Ctrl Pts',(-44.4645950315289,30.4410392847555,
-40.6898685245315));
#255151=CARTESIAN_POINT('Ctrl Pts',(-44.4371992237873,30.4338676574989,
-40.6735398509862));
#255152=CARTESIAN_POINT('Ctrl Pts',(-44.4233828828253,30.4306039319716,
-40.6654653393082));
#255153=CARTESIAN_POINT('Ctrl Pts',(-44.395457566773,30.4247250011004,-40.6494724436125));
#255154=CARTESIAN_POINT('Ctrl Pts',(-44.3814368244576,30.4221299378924,
-40.6416053105951));
#255155=CARTESIAN_POINT('Ctrl Pts',(-44.353398925472,30.4176419772095,-40.6261940087904));
#255156=CARTESIAN_POINT('Ctrl Pts',(-44.3393578467875,30.4157440298243,
-40.6186361329255));
#255157=CARTESIAN_POINT('Ctrl Pts',(-44.2971907773647,30.4110825461462,
-40.5964157409664));
#255158=CARTESIAN_POINT('Ctrl Pts',(-44.2690063197214,30.4093460565949,
-40.5821970282665));
#255159=CARTESIAN_POINT('Ctrl Pts',(-44.212497942469,30.4086221665927,-40.5549656043439));
#255160=CARTESIAN_POINT('Ctrl Pts',(-44.1841675064314,30.4096363406377,
-40.5419505068598));
#255161=CARTESIAN_POINT('Ctrl Pts',(-44.1486758957365,30.4126704859088,
-40.5264682752254));
#255162=CARTESIAN_POINT('Ctrl Pts',(-44.141568690144,30.4133673915631,-40.5234096239519));
#255163=CARTESIAN_POINT('Ctrl Pts',(-44.1273541295014,30.414939058346,-40.5173753852017));
#255164=CARTESIAN_POINT('Ctrl Pts',(-44.1202325648852,30.4158161528369,
-40.5143941227858));
#255165=CARTESIAN_POINT('Ctrl Pts',(-44.0989269046614,30.418710900521,-40.5056018445424));
#255166=CARTESIAN_POINT('Ctrl Pts',(-44.0848361489451,30.4209852789275,
-40.4999555272545));
#255167=CARTESIAN_POINT('Ctrl Pts',(-44.0428355440345,30.4288357011986,
-40.4836289969086));
#255168=CARTESIAN_POINT('Ctrl Pts',(-44.001418907738,30.4387301387603,-40.4685417636913));
#255169=CARTESIAN_POINT('Ctrl Pts',(-43.9473552852602,30.4559806561897,
-40.4508995609031));
#255170=CARTESIAN_POINT('Ctrl Pts',(-43.9073915907435,30.4709642266074,
-40.4389183731711));
#255171=CARTESIAN_POINT('Ctrl Pts',(-43.8811432548962,30.4823370897352,
-40.4317784203789));
#255172=CARTESIAN_POINT('Ctrl Pts',(-43.8550972458946,30.4944149327137,
-40.4250719137776));
#255173=CARTESIAN_POINT('Ctrl Pts',(-43.8421555815742,30.5008203273088,
-40.4219325711588));
#255174=CARTESIAN_POINT('Ctrl Pts',(-43.8167947927211,30.5141840584711,
-40.4161689437405));
#255175=CARTESIAN_POINT('Ctrl Pts',(-43.8043130802594,30.5211703528968,
-40.413528034466));
#255176=CARTESIAN_POINT('Ctrl Pts',(-43.7797793173031,30.5357258010655,
-40.4087317905317));
#255177=CARTESIAN_POINT('Ctrl Pts',(-43.7436043213473,30.5584424906522,
-40.4022611528103));
#255178=CARTESIAN_POINT('Ctrl Pts',(-43.7092889915882,30.583786036936,-40.397944872434));
#255179=CARTESIAN_POINT('Ctrl Pts',(-43.6651994519323,30.6199287507259,
-40.394121352571));
#255180=CARTESIAN_POINT('Ctrl Pts',(-43.6439827068456,30.6391798378995,
-40.3931753351425));
#255181=CARTESIAN_POINT('Ctrl Pts',(-43.6032932824946,30.680108587057,-40.3932905044721));
#255182=CARTESIAN_POINT('Ctrl Pts',(-43.5841829799745,30.7014201645355,
-40.3943499059801));
#255183=CARTESIAN_POINT('Ctrl Pts',(-43.5483166082379,30.7456951818503,
-40.3983955355947));
#255184=CARTESIAN_POINT('Ctrl Pts',(-43.5148120542517,30.7916143604394,
-40.4043679292189));
#255185=CARTESIAN_POINT('Ctrl Pts',(-43.4859931451963,30.8408014772341,
-40.4141590917094));
#255186=CARTESIAN_POINT('Ctrl Pts',(-43.469474574758,30.8725808034089,-40.4214902069511));
#255187=CARTESIAN_POINT('Ctrl Pts',(-43.4662461658165,30.8789901287051,
-40.4230180755467));
#255188=CARTESIAN_POINT('Ctrl Pts',(-43.4599404108544,30.8919125782622,
-40.4261957226772));
#255189=CARTESIAN_POINT('Ctrl Pts',(-43.4568618652692,30.8984301381776,
-40.4278470523708));
#255190=CARTESIAN_POINT('Ctrl Pts',(-43.4479066843131,30.9180293597941,
-40.4329571814025));
#255191=CARTESIAN_POINT('Ctrl Pts',(-43.4366800830858,30.9443463169446,
-40.440199707327));
#255192=CARTESIAN_POINT('Ctrl Pts',(-43.4219268251392,30.9843790154574,
-40.4523233881121));
#255193=CARTESIAN_POINT('Ctrl Pts',(-43.4092278315493,31.0249558361973,
-40.4656821965631));
#255194=CARTESIAN_POINT('Ctrl Pts',(-43.3985649158327,31.0660734353404,
-40.4802626336878));
#255195=CARTESIAN_POINT('Ctrl Pts',(-43.3928117504253,31.0938450909326,
-40.4907938342908));
#255196=CARTESIAN_POINT('Ctrl Pts',(-43.3877402558097,31.1217978520093,
-40.5017316825792));
#255197=CARTESIAN_POINT('Ctrl Pts',(-43.3855448869231,31.1358715333473,
-40.5074069308404));
#255198=CARTESIAN_POINT('Ctrl Pts',(-43.3818466485176,31.1641754295066,
-40.5191561881817));
#255199=CARTESIAN_POINT('Ctrl Pts',(-43.3803394900793,31.1784722137567,
-40.5252598906186));
#255200=CARTESIAN_POINT('Ctrl Pts',(-43.3780514709974,31.2069533499868,
-40.5377524690855));
#255201=CARTESIAN_POINT('Ctrl Pts',(-43.3764764291988,31.2353806198054,
-40.5505518795279));
#255202=CARTESIAN_POINT('Ctrl Pts',(-43.3761228002374,31.292003207243,-40.577339198747));
#255203=CARTESIAN_POINT('Ctrl Pts',(-43.3798904844517,31.3482922086547,
-40.6058744004623));
#255204=CARTESIAN_POINT('Ctrl Pts',(-43.3877424304871,31.4042485256067,
-40.6361260433691));
#255205=CARTESIAN_POINT('Ctrl Pts',(-43.393042276717,31.4321193306868,-40.6518290622461));
#255206=CARTESIAN_POINT('Ctrl Pts',(-43.3990345440792,31.4599262492628,
-40.6678171709904));
#255207=CARTESIAN_POINT('Ctrl Pts',(-43.4023871385948,31.4738288295879,
-40.6759732487162));
#255208=CARTESIAN_POINT('Ctrl Pts',(-43.4097262599636,31.5013102698765,
-40.6924188649606));
#255209=CARTESIAN_POINT('Ctrl Pts',(-43.4137223958007,31.5149386860624,
-40.7007364096885));
#255210=CARTESIAN_POINT('Ctrl Pts',(-43.4266697743275,31.5554481319482,
-40.7259437634106));
#255211=CARTESIAN_POINT('Ctrl Pts',(-43.4365815013438,31.5819735775504,
-40.743098588818));
#255212=CARTESIAN_POINT('Ctrl Pts',(-43.453362100664,31.6210434116697,-40.7693485791028));
#255213=CARTESIAN_POINT('Ctrl Pts',(-43.4592720436944,31.6339404199602,
-40.77818065559));
#255214=CARTESIAN_POINT('Ctrl Pts',(-43.471748387858,31.6595177912398,-40.7960360397975));
#255215=CARTESIAN_POINT('Ctrl Pts',(-43.4782913690647,31.6721475181291,
-40.8050245716083));
#255216=CARTESIAN_POINT('Ctrl Pts',(-43.4987158872668,31.7093568101663,
-40.832021101787));
#255217=CARTESIAN_POINT('Ctrl Pts',(-43.5134312848982,31.7333600460206,
-40.8501267844669));
#255218=CARTESIAN_POINT('Ctrl Pts',(-43.5449969636312,31.7797747067972,
-40.8865288544817));
#255219=CARTESIAN_POINT('Ctrl Pts',(-43.570273480101,31.8133992725601,-40.9139774903764));
#255220=CARTESIAN_POINT('Ctrl Pts',(-43.6071874842548,31.8558549470217,
-40.9508682927202));
#255221=CARTESIAN_POINT('Ctrl Pts',(-43.6267265436653,31.8762775041081,
-40.9694100075909));
#255222=CARTESIAN_POINT('Ctrl Pts',(-43.6468212761471,31.8962967826001,
-40.9880061403947));
#255223=CARTESIAN_POINT('Ctrl Pts',(-43.6571524242715,31.9061057307006,
-40.997334528722));
#255224=CARTESIAN_POINT('Ctrl Pts',(-43.6781351765956,31.9250932263188,
-41.0158316653051));
#255225=CARTESIAN_POINT('Ctrl Pts',(-43.6888325213991,31.9343181422645,
-41.0250431278314));
#255226=CARTESIAN_POINT('Ctrl Pts',(-43.7214683281725,31.961133026229,-41.0525078158304));
#255227=CARTESIAN_POINT('Ctrl Pts',(-43.744000771517,31.977916302359,-41.070639272709));
#255228=CARTESIAN_POINT('Ctrl Pts',(-43.7905699795511,32.0092811177654,
-41.106520902203));
#255229=CARTESIAN_POINT('Ctrl Pts',(-43.8266341229871,32.0311632771839,
-41.1331548827895));
#255230=CARTESIAN_POINT('Ctrl Pts',(-43.8644344365312,32.050527928199,-41.1593656410909));
#255231=CARTESIAN_POINT('Ctrl Pts',(-43.8900335656271,32.0628690313763,
-41.1767476889401));
#255232=CARTESIAN_POINT('Ctrl Pts',(-43.903042008964,32.0687560539784,-41.1853974312384));
#255233=CARTESIAN_POINT('Ctrl Pts',(-43.9291618902095,32.0798229381751,
-41.2024070088898));
#255234=CARTESIAN_POINT('Ctrl Pts',(-43.9423286751247,32.0850301956599,
-41.2108047653586));
#255235=CARTESIAN_POINT('Ctrl Pts',(-43.9688389276373,32.0947834481969,
-41.2273662374836));
#255236=CARTESIAN_POINT('Ctrl Pts',(-44.0088868242005,32.1084293286422,
-41.2518690158044));
#255237=CARTESIAN_POINT('Ctrl Pts',(-44.0634057706764,32.1227159830699,
-41.2831968728749));
#255238=CARTESIAN_POINT('Ctrl Pts',(-44.1051448739617,32.1304686073096,
-41.30568419746));
#255239=CARTESIAN_POINT('Ctrl Pts',(-44.1331632182567,32.1349666221674,
-41.3204486001008));
#255240=CARTESIAN_POINT('Ctrl Pts',(-44.1472622735965,32.1368798783668,
-41.3277141420552));
#255241=CARTESIAN_POINT('Ctrl Pts',(-44.1685768983456,32.1392377391899,
-41.3384485067576));
#255242=CARTESIAN_POINT('Ctrl Pts',(-44.1757038998442,32.1399371964,-41.3419962566417));
#255243=CARTESIAN_POINT('Ctrl Pts',(-44.1899298892594,32.1411565650423,
-41.3489954369734));
#255244=CARTESIAN_POINT('Ctrl Pts',(-44.1970429564213,32.1416781032566,
-41.3524539903966));
#255245=CARTESIAN_POINT('Ctrl Pts',(-44.2183581262916,32.1429776302475,
-41.3626954949199));
#255246=CARTESIAN_POINT('Ctrl Pts',(-44.232556678806,32.1434929542666,-41.3693546778539));
#255247=CARTESIAN_POINT('Ctrl Pts',(-44.2750884056492,32.1439936324359,
-41.3888189062651));
#255248=CARTESIAN_POINT('Ctrl Pts',(-44.3033804172497,32.1429384256622,
-41.4011231160504));
#255249=CARTESIAN_POINT('Ctrl Pts',(-44.3598247343314,32.13804594572,-41.4243882373187));
#255250=CARTESIAN_POINT('Ctrl Pts',(-44.3879848006206,32.1342064546963,
-41.4353516241949));
#255251=CARTESIAN_POINT('Ctrl Pts',(-44.4230841862873,32.1276226980045,
-41.4481948195873));
#255252=CARTESIAN_POINT('Ctrl Pts',(-44.4301039616143,32.126214419323,-41.4507215814638));
#255253=CARTESIAN_POINT('Ctrl Pts',(-44.4441256434231,32.1232190082407,
-41.455685422358));
#255254=CARTESIAN_POINT('Ctrl Pts',(-44.4511413829898,32.1216281453652,
-41.4581270453932));
#255255=CARTESIAN_POINT('Ctrl Pts',(-44.472106554004,32.1165956901708,-41.4652964871519));
#255256=CARTESIAN_POINT('Ctrl Pts',(-44.4859328208737,32.1129061786889,
-41.4698557698741));
#255257=CARTESIAN_POINT('Ctrl Pts',(-44.5270324780087,32.1008340938932,
-41.4829067838587));
#255258=CARTESIAN_POINT('Ctrl Pts',(-44.5673316800757,32.08677017453,-41.4946921125766));
#255259=CARTESIAN_POINT('Ctrl Pts',(-44.6194780799712,32.0640738471498,
-41.5079096337926));
#255260=CARTESIAN_POINT('Ctrl Pts',(-44.6577884739158,32.045065905176,-41.5165678887371));
#255261=CARTESIAN_POINT('Ctrl Pts',(-44.6827916371924,32.031050813041,-41.5214942665077));
#255262=CARTESIAN_POINT('Ctrl Pts',(-44.7075150580676,32.0163554529027,
-41.5259894017533));
#255263=CARTESIAN_POINT('Ctrl Pts',(-44.7197631353705,32.0086467826241,
-41.5280237577537));
#255264=CARTESIAN_POINT('Ctrl Pts',(-44.7436779765282,31.9927322821733,
-41.5316086326721));
#255265=CARTESIAN_POINT('Ctrl Pts',(-44.7554039451266,31.9844926239501,
-41.5331705278033));
#255266=CARTESIAN_POINT('Ctrl Pts',(-44.7783650010144,31.9674779303508,
-41.5358342782831));
#255267=CARTESIAN_POINT('Ctrl Pts',(-44.8120876763637,31.941142023486,-41.5391427937509));
#255268=CARTESIAN_POINT('Ctrl Pts',(-44.8542060542843,31.9028069711657,
-41.5408368316843));
#255269=CARTESIAN_POINT('Ctrl Pts',(-44.883650374082,31.8716290815775,-41.5400605624154));
#255270=CARTESIAN_POINT('Ctrl Pts',(-44.9027957424029,31.8502960261458,
-41.5390808606534));
#255271=CARTESIAN_POINT('Ctrl Pts',(-44.912124025092,31.8393588588263,-41.5383603441012));
#255272=CARTESIAN_POINT('Ctrl Pts',(-44.9302963003321,31.816913187918,-41.5364463589967));
#255273=CARTESIAN_POINT('Ctrl Pts',(-44.9390653236876,31.8054960967264,
-41.5352602514373));
#255274=CARTESIAN_POINT('Ctrl Pts',(-44.9559494861592,31.7823260274566,
-41.532444286592));
#255275=CARTESIAN_POINT('Ctrl Pts',(-44.9803129684955,31.7470436123751,
-41.5275522735743));
#255276=CARTESIAN_POINT('Ctrl Pts',(-45.00183725318,31.7102129370948,-41.5206914933375));
#255277=CARTESIAN_POINT('Ctrl Pts',(-45.0280427451288,31.6597446570548,
-41.5098099510806));
#255278=CARTESIAN_POINT('Ctrl Pts',(-45.0398987329805,31.6338241168053,
-41.5034995556801));
#255279=CARTESIAN_POINT('Ctrl Pts',(-45.0531290598229,31.6005723463994,
-41.4945098705711));
#255280=CARTESIAN_POINT('Ctrl Pts',(-45.0556963147994,31.5938738844661,
-41.4926546478805));
#255281=CARTESIAN_POINT('Ctrl Pts',(-45.0606676096559,31.5803990532317,
-41.4888352403062));
#255282=CARTESIAN_POINT('Ctrl Pts',(-45.0630762139805,31.5736079348959,
-41.4868664774371));
#255283=CARTESIAN_POINT('Ctrl Pts',(-45.0700329505347,31.5531765604049,
-41.4808121016924));
#255284=CARTESIAN_POINT('Ctrl Pts',(-45.0743018132827,31.5395152309552,
-41.4765904297482));
#255285=CARTESIAN_POINT('Ctrl Pts',(-45.0860497029301,31.4983488303989,
-41.4633620161014));
#255286=CARTESIAN_POINT('Ctrl Pts',(-45.0988767040151,31.4430340104486,
-41.4442426901641));
#255287=CARTESIAN_POINT('Ctrl Pts',(-45.1061818129997,31.386882792419,-41.4222207481485));
#255288=CARTESIAN_POINT('Ctrl Pts',(-45.1095857869151,31.3444641027996,
-41.4046111316328));
#255289=CARTESIAN_POINT('Ctrl Pts',(-45.1103739871937,31.3302675876129,
-41.3985560195248));
#255290=CARTESIAN_POINT('Ctrl Pts',(-45.1110306052012,31.30890259785,-41.3891987399731));
#255291=CARTESIAN_POINT('Ctrl Pts',(-45.1111617199316,31.3017636946428,
-41.3860313075819));
#255292=CARTESIAN_POINT('Ctrl Pts',(-45.1112472734604,31.2874686716035,
-41.3796068875509));
#255293=CARTESIAN_POINT('Ctrl Pts',(-45.111201351958,31.2802974166487,-41.3763428889219));
#255294=CARTESIAN_POINT('Ctrl Pts',(-45.1107973541963,31.25882908612,-41.3664479958234));
#255295=CARTESIAN_POINT('Ctrl Pts',(-45.11017580813,31.2446005169708,-41.3597259135069));
#255296=CARTESIAN_POINT('Ctrl Pts',(-45.1082442962718,31.2162677536902,
-41.3460176286356));
#255297=CARTESIAN_POINT('Ctrl Pts',(-45.104314463686,31.1739750543259,-41.3250680443717));
#255298=CARTESIAN_POINT('Ctrl Pts',(-45.0950241996196,31.1183949914011,
-41.295609869938));
#255299=CARTESIAN_POINT('Ctrl Pts',(-45.0817381040079,31.0636149263882,
-41.264634106957));
#255300=CARTESIAN_POINT('Ctrl Pts',(-45.0737554763462,31.0364928582332,
-41.2486352837062));
#255301=CARTESIAN_POINT('Ctrl Pts',(-45.0650963255467,31.0095068957897,
-41.2323777508457));
#255302=CARTESIAN_POINT('Ctrl Pts',(-45.0604265398991,30.996076905732,-41.224116427314));
#255303=CARTESIAN_POINT('Ctrl Pts',(-45.0504049610752,30.9693743366894,
-41.2073411015006));
#255304=CARTESIAN_POINT('Ctrl Pts',(-45.0450945767524,30.9562107421528,
-41.1988958018751));
#255305=CARTESIAN_POINT('Ctrl Pts',(-45.0394875320819,30.9432190801919,
-41.190386719266));
#255306=CARTESIAN_POINT('',(-45.413889917786,33.3235045267141,-40.0133525317522));
#255307=CARTESIAN_POINT('Ctrl Pts',(-43.399376135545,33.205102110798,-39.5898551246884));
#255308=CARTESIAN_POINT('Ctrl Pts',(-43.4519070146144,33.2400854050083,
-39.607463913371));
#255309=CARTESIAN_POINT('Ctrl Pts',(-43.5337620388772,33.2891936594495,
-39.6337707491335));
#255310=CARTESIAN_POINT('Ctrl Pts',(-43.6195680771379,33.3326108090195,
-39.6596645368951));
#255311=CARTESIAN_POINT('Ctrl Pts',(-43.6784022657394,33.3605926156183,
-39.6770465847445));
#255312=CARTESIAN_POINT('Ctrl Pts',(-43.7083060299631,33.3739265642863,
-39.6856963270425));
#255313=CARTESIAN_POINT('Ctrl Pts',(-43.7683631864552,33.3989633419485,
-39.7027059046941));
#255314=CARTESIAN_POINT('Ctrl Pts',(-43.7986437698924,33.4107283136069,
-39.7111036611629));
#255315=CARTESIAN_POINT('Ctrl Pts',(-43.8596236543864,33.432731604347,-39.7276651332879));
#255316=CARTESIAN_POINT('Ctrl Pts',(-43.9517617731223,33.4634644421701,
-39.7521679116086));
#255317=CARTESIAN_POINT('Ctrl Pts',(-44.0772655876523,33.4954182164341,
-39.7834957686792));
#255318=CARTESIAN_POINT('Ctrl Pts',(-44.1734028302798,33.5125433235231,
-39.8059830932642));
#255319=CARTESIAN_POINT('Ctrl Pts',(-44.2379488567859,33.5224120576217,
-39.8207474959053));
#255320=CARTESIAN_POINT('Ctrl Pts',(-44.2704347193422,33.5265712650576,
-39.8280130378593));
#255321=CARTESIAN_POINT('Ctrl Pts',(-44.3195548787318,33.5316274184839,
-39.8387474025619));
#255322=CARTESIAN_POINT('Ctrl Pts',(-44.3359807184467,33.5331131204799,
-39.8422951524459));
#255323=CARTESIAN_POINT('Ctrl Pts',(-44.3687707333322,33.5356713331865,
-39.8492943327777));
#255324=CARTESIAN_POINT('Ctrl Pts',(-44.3851673533813,33.5367473433996,
-39.8527528862009));
#255325=CARTESIAN_POINT('Ctrl Pts',(-44.4343061264537,33.5393650105759,
-39.8629943907241));
#255326=CARTESIAN_POINT('Ctrl Pts',(-44.4670443896497,33.5403015249987,
-39.8696535736582));
#255327=CARTESIAN_POINT('Ctrl Pts',(-44.5651287758397,33.5407036712734,
-39.8891178020695));
#255328=CARTESIAN_POINT('Ctrl Pts',(-44.6303969251806,33.5377724131818,
-39.9014220118547));
#255329=CARTESIAN_POINT('Ctrl Pts',(-44.7606561433707,33.5255015904578,
-39.924687133123));
#255330=CARTESIAN_POINT('Ctrl Pts',(-44.8256651474086,33.516156778985,-39.93565052));
#255331=CARTESIAN_POINT('Ctrl Pts',(-44.9067230595199,33.5003653725032,
-39.9484937153914));
#255332=CARTESIAN_POINT('Ctrl Pts',(-44.9229358898309,33.4969961660477,
-39.9510204772682));
#255333=CARTESIAN_POINT('Ctrl Pts',(-44.9553232364802,33.4898458857957,
-39.9559843181622));
#255334=CARTESIAN_POINT('Ctrl Pts',(-44.9715297170939,33.48605597099,-39.9584259411976));
#255335=CARTESIAN_POINT('Ctrl Pts',(-45.0199641404161,33.4740887742096,
-39.965595382956));
#255336=CARTESIAN_POINT('Ctrl Pts',(-45.0519120411053,33.4653422982392,
-39.9701546656783));
#255337=CARTESIAN_POINT('Ctrl Pts',(-45.1468975937756,33.4367966020141,
-39.983205679663));
#255338=CARTESIAN_POINT('Ctrl Pts',(-45.2400693383874,33.4036742979489,
-39.9949910083808));
#255339=CARTESIAN_POINT('Ctrl Pts',(-45.3486712153738,33.3557567039275,
-40.0068900294228));
#255340=CARTESIAN_POINT('Ctrl Pts',(-45.3961814822964,33.332503308482,-40.0116442129886));
#255341=CARTESIAN_POINT('Ctrl Pts',(-45.4138896478391,33.3235054357711,
-40.0133501741483));
#255342=CARTESIAN_POINT('Ctrl Pts',(-45.4138896492504,33.3235039948814,
-40.0133529162944));
#255343=CARTESIAN_POINT('Ctrl Pts',(-45.220007869287,33.4018089092386,-40.0137878164737));
#255344=CARTESIAN_POINT('Ctrl Pts',(-45.0135121509523,33.4437912620812,
-40.0118840249176));
#255345=CARTESIAN_POINT('Ctrl Pts',(-44.6315114877946,33.4515951730344,
-40.0050871993533));
#255346=CARTESIAN_POINT('Ctrl Pts',(-44.4590991737821,33.4292864011566,
-40.0008095143876));
#255347=CARTESIAN_POINT('Ctrl Pts',(-44.0965692082188,33.3271748070394,
-39.9897581690022));
#255348=CARTESIAN_POINT('Ctrl Pts',(-43.9111554000927,33.2383845853547,
-39.9827536906167));
#255349=CARTESIAN_POINT('Ctrl Pts',(-43.5996400949778,33.0179220859889,
-39.9689626255907));
#255350=CARTESIAN_POINT('Ctrl Pts',(-43.4715347449999,32.8953861314864,
-39.962602231998));
#255351=CARTESIAN_POINT('Ctrl Pts',(-43.3633208282253,32.7547543987198,
-39.9581074212483));
#255352=CARTESIAN_POINT('Ctrl Pts',(-43.0534148594278,32.3583957084033,
-39.8341886583259));
#255353=CARTESIAN_POINT('Ctrl Pts',(-43.085178776931,32.5092364820398,-39.7972070934614));
#255354=CARTESIAN_POINT('Ctrl Pts',(-43.1311025668885,32.6568722937985,
-39.7575468725598));
#255355=CARTESIAN_POINT('Ctrl Pts',(-43.2471037313335,32.939586900846,-39.6756564072208));
#255356=CARTESIAN_POINT('Ctrl Pts',(-43.3174654472053,33.0756353558302,
-39.6331721875354));
#255357=CARTESIAN_POINT('Ctrl Pts',(-43.3993761267971,33.2051021146614,
-39.5898551195224));
#255358=CARTESIAN_POINT('Ctrl Pts',(-46.6981266849492,30.7091523375488,
-39.2904704603133));
#255359=CARTESIAN_POINT('Ctrl Pts',(-46.6689684123063,30.6404043382273,
-39.273452295095));
#255360=CARTESIAN_POINT('Ctrl Pts',(-46.6043681216411,30.5066861069553,
-39.238925705885));
#255361=CARTESIAN_POINT('Ctrl Pts',(-46.5083209189471,30.3487389562033,
-39.1945593129175));
#255362=CARTESIAN_POINT('Ctrl Pts',(-46.4437937583117,30.2581216171786,
-39.1673894861782));
#255363=CARTESIAN_POINT('Ctrl Pts',(-46.3992224148768,30.1986447451181,
-39.1491520227249));
#255364=CARTESIAN_POINT('Ctrl Pts',(-46.3761748773305,30.1693908446446,
-39.1399767764946));
#255365=CARTESIAN_POINT('Ctrl Pts',(-46.3284414024809,30.1117648114071,
-39.1214771434543));
#255366=CARTESIAN_POINT('Ctrl Pts',(-46.3038983378397,30.083571828401,-39.112209259666));
#255367=CARTESIAN_POINT('Ctrl Pts',(-46.253707387608,30.0286632749651,-39.0937226519629));
#255368=CARTESIAN_POINT('Ctrl Pts',(-46.2280147026909,30.001893564456,-39.0844865568113));
#255369=CARTESIAN_POINT('Ctrl Pts',(-46.1492148010453,29.9236586721517,
-39.0568159196779));
#255370=CARTESIAN_POINT('Ctrl Pts',(-46.0669347173688,29.8495134741745,
-39.0292038481275));
#255371=CARTESIAN_POINT('Ctrl Pts',(-45.9503410384262,29.7587889734315,
-38.9925114043613));
#255372=CARTESIAN_POINT('Ctrl Pts',(-45.8594191065401,29.6948377475824,
-38.9650526418885));
#255373=CARTESIAN_POINT('Ctrl Pts',(-45.7964751089327,29.6549785818455,
-38.9467936623891));
#255374=CARTESIAN_POINT('Ctrl Pts',(-45.748348603817,29.6261284949947,-38.9331097524421));
#255375=CARTESIAN_POINT('Ctrl Pts',(-45.7321473284057,29.616684052073,-38.9285487676403));
#255376=CARTESIAN_POINT('Ctrl Pts',(-45.6996106203311,29.5982459977232,
-38.9194791520014));
#255377=CARTESIAN_POINT('Ctrl Pts',(-45.683249044345,29.5892352448745,-38.9149628379356));
#255378=CARTESIAN_POINT('Ctrl Pts',(-45.6010439155842,29.5452684013657,
-38.8924942188443));
#255379=CARTESIAN_POINT('Ctrl Pts',(-45.4667739830181,29.4816584171599,
-38.8571935516581));
#255380=CARTESIAN_POINT('Ctrl Pts',(-45.2922645146651,29.4187721922835,
-38.8147007629208));
#255381=CARTESIAN_POINT('Ctrl Pts',(-45.184512437616,29.3885937253944,-38.7899522655792));
#255382=CARTESIAN_POINT('Ctrl Pts',(-45.1119891467798,29.3701842541612,
-38.7736235920333));
#255383=CARTESIAN_POINT('Ctrl Pts',(-45.0754052578815,29.3618381514785,
-38.7655490803555));
#255384=CARTESIAN_POINT('Ctrl Pts',(-45.0014447932705,29.3468760834356,
-38.7495561846596));
#255385=CARTESIAN_POINT('Ctrl Pts',(-44.964301863367,29.3403115562353,-38.7416890516424));
#255386=CARTESIAN_POINT('Ctrl Pts',(-44.8900079594565,29.3290481892184,
-38.726277749838));
#255387=CARTESIAN_POINT('Ctrl Pts',(-44.8527936282157,29.324336495618,-38.7187198739728));
#255388=CARTESIAN_POINT('Ctrl Pts',(-44.7410083373266,29.3129455735289,
-38.6964994820139));
#255389=CARTESIAN_POINT('Ctrl Pts',(-44.6662563757167,29.3089967422249,
-38.6822807693139));
#255390=CARTESIAN_POINT('Ctrl Pts',(-44.516312468428,29.3084067934202,-38.6550493453909));
#255391=CARTESIAN_POINT('Ctrl Pts',(-44.441103189525,29.3117700143417,-38.6420342479066));
#255392=CARTESIAN_POINT('Ctrl Pts',(-44.3468378615956,29.3206690055189,
-38.6265520162729));
#255393=CARTESIAN_POINT('Ctrl Pts',(-44.3279589148655,29.3226883315868,
-38.6234933649988));
#255394=CARTESIAN_POINT('Ctrl Pts',(-44.2901960653062,29.3271995080042,
-38.6174591262491));
#255395=CARTESIAN_POINT('Ctrl Pts',(-44.271274393292,29.329697893027,-38.614477863833));
#255396=CARTESIAN_POINT('Ctrl Pts',(-44.2146592782019,29.3378915995821,
-38.60568558559));
#255397=CARTESIAN_POINT('Ctrl Pts',(-44.1772069502033,29.344266758826,-38.6000392683017));
#255398=CARTESIAN_POINT('Ctrl Pts',(-44.0655444875092,29.3661148598052,
-38.5837127379559));
#255399=CARTESIAN_POINT('Ctrl Pts',(-43.9553791862171,29.3933792052515,
-38.5686255047386));
#255400=CARTESIAN_POINT('Ctrl Pts',(-43.8114622524781,29.4404829778103,
-38.5509833019505));
#255401=CARTESIAN_POINT('Ctrl Pts',(-43.705021834675,29.481230340464,-38.5390021142185));
#255402=CARTESIAN_POINT('Ctrl Pts',(-43.6350719757086,29.512061063653,-38.5318621614261));
#255403=CARTESIAN_POINT('Ctrl Pts',(-43.5656410085295,29.5447591316771,
-38.525155654825));
#255404=CARTESIAN_POINT('Ctrl Pts',(-43.5311320054746,29.5620794464364,
-38.5220163122062));
#255405=CARTESIAN_POINT('Ctrl Pts',(-43.4634866412134,29.5981758355574,
-38.5162526847879));
#255406=CARTESIAN_POINT('Ctrl Pts',(-43.4301834663392,29.6170276546,-38.5136117755133));
#255407=CARTESIAN_POINT('Ctrl Pts',(-43.3647025891651,29.6562685687332,
-38.5088155315793));
#255408=CARTESIAN_POINT('Ctrl Pts',(-43.2681192378476,29.7174608121974,
-38.5023448938576));
#255409=CARTESIAN_POINT('Ctrl Pts',(-43.1764049274077,29.7855824582168,
-38.4980286134812));
#255410=CARTESIAN_POINT('Ctrl Pts',(-43.0584774180437,29.8826126224142,
-38.4942050936184));
#255411=CARTESIAN_POINT('Ctrl Pts',(-43.001681818637,29.9342392650769,-38.4932590761897));
#255412=CARTESIAN_POINT('Ctrl Pts',(-42.8926599718677,30.0438904492243,
-38.4933742455196));
#255413=CARTESIAN_POINT('Ctrl Pts',(-42.8414047150844,30.1009342501745,
-38.4944336470273));
#255414=CARTESIAN_POINT('Ctrl Pts',(-42.7451036203247,30.2193471227021,
-38.498479276642));
#255415=CARTESIAN_POINT('Ctrl Pts',(-42.6550322643363,30.3420646399833,
-38.5044516702661));
#255416=CARTESIAN_POINT('Ctrl Pts',(-42.5773225406025,30.4733365238586,
-38.5142428327574));
#255417=CARTESIAN_POINT('Ctrl Pts',(-42.5326943378214,30.5580963840027,
-38.5215739479982));
#255418=CARTESIAN_POINT('Ctrl Pts',(-42.5239673850246,30.5751883092729,
-38.5231018165939));
#255419=CARTESIAN_POINT('Ctrl Pts',(-42.5069121510755,30.60964376351,-38.5262794637242));
#255420=CARTESIAN_POINT('Ctrl Pts',(-42.4985805781952,30.627019094627,-38.5279307934181));
#255421=CARTESIAN_POINT('Ctrl Pts',(-42.4743295471271,30.6792614198295,
-38.5330409224498));
#255422=CARTESIAN_POINT('Ctrl Pts',(-42.4438856226513,30.7493896366731,
-38.5402834483744));
#255423=CARTESIAN_POINT('Ctrl Pts',(-42.4037483179465,30.8560072598611,
-38.5524071291592));
#255424=CARTESIAN_POINT('Ctrl Pts',(-42.3690543371876,30.9640160484273,
-38.5657659376104));
#255425=CARTESIAN_POINT('Ctrl Pts',(-42.3397558527982,31.0734075527136,
-38.5803463747351));
#255426=CARTESIAN_POINT('Ctrl Pts',(-42.3238156343608,31.1472555030051,
-38.5908775753381));
#255427=CARTESIAN_POINT('Ctrl Pts',(-42.3096820427396,31.2215665449467,
-38.6018154236264));
#255428=CARTESIAN_POINT('Ctrl Pts',(-42.3035171869091,31.2589715314082,
-38.6074906718877));
#255429=CARTESIAN_POINT('Ctrl Pts',(-42.2930235524414,31.3341791410138,
-38.6192399292287));
#255430=CARTESIAN_POINT('Ctrl Pts',(-42.2886818075092,31.3721585359098,
-38.6253436316658));
#255431=CARTESIAN_POINT('Ctrl Pts',(-42.281930630611,31.4478003630713,-38.6378362101326));
#255432=CARTESIAN_POINT('Ctrl Pts',(-42.277074994566,31.5232809912004,-38.6506356205751));
#255433=CARTESIAN_POINT('Ctrl Pts',(-42.2747992363309,31.6735553614761,
-38.6774229397946));
#255434=CARTESIAN_POINT('Ctrl Pts',(-42.2834818483937,31.8228397562226,
-38.7059581415094));
#255435=CARTESIAN_POINT('Ctrl Pts',(-42.3030248127084,31.9711385758679,
-38.7362097844166));
#255436=CARTESIAN_POINT('Ctrl Pts',(-42.3164494406915,32.0449687602614,
-38.7519128032936));
#255437=CARTESIAN_POINT('Ctrl Pts',(-42.3317154579634,32.1186122141692,
-38.7679009120377));
#255438=CARTESIAN_POINT('Ctrl Pts',(-42.3402956643805,32.1554227583218,
-38.7760569897633));
#255439=CARTESIAN_POINT('Ctrl Pts',(-42.3591481714288,32.228169160774,-38.7925026060078));
#255440=CARTESIAN_POINT('Ctrl Pts',(-42.3694448348212,32.2642362896146,
-38.8008201507359));
#255441=CARTESIAN_POINT('Ctrl Pts',(-42.4028917825415,32.3714169561226,
-38.8260275044574));
#255442=CARTESIAN_POINT('Ctrl Pts',(-42.428602574983,32.4415633880281,-38.8431823298655));
#255443=CARTESIAN_POINT('Ctrl Pts',(-42.4722685042023,32.5448307979217,
-38.8694323201497));
#255444=CARTESIAN_POINT('Ctrl Pts',(-42.4876674804306,32.5789105800712,
-38.8782643966373));
#255445=CARTESIAN_POINT('Ctrl Pts',(-42.5202146590728,32.6464795812123,
-38.8961197808447));
#255446=CARTESIAN_POINT('Ctrl Pts',(-42.5373018269229,32.6798350022668,
-38.9051083126545));
#255447=CARTESIAN_POINT('Ctrl Pts',(-42.5906929412925,32.7780783962456,
-38.9321048428364));
#255448=CARTESIAN_POINT('Ctrl Pts',(-42.629225789877,32.8414173722334,-38.9502105255135));
#255449=CARTESIAN_POINT('Ctrl Pts',(-42.7120000069194,32.9638220552461,
-38.9866125955294));
#255450=CARTESIAN_POINT('Ctrl Pts',(-42.7783647966162,33.0524402968179,
-39.0140612314234));
#255451=CARTESIAN_POINT('Ctrl Pts',(-42.8754380724448,33.1642175243331,
-39.0509520337677));
#255452=CARTESIAN_POINT('Ctrl Pts',(-42.9268673384212,33.2179450225078,
-39.0694937486382));
#255453=CARTESIAN_POINT('Ctrl Pts',(-42.9797817061918,33.2705900457306,
-39.088089881442));
#255454=CARTESIAN_POINT('Ctrl Pts',(-43.0069972096607,33.2963736994336,
-39.097418269769));
#255455=CARTESIAN_POINT('Ctrl Pts',(-43.0622936398443,33.3462615369726,
-39.1159154063528));
#255456=CARTESIAN_POINT('Ctrl Pts',(-43.0904949946047,33.3704876748183,
-39.1251268688783));
#255457=CARTESIAN_POINT('Ctrl Pts',(-43.176562606447,33.4408730143712,-39.1525915568785));
#255458=CARTESIAN_POINT('Ctrl Pts',(-43.2360245534179,33.4848790444095,
-39.1707230137558));
#255459=CARTESIAN_POINT('Ctrl Pts',(-43.358992255749,33.5670176609587,-39.2066046432507));
#255460=CARTESIAN_POINT('Ctrl Pts',(-43.4542745623933,33.6242424638975,
-39.233238623837));
#255461=CARTESIAN_POINT('Ctrl Pts',(-43.5542222374601,33.6747516510336,
-39.2594493821381));
#255462=CARTESIAN_POINT('Ctrl Pts',(-43.6219256430316,33.7069073870393,
-39.2768314299875));
#255463=CARTESIAN_POINT('Ctrl Pts',(-43.6563381479934,33.7222286468184,
-39.2854811722856));
#255464=CARTESIAN_POINT('Ctrl Pts',(-43.7254519170511,33.7509934760635,
-39.3024907499371));
#255465=CARTESIAN_POINT('Ctrl Pts',(-43.7602995448845,33.7645084608315,
-39.3108885064059));
#255466=CARTESIAN_POINT('Ctrl Pts',(-43.8304781084082,33.789780836939,-39.3274499785309));
#255467=CARTESIAN_POINT('Ctrl Pts',(-43.9365171946568,33.8250735562425,
-39.3519527568515));
#255468=CARTESIAN_POINT('Ctrl Pts',(-44.0809642638621,33.8617420360433,
-39.3832806139221));
#255469=CARTESIAN_POINT('Ctrl Pts',(-44.1916183723467,33.8813683146414,
-39.4057679385072));
#255470=CARTESIAN_POINT('Ctrl Pts',(-44.2659122959159,33.8926702964892,
-39.4205323411483));
#255471=CARTESIAN_POINT('Ctrl Pts',(-44.3033049221432,33.8974288658374,
-39.4277978831022));
#255472=CARTESIAN_POINT('Ctrl Pts',(-44.3598453576919,33.9032050944765,
-39.4385322478049));
#255473=CARTESIAN_POINT('Ctrl Pts',(-44.3787527158677,33.9049006163346,
-39.4420799976889));
#255474=CARTESIAN_POINT('Ctrl Pts',(-44.4164967874688,33.9078161173588,
-39.4490791780208));
#255475=CARTESIAN_POINT('Ctrl Pts',(-44.4353708468856,33.9090400957878,
-39.4525377314439));
#255476=CARTESIAN_POINT('Ctrl Pts',(-44.4919347179527,33.9120095261765,
-39.462779235967));
#255477=CARTESIAN_POINT('Ctrl Pts',(-44.52962054914,33.9130584408517,-39.4694384189012));
#255478=CARTESIAN_POINT('Ctrl Pts',(-44.6425299001817,33.9134342925821,
-39.4889026473125));
#255479=CARTESIAN_POINT('Ctrl Pts',(-44.7176656228988,33.9100023852834,
-39.5012068570978));
#255480=CARTESIAN_POINT('Ctrl Pts',(-44.867623327666,33.8957625538083,-39.524471978366));
#255481=CARTESIAN_POINT('Ctrl Pts',(-44.9424659600731,33.8849485744664,
-39.5354353652432));
#255482=CARTESIAN_POINT('Ctrl Pts',(-45.0357885152669,33.8666999843662,
-39.5482785606344));
#255483=CARTESIAN_POINT('Ctrl Pts',(-45.0544546343785,33.8628074782943,
-39.5508053225112));
#255484=CARTESIAN_POINT('Ctrl Pts',(-45.091743102575,33.8545484160302,-39.5557691634051));
#255485=CARTESIAN_POINT('Ctrl Pts',(-45.1104022544846,33.850171655015,-39.5582107864407));
#255486=CARTESIAN_POINT('Ctrl Pts',(-45.1661672125598,33.8363538303533,
-39.5653802281989));
#255487=CARTESIAN_POINT('Ctrl Pts',(-45.2029511118778,33.8262578362557,
-39.5699395109212));
#255488=CARTESIAN_POINT('Ctrl Pts',(-45.312316831343,33.7933159380614,-39.582990524906));
#255489=CARTESIAN_POINT('Ctrl Pts',(-45.4195983160475,33.7551076509549,
-39.5947758536238));
#255490=CARTESIAN_POINT('Ctrl Pts',(-45.5585113890164,33.6937328563153,
-39.6079933748399));
#255491=CARTESIAN_POINT('Ctrl Pts',(-45.6606150024606,33.6424505696195,
-39.6166516297843));
#255492=CARTESIAN_POINT('Ctrl Pts',(-45.7272860947277,33.6047101271221,
-39.6215780075552));
#255493=CARTESIAN_POINT('Ctrl Pts',(-45.7932287365117,33.5651705839516,
-39.6260731428005));
#255494=CARTESIAN_POINT('Ctrl Pts',(-45.8259059249178,33.5444453395394,
-39.6281074988013));
#255495=CARTESIAN_POINT('Ctrl Pts',(-45.8897275017006,33.5016881508368,
-39.6316923737189));
#255496=CARTESIAN_POINT('Ctrl Pts',(-45.9210297733036,33.4795651380848,
-39.6332542688506));
#255497=CARTESIAN_POINT('Ctrl Pts',(-45.9823424846244,33.4339088874735,
-39.6359180193303));
#255498=CARTESIAN_POINT('Ctrl Pts',(-46.0724202597563,33.3632801300718,
-39.6392265347984));
#255499=CARTESIAN_POINT('Ctrl Pts',(-46.1850394564173,33.2606222983665,
-39.6409205727319));
#255500=CARTESIAN_POINT('Ctrl Pts',(-46.2638636333332,33.1772336958075,
-39.6401443034625));
#255501=CARTESIAN_POINT('Ctrl Pts',(-46.3151397511292,33.1201974856456,
-39.6391646017005));
#255502=CARTESIAN_POINT('Ctrl Pts',(-46.3401349353408,33.0909661742941,
-39.6384440851485));
#255503=CARTESIAN_POINT('Ctrl Pts',(-46.3888523044997,33.0309971480077,
-39.6365301000439));
#255504=CARTESIAN_POINT('Ctrl Pts',(-46.4123735341802,33.0005036828642,
-39.6353439924849));
#255505=CARTESIAN_POINT('Ctrl Pts',(-46.4576879006691,32.9386388625828,
-39.6325280276393));
#255506=CARTESIAN_POINT('Ctrl Pts',(-46.52311576659,32.8444620833496,-39.6276360146217));
#255507=CARTESIAN_POINT('Ctrl Pts',(-46.5810426872604,32.7462345994881,
-39.6207752343847));
#255508=CARTESIAN_POINT('Ctrl Pts',(-46.6516918187307,32.6117039458857,
-39.6098936921283));
#255509=CARTESIAN_POINT('Ctrl Pts',(-46.683723185051,32.5426422373878,-39.6035832967262));
#255510=CARTESIAN_POINT('Ctrl Pts',(-46.7195635412788,32.4540883209461,
-39.5945936116187));
#255511=CARTESIAN_POINT('Ctrl Pts',(-46.7265235775841,32.4362514419463,
-39.5927383889278));
#255512=CARTESIAN_POINT('Ctrl Pts',(-46.7400123459627,32.4003742100513,
-39.5889189813535));
#255513=CARTESIAN_POINT('Ctrl Pts',(-46.7465535157541,32.3822946053341,
-39.5869502184844));
#255514=CARTESIAN_POINT('Ctrl Pts',(-46.7654644360989,32.3279072933142,
-39.5808958427402));
#255515=CARTESIAN_POINT('Ctrl Pts',(-46.7770937339888,32.2915493874551,
-39.5766741707955));
#255516=CARTESIAN_POINT('Ctrl Pts',(-46.8091770518909,32.182013131159,-39.5634457571489));
#255517=CARTESIAN_POINT('Ctrl Pts',(-46.8444383818759,32.034891308334,-39.5443264312115));
#255518=CARTESIAN_POINT('Ctrl Pts',(-46.8650708643864,31.8856621776612,
-39.5223044891954));
#255519=CARTESIAN_POINT('Ctrl Pts',(-46.8750487417844,31.7729724844591,
-39.50469487268));
#255520=CARTESIAN_POINT('Ctrl Pts',(-46.8774570362353,31.7352651712118,
-39.4986397605723));
#255521=CARTESIAN_POINT('Ctrl Pts',(-46.8796767940079,31.6785286095959,
-39.4892824810203));
#255522=CARTESIAN_POINT('Ctrl Pts',(-46.8801843407089,31.6595724593507,
-39.4861150486293));
#255523=CARTESIAN_POINT('Ctrl Pts',(-46.8807312344332,31.6216180949417,
-39.479690628598));
#255524=CARTESIAN_POINT('Ctrl Pts',(-46.8807699646674,31.6025797052015,
-39.4764266299692));
#255525=CARTESIAN_POINT('Ctrl Pts',(-46.8801790388754,31.5455906639181,
-39.4665317368708));
#255526=CARTESIAN_POINT('Ctrl Pts',(-46.8788490796135,31.5078273383739,
-39.4598096545541));
#255527=CARTESIAN_POINT('Ctrl Pts',(-46.874360617844,31.4326451774338,-39.4461013696832));
#255528=CARTESIAN_POINT('Ctrl Pts',(-46.864884835636,31.320441459725,-39.4251517854185));
#255529=CARTESIAN_POINT('Ctrl Pts',(-46.8414902947658,31.1730719473388,
-39.3956936109857));
#255530=CARTESIAN_POINT('Ctrl Pts',(-46.8074810934279,31.0279105813681,
-39.364717848004));
#255531=CARTESIAN_POINT('Ctrl Pts',(-46.7869180083019,30.9560697433081,
-39.3487190247537));
#255532=CARTESIAN_POINT('Ctrl Pts',(-46.7645577771926,30.884604709384,-39.332461491893));
#255533=CARTESIAN_POINT('Ctrl Pts',(-46.7524740339114,30.8490466969583,
-39.3242001683612));
#255534=CARTESIAN_POINT('Ctrl Pts',(-46.7264943673172,30.7783632715819,
-39.3074248425479));
#255535=CARTESIAN_POINT('Ctrl Pts',(-46.7127058212706,30.7435263372096,
-39.2989795429224));
#255536=CARTESIAN_POINT('Ctrl Pts',(-46.6981266849492,30.7091523375488,
-39.2904704603133));
#255537=CARTESIAN_POINT('Ctrl Pts',(-45.0394875320819,30.9432190801919,
-41.190386719266));
#255538=CARTESIAN_POINT('Ctrl Pts',(-45.0282734427409,30.91723575627,-41.1733685540478));
#255539=CARTESIAN_POINT('Ctrl Pts',(-45.0034876660128,30.8666726764904,
-41.1388419648381));
#255540=CARTESIAN_POINT('Ctrl Pts',(-44.9667665375866,30.8068862988478,
-41.09447557187));
#255541=CARTESIAN_POINT('Ctrl Pts',(-44.9421458413835,30.7725558756156,
-41.0673057451311));
#255542=CARTESIAN_POINT('Ctrl Pts',(-44.9251493960809,30.7500159625169,
-41.0490682816776));
#255543=CARTESIAN_POINT('Ctrl Pts',(-44.9163654668634,30.7389260450349,
-41.0398930354472));
#255544=CARTESIAN_POINT('Ctrl Pts',(-44.8981827131164,30.7170729960788,
-41.0213934024069));
#255545=CARTESIAN_POINT('Ctrl Pts',(-44.888838333634,30.7063777841388,-41.0121255186188));
#255546=CARTESIAN_POINT('Ctrl Pts',(-44.8697378119757,30.6855401076749,
-40.9936389109155));
#255547=CARTESIAN_POINT('Ctrl Pts',(-44.8599646045333,30.6753771122426,
-40.984402815764));
#255548=CARTESIAN_POINT('Ctrl Pts',(-44.8300025766326,30.6456635434001,
-40.9567321786306));
#255549=CARTESIAN_POINT('Ctrl Pts',(-44.7987417882795,30.6174785558847,
-40.9291201070801));
#255550=CARTESIAN_POINT('Ctrl Pts',(-44.7544912812914,30.5829390177582,
-40.8924276633141));
#255551=CARTESIAN_POINT('Ctrl Pts',(-44.7200063674423,30.5585634922437,
-40.8649689008411));
#255552=CARTESIAN_POINT('Ctrl Pts',(-44.6961476159991,30.5433500948652,
-40.8467099213417));
#255553=CARTESIAN_POINT('Ctrl Pts',(-44.6779108400504,30.5323301088838,
-40.8330260113948));
#255554=CARTESIAN_POINT('Ctrl Pts',(-44.6717725199842,30.5287210947847,
-40.8284650265932));
#255555=CARTESIAN_POINT('Ctrl Pts',(-44.6594468286685,30.521672327511,-40.8193954109541));
#255556=CARTESIAN_POINT('Ctrl Pts',(-44.6532495459125,30.5182260348866,
-40.8148790968875));
#255557=CARTESIAN_POINT('Ctrl Pts',(-44.6221170703041,30.5014023919654,
-40.7924104777995));
#255558=CARTESIAN_POINT('Ctrl Pts',(-44.5712944462502,30.4770113822335,
-40.7571098106096));
#255559=CARTESIAN_POINT('Ctrl Pts',(-44.5053084694641,30.4527583886953,
-40.7146170218743));
#255560=CARTESIAN_POINT('Ctrl Pts',(-44.4645950315289,30.4410392847555,
-40.6898685245315));
#255561=CARTESIAN_POINT('Ctrl Pts',(-44.4371992237873,30.4338676574989,
-40.6735398509862));
#255562=CARTESIAN_POINT('Ctrl Pts',(-44.4233828828253,30.4306039319716,
-40.6654653393082));
#255563=CARTESIAN_POINT('Ctrl Pts',(-44.395457566773,30.4247250011004,-40.6494724436125));
#255564=CARTESIAN_POINT('Ctrl Pts',(-44.3814368244576,30.4221299378924,
-40.6416053105951));
#255565=CARTESIAN_POINT('Ctrl Pts',(-44.353398925472,30.4176419772095,-40.6261940087904));
#255566=CARTESIAN_POINT('Ctrl Pts',(-44.3393578467875,30.4157440298243,
-40.6186361329255));
#255567=CARTESIAN_POINT('Ctrl Pts',(-44.2971907773647,30.4110825461462,
-40.5964157409664));
#255568=CARTESIAN_POINT('Ctrl Pts',(-44.2690063197214,30.4093460565949,
-40.5821970282665));
#255569=CARTESIAN_POINT('Ctrl Pts',(-44.212497942469,30.4086221665927,-40.5549656043439));
#255570=CARTESIAN_POINT('Ctrl Pts',(-44.1841675064314,30.4096363406377,
-40.5419505068598));
#255571=CARTESIAN_POINT('Ctrl Pts',(-44.1486758957365,30.4126704859088,
-40.5264682752254));
#255572=CARTESIAN_POINT('Ctrl Pts',(-44.141568690144,30.4133673915631,-40.5234096239519));
#255573=CARTESIAN_POINT('Ctrl Pts',(-44.1273541295014,30.414939058346,-40.5173753852017));
#255574=CARTESIAN_POINT('Ctrl Pts',(-44.1202325648852,30.4158161528369,
-40.5143941227858));
#255575=CARTESIAN_POINT('Ctrl Pts',(-44.0989269046614,30.418710900521,-40.5056018445424));
#255576=CARTESIAN_POINT('Ctrl Pts',(-44.0848361489451,30.4209852789275,
-40.4999555272545));
#255577=CARTESIAN_POINT('Ctrl Pts',(-44.0428355440345,30.4288357011986,
-40.4836289969086));
#255578=CARTESIAN_POINT('Ctrl Pts',(-44.001418907738,30.4387301387603,-40.4685417636913));
#255579=CARTESIAN_POINT('Ctrl Pts',(-43.9473552852602,30.4559806561897,
-40.4508995609031));
#255580=CARTESIAN_POINT('Ctrl Pts',(-43.9073915907435,30.4709642266074,
-40.4389183731711));
#255581=CARTESIAN_POINT('Ctrl Pts',(-43.8811432548962,30.4823370897352,
-40.4317784203789));
#255582=CARTESIAN_POINT('Ctrl Pts',(-43.8550972458946,30.4944149327137,
-40.4250719137776));
#255583=CARTESIAN_POINT('Ctrl Pts',(-43.8421555815742,30.5008203273088,
-40.4219325711588));
#255584=CARTESIAN_POINT('Ctrl Pts',(-43.8167947927211,30.5141840584711,
-40.4161689437405));
#255585=CARTESIAN_POINT('Ctrl Pts',(-43.8043130802594,30.5211703528968,
-40.413528034466));
#255586=CARTESIAN_POINT('Ctrl Pts',(-43.7797793173031,30.5357258010655,
-40.4087317905317));
#255587=CARTESIAN_POINT('Ctrl Pts',(-43.7436043213473,30.5584424906522,
-40.4022611528103));
#255588=CARTESIAN_POINT('Ctrl Pts',(-43.7092889915882,30.583786036936,-40.397944872434));
#255589=CARTESIAN_POINT('Ctrl Pts',(-43.6651994519323,30.6199287507259,
-40.394121352571));
#255590=CARTESIAN_POINT('Ctrl Pts',(-43.6439827068456,30.6391798378995,
-40.3931753351425));
#255591=CARTESIAN_POINT('Ctrl Pts',(-43.6032932824946,30.680108587057,-40.3932905044721));
#255592=CARTESIAN_POINT('Ctrl Pts',(-43.5841829799745,30.7014201645355,
-40.3943499059801));
#255593=CARTESIAN_POINT('Ctrl Pts',(-43.5483166082379,30.7456951818503,
-40.3983955355947));
#255594=CARTESIAN_POINT('Ctrl Pts',(-43.5148120542517,30.7916143604394,
-40.4043679292189));
#255595=CARTESIAN_POINT('Ctrl Pts',(-43.4859931451963,30.8408014772341,
-40.4141590917094));
#255596=CARTESIAN_POINT('Ctrl Pts',(-43.469474574758,30.8725808034089,-40.4214902069511));
#255597=CARTESIAN_POINT('Ctrl Pts',(-43.4662461658165,30.8789901287051,
-40.4230180755467));
#255598=CARTESIAN_POINT('Ctrl Pts',(-43.4599404108544,30.8919125782622,
-40.4261957226772));
#255599=CARTESIAN_POINT('Ctrl Pts',(-43.4568618652692,30.8984301381776,
-40.4278470523708));
#255600=CARTESIAN_POINT('Ctrl Pts',(-43.4479066843131,30.9180293597941,
-40.4329571814025));
#255601=CARTESIAN_POINT('Ctrl Pts',(-43.4366800830858,30.9443463169446,
-40.440199707327));
#255602=CARTESIAN_POINT('Ctrl Pts',(-43.4219268251392,30.9843790154574,
-40.4523233881121));
#255603=CARTESIAN_POINT('Ctrl Pts',(-43.4092278315493,31.0249558361973,
-40.4656821965631));
#255604=CARTESIAN_POINT('Ctrl Pts',(-43.3985649158327,31.0660734353404,
-40.4802626336878));
#255605=CARTESIAN_POINT('Ctrl Pts',(-43.3928117504253,31.0938450909326,
-40.4907938342908));
#255606=CARTESIAN_POINT('Ctrl Pts',(-43.3877402558097,31.1217978520093,
-40.5017316825792));
#255607=CARTESIAN_POINT('Ctrl Pts',(-43.3855448869231,31.1358715333473,
-40.5074069308404));
#255608=CARTESIAN_POINT('Ctrl Pts',(-43.3818466485176,31.1641754295066,
-40.5191561881817));
#255609=CARTESIAN_POINT('Ctrl Pts',(-43.3803394900793,31.1784722137567,
-40.5252598906186));
#255610=CARTESIAN_POINT('Ctrl Pts',(-43.3780514709974,31.2069533499868,
-40.5377524690855));
#255611=CARTESIAN_POINT('Ctrl Pts',(-43.3764764291988,31.2353806198054,
-40.5505518795279));
#255612=CARTESIAN_POINT('Ctrl Pts',(-43.3761228002374,31.292003207243,-40.577339198747));
#255613=CARTESIAN_POINT('Ctrl Pts',(-43.3798904844517,31.3482922086547,
-40.6058744004623));
#255614=CARTESIAN_POINT('Ctrl Pts',(-43.3877424304871,31.4042485256067,
-40.6361260433691));
#255615=CARTESIAN_POINT('Ctrl Pts',(-43.393042276717,31.4321193306868,-40.6518290622461));
#255616=CARTESIAN_POINT('Ctrl Pts',(-43.3990345440792,31.4599262492628,
-40.6678171709904));
#255617=CARTESIAN_POINT('Ctrl Pts',(-43.4023871385948,31.4738288295879,
-40.6759732487162));
#255618=CARTESIAN_POINT('Ctrl Pts',(-43.4097262599636,31.5013102698765,
-40.6924188649606));
#255619=CARTESIAN_POINT('Ctrl Pts',(-43.4137223958007,31.5149386860624,
-40.7007364096885));
#255620=CARTESIAN_POINT('Ctrl Pts',(-43.4266697743275,31.5554481319482,
-40.7259437634106));
#255621=CARTESIAN_POINT('Ctrl Pts',(-43.4365815013438,31.5819735775504,
-40.743098588818));
#255622=CARTESIAN_POINT('Ctrl Pts',(-43.453362100664,31.6210434116697,-40.7693485791028));
#255623=CARTESIAN_POINT('Ctrl Pts',(-43.4592720436944,31.6339404199602,
-40.77818065559));
#255624=CARTESIAN_POINT('Ctrl Pts',(-43.471748387858,31.6595177912398,-40.7960360397975));
#255625=CARTESIAN_POINT('Ctrl Pts',(-43.4782913690647,31.6721475181291,
-40.8050245716083));
#255626=CARTESIAN_POINT('Ctrl Pts',(-43.4987158872668,31.7093568101663,
-40.832021101787));
#255627=CARTESIAN_POINT('Ctrl Pts',(-43.5134312848982,31.7333600460206,
-40.8501267844669));
#255628=CARTESIAN_POINT('Ctrl Pts',(-43.5449969636312,31.7797747067972,
-40.8865288544817));
#255629=CARTESIAN_POINT('Ctrl Pts',(-43.570273480101,31.8133992725601,-40.9139774903764));
#255630=CARTESIAN_POINT('Ctrl Pts',(-43.6071874842548,31.8558549470217,
-40.9508682927202));
#255631=CARTESIAN_POINT('Ctrl Pts',(-43.6267265436653,31.8762775041081,
-40.9694100075909));
#255632=CARTESIAN_POINT('Ctrl Pts',(-43.6468212761471,31.8962967826001,
-40.9880061403947));
#255633=CARTESIAN_POINT('Ctrl Pts',(-43.6571524242715,31.9061057307006,
-40.997334528722));
#255634=CARTESIAN_POINT('Ctrl Pts',(-43.6781351765956,31.9250932263188,
-41.0158316653051));
#255635=CARTESIAN_POINT('Ctrl Pts',(-43.6888325213991,31.9343181422645,
-41.0250431278314));
#255636=CARTESIAN_POINT('Ctrl Pts',(-43.7214683281725,31.961133026229,-41.0525078158304));
#255637=CARTESIAN_POINT('Ctrl Pts',(-43.744000771517,31.977916302359,-41.070639272709));
#255638=CARTESIAN_POINT('Ctrl Pts',(-43.7905699795511,32.0092811177654,
-41.106520902203));
#255639=CARTESIAN_POINT('Ctrl Pts',(-43.8266341229871,32.0311632771839,
-41.1331548827895));
#255640=CARTESIAN_POINT('Ctrl Pts',(-43.8644344365312,32.050527928199,-41.1593656410909));
#255641=CARTESIAN_POINT('Ctrl Pts',(-43.8900335656271,32.0628690313763,
-41.1767476889401));
#255642=CARTESIAN_POINT('Ctrl Pts',(-43.903042008964,32.0687560539784,-41.1853974312384));
#255643=CARTESIAN_POINT('Ctrl Pts',(-43.9291618902095,32.0798229381751,
-41.2024070088898));
#255644=CARTESIAN_POINT('Ctrl Pts',(-43.9423286751247,32.0850301956599,
-41.2108047653586));
#255645=CARTESIAN_POINT('Ctrl Pts',(-43.9688389276373,32.0947834481969,
-41.2273662374836));
#255646=CARTESIAN_POINT('Ctrl Pts',(-44.0088868242005,32.1084293286422,
-41.2518690158044));
#255647=CARTESIAN_POINT('Ctrl Pts',(-44.0634057706764,32.1227159830699,
-41.2831968728749));
#255648=CARTESIAN_POINT('Ctrl Pts',(-44.1051448739617,32.1304686073096,
-41.30568419746));
#255649=CARTESIAN_POINT('Ctrl Pts',(-44.1331632182567,32.1349666221674,
-41.3204486001008));
#255650=CARTESIAN_POINT('Ctrl Pts',(-44.1472622735965,32.1368798783668,
-41.3277141420552));
#255651=CARTESIAN_POINT('Ctrl Pts',(-44.1685768983456,32.1392377391899,
-41.3384485067576));
#255652=CARTESIAN_POINT('Ctrl Pts',(-44.1757038998442,32.1399371964,-41.3419962566417));
#255653=CARTESIAN_POINT('Ctrl Pts',(-44.1899298892594,32.1411565650423,
-41.3489954369734));
#255654=CARTESIAN_POINT('Ctrl Pts',(-44.1970429564213,32.1416781032566,
-41.3524539903966));
#255655=CARTESIAN_POINT('Ctrl Pts',(-44.2183581262916,32.1429776302475,
-41.3626954949199));
#255656=CARTESIAN_POINT('Ctrl Pts',(-44.232556678806,32.1434929542666,-41.3693546778539));
#255657=CARTESIAN_POINT('Ctrl Pts',(-44.2750884056492,32.1439936324359,
-41.3888189062651));
#255658=CARTESIAN_POINT('Ctrl Pts',(-44.3033804172497,32.1429384256622,
-41.4011231160504));
#255659=CARTESIAN_POINT('Ctrl Pts',(-44.3598247343314,32.13804594572,-41.4243882373187));
#255660=CARTESIAN_POINT('Ctrl Pts',(-44.3879848006206,32.1342064546963,
-41.4353516241949));
#255661=CARTESIAN_POINT('Ctrl Pts',(-44.4230841862873,32.1276226980045,
-41.4481948195873));
#255662=CARTESIAN_POINT('Ctrl Pts',(-44.4301039616143,32.126214419323,-41.4507215814638));
#255663=CARTESIAN_POINT('Ctrl Pts',(-44.4441256434231,32.1232190082407,
-41.455685422358));
#255664=CARTESIAN_POINT('Ctrl Pts',(-44.4511413829898,32.1216281453652,
-41.4581270453932));
#255665=CARTESIAN_POINT('Ctrl Pts',(-44.472106554004,32.1165956901708,-41.4652964871519));
#255666=CARTESIAN_POINT('Ctrl Pts',(-44.4859328208737,32.1129061786889,
-41.4698557698741));
#255667=CARTESIAN_POINT('Ctrl Pts',(-44.5270324780087,32.1008340938932,
-41.4829067838587));
#255668=CARTESIAN_POINT('Ctrl Pts',(-44.5673316800757,32.08677017453,-41.4946921125766));
#255669=CARTESIAN_POINT('Ctrl Pts',(-44.6194780799712,32.0640738471498,
-41.5079096337926));
#255670=CARTESIAN_POINT('Ctrl Pts',(-44.6577884739158,32.045065905176,-41.5165678887371));
#255671=CARTESIAN_POINT('Ctrl Pts',(-44.6827916371924,32.031050813041,-41.5214942665077));
#255672=CARTESIAN_POINT('Ctrl Pts',(-44.7075150580676,32.0163554529027,
-41.5259894017533));
#255673=CARTESIAN_POINT('Ctrl Pts',(-44.7197631353705,32.0086467826241,
-41.5280237577537));
#255674=CARTESIAN_POINT('Ctrl Pts',(-44.7436779765282,31.9927322821733,
-41.5316086326721));
#255675=CARTESIAN_POINT('Ctrl Pts',(-44.7554039451266,31.9844926239501,
-41.5331705278033));
#255676=CARTESIAN_POINT('Ctrl Pts',(-44.7783650010144,31.9674779303508,
-41.5358342782831));
#255677=CARTESIAN_POINT('Ctrl Pts',(-44.8120876763637,31.941142023486,-41.5391427937509));
#255678=CARTESIAN_POINT('Ctrl Pts',(-44.8542060542843,31.9028069711657,
-41.5408368316843));
#255679=CARTESIAN_POINT('Ctrl Pts',(-44.883650374082,31.8716290815775,-41.5400605624154));
#255680=CARTESIAN_POINT('Ctrl Pts',(-44.9027957424029,31.8502960261458,
-41.5390808606534));
#255681=CARTESIAN_POINT('Ctrl Pts',(-44.912124025092,31.8393588588263,-41.5383603441012));
#255682=CARTESIAN_POINT('Ctrl Pts',(-44.9302963003321,31.816913187918,-41.5364463589967));
#255683=CARTESIAN_POINT('Ctrl Pts',(-44.9390653236876,31.8054960967264,
-41.5352602514373));
#255684=CARTESIAN_POINT('Ctrl Pts',(-44.9559494861592,31.7823260274566,
-41.532444286592));
#255685=CARTESIAN_POINT('Ctrl Pts',(-44.9803129684955,31.7470436123751,
-41.5275522735743));
#255686=CARTESIAN_POINT('Ctrl Pts',(-45.00183725318,31.7102129370948,-41.5206914933375));
#255687=CARTESIAN_POINT('Ctrl Pts',(-45.0280427451288,31.6597446570548,
-41.5098099510806));
#255688=CARTESIAN_POINT('Ctrl Pts',(-45.0398987329805,31.6338241168053,
-41.5034995556801));
#255689=CARTESIAN_POINT('Ctrl Pts',(-45.0531290598229,31.6005723463994,
-41.4945098705711));
#255690=CARTESIAN_POINT('Ctrl Pts',(-45.0556963147994,31.5938738844661,
-41.4926546478805));
#255691=CARTESIAN_POINT('Ctrl Pts',(-45.0606676096559,31.5803990532317,
-41.4888352403062));
#255692=CARTESIAN_POINT('Ctrl Pts',(-45.0630762139805,31.5736079348959,
-41.4868664774371));
#255693=CARTESIAN_POINT('Ctrl Pts',(-45.0700329505347,31.5531765604049,
-41.4808121016924));
#255694=CARTESIAN_POINT('Ctrl Pts',(-45.0743018132827,31.5395152309552,
-41.4765904297482));
#255695=CARTESIAN_POINT('Ctrl Pts',(-45.0860497029301,31.4983488303989,
-41.4633620161014));
#255696=CARTESIAN_POINT('Ctrl Pts',(-45.0988767040151,31.4430340104486,
-41.4442426901641));
#255697=CARTESIAN_POINT('Ctrl Pts',(-45.1061818129997,31.386882792419,-41.4222207481485));
#255698=CARTESIAN_POINT('Ctrl Pts',(-45.1095857869151,31.3444641027996,
-41.4046111316328));
#255699=CARTESIAN_POINT('Ctrl Pts',(-45.1103739871937,31.3302675876129,
-41.3985560195248));
#255700=CARTESIAN_POINT('Ctrl Pts',(-45.1110306052012,31.30890259785,-41.3891987399731));
#255701=CARTESIAN_POINT('Ctrl Pts',(-45.1111617199316,31.3017636946428,
-41.3860313075819));
#255702=CARTESIAN_POINT('Ctrl Pts',(-45.1112472734604,31.2874686716035,
-41.3796068875509));
#255703=CARTESIAN_POINT('Ctrl Pts',(-45.111201351958,31.2802974166487,-41.3763428889219));
#255704=CARTESIAN_POINT('Ctrl Pts',(-45.1107973541963,31.25882908612,-41.3664479958234));
#255705=CARTESIAN_POINT('Ctrl Pts',(-45.11017580813,31.2446005169708,-41.3597259135069));
#255706=CARTESIAN_POINT('Ctrl Pts',(-45.1082442962718,31.2162677536902,
-41.3460176286356));
#255707=CARTESIAN_POINT('Ctrl Pts',(-45.104314463686,31.1739750543259,-41.3250680443717));
#255708=CARTESIAN_POINT('Ctrl Pts',(-45.0950241996196,31.1183949914011,
-41.295609869938));
#255709=CARTESIAN_POINT('Ctrl Pts',(-45.0817381040079,31.0636149263882,
-41.264634106957));
#255710=CARTESIAN_POINT('Ctrl Pts',(-45.0737554763462,31.0364928582332,
-41.2486352837062));
#255711=CARTESIAN_POINT('Ctrl Pts',(-45.0650963255467,31.0095068957897,
-41.2323777508457));
#255712=CARTESIAN_POINT('Ctrl Pts',(-45.0604265398991,30.996076905732,-41.224116427314));
#255713=CARTESIAN_POINT('Ctrl Pts',(-45.0504049610752,30.9693743366894,
-41.2073411015006));
#255714=CARTESIAN_POINT('Ctrl Pts',(-45.0450945767524,30.9562107421528,
-41.1988958018751));
#255715=CARTESIAN_POINT('Ctrl Pts',(-45.0394875320819,30.9432190801919,
-41.190386719266));
#255716=CARTESIAN_POINT('',(-42.6662672096693,32.3203213022045,-39.2608974781454));
#255717=CARTESIAN_POINT('',(-42.7562642394046,32.238293307241,-39.4336017780241));
#255718=CARTESIAN_POINT('',(-42.6662672096693,32.3203213022045,-39.2608974781454));
#255719=CARTESIAN_POINT('Origin',(-44.4753294917431,31.5614417668058,-39.4557296694497));
#255720=CARTESIAN_POINT('Ctrl Pts',(-43.0434008892766,32.902468814613,-39.4567761948493));
#255721=CARTESIAN_POINT('Ctrl Pts',(-42.9769841821306,32.8009549221958,
-39.4517406334174));
#255722=CARTESIAN_POINT('Ctrl Pts',(-42.919362741941,32.6938935737936,-39.4472380210389));
#255723=CARTESIAN_POINT('Ctrl Pts',(-42.8231628417698,32.4713594324972,
-39.4394681758366));
#255724=CARTESIAN_POINT('Ctrl Pts',(-42.7846681593587,32.3561866606744,
-39.4362084259695));
#255725=CARTESIAN_POINT('Ctrl Pts',(-42.7562642394046,32.2382933072411,
-39.4336017780242));
#255726=CARTESIAN_POINT('Ctrl Pts',(-42.4577131944625,32.5104083279569,
-38.8606823233882));
#255727=CARTESIAN_POINT('Ctrl Pts',(-42.4722685042022,32.5448307979214,
-38.8694323201496));
#255728=CARTESIAN_POINT('Ctrl Pts',(-42.4876674804305,32.5789105800709,
-38.8782643966372));
#255729=CARTESIAN_POINT('Ctrl Pts',(-42.5202146590728,32.6464795812123,
-38.8961197808447));
#255730=CARTESIAN_POINT('Ctrl Pts',(-42.5373018269229,32.6798350022668,
-38.9051083126545));
#255731=CARTESIAN_POINT('Ctrl Pts',(-42.5906929412925,32.7780783962456,
-38.9321048428364));
#255732=CARTESIAN_POINT('Ctrl Pts',(-42.629225789877,32.8414173722334,-38.9502105255134));
#255733=CARTESIAN_POINT('Ctrl Pts',(-42.7120000069194,32.9638220552461,
-38.9866125955295));
#255734=CARTESIAN_POINT('Ctrl Pts',(-42.7562439327448,33.0229003355902,
-39.0049117194725));
#255735=CARTESIAN_POINT('Ctrl Pts',(-42.8269002201102,33.1083282766067,
-39.0325063049612));
#255736=CARTESIAN_POINT('Ctrl Pts',(-42.851168481378,33.1362718559733,-39.0417288667405));
#255737=CARTESIAN_POINT('Ctrl Pts',(-42.9011535535061,33.1910821810744,
-39.0602232021637));
#255738=CARTESIAN_POINT('Ctrl Pts',(-42.9268673384213,33.2179450225078,
-39.0694937486382));
#255739=CARTESIAN_POINT('Ctrl Pts',(-42.9797817061917,33.2705900457306,
-39.088089881442));
#255740=CARTESIAN_POINT('Ctrl Pts',(-43.0069972096607,33.2963736994337,
-39.097418269769));
#255741=CARTESIAN_POINT('Ctrl Pts',(-43.0622936398443,33.3462615369725,
-39.1159154063528));
#255742=CARTESIAN_POINT('Ctrl Pts',(-43.0904949946047,33.3704876748183,
-39.1251268688782));
#255743=CARTESIAN_POINT('Ctrl Pts',(-43.176562606447,33.4408730143711,-39.1525915568785));
#255744=CARTESIAN_POINT('Ctrl Pts',(-43.2360245534179,33.4848790444095,
-39.1707230137558));
#255745=CARTESIAN_POINT('Ctrl Pts',(-43.3282503301662,33.5464830068215,
-39.1976342358769));
#255746=CARTESIAN_POINT('Ctrl Pts',(-43.3595022265301,33.5662859367769,
-39.2065582055264));
#255747=CARTESIAN_POINT('Ctrl Pts',(-43.423032399699,33.604418869649,-39.2243132114598));
#255748=CARTESIAN_POINT('Ctrl Pts',(-43.4553106319894,33.6227489368786,
-39.2331442507783));
#255749=CARTESIAN_POINT('Ctrl Pts',(-43.5209070247133,33.6579164232732,
-39.2507127863664));
#255750=CARTESIAN_POINT('Ctrl Pts',(-43.5542222374601,33.6747516510336,
-39.2594493821381));
#255751=CARTESIAN_POINT('Ctrl Pts',(-43.6219256430316,33.7069073870392,
-39.2768314299875));
#255752=CARTESIAN_POINT('Ctrl Pts',(-43.6563381479934,33.7222286468184,
-39.2854811722856));
#255753=CARTESIAN_POINT('Ctrl Pts',(-43.7254519170511,33.7509934760634,
-39.3024907499371));
#255754=CARTESIAN_POINT('Ctrl Pts',(-43.7602995448845,33.7645084608315,
-39.3108885064059));
#255755=CARTESIAN_POINT('Ctrl Pts',(-43.8304781084082,33.789780836939,-39.3274499785309));
#255756=CARTESIAN_POINT('Ctrl Pts',(-43.8658243285985,33.8015455603985,
-39.3356176307442));
#255757=CARTESIAN_POINT('Ctrl Pts',(-43.9726293607703,33.8342393174696,
-39.3597845530997));
#255758=CARTESIAN_POINT('Ctrl Pts',(-44.0448528416425,33.8525737420732,
-39.3754485022349));
#255759=CARTESIAN_POINT('Ctrl Pts',(-44.1547335161489,33.874826743562,-39.3982722291653));
#255760=CARTESIAN_POINT('Ctrl Pts',(-44.1916183723467,33.8813683146414,
-39.4057679385072));
#255761=CARTESIAN_POINT('Ctrl Pts',(-44.2659122959158,33.8926702964892,
-39.4205323411483));
#255762=CARTESIAN_POINT('Ctrl Pts',(-44.3033049221432,33.8974288658374,
-39.4277978831022));
#255763=CARTESIAN_POINT('Ctrl Pts',(-44.3598453576919,33.9032050944765,
-39.4385322478049));
#255764=CARTESIAN_POINT('Ctrl Pts',(-44.3787527158677,33.9049006163346,
-39.4420799976889));
#255765=CARTESIAN_POINT('Ctrl Pts',(-44.4164967874688,33.9078161173588,
-39.4490791780208));
#255766=CARTESIAN_POINT('Ctrl Pts',(-44.4353708468856,33.9090400957878,
-39.4525377314439));
#255767=CARTESIAN_POINT('Ctrl Pts',(-44.4919347179527,33.9120095261766,
-39.462779235967));
#255768=CARTESIAN_POINT('Ctrl Pts',(-44.52962054914,33.9130584408517,-39.4694384189012));
#255769=CARTESIAN_POINT('Ctrl Pts',(-44.6425299001817,33.9134342925821,
-39.4889026473125));
#255770=CARTESIAN_POINT('Ctrl Pts',(-44.7176656228988,33.9100023852834,
-39.5012068570978));
#255771=CARTESIAN_POINT('Ctrl Pts',(-44.867623327666,33.8957625538083,-39.524471978366));
#255772=CARTESIAN_POINT('Ctrl Pts',(-44.9424659600731,33.8849485744664,
-39.5354353652432));
#255773=CARTESIAN_POINT('Ctrl Pts',(-45.0357885152669,33.8666999843662,
-39.5482785606344));
#255774=CARTESIAN_POINT('Ctrl Pts',(-45.0544546343785,33.8628074782943,
-39.5508053225112));
#255775=CARTESIAN_POINT('Ctrl Pts',(-45.0917431025751,33.8545484160302,
-39.5557691634051));
#255776=CARTESIAN_POINT('Ctrl Pts',(-45.1104022544846,33.8501716550149,
-39.5582107864407));
#255777=CARTESIAN_POINT('Ctrl Pts',(-45.1661672125598,33.8363538303533,
-39.565380228199));
#255778=CARTESIAN_POINT('Ctrl Pts',(-45.2029511118778,33.8262578362557,
-39.5699395109212));
#255779=CARTESIAN_POINT('Ctrl Pts',(-45.2758615915212,33.8042965707928,
-39.578640186911));
#255780=CARTESIAN_POINT('Ctrl Pts',(-45.3119687135373,33.792436319941,-39.5827791123973));
#255781=CARTESIAN_POINT('Ctrl Pts',(-45.3834929078587,33.7669724252328,
-39.5906388675035));
#255782=CARTESIAN_POINT('Ctrl Pts',(-45.4189099726225,33.753368762151,-39.59435969177));
#255783=CARTESIAN_POINT('Ctrl Pts',(-45.4890551197469,33.7244209300036,
-39.6013847808703));
#255784=CARTESIAN_POINT('Ctrl Pts',(-45.5237832050323,33.7090767682036,
-39.60468904687));
#255785=CARTESIAN_POINT('Ctrl Pts',(-45.5925464188782,33.6766380670054,
-39.6108794240926));
#255786=CARTESIAN_POINT('Ctrl Pts',(-45.6265815610841,33.6595435620003,
-39.6137655431243));
#255787=CARTESIAN_POINT('Ctrl Pts',(-45.6939497262655,33.6235811757592,
-39.6191148199286));
#255788=CARTESIAN_POINT('Ctrl Pts',(-45.7272860947277,33.6047101271221,
-39.6215780075552));
#255789=CARTESIAN_POINT('Ctrl Pts',(-45.7932287365117,33.5651705839516,
-39.6260731428005));
#255790=CARTESIAN_POINT('Ctrl Pts',(-45.8259059249178,33.5444453395394,
-39.6281074988012));
#255791=CARTESIAN_POINT('Ctrl Pts',(-45.8897275017006,33.5016881508368,
-39.6316923737189));
#255792=CARTESIAN_POINT('Ctrl Pts',(-45.9210297733036,33.4795651380847,
-39.6332542688506));
#255793=CARTESIAN_POINT('Ctrl Pts',(-45.9823424846244,33.4339088874735,
-39.6359180193303));
#255794=CARTESIAN_POINT('Ctrl Pts',(-46.0123687620003,33.4103663679687,
-39.6370209899198));
#255795=CARTESIAN_POINT('Ctrl Pts',(-46.1005740569048,33.337614535667,-39.639649668426));
#255796=CARTESIAN_POINT('Ctrl Pts',(-46.1568837651934,33.2862857446323,
-39.6404967282823));
#255797=CARTESIAN_POINT('Ctrl Pts',(-46.2375893041651,33.2050303462875,
-39.6404032087595));
#255798=CARTESIAN_POINT('Ctrl Pts',(-46.2638636333332,33.1772336958076,
-39.6401443034625));
#255799=CARTESIAN_POINT('Ctrl Pts',(-46.3151397511292,33.1201974856456,
-39.6391646017005));
#255800=CARTESIAN_POINT('Ctrl Pts',(-46.3401349353408,33.0909661742941,
-39.6384440851485));
#255801=CARTESIAN_POINT('Ctrl Pts',(-46.3888523044997,33.0309971480077,
-39.6365301000439));
#255802=CARTESIAN_POINT('Ctrl Pts',(-46.4123735341802,33.0005036828642,
-39.6353439924849));
#255803=CARTESIAN_POINT('Ctrl Pts',(-46.4576879006691,32.9386388625828,
-39.6325280276392));
#255804=CARTESIAN_POINT('Ctrl Pts',(-46.4794979867991,32.9072463828166,
-39.6308974590955));
#255805=CARTESIAN_POINT('Ctrl Pts',(-46.5424231451674,32.8117200287728,
-39.625348882952));
#255806=CARTESIAN_POINT('Ctrl Pts',(-46.5810426872604,32.7462345994881,
-39.6207752343847));
#255807=CARTESIAN_POINT('Ctrl Pts',(-46.6516918187306,32.6117039458857,
-39.6098936921283));
#255808=CARTESIAN_POINT('Ctrl Pts',(-46.683723185051,32.5426422373878,-39.6035832967262));
#255809=CARTESIAN_POINT('Ctrl Pts',(-46.7195635412788,32.4540883209462,
-39.5945936116187));
#255810=CARTESIAN_POINT('Ctrl Pts',(-46.726523577584,32.4362514419463,-39.5927383889277));
#255811=CARTESIAN_POINT('Ctrl Pts',(-46.7400123459627,32.4003742100513,
-39.5889189813535));
#255812=CARTESIAN_POINT('Ctrl Pts',(-46.7465535157541,32.3822946053341,
-39.5869502184844));
#255813=CARTESIAN_POINT('Ctrl Pts',(-46.7654644360989,32.3279072933141,
-39.5808958427402));
#255814=CARTESIAN_POINT('Ctrl Pts',(-46.7770937339888,32.2915493874552,
-39.5766741707955));
#255815=CARTESIAN_POINT('Ctrl Pts',(-46.7984826125902,32.218525216591,-39.5678552283644));
#255816=CARTESIAN_POINT('Ctrl Pts',(-46.8082356969316,32.1818782626467,
-39.5632601453561));
#255817=CARTESIAN_POINT('Ctrl Pts',(-46.825891612219,32.1083194036329,-39.5537041764669));
#255818=CARTESIAN_POINT('Ctrl Pts',(-46.8337943341285,32.0714074828253,
-39.5487432700414));
#255819=CARTESIAN_POINT('Ctrl Pts',(-46.8547548417649,31.9602784784655,
-39.5333157914925));
#255820=CARTESIAN_POINT('Ctrl Pts',(-46.8650708643863,31.8856621776612,
-39.5223044891954));
#255821=CARTESIAN_POINT('Ctrl Pts',(-46.8750487417844,31.7729724844591,
-39.50469487268));
#255822=CARTESIAN_POINT('Ctrl Pts',(-46.8774570362353,31.7352651712118,
-39.4986397605722));
#255823=CARTESIAN_POINT('Ctrl Pts',(-46.8796767940079,31.6785286095959,
-39.4892824810203));
#255824=CARTESIAN_POINT('Ctrl Pts',(-46.8801843407089,31.6595724593507,
-39.4861150486293));
#255825=CARTESIAN_POINT('Ctrl Pts',(-46.8807312344333,31.6216180949417,
-39.479690628598));
#255826=CARTESIAN_POINT('Ctrl Pts',(-46.8807699646674,31.6025797052015,
-39.4764266299692));
#255827=CARTESIAN_POINT('Ctrl Pts',(-46.8801790388754,31.5455906639181,
-39.4665317368708));
#255828=CARTESIAN_POINT('Ctrl Pts',(-46.8788490796135,31.5078273383739,
-39.4598096545541));
#255829=CARTESIAN_POINT('Ctrl Pts',(-46.874360617844,31.4326451774337,-39.4461013696832));
#255830=CARTESIAN_POINT('Ctrl Pts',(-46.8712024719357,31.3952438451296,
-39.4391182381771));
#255831=CARTESIAN_POINT('Ctrl Pts',(-46.859034870425,31.2835993575687,-39.4177870553822));
#255832=CARTESIAN_POINT('Ctrl Pts',(-46.8473376289695,31.2099145948488,
-39.4030579748028));
#255833=CARTESIAN_POINT('Ctrl Pts',(-46.8244863951756,31.1004910081606,
-39.3802058074804));
#255834=CARTESIAN_POINT('Ctrl Pts',(-46.8159835780379,31.0642007181804,
-39.3724617858671));
#255835=CARTESIAN_POINT('Ctrl Pts',(-46.7971994280146,30.9919902987916,
-39.3567184383004));
#255836=CARTESIAN_POINT('Ctrl Pts',(-46.7869180083019,30.9560697433081,
-39.3487190247537));
#255837=CARTESIAN_POINT('Ctrl Pts',(-46.7645577771926,30.884604709384,-39.332461491893));
#255838=CARTESIAN_POINT('Ctrl Pts',(-46.7524740339114,30.8490466969583,
-39.3242001683612));
#255839=CARTESIAN_POINT('Ctrl Pts',(-46.7264943673172,30.778363271582,-39.3074248425479));
#255840=CARTESIAN_POINT('Ctrl Pts',(-46.7127058212706,30.7435263372096,
-39.2989795429224));
#255841=CARTESIAN_POINT('Ctrl Pts',(-46.6981266849492,30.7091523375488,
-39.2904704603133));
#255842=CARTESIAN_POINT('Ctrl Pts',(-42.6662678860477,32.3203206857175,
-39.2608987761157));
#255843=CARTESIAN_POINT('Ctrl Pts',(-42.678935401819,32.3502354261213,-39.2696487728771));
#255844=CARTESIAN_POINT('Ctrl Pts',(-42.6923355177353,32.3798530670723,
-39.2784808493646));
#255845=CARTESIAN_POINT('Ctrl Pts',(-42.7206547846785,32.4385765514345,
-39.2963362335721));
#255846=CARTESIAN_POINT('Ctrl Pts',(-42.7355208246471,32.4675661149098,
-39.3053247653821));
#255847=CARTESIAN_POINT('Ctrl Pts',(-42.7819675412757,32.5529527044587,
-39.3323212955634));
#255848=CARTESIAN_POINT('Ctrl Pts',(-42.8154832551899,32.6080056255704,
-39.350426978241));
#255849=CARTESIAN_POINT('Ctrl Pts',(-42.8874704180899,32.7144030466848,
-39.3868290482568));
#255850=CARTESIAN_POINT('Ctrl Pts',(-42.9259440972401,32.7657584717183,
-39.4051281722));
#255851=CARTESIAN_POINT('Ctrl Pts',(-42.9873793042677,32.8400236828058,
-39.4327227576885));
#255852=CARTESIAN_POINT('Ctrl Pts',(-43.0084794421579,32.864316719619,-39.4419453194678));
#255853=CARTESIAN_POINT('Ctrl Pts',(-43.0519372785408,32.9119682754171,
-39.4604396548911));
#255854=CARTESIAN_POINT('Ctrl Pts',(-43.0742923458191,32.9353234004109,
-39.4697102013656));
#255855=CARTESIAN_POINT('Ctrl Pts',(-43.1202932730876,32.9810958260852,
-39.4883063341693));
#255856=CARTESIAN_POINT('Ctrl Pts',(-43.1439520951656,33.0035144156811,
-39.4976347224965));
#255857=CARTESIAN_POINT('Ctrl Pts',(-43.1920203654931,33.0468931109494,
-39.5161318590801));
#255858=CARTESIAN_POINT('Ctrl Pts',(-43.2165345089143,33.0679592485651,
-39.5253433216058));
#255859=CARTESIAN_POINT('Ctrl Pts',(-43.2913467365328,33.1291664924534,
-39.5528080096058));
#255860=CARTESIAN_POINT('Ctrl Pts',(-43.3430295011989,33.16743806238,-39.5709394664834));
#255861=CARTESIAN_POINT('Ctrl Pts',(-43.42318529819,33.2210204170675,-39.5978506886043));
#255862=CARTESIAN_POINT('Ctrl Pts',(-43.4503464116134,33.2382458390107,
-39.6067746582539));
#255863=CARTESIAN_POINT('Ctrl Pts',(-43.5055592644833,33.2714177212331,
-39.6245296641872));
#255864=CARTESIAN_POINT('Ctrl Pts',(-43.5336109652927,33.2873642373592,
-39.6333607035057));
#255865=CARTESIAN_POINT('Ctrl Pts',(-43.5906167586109,33.3179611793576,
-39.6509292390937));
#255866=CARTESIAN_POINT('Ctrl Pts',(-43.6195682890663,33.3326096993947,
-39.6596658348655));
#255867=CARTESIAN_POINT('Ctrl Pts',(-43.6784024489033,33.3605914924566,
-39.6770478827149));
#255868=CARTESIAN_POINT('Ctrl Pts',(-43.7083061985044,33.3739254346794,
-39.685697625013));
#255869=CARTESIAN_POINT('Ctrl Pts',(-43.7683633256242,33.3989622002509,
-39.7027072026645));
#255870=CARTESIAN_POINT('Ctrl Pts',(-43.7986438942497,33.4107271662336,
-39.7111049591333));
#255871=CARTESIAN_POINT('Ctrl Pts',(-43.8596237489107,33.4327304463716,
-39.7276664312583));
#255872=CARTESIAN_POINT('Ctrl Pts',(-43.8903363171894,33.4429751408118,
-39.7358340834717));
#255873=CARTESIAN_POINT('Ctrl Pts',(-43.9831381063675,33.4714505290734,
-39.7600010058271));
#255874=CARTESIAN_POINT('Ctrl Pts',(-44.045889936343,33.4874275689807,-39.7756649549624));
#255875=CARTESIAN_POINT('Ctrl Pts',(-44.1413569064837,33.5068342142111,
-39.7984886818927));
#255876=CARTESIAN_POINT('Ctrl Pts',(-44.1734027712035,33.5125421273567,
-39.8059843912346));
#255877=CARTESIAN_POINT('Ctrl Pts',(-44.2379487660953,33.522410856807,-39.8207487938757));
#255878=CARTESIAN_POINT('Ctrl Pts',(-44.2704346127381,33.5265700622991,
-39.8280143358296));
#255879=CARTESIAN_POINT('Ctrl Pts',(-44.3195547480624,33.53162621339,-39.8387487005323));
#255880=CARTESIAN_POINT('Ctrl Pts',(-44.3359805797293,33.5331119147056,
-39.8422964504163));
#255881=CARTESIAN_POINT('Ctrl Pts',(-44.368770578548,33.5356701262535,-39.8492956307481));
#255882=CARTESIAN_POINT('Ctrl Pts',(-44.3851671905622,33.5367461359866,
-39.8527541841713));
#255883=CARTESIAN_POINT('Ctrl Pts',(-44.4343059395537,33.5393638020221,
-39.8629956886945));
#255884=CARTESIAN_POINT('Ctrl Pts',(-44.4670441867038,33.5403003160803,
-39.8696548716286));
#255885=CARTESIAN_POINT('Ctrl Pts',(-44.5651285248139,33.5407024624404,
-39.8891191000399));
#255886=CARTESIAN_POINT('Ctrl Pts',(-44.6303966421524,33.5377712059725,
-39.9014233098251));
#255887=CARTESIAN_POINT('Ctrl Pts',(-44.7606557964568,33.5255003896343,
-39.9246884310934));
#255888=CARTESIAN_POINT('Ctrl Pts',(-44.8256647686024,33.5161555829264,
-39.9356518179704));
#255889=CARTESIAN_POINT('Ctrl Pts',(-44.9067226409372,33.5003641844135,
-39.9484950133618));
#255890=CARTESIAN_POINT('Ctrl Pts',(-44.9229354632917,33.4969949796552,
-39.9510217752386));
#255891=CARTESIAN_POINT('Ctrl Pts',(-44.9553227940458,33.4898447029991,
-39.9559856161326));
#255892=CARTESIAN_POINT('Ctrl Pts',(-44.971529266705,33.4860547900967,-39.958427239168));
#255893=CARTESIAN_POINT('Ctrl Pts',(-45.019963666253,33.4740875993182,-39.9655966809264));
#255894=CARTESIAN_POINT('Ctrl Pts',(-45.0519115512582,33.4653411277245,
-39.9701559636487));
#255895=CARTESIAN_POINT('Ctrl Pts',(-45.1152352219466,33.4463106730797,
-39.9788566396385));
#255896=CARTESIAN_POINT('Ctrl Pts',(-45.1465941073248,33.436031038673,-39.9829955651248));
#255897=CARTESIAN_POINT('Ctrl Pts',(-45.2087113592473,33.4139567327306,
-39.9908553202309));
#255898=CARTESIAN_POINT('Ctrl Pts',(-45.2394697192292,33.4021620444808,
-39.9945761444974));
#255899=CARTESIAN_POINT('Ctrl Pts',(-45.3003868460925,33.3770601489593,
-40.0016012335977));
#255900=CARTESIAN_POINT('Ctrl Pts',(-45.3305456155218,33.3637529479941,
-40.0049054995974));
#255901=CARTESIAN_POINT('Ctrl Pts',(-45.3902600985989,33.3356174580523,
-40.01109587682));
#255902=CARTESIAN_POINT('Ctrl Pts',(-45.4198158241265,33.3207891989555,
-40.0139819958517));
#255903=CARTESIAN_POINT('Ctrl Pts',(-45.4783162406983,33.289591616671,-40.0193312726561));
#255904=CARTESIAN_POINT('Ctrl Pts',(-45.5072638360001,33.2732195440424,
-40.0217944602826));
#255905=CARTESIAN_POINT('Ctrl Pts',(-45.5645236685819,33.2389134161644,
-40.0262895955279));
#255906=CARTESIAN_POINT('Ctrl Pts',(-45.5928974744892,33.2209301068779,
-40.0283239515286));
#255907=CARTESIAN_POINT('Ctrl Pts',(-45.6483127164684,33.183827317638,-40.0319088264464));
#255908=CARTESIAN_POINT('Ctrl Pts',(-45.6754912491912,33.164628826888,-40.033470721578));
#255909=CARTESIAN_POINT('Ctrl Pts',(-45.7287252026082,33.1250059065848,
-40.0361344720577));
#255910=CARTESIAN_POINT('Ctrl Pts',(-45.7547943757217,33.1045734241173,
-40.0372374426473));
#255911=CARTESIAN_POINT('Ctrl Pts',(-45.8313729898423,33.0414293618193,
-40.0398661211534));
#255912=CARTESIAN_POINT('Ctrl Pts',(-45.8802572019016,32.996875335828,-40.0407131810096));
#255913=CARTESIAN_POINT('Ctrl Pts',(-45.9503152695219,32.9263392450608,
-40.0406196614869));
#255914=CARTESIAN_POINT('Ctrl Pts',(-45.9731223693318,32.9022087072537,
-40.04036075619));
#255915=CARTESIAN_POINT('Ctrl Pts',(-46.0176301600934,32.8526933495872,
-40.0393810544279));
#255916=CARTESIAN_POINT('Ctrl Pts',(-46.0393251189803,32.8273156909405,
-40.0386605378759));
#255917=CARTESIAN_POINT('Ctrl Pts',(-46.0816081786906,32.7752509415469,
-40.0367465527713));
#255918=CARTESIAN_POINT('Ctrl Pts',(-46.1020218631531,32.7487759054673,
-40.0355604452122));
#255919=CARTESIAN_POINT('Ctrl Pts',(-46.1413474207414,32.6950621160095,
-40.0327444803666));
#255920=CARTESIAN_POINT('Ctrl Pts',(-46.1602740044506,32.6678050222156,
-40.0311139118228));
#255921=CARTESIAN_POINT('Ctrl Pts',(-46.2148766161292,32.5848603625352,
-40.0255653356794));
#255922=CARTESIAN_POINT('Ctrl Pts',(-46.2483838166511,32.5279971310113,
-40.0209916871121));
#255923=CARTESIAN_POINT('Ctrl Pts',(-46.3096709166782,32.4111741762596,
-40.0101101448556));
#255924=CARTESIAN_POINT('Ctrl Pts',(-46.337452349158,32.351200134253,-40.0037997494539));
#255925=CARTESIAN_POINT('Ctrl Pts',(-46.3685299134922,32.2742955884667,
-39.9948100643461));
#255926=CARTESIAN_POINT('Ctrl Pts',(-46.3745646125082,32.2588050117033,
-39.9929548416551));
#255927=CARTESIAN_POINT('Ctrl Pts',(-46.3862591791565,32.2276468348101,
-39.9891354340809));
#255928=CARTESIAN_POINT('Ctrl Pts',(-46.3919298260057,32.2119451443588,
-39.9871666712118));
#255929=CARTESIAN_POINT('Ctrl Pts',(-46.4083226032432,32.1647106343652,
-39.9811122954676));
#255930=CARTESIAN_POINT('Ctrl Pts',(-46.418401428985,32.1331337514891,-39.9768906235228));
#255931=CARTESIAN_POINT('Ctrl Pts',(-46.4369345420855,32.0697109656014,
-39.9680716810918));
#255932=CARTESIAN_POINT('Ctrl Pts',(-46.4453831985413,32.0378818340676,
-39.9634765980836));
#255933=CARTESIAN_POINT('Ctrl Pts',(-46.4606729029267,31.9739922725109,
-39.9539206291942));
#255934=CARTESIAN_POINT('Ctrl Pts',(-46.4675138561323,31.9419318287439,
-39.9489597227689));
#255935=CARTESIAN_POINT('Ctrl Pts',(-46.4856493778314,31.8454072024775,
-39.9335322442199));
#255936=CARTESIAN_POINT('Ctrl Pts',(-46.4945617255914,31.78059453833,-39.9225209419229));
#255937=CARTESIAN_POINT('Ctrl Pts',(-46.50315481336,31.6827073984777,-39.9049113254075));
#255938=CARTESIAN_POINT('Ctrl Pts',(-46.5052218357471,31.6499526236153,
-39.8988562132996));
#255939=CARTESIAN_POINT('Ctrl Pts',(-46.5071123188746,31.6006670667202,
-39.8894989337477));
#255940=CARTESIAN_POINT('Ctrl Pts',(-46.5075405703607,31.5842002139207,
-39.8863315013567));
#255941=CARTESIAN_POINT('Ctrl Pts',(-46.5079902829931,31.5512296784738,
-39.8799070813255));
#255942=CARTESIAN_POINT('Ctrl Pts',(-46.5080111813793,31.5346910950095,
-39.8766430826966));
#255943=CARTESIAN_POINT('Ctrl Pts',(-46.5074596318877,31.4851844744852,
-39.8667481895982));
#255944=CARTESIAN_POINT('Ctrl Pts',(-46.5062788995272,31.4523787341376,
-39.8600261072815));
#255945=CARTESIAN_POINT('Ctrl Pts',(-46.5023290580356,31.3870653764436,
-39.8463178224105));
#255946=CARTESIAN_POINT('Ctrl Pts',(-46.4995602704424,31.3545729642139,
-39.8393346909045));
#255947=CARTESIAN_POINT('Ctrl Pts',(-46.4889145018408,31.2575800929905,
-39.8180035081097));
#255948=CARTESIAN_POINT('Ctrl Pts',(-46.4787027861653,31.1935630330159,
-39.8032744275302));
#255949=CARTESIAN_POINT('Ctrl Pts',(-46.4587767101283,31.0984927565591,
-39.7804222602078));
#255950=CARTESIAN_POINT('Ctrl Pts',(-46.4513652889539,31.0669621539425,
-39.7726782385945));
#255951=CARTESIAN_POINT('Ctrl Pts',(-46.4349975412466,31.0042213777813,
-39.7569348910278));
#255952=CARTESIAN_POINT('Ctrl Pts',(-46.4260411389904,30.9730108340646,
-39.7489354774811));
#255953=CARTESIAN_POINT('Ctrl Pts',(-46.4065670339061,30.9109152953089,
-39.7326779446204));
#255954=CARTESIAN_POINT('Ctrl Pts',(-46.3960450372602,30.8800185402287,
-39.7244166210886));
#255955=CARTESIAN_POINT('Ctrl Pts',(-46.3734269342347,30.8185996612379,
-39.7076412952753));
#255956=CARTESIAN_POINT('Ctrl Pts',(-46.3614243089069,30.7883282055528,
-39.6991959956498));
#255957=CARTESIAN_POINT('Ctrl Pts',(-46.3487351394075,30.7584583851184,
-39.6906869130407));
#255958=CARTESIAN_POINT('',(-42.4577131917459,32.5104083291869,-38.8606823230689));
#255959=CARTESIAN_POINT('',(-42.4577131944625,32.5104083279569,-38.8606823233882));
#255960=CARTESIAN_POINT('',(-46.6981266849484,30.7091523375492,-39.2904704603132));
#255961=CARTESIAN_POINT('Ctrl Pts',(-42.4577131904514,32.5104083297438,
-38.8606823230314));
#255962=CARTESIAN_POINT('Ctrl Pts',(-42.4722685042036,32.5448307979246,
-38.8694323201505));
#255963=CARTESIAN_POINT('Ctrl Pts',(-42.4876674804313,32.5789105800726,
-38.8782643966377));
#255964=CARTESIAN_POINT('Ctrl Pts',(-42.5202146590728,32.6464795812123,
-38.8961197808447));
#255965=CARTESIAN_POINT('Ctrl Pts',(-42.5373018269229,32.6798350022668,
-38.9051083126545));
#255966=CARTESIAN_POINT('Ctrl Pts',(-42.5906929412925,32.7780783962456,
-38.9321048428364));
#255967=CARTESIAN_POINT('Ctrl Pts',(-42.629225789877,32.8414173722334,-38.9502105255134));
#255968=CARTESIAN_POINT('Ctrl Pts',(-42.7120000069194,32.9638220552461,
-38.9866125955295));
#255969=CARTESIAN_POINT('Ctrl Pts',(-42.7562439327448,33.0229003355902,
-39.0049117194725));
#255970=CARTESIAN_POINT('Ctrl Pts',(-42.8269002201102,33.1083282766067,
-39.0325063049612));
#255971=CARTESIAN_POINT('Ctrl Pts',(-42.851168481378,33.1362718559733,-39.0417288667405));
#255972=CARTESIAN_POINT('Ctrl Pts',(-42.9011535535061,33.1910821810744,
-39.0602232021637));
#255973=CARTESIAN_POINT('Ctrl Pts',(-42.9268673384213,33.2179450225078,
-39.0694937486382));
#255974=CARTESIAN_POINT('Ctrl Pts',(-42.9797817061917,33.2705900457306,
-39.088089881442));
#255975=CARTESIAN_POINT('Ctrl Pts',(-43.0069972096607,33.2963736994337,
-39.097418269769));
#255976=CARTESIAN_POINT('Ctrl Pts',(-43.0622936398443,33.3462615369725,
-39.1159154063528));
#255977=CARTESIAN_POINT('Ctrl Pts',(-43.0904949946047,33.3704876748183,
-39.1251268688782));
#255978=CARTESIAN_POINT('Ctrl Pts',(-43.176562606447,33.4408730143711,-39.1525915568785));
#255979=CARTESIAN_POINT('Ctrl Pts',(-43.2360245534179,33.4848790444095,
-39.1707230137558));
#255980=CARTESIAN_POINT('Ctrl Pts',(-43.3282503301662,33.5464830068215,
-39.1976342358769));
#255981=CARTESIAN_POINT('Ctrl Pts',(-43.3595022265301,33.5662859367769,
-39.2065582055264));
#255982=CARTESIAN_POINT('Ctrl Pts',(-43.423032399699,33.604418869649,-39.2243132114598));
#255983=CARTESIAN_POINT('Ctrl Pts',(-43.4553106319894,33.6227489368786,
-39.2331442507783));
#255984=CARTESIAN_POINT('Ctrl Pts',(-43.5209070247133,33.6579164232732,
-39.2507127863664));
#255985=CARTESIAN_POINT('Ctrl Pts',(-43.5542222374601,33.6747516510336,
-39.2594493821381));
#255986=CARTESIAN_POINT('Ctrl Pts',(-43.6219256430316,33.7069073870392,
-39.2768314299875));
#255987=CARTESIAN_POINT('Ctrl Pts',(-43.6563381479934,33.7222286468184,
-39.2854811722856));
#255988=CARTESIAN_POINT('Ctrl Pts',(-43.7254519170511,33.7509934760634,
-39.3024907499371));
#255989=CARTESIAN_POINT('Ctrl Pts',(-43.7602995448845,33.7645084608315,
-39.3108885064059));
#255990=CARTESIAN_POINT('Ctrl Pts',(-43.8304781084082,33.789780836939,-39.3274499785309));
#255991=CARTESIAN_POINT('Ctrl Pts',(-43.8658243285985,33.8015455603985,
-39.3356176307442));
#255992=CARTESIAN_POINT('Ctrl Pts',(-43.9726293607703,33.8342393174696,
-39.3597845530997));
#255993=CARTESIAN_POINT('Ctrl Pts',(-44.0448528416425,33.8525737420732,
-39.3754485022349));
#255994=CARTESIAN_POINT('Ctrl Pts',(-44.1547335161489,33.874826743562,-39.3982722291653));
#255995=CARTESIAN_POINT('Ctrl Pts',(-44.1916183723467,33.8813683146414,
-39.4057679385072));
#255996=CARTESIAN_POINT('Ctrl Pts',(-44.2659122959158,33.8926702964892,
-39.4205323411483));
#255997=CARTESIAN_POINT('Ctrl Pts',(-44.3033049221432,33.8974288658374,
-39.4277978831022));
#255998=CARTESIAN_POINT('Ctrl Pts',(-44.3598453576919,33.9032050944765,
-39.4385322478049));
#255999=CARTESIAN_POINT('Ctrl Pts',(-44.3787527158677,33.9049006163346,
-39.4420799976889));
#256000=CARTESIAN_POINT('Ctrl Pts',(-44.4164967874688,33.9078161173588,
-39.4490791780208));
#256001=CARTESIAN_POINT('Ctrl Pts',(-44.4353708468856,33.9090400957878,
-39.4525377314439));
#256002=CARTESIAN_POINT('Ctrl Pts',(-44.4919347179527,33.9120095261766,
-39.462779235967));
#256003=CARTESIAN_POINT('Ctrl Pts',(-44.52962054914,33.9130584408517,-39.4694384189012));
#256004=CARTESIAN_POINT('Ctrl Pts',(-44.6425299001817,33.9134342925821,
-39.4889026473125));
#256005=CARTESIAN_POINT('Ctrl Pts',(-44.7176656228988,33.9100023852834,
-39.5012068570978));
#256006=CARTESIAN_POINT('Ctrl Pts',(-44.867623327666,33.8957625538083,-39.524471978366));
#256007=CARTESIAN_POINT('Ctrl Pts',(-44.9424659600731,33.8849485744664,
-39.5354353652432));
#256008=CARTESIAN_POINT('Ctrl Pts',(-45.0357885152669,33.8666999843662,
-39.5482785606344));
#256009=CARTESIAN_POINT('Ctrl Pts',(-45.0544546343785,33.8628074782943,
-39.5508053225112));
#256010=CARTESIAN_POINT('Ctrl Pts',(-45.0917431025751,33.8545484160302,
-39.5557691634051));
#256011=CARTESIAN_POINT('Ctrl Pts',(-45.1104022544846,33.8501716550149,
-39.5582107864407));
#256012=CARTESIAN_POINT('Ctrl Pts',(-45.1661672125598,33.8363538303533,
-39.565380228199));
#256013=CARTESIAN_POINT('Ctrl Pts',(-45.2029511118778,33.8262578362557,
-39.5699395109212));
#256014=CARTESIAN_POINT('Ctrl Pts',(-45.2758615915212,33.8042965707928,
-39.578640186911));
#256015=CARTESIAN_POINT('Ctrl Pts',(-45.3119687135373,33.792436319941,-39.5827791123973));
#256016=CARTESIAN_POINT('Ctrl Pts',(-45.3834929078587,33.7669724252328,
-39.5906388675035));
#256017=CARTESIAN_POINT('Ctrl Pts',(-45.4189099726225,33.753368762151,-39.59435969177));
#256018=CARTESIAN_POINT('Ctrl Pts',(-45.4890551197469,33.7244209300036,
-39.6013847808703));
#256019=CARTESIAN_POINT('Ctrl Pts',(-45.5237832050323,33.7090767682036,
-39.60468904687));
#256020=CARTESIAN_POINT('Ctrl Pts',(-45.5925464188782,33.6766380670054,
-39.6108794240926));
#256021=CARTESIAN_POINT('Ctrl Pts',(-45.6265815610841,33.6595435620003,
-39.6137655431243));
#256022=CARTESIAN_POINT('Ctrl Pts',(-45.6939497262655,33.6235811757592,
-39.6191148199286));
#256023=CARTESIAN_POINT('Ctrl Pts',(-45.7272860947277,33.6047101271221,
-39.6215780075552));
#256024=CARTESIAN_POINT('Ctrl Pts',(-45.7932287365117,33.5651705839516,
-39.6260731428005));
#256025=CARTESIAN_POINT('Ctrl Pts',(-45.8259059249178,33.5444453395394,
-39.6281074988012));
#256026=CARTESIAN_POINT('Ctrl Pts',(-45.8897275017006,33.5016881508368,
-39.6316923737189));
#256027=CARTESIAN_POINT('Ctrl Pts',(-45.9210297733036,33.4795651380847,
-39.6332542688506));
#256028=CARTESIAN_POINT('Ctrl Pts',(-45.9823424846244,33.4339088874735,
-39.6359180193303));
#256029=CARTESIAN_POINT('Ctrl Pts',(-46.0123687620003,33.4103663679687,
-39.6370209899198));
#256030=CARTESIAN_POINT('Ctrl Pts',(-46.1005740569048,33.337614535667,-39.639649668426));
#256031=CARTESIAN_POINT('Ctrl Pts',(-46.1568837651934,33.2862857446323,
-39.6404967282823));
#256032=CARTESIAN_POINT('Ctrl Pts',(-46.2375893041651,33.2050303462875,
-39.6404032087595));
#256033=CARTESIAN_POINT('Ctrl Pts',(-46.2638636333332,33.1772336958076,
-39.6401443034625));
#256034=CARTESIAN_POINT('Ctrl Pts',(-46.3151397511292,33.1201974856456,
-39.6391646017005));
#256035=CARTESIAN_POINT('Ctrl Pts',(-46.3401349353408,33.0909661742941,
-39.6384440851485));
#256036=CARTESIAN_POINT('Ctrl Pts',(-46.3888523044997,33.0309971480077,
-39.6365301000439));
#256037=CARTESIAN_POINT('Ctrl Pts',(-46.4123735341802,33.0005036828642,
-39.6353439924849));
#256038=CARTESIAN_POINT('Ctrl Pts',(-46.4576879006691,32.9386388625828,
-39.6325280276392));
#256039=CARTESIAN_POINT('Ctrl Pts',(-46.4794979867991,32.9072463828166,
-39.6308974590955));
#256040=CARTESIAN_POINT('Ctrl Pts',(-46.5424231451674,32.8117200287728,
-39.625348882952));
#256041=CARTESIAN_POINT('Ctrl Pts',(-46.5810426872604,32.7462345994881,
-39.6207752343847));
#256042=CARTESIAN_POINT('Ctrl Pts',(-46.6516918187306,32.6117039458857,
-39.6098936921283));
#256043=CARTESIAN_POINT('Ctrl Pts',(-46.683723185051,32.5426422373878,-39.6035832967262));
#256044=CARTESIAN_POINT('Ctrl Pts',(-46.7195635412788,32.4540883209462,
-39.5945936116187));
#256045=CARTESIAN_POINT('Ctrl Pts',(-46.726523577584,32.4362514419463,-39.5927383889277));
#256046=CARTESIAN_POINT('Ctrl Pts',(-46.7400123459627,32.4003742100513,
-39.5889189813535));
#256047=CARTESIAN_POINT('Ctrl Pts',(-46.7465535157541,32.3822946053341,
-39.5869502184844));
#256048=CARTESIAN_POINT('Ctrl Pts',(-46.7654644360989,32.3279072933141,
-39.5808958427402));
#256049=CARTESIAN_POINT('Ctrl Pts',(-46.7770937339888,32.2915493874552,
-39.5766741707955));
#256050=CARTESIAN_POINT('Ctrl Pts',(-46.7984826125902,32.218525216591,-39.5678552283644));
#256051=CARTESIAN_POINT('Ctrl Pts',(-46.8082356969316,32.1818782626467,
-39.5632601453561));
#256052=CARTESIAN_POINT('Ctrl Pts',(-46.825891612219,32.1083194036329,-39.5537041764669));
#256053=CARTESIAN_POINT('Ctrl Pts',(-46.8337943341285,32.0714074828253,
-39.5487432700414));
#256054=CARTESIAN_POINT('Ctrl Pts',(-46.8547548417649,31.9602784784655,
-39.5333157914925));
#256055=CARTESIAN_POINT('Ctrl Pts',(-46.8650708643863,31.8856621776612,
-39.5223044891954));
#256056=CARTESIAN_POINT('Ctrl Pts',(-46.8750487417844,31.7729724844591,
-39.50469487268));
#256057=CARTESIAN_POINT('Ctrl Pts',(-46.8774570362353,31.7352651712118,
-39.4986397605722));
#256058=CARTESIAN_POINT('Ctrl Pts',(-46.8796767940079,31.6785286095959,
-39.4892824810203));
#256059=CARTESIAN_POINT('Ctrl Pts',(-46.8801843407089,31.6595724593507,
-39.4861150486293));
#256060=CARTESIAN_POINT('Ctrl Pts',(-46.8807312344333,31.6216180949417,
-39.479690628598));
#256061=CARTESIAN_POINT('Ctrl Pts',(-46.8807699646674,31.6025797052015,
-39.4764266299692));
#256062=CARTESIAN_POINT('Ctrl Pts',(-46.8801790388754,31.5455906639181,
-39.4665317368708));
#256063=CARTESIAN_POINT('Ctrl Pts',(-46.8788490796135,31.5078273383739,
-39.4598096545541));
#256064=CARTESIAN_POINT('Ctrl Pts',(-46.874360617844,31.4326451774337,-39.4461013696832));
#256065=CARTESIAN_POINT('Ctrl Pts',(-46.8712024719357,31.3952438451296,
-39.4391182381771));
#256066=CARTESIAN_POINT('Ctrl Pts',(-46.859034870425,31.2835993575687,-39.4177870553822));
#256067=CARTESIAN_POINT('Ctrl Pts',(-46.8473376289695,31.2099145948488,
-39.4030579748028));
#256068=CARTESIAN_POINT('Ctrl Pts',(-46.8244863951756,31.1004910081606,
-39.3802058074804));
#256069=CARTESIAN_POINT('Ctrl Pts',(-46.8159835780379,31.0642007181804,
-39.3724617858671));
#256070=CARTESIAN_POINT('Ctrl Pts',(-46.7971994280146,30.9919902987916,
-39.3567184383004));
#256071=CARTESIAN_POINT('Ctrl Pts',(-46.7869180083019,30.9560697433081,
-39.3487190247537));
#256072=CARTESIAN_POINT('Ctrl Pts',(-46.7645577771926,30.884604709384,-39.332461491893));
#256073=CARTESIAN_POINT('Ctrl Pts',(-46.7524740339114,30.8490466969583,
-39.3242001683612));
#256074=CARTESIAN_POINT('Ctrl Pts',(-46.7264943673172,30.778363271582,-39.3074248425479));
#256075=CARTESIAN_POINT('Ctrl Pts',(-46.7127058212706,30.7435263372096,
-39.2989795429224));
#256076=CARTESIAN_POINT('Ctrl Pts',(-46.6981266849484,30.7091523375492,
-39.2904704603132));
#256077=CARTESIAN_POINT('',(-46.348736272544,30.7584582252104,-39.6906856150703));
#256078=CARTESIAN_POINT('',(-46.6981266849484,30.7091523375492,-39.2904704603132));
#256079=CARTESIAN_POINT('',(-46.5057017799105,31.6353141775361,-39.8960581789586));
#256080=CARTESIAN_POINT('Ctrl Pts',(-46.5057014676852,31.6353142217915,
-39.89605787487));
#256081=CARTESIAN_POINT('Ctrl Pts',(-46.5059898391685,31.6292400867244,
-39.8949168219445));
#256082=CARTESIAN_POINT('Ctrl Pts',(-46.5062503858504,31.6231697137711,
-39.8937699034812));
#256083=CARTESIAN_POINT('Ctrl Pts',(-46.5071135271648,31.6006673192385,
-39.8894976357773));
#256084=CARTESIAN_POINT('Ctrl Pts',(-46.5075417789082,31.5842004583658,
-39.8863302033863));
#256085=CARTESIAN_POINT('Ctrl Pts',(-46.5079914918558,31.5512299067555,
-39.8799057833551));
#256086=CARTESIAN_POINT('Ctrl Pts',(-46.5080123902999,31.5346913151838,
-39.8766417847262));
#256087=CARTESIAN_POINT('Ctrl Pts',(-46.5074608406805,31.4851846703929,
-39.8667468916278));
#256088=CARTESIAN_POINT('Ctrl Pts',(-46.506280107836,31.4523789139669,-39.8600248093111));
#256089=CARTESIAN_POINT('Ctrl Pts',(-46.5023302645975,31.3870655242667,
-39.8463165244401));
#256090=CARTESIAN_POINT('Ctrl Pts',(-46.4940227302404,31.289588481428,-39.8253669401756));
#256091=CARTESIAN_POINT('Ctrl Pts',(-46.4735992389084,31.1615543100329,
-39.7959087657426));
#256092=CARTESIAN_POINT('Ctrl Pts',(-46.4439553357389,31.0354316602054,
-39.764933002761));
#256093=CARTESIAN_POINT('Ctrl Pts',(-46.4260423093758,30.9730107791217,
-39.7489341795107));
#256094=CARTESIAN_POINT('Ctrl Pts',(-46.4065681949313,30.9109152099792,
-39.7326766466501));
#256095=CARTESIAN_POINT('Ctrl Pts',(-46.3960461932204,30.8800184397817,
-39.7244153231182));
#256096=CARTESIAN_POINT('Ctrl Pts',(-46.3734280792928,30.8185995307444,
-39.7076399973049));
#256097=CARTESIAN_POINT('Ctrl Pts',(-46.3614254481729,30.7883280602527,
-39.6991946976795));
#256098=CARTESIAN_POINT('Ctrl Pts',(-46.348736272544,30.7584582252104,-39.6906856150703));
#256099=CARTESIAN_POINT('Ctrl Pts',(-46.5057014676852,31.6353142217915,
-39.89605787487));
#256100=CARTESIAN_POINT('Ctrl Pts',(-46.504431262165,31.6620633341882,-39.9010881326463));
#256101=CARTESIAN_POINT('Ctrl Pts',(-46.5026263105811,31.688741807057,-39.9059955470865));
#256102=CARTESIAN_POINT('Ctrl Pts',(-46.4945629272159,31.7805948790823,
-39.9225196439524));
#256103=CARTESIAN_POINT('Ctrl Pts',(-46.4856505749035,31.8454075750247,
-39.9335309462494));
#256104=CARTESIAN_POINT('Ctrl Pts',(-46.4675150440425,31.9419322486556,
-39.9489584247984));
#256105=CARTESIAN_POINT('Ctrl Pts',(-46.4606740873934,31.9739927081568,
-39.9539193312238));
#256106=CARTESIAN_POINT('Ctrl Pts',(-46.445384375334,32.0378823010726,-39.9634753001132));
#256107=CARTESIAN_POINT('Ctrl Pts',(-46.4369357146477,32.0697114482314,
-39.9680703831214));
#256108=CARTESIAN_POINT('Ctrl Pts',(-46.4184025922855,32.1331342652581,
-39.9768893255524));
#256109=CARTESIAN_POINT('Ctrl Pts',(-46.4083237615152,32.1647111636399,
-39.9811109974971));
#256110=CARTESIAN_POINT('Ctrl Pts',(-46.391930976111,32.2119456968313,-39.9871653732414));
#256111=CARTESIAN_POINT('Ctrl Pts',(-46.3862603264385,32.2276473949945,
-39.9891341361105));
#256112=CARTESIAN_POINT('Ctrl Pts',(-46.3745657539713,32.2588055871924,
-39.9929535436847));
#256113=CARTESIAN_POINT('Ctrl Pts',(-46.3685310519543,32.2742961715653,
-39.9948087663756));
#256114=CARTESIAN_POINT('Ctrl Pts',(-46.3374534721736,32.3512007551325,
-40.0037984514834));
#256115=CARTESIAN_POINT('Ctrl Pts',(-46.3096720259105,32.4111748266119,
-40.0101088468852));
#256116=CARTESIAN_POINT('Ctrl Pts',(-46.2483848955207,32.5279978387927,
-40.0209903891417));
#256117=CARTESIAN_POINT('Ctrl Pts',(-46.2148776784186,32.58486109828,-40.025564037709));
#256118=CARTESIAN_POINT('Ctrl Pts',(-46.1602750397486,32.6678057987649,
-40.0311126138524));
#256119=CARTESIAN_POINT('Ctrl Pts',(-46.1413484466877,32.6950629059706,
-40.0327431823962));
#256120=CARTESIAN_POINT('Ctrl Pts',(-46.1020228696767,32.7487767218636,
-40.0355591472418));
#256121=CARTESIAN_POINT('Ctrl Pts',(-46.0816091751359,32.7752517709756,
-40.0367452548009));
#256122=CARTESIAN_POINT('Ctrl Pts',(-46.039326094558,32.8273165460041,-40.0386592399055));
#256123=CARTESIAN_POINT('Ctrl Pts',(-46.0176311249679,32.8526942171489,
-40.0393797564574));
#256124=CARTESIAN_POINT('Ctrl Pts',(-45.9731233122554,32.9022095992068,
-40.0403594582195));
#256125=CARTESIAN_POINT('Ctrl Pts',(-45.9503162012007,32.9263401489037,
-40.0406183635165));
#256126=CARTESIAN_POINT('Ctrl Pts',(-45.8802580990489,32.9968762744355,
-40.0407118830392));
#256127=CARTESIAN_POINT('Ctrl Pts',(-45.8313738629074,33.0414303223986,
-40.039864823183));
#256128=CARTESIAN_POINT('Ctrl Pts',(-45.7547952110795,33.1045744158562,
-40.0372361446768));
#256129=CARTESIAN_POINT('Ctrl Pts',(-45.7287260251324,33.1250069084101,
-40.0361331740873));
#256130=CARTESIAN_POINT('Ctrl Pts',(-45.6754920455146,33.1646298482803,
-40.0334694236076));
#256131=CARTESIAN_POINT('Ctrl Pts',(-45.6483134994178,33.1838283485151,
-40.0319075284759));
#256132=CARTESIAN_POINT('Ctrl Pts',(-45.5928982301755,33.2209311560931,
-40.0283226535581));
#256133=CARTESIAN_POINT('Ctrl Pts',(-45.5645244103116,33.2389144742721,
-40.0262882975575));
#256134=CARTESIAN_POINT('Ctrl Pts',(-45.5072645495699,33.2732206191231,
-40.0217931623121));
#256135=CARTESIAN_POINT('Ctrl Pts',(-45.4783169400346,33.2895926998564,
-40.0193299746856));
#256136=CARTESIAN_POINT('Ctrl Pts',(-45.4373898222728,33.3114186492017,
-40.0155876017777));
#256137=CARTESIAN_POINT('Ctrl Pts',(-45.4256642380104,33.3175230028014,
-40.0144861643931));
#256138=CARTESIAN_POINT('Ctrl Pts',(-45.4138902706673,33.3235051193248,
-40.0133502342376));
#256139=CARTESIAN_POINT('Origin',(-44.5079524583202,31.5404524382932,-52.920575));
#256140=CARTESIAN_POINT('Ctrl Pts',(-42.8392071752677,31.5404524382931,
-52.4912));
#256141=CARTESIAN_POINT('Ctrl Pts',(-42.8392071752677,32.5039029766724,
-52.4328666666667));
#256142=CARTESIAN_POINT('Ctrl Pts',(-43.6735798167939,32.985628245862,-52.3745333333334));
#256143=CARTESIAN_POINT('Ctrl Pts',(-44.5079524583201,33.4673535150516,
-52.3162000000001));
#256144=CARTESIAN_POINT('Ctrl Pts',(-45.3423250998464,32.985628245862,-52.2578666666667));
#256145=CARTESIAN_POINT('Ctrl Pts',(-46.1766977413726,32.5039029766724,
-52.1995333333334));
#256146=CARTESIAN_POINT('Ctrl Pts',(-46.1766977413726,31.5404524382932,
-52.1412));
#256147=CARTESIAN_POINT('Ctrl Pts',(-46.1766977413726,30.5770018999139,
-52.0828666666667));
#256148=CARTESIAN_POINT('Ctrl Pts',(-45.3423250998464,30.0952766307242,
-52.0245333333333));
#256149=CARTESIAN_POINT('Ctrl Pts',(-44.5079524583202,29.6135513615346,
-51.9662));
#256150=CARTESIAN_POINT('Ctrl Pts',(-43.6735798167939,30.0952766307242,
-51.9078666666667));
#256151=CARTESIAN_POINT('Ctrl Pts',(-42.8392071752677,30.5770018999139,
-51.8495333333334));
#256152=CARTESIAN_POINT('Ctrl Pts',(-42.8392071752677,31.5404524382931,
-51.7912));
#256153=CARTESIAN_POINT('Ctrl Pts',(-42.8392071752677,31.5404524382931,
-52.64995));
#256154=CARTESIAN_POINT('Ctrl Pts',(-42.8392071752677,32.5039029766724,
-52.5916166666667));
#256155=CARTESIAN_POINT('Ctrl Pts',(-43.6735798167939,32.985628245862,-52.5332833333334));
#256156=CARTESIAN_POINT('Ctrl Pts',(-44.5079524583201,33.4673535150516,
-52.47495));
#256157=CARTESIAN_POINT('Ctrl Pts',(-45.3423250998464,32.985628245862,-52.4166166666667));
#256158=CARTESIAN_POINT('Ctrl Pts',(-46.1766977413726,32.5039029766724,
-52.3582833333334));
#256159=CARTESIAN_POINT('Ctrl Pts',(-46.1766977413726,31.5404524382932,
-52.29995));
#256160=CARTESIAN_POINT('Ctrl Pts',(-46.1766977413726,30.5770018999139,
-52.2416166666667));
#256161=CARTESIAN_POINT('Ctrl Pts',(-45.3423250998464,30.0952766307242,
-52.1832833333333));
#256162=CARTESIAN_POINT('Ctrl Pts',(-44.5079524583202,29.6135513615346,
-52.12495));
#256163=CARTESIAN_POINT('Ctrl Pts',(-43.6735798167939,30.0952766307242,
-52.0666166666667));
#256164=CARTESIAN_POINT('Ctrl Pts',(-42.8392071752677,30.5770018999139,
-52.0082833333333));
#256165=CARTESIAN_POINT('Ctrl Pts',(-42.8392071752677,31.5404524382931,
-51.94995));
#256166=CARTESIAN_POINT('Ctrl Pts',(-46.5766932247455,31.5404524382932,
-52.6102625));
#256167=CARTESIAN_POINT('Ctrl Pts',(-46.5766932247455,30.3460643999139,
-52.5519291666666));
#256168=CARTESIAN_POINT('Ctrl Pts',(-45.5423228415329,29.7488703807243,
-52.4935958333333));
#256169=CARTESIAN_POINT('Ctrl Pts',(-44.5079524583202,29.1516763615346,
-52.4352625));
#256170=CARTESIAN_POINT('Ctrl Pts',(-43.4735820751074,29.7488703807243,
-52.3769291666667));
#256171=CARTESIAN_POINT('Ctrl Pts',(-42.4392116918948,30.3460643999138,
-52.3185958333334));
#256172=CARTESIAN_POINT('Ctrl Pts',(-42.4392116918948,31.5404524382931,
-52.2602625));
#256173=CARTESIAN_POINT('Ctrl Pts',(-42.4392116918947,32.7348404766723,
-52.2019291666667));
#256174=CARTESIAN_POINT('Ctrl Pts',(-43.4735820751074,33.332034495862,-52.1435958333333));
#256175=CARTESIAN_POINT('Ctrl Pts',(-44.5079524583201,33.9292285150516,
-52.0852625));
#256176=CARTESIAN_POINT('Ctrl Pts',(-45.5423228415328,33.332034495862,-52.0269291666667));
#256177=CARTESIAN_POINT('Ctrl Pts',(-46.5766932247455,32.7348404766724,
-51.9685958333333));
#256178=CARTESIAN_POINT('Ctrl Pts',(-46.5766932247455,31.5404524382932,
-51.9102625));
#256179=CARTESIAN_POINT('Ctrl Pts',(-46.5766932247455,30.3460643999139,
-51.8519291666667));
#256180=CARTESIAN_POINT('Ctrl Pts',(-45.5423228415329,29.7488703807243,
-51.7935958333333));
#256181=CARTESIAN_POINT('Ctrl Pts',(-44.5079524583202,29.1516763615346,
-51.7352625));
#256182=CARTESIAN_POINT('Ctrl Pts',(-43.4735820751074,29.7488703807243,
-51.6769291666667));
#256183=CARTESIAN_POINT('Ctrl Pts',(-42.4392116918948,30.3460643999138,
-51.6185958333333));
#256184=CARTESIAN_POINT('Ctrl Pts',(-42.4392116918948,31.5404524382931,
-51.5602625));
#256185=CARTESIAN_POINT('Ctrl Pts',(-42.4392116918947,32.7348404766723,
-51.5019291666666));
#256186=CARTESIAN_POINT('Ctrl Pts',(-43.4735820751074,33.332034495862,-51.4435958333333));
#256187=CARTESIAN_POINT('Ctrl Pts',(-44.5079524583201,33.9292285150516,
-51.3852625));
#256188=CARTESIAN_POINT('Ctrl Pts',(-45.5423228415328,33.332034495862,-51.3269291666667));
#256189=CARTESIAN_POINT('Ctrl Pts',(-46.5766932247455,32.7348404766724,
-51.2685958333333));
#256190=CARTESIAN_POINT('Ctrl Pts',(-46.5766932247455,31.5404524382932,
-51.2102625));
#256191=CARTESIAN_POINT('Ctrl Pts',(-46.5766932247455,30.3460643999139,
-51.1519291666666));
#256192=CARTESIAN_POINT('Ctrl Pts',(-45.5423228415329,29.7488703807243,
-51.0935958333334));
#256193=CARTESIAN_POINT('Ctrl Pts',(-44.5079524583202,29.1516763615346,
-51.0352625));
#256194=CARTESIAN_POINT('Ctrl Pts',(-43.4735820751074,29.7488703807243,
-50.9769291666667));
#256195=CARTESIAN_POINT('Ctrl Pts',(-42.4392116918948,30.3460643999138,
-50.9185958333333));
#256196=CARTESIAN_POINT('Ctrl Pts',(-42.4392116918948,31.5404524382931,
-50.8602625));
#256197=CARTESIAN_POINT('Ctrl Pts',(-42.4392116918947,32.7348404766723,
-50.8019291666667));
#256198=CARTESIAN_POINT('Ctrl Pts',(-43.4735820751074,33.332034495862,-50.7435958333333));
#256199=CARTESIAN_POINT('Ctrl Pts',(-44.5079524583201,33.9292285150516,
-50.6852625));
#256200=CARTESIAN_POINT('Ctrl Pts',(-45.5423228415328,33.332034495862,-50.6269291666667));
#256201=CARTESIAN_POINT('Ctrl Pts',(-46.5766932247455,32.7348404766724,
-50.5685958333333));
#256202=CARTESIAN_POINT('Ctrl Pts',(-46.5766932247455,31.5404524382932,
-50.5102625));
#256203=CARTESIAN_POINT('Ctrl Pts',(-46.5766932247455,30.3460643999139,
-50.4519291666667));
#256204=CARTESIAN_POINT('Ctrl Pts',(-45.5423228415329,29.7488703807243,
-50.3935958333333));
#256205=CARTESIAN_POINT('Ctrl Pts',(-44.5079524583202,29.1516763615346,
-50.3352625));
#256206=CARTESIAN_POINT('Ctrl Pts',(-43.4735820751074,29.7488703807243,
-50.2769291666667));
#256207=CARTESIAN_POINT('Ctrl Pts',(-42.4392116918948,30.3460643999138,
-50.2185958333333));
#256208=CARTESIAN_POINT('Ctrl Pts',(-42.4392116918948,31.5404524382931,
-50.1602625));
#256209=CARTESIAN_POINT('Ctrl Pts',(-42.4392116918947,32.7348404766723,
-50.1019291666667));
#256210=CARTESIAN_POINT('Ctrl Pts',(-43.4735820751074,33.332034495862,-50.0435958333333));
#256211=CARTESIAN_POINT('Ctrl Pts',(-44.5079524583201,33.9292285150516,
-49.9852625));
#256212=CARTESIAN_POINT('Ctrl Pts',(-45.5423228415328,33.332034495862,-49.9269291666667));
#256213=CARTESIAN_POINT('Ctrl Pts',(-46.5766932247455,32.7348404766724,
-49.8685958333333));
#256214=CARTESIAN_POINT('Ctrl Pts',(-46.5766932247455,31.5404524382932,
-49.8102625));
#256215=CARTESIAN_POINT('Ctrl Pts',(-46.5766932247455,30.3460643999139,
-49.7519291666667));
#256216=CARTESIAN_POINT('Ctrl Pts',(-45.5423228415329,29.7488703807243,
-49.6935958333334));
#256217=CARTESIAN_POINT('Ctrl Pts',(-44.5079524583202,29.1516763615346,
-49.6352625));
#256218=CARTESIAN_POINT('Ctrl Pts',(-43.4735820751074,29.7488703807243,
-49.5769291666667));
#256219=CARTESIAN_POINT('Ctrl Pts',(-42.4392116918948,30.3460643999138,
-49.5185958333334));
#256220=CARTESIAN_POINT('Ctrl Pts',(-42.4392116918948,31.5404524382931,
-49.4602625));
#256221=CARTESIAN_POINT('Ctrl Pts',(-42.4392116918947,32.7348404766723,
-49.4019291666667));
#256222=CARTESIAN_POINT('Ctrl Pts',(-43.4735820751074,33.332034495862,-49.3435958333333));
#256223=CARTESIAN_POINT('Ctrl Pts',(-44.5079524583201,33.9292285150516,
-49.2852625));
#256224=CARTESIAN_POINT('Ctrl Pts',(-45.5423228415328,33.332034495862,-49.2269291666667));
#256225=CARTESIAN_POINT('Ctrl Pts',(-46.5766932247455,32.7348404766724,
-49.1685958333334));
#256226=CARTESIAN_POINT('Ctrl Pts',(-46.5766932247455,31.5404524382932,
-49.1102625));
#256227=CARTESIAN_POINT('Ctrl Pts',(-46.5766932247455,30.3460643999139,
-49.0519291666667));
#256228=CARTESIAN_POINT('Ctrl Pts',(-45.5423228415329,29.7488703807243,
-48.9935958333333));
#256229=CARTESIAN_POINT('Ctrl Pts',(-44.5079524583202,29.1516763615346,
-48.9352625));
#256230=CARTESIAN_POINT('Ctrl Pts',(-43.4735820751074,29.7488703807243,
-48.8769291666667));
#256231=CARTESIAN_POINT('Ctrl Pts',(-42.4392116918948,30.3460643999138,
-48.8185958333333));
#256232=CARTESIAN_POINT('Ctrl Pts',(-42.4392116918948,31.5404524382931,
-48.7602625));
#256233=CARTESIAN_POINT('Ctrl Pts',(-42.4392116918947,32.7348404766723,
-48.7019291666667));
#256234=CARTESIAN_POINT('Ctrl Pts',(-43.4735820751074,33.332034495862,-48.6435958333333));
#256235=CARTESIAN_POINT('Ctrl Pts',(-44.5079524583201,33.9292285150516,
-48.5852625));
#256236=CARTESIAN_POINT('Ctrl Pts',(-45.5423228415328,33.332034495862,-48.5269291666667));
#256237=CARTESIAN_POINT('Ctrl Pts',(-46.5766932247455,32.7348404766724,
-48.4685958333333));
#256238=CARTESIAN_POINT('Ctrl Pts',(-46.5766932247455,31.5404524382932,
-48.4102625));
#256239=CARTESIAN_POINT('Ctrl Pts',(-46.5766932247455,30.3460643999139,
-48.3519291666667));
#256240=CARTESIAN_POINT('Ctrl Pts',(-45.5423228415329,29.7488703807243,
-48.2935958333333));
#256241=CARTESIAN_POINT('Ctrl Pts',(-44.5079524583202,29.1516763615346,
-48.2352625));
#256242=CARTESIAN_POINT('Ctrl Pts',(-43.4735820751074,29.7488703807243,
-48.1769291666667));
#256243=CARTESIAN_POINT('Ctrl Pts',(-42.4392116918948,30.3460643999138,
-48.1185958333334));
#256244=CARTESIAN_POINT('Ctrl Pts',(-42.4392116918948,31.5404524382931,
-48.0602625));
#256245=CARTESIAN_POINT('Ctrl Pts',(-42.4392116918947,32.7348404766723,
-48.0019291666667));
#256246=CARTESIAN_POINT('Ctrl Pts',(-43.4735820751074,33.332034495862,-47.9435958333334));
#256247=CARTESIAN_POINT('Ctrl Pts',(-44.5079524583201,33.9292285150516,
-47.8852625));
#256248=CARTESIAN_POINT('Ctrl Pts',(-45.5423228415328,33.332034495862,-47.8269291666667));
#256249=CARTESIAN_POINT('Ctrl Pts',(-46.5766932247455,32.7348404766724,
-47.7685958333333));
#256250=CARTESIAN_POINT('Ctrl Pts',(-46.5766932247455,31.5404524382932,
-47.7102625));
#256251=CARTESIAN_POINT('Ctrl Pts',(-46.5766932247455,30.3460643999139,
-47.6519291666667));
#256252=CARTESIAN_POINT('Ctrl Pts',(-45.5423228415329,29.7488703807243,
-47.5935958333333));
#256253=CARTESIAN_POINT('Ctrl Pts',(-44.5079524583202,29.1516763615346,
-47.5352625));
#256254=CARTESIAN_POINT('Ctrl Pts',(-43.4735820751074,29.7488703807243,
-47.4769291666667));
#256255=CARTESIAN_POINT('Ctrl Pts',(-42.4392116918948,30.3460643999138,
-47.4185958333333));
#256256=CARTESIAN_POINT('Ctrl Pts',(-42.4392116918948,31.5404524382931,
-47.3602625));
#256257=CARTESIAN_POINT('Ctrl Pts',(-42.4392116918947,32.7348404766723,
-47.3019291666666));
#256258=CARTESIAN_POINT('Ctrl Pts',(-43.4735820751074,33.332034495862,-47.2435958333333));
#256259=CARTESIAN_POINT('Ctrl Pts',(-44.5079524583201,33.9292285150516,
-47.1852625));
#256260=CARTESIAN_POINT('Ctrl Pts',(-45.5423228415328,33.332034495862,-47.1269291666667));
#256261=CARTESIAN_POINT('Ctrl Pts',(-46.5766932247455,32.7348404766724,
-47.0685958333333));
#256262=CARTESIAN_POINT('Ctrl Pts',(-46.5766932247455,31.5404524382932,
-47.0102625));
#256263=CARTESIAN_POINT('Ctrl Pts',(-46.5766932247455,30.3460643999139,
-46.9519291666667));
#256264=CARTESIAN_POINT('Ctrl Pts',(-45.5423228415329,29.7488703807243,
-46.8935958333333));
#256265=CARTESIAN_POINT('Ctrl Pts',(-44.5079524583202,29.1516763615346,
-46.8352625));
#256266=CARTESIAN_POINT('Ctrl Pts',(-43.4735820751074,29.7488703807243,
-46.7769291666667));
#256267=CARTESIAN_POINT('Ctrl Pts',(-42.4392116918948,30.3460643999138,
-46.7185958333333));
#256268=CARTESIAN_POINT('Ctrl Pts',(-42.4392116918948,31.5404524382931,
-46.6602625));
#256269=CARTESIAN_POINT('Ctrl Pts',(-42.4392116918948,32.7348404766723,
-46.6019291666667));
#256270=CARTESIAN_POINT('Ctrl Pts',(-43.4735820751074,33.332034495862,-46.5435958333334));
#256271=CARTESIAN_POINT('Ctrl Pts',(-44.5079524583201,33.9292285150516,
-46.4852625));
#256272=CARTESIAN_POINT('Ctrl Pts',(-45.5423228415328,33.332034495862,-46.4269291666667));
#256273=CARTESIAN_POINT('Ctrl Pts',(-46.5766932247455,32.7348404766724,
-46.3685958333333));
#256274=CARTESIAN_POINT('Ctrl Pts',(-46.5766932247455,31.5404524382932,
-46.3102625));
#256275=CARTESIAN_POINT('Ctrl Pts',(-46.5766932247455,30.3460643999139,
-46.2519291666667));
#256276=CARTESIAN_POINT('Ctrl Pts',(-45.5423228415329,29.7488703807243,
-46.1935958333333));
#256277=CARTESIAN_POINT('Ctrl Pts',(-44.5079524583202,29.1516763615346,
-46.1352625));
#256278=CARTESIAN_POINT('Ctrl Pts',(-43.4735820751074,29.7488703807243,
-46.0769291666667));
#256279=CARTESIAN_POINT('Ctrl Pts',(-42.4392116918948,30.3460643999138,
-46.0185958333334));
#256280=CARTESIAN_POINT('Ctrl Pts',(-42.4392116918948,31.5404524382931,
-45.9602625));
#256281=CARTESIAN_POINT('Ctrl Pts',(-42.4392116918948,32.7348404766723,
-45.9019291666667));
#256282=CARTESIAN_POINT('Ctrl Pts',(-43.4735820751074,33.332034495862,-45.8435958333333));
#256283=CARTESIAN_POINT('Ctrl Pts',(-44.5079524583201,33.9292285150516,
-45.7852625));
#256284=CARTESIAN_POINT('Ctrl Pts',(-45.5423228415328,33.332034495862,-45.7269291666667));
#256285=CARTESIAN_POINT('Ctrl Pts',(-46.5766932247455,32.7348404766724,
-45.6685958333334));
#256286=CARTESIAN_POINT('Ctrl Pts',(-46.5766932247455,31.5404524382932,
-45.6102625));
#256287=CARTESIAN_POINT('Ctrl Pts',(-46.5766932247455,30.3460643999139,
-45.5519291666667));
#256288=CARTESIAN_POINT('Ctrl Pts',(-45.5423228415329,29.7488703807243,
-45.4935958333333));
#256289=CARTESIAN_POINT('Ctrl Pts',(-44.5079524583202,29.1516763615346,
-45.4352625));
#256290=CARTESIAN_POINT('Ctrl Pts',(-43.4735820751074,29.7488703807243,
-45.3769291666667));
#256291=CARTESIAN_POINT('Ctrl Pts',(-42.4392116918948,30.3460643999138,
-45.3185958333333));
#256292=CARTESIAN_POINT('Ctrl Pts',(-42.4392116918948,31.5404524382931,
-45.2602625));
#256293=CARTESIAN_POINT('Ctrl Pts',(-42.4392116918948,32.7348404766723,
-45.2019291666667));
#256294=CARTESIAN_POINT('Ctrl Pts',(-43.4735820751074,33.332034495862,-45.1435958333333));
#256295=CARTESIAN_POINT('Ctrl Pts',(-44.5079524583201,33.9292285150516,
-45.0852625));
#256296=CARTESIAN_POINT('Ctrl Pts',(-45.5423228415328,33.332034495862,-45.0269291666667));
#256297=CARTESIAN_POINT('Ctrl Pts',(-46.5766932247455,32.7348404766724,
-44.9685958333334));
#256298=CARTESIAN_POINT('Ctrl Pts',(-46.5766932247455,31.5404524382932,
-44.9102625));
#256299=CARTESIAN_POINT('Ctrl Pts',(-46.5766932247455,30.3460643999139,
-44.8519291666667));
#256300=CARTESIAN_POINT('Ctrl Pts',(-45.5423228415329,29.7488703807243,
-44.7935958333333));
#256301=CARTESIAN_POINT('Ctrl Pts',(-44.5079524583202,29.1516763615346,
-44.7352625));
#256302=CARTESIAN_POINT('Ctrl Pts',(-43.4735820751074,29.7488703807243,
-44.6769291666667));
#256303=CARTESIAN_POINT('Ctrl Pts',(-42.4392116918948,30.3460643999138,
-44.6185958333334));
#256304=CARTESIAN_POINT('Ctrl Pts',(-42.4392116918948,31.5404524382931,
-44.5602625));
#256305=CARTESIAN_POINT('Ctrl Pts',(-42.4392116918948,32.7348404766723,
-44.5019291666667));
#256306=CARTESIAN_POINT('Ctrl Pts',(-43.4735820751074,33.332034495862,-44.4435958333333));
#256307=CARTESIAN_POINT('Ctrl Pts',(-44.5079524583201,33.9292285150516,
-44.3852625));
#256308=CARTESIAN_POINT('Ctrl Pts',(-45.5423228415328,33.332034495862,-44.3269291666667));
#256309=CARTESIAN_POINT('Ctrl Pts',(-46.5766932247455,32.7348404766724,
-44.2685958333334));
#256310=CARTESIAN_POINT('Ctrl Pts',(-46.5766932247455,31.5404524382932,
-44.2102625));
#256311=CARTESIAN_POINT('Ctrl Pts',(-46.5766932247455,30.3460643999139,
-44.1519291666667));
#256312=CARTESIAN_POINT('Ctrl Pts',(-45.5423228415329,29.7488703807243,
-44.0935958333334));
#256313=CARTESIAN_POINT('Ctrl Pts',(-44.5079524583202,29.1516763615346,
-44.0352625));
#256314=CARTESIAN_POINT('Ctrl Pts',(-43.4735820751074,29.7488703807243,
-43.9769291666667));
#256315=CARTESIAN_POINT('Ctrl Pts',(-42.4392116918948,30.3460643999138,
-43.9185958333333));
#256316=CARTESIAN_POINT('Ctrl Pts',(-42.4392116918948,31.5404524382931,
-43.8602625));
#256317=CARTESIAN_POINT('Ctrl Pts',(-42.4392116918948,32.7348404766723,
-43.8019291666667));
#256318=CARTESIAN_POINT('Ctrl Pts',(-43.4735820751074,33.332034495862,-43.7435958333334));
#256319=CARTESIAN_POINT('Ctrl Pts',(-44.5079524583201,33.9292285150516,
-43.6852625));
#256320=CARTESIAN_POINT('Ctrl Pts',(-45.5423228415328,33.332034495862,-43.6269291666667));
#256321=CARTESIAN_POINT('Ctrl Pts',(-46.5766932247455,32.7348404766724,
-43.5685958333333));
#256322=CARTESIAN_POINT('Ctrl Pts',(-46.5766932247455,31.5404524382932,
-43.5102625));
#256323=CARTESIAN_POINT('Ctrl Pts',(-46.5766932247455,30.3460643999139,
-43.4519291666667));
#256324=CARTESIAN_POINT('Ctrl Pts',(-45.5423228415329,29.7488703807243,
-43.3935958333334));
#256325=CARTESIAN_POINT('Ctrl Pts',(-44.5079524583202,29.1516763615346,
-43.3352625));
#256326=CARTESIAN_POINT('Ctrl Pts',(-43.4735820751074,29.7488703807243,
-43.2769291666667));
#256327=CARTESIAN_POINT('Ctrl Pts',(-42.4392116918948,30.3460643999138,
-43.2185958333333));
#256328=CARTESIAN_POINT('Ctrl Pts',(-42.4392116918948,31.5404524382931,
-43.1602625));
#256329=CARTESIAN_POINT('Ctrl Pts',(-42.4392116918948,32.7348404766723,
-43.1019291666667));
#256330=CARTESIAN_POINT('Ctrl Pts',(-43.4735820751074,33.332034495862,-43.0435958333334));
#256331=CARTESIAN_POINT('Ctrl Pts',(-44.5079524583201,33.9292285150516,
-42.9852625));
#256332=CARTESIAN_POINT('Ctrl Pts',(-45.5423228415328,33.332034495862,-42.9269291666667));
#256333=CARTESIAN_POINT('Ctrl Pts',(-46.5766932247455,32.7348404766724,
-42.8685958333333));
#256334=CARTESIAN_POINT('Ctrl Pts',(-46.5766932247455,31.5404524382932,
-42.8102625));
#256335=CARTESIAN_POINT('Ctrl Pts',(-46.5766932247455,30.3460643999139,
-42.7519291666666));
#256336=CARTESIAN_POINT('Ctrl Pts',(-45.5423228415329,29.7488703807243,
-42.6935958333333));
#256337=CARTESIAN_POINT('Ctrl Pts',(-44.5079524583202,29.1516763615346,
-42.6352625));
#256338=CARTESIAN_POINT('Ctrl Pts',(-43.4735820751074,29.7488703807243,
-42.5769291666667));
#256339=CARTESIAN_POINT('Ctrl Pts',(-42.4392116918948,30.3460643999138,
-42.5185958333333));
#256340=CARTESIAN_POINT('Ctrl Pts',(-42.4392116918948,31.5404524382931,
-42.4602625));
#256341=CARTESIAN_POINT('Ctrl Pts',(-42.4392116918948,32.7348404766723,
-42.4019291666666));
#256342=CARTESIAN_POINT('Ctrl Pts',(-43.4735820751074,33.332034495862,-42.3435958333334));
#256343=CARTESIAN_POINT('Ctrl Pts',(-44.5079524583201,33.9292285150516,
-42.2852625));
#256344=CARTESIAN_POINT('Ctrl Pts',(-45.5423228415328,33.332034495862,-42.2269291666667));
#256345=CARTESIAN_POINT('Ctrl Pts',(-46.5766932247455,32.7348404766724,
-42.1685958333333));
#256346=CARTESIAN_POINT('Ctrl Pts',(-46.5766932247455,31.5404524382932,
-42.1102625));
#256347=CARTESIAN_POINT('Ctrl Pts',(-46.5766932247455,30.3460643999139,
-42.0519291666666));
#256348=CARTESIAN_POINT('Ctrl Pts',(-45.5423228415329,29.7488703807243,
-41.9935958333334));
#256349=CARTESIAN_POINT('Ctrl Pts',(-44.5079524583202,29.1516763615346,
-41.9352625));
#256350=CARTESIAN_POINT('Ctrl Pts',(-43.4735820751074,29.7488703807243,
-41.8769291666667));
#256351=CARTESIAN_POINT('Ctrl Pts',(-42.4392116918948,30.3460643999138,
-41.8185958333333));
#256352=CARTESIAN_POINT('Ctrl Pts',(-42.4392116918948,31.5404524382931,
-41.7602625));
#256353=CARTESIAN_POINT('Ctrl Pts',(-42.4392116918948,32.7348404766723,
-41.7019291666666));
#256354=CARTESIAN_POINT('Ctrl Pts',(-43.4735820751074,33.332034495862,-41.6435958333334));
#256355=CARTESIAN_POINT('Ctrl Pts',(-44.5079524583201,33.9292285150516,
-41.5852625));
#256356=CARTESIAN_POINT('Ctrl Pts',(-45.5423228415328,33.332034495862,-41.5269291666667));
#256357=CARTESIAN_POINT('Ctrl Pts',(-46.5766932247455,32.7348404766724,
-41.4685958333333));
#256358=CARTESIAN_POINT('Ctrl Pts',(-46.5766932247455,31.5404524382932,
-41.4102625));
#256359=CARTESIAN_POINT('Ctrl Pts',(-46.5766932247455,30.3460643999139,
-41.3519291666666));
#256360=CARTESIAN_POINT('Ctrl Pts',(-45.5423228415329,29.7488703807243,
-41.2935958333334));
#256361=CARTESIAN_POINT('Ctrl Pts',(-44.5079524583202,29.1516763615346,
-41.2352625));
#256362=CARTESIAN_POINT('Ctrl Pts',(-43.4735820751074,29.7488703807243,
-41.1769291666667));
#256363=CARTESIAN_POINT('Ctrl Pts',(-42.4392116918948,30.3460643999138,
-41.1185958333333));
#256364=CARTESIAN_POINT('Ctrl Pts',(-42.4392116918948,31.5404524382931,
-41.0602625));
#256365=CARTESIAN_POINT('Ctrl Pts',(-42.4392116918948,32.7348404766723,
-41.0019291666666));
#256366=CARTESIAN_POINT('Ctrl Pts',(-43.4735820751074,33.332034495862,-40.9435958333334));
#256367=CARTESIAN_POINT('Ctrl Pts',(-44.5079524583201,33.9292285150516,
-40.8852625));
#256368=CARTESIAN_POINT('Ctrl Pts',(-45.5423228415328,33.332034495862,-40.8269291666667));
#256369=CARTESIAN_POINT('Ctrl Pts',(-46.5766932247455,32.7348404766724,
-40.7685958333333));
#256370=CARTESIAN_POINT('Ctrl Pts',(-46.5766932247455,31.5404524382932,
-40.7102625));
#256371=CARTESIAN_POINT('Ctrl Pts',(-46.5766932247455,30.3460643999139,
-40.6519291666667));
#256372=CARTESIAN_POINT('Ctrl Pts',(-45.5423228415329,29.7488703807243,
-40.5935958333334));
#256373=CARTESIAN_POINT('Ctrl Pts',(-44.5079524583202,29.1516763615346,
-40.5352625));
#256374=CARTESIAN_POINT('Ctrl Pts',(-43.4735820751074,29.7488703807243,
-40.4769291666667));
#256375=CARTESIAN_POINT('Ctrl Pts',(-42.4392116918948,30.3460643999138,
-40.4185958333333));
#256376=CARTESIAN_POINT('Ctrl Pts',(-42.4392116918948,31.5404524382931,
-40.3602625));
#256377=CARTESIAN_POINT('Ctrl Pts',(-42.4392116918948,32.7348404766723,
-40.3019291666667));
#256378=CARTESIAN_POINT('Ctrl Pts',(-43.4735820751074,33.332034495862,-40.2435958333334));
#256379=CARTESIAN_POINT('Ctrl Pts',(-44.5079524583201,33.9292285150516,
-40.1852625));
#256380=CARTESIAN_POINT('Ctrl Pts',(-45.5423228415328,33.332034495862,-40.1269291666666));
#256381=CARTESIAN_POINT('Ctrl Pts',(-46.5766932247455,32.7348404766724,
-40.0685958333333));
#256382=CARTESIAN_POINT('Ctrl Pts',(-46.5766932247455,31.5404524382932,
-40.0102625));
#256383=CARTESIAN_POINT('Ctrl Pts',(-46.5766932247455,30.3460643999139,
-39.9519291666667));
#256384=CARTESIAN_POINT('Ctrl Pts',(-45.5423228415329,29.7488703807243,
-39.8935958333334));
#256385=CARTESIAN_POINT('Ctrl Pts',(-44.5079524583202,29.1516763615346,
-39.8352625));
#256386=CARTESIAN_POINT('Ctrl Pts',(-43.4735820751074,29.7488703807243,
-39.7769291666666));
#256387=CARTESIAN_POINT('Ctrl Pts',(-42.4392116918948,30.3460643999138,
-39.7185958333334));
#256388=CARTESIAN_POINT('Ctrl Pts',(-42.4392116918948,31.5404524382931,
-39.6602625));
#256389=CARTESIAN_POINT('Ctrl Pts',(-42.4392116918948,32.7348404766723,
-39.6019291666667));
#256390=CARTESIAN_POINT('Ctrl Pts',(-43.4735820751074,33.332034495862,-39.5435958333333));
#256391=CARTESIAN_POINT('Ctrl Pts',(-44.5079524583201,33.9292285150516,
-39.4852625));
#256392=CARTESIAN_POINT('Ctrl Pts',(-45.5423228415328,33.332034495862,-39.4269291666667));
#256393=CARTESIAN_POINT('Ctrl Pts',(-46.5766932247455,32.7348404766724,
-39.3685958333334));
#256394=CARTESIAN_POINT('Ctrl Pts',(-46.5766932247455,31.5404524382932,
-39.3102625));
#256395=CARTESIAN_POINT('Ctrl Pts',(-46.5766932247455,30.3460643999139,
-39.2519291666667));
#256396=CARTESIAN_POINT('Ctrl Pts',(-45.5423228415329,29.7488703807243,
-39.1935958333334));
#256397=CARTESIAN_POINT('Ctrl Pts',(-44.5079524583202,29.1516763615346,
-39.1352625));
#256398=CARTESIAN_POINT('Ctrl Pts',(-43.4735820751074,29.7488703807243,
-39.0769291666667));
#256399=CARTESIAN_POINT('Ctrl Pts',(-42.4392116918948,30.3460643999138,
-39.0185958333333));
#256400=CARTESIAN_POINT('Ctrl Pts',(-42.4392116918948,31.5404524382931,
-38.9602625));
#256401=CARTESIAN_POINT('Ctrl Pts',(-42.4392116918948,32.7348404766723,
-38.9019291666667));
#256402=CARTESIAN_POINT('Ctrl Pts',(-43.4735820751074,33.332034495862,-38.8435958333333));
#256403=CARTESIAN_POINT('Ctrl Pts',(-44.5079524583201,33.9292285150516,
-38.7852625));
#256404=CARTESIAN_POINT('Ctrl Pts',(-45.5423228415328,33.332034495862,-38.7269291666667));
#256405=CARTESIAN_POINT('Ctrl Pts',(-46.5766932247455,32.7348404766724,
-38.6685958333334));
#256406=CARTESIAN_POINT('Ctrl Pts',(-46.5766932247455,31.5404524382932,
-38.6102625));
#256407=CARTESIAN_POINT('Ctrl Pts',(-46.5766932247455,30.3460643999139,
-38.5519291666667));
#256408=CARTESIAN_POINT('Ctrl Pts',(-45.5423228415329,29.7488703807243,
-38.4935958333334));
#256409=CARTESIAN_POINT('Ctrl Pts',(-44.5079524583202,29.1516763615346,
-38.4352625));
#256410=CARTESIAN_POINT('Ctrl Pts',(-43.4735820751074,29.7488703807243,
-38.3769291666666));
#256411=CARTESIAN_POINT('Ctrl Pts',(-42.4392116918948,30.3460643999138,
-38.3185958333333));
#256412=CARTESIAN_POINT('Ctrl Pts',(-42.4392116918948,31.5404524382931,
-38.2602625));
#256413=CARTESIAN_POINT('Ctrl Pts',(-42.4392116918948,32.7348404766723,
-38.2019291666667));
#256414=CARTESIAN_POINT('Ctrl Pts',(-43.4735820751074,33.332034495862,-38.1435958333334));
#256415=CARTESIAN_POINT('Ctrl Pts',(-44.5079524583201,33.9292285150516,
-38.0852625));
#256416=CARTESIAN_POINT('Ctrl Pts',(-45.5423228415328,33.332034495862,-38.0269291666667));
#256417=CARTESIAN_POINT('Ctrl Pts',(-46.5766932247455,32.7348404766724,
-37.9685958333333));
#256418=CARTESIAN_POINT('Ctrl Pts',(-46.5766932247455,31.5404524382932,
-37.9102625));
#256419=CARTESIAN_POINT('Ctrl Pts',(-46.5766932247455,30.3460643999139,
-37.8519291666667));
#256420=CARTESIAN_POINT('Ctrl Pts',(-45.5423228415329,29.7488703807243,
-37.7935958333334));
#256421=CARTESIAN_POINT('Ctrl Pts',(-44.5079524583202,29.1516763615346,
-37.7352625));
#256422=CARTESIAN_POINT('Ctrl Pts',(-43.4735820751074,29.7488703807243,
-37.6769291666667));
#256423=CARTESIAN_POINT('Ctrl Pts',(-42.4392116918948,30.3460643999138,
-37.6185958333333));
#256424=CARTESIAN_POINT('Ctrl Pts',(-42.4392116918948,31.5404524382931,
-37.5602625));
#256425=CARTESIAN_POINT('Ctrl Pts',(-42.4392116918948,32.7348404766723,
-37.5019291666666));
#256426=CARTESIAN_POINT('Ctrl Pts',(-43.4735820751074,33.332034495862,-37.4435958333333));
#256427=CARTESIAN_POINT('Ctrl Pts',(-44.5079524583201,33.9292285150516,
-37.3852625));
#256428=CARTESIAN_POINT('Ctrl Pts',(-45.5423228415328,33.332034495862,-37.3269291666667));
#256429=CARTESIAN_POINT('Ctrl Pts',(-46.5766932247455,32.7348404766724,
-37.2685958333333));
#256430=CARTESIAN_POINT('Ctrl Pts',(-46.5766932247455,31.5404524382932,
-37.2102625));
#256431=CARTESIAN_POINT('Ctrl Pts',(-46.5766932247455,30.3460643999139,
-37.1519291666667));
#256432=CARTESIAN_POINT('Ctrl Pts',(-45.5423228415329,29.7488703807243,
-37.0935958333333));
#256433=CARTESIAN_POINT('Ctrl Pts',(-44.5079524583202,29.1516763615346,
-37.0352625));
#256434=CARTESIAN_POINT('Ctrl Pts',(-43.4735820751074,29.7488703807243,
-36.9769291666667));
#256435=CARTESIAN_POINT('Ctrl Pts',(-42.4392116918948,30.3460643999138,
-36.9185958333333));
#256436=CARTESIAN_POINT('Ctrl Pts',(-42.4392116918948,31.5404524382931,
-36.8602625));
#256437=CARTESIAN_POINT('Ctrl Pts',(-42.4392116918948,32.7348404766723,
-36.8019291666666));
#256438=CARTESIAN_POINT('Ctrl Pts',(-43.4735820751074,33.332034495862,-36.7435958333334));
#256439=CARTESIAN_POINT('Ctrl Pts',(-44.5079524583201,33.9292285150516,
-36.6852625));
#256440=CARTESIAN_POINT('Ctrl Pts',(-45.5423228415328,33.332034495862,-36.6269291666666));
#256441=CARTESIAN_POINT('Ctrl Pts',(-45.6766051604214,33.2545065629043,
-36.6193563132714));
#256442=CARTESIAN_POINT('Ctrl Pts',(-45.7978303778612,33.1578278775004,
-36.611216324118));
#256443=CARTESIAN_POINT('Ctrl Pts',(-46.1766977413726,31.5404524382932,
-52.8412));
#256444=CARTESIAN_POINT('Ctrl Pts',(-46.1766977413726,30.5770018999139,
-52.7828666666667));
#256445=CARTESIAN_POINT('Ctrl Pts',(-45.3423250998464,30.0952766307242,
-52.7245333333334));
#256446=CARTESIAN_POINT('Ctrl Pts',(-44.5079524583202,29.6135513615346,
-52.6662));
#256447=CARTESIAN_POINT('Ctrl Pts',(-43.6735798167939,30.0952766307242,
-52.6078666666667));
#256448=CARTESIAN_POINT('Ctrl Pts',(-42.8392071752677,30.5770018999139,
-52.5495333333333));
#256449=CARTESIAN_POINT('Ctrl Pts',(-42.8392071752677,31.5404524382931,
-52.4912));
#256450=CARTESIAN_POINT('Ctrl Pts',(-42.8392071752677,32.5039029766724,
-52.4328666666667));
#256451=CARTESIAN_POINT('Ctrl Pts',(-43.6735798167939,32.985628245862,-52.3745333333334));
#256452=CARTESIAN_POINT('Ctrl Pts',(-44.5079524583201,33.4673535150516,
-52.3162000000001));
#256453=CARTESIAN_POINT('Ctrl Pts',(-45.3423250998464,32.985628245862,-52.2578666666667));
#256454=CARTESIAN_POINT('Ctrl Pts',(-46.1766977413726,32.5039029766724,
-52.1995333333334));
#256455=CARTESIAN_POINT('Ctrl Pts',(-46.1766977413726,31.5404524382932,
-52.1412));
#256456=CARTESIAN_POINT('Ctrl Pts',(-46.1766977413726,30.5770018999139,
-52.0828666666667));
#256457=CARTESIAN_POINT('Ctrl Pts',(-45.3423250998464,30.0952766307242,
-52.0245333333333));
#256458=CARTESIAN_POINT('Ctrl Pts',(-44.5079524583202,29.6135513615346,
-51.9662));
#256459=CARTESIAN_POINT('Ctrl Pts',(-43.6735798167939,30.0952766307242,
-51.9078666666667));
#256460=CARTESIAN_POINT('Ctrl Pts',(-42.8392071752677,30.5770018999139,
-51.8495333333334));
#256461=CARTESIAN_POINT('Ctrl Pts',(-42.8392071752677,31.5404524382931,
-51.7912));
#256462=CARTESIAN_POINT('Ctrl Pts',(-42.8392071752677,32.5039029766724,
-51.7328666666667));
#256463=CARTESIAN_POINT('Ctrl Pts',(-43.6735798167939,32.985628245862,-51.6745333333333));
#256464=CARTESIAN_POINT('Ctrl Pts',(-44.5079524583201,33.4673535150516,
-51.6162));
#256465=CARTESIAN_POINT('Ctrl Pts',(-45.3423250998464,32.985628245862,-51.5578666666667));
#256466=CARTESIAN_POINT('Ctrl Pts',(-46.1766977413726,32.5039029766724,
-51.4995333333333));
#256467=CARTESIAN_POINT('Ctrl Pts',(-46.1766977413726,31.5404524382932,
-51.4412));
#256468=CARTESIAN_POINT('Ctrl Pts',(-46.1766977413726,30.5770018999139,
-51.3828666666667));
#256469=CARTESIAN_POINT('Ctrl Pts',(-45.3423250998464,30.0952766307242,
-51.3245333333334));
#256470=CARTESIAN_POINT('Ctrl Pts',(-44.5079524583202,29.6135513615346,
-51.2662));
#256471=CARTESIAN_POINT('Ctrl Pts',(-43.6735798167939,30.0952766307242,
-51.2078666666667));
#256472=CARTESIAN_POINT('Ctrl Pts',(-42.8392071752677,30.5770018999139,
-51.1495333333333));
#256473=CARTESIAN_POINT('Ctrl Pts',(-42.8392071752677,31.5404524382931,
-51.0912));
#256474=CARTESIAN_POINT('Ctrl Pts',(-42.8392071752677,32.5039029766724,
-51.0328666666667));
#256475=CARTESIAN_POINT('Ctrl Pts',(-43.6735798167939,32.985628245862,-50.9745333333333));
#256476=CARTESIAN_POINT('Ctrl Pts',(-44.5079524583201,33.4673535150516,
-50.9162));
#256477=CARTESIAN_POINT('Ctrl Pts',(-45.3423250998464,32.985628245862,-50.8578666666667));
#256478=CARTESIAN_POINT('Ctrl Pts',(-46.1766977413726,32.5039029766724,
-50.7995333333333));
#256479=CARTESIAN_POINT('Ctrl Pts',(-46.1766977413726,31.5404524382932,
-50.7412));
#256480=CARTESIAN_POINT('Ctrl Pts',(-46.1766977413726,30.5770018999139,
-50.6828666666667));
#256481=CARTESIAN_POINT('Ctrl Pts',(-45.3423250998464,30.0952766307242,
-50.6245333333333));
#256482=CARTESIAN_POINT('Ctrl Pts',(-44.5079524583202,29.6135513615346,
-50.5662));
#256483=CARTESIAN_POINT('Ctrl Pts',(-43.6735798167939,30.0952766307242,
-50.5078666666667));
#256484=CARTESIAN_POINT('Ctrl Pts',(-42.8392071752677,30.5770018999139,
-50.4495333333333));
#256485=CARTESIAN_POINT('Ctrl Pts',(-42.8392071752677,31.5404524382931,
-50.3912));
#256486=CARTESIAN_POINT('Ctrl Pts',(-42.8392071752677,32.5039029766724,
-50.3328666666666));
#256487=CARTESIAN_POINT('Ctrl Pts',(-43.6735798167939,32.985628245862,-50.2745333333333));
#256488=CARTESIAN_POINT('Ctrl Pts',(-44.5079524583201,33.4673535150516,
-50.2162));
#256489=CARTESIAN_POINT('Ctrl Pts',(-45.3423250998464,32.985628245862,-50.1578666666667));
#256490=CARTESIAN_POINT('Ctrl Pts',(-46.1766977413726,32.5039029766724,
-50.0995333333333));
#256491=CARTESIAN_POINT('Ctrl Pts',(-46.1766977413726,31.5404524382932,
-50.0412));
#256492=CARTESIAN_POINT('Ctrl Pts',(-46.1766977413726,30.5770018999139,
-49.9828666666667));
#256493=CARTESIAN_POINT('Ctrl Pts',(-45.3423250998464,30.0952766307242,
-49.9245333333334));
#256494=CARTESIAN_POINT('Ctrl Pts',(-44.5079524583202,29.6135513615346,
-49.8662));
#256495=CARTESIAN_POINT('Ctrl Pts',(-43.6735798167939,30.0952766307242,
-49.8078666666667));
#256496=CARTESIAN_POINT('Ctrl Pts',(-42.8392071752677,30.5770018999139,
-49.7495333333333));
#256497=CARTESIAN_POINT('Ctrl Pts',(-42.8392071752677,31.5404524382931,
-49.6912));
#256498=CARTESIAN_POINT('Ctrl Pts',(-42.8392071752677,32.5039029766724,
-49.6328666666667));
#256499=CARTESIAN_POINT('Ctrl Pts',(-43.6735798167939,32.985628245862,-49.5745333333333));
#256500=CARTESIAN_POINT('Ctrl Pts',(-44.5079524583201,33.4673535150516,
-49.5162));
#256501=CARTESIAN_POINT('Ctrl Pts',(-45.3423250998464,32.985628245862,-49.4578666666667));
#256502=CARTESIAN_POINT('Ctrl Pts',(-46.1766977413726,32.5039029766724,
-49.3995333333333));
#256503=CARTESIAN_POINT('Ctrl Pts',(-46.1766977413726,31.5404524382932,
-49.3412));
#256504=CARTESIAN_POINT('Ctrl Pts',(-46.1766977413726,30.5770018999139,
-49.2828666666666));
#256505=CARTESIAN_POINT('Ctrl Pts',(-45.3423250998464,30.0952766307242,
-49.2245333333333));
#256506=CARTESIAN_POINT('Ctrl Pts',(-44.5079524583202,29.6135513615346,
-49.1662));
#256507=CARTESIAN_POINT('Ctrl Pts',(-43.6735798167939,30.0952766307242,
-49.1078666666667));
#256508=CARTESIAN_POINT('Ctrl Pts',(-42.8392071752677,30.5770018999139,
-49.0495333333334));
#256509=CARTESIAN_POINT('Ctrl Pts',(-42.8392071752677,31.5404524382931,
-48.9912));
#256510=CARTESIAN_POINT('Ctrl Pts',(-42.8392071752677,32.5039029766724,
-48.9328666666667));
#256511=CARTESIAN_POINT('Ctrl Pts',(-43.6735798167939,32.985628245862,-48.8745333333333));
#256512=CARTESIAN_POINT('Ctrl Pts',(-44.5079524583201,33.4673535150516,
-48.8162));
#256513=CARTESIAN_POINT('Ctrl Pts',(-45.3423250998464,32.985628245862,-48.7578666666667));
#256514=CARTESIAN_POINT('Ctrl Pts',(-46.1766977413726,32.5039029766724,
-48.6995333333334));
#256515=CARTESIAN_POINT('Ctrl Pts',(-46.1766977413726,31.5404524382932,
-48.6412));
#256516=CARTESIAN_POINT('Ctrl Pts',(-46.1766977413726,30.5770018999139,
-48.5828666666667));
#256517=CARTESIAN_POINT('Ctrl Pts',(-45.3423250998464,30.0952766307242,
-48.5245333333333));
#256518=CARTESIAN_POINT('Ctrl Pts',(-44.5079524583202,29.6135513615346,
-48.4662));
#256519=CARTESIAN_POINT('Ctrl Pts',(-43.6735798167939,30.0952766307242,
-48.4078666666667));
#256520=CARTESIAN_POINT('Ctrl Pts',(-42.8392071752677,30.5770018999139,
-48.3495333333333));
#256521=CARTESIAN_POINT('Ctrl Pts',(-42.8392071752677,31.5404524382931,
-48.2912));
#256522=CARTESIAN_POINT('Ctrl Pts',(-42.8392071752677,32.5039029766724,
-48.2328666666667));
#256523=CARTESIAN_POINT('Ctrl Pts',(-43.6735798167939,32.985628245862,-48.1745333333334));
#256524=CARTESIAN_POINT('Ctrl Pts',(-44.5079524583201,33.4673535150516,
-48.1162));
#256525=CARTESIAN_POINT('Ctrl Pts',(-45.3423250998464,32.985628245862,-48.0578666666667));
#256526=CARTESIAN_POINT('Ctrl Pts',(-46.1766977413726,32.5039029766724,
-47.9995333333334));
#256527=CARTESIAN_POINT('Ctrl Pts',(-46.1766977413726,31.5404524382932,
-47.9412));
#256528=CARTESIAN_POINT('Ctrl Pts',(-46.1766977413726,30.5770018999139,
-47.8828666666667));
#256529=CARTESIAN_POINT('Ctrl Pts',(-45.3423250998464,30.0952766307242,
-47.8245333333333));
#256530=CARTESIAN_POINT('Ctrl Pts',(-44.5079524583202,29.6135513615346,
-47.7662));
#256531=CARTESIAN_POINT('Ctrl Pts',(-43.6735798167939,30.0952766307242,
-47.7078666666667));
#256532=CARTESIAN_POINT('Ctrl Pts',(-42.8392071752677,30.5770018999139,
-47.6495333333334));
#256533=CARTESIAN_POINT('Ctrl Pts',(-42.8392071752677,31.5404524382931,
-47.5912));
#256534=CARTESIAN_POINT('Ctrl Pts',(-42.8392071752677,32.5039029766724,
-47.5328666666667));
#256535=CARTESIAN_POINT('Ctrl Pts',(-43.6735798167939,32.985628245862,-47.4745333333334));
#256536=CARTESIAN_POINT('Ctrl Pts',(-44.5079524583201,33.4673535150516,
-47.4162));
#256537=CARTESIAN_POINT('Ctrl Pts',(-45.3423250998464,32.985628245862,-47.3578666666667));
#256538=CARTESIAN_POINT('Ctrl Pts',(-46.1766977413726,32.5039029766724,
-47.2995333333334));
#256539=CARTESIAN_POINT('Ctrl Pts',(-46.1766977413726,31.5404524382932,
-47.2412));
#256540=CARTESIAN_POINT('Ctrl Pts',(-46.1766977413726,30.5770018999139,
-47.1828666666667));
#256541=CARTESIAN_POINT('Ctrl Pts',(-45.3423250998464,30.0952766307242,
-47.1245333333333));
#256542=CARTESIAN_POINT('Ctrl Pts',(-44.5079524583202,29.6135513615346,
-47.0662));
#256543=CARTESIAN_POINT('Ctrl Pts',(-43.6735798167939,30.0952766307242,
-47.0078666666667));
#256544=CARTESIAN_POINT('Ctrl Pts',(-42.8392071752677,30.5770018999139,
-46.9495333333334));
#256545=CARTESIAN_POINT('Ctrl Pts',(-42.8392071752677,31.5404524382931,
-46.8912));
#256546=CARTESIAN_POINT('Ctrl Pts',(-42.8392071752677,32.5039029766724,
-46.8328666666667));
#256547=CARTESIAN_POINT('Ctrl Pts',(-43.6735798167939,32.985628245862,-46.7745333333333));
#256548=CARTESIAN_POINT('Ctrl Pts',(-44.5079524583201,33.4673535150516,
-46.7162));
#256549=CARTESIAN_POINT('Ctrl Pts',(-45.3423250998464,32.985628245862,-46.6578666666667));
#256550=CARTESIAN_POINT('Ctrl Pts',(-46.1766977413726,32.5039029766724,
-46.5995333333333));
#256551=CARTESIAN_POINT('Ctrl Pts',(-46.1766977413726,31.5404524382932,
-46.5412));
#256552=CARTESIAN_POINT('Ctrl Pts',(-46.1766977413726,30.5770018999139,
-46.4828666666667));
#256553=CARTESIAN_POINT('Ctrl Pts',(-45.3423250998464,30.0952766307242,
-46.4245333333333));
#256554=CARTESIAN_POINT('Ctrl Pts',(-44.5079524583202,29.6135513615346,
-46.3662));
#256555=CARTESIAN_POINT('Ctrl Pts',(-43.6735798167939,30.0952766307242,
-46.3078666666667));
#256556=CARTESIAN_POINT('Ctrl Pts',(-42.8392071752677,30.5770018999139,
-46.2495333333334));
#256557=CARTESIAN_POINT('Ctrl Pts',(-42.8392071752677,31.5404524382931,
-46.1912));
#256558=CARTESIAN_POINT('Ctrl Pts',(-42.8392071752677,32.5039029766724,
-46.1328666666667));
#256559=CARTESIAN_POINT('Ctrl Pts',(-43.6735798167939,32.985628245862,-46.0745333333334));
#256560=CARTESIAN_POINT('Ctrl Pts',(-44.5079524583201,33.4673535150516,
-46.0162));
#256561=CARTESIAN_POINT('Ctrl Pts',(-45.3423250998464,32.985628245862,-45.9578666666667));
#256562=CARTESIAN_POINT('Ctrl Pts',(-46.1766977413726,32.5039029766724,
-45.8995333333333));
#256563=CARTESIAN_POINT('Ctrl Pts',(-46.1766977413726,31.5404524382932,
-45.8412));
#256564=CARTESIAN_POINT('Ctrl Pts',(-46.1766977413726,30.5770018999139,
-45.7828666666667));
#256565=CARTESIAN_POINT('Ctrl Pts',(-45.3423250998464,30.0952766307242,
-45.7245333333333));
#256566=CARTESIAN_POINT('Ctrl Pts',(-44.5079524583202,29.6135513615346,
-45.6662));
#256567=CARTESIAN_POINT('Ctrl Pts',(-43.6735798167939,30.0952766307242,
-45.6078666666667));
#256568=CARTESIAN_POINT('Ctrl Pts',(-42.8392071752677,30.5770018999139,
-45.5495333333333));
#256569=CARTESIAN_POINT('Ctrl Pts',(-42.8392071752677,31.5404524382931,
-45.4912));
#256570=CARTESIAN_POINT('Ctrl Pts',(-42.8392071752677,32.5039029766724,
-45.4328666666666));
#256571=CARTESIAN_POINT('Ctrl Pts',(-43.6735798167939,32.985628245862,-45.3745333333333));
#256572=CARTESIAN_POINT('Ctrl Pts',(-44.5079524583201,33.4673535150516,
-45.3162));
#256573=CARTESIAN_POINT('Ctrl Pts',(-45.3423250998464,32.985628245862,-45.2578666666667));
#256574=CARTESIAN_POINT('Ctrl Pts',(-46.1766977413726,32.5039029766724,
-45.1995333333333));
#256575=CARTESIAN_POINT('Ctrl Pts',(-46.1766977413726,31.5404524382932,
-45.1412));
#256576=CARTESIAN_POINT('Ctrl Pts',(-46.1766977413726,30.5770018999139,
-45.0828666666667));
#256577=CARTESIAN_POINT('Ctrl Pts',(-45.3423250998464,30.0952766307242,
-45.0245333333333));
#256578=CARTESIAN_POINT('Ctrl Pts',(-44.5079524583202,29.6135513615346,
-44.9662));
#256579=CARTESIAN_POINT('Ctrl Pts',(-43.6735798167939,30.0952766307242,
-44.9078666666666));
#256580=CARTESIAN_POINT('Ctrl Pts',(-42.8392071752677,30.5770018999139,
-44.8495333333333));
#256581=CARTESIAN_POINT('Ctrl Pts',(-42.8392071752677,31.5404524382931,
-44.7912));
#256582=CARTESIAN_POINT('Ctrl Pts',(-42.8392071752677,32.5039029766724,
-44.7328666666666));
#256583=CARTESIAN_POINT('Ctrl Pts',(-43.6735798167939,32.985628245862,-44.6745333333334));
#256584=CARTESIAN_POINT('Ctrl Pts',(-44.5079524583201,33.4673535150516,
-44.6162));
#256585=CARTESIAN_POINT('Ctrl Pts',(-45.3423250998464,32.985628245862,-44.5578666666667));
#256586=CARTESIAN_POINT('Ctrl Pts',(-46.1766977413726,32.5039029766724,
-44.4995333333333));
#256587=CARTESIAN_POINT('Ctrl Pts',(-46.1766977413726,31.5404524382932,
-44.4412));
#256588=CARTESIAN_POINT('Ctrl Pts',(-46.1766977413726,30.5770018999139,
-44.3828666666667));
#256589=CARTESIAN_POINT('Ctrl Pts',(-45.3423250998464,30.0952766307242,
-44.3245333333334));
#256590=CARTESIAN_POINT('Ctrl Pts',(-44.5079524583202,29.6135513615346,
-44.2662));
#256591=CARTESIAN_POINT('Ctrl Pts',(-43.6735798167939,30.0952766307242,
-44.2078666666667));
#256592=CARTESIAN_POINT('Ctrl Pts',(-42.8392071752677,30.5770018999139,
-44.1495333333334));
#256593=CARTESIAN_POINT('Ctrl Pts',(-42.8392071752677,31.5404524382931,
-44.0912));
#256594=CARTESIAN_POINT('Ctrl Pts',(-42.8392071752677,32.5039029766724,
-44.0328666666667));
#256595=CARTESIAN_POINT('Ctrl Pts',(-43.6735798167939,32.985628245862,-43.9745333333333));
#256596=CARTESIAN_POINT('Ctrl Pts',(-44.5079524583201,33.4673535150516,
-43.9162));
#256597=CARTESIAN_POINT('Ctrl Pts',(-45.3423250998464,32.985628245862,-43.8578666666667));
#256598=CARTESIAN_POINT('Ctrl Pts',(-46.1766977413726,32.5039029766724,
-43.7995333333334));
#256599=CARTESIAN_POINT('Ctrl Pts',(-46.1766977413726,31.5404524382932,
-43.7412));
#256600=CARTESIAN_POINT('Ctrl Pts',(-46.1766977413726,30.5770018999139,
-43.6828666666667));
#256601=CARTESIAN_POINT('Ctrl Pts',(-45.3423250998464,30.0952766307242,
-43.6245333333333));
#256602=CARTESIAN_POINT('Ctrl Pts',(-44.5079524583202,29.6135513615346,
-43.5662));
#256603=CARTESIAN_POINT('Ctrl Pts',(-43.6735798167939,30.0952766307242,
-43.5078666666667));
#256604=CARTESIAN_POINT('Ctrl Pts',(-42.8392071752677,30.5770018999139,
-43.4495333333334));
#256605=CARTESIAN_POINT('Ctrl Pts',(-42.8392071752677,31.5404524382931,
-43.3912));
#256606=CARTESIAN_POINT('Ctrl Pts',(-42.8392071752677,32.5039029766724,
-43.3328666666667));
#256607=CARTESIAN_POINT('Ctrl Pts',(-43.6735798167939,32.985628245862,-43.2745333333334));
#256608=CARTESIAN_POINT('Ctrl Pts',(-44.5079524583201,33.4673535150516,
-43.2162));
#256609=CARTESIAN_POINT('Ctrl Pts',(-45.3423250998464,32.985628245862,-43.1578666666667));
#256610=CARTESIAN_POINT('Ctrl Pts',(-46.1766977413726,32.5039029766724,
-43.0995333333334));
#256611=CARTESIAN_POINT('Ctrl Pts',(-46.1766977413726,31.5404524382932,
-43.0412));
#256612=CARTESIAN_POINT('Ctrl Pts',(-46.1766977413726,30.5770018999139,
-42.9828666666667));
#256613=CARTESIAN_POINT('Ctrl Pts',(-45.3423250998464,30.0952766307242,
-42.9245333333334));
#256614=CARTESIAN_POINT('Ctrl Pts',(-44.5079524583202,29.6135513615346,
-42.8662));
#256615=CARTESIAN_POINT('Ctrl Pts',(-43.6735798167939,30.0952766307242,
-42.8078666666667));
#256616=CARTESIAN_POINT('Ctrl Pts',(-42.8392071752677,30.5770018999139,
-42.7495333333334));
#256617=CARTESIAN_POINT('Ctrl Pts',(-42.8392071752677,31.5404524382931,
-42.6912));
#256618=CARTESIAN_POINT('Ctrl Pts',(-42.8392071752677,32.5039029766724,
-42.6328666666667));
#256619=CARTESIAN_POINT('Ctrl Pts',(-43.6735798167939,32.985628245862,-42.5745333333333));
#256620=CARTESIAN_POINT('Ctrl Pts',(-44.5079524583201,33.4673535150516,
-42.5162));
#256621=CARTESIAN_POINT('Ctrl Pts',(-45.3423250998464,32.985628245862,-42.4578666666667));
#256622=CARTESIAN_POINT('Ctrl Pts',(-46.1766977413726,32.5039029766724,
-42.3995333333334));
#256623=CARTESIAN_POINT('Ctrl Pts',(-46.1766977413726,31.5404524382932,
-42.3412));
#256624=CARTESIAN_POINT('Ctrl Pts',(-46.1766977413726,30.5770018999139,
-42.2828666666667));
#256625=CARTESIAN_POINT('Ctrl Pts',(-45.3423250998464,30.0952766307242,
-42.2245333333333));
#256626=CARTESIAN_POINT('Ctrl Pts',(-44.5079524583202,29.6135513615346,
-42.1662));
#256627=CARTESIAN_POINT('Ctrl Pts',(-43.6735798167939,30.0952766307242,
-42.1078666666667));
#256628=CARTESIAN_POINT('Ctrl Pts',(-42.8392071752677,30.5770018999139,
-42.0495333333334));
#256629=CARTESIAN_POINT('Ctrl Pts',(-42.8392071752677,31.5404524382931,
-41.9912));
#256630=CARTESIAN_POINT('Ctrl Pts',(-42.8392071752677,32.5039029766724,
-41.9328666666667));
#256631=CARTESIAN_POINT('Ctrl Pts',(-43.6735798167939,32.985628245862,-41.8745333333334));
#256632=CARTESIAN_POINT('Ctrl Pts',(-44.5079524583201,33.4673535150516,
-41.8162));
#256633=CARTESIAN_POINT('Ctrl Pts',(-45.3423250998464,32.985628245862,-41.7578666666667));
#256634=CARTESIAN_POINT('Ctrl Pts',(-46.1766977413726,32.5039029766724,
-41.6995333333333));
#256635=CARTESIAN_POINT('Ctrl Pts',(-46.1766977413726,31.5404524382932,
-41.6412));
#256636=CARTESIAN_POINT('Ctrl Pts',(-46.1766977413726,30.5770018999139,
-41.5828666666667));
#256637=CARTESIAN_POINT('Ctrl Pts',(-45.3423250998464,30.0952766307242,
-41.5245333333334));
#256638=CARTESIAN_POINT('Ctrl Pts',(-44.5079524583202,29.6135513615346,
-41.4662));
#256639=CARTESIAN_POINT('Ctrl Pts',(-43.6735798167939,30.0952766307242,
-41.4078666666667));
#256640=CARTESIAN_POINT('Ctrl Pts',(-42.8392071752677,30.5770018999139,
-41.3495333333333));
#256641=CARTESIAN_POINT('Ctrl Pts',(-42.8392071752677,31.5404524382931,
-41.2912));
#256642=CARTESIAN_POINT('Ctrl Pts',(-42.8392071752677,32.5039029766724,
-41.2328666666667));
#256643=CARTESIAN_POINT('Ctrl Pts',(-43.6735798167939,32.985628245862,-41.1745333333334));
#256644=CARTESIAN_POINT('Ctrl Pts',(-44.5079524583201,33.4673535150516,
-41.1162));
#256645=CARTESIAN_POINT('Ctrl Pts',(-45.3423250998464,32.985628245862,-41.0578666666667));
#256646=CARTESIAN_POINT('Ctrl Pts',(-46.1766977413726,32.5039029766724,
-40.9995333333333));
#256647=CARTESIAN_POINT('Ctrl Pts',(-46.1766977413726,31.5404524382932,
-40.9412));
#256648=CARTESIAN_POINT('Ctrl Pts',(-46.1766977413726,30.5770018999139,
-40.8828666666667));
#256649=CARTESIAN_POINT('Ctrl Pts',(-45.3423250998464,30.0952766307242,
-40.8245333333333));
#256650=CARTESIAN_POINT('Ctrl Pts',(-44.5079524583202,29.6135513615346,
-40.7662));
#256651=CARTESIAN_POINT('Ctrl Pts',(-43.6735798167939,30.0952766307242,
-40.7078666666667));
#256652=CARTESIAN_POINT('Ctrl Pts',(-42.8392071752677,30.5770018999139,
-40.6495333333333));
#256653=CARTESIAN_POINT('Ctrl Pts',(-42.8392071752677,31.5404524382931,
-40.5912));
#256654=CARTESIAN_POINT('Ctrl Pts',(-42.8392071752677,32.5039029766724,
-40.5328666666667));
#256655=CARTESIAN_POINT('Ctrl Pts',(-43.6735798167939,32.985628245862,-40.4745333333334));
#256656=CARTESIAN_POINT('Ctrl Pts',(-44.5079524583201,33.4673535150516,
-40.4162));
#256657=CARTESIAN_POINT('Ctrl Pts',(-45.3423250998464,32.985628245862,-40.3578666666667));
#256658=CARTESIAN_POINT('Ctrl Pts',(-46.1766977413726,32.5039029766724,
-40.2995333333333));
#256659=CARTESIAN_POINT('Ctrl Pts',(-46.1766977413726,31.5404524382932,
-40.2412));
#256660=CARTESIAN_POINT('Ctrl Pts',(-46.1766977413726,30.5770018999139,
-40.1828666666667));
#256661=CARTESIAN_POINT('Ctrl Pts',(-45.3423250998464,30.0952766307242,
-40.1245333333334));
#256662=CARTESIAN_POINT('Ctrl Pts',(-44.5079524583202,29.6135513615346,
-40.0662));
#256663=CARTESIAN_POINT('Ctrl Pts',(-43.6735798167939,30.0952766307242,
-40.0078666666667));
#256664=CARTESIAN_POINT('Ctrl Pts',(-42.8392071752677,30.5770018999139,
-39.9495333333333));
#256665=CARTESIAN_POINT('Ctrl Pts',(-42.8392071752677,31.5404524382931,
-39.8912));
#256666=CARTESIAN_POINT('Ctrl Pts',(-42.8392071752677,32.5039029766724,
-39.8328666666666));
#256667=CARTESIAN_POINT('Ctrl Pts',(-43.6735798167939,32.985628245862,-39.7745333333334));
#256668=CARTESIAN_POINT('Ctrl Pts',(-44.5079524583201,33.4673535150516,
-39.7162));
#256669=CARTESIAN_POINT('Ctrl Pts',(-45.3423250998464,32.985628245862,-39.6578666666667));
#256670=CARTESIAN_POINT('Ctrl Pts',(-46.1766977413726,32.5039029766724,
-39.5995333333333));
#256671=CARTESIAN_POINT('Ctrl Pts',(-46.1766977413726,31.5404524382932,
-39.5412));
#256672=CARTESIAN_POINT('Ctrl Pts',(-46.1766977413726,30.5770018999139,
-39.4828666666666));
#256673=CARTESIAN_POINT('Ctrl Pts',(-45.3423250998464,30.0952766307242,
-39.4245333333334));
#256674=CARTESIAN_POINT('Ctrl Pts',(-44.5079524583202,29.6135513615346,
-39.3662));
#256675=CARTESIAN_POINT('Ctrl Pts',(-43.6735798167939,30.0952766307242,
-39.3078666666666));
#256676=CARTESIAN_POINT('Ctrl Pts',(-42.8392071752677,30.5770018999139,
-39.2495333333333));
#256677=CARTESIAN_POINT('Ctrl Pts',(-42.8392071752677,31.5404524382931,
-39.1912));
#256678=CARTESIAN_POINT('Ctrl Pts',(-42.8392071752677,32.5039029766724,
-39.1328666666667));
#256679=CARTESIAN_POINT('Ctrl Pts',(-43.6735798167939,32.985628245862,-39.0745333333333));
#256680=CARTESIAN_POINT('Ctrl Pts',(-44.5079524583201,33.4673535150516,
-39.0162));
#256681=CARTESIAN_POINT('Ctrl Pts',(-45.3423250998464,32.985628245862,-38.9578666666667));
#256682=CARTESIAN_POINT('Ctrl Pts',(-46.1766977413726,32.5039029766724,
-38.8995333333334));
#256683=CARTESIAN_POINT('Ctrl Pts',(-46.1766977413726,31.5404524382932,
-38.8412));
#256684=CARTESIAN_POINT('Ctrl Pts',(-46.1766977413726,30.5770018999139,
-38.7828666666667));
#256685=CARTESIAN_POINT('Ctrl Pts',(-45.3423250998464,30.0952766307242,
-38.7245333333334));
#256686=CARTESIAN_POINT('Ctrl Pts',(-44.5079524583202,29.6135513615346,
-38.6662));
#256687=CARTESIAN_POINT('Ctrl Pts',(-43.6735798167939,30.0952766307242,
-38.6078666666667));
#256688=CARTESIAN_POINT('Ctrl Pts',(-42.8392071752677,30.5770018999139,
-38.5495333333334));
#256689=CARTESIAN_POINT('Ctrl Pts',(-42.8392071752677,31.5404524382931,
-38.4912));
#256690=CARTESIAN_POINT('Ctrl Pts',(-42.8392071752677,32.5039029766724,
-38.4328666666667));
#256691=CARTESIAN_POINT('Ctrl Pts',(-43.6735798167939,32.985628245862,-38.3745333333333));
#256692=CARTESIAN_POINT('Ctrl Pts',(-44.5079524583201,33.4673535150516,
-38.3162));
#256693=CARTESIAN_POINT('Ctrl Pts',(-45.3423250998464,32.985628245862,-38.2578666666667));
#256694=CARTESIAN_POINT('Ctrl Pts',(-46.1766977413726,32.5039029766724,
-38.1995333333333));
#256695=CARTESIAN_POINT('Ctrl Pts',(-46.1766977413726,31.5404524382932,
-38.1412));
#256696=CARTESIAN_POINT('Ctrl Pts',(-46.1766977413726,30.5770018999139,
-38.0828666666667));
#256697=CARTESIAN_POINT('Ctrl Pts',(-45.3423250998464,30.0952766307242,
-38.0245333333334));
#256698=CARTESIAN_POINT('Ctrl Pts',(-44.5079524583202,29.6135513615346,
-37.9662));
#256699=CARTESIAN_POINT('Ctrl Pts',(-43.6735798167939,30.0952766307242,
-37.9078666666667));
#256700=CARTESIAN_POINT('Ctrl Pts',(-42.8392071752677,30.5770018999139,
-37.8495333333334));
#256701=CARTESIAN_POINT('Ctrl Pts',(-42.8392071752677,31.5404524382931,
-37.7912));
#256702=CARTESIAN_POINT('Ctrl Pts',(-42.8392071752677,32.5039029766724,
-37.7328666666667));
#256703=CARTESIAN_POINT('Ctrl Pts',(-43.6735798167939,32.985628245862,-37.6745333333334));
#256704=CARTESIAN_POINT('Ctrl Pts',(-44.5079524583201,33.4673535150516,
-37.6162));
#256705=CARTESIAN_POINT('Ctrl Pts',(-45.3423250998464,32.985628245862,-37.5578666666667));
#256706=CARTESIAN_POINT('Ctrl Pts',(-46.1766977413726,32.5039029766724,
-37.4995333333334));
#256707=CARTESIAN_POINT('Ctrl Pts',(-46.1766977413726,31.5404524382932,
-37.4412));
#256708=CARTESIAN_POINT('Ctrl Pts',(-46.1766977413726,30.5770018999139,
-37.3828666666667));
#256709=CARTESIAN_POINT('Ctrl Pts',(-45.3423250998464,30.0952766307242,
-37.3245333333333));
#256710=CARTESIAN_POINT('Ctrl Pts',(-44.5079524583202,29.6135513615346,
-37.2662));
#256711=CARTESIAN_POINT('Ctrl Pts',(-43.6735798167939,30.0952766307242,
-37.2078666666667));
#256712=CARTESIAN_POINT('Ctrl Pts',(-42.8392071752677,30.5770018999139,
-37.1495333333334));
#256713=CARTESIAN_POINT('Ctrl Pts',(-42.8392071752677,31.5404524382931,
-37.0912));
#256714=CARTESIAN_POINT('Ctrl Pts',(-42.8392071752677,32.5039029766724,
-37.0328666666667));
#256715=CARTESIAN_POINT('Ctrl Pts',(-43.6735798167939,32.985628245862,-36.9745333333333));
#256716=CARTESIAN_POINT('Ctrl Pts',(-44.5079524583201,33.4673535150516,
-36.9162));
#256717=CARTESIAN_POINT('Ctrl Pts',(-45.3423250998464,32.985628245862,-36.8578666666667));
#256718=CARTESIAN_POINT('Ctrl Pts',(-45.4506436431261,32.9230905057412,
-36.8502938132714));
#256719=CARTESIAN_POINT('Ctrl Pts',(-45.548429703648,32.8451048524115,-36.8421538241181));
#256720=CARTESIAN_POINT('Ctrl Pts',(-45.1065105640991,29.6321241563178,
-39.2098675790904));
#256721=CARTESIAN_POINT('Ctrl Pts',(-44.8761803077342,29.6051666105646,
-39.2221339827541));
#256722=CARTESIAN_POINT('Ctrl Pts',(-44.6436379954239,29.607165620836,-39.2270640528163));
#256723=CARTESIAN_POINT('Ctrl Pts',(-44.2077922427375,29.6727869442853,
-39.22565455626));
#256724=CARTESIAN_POINT('Ctrl Pts',(-44.0062031944438,29.7300950035031,
-39.220445337313));
#256725=CARTESIAN_POINT('Ctrl Pts',(-43.7098713630896,29.86081135322,-39.2079104317569));
#256726=CARTESIAN_POINT('Ctrl Pts',(-43.60926248355,29.9148659151021,-39.2029328369672));
#256727=CARTESIAN_POINT('Ctrl Pts',(-43.4947753987298,29.9878345433764,
-39.1954110293585));
#256728=CARTESIAN_POINT('Ctrl Pts',(-43.4770495704002,29.9994758178606,
-39.1941827039815));
#256729=CARTESIAN_POINT('Ctrl Pts',(-43.4573679760584,30.0127891661798,
-39.1927474179514));
#256730=CARTESIAN_POINT('Ctrl Pts',(-43.455236241125,30.0142363143022,-39.1925910112225));
#256731=CARTESIAN_POINT('Ctrl Pts',(-43.4509772683043,30.0171379110115,
-39.1922766338915));
#256732=CARTESIAN_POINT('Ctrl Pts',(-43.448850057475,30.0185923429967,-39.1921186649498));
#256733=CARTESIAN_POINT('Ctrl Pts',(-43.3720581307162,30.0712848254434,
-39.1863818256824));
#256734=CARTESIAN_POINT('Ctrl Pts',(-43.3005780774843,30.1267697410433,
-39.1798786632206));
#256735=CARTESIAN_POINT('Ctrl Pts',(-43.1313005315916,30.2748214743608,
-39.1616036912891));
#256736=CARTESIAN_POINT('Ctrl Pts',(-43.038186711969,30.3718329559061,-39.1488638155419));
#256737=CARTESIAN_POINT('Ctrl Pts',(-42.7806050039729,30.6908099865963,
-39.104922208377));
#256738=CARTESIAN_POINT('Ctrl Pts',(-42.6474050756438,30.9323003143339,
-39.0690165286225));
#256739=CARTESIAN_POINT('Ctrl Pts',(-42.5442998877123,31.2160759566304,
-39.0229211248878));
#256740=CARTESIAN_POINT('Ctrl Pts',(-42.5351088114909,31.2426960773276,
-39.0185610256159));
#256741=CARTESIAN_POINT('Ctrl Pts',(-42.5264442257536,31.2691195439559,
-39.0141970763358));
#256742=CARTESIAN_POINT('Ctrl Pts',(-46.5766932247455,31.5404524382932,
-52.6102625));
#256743=CARTESIAN_POINT('Ctrl Pts',(-46.5766932247455,30.3460643999139,
-52.5519291666666));
#256744=CARTESIAN_POINT('Ctrl Pts',(-45.5423228415329,29.7488703807243,
-52.4935958333333));
#256745=CARTESIAN_POINT('Ctrl Pts',(-44.5079524583202,29.1516763615346,
-52.4352625));
#256746=CARTESIAN_POINT('Ctrl Pts',(-43.4735820751074,29.7488703807243,
-52.3769291666667));
#256747=CARTESIAN_POINT('Ctrl Pts',(-42.4392116918948,30.3460643999138,
-52.3185958333334));
#256748=CARTESIAN_POINT('Ctrl Pts',(-42.4392116918948,31.5404524382931,
-52.2602625));
#256749=CARTESIAN_POINT('Ctrl Pts',(-42.4392116918947,32.7348404766723,
-52.2019291666667));
#256750=CARTESIAN_POINT('Ctrl Pts',(-43.4735820751074,33.332034495862,-52.1435958333333));
#256751=CARTESIAN_POINT('Ctrl Pts',(-44.5079524583201,33.9292285150516,
-52.0852625));
#256752=CARTESIAN_POINT('Ctrl Pts',(-45.5423228415328,33.332034495862,-52.0269291666667));
#256753=CARTESIAN_POINT('Ctrl Pts',(-46.5766932247455,32.7348404766724,
-51.9685958333333));
#256754=CARTESIAN_POINT('Ctrl Pts',(-46.5766932247455,31.5404524382932,
-51.9102625));
#256755=CARTESIAN_POINT('Ctrl Pts',(-46.5766932247455,30.3460643999139,
-51.8519291666667));
#256756=CARTESIAN_POINT('Ctrl Pts',(-45.5423228415329,29.7488703807243,
-51.7935958333333));
#256757=CARTESIAN_POINT('Ctrl Pts',(-44.5079524583202,29.1516763615346,
-51.7352625));
#256758=CARTESIAN_POINT('Ctrl Pts',(-43.4735820751074,29.7488703807243,
-51.6769291666667));
#256759=CARTESIAN_POINT('Ctrl Pts',(-42.4392116918948,30.3460643999138,
-51.6185958333333));
#256760=CARTESIAN_POINT('Ctrl Pts',(-42.4392116918948,31.5404524382931,
-51.5602625));
#256761=CARTESIAN_POINT('Ctrl Pts',(-42.4392116918947,32.7348404766723,
-51.5019291666666));
#256762=CARTESIAN_POINT('Ctrl Pts',(-43.4735820751074,33.332034495862,-51.4435958333333));
#256763=CARTESIAN_POINT('Ctrl Pts',(-44.5079524583201,33.9292285150516,
-51.3852625));
#256764=CARTESIAN_POINT('Ctrl Pts',(-45.5423228415328,33.332034495862,-51.3269291666667));
#256765=CARTESIAN_POINT('Ctrl Pts',(-46.5766932247455,32.7348404766724,
-51.2685958333333));
#256766=CARTESIAN_POINT('Ctrl Pts',(-46.5766932247455,31.5404524382932,
-51.2102625));
#256767=CARTESIAN_POINT('Ctrl Pts',(-46.5766932247455,30.3460643999139,
-51.1519291666666));
#256768=CARTESIAN_POINT('Ctrl Pts',(-45.5423228415329,29.7488703807243,
-51.0935958333334));
#256769=CARTESIAN_POINT('Ctrl Pts',(-44.5079524583202,29.1516763615346,
-51.0352625));
#256770=CARTESIAN_POINT('Ctrl Pts',(-43.4735820751074,29.7488703807243,
-50.9769291666667));
#256771=CARTESIAN_POINT('Ctrl Pts',(-42.4392116918948,30.3460643999138,
-50.9185958333333));
#256772=CARTESIAN_POINT('Ctrl Pts',(-42.4392116918948,31.5404524382931,
-50.8602625));
#256773=CARTESIAN_POINT('Ctrl Pts',(-42.4392116918947,32.7348404766723,
-50.8019291666667));
#256774=CARTESIAN_POINT('Ctrl Pts',(-43.4735820751074,33.332034495862,-50.7435958333333));
#256775=CARTESIAN_POINT('Ctrl Pts',(-44.5079524583201,33.9292285150516,
-50.6852625));
#256776=CARTESIAN_POINT('Ctrl Pts',(-45.5423228415328,33.332034495862,-50.6269291666667));
#256777=CARTESIAN_POINT('Ctrl Pts',(-46.5766932247455,32.7348404766724,
-50.5685958333333));
#256778=CARTESIAN_POINT('Ctrl Pts',(-46.5766932247455,31.5404524382932,
-50.5102625));
#256779=CARTESIAN_POINT('Ctrl Pts',(-46.5766932247455,30.3460643999139,
-50.4519291666667));
#256780=CARTESIAN_POINT('Ctrl Pts',(-45.5423228415329,29.7488703807243,
-50.3935958333333));
#256781=CARTESIAN_POINT('Ctrl Pts',(-44.5079524583202,29.1516763615346,
-50.3352625));
#256782=CARTESIAN_POINT('Ctrl Pts',(-43.4735820751074,29.7488703807243,
-50.2769291666667));
#256783=CARTESIAN_POINT('Ctrl Pts',(-42.4392116918948,30.3460643999138,
-50.2185958333333));
#256784=CARTESIAN_POINT('Ctrl Pts',(-42.4392116918948,31.5404524382931,
-50.1602625));
#256785=CARTESIAN_POINT('Ctrl Pts',(-42.4392116918947,32.7348404766723,
-50.1019291666667));
#256786=CARTESIAN_POINT('Ctrl Pts',(-43.4735820751074,33.332034495862,-50.0435958333333));
#256787=CARTESIAN_POINT('Ctrl Pts',(-44.5079524583201,33.9292285150516,
-49.9852625));
#256788=CARTESIAN_POINT('Ctrl Pts',(-45.5423228415328,33.332034495862,-49.9269291666667));
#256789=CARTESIAN_POINT('Ctrl Pts',(-46.5766932247455,32.7348404766724,
-49.8685958333333));
#256790=CARTESIAN_POINT('Ctrl Pts',(-46.5766932247455,31.5404524382932,
-49.8102625));
#256791=CARTESIAN_POINT('Ctrl Pts',(-46.5766932247455,30.3460643999139,
-49.7519291666667));
#256792=CARTESIAN_POINT('Ctrl Pts',(-45.5423228415329,29.7488703807243,
-49.6935958333334));
#256793=CARTESIAN_POINT('Ctrl Pts',(-44.5079524583202,29.1516763615346,
-49.6352625));
#256794=CARTESIAN_POINT('Ctrl Pts',(-43.4735820751074,29.7488703807243,
-49.5769291666667));
#256795=CARTESIAN_POINT('Ctrl Pts',(-42.4392116918948,30.3460643999138,
-49.5185958333334));
#256796=CARTESIAN_POINT('Ctrl Pts',(-42.4392116918948,31.5404524382931,
-49.4602625));
#256797=CARTESIAN_POINT('Ctrl Pts',(-42.4392116918947,32.7348404766723,
-49.4019291666667));
#256798=CARTESIAN_POINT('Ctrl Pts',(-43.4735820751074,33.332034495862,-49.3435958333333));
#256799=CARTESIAN_POINT('Ctrl Pts',(-44.5079524583201,33.9292285150516,
-49.2852625));
#256800=CARTESIAN_POINT('Ctrl Pts',(-45.5423228415328,33.332034495862,-49.2269291666667));
#256801=CARTESIAN_POINT('Ctrl Pts',(-46.5766932247455,32.7348404766724,
-49.1685958333334));
#256802=CARTESIAN_POINT('Ctrl Pts',(-46.5766932247455,31.5404524382932,
-49.1102625));
#256803=CARTESIAN_POINT('Ctrl Pts',(-46.5766932247455,30.3460643999139,
-49.0519291666667));
#256804=CARTESIAN_POINT('Ctrl Pts',(-45.5423228415329,29.7488703807243,
-48.9935958333333));
#256805=CARTESIAN_POINT('Ctrl Pts',(-44.5079524583202,29.1516763615346,
-48.9352625));
#256806=CARTESIAN_POINT('Ctrl Pts',(-43.4735820751074,29.7488703807243,
-48.8769291666667));
#256807=CARTESIAN_POINT('Ctrl Pts',(-42.4392116918948,30.3460643999138,
-48.8185958333333));
#256808=CARTESIAN_POINT('Ctrl Pts',(-42.4392116918948,31.5404524382931,
-48.7602625));
#256809=CARTESIAN_POINT('Ctrl Pts',(-42.4392116918947,32.7348404766723,
-48.7019291666667));
#256810=CARTESIAN_POINT('Ctrl Pts',(-43.4735820751074,33.332034495862,-48.6435958333333));
#256811=CARTESIAN_POINT('Ctrl Pts',(-44.5079524583201,33.9292285150516,
-48.5852625));
#256812=CARTESIAN_POINT('Ctrl Pts',(-45.5423228415328,33.332034495862,-48.5269291666667));
#256813=CARTESIAN_POINT('Ctrl Pts',(-46.5766932247455,32.7348404766724,
-48.4685958333333));
#256814=CARTESIAN_POINT('Ctrl Pts',(-46.5766932247455,31.5404524382932,
-48.4102625));
#256815=CARTESIAN_POINT('Ctrl Pts',(-46.5766932247455,30.3460643999139,
-48.3519291666667));
#256816=CARTESIAN_POINT('Ctrl Pts',(-45.5423228415329,29.7488703807243,
-48.2935958333333));
#256817=CARTESIAN_POINT('Ctrl Pts',(-44.5079524583202,29.1516763615346,
-48.2352625));
#256818=CARTESIAN_POINT('Ctrl Pts',(-43.4735820751074,29.7488703807243,
-48.1769291666667));
#256819=CARTESIAN_POINT('Ctrl Pts',(-42.4392116918948,30.3460643999138,
-48.1185958333334));
#256820=CARTESIAN_POINT('Ctrl Pts',(-42.4392116918948,31.5404524382931,
-48.0602625));
#256821=CARTESIAN_POINT('Ctrl Pts',(-42.4392116918947,32.7348404766723,
-48.0019291666667));
#256822=CARTESIAN_POINT('Ctrl Pts',(-43.4735820751074,33.332034495862,-47.9435958333334));
#256823=CARTESIAN_POINT('Ctrl Pts',(-44.5079524583201,33.9292285150516,
-47.8852625));
#256824=CARTESIAN_POINT('Ctrl Pts',(-45.5423228415328,33.332034495862,-47.8269291666667));
#256825=CARTESIAN_POINT('Ctrl Pts',(-46.5766932247455,32.7348404766724,
-47.7685958333333));
#256826=CARTESIAN_POINT('Ctrl Pts',(-46.5766932247455,31.5404524382932,
-47.7102625));
#256827=CARTESIAN_POINT('Ctrl Pts',(-46.5766932247455,30.3460643999139,
-47.6519291666667));
#256828=CARTESIAN_POINT('Ctrl Pts',(-45.5423228415329,29.7488703807243,
-47.5935958333333));
#256829=CARTESIAN_POINT('Ctrl Pts',(-44.5079524583202,29.1516763615346,
-47.5352625));
#256830=CARTESIAN_POINT('Ctrl Pts',(-43.4735820751074,29.7488703807243,
-47.4769291666667));
#256831=CARTESIAN_POINT('Ctrl Pts',(-42.4392116918948,30.3460643999138,
-47.4185958333333));
#256832=CARTESIAN_POINT('Ctrl Pts',(-42.4392116918948,31.5404524382931,
-47.3602625));
#256833=CARTESIAN_POINT('Ctrl Pts',(-42.4392116918947,32.7348404766723,
-47.3019291666666));
#256834=CARTESIAN_POINT('Ctrl Pts',(-43.4735820751074,33.332034495862,-47.2435958333333));
#256835=CARTESIAN_POINT('Ctrl Pts',(-44.5079524583201,33.9292285150516,
-47.1852625));
#256836=CARTESIAN_POINT('Ctrl Pts',(-45.5423228415328,33.332034495862,-47.1269291666667));
#256837=CARTESIAN_POINT('Ctrl Pts',(-46.5766932247455,32.7348404766724,
-47.0685958333333));
#256838=CARTESIAN_POINT('Ctrl Pts',(-46.5766932247455,31.5404524382932,
-47.0102625));
#256839=CARTESIAN_POINT('Ctrl Pts',(-46.5766932247455,30.3460643999139,
-46.9519291666667));
#256840=CARTESIAN_POINT('Ctrl Pts',(-45.5423228415329,29.7488703807243,
-46.8935958333333));
#256841=CARTESIAN_POINT('Ctrl Pts',(-44.5079524583202,29.1516763615346,
-46.8352625));
#256842=CARTESIAN_POINT('Ctrl Pts',(-43.4735820751074,29.7488703807243,
-46.7769291666667));
#256843=CARTESIAN_POINT('Ctrl Pts',(-42.4392116918948,30.3460643999138,
-46.7185958333333));
#256844=CARTESIAN_POINT('Ctrl Pts',(-42.4392116918948,31.5404524382931,
-46.6602625));
#256845=CARTESIAN_POINT('Ctrl Pts',(-42.4392116918948,32.7348404766723,
-46.6019291666667));
#256846=CARTESIAN_POINT('Ctrl Pts',(-43.4735820751074,33.332034495862,-46.5435958333334));
#256847=CARTESIAN_POINT('Ctrl Pts',(-44.5079524583201,33.9292285150516,
-46.4852625));
#256848=CARTESIAN_POINT('Ctrl Pts',(-45.5423228415328,33.332034495862,-46.4269291666667));
#256849=CARTESIAN_POINT('Ctrl Pts',(-46.5766932247455,32.7348404766724,
-46.3685958333333));
#256850=CARTESIAN_POINT('Ctrl Pts',(-46.5766932247455,31.5404524382932,
-46.3102625));
#256851=CARTESIAN_POINT('Ctrl Pts',(-46.5766932247455,30.3460643999139,
-46.2519291666667));
#256852=CARTESIAN_POINT('Ctrl Pts',(-45.5423228415329,29.7488703807243,
-46.1935958333333));
#256853=CARTESIAN_POINT('Ctrl Pts',(-44.5079524583202,29.1516763615346,
-46.1352625));
#256854=CARTESIAN_POINT('Ctrl Pts',(-43.4735820751074,29.7488703807243,
-46.0769291666667));
#256855=CARTESIAN_POINT('Ctrl Pts',(-42.4392116918948,30.3460643999138,
-46.0185958333334));
#256856=CARTESIAN_POINT('Ctrl Pts',(-42.4392116918948,31.5404524382931,
-45.9602625));
#256857=CARTESIAN_POINT('Ctrl Pts',(-42.4392116918948,32.7348404766723,
-45.9019291666667));
#256858=CARTESIAN_POINT('Ctrl Pts',(-43.4735820751074,33.332034495862,-45.8435958333333));
#256859=CARTESIAN_POINT('Ctrl Pts',(-44.5079524583201,33.9292285150516,
-45.7852625));
#256860=CARTESIAN_POINT('Ctrl Pts',(-45.5423228415328,33.332034495862,-45.7269291666667));
#256861=CARTESIAN_POINT('Ctrl Pts',(-46.5766932247455,32.7348404766724,
-45.6685958333334));
#256862=CARTESIAN_POINT('Ctrl Pts',(-46.5766932247455,31.5404524382932,
-45.6102625));
#256863=CARTESIAN_POINT('Ctrl Pts',(-46.5766932247455,30.3460643999139,
-45.5519291666667));
#256864=CARTESIAN_POINT('Ctrl Pts',(-45.5423228415329,29.7488703807243,
-45.4935958333333));
#256865=CARTESIAN_POINT('Ctrl Pts',(-44.5079524583202,29.1516763615346,
-45.4352625));
#256866=CARTESIAN_POINT('Ctrl Pts',(-43.4735820751074,29.7488703807243,
-45.3769291666667));
#256867=CARTESIAN_POINT('Ctrl Pts',(-42.4392116918948,30.3460643999138,
-45.3185958333333));
#256868=CARTESIAN_POINT('Ctrl Pts',(-42.4392116918948,31.5404524382931,
-45.2602625));
#256869=CARTESIAN_POINT('Ctrl Pts',(-42.4392116918948,32.7348404766723,
-45.2019291666667));
#256870=CARTESIAN_POINT('Ctrl Pts',(-43.4735820751074,33.332034495862,-45.1435958333333));
#256871=CARTESIAN_POINT('Ctrl Pts',(-44.5079524583201,33.9292285150516,
-45.0852625));
#256872=CARTESIAN_POINT('Ctrl Pts',(-45.5423228415328,33.332034495862,-45.0269291666667));
#256873=CARTESIAN_POINT('Ctrl Pts',(-46.5766932247455,32.7348404766724,
-44.9685958333334));
#256874=CARTESIAN_POINT('Ctrl Pts',(-46.5766932247455,31.5404524382932,
-44.9102625));
#256875=CARTESIAN_POINT('Ctrl Pts',(-46.5766932247455,30.3460643999139,
-44.8519291666667));
#256876=CARTESIAN_POINT('Ctrl Pts',(-45.5423228415329,29.7488703807243,
-44.7935958333333));
#256877=CARTESIAN_POINT('Ctrl Pts',(-44.5079524583202,29.1516763615346,
-44.7352625));
#256878=CARTESIAN_POINT('Ctrl Pts',(-43.4735820751074,29.7488703807243,
-44.6769291666667));
#256879=CARTESIAN_POINT('Ctrl Pts',(-42.4392116918948,30.3460643999138,
-44.6185958333334));
#256880=CARTESIAN_POINT('Ctrl Pts',(-42.4392116918948,31.5404524382931,
-44.5602625));
#256881=CARTESIAN_POINT('Ctrl Pts',(-42.4392116918948,32.7348404766723,
-44.5019291666667));
#256882=CARTESIAN_POINT('Ctrl Pts',(-43.4735820751074,33.332034495862,-44.4435958333333));
#256883=CARTESIAN_POINT('Ctrl Pts',(-44.5079524583201,33.9292285150516,
-44.3852625));
#256884=CARTESIAN_POINT('Ctrl Pts',(-45.5423228415328,33.332034495862,-44.3269291666667));
#256885=CARTESIAN_POINT('Ctrl Pts',(-46.5766932247455,32.7348404766724,
-44.2685958333334));
#256886=CARTESIAN_POINT('Ctrl Pts',(-46.5766932247455,31.5404524382932,
-44.2102625));
#256887=CARTESIAN_POINT('Ctrl Pts',(-46.5766932247455,30.3460643999139,
-44.1519291666667));
#256888=CARTESIAN_POINT('Ctrl Pts',(-45.5423228415329,29.7488703807243,
-44.0935958333334));
#256889=CARTESIAN_POINT('Ctrl Pts',(-44.5079524583202,29.1516763615346,
-44.0352625));
#256890=CARTESIAN_POINT('Ctrl Pts',(-43.4735820751074,29.7488703807243,
-43.9769291666667));
#256891=CARTESIAN_POINT('Ctrl Pts',(-42.4392116918948,30.3460643999138,
-43.9185958333333));
#256892=CARTESIAN_POINT('Ctrl Pts',(-42.4392116918948,31.5404524382931,
-43.8602625));
#256893=CARTESIAN_POINT('Ctrl Pts',(-42.4392116918948,32.7348404766723,
-43.8019291666667));
#256894=CARTESIAN_POINT('Ctrl Pts',(-43.4735820751074,33.332034495862,-43.7435958333334));
#256895=CARTESIAN_POINT('Ctrl Pts',(-44.5079524583201,33.9292285150516,
-43.6852625));
#256896=CARTESIAN_POINT('Ctrl Pts',(-45.5423228415328,33.332034495862,-43.6269291666667));
#256897=CARTESIAN_POINT('Ctrl Pts',(-46.5766932247455,32.7348404766724,
-43.5685958333333));
#256898=CARTESIAN_POINT('Ctrl Pts',(-46.5766932247455,31.5404524382932,
-43.5102625));
#256899=CARTESIAN_POINT('Ctrl Pts',(-46.5766932247455,30.3460643999139,
-43.4519291666667));
#256900=CARTESIAN_POINT('Ctrl Pts',(-45.5423228415329,29.7488703807243,
-43.3935958333334));
#256901=CARTESIAN_POINT('Ctrl Pts',(-44.5079524583202,29.1516763615346,
-43.3352625));
#256902=CARTESIAN_POINT('Ctrl Pts',(-43.4735820751074,29.7488703807243,
-43.2769291666667));
#256903=CARTESIAN_POINT('Ctrl Pts',(-42.4392116918948,30.3460643999138,
-43.2185958333333));
#256904=CARTESIAN_POINT('Ctrl Pts',(-42.4392116918948,31.5404524382931,
-43.1602625));
#256905=CARTESIAN_POINT('Ctrl Pts',(-42.4392116918948,32.7348404766723,
-43.1019291666667));
#256906=CARTESIAN_POINT('Ctrl Pts',(-43.4735820751074,33.332034495862,-43.0435958333334));
#256907=CARTESIAN_POINT('Ctrl Pts',(-44.5079524583201,33.9292285150516,
-42.9852625));
#256908=CARTESIAN_POINT('Ctrl Pts',(-45.5423228415328,33.332034495862,-42.9269291666667));
#256909=CARTESIAN_POINT('Ctrl Pts',(-46.5766932247455,32.7348404766724,
-42.8685958333333));
#256910=CARTESIAN_POINT('Ctrl Pts',(-46.5766932247455,31.5404524382932,
-42.8102625));
#256911=CARTESIAN_POINT('Ctrl Pts',(-46.5766932247455,30.3460643999139,
-42.7519291666666));
#256912=CARTESIAN_POINT('Ctrl Pts',(-45.5423228415329,29.7488703807243,
-42.6935958333333));
#256913=CARTESIAN_POINT('Ctrl Pts',(-44.5079524583202,29.1516763615346,
-42.6352625));
#256914=CARTESIAN_POINT('Ctrl Pts',(-43.4735820751074,29.7488703807243,
-42.5769291666667));
#256915=CARTESIAN_POINT('Ctrl Pts',(-42.4392116918948,30.3460643999138,
-42.5185958333333));
#256916=CARTESIAN_POINT('Ctrl Pts',(-42.4392116918948,31.5404524382931,
-42.4602625));
#256917=CARTESIAN_POINT('Ctrl Pts',(-42.4392116918948,32.7348404766723,
-42.4019291666666));
#256918=CARTESIAN_POINT('Ctrl Pts',(-43.4735820751074,33.332034495862,-42.3435958333334));
#256919=CARTESIAN_POINT('Ctrl Pts',(-44.5079524583201,33.9292285150516,
-42.2852625));
#256920=CARTESIAN_POINT('Ctrl Pts',(-45.5423228415328,33.332034495862,-42.2269291666667));
#256921=CARTESIAN_POINT('Ctrl Pts',(-46.5766932247455,32.7348404766724,
-42.1685958333333));
#256922=CARTESIAN_POINT('Ctrl Pts',(-46.5766932247455,31.5404524382932,
-42.1102625));
#256923=CARTESIAN_POINT('Ctrl Pts',(-46.5766932247455,30.3460643999139,
-42.0519291666666));
#256924=CARTESIAN_POINT('Ctrl Pts',(-45.5423228415329,29.7488703807243,
-41.9935958333334));
#256925=CARTESIAN_POINT('Ctrl Pts',(-44.5079524583202,29.1516763615346,
-41.9352625));
#256926=CARTESIAN_POINT('Ctrl Pts',(-43.4735820751074,29.7488703807243,
-41.8769291666667));
#256927=CARTESIAN_POINT('Ctrl Pts',(-42.4392116918948,30.3460643999138,
-41.8185958333333));
#256928=CARTESIAN_POINT('Ctrl Pts',(-42.4392116918948,31.5404524382931,
-41.7602625));
#256929=CARTESIAN_POINT('Ctrl Pts',(-42.4392116918948,32.7348404766723,
-41.7019291666666));
#256930=CARTESIAN_POINT('Ctrl Pts',(-43.4735820751074,33.332034495862,-41.6435958333334));
#256931=CARTESIAN_POINT('Ctrl Pts',(-44.5079524583201,33.9292285150516,
-41.5852625));
#256932=CARTESIAN_POINT('Ctrl Pts',(-45.5423228415328,33.332034495862,-41.5269291666667));
#256933=CARTESIAN_POINT('Ctrl Pts',(-46.5766932247455,32.7348404766724,
-41.4685958333333));
#256934=CARTESIAN_POINT('Ctrl Pts',(-46.5766932247455,31.5404524382932,
-41.4102625));
#256935=CARTESIAN_POINT('Ctrl Pts',(-46.5766932247455,30.3460643999139,
-41.3519291666666));
#256936=CARTESIAN_POINT('Ctrl Pts',(-45.5423228415329,29.7488703807243,
-41.2935958333334));
#256937=CARTESIAN_POINT('Ctrl Pts',(-44.5079524583202,29.1516763615346,
-41.2352625));
#256938=CARTESIAN_POINT('Ctrl Pts',(-43.4735820751074,29.7488703807243,
-41.1769291666667));
#256939=CARTESIAN_POINT('Ctrl Pts',(-42.4392116918948,30.3460643999138,
-41.1185958333333));
#256940=CARTESIAN_POINT('Ctrl Pts',(-42.4392116918948,31.5404524382931,
-41.0602625));
#256941=CARTESIAN_POINT('Ctrl Pts',(-42.4392116918948,32.7348404766723,
-41.0019291666666));
#256942=CARTESIAN_POINT('Ctrl Pts',(-43.4735820751074,33.332034495862,-40.9435958333334));
#256943=CARTESIAN_POINT('Ctrl Pts',(-44.5079524583201,33.9292285150516,
-40.8852625));
#256944=CARTESIAN_POINT('Ctrl Pts',(-45.5423228415328,33.332034495862,-40.8269291666667));
#256945=CARTESIAN_POINT('Ctrl Pts',(-46.5766932247455,32.7348404766724,
-40.7685958333333));
#256946=CARTESIAN_POINT('Ctrl Pts',(-46.5766932247455,31.5404524382932,
-40.7102625));
#256947=CARTESIAN_POINT('Ctrl Pts',(-46.5766932247455,30.3460643999139,
-40.6519291666667));
#256948=CARTESIAN_POINT('Ctrl Pts',(-45.5423228415329,29.7488703807243,
-40.5935958333334));
#256949=CARTESIAN_POINT('Ctrl Pts',(-44.5079524583202,29.1516763615346,
-40.5352625));
#256950=CARTESIAN_POINT('Ctrl Pts',(-43.4735820751074,29.7488703807243,
-40.4769291666667));
#256951=CARTESIAN_POINT('Ctrl Pts',(-42.4392116918948,30.3460643999138,
-40.4185958333333));
#256952=CARTESIAN_POINT('Ctrl Pts',(-42.4392116918948,31.5404524382931,
-40.3602625));
#256953=CARTESIAN_POINT('Ctrl Pts',(-42.4392116918948,32.7348404766723,
-40.3019291666667));
#256954=CARTESIAN_POINT('Ctrl Pts',(-43.4735820751074,33.332034495862,-40.2435958333334));
#256955=CARTESIAN_POINT('Ctrl Pts',(-44.5079524583201,33.9292285150516,
-40.1852625));
#256956=CARTESIAN_POINT('Ctrl Pts',(-45.5423228415328,33.332034495862,-40.1269291666666));
#256957=CARTESIAN_POINT('Ctrl Pts',(-46.5766932247455,32.7348404766724,
-40.0685958333333));
#256958=CARTESIAN_POINT('Ctrl Pts',(-46.5766932247455,31.5404524382932,
-40.0102625));
#256959=CARTESIAN_POINT('Ctrl Pts',(-46.5766932247455,30.3460643999139,
-39.9519291666667));
#256960=CARTESIAN_POINT('Ctrl Pts',(-45.5423228415329,29.7488703807243,
-39.8935958333334));
#256961=CARTESIAN_POINT('Ctrl Pts',(-44.5079524583202,29.1516763615346,
-39.8352625));
#256962=CARTESIAN_POINT('Ctrl Pts',(-43.4735820751074,29.7488703807243,
-39.7769291666666));
#256963=CARTESIAN_POINT('Ctrl Pts',(-42.4392116918948,30.3460643999138,
-39.7185958333334));
#256964=CARTESIAN_POINT('Ctrl Pts',(-42.4392116918948,31.5404524382931,
-39.6602625));
#256965=CARTESIAN_POINT('Ctrl Pts',(-42.4392116918948,32.7348404766723,
-39.6019291666667));
#256966=CARTESIAN_POINT('Ctrl Pts',(-43.4735820751074,33.332034495862,-39.5435958333333));
#256967=CARTESIAN_POINT('Ctrl Pts',(-44.5079524583201,33.9292285150516,
-39.4852625));
#256968=CARTESIAN_POINT('Ctrl Pts',(-45.5423228415328,33.332034495862,-39.4269291666667));
#256969=CARTESIAN_POINT('Ctrl Pts',(-46.5766932247455,32.7348404766724,
-39.3685958333334));
#256970=CARTESIAN_POINT('Ctrl Pts',(-46.5766932247455,31.5404524382932,
-39.3102625));
#256971=CARTESIAN_POINT('Ctrl Pts',(-46.5766932247455,30.3460643999139,
-39.2519291666667));
#256972=CARTESIAN_POINT('Ctrl Pts',(-45.5423228415329,29.7488703807243,
-39.1935958333334));
#256973=CARTESIAN_POINT('Ctrl Pts',(-44.5079524583202,29.1516763615346,
-39.1352625));
#256974=CARTESIAN_POINT('Ctrl Pts',(-43.4735820751074,29.7488703807243,
-39.0769291666667));
#256975=CARTESIAN_POINT('Ctrl Pts',(-42.4392116918948,30.3460643999138,
-39.0185958333333));
#256976=CARTESIAN_POINT('Ctrl Pts',(-42.4392116918948,31.5404524382931,
-38.9602625));
#256977=CARTESIAN_POINT('Ctrl Pts',(-42.4392116918948,32.7348404766723,
-38.9019291666667));
#256978=CARTESIAN_POINT('Ctrl Pts',(-43.4735820751074,33.332034495862,-38.8435958333333));
#256979=CARTESIAN_POINT('Ctrl Pts',(-44.5079524583201,33.9292285150516,
-38.7852625));
#256980=CARTESIAN_POINT('Ctrl Pts',(-45.5423228415328,33.332034495862,-38.7269291666667));
#256981=CARTESIAN_POINT('Ctrl Pts',(-46.5766932247455,32.7348404766724,
-38.6685958333334));
#256982=CARTESIAN_POINT('Ctrl Pts',(-46.5766932247455,31.5404524382932,
-38.6102625));
#256983=CARTESIAN_POINT('Ctrl Pts',(-46.5766932247455,30.3460643999139,
-38.5519291666667));
#256984=CARTESIAN_POINT('Ctrl Pts',(-45.5423228415329,29.7488703807243,
-38.4935958333334));
#256985=CARTESIAN_POINT('Ctrl Pts',(-44.5079524583202,29.1516763615346,
-38.4352625));
#256986=CARTESIAN_POINT('Ctrl Pts',(-43.4735820751074,29.7488703807243,
-38.3769291666666));
#256987=CARTESIAN_POINT('Ctrl Pts',(-42.4392116918948,30.3460643999138,
-38.3185958333333));
#256988=CARTESIAN_POINT('Ctrl Pts',(-42.4392116918948,31.5404524382931,
-38.2602625));
#256989=CARTESIAN_POINT('Ctrl Pts',(-42.4392116918948,32.7348404766723,
-38.2019291666667));
#256990=CARTESIAN_POINT('Ctrl Pts',(-43.4735820751074,33.332034495862,-38.1435958333334));
#256991=CARTESIAN_POINT('Ctrl Pts',(-44.5079524583201,33.9292285150516,
-38.0852625));
#256992=CARTESIAN_POINT('Ctrl Pts',(-45.5423228415328,33.332034495862,-38.0269291666667));
#256993=CARTESIAN_POINT('Ctrl Pts',(-46.5766932247455,32.7348404766724,
-37.9685958333333));
#256994=CARTESIAN_POINT('Ctrl Pts',(-46.5766932247455,31.5404524382932,
-37.9102625));
#256995=CARTESIAN_POINT('Ctrl Pts',(-46.5766932247455,30.3460643999139,
-37.8519291666667));
#256996=CARTESIAN_POINT('Ctrl Pts',(-45.5423228415329,29.7488703807243,
-37.7935958333334));
#256997=CARTESIAN_POINT('Ctrl Pts',(-44.5079524583202,29.1516763615346,
-37.7352625));
#256998=CARTESIAN_POINT('Ctrl Pts',(-43.4735820751074,29.7488703807243,
-37.6769291666667));
#256999=CARTESIAN_POINT('Ctrl Pts',(-42.4392116918948,30.3460643999138,
-37.6185958333333));
#257000=CARTESIAN_POINT('Ctrl Pts',(-42.4392116918948,31.5404524382931,
-37.5602625));
#257001=CARTESIAN_POINT('Ctrl Pts',(-42.4392116918948,32.7348404766723,
-37.5019291666666));
#257002=CARTESIAN_POINT('Ctrl Pts',(-43.4735820751074,33.332034495862,-37.4435958333333));
#257003=CARTESIAN_POINT('Ctrl Pts',(-44.5079524583201,33.9292285150516,
-37.3852625));
#257004=CARTESIAN_POINT('Ctrl Pts',(-45.5423228415328,33.332034495862,-37.3269291666667));
#257005=CARTESIAN_POINT('Ctrl Pts',(-46.5766932247455,32.7348404766724,
-37.2685958333333));
#257006=CARTESIAN_POINT('Ctrl Pts',(-46.5766932247455,31.5404524382932,
-37.2102625));
#257007=CARTESIAN_POINT('Ctrl Pts',(-46.5766932247455,30.3460643999139,
-37.1519291666667));
#257008=CARTESIAN_POINT('Ctrl Pts',(-45.5423228415329,29.7488703807243,
-37.0935958333333));
#257009=CARTESIAN_POINT('Ctrl Pts',(-44.5079524583202,29.1516763615346,
-37.0352625));
#257010=CARTESIAN_POINT('Ctrl Pts',(-43.4735820751074,29.7488703807243,
-36.9769291666667));
#257011=CARTESIAN_POINT('Ctrl Pts',(-42.4392116918948,30.3460643999138,
-36.9185958333333));
#257012=CARTESIAN_POINT('Ctrl Pts',(-42.4392116918948,31.5404524382931,
-36.8602625));
#257013=CARTESIAN_POINT('Ctrl Pts',(-42.4392116918948,32.7348404766723,
-36.8019291666666));
#257014=CARTESIAN_POINT('Ctrl Pts',(-43.4735820751074,33.332034495862,-36.7435958333334));
#257015=CARTESIAN_POINT('Ctrl Pts',(-44.5079524583201,33.9292285150516,
-36.6852625));
#257016=CARTESIAN_POINT('Ctrl Pts',(-45.5423228415328,33.332034495862,-36.6269291666666));
#257017=CARTESIAN_POINT('Ctrl Pts',(-45.6766051604214,33.2545065629043,
-36.6193563132714));
#257018=CARTESIAN_POINT('Ctrl Pts',(-45.7978303778612,33.1578278775004,
-36.611216324118));
#257019=CARTESIAN_POINT('Ctrl Pts',(-46.1766975859751,31.5404524382932,
-52.8412000897188));
#257020=CARTESIAN_POINT('Ctrl Pts',(-46.1766975859751,30.5770019896326,
-52.7828667563854));
#257021=CARTESIAN_POINT('Ctrl Pts',(-45.3423250221477,30.0952767653024,
-52.7245334230522));
#257022=CARTESIAN_POINT('Ctrl Pts',(-44.5079524583202,29.6135515409722,
-52.6662000897188));
#257023=CARTESIAN_POINT('Ctrl Pts',(-43.6735798944927,30.0952767653024,
-52.6078667563855));
#257024=CARTESIAN_POINT('Ctrl Pts',(-42.8392073306652,30.5770019896326,
-52.5495334230521));
#257025=CARTESIAN_POINT('Ctrl Pts',(-42.8392073306652,31.5404524382931,
-52.4912000897188));
#257026=CARTESIAN_POINT('Ctrl Pts',(-42.8392073306652,32.5039028869536,
-52.4328667563855));
#257027=CARTESIAN_POINT('Ctrl Pts',(-43.6735798944926,32.9856281112839,
-52.3745334230522));
#257028=CARTESIAN_POINT('Ctrl Pts',(-44.5079524583201,33.4673533356141,
-52.3162000897188));
#257029=CARTESIAN_POINT('Ctrl Pts',(-45.3423250221477,32.9856281112839,
-52.2578667563855));
#257030=CARTESIAN_POINT('Ctrl Pts',(-46.1766975859751,32.5039028869536,
-52.1995334230521));
#257031=CARTESIAN_POINT('Ctrl Pts',(-46.1766975859751,31.5404524382932,
-52.1412000897188));
#257032=CARTESIAN_POINT('Ctrl Pts',(-46.1766975859751,30.5770019896326,
-52.0828667563854));
#257033=CARTESIAN_POINT('Ctrl Pts',(-45.3423250221477,30.0952767653024,
-52.0245334230521));
#257034=CARTESIAN_POINT('Ctrl Pts',(-44.5079524583202,29.6135515409722,
-51.9662000897188));
#257035=CARTESIAN_POINT('Ctrl Pts',(-43.6735798944927,30.0952767653024,
-51.9078667563855));
#257036=CARTESIAN_POINT('Ctrl Pts',(-42.8392073306652,30.5770019896326,
-51.8495334230521));
#257037=CARTESIAN_POINT('Ctrl Pts',(-42.8392073306652,31.5404524382931,
-51.7912000897188));
#257038=CARTESIAN_POINT('Ctrl Pts',(-42.8392073306652,32.5039028869536,
-51.7328667563854));
#257039=CARTESIAN_POINT('Ctrl Pts',(-43.6735798944926,32.9856281112839,
-51.6745334230521));
#257040=CARTESIAN_POINT('Ctrl Pts',(-44.5079524583201,33.4673533356141,
-51.6162000897188));
#257041=CARTESIAN_POINT('Ctrl Pts',(-45.3423250221477,32.9856281112839,
-51.5578667563855));
#257042=CARTESIAN_POINT('Ctrl Pts',(-46.1766975859751,32.5039028869536,
-51.4995334230521));
#257043=CARTESIAN_POINT('Ctrl Pts',(-46.1766975859751,31.5404524382932,
-51.4412000897188));
#257044=CARTESIAN_POINT('Ctrl Pts',(-46.1766975859751,30.5770019896326,
-51.3828667563855));
#257045=CARTESIAN_POINT('Ctrl Pts',(-45.3423250221477,30.0952767653024,
-51.3245334230522));
#257046=CARTESIAN_POINT('Ctrl Pts',(-44.5079524583202,29.6135515409722,
-51.2662000897188));
#257047=CARTESIAN_POINT('Ctrl Pts',(-43.6735798944927,30.0952767653024,
-51.2078667563855));
#257048=CARTESIAN_POINT('Ctrl Pts',(-42.8392073306652,30.5770019896326,
-51.1495334230521));
#257049=CARTESIAN_POINT('Ctrl Pts',(-42.8392073306652,31.5404524382931,
-51.0912000897188));
#257050=CARTESIAN_POINT('Ctrl Pts',(-42.8392073306652,32.5039028869536,
-51.0328667563854));
#257051=CARTESIAN_POINT('Ctrl Pts',(-43.6735798944926,32.9856281112839,
-50.9745334230521));
#257052=CARTESIAN_POINT('Ctrl Pts',(-44.5079524583201,33.4673533356141,
-50.9162000897188));
#257053=CARTESIAN_POINT('Ctrl Pts',(-45.3423250221477,32.9856281112839,
-50.8578667563855));
#257054=CARTESIAN_POINT('Ctrl Pts',(-46.1766975859751,32.5039028869536,
-50.7995334230521));
#257055=CARTESIAN_POINT('Ctrl Pts',(-46.1766975859751,31.5404524382932,
-50.7412000897188));
#257056=CARTESIAN_POINT('Ctrl Pts',(-46.1766975859751,30.5770019896326,
-50.6828667563855));
#257057=CARTESIAN_POINT('Ctrl Pts',(-45.3423250221477,30.0952767653024,
-50.6245334230521));
#257058=CARTESIAN_POINT('Ctrl Pts',(-44.5079524583202,29.6135515409722,
-50.5662000897188));
#257059=CARTESIAN_POINT('Ctrl Pts',(-43.6735798944927,30.0952767653024,
-50.5078667563855));
#257060=CARTESIAN_POINT('Ctrl Pts',(-42.8392073306652,30.5770019896326,
-50.4495334230521));
#257061=CARTESIAN_POINT('Ctrl Pts',(-42.8392073306652,31.5404524382931,
-50.3912000897188));
#257062=CARTESIAN_POINT('Ctrl Pts',(-42.8392073306652,32.5039028869536,
-50.3328667563854));
#257063=CARTESIAN_POINT('Ctrl Pts',(-43.6735798944926,32.9856281112839,
-50.2745334230521));
#257064=CARTESIAN_POINT('Ctrl Pts',(-44.5079524583201,33.4673533356141,
-50.2162000897188));
#257065=CARTESIAN_POINT('Ctrl Pts',(-45.3423250221477,32.9856281112839,
-50.1578667563855));
#257066=CARTESIAN_POINT('Ctrl Pts',(-46.1766975859751,32.5039028869536,
-50.0995334230521));
#257067=CARTESIAN_POINT('Ctrl Pts',(-46.1766975859751,31.5404524382932,
-50.0412000897188));
#257068=CARTESIAN_POINT('Ctrl Pts',(-46.1766975859751,30.5770019896326,
-49.9828667563855));
#257069=CARTESIAN_POINT('Ctrl Pts',(-45.3423250221477,30.0952767653024,
-49.9245334230522));
#257070=CARTESIAN_POINT('Ctrl Pts',(-44.5079524583202,29.6135515409722,
-49.8662000897188));
#257071=CARTESIAN_POINT('Ctrl Pts',(-43.6735798944927,30.0952767653024,
-49.8078667563855));
#257072=CARTESIAN_POINT('Ctrl Pts',(-42.8392073306652,30.5770019896326,
-49.7495334230521));
#257073=CARTESIAN_POINT('Ctrl Pts',(-42.8392073306652,31.5404524382931,
-49.6912000897188));
#257074=CARTESIAN_POINT('Ctrl Pts',(-42.8392073306652,32.5039028869536,
-49.6328667563854));
#257075=CARTESIAN_POINT('Ctrl Pts',(-43.6735798944926,32.9856281112839,
-49.5745334230521));
#257076=CARTESIAN_POINT('Ctrl Pts',(-44.5079524583201,33.4673533356141,
-49.5162000897188));
#257077=CARTESIAN_POINT('Ctrl Pts',(-45.3423250221477,32.9856281112839,
-49.4578667563855));
#257078=CARTESIAN_POINT('Ctrl Pts',(-46.1766975859751,32.5039028869536,
-49.3995334230521));
#257079=CARTESIAN_POINT('Ctrl Pts',(-46.1766975859751,31.5404524382932,
-49.3412000897188));
#257080=CARTESIAN_POINT('Ctrl Pts',(-46.1766975859751,30.5770019896326,
-49.2828667563854));
#257081=CARTESIAN_POINT('Ctrl Pts',(-45.3423250221477,30.0952767653024,
-49.2245334230521));
#257082=CARTESIAN_POINT('Ctrl Pts',(-44.5079524583202,29.6135515409722,
-49.1662000897188));
#257083=CARTESIAN_POINT('Ctrl Pts',(-43.6735798944927,30.0952767653024,
-49.1078667563855));
#257084=CARTESIAN_POINT('Ctrl Pts',(-42.8392073306652,30.5770019896326,
-49.0495334230521));
#257085=CARTESIAN_POINT('Ctrl Pts',(-42.8392073306652,31.5404524382931,
-48.9912000897188));
#257086=CARTESIAN_POINT('Ctrl Pts',(-42.8392073306652,32.5039028869536,
-48.9328667563854));
#257087=CARTESIAN_POINT('Ctrl Pts',(-43.6735798944926,32.9856281112839,
-48.8745334230521));
#257088=CARTESIAN_POINT('Ctrl Pts',(-44.5079524583201,33.4673533356141,
-48.8162000897187));
#257089=CARTESIAN_POINT('Ctrl Pts',(-45.3423250221477,32.9856281112839,
-48.7578667563855));
#257090=CARTESIAN_POINT('Ctrl Pts',(-46.1766975859751,32.5039028869536,
-48.6995334230521));
#257091=CARTESIAN_POINT('Ctrl Pts',(-46.1766975859751,31.5404524382932,
-48.6412000897188));
#257092=CARTESIAN_POINT('Ctrl Pts',(-46.1766975859751,30.5770019896326,
-48.5828667563854));
#257093=CARTESIAN_POINT('Ctrl Pts',(-45.3423250221477,30.0952767653024,
-48.5245334230521));
#257094=CARTESIAN_POINT('Ctrl Pts',(-44.5079524583202,29.6135515409722,
-48.4662000897187));
#257095=CARTESIAN_POINT('Ctrl Pts',(-43.6735798944927,30.0952767653024,
-48.4078667563855));
#257096=CARTESIAN_POINT('Ctrl Pts',(-42.8392073306652,30.5770019896326,
-48.3495334230521));
#257097=CARTESIAN_POINT('Ctrl Pts',(-42.8392073306652,31.5404524382931,
-48.2912000897188));
#257098=CARTESIAN_POINT('Ctrl Pts',(-42.8392073306652,32.5039028869536,
-48.2328667563854));
#257099=CARTESIAN_POINT('Ctrl Pts',(-43.6735798944926,32.9856281112839,
-48.1745334230522));
#257100=CARTESIAN_POINT('Ctrl Pts',(-44.5079524583201,33.4673533356141,
-48.1162000897187));
#257101=CARTESIAN_POINT('Ctrl Pts',(-45.3423250221477,32.9856281112839,
-48.0578667563855));
#257102=CARTESIAN_POINT('Ctrl Pts',(-46.1766975859751,32.5039028869536,
-47.9995334230521));
#257103=CARTESIAN_POINT('Ctrl Pts',(-46.1766975859751,31.5404524382932,
-47.9412000897188));
#257104=CARTESIAN_POINT('Ctrl Pts',(-46.1766975859751,30.5770019896326,
-47.8828667563854));
#257105=CARTESIAN_POINT('Ctrl Pts',(-45.3423250221477,30.0952767653024,
-47.8245334230521));
#257106=CARTESIAN_POINT('Ctrl Pts',(-44.5079524583202,29.6135515409722,
-47.7662000897188));
#257107=CARTESIAN_POINT('Ctrl Pts',(-43.6735798944927,30.0952767653024,
-47.7078667563855));
#257108=CARTESIAN_POINT('Ctrl Pts',(-42.8392073306652,30.5770019896326,
-47.6495334230521));
#257109=CARTESIAN_POINT('Ctrl Pts',(-42.8392073306652,31.5404524382931,
-47.5912000897188));
#257110=CARTESIAN_POINT('Ctrl Pts',(-42.8392073306652,32.5039028869536,
-47.5328667563854));
#257111=CARTESIAN_POINT('Ctrl Pts',(-43.6735798944926,32.9856281112839,
-47.4745334230522));
#257112=CARTESIAN_POINT('Ctrl Pts',(-44.5079524583201,33.4673533356141,
-47.4162000897188));
#257113=CARTESIAN_POINT('Ctrl Pts',(-45.3423250221477,32.9856281112839,
-47.3578667563855));
#257114=CARTESIAN_POINT('Ctrl Pts',(-46.1766975859751,32.5039028869536,
-47.2995334230521));
#257115=CARTESIAN_POINT('Ctrl Pts',(-46.1766975859751,31.5404524382932,
-47.2412000897188));
#257116=CARTESIAN_POINT('Ctrl Pts',(-46.1766975859751,30.5770019896326,
-47.1828667563854));
#257117=CARTESIAN_POINT('Ctrl Pts',(-45.3423250221477,30.0952767653024,
-47.1245334230521));
#257118=CARTESIAN_POINT('Ctrl Pts',(-44.5079524583202,29.6135515409722,
-47.0662000897188));
#257119=CARTESIAN_POINT('Ctrl Pts',(-43.6735798944927,30.0952767653024,
-47.0078667563855));
#257120=CARTESIAN_POINT('Ctrl Pts',(-42.8392073306652,30.5770019896326,
-46.9495334230521));
#257121=CARTESIAN_POINT('Ctrl Pts',(-42.8392073306652,31.5404524382931,
-46.8912000897188));
#257122=CARTESIAN_POINT('Ctrl Pts',(-42.8392073306652,32.5039028869536,
-46.8328667563854));
#257123=CARTESIAN_POINT('Ctrl Pts',(-43.6735798944926,32.9856281112839,
-46.7745334230521));
#257124=CARTESIAN_POINT('Ctrl Pts',(-44.5079524583201,33.4673533356141,
-46.7162000897188));
#257125=CARTESIAN_POINT('Ctrl Pts',(-45.3423250221477,32.9856281112839,
-46.6578667563855));
#257126=CARTESIAN_POINT('Ctrl Pts',(-46.1766975859751,32.5039028869536,
-46.5995334230521));
#257127=CARTESIAN_POINT('Ctrl Pts',(-46.1766975859751,31.5404524382932,
-46.5412000897188));
#257128=CARTESIAN_POINT('Ctrl Pts',(-46.1766975859751,30.5770019896326,
-46.4828667563854));
#257129=CARTESIAN_POINT('Ctrl Pts',(-45.3423250221477,30.0952767653024,
-46.4245334230521));
#257130=CARTESIAN_POINT('Ctrl Pts',(-44.5079524583202,29.6135515409722,
-46.3662000897188));
#257131=CARTESIAN_POINT('Ctrl Pts',(-43.6735798944927,30.0952767653024,
-46.3078667563855));
#257132=CARTESIAN_POINT('Ctrl Pts',(-42.8392073306652,30.5770019896326,
-46.2495334230521));
#257133=CARTESIAN_POINT('Ctrl Pts',(-42.8392073306652,31.5404524382931,
-46.1912000897188));
#257134=CARTESIAN_POINT('Ctrl Pts',(-42.8392073306652,32.5039028869536,
-46.1328667563855));
#257135=CARTESIAN_POINT('Ctrl Pts',(-43.6735798944926,32.9856281112839,
-46.0745334230522));
#257136=CARTESIAN_POINT('Ctrl Pts',(-44.5079524583201,33.4673533356141,
-46.0162000897188));
#257137=CARTESIAN_POINT('Ctrl Pts',(-45.3423250221477,32.9856281112839,
-45.9578667563855));
#257138=CARTESIAN_POINT('Ctrl Pts',(-46.1766975859751,32.5039028869536,
-45.8995334230521));
#257139=CARTESIAN_POINT('Ctrl Pts',(-46.1766975859751,31.5404524382932,
-45.8412000897188));
#257140=CARTESIAN_POINT('Ctrl Pts',(-46.1766975859751,30.5770019896326,
-45.7828667563855));
#257141=CARTESIAN_POINT('Ctrl Pts',(-45.3423250221477,30.0952767653024,
-45.7245334230521));
#257142=CARTESIAN_POINT('Ctrl Pts',(-44.5079524583202,29.6135515409722,
-45.6662000897188));
#257143=CARTESIAN_POINT('Ctrl Pts',(-43.6735798944927,30.0952767653024,
-45.6078667563855));
#257144=CARTESIAN_POINT('Ctrl Pts',(-42.8392073306652,30.5770019896326,
-45.5495334230521));
#257145=CARTESIAN_POINT('Ctrl Pts',(-42.8392073306652,31.5404524382931,
-45.4912000897188));
#257146=CARTESIAN_POINT('Ctrl Pts',(-42.8392073306652,32.5039028869536,
-45.4328667563854));
#257147=CARTESIAN_POINT('Ctrl Pts',(-43.6735798944926,32.9856281112839,
-45.3745334230521));
#257148=CARTESIAN_POINT('Ctrl Pts',(-44.5079524583201,33.4673533356141,
-45.3162000897188));
#257149=CARTESIAN_POINT('Ctrl Pts',(-45.3423250221477,32.9856281112839,
-45.2578667563855));
#257150=CARTESIAN_POINT('Ctrl Pts',(-46.1766975859751,32.5039028869536,
-45.1995334230521));
#257151=CARTESIAN_POINT('Ctrl Pts',(-46.1766975859751,31.5404524382932,
-45.1412000897188));
#257152=CARTESIAN_POINT('Ctrl Pts',(-46.1766975859751,30.5770019896326,
-45.0828667563855));
#257153=CARTESIAN_POINT('Ctrl Pts',(-45.3423250221477,30.0952767653024,
-45.0245334230521));
#257154=CARTESIAN_POINT('Ctrl Pts',(-44.5079524583202,29.6135515409722,
-44.9662000897188));
#257155=CARTESIAN_POINT('Ctrl Pts',(-43.6735798944927,30.0952767653024,
-44.9078667563854));
#257156=CARTESIAN_POINT('Ctrl Pts',(-42.8392073306652,30.5770019896326,
-44.8495334230521));
#257157=CARTESIAN_POINT('Ctrl Pts',(-42.8392073306652,31.5404524382931,
-44.7912000897188));
#257158=CARTESIAN_POINT('Ctrl Pts',(-42.8392073306652,32.5039028869536,
-44.7328667563854));
#257159=CARTESIAN_POINT('Ctrl Pts',(-43.6735798944926,32.9856281112839,
-44.6745334230521));
#257160=CARTESIAN_POINT('Ctrl Pts',(-44.5079524583201,33.4673533356141,
-44.6162000897188));
#257161=CARTESIAN_POINT('Ctrl Pts',(-45.3423250221477,32.9856281112839,
-44.5578667563855));
#257162=CARTESIAN_POINT('Ctrl Pts',(-46.1766975859751,32.5039028869536,
-44.4995334230521));
#257163=CARTESIAN_POINT('Ctrl Pts',(-46.1766975859751,31.5404524382932,
-44.4412000897188));
#257164=CARTESIAN_POINT('Ctrl Pts',(-46.1766975859751,30.5770019896326,
-44.3828667563854));
#257165=CARTESIAN_POINT('Ctrl Pts',(-45.3423250221477,30.0952767653024,
-44.3245334230521));
#257166=CARTESIAN_POINT('Ctrl Pts',(-44.5079524583202,29.6135515409722,
-44.2662000897188));
#257167=CARTESIAN_POINT('Ctrl Pts',(-43.6735798944927,30.0952767653024,
-44.2078667563855));
#257168=CARTESIAN_POINT('Ctrl Pts',(-42.8392073306652,30.5770019896326,
-44.1495334230521));
#257169=CARTESIAN_POINT('Ctrl Pts',(-42.8392073306652,31.5404524382931,
-44.0912000897188));
#257170=CARTESIAN_POINT('Ctrl Pts',(-42.8392073306652,32.5039028869536,
-44.0328667563854));
#257171=CARTESIAN_POINT('Ctrl Pts',(-43.6735798944926,32.9856281112839,
-43.9745334230521));
#257172=CARTESIAN_POINT('Ctrl Pts',(-44.5079524583201,33.4673533356141,
-43.9162000897188));
#257173=CARTESIAN_POINT('Ctrl Pts',(-45.3423250221477,32.9856281112839,
-43.8578667563855));
#257174=CARTESIAN_POINT('Ctrl Pts',(-46.1766975859751,32.5039028869536,
-43.7995334230521));
#257175=CARTESIAN_POINT('Ctrl Pts',(-46.1766975859751,31.5404524382932,
-43.7412000897188));
#257176=CARTESIAN_POINT('Ctrl Pts',(-46.1766975859751,30.5770019896326,
-43.6828667563854));
#257177=CARTESIAN_POINT('Ctrl Pts',(-45.3423250221477,30.0952767653024,
-43.6245334230521));
#257178=CARTESIAN_POINT('Ctrl Pts',(-44.5079524583202,29.6135515409722,
-43.5662000897188));
#257179=CARTESIAN_POINT('Ctrl Pts',(-43.6735798944927,30.0952767653024,
-43.5078667563854));
#257180=CARTESIAN_POINT('Ctrl Pts',(-42.8392073306652,30.5770019896326,
-43.4495334230521));
#257181=CARTESIAN_POINT('Ctrl Pts',(-42.8392073306652,31.5404524382931,
-43.3912000897188));
#257182=CARTESIAN_POINT('Ctrl Pts',(-42.8392073306652,32.5039028869536,
-43.3328667563854));
#257183=CARTESIAN_POINT('Ctrl Pts',(-43.6735798944926,32.9856281112839,
-43.2745334230521));
#257184=CARTESIAN_POINT('Ctrl Pts',(-44.5079524583201,33.4673533356141,
-43.2162000897188));
#257185=CARTESIAN_POINT('Ctrl Pts',(-45.3423250221477,32.9856281112839,
-43.1578667563855));
#257186=CARTESIAN_POINT('Ctrl Pts',(-46.1766975859751,32.5039028869536,
-43.0995334230521));
#257187=CARTESIAN_POINT('Ctrl Pts',(-46.1766975859751,31.5404524382932,
-43.0412000897188));
#257188=CARTESIAN_POINT('Ctrl Pts',(-46.1766975859751,30.5770019896326,
-42.9828667563854));
#257189=CARTESIAN_POINT('Ctrl Pts',(-45.3423250221477,30.0952767653024,
-42.9245334230521));
#257190=CARTESIAN_POINT('Ctrl Pts',(-44.5079524583202,29.6135515409722,
-42.8662000897187));
#257191=CARTESIAN_POINT('Ctrl Pts',(-43.6735798944927,30.0952767653024,
-42.8078667563855));
#257192=CARTESIAN_POINT('Ctrl Pts',(-42.8392073306652,30.5770019896326,
-42.7495334230521));
#257193=CARTESIAN_POINT('Ctrl Pts',(-42.8392073306652,31.5404524382931,
-42.6912000897188));
#257194=CARTESIAN_POINT('Ctrl Pts',(-42.8392073306652,32.5039028869536,
-42.6328667563855));
#257195=CARTESIAN_POINT('Ctrl Pts',(-43.6735798944926,32.9856281112839,
-42.5745334230521));
#257196=CARTESIAN_POINT('Ctrl Pts',(-44.5079524583201,33.4673533356141,
-42.5162000897188));
#257197=CARTESIAN_POINT('Ctrl Pts',(-45.3423250221477,32.9856281112839,
-42.4578667563855));
#257198=CARTESIAN_POINT('Ctrl Pts',(-46.1766975859751,32.5039028869536,
-42.3995334230521));
#257199=CARTESIAN_POINT('Ctrl Pts',(-46.1766975859751,31.5404524382932,
-42.3412000897188));
#257200=CARTESIAN_POINT('Ctrl Pts',(-46.1766975859751,30.5770019896326,
-42.2828667563854));
#257201=CARTESIAN_POINT('Ctrl Pts',(-45.3423250221477,30.0952767653024,
-42.2245334230521));
#257202=CARTESIAN_POINT('Ctrl Pts',(-44.5079524583202,29.6135515409722,
-42.1662000897188));
#257203=CARTESIAN_POINT('Ctrl Pts',(-43.6735798944927,30.0952767653024,
-42.1078667563855));
#257204=CARTESIAN_POINT('Ctrl Pts',(-42.8392073306652,30.5770019896326,
-42.0495334230521));
#257205=CARTESIAN_POINT('Ctrl Pts',(-42.8392073306652,31.5404524382931,
-41.9912000897188));
#257206=CARTESIAN_POINT('Ctrl Pts',(-42.8392073306652,32.5039028869536,
-41.9328667563855));
#257207=CARTESIAN_POINT('Ctrl Pts',(-43.6735798944926,32.9856281112839,
-41.8745334230521));
#257208=CARTESIAN_POINT('Ctrl Pts',(-44.5079524583201,33.4673533356141,
-41.8162000897188));
#257209=CARTESIAN_POINT('Ctrl Pts',(-45.3423250221477,32.9856281112839,
-41.7578667563855));
#257210=CARTESIAN_POINT('Ctrl Pts',(-46.1766975859751,32.5039028869536,
-41.6995334230521));
#257211=CARTESIAN_POINT('Ctrl Pts',(-46.1766975859751,31.5404524382932,
-41.6412000897188));
#257212=CARTESIAN_POINT('Ctrl Pts',(-46.1766975859751,30.5770019896326,
-41.5828667563854));
#257213=CARTESIAN_POINT('Ctrl Pts',(-45.3423250221477,30.0952767653024,
-41.5245334230521));
#257214=CARTESIAN_POINT('Ctrl Pts',(-44.5079524583202,29.6135515409722,
-41.4662000897188));
#257215=CARTESIAN_POINT('Ctrl Pts',(-43.6735798944927,30.0952767653024,
-41.4078667563855));
#257216=CARTESIAN_POINT('Ctrl Pts',(-42.8392073306652,30.5770019896326,
-41.3495334230521));
#257217=CARTESIAN_POINT('Ctrl Pts',(-42.8392073306652,31.5404524382931,
-41.2912000897188));
#257218=CARTESIAN_POINT('Ctrl Pts',(-42.8392073306652,32.5039028869536,
-41.2328667563855));
#257219=CARTESIAN_POINT('Ctrl Pts',(-43.6735798944926,32.9856281112839,
-41.1745334230521));
#257220=CARTESIAN_POINT('Ctrl Pts',(-44.5079524583201,33.4673533356141,
-41.1162000897188));
#257221=CARTESIAN_POINT('Ctrl Pts',(-45.3423250221477,32.9856281112839,
-41.0578667563855));
#257222=CARTESIAN_POINT('Ctrl Pts',(-46.1766975859751,32.5039028869536,
-40.9995334230521));
#257223=CARTESIAN_POINT('Ctrl Pts',(-46.1766975859751,31.5404524382932,
-40.9412000897188));
#257224=CARTESIAN_POINT('Ctrl Pts',(-46.1766975859751,30.5770019896326,
-40.8828667563855));
#257225=CARTESIAN_POINT('Ctrl Pts',(-45.3423250221477,30.0952767653024,
-40.8245334230521));
#257226=CARTESIAN_POINT('Ctrl Pts',(-44.5079524583202,29.6135515409722,
-40.7662000897188));
#257227=CARTESIAN_POINT('Ctrl Pts',(-43.6735798944927,30.0952767653024,
-40.7078667563855));
#257228=CARTESIAN_POINT('Ctrl Pts',(-42.8392073306652,30.5770019896326,
-40.6495334230521));
#257229=CARTESIAN_POINT('Ctrl Pts',(-42.8392073306652,31.5404524382931,
-40.5912000897188));
#257230=CARTESIAN_POINT('Ctrl Pts',(-42.8392073306652,32.5039028869536,
-40.5328667563855));
#257231=CARTESIAN_POINT('Ctrl Pts',(-43.6735798944926,32.9856281112839,
-40.4745334230521));
#257232=CARTESIAN_POINT('Ctrl Pts',(-44.5079524583201,33.4673533356141,
-40.4162000897188));
#257233=CARTESIAN_POINT('Ctrl Pts',(-45.3423250221477,32.9856281112839,
-40.3578667563855));
#257234=CARTESIAN_POINT('Ctrl Pts',(-46.1766975859751,32.5039028869536,
-40.2995334230521));
#257235=CARTESIAN_POINT('Ctrl Pts',(-46.1766975859751,31.5404524382932,
-40.2412000897188));
#257236=CARTESIAN_POINT('Ctrl Pts',(-46.1766975859751,30.5770019896326,
-40.1828667563855));
#257237=CARTESIAN_POINT('Ctrl Pts',(-45.3423250221477,30.0952767653024,
-40.1245334230521));
#257238=CARTESIAN_POINT('Ctrl Pts',(-44.5079524583202,29.6135515409722,
-40.0662000897188));
#257239=CARTESIAN_POINT('Ctrl Pts',(-43.6735798944927,30.0952767653024,
-40.0078667563855));
#257240=CARTESIAN_POINT('Ctrl Pts',(-42.8392073306652,30.5770019896326,
-39.9495334230521));
#257241=CARTESIAN_POINT('Ctrl Pts',(-42.8392073306652,31.5404524382931,
-39.8912000897188));
#257242=CARTESIAN_POINT('Ctrl Pts',(-42.8392073306652,32.5039028869536,
-39.8328667563854));
#257243=CARTESIAN_POINT('Ctrl Pts',(-43.6735798944926,32.9856281112839,
-39.7745334230521));
#257244=CARTESIAN_POINT('Ctrl Pts',(-44.5079524583201,33.4673533356141,
-39.7162000897188));
#257245=CARTESIAN_POINT('Ctrl Pts',(-45.3423250221477,32.9856281112839,
-39.6578667563855));
#257246=CARTESIAN_POINT('Ctrl Pts',(-46.1766975859751,32.5039028869536,
-39.5995334230521));
#257247=CARTESIAN_POINT('Ctrl Pts',(-46.1766975859751,31.5404524382932,
-39.5412000897188));
#257248=CARTESIAN_POINT('Ctrl Pts',(-46.1766975859751,30.5770019896326,
-39.4828667563854));
#257249=CARTESIAN_POINT('Ctrl Pts',(-45.3423250221477,30.0952767653024,
-39.4245334230521));
#257250=CARTESIAN_POINT('Ctrl Pts',(-44.5079524583202,29.6135515409722,
-39.3662000897187));
#257251=CARTESIAN_POINT('Ctrl Pts',(-43.6735798944927,30.0952767653024,
-39.3078667563854));
#257252=CARTESIAN_POINT('Ctrl Pts',(-42.8392073306652,30.5770019896326,
-39.2495334230521));
#257253=CARTESIAN_POINT('Ctrl Pts',(-42.8392073306652,31.5404524382931,
-39.1912000897188));
#257254=CARTESIAN_POINT('Ctrl Pts',(-42.8392073306652,32.5039028869536,
-39.1328667563854));
#257255=CARTESIAN_POINT('Ctrl Pts',(-43.6735798944926,32.9856281112839,
-39.0745334230521));
#257256=CARTESIAN_POINT('Ctrl Pts',(-44.5079524583201,33.4673533356141,
-39.0162000897188));
#257257=CARTESIAN_POINT('Ctrl Pts',(-45.3423250221477,32.9856281112839,
-38.9578667563855));
#257258=CARTESIAN_POINT('Ctrl Pts',(-46.1766975859751,32.5039028869536,
-38.8995334230521));
#257259=CARTESIAN_POINT('Ctrl Pts',(-46.1766975859751,31.5404524382932,
-38.8412000897188));
#257260=CARTESIAN_POINT('Ctrl Pts',(-46.1766975859751,30.5770019896326,
-38.7828667563854));
#257261=CARTESIAN_POINT('Ctrl Pts',(-45.3423250221477,30.0952767653024,
-38.7245334230521));
#257262=CARTESIAN_POINT('Ctrl Pts',(-44.5079524583202,29.6135515409722,
-38.6662000897187));
#257263=CARTESIAN_POINT('Ctrl Pts',(-43.6735798944927,30.0952767653024,
-38.6078667563855));
#257264=CARTESIAN_POINT('Ctrl Pts',(-42.8392073306652,30.5770019896326,
-38.5495334230521));
#257265=CARTESIAN_POINT('Ctrl Pts',(-42.8392073306652,31.5404524382931,
-38.4912000897188));
#257266=CARTESIAN_POINT('Ctrl Pts',(-42.8392073306652,32.5039028869536,
-38.4328667563854));
#257267=CARTESIAN_POINT('Ctrl Pts',(-43.6735798944926,32.9856281112839,
-38.3745334230521));
#257268=CARTESIAN_POINT('Ctrl Pts',(-44.5079524583201,33.4673533356141,
-38.3162000897187));
#257269=CARTESIAN_POINT('Ctrl Pts',(-45.3423250221477,32.9856281112839,
-38.2578667563855));
#257270=CARTESIAN_POINT('Ctrl Pts',(-46.1766975859751,32.5039028869536,
-38.1995334230521));
#257271=CARTESIAN_POINT('Ctrl Pts',(-46.1766975859751,31.5404524382932,
-38.1412000897188));
#257272=CARTESIAN_POINT('Ctrl Pts',(-46.1766975859751,30.5770019896326,
-38.0828667563854));
#257273=CARTESIAN_POINT('Ctrl Pts',(-45.3423250221477,30.0952767653024,
-38.0245334230521));
#257274=CARTESIAN_POINT('Ctrl Pts',(-44.5079524583202,29.6135515409722,
-37.9662000897188));
#257275=CARTESIAN_POINT('Ctrl Pts',(-43.6735798944927,30.0952767653024,
-37.9078667563855));
#257276=CARTESIAN_POINT('Ctrl Pts',(-42.8392073306652,30.5770019896326,
-37.8495334230521));
#257277=CARTESIAN_POINT('Ctrl Pts',(-42.8392073306652,31.5404524382931,
-37.7912000897188));
#257278=CARTESIAN_POINT('Ctrl Pts',(-42.8392073306652,32.5039028869536,
-37.7328667563854));
#257279=CARTESIAN_POINT('Ctrl Pts',(-43.6735798944926,32.9856281112839,
-37.6745334230521));
#257280=CARTESIAN_POINT('Ctrl Pts',(-44.5079524583201,33.4673533356141,
-37.6162000897188));
#257281=CARTESIAN_POINT('Ctrl Pts',(-45.3423250221477,32.9856281112839,
-37.5578667563855));
#257282=CARTESIAN_POINT('Ctrl Pts',(-46.1766975859751,32.5039028869536,
-37.4995334230521));
#257283=CARTESIAN_POINT('Ctrl Pts',(-46.1766975859751,31.5404524382932,
-37.4412000897188));
#257284=CARTESIAN_POINT('Ctrl Pts',(-46.1766975859751,30.5770019896326,
-37.3828667563855));
#257285=CARTESIAN_POINT('Ctrl Pts',(-45.3423250221477,30.0952767653024,
-37.3245334230521));
#257286=CARTESIAN_POINT('Ctrl Pts',(-44.5079524583202,29.6135515409722,
-37.2662000897188));
#257287=CARTESIAN_POINT('Ctrl Pts',(-43.6735798944927,30.0952767653024,
-37.2078667563855));
#257288=CARTESIAN_POINT('Ctrl Pts',(-42.8392073306652,30.5770019896326,
-37.1495334230521));
#257289=CARTESIAN_POINT('Ctrl Pts',(-42.8392073306652,31.5404524382931,
-37.0912000897188));
#257290=CARTESIAN_POINT('Ctrl Pts',(-42.8392073306652,32.5039028869536,
-37.0328667563855));
#257291=CARTESIAN_POINT('Ctrl Pts',(-43.6735798944926,32.9856281112839,
-36.9745334230521));
#257292=CARTESIAN_POINT('Ctrl Pts',(-44.5079524583201,33.4673533356141,
-36.9162000897188));
#257293=CARTESIAN_POINT('Ctrl Pts',(-45.3423250221477,32.9856281112839,
-36.8578667563855));
#257294=CARTESIAN_POINT('Ctrl Pts',(-45.4506435553405,32.9230903769867,
-36.8502939029902));
#257295=CARTESIAN_POINT('Ctrl Pts',(-45.5484296067563,32.8451047309192,
-36.8421539138368));
#257296=CARTESIAN_POINT('Ctrl Pts',(-46.5079524583201,31.5404524382926,
-52.64995));
#257297=CARTESIAN_POINT('Ctrl Pts',(-46.4950120245211,31.3925617663045,
-52.64995));
#257298=CARTESIAN_POINT('Ctrl Pts',(-46.4647658835106,31.2467042332267,
-52.64995));
#257299=CARTESIAN_POINT('Ctrl Pts',(-46.374803322878,30.9770256287474,-52.64995));
#257300=CARTESIAN_POINT('Ctrl Pts',(-46.318075281921,30.8531799156226,-52.64995));
#257301=CARTESIAN_POINT('Ctrl Pts',(-46.1241199408216,30.5276040394677,
-52.64995));
#257302=CARTESIAN_POINT('Ctrl Pts',(-45.9605617229685,30.3447545989436,
-52.6499500000001));
#257303=CARTESIAN_POINT('Ctrl Pts',(-45.6181630929711,30.0852600117117,
-52.6499500000001));
#257304=CARTESIAN_POINT('Ctrl Pts',(-45.4037244819514,29.9562168938456,
-52.6499500000282));
#257305=CARTESIAN_POINT('Ctrl Pts',(-44.9862869603902,29.8483847666303,
-52.6499500000282));
#257306=CARTESIAN_POINT('Ctrl Pts',(-44.8386017522404,29.8303377940401,
-52.64995));
#257307=CARTESIAN_POINT('Ctrl Pts',(-44.5503390053885,29.8332193714484,
-52.64995));
#257308=CARTESIAN_POINT('Ctrl Pts',(-44.4109642294216,29.8520756782854,
-52.64995));
#257309=CARTESIAN_POINT('Ctrl Pts',(-44.2755200796091,29.8879736913688,
-52.64995));
#257310=CARTESIAN_POINT('Ctrl Pts',(-44.5079524583208,29.5404524382925,
-40.5749499999997));
#257311=CARTESIAN_POINT('Ctrl Pts',(-44.3968299128524,29.5404524382925,
-40.568467851514));
#257312=CARTESIAN_POINT('Ctrl Pts',(-44.2856405135298,29.5497134444641,
-40.5619818032202));
#257313=CARTESIAN_POINT('Ctrl Pts',(-43.9253649275659,29.6104363327409,
-40.5409657273724));
#257314=CARTESIAN_POINT('Ctrl Pts',(-43.6855666100239,29.6998090325789,
-40.5272829764295));
#257315=CARTESIAN_POINT('Ctrl Pts',(-43.2423657182469,29.9692774273866,
-40.5007432393533));
#257316=CARTESIAN_POINT('Ctrl Pts',(-43.0454921814785,30.1506824820443,
-40.4858368470313));
#257317=CARTESIAN_POINT('Ctrl Pts',(-42.7368235400766,30.5756684261979,
-40.4553645085971));
#257318=CARTESIAN_POINT('Ctrl Pts',(-42.6264497148207,30.8140446972255,
-40.4401029441556));
#257319=CARTESIAN_POINT('Ctrl Pts',(-42.5046488178855,31.3138038931373,
-40.4113035086948));
#257320=CARTESIAN_POINT('Ctrl Pts',(-42.4920854562892,31.5698862113898,
-40.3989258478379));
#257321=CARTESIAN_POINT('Ctrl Pts',(-42.5653797870039,32.0862857493079,
-40.3707005479556));
#257322=CARTESIAN_POINT('Ctrl Pts',(-42.6556867547492,32.3408286617681,
-40.3552075580647));
#257323=CARTESIAN_POINT('Ctrl Pts',(-42.9257217377094,32.7905245969834,
-40.324613731669));
#257324=CARTESIAN_POINT('Ctrl Pts',(-43.0994167252046,32.9834335181717,
-40.309802226329));
#257325=CARTESIAN_POINT('Ctrl Pts',(-43.5123894580008,33.2943941768154,
-40.2820480315413));
#257326=CARTESIAN_POINT('Ctrl Pts',(-43.7482931115836,33.4087109993068,
-40.2692634618935));
#257327=CARTESIAN_POINT('Ctrl Pts',(-44.2549423409082,33.5418863052154,
-40.2397089235162));
#257328=CARTESIAN_POINT('Ctrl Pts',(-44.5211480844148,33.5577692603707,
-40.2241802551449));
#257329=CARTESIAN_POINT('Ctrl Pts',(-45.034518162743,33.4865628518253,-40.1942336672423));
#257330=CARTESIAN_POINT('Ctrl Pts',(-45.2774019700598,33.4039470825283,
-40.1800654451487));
#257331=CARTESIAN_POINT('Ctrl Pts',(-45.7285228007267,33.1468187134193,
-40.1537500633597));
#257332=CARTESIAN_POINT('Ctrl Pts',(-45.9304658971415,32.9711079469821,
-40.1390674255521));
#257333=CARTESIAN_POINT('Ctrl Pts',(-46.2515389935812,32.5543478314764,
-40.1086488441459));
#257334=CARTESIAN_POINT('Ctrl Pts',(-46.3688060858683,32.3184704964571,
-40.0933124677031));
#257335=CARTESIAN_POINT('Ctrl Pts',(-46.5042019275048,31.8220614198178,
-40.0642857548446));
#257336=CARTESIAN_POINT('Ctrl Pts',(-46.5237882527671,31.5669899543883,
-40.051752503518));
#257337=CARTESIAN_POINT('Ctrl Pts',(-46.4653120508861,31.0514704111867,
-40.0240038547637));
#257338=CARTESIAN_POINT('Ctrl Pts',(-46.3832833125564,30.7965049593682,
-40.0087309673246));
#257339=CARTESIAN_POINT('Ctrl Pts',(-46.1281397073777,30.3398162423274,
-39.9782182103898));
#257340=CARTESIAN_POINT('Ctrl Pts',(-45.9599378712318,30.141059404952,-39.9632714960655));
#257341=CARTESIAN_POINT('Ctrl Pts',(-45.5574367799837,29.8185237628238,
-39.9352379774211));
#257342=CARTESIAN_POINT('Ctrl Pts',(-45.3270340049066,29.6977457571994,
-39.9227297568837));
#257343=CARTESIAN_POINT('Ctrl Pts',(-44.8940104176252,29.5684904717941,
-39.8974700476257));
#257344=CARTESIAN_POINT('Ctrl Pts',(-44.7012947640528,29.5404524382925,
-39.8862283011673));
#257345=CARTESIAN_POINT('Ctrl Pts',(-44.5079524583208,29.5404524382925,
-39.8749499999996));
#257346=CARTESIAN_POINT('Ctrl Pts',(-46.1766977413726,31.5404524382932,
-52.99995));
#257347=CARTESIAN_POINT('Ctrl Pts',(-46.1766977413726,30.5770018999139,
-52.9416166666667));
#257348=CARTESIAN_POINT('Ctrl Pts',(-45.3423250998464,30.0952766307242,
-52.8832833333334));
#257349=CARTESIAN_POINT('Ctrl Pts',(-44.5079524583202,29.6135513615346,
-52.82495));
#257350=CARTESIAN_POINT('Ctrl Pts',(-43.6735798167939,30.0952766307242,
-52.7666166666667));
#257351=CARTESIAN_POINT('Ctrl Pts',(-42.8392071752677,30.5770018999139,
-52.7082833333333));
#257352=CARTESIAN_POINT('Ctrl Pts',(-42.8392071752677,31.5404524382931,
-52.64995));
#257353=CARTESIAN_POINT('Ctrl Pts',(-42.8392071752677,32.5039029766724,
-52.5916166666666));
#257354=CARTESIAN_POINT('Ctrl Pts',(-43.6735798167939,32.985628245862,-52.5332833333334));
#257355=CARTESIAN_POINT('Ctrl Pts',(-44.5079524583201,33.4673535150516,
-52.4749500000001));
#257356=CARTESIAN_POINT('Ctrl Pts',(-45.3423250998464,32.985628245862,-52.4166166666667));
#257357=CARTESIAN_POINT('Ctrl Pts',(-46.1766977413726,32.5039029766724,
-52.3582833333334));
#257358=CARTESIAN_POINT('Ctrl Pts',(-46.1766977413726,31.5404524382932,
-52.29995));
#257359=CARTESIAN_POINT('Ctrl Pts',(-46.1766977413726,30.5770018999139,
-52.2416166666667));
#257360=CARTESIAN_POINT('Ctrl Pts',(-45.3423250998464,30.0952766307242,
-52.1832833333333));
#257361=CARTESIAN_POINT('Ctrl Pts',(-44.5079524583202,29.6135513615346,
-52.12495));
#257362=CARTESIAN_POINT('Ctrl Pts',(-43.6735798167939,30.0952766307242,
-52.0666166666667));
#257363=CARTESIAN_POINT('Ctrl Pts',(-42.8392071752677,30.5770018999139,
-52.0082833333333));
#257364=CARTESIAN_POINT('Ctrl Pts',(-42.8392071752677,31.5404524382931,
-51.94995));
#257365=CARTESIAN_POINT('Ctrl Pts',(-42.8392071752677,32.5039029766724,
-51.8916166666667));
#257366=CARTESIAN_POINT('Ctrl Pts',(-43.6735798167939,32.985628245862,-51.8332833333333));
#257367=CARTESIAN_POINT('Ctrl Pts',(-44.5079524583201,33.4673535150516,
-51.77495));
#257368=CARTESIAN_POINT('Ctrl Pts',(-45.3423250998464,32.985628245862,-51.7166166666667));
#257369=CARTESIAN_POINT('Ctrl Pts',(-46.1766977413726,32.5039029766724,
-51.6582833333333));
#257370=CARTESIAN_POINT('Ctrl Pts',(-46.1766977413726,31.5404524382932,
-51.59995));
#257371=CARTESIAN_POINT('Ctrl Pts',(-46.1766977413726,30.5770018999139,
-51.5416166666667));
#257372=CARTESIAN_POINT('Ctrl Pts',(-45.3423250998464,30.0952766307242,
-51.4832833333333));
#257373=CARTESIAN_POINT('Ctrl Pts',(-44.5079524583202,29.6135513615346,
-51.42495));
#257374=CARTESIAN_POINT('Ctrl Pts',(-43.6735798167939,30.0952766307242,
-51.3666166666667));
#257375=CARTESIAN_POINT('Ctrl Pts',(-42.8392071752677,30.5770018999139,
-51.3082833333333));
#257376=CARTESIAN_POINT('Ctrl Pts',(-42.8392071752677,31.5404524382931,
-51.24995));
#257377=CARTESIAN_POINT('Ctrl Pts',(-42.8392071752677,32.5039029766724,
-51.1916166666667));
#257378=CARTESIAN_POINT('Ctrl Pts',(-43.6735798167939,32.985628245862,-51.1332833333333));
#257379=CARTESIAN_POINT('Ctrl Pts',(-44.5079524583201,33.4673535150516,
-51.07495));
#257380=CARTESIAN_POINT('Ctrl Pts',(-45.3423250998464,32.985628245862,-51.0166166666667));
#257381=CARTESIAN_POINT('Ctrl Pts',(-46.1766977413726,32.5039029766724,
-50.9582833333334));
#257382=CARTESIAN_POINT('Ctrl Pts',(-46.1766977413726,31.5404524382932,
-50.89995));
#257383=CARTESIAN_POINT('Ctrl Pts',(-46.1766977413726,30.5770018999139,
-50.8416166666667));
#257384=CARTESIAN_POINT('Ctrl Pts',(-45.3423250998464,30.0952766307242,
-50.7832833333333));
#257385=CARTESIAN_POINT('Ctrl Pts',(-44.5079524583202,29.6135513615346,
-50.72495));
#257386=CARTESIAN_POINT('Ctrl Pts',(-43.6735798167939,30.0952766307242,
-50.6666166666667));
#257387=CARTESIAN_POINT('Ctrl Pts',(-42.8392071752677,30.5770018999139,
-50.6082833333334));
#257388=CARTESIAN_POINT('Ctrl Pts',(-42.8392071752677,31.5404524382931,
-50.54995));
#257389=CARTESIAN_POINT('Ctrl Pts',(-42.8392071752677,32.5039029766724,
-50.4916166666667));
#257390=CARTESIAN_POINT('Ctrl Pts',(-43.6735798167939,32.985628245862,-50.4332833333333));
#257391=CARTESIAN_POINT('Ctrl Pts',(-44.5079524583201,33.4673535150516,
-50.37495));
#257392=CARTESIAN_POINT('Ctrl Pts',(-45.3423250998464,32.985628245862,-50.3166166666667));
#257393=CARTESIAN_POINT('Ctrl Pts',(-46.1766977413726,32.5039029766724,
-50.2582833333334));
#257394=CARTESIAN_POINT('Ctrl Pts',(-46.1766977413726,31.5404524382932,
-50.19995));
#257395=CARTESIAN_POINT('Ctrl Pts',(-46.1766977413726,30.5770018999139,
-50.1416166666667));
#257396=CARTESIAN_POINT('Ctrl Pts',(-45.3423250998464,30.0952766307242,
-50.0832833333333));
#257397=CARTESIAN_POINT('Ctrl Pts',(-44.5079524583202,29.6135513615346,
-50.02495));
#257398=CARTESIAN_POINT('Ctrl Pts',(-43.6735798167939,30.0952766307242,
-49.9666166666667));
#257399=CARTESIAN_POINT('Ctrl Pts',(-42.8392071752677,30.5770018999139,
-49.9082833333334));
#257400=CARTESIAN_POINT('Ctrl Pts',(-42.8392071752677,31.5404524382931,
-49.84995));
#257401=CARTESIAN_POINT('Ctrl Pts',(-42.8392071752677,32.5039029766724,
-49.7916166666667));
#257402=CARTESIAN_POINT('Ctrl Pts',(-43.6735798167939,32.985628245862,-49.7332833333333));
#257403=CARTESIAN_POINT('Ctrl Pts',(-44.5079524583201,33.4673535150516,
-49.67495));
#257404=CARTESIAN_POINT('Ctrl Pts',(-45.3423250998464,32.985628245862,-49.6166166666667));
#257405=CARTESIAN_POINT('Ctrl Pts',(-46.1766977413726,32.5039029766724,
-49.5582833333334));
#257406=CARTESIAN_POINT('Ctrl Pts',(-46.1766977413726,31.5404524382932,
-49.49995));
#257407=CARTESIAN_POINT('Ctrl Pts',(-46.1766977413726,30.5770018999139,
-49.4416166666667));
#257408=CARTESIAN_POINT('Ctrl Pts',(-45.3423250998464,30.0952766307242,
-49.3832833333334));
#257409=CARTESIAN_POINT('Ctrl Pts',(-44.5079524583202,29.6135513615346,
-49.32495));
#257410=CARTESIAN_POINT('Ctrl Pts',(-43.6735798167939,30.0952766307242,
-49.2666166666667));
#257411=CARTESIAN_POINT('Ctrl Pts',(-42.8392071752677,30.5770018999139,
-49.2082833333334));
#257412=CARTESIAN_POINT('Ctrl Pts',(-42.8392071752677,31.5404524382931,
-49.14995));
#257413=CARTESIAN_POINT('Ctrl Pts',(-42.8392071752677,32.5039029766724,
-49.0916166666667));
#257414=CARTESIAN_POINT('Ctrl Pts',(-43.6735798167939,32.985628245862,-49.0332833333333));
#257415=CARTESIAN_POINT('Ctrl Pts',(-44.5079524583201,33.4673535150516,
-48.97495));
#257416=CARTESIAN_POINT('Ctrl Pts',(-45.3423250998464,32.985628245862,-48.9166166666667));
#257417=CARTESIAN_POINT('Ctrl Pts',(-46.1766977413726,32.5039029766724,
-48.8582833333333));
#257418=CARTESIAN_POINT('Ctrl Pts',(-46.1766977413726,31.5404524382932,
-48.79995));
#257419=CARTESIAN_POINT('Ctrl Pts',(-46.1766977413726,30.5770018999139,
-48.7416166666667));
#257420=CARTESIAN_POINT('Ctrl Pts',(-45.3423250998464,30.0952766307242,
-48.6832833333333));
#257421=CARTESIAN_POINT('Ctrl Pts',(-44.5079524583202,29.6135513615346,
-48.62495));
#257422=CARTESIAN_POINT('Ctrl Pts',(-43.6735798167939,30.0952766307242,
-48.5666166666667));
#257423=CARTESIAN_POINT('Ctrl Pts',(-42.8392071752677,30.5770018999139,
-48.5082833333333));
#257424=CARTESIAN_POINT('Ctrl Pts',(-42.8392071752677,31.5404524382931,
-48.44995));
#257425=CARTESIAN_POINT('Ctrl Pts',(-42.8392071752677,32.5039029766724,
-48.3916166666667));
#257426=CARTESIAN_POINT('Ctrl Pts',(-43.6735798167939,32.985628245862,-48.3332833333333));
#257427=CARTESIAN_POINT('Ctrl Pts',(-44.5079524583201,33.4673535150516,
-48.27495));
#257428=CARTESIAN_POINT('Ctrl Pts',(-45.3423250998464,32.985628245862,-48.2166166666667));
#257429=CARTESIAN_POINT('Ctrl Pts',(-46.1766977413726,32.5039029766724,
-48.1582833333333));
#257430=CARTESIAN_POINT('Ctrl Pts',(-46.1766977413726,31.5404524382932,
-48.09995));
#257431=CARTESIAN_POINT('Ctrl Pts',(-46.1766977413726,30.5770018999139,
-48.0416166666667));
#257432=CARTESIAN_POINT('Ctrl Pts',(-45.3423250998464,30.0952766307242,
-47.9832833333334));
#257433=CARTESIAN_POINT('Ctrl Pts',(-44.5079524583202,29.6135513615346,
-47.92495));
#257434=CARTESIAN_POINT('Ctrl Pts',(-43.6735798167939,30.0952766307242,
-47.8666166666667));
#257435=CARTESIAN_POINT('Ctrl Pts',(-42.8392071752677,30.5770018999139,
-47.8082833333333));
#257436=CARTESIAN_POINT('Ctrl Pts',(-42.8392071752677,31.5404524382931,
-47.74995));
#257437=CARTESIAN_POINT('Ctrl Pts',(-42.8392071752677,32.5039029766724,
-47.6916166666667));
#257438=CARTESIAN_POINT('Ctrl Pts',(-43.6735798167939,32.985628245862,-47.6332833333333));
#257439=CARTESIAN_POINT('Ctrl Pts',(-44.5079524583201,33.4673535150516,
-47.57495));
#257440=CARTESIAN_POINT('Ctrl Pts',(-45.3423250998464,32.985628245862,-47.5166166666667));
#257441=CARTESIAN_POINT('Ctrl Pts',(-46.1766977413726,32.5039029766724,
-47.4582833333333));
#257442=CARTESIAN_POINT('Ctrl Pts',(-46.1766977413726,31.5404524382932,
-47.39995));
#257443=CARTESIAN_POINT('Ctrl Pts',(-46.1766977413726,30.5770018999139,
-47.3416166666666));
#257444=CARTESIAN_POINT('Ctrl Pts',(-45.3423250998464,30.0952766307242,
-47.2832833333333));
#257445=CARTESIAN_POINT('Ctrl Pts',(-44.5079524583202,29.6135513615346,
-47.22495));
#257446=CARTESIAN_POINT('Ctrl Pts',(-43.6735798167939,30.0952766307242,
-47.1666166666667));
#257447=CARTESIAN_POINT('Ctrl Pts',(-42.8392071752677,30.5770018999139,
-47.1082833333333));
#257448=CARTESIAN_POINT('Ctrl Pts',(-42.8392071752677,31.5404524382931,
-47.04995));
#257449=CARTESIAN_POINT('Ctrl Pts',(-42.8392071752677,32.5039029766724,
-46.9916166666667));
#257450=CARTESIAN_POINT('Ctrl Pts',(-43.6735798167939,32.985628245862,-46.9332833333333));
#257451=CARTESIAN_POINT('Ctrl Pts',(-44.5079524583201,33.4673535150516,
-46.87495));
#257452=CARTESIAN_POINT('Ctrl Pts',(-45.3423250998464,32.985628245862,-46.8166166666667));
#257453=CARTESIAN_POINT('Ctrl Pts',(-46.1766977413726,32.5039029766724,
-46.7582833333333));
#257454=CARTESIAN_POINT('Ctrl Pts',(-46.1766977413726,31.5404524382932,
-46.69995));
#257455=CARTESIAN_POINT('Ctrl Pts',(-46.1766977413726,30.5770018999139,
-46.6416166666666));
#257456=CARTESIAN_POINT('Ctrl Pts',(-45.3423250998464,30.0952766307242,
-46.5832833333334));
#257457=CARTESIAN_POINT('Ctrl Pts',(-44.5079524583202,29.6135513615346,
-46.52495));
#257458=CARTESIAN_POINT('Ctrl Pts',(-43.6735798167939,30.0952766307242,
-46.4666166666667));
#257459=CARTESIAN_POINT('Ctrl Pts',(-42.8392071752677,30.5770018999139,
-46.4082833333333));
#257460=CARTESIAN_POINT('Ctrl Pts',(-42.8392071752677,31.5404524382931,
-46.34995));
#257461=CARTESIAN_POINT('Ctrl Pts',(-42.8392071752677,32.5039029766724,
-46.2916166666667));
#257462=CARTESIAN_POINT('Ctrl Pts',(-43.6735798167939,32.985628245862,-46.2332833333334));
#257463=CARTESIAN_POINT('Ctrl Pts',(-44.5079524583201,33.4673535150516,
-46.17495));
#257464=CARTESIAN_POINT('Ctrl Pts',(-45.3423250998464,32.985628245862,-46.1166166666667));
#257465=CARTESIAN_POINT('Ctrl Pts',(-46.1766977413726,32.5039029766724,
-46.0582833333333));
#257466=CARTESIAN_POINT('Ctrl Pts',(-46.1766977413726,31.5404524382932,
-45.99995));
#257467=CARTESIAN_POINT('Ctrl Pts',(-46.1766977413726,30.5770018999139,
-45.9416166666667));
#257468=CARTESIAN_POINT('Ctrl Pts',(-45.3423250998464,30.0952766307242,
-45.8832833333333));
#257469=CARTESIAN_POINT('Ctrl Pts',(-44.5079524583202,29.6135513615346,
-45.82495));
#257470=CARTESIAN_POINT('Ctrl Pts',(-43.6735798167939,30.0952766307242,
-45.7666166666667));
#257471=CARTESIAN_POINT('Ctrl Pts',(-42.8392071752677,30.5770018999139,
-45.7082833333333));
#257472=CARTESIAN_POINT('Ctrl Pts',(-42.8392071752677,31.5404524382931,
-45.64995));
#257473=CARTESIAN_POINT('Ctrl Pts',(-42.8392071752677,32.5039029766724,
-45.5916166666667));
#257474=CARTESIAN_POINT('Ctrl Pts',(-43.6735798167939,32.985628245862,-45.5332833333333));
#257475=CARTESIAN_POINT('Ctrl Pts',(-44.5079524583201,33.4673535150516,
-45.47495));
#257476=CARTESIAN_POINT('Ctrl Pts',(-45.3423250998464,32.985628245862,-45.4166166666667));
#257477=CARTESIAN_POINT('Ctrl Pts',(-46.1766977413726,32.5039029766724,
-45.3582833333333));
#257478=CARTESIAN_POINT('Ctrl Pts',(-46.1766977413726,31.5404524382932,
-45.29995));
#257479=CARTESIAN_POINT('Ctrl Pts',(-46.1766977413726,30.5770018999139,
-45.2416166666667));
#257480=CARTESIAN_POINT('Ctrl Pts',(-45.3423250998464,30.0952766307242,
-45.1832833333333));
#257481=CARTESIAN_POINT('Ctrl Pts',(-44.5079524583202,29.6135513615346,
-45.12495));
#257482=CARTESIAN_POINT('Ctrl Pts',(-43.6735798167939,30.0952766307242,
-45.0666166666667));
#257483=CARTESIAN_POINT('Ctrl Pts',(-42.8392071752677,30.5770018999139,
-45.0082833333334));
#257484=CARTESIAN_POINT('Ctrl Pts',(-42.8392071752677,31.5404524382931,
-44.94995));
#257485=CARTESIAN_POINT('Ctrl Pts',(-42.8392071752677,32.5039029766724,
-44.8916166666667));
#257486=CARTESIAN_POINT('Ctrl Pts',(-43.6735798167939,32.985628245862,-44.8332833333334));
#257487=CARTESIAN_POINT('Ctrl Pts',(-44.5079524583201,33.4673535150516,
-44.77495));
#257488=CARTESIAN_POINT('Ctrl Pts',(-45.3423250998464,32.985628245862,-44.7166166666667));
#257489=CARTESIAN_POINT('Ctrl Pts',(-46.1766977413726,32.5039029766724,
-44.6582833333333));
#257490=CARTESIAN_POINT('Ctrl Pts',(-46.1766977413726,31.5404524382932,
-44.59995));
#257491=CARTESIAN_POINT('Ctrl Pts',(-46.1766977413726,30.5770018999139,
-44.5416166666667));
#257492=CARTESIAN_POINT('Ctrl Pts',(-45.3423250998464,30.0952766307242,
-44.4832833333334));
#257493=CARTESIAN_POINT('Ctrl Pts',(-44.5079524583202,29.6135513615346,
-44.42495));
#257494=CARTESIAN_POINT('Ctrl Pts',(-43.6735798167939,30.0952766307242,
-44.3666166666667));
#257495=CARTESIAN_POINT('Ctrl Pts',(-42.8392071752677,30.5770018999139,
-44.3082833333334));
#257496=CARTESIAN_POINT('Ctrl Pts',(-42.8392071752677,31.5404524382931,
-44.24995));
#257497=CARTESIAN_POINT('Ctrl Pts',(-42.8392071752677,32.5039029766724,
-44.1916166666667));
#257498=CARTESIAN_POINT('Ctrl Pts',(-43.6735798167939,32.985628245862,-44.1332833333334));
#257499=CARTESIAN_POINT('Ctrl Pts',(-44.5079524583201,33.4673535150516,
-44.07495));
#257500=CARTESIAN_POINT('Ctrl Pts',(-45.3423250998464,32.985628245862,-44.0166166666667));
#257501=CARTESIAN_POINT('Ctrl Pts',(-46.1766977413726,32.5039029766724,
-43.9582833333334));
#257502=CARTESIAN_POINT('Ctrl Pts',(-46.1766977413726,31.5404524382932,
-43.89995));
#257503=CARTESIAN_POINT('Ctrl Pts',(-46.1766977413726,30.5770018999139,
-43.8416166666667));
#257504=CARTESIAN_POINT('Ctrl Pts',(-45.3423250998464,30.0952766307242,
-43.7832833333334));
#257505=CARTESIAN_POINT('Ctrl Pts',(-44.5079524583202,29.6135513615346,
-43.72495));
#257506=CARTESIAN_POINT('Ctrl Pts',(-43.6735798167939,30.0952766307242,
-43.6666166666667));
#257507=CARTESIAN_POINT('Ctrl Pts',(-42.8392071752677,30.5770018999139,
-43.6082833333333));
#257508=CARTESIAN_POINT('Ctrl Pts',(-42.8392071752677,31.5404524382931,
-43.54995));
#257509=CARTESIAN_POINT('Ctrl Pts',(-42.8392071752677,32.5039029766724,
-43.4916166666667));
#257510=CARTESIAN_POINT('Ctrl Pts',(-43.6735798167939,32.985628245862,-43.4332833333333));
#257511=CARTESIAN_POINT('Ctrl Pts',(-44.5079524583201,33.4673535150516,
-43.37495));
#257512=CARTESIAN_POINT('Ctrl Pts',(-45.3423250998464,32.985628245862,-43.3166166666667));
#257513=CARTESIAN_POINT('Ctrl Pts',(-46.1766977413726,32.5039029766724,
-43.2582833333333));
#257514=CARTESIAN_POINT('Ctrl Pts',(-46.1766977413726,31.5404524382932,
-43.19995));
#257515=CARTESIAN_POINT('Ctrl Pts',(-46.1766977413726,30.5770018999139,
-43.1416166666666));
#257516=CARTESIAN_POINT('Ctrl Pts',(-45.3423250998464,30.0952766307242,
-43.0832833333333));
#257517=CARTESIAN_POINT('Ctrl Pts',(-44.5079524583202,29.6135513615346,
-43.02495));
#257518=CARTESIAN_POINT('Ctrl Pts',(-43.6735798167939,30.0952766307242,
-42.9666166666667));
#257519=CARTESIAN_POINT('Ctrl Pts',(-42.8392071752677,30.5770018999139,
-42.9082833333333));
#257520=CARTESIAN_POINT('Ctrl Pts',(-42.8392071752677,31.5404524382931,
-42.84995));
#257521=CARTESIAN_POINT('Ctrl Pts',(-42.8392071752677,32.5039029766724,
-42.7916166666667));
#257522=CARTESIAN_POINT('Ctrl Pts',(-43.6735798167939,32.985628245862,-42.7332833333334));
#257523=CARTESIAN_POINT('Ctrl Pts',(-44.5079524583201,33.4673535150516,
-42.67495));
#257524=CARTESIAN_POINT('Ctrl Pts',(-45.3423250998464,32.985628245862,-42.6166166666667));
#257525=CARTESIAN_POINT('Ctrl Pts',(-46.1766977413726,32.5039029766724,
-42.5582833333333));
#257526=CARTESIAN_POINT('Ctrl Pts',(-46.1766977413726,31.5404524382932,
-42.49995));
#257527=CARTESIAN_POINT('Ctrl Pts',(-46.1766977413726,30.5770018999139,
-42.4416166666667));
#257528=CARTESIAN_POINT('Ctrl Pts',(-45.3423250998464,30.0952766307242,
-42.3832833333333));
#257529=CARTESIAN_POINT('Ctrl Pts',(-44.5079524583202,29.6135513615346,
-42.32495));
#257530=CARTESIAN_POINT('Ctrl Pts',(-43.6735798167939,30.0952766307242,
-42.2666166666667));
#257531=CARTESIAN_POINT('Ctrl Pts',(-42.8392071752677,30.5770018999139,
-42.2082833333333));
#257532=CARTESIAN_POINT('Ctrl Pts',(-42.8392071752677,31.5404524382931,
-42.14995));
#257533=CARTESIAN_POINT('Ctrl Pts',(-42.8392071752677,32.5039029766724,
-42.0916166666667));
#257534=CARTESIAN_POINT('Ctrl Pts',(-43.6735798167939,32.985628245862,-42.0332833333334));
#257535=CARTESIAN_POINT('Ctrl Pts',(-44.5079524583201,33.4673535150516,
-41.97495));
#257536=CARTESIAN_POINT('Ctrl Pts',(-45.3423250998464,32.985628245862,-41.9166166666666));
#257537=CARTESIAN_POINT('Ctrl Pts',(-46.1766977413726,32.5039029766724,
-41.8582833333333));
#257538=CARTESIAN_POINT('Ctrl Pts',(-46.1766977413726,31.5404524382932,
-41.79995));
#257539=CARTESIAN_POINT('Ctrl Pts',(-46.1766977413726,30.5770018999139,
-41.7416166666667));
#257540=CARTESIAN_POINT('Ctrl Pts',(-45.3423250998464,30.0952766307242,
-41.6832833333333));
#257541=CARTESIAN_POINT('Ctrl Pts',(-44.5079524583202,29.6135513615346,
-41.62495));
#257542=CARTESIAN_POINT('Ctrl Pts',(-43.6735798167939,30.0952766307242,
-41.5666166666667));
#257543=CARTESIAN_POINT('Ctrl Pts',(-42.8392071752677,30.5770018999139,
-41.5082833333334));
#257544=CARTESIAN_POINT('Ctrl Pts',(-42.8392071752677,31.5404524382931,
-41.44995));
#257545=CARTESIAN_POINT('Ctrl Pts',(-42.8392071752677,32.5039029766724,
-41.3916166666667));
#257546=CARTESIAN_POINT('Ctrl Pts',(-43.6735798167939,32.985628245862,-41.3332833333334));
#257547=CARTESIAN_POINT('Ctrl Pts',(-44.5079524583201,33.4673535150516,
-41.27495));
#257548=CARTESIAN_POINT('Ctrl Pts',(-45.3423250998464,32.985628245862,-41.2166166666667));
#257549=CARTESIAN_POINT('Ctrl Pts',(-46.1766977413726,32.5039029766724,
-41.1582833333333));
#257550=CARTESIAN_POINT('Ctrl Pts',(-46.1766977413726,31.5404524382932,
-41.09995));
#257551=CARTESIAN_POINT('Ctrl Pts',(-46.1766977413726,30.5770018999139,
-41.0416166666667));
#257552=CARTESIAN_POINT('Ctrl Pts',(-45.3423250998464,30.0952766307242,
-40.9832833333333));
#257553=CARTESIAN_POINT('Ctrl Pts',(-44.5079524583202,29.6135513615346,
-40.92495));
#257554=CARTESIAN_POINT('Ctrl Pts',(-43.6735798167939,30.0952766307242,
-40.8666166666667));
#257555=CARTESIAN_POINT('Ctrl Pts',(-42.8392071752677,30.5770018999139,
-40.8082833333334));
#257556=CARTESIAN_POINT('Ctrl Pts',(-42.8392071752677,31.5404524382931,
-40.74995));
#257557=CARTESIAN_POINT('Ctrl Pts',(-42.8392071752677,32.5039029766724,
-40.6916166666667));
#257558=CARTESIAN_POINT('Ctrl Pts',(-43.6735798167939,32.985628245862,-40.6332833333334));
#257559=CARTESIAN_POINT('Ctrl Pts',(-44.5079524583201,33.4673535150516,
-40.57495));
#257560=CARTESIAN_POINT('Ctrl Pts',(-45.3423250998464,32.985628245862,-40.5166166666666));
#257561=CARTESIAN_POINT('Ctrl Pts',(-46.1766977413726,32.5039029766724,
-40.4582833333333));
#257562=CARTESIAN_POINT('Ctrl Pts',(-46.1766977413726,31.5404524382932,
-40.39995));
#257563=CARTESIAN_POINT('Ctrl Pts',(-46.1766977413726,30.5770018999139,
-40.3416166666667));
#257564=CARTESIAN_POINT('Ctrl Pts',(-45.3423250998464,30.0952766307242,
-40.2832833333334));
#257565=CARTESIAN_POINT('Ctrl Pts',(-44.5079524583202,29.6135513615346,
-40.22495));
#257566=CARTESIAN_POINT('Ctrl Pts',(-43.6735798167939,30.0952766307242,
-40.1666166666667));
#257567=CARTESIAN_POINT('Ctrl Pts',(-42.8392071752677,30.5770018999139,
-40.1082833333334));
#257568=CARTESIAN_POINT('Ctrl Pts',(-42.8392071752677,31.5404524382931,
-40.04995));
#257569=CARTESIAN_POINT('Ctrl Pts',(-42.8392071752677,32.5039029766724,
-39.9916166666667));
#257570=CARTESIAN_POINT('Ctrl Pts',(-43.6735798167939,32.985628245862,-39.9332833333333));
#257571=CARTESIAN_POINT('Ctrl Pts',(-44.5079524583201,33.4673535150516,
-39.87495));
#257572=CARTESIAN_POINT('Ctrl Pts',(-45.3423250998464,32.985628245862,-39.8166166666667));
#257573=CARTESIAN_POINT('Ctrl Pts',(-46.1766977413726,32.5039029766724,
-39.7582833333334));
#257574=CARTESIAN_POINT('Ctrl Pts',(-46.1766977413726,31.5404524382932,
-39.69995));
#257575=CARTESIAN_POINT('Ctrl Pts',(-46.1766977413726,30.5770018999139,
-39.6416166666667));
#257576=CARTESIAN_POINT('Ctrl Pts',(-45.3423250998464,30.0952766307242,
-39.5832833333333));
#257577=CARTESIAN_POINT('Ctrl Pts',(-44.5079524583202,29.6135513615346,
-39.52495));
#257578=CARTESIAN_POINT('Ctrl Pts',(-43.6735798167939,30.0952766307242,
-39.4666166666667));
#257579=CARTESIAN_POINT('Ctrl Pts',(-42.8392071752677,30.5770018999139,
-39.4082833333333));
#257580=CARTESIAN_POINT('Ctrl Pts',(-42.8392071752677,31.5404524382931,
-39.34995));
#257581=CARTESIAN_POINT('Ctrl Pts',(-42.8392071752677,32.5039029766724,
-39.2916166666667));
#257582=CARTESIAN_POINT('Ctrl Pts',(-43.6735798167939,32.985628245862,-39.2332833333333));
#257583=CARTESIAN_POINT('Ctrl Pts',(-44.5079524583201,33.4673535150516,
-39.17495));
#257584=CARTESIAN_POINT('Ctrl Pts',(-45.3423250998464,32.985628245862,-39.1166166666667));
#257585=CARTESIAN_POINT('Ctrl Pts',(-46.1766977413726,32.5039029766724,
-39.0582833333333));
#257586=CARTESIAN_POINT('Ctrl Pts',(-46.1766977413726,31.5404524382932,
-38.99995));
#257587=CARTESIAN_POINT('Ctrl Pts',(-46.1766977413726,30.5770018999139,
-38.9416166666667));
#257588=CARTESIAN_POINT('Ctrl Pts',(-45.3423250998464,30.0952766307242,
-38.8832833333334));
#257589=CARTESIAN_POINT('Ctrl Pts',(-44.5079524583202,29.6135513615346,
-38.82495));
#257590=CARTESIAN_POINT('Ctrl Pts',(-43.6735798167939,30.0952766307242,
-38.7666166666667));
#257591=CARTESIAN_POINT('Ctrl Pts',(-42.8392071752677,30.5770018999139,
-38.7082833333333));
#257592=CARTESIAN_POINT('Ctrl Pts',(-42.8392071752677,31.5404524382931,
-38.64995));
#257593=CARTESIAN_POINT('Ctrl Pts',(-42.8392071752677,32.5039029766724,
-38.5916166666667));
#257594=CARTESIAN_POINT('Ctrl Pts',(-43.6735798167939,32.985628245862,-38.5332833333334));
#257595=CARTESIAN_POINT('Ctrl Pts',(-44.5079524583201,33.4673535150516,
-38.47495));
#257596=CARTESIAN_POINT('Ctrl Pts',(-45.3423250998464,32.985628245862,-38.4166166666667));
#257597=CARTESIAN_POINT('Ctrl Pts',(-46.1766977413726,32.5039029766724,
-38.3582833333333));
#257598=CARTESIAN_POINT('Ctrl Pts',(-46.1766977413726,31.5404524382932,
-38.29995));
#257599=CARTESIAN_POINT('Ctrl Pts',(-46.1766977413726,30.5770018999139,
-38.2416166666667));
#257600=CARTESIAN_POINT('Ctrl Pts',(-45.3423250998464,30.0952766307242,
-38.1832833333333));
#257601=CARTESIAN_POINT('Ctrl Pts',(-44.5079524583202,29.6135513615346,
-38.12495));
#257602=CARTESIAN_POINT('Ctrl Pts',(-43.6735798167939,30.0952766307242,
-38.0666166666667));
#257603=CARTESIAN_POINT('Ctrl Pts',(-42.8392071752677,30.5770018999139,
-38.0082833333333));
#257604=CARTESIAN_POINT('Ctrl Pts',(-42.8392071752677,31.5404524382931,
-37.94995));
#257605=CARTESIAN_POINT('Ctrl Pts',(-42.8392071752677,32.5039029766724,
-37.8916166666667));
#257606=CARTESIAN_POINT('Ctrl Pts',(-43.6735798167939,32.985628245862,-37.8332833333334));
#257607=CARTESIAN_POINT('Ctrl Pts',(-44.5079524583201,33.4673535150516,
-37.77495));
#257608=CARTESIAN_POINT('Ctrl Pts',(-45.3423250998464,32.985628245862,-37.7166166666667));
#257609=CARTESIAN_POINT('Ctrl Pts',(-46.1766977413726,32.5039029766724,
-37.6582833333333));
#257610=CARTESIAN_POINT('Ctrl Pts',(-46.1766977413726,31.5404524382932,
-37.59995));
#257611=CARTESIAN_POINT('Ctrl Pts',(-46.1766977413726,30.5770018999139,
-37.5416166666667));
#257612=CARTESIAN_POINT('Ctrl Pts',(-45.3423250998464,30.0952766307242,
-37.4832833333334));
#257613=CARTESIAN_POINT('Ctrl Pts',(-44.5079524583202,29.6135513615346,
-37.42495));
#257614=CARTESIAN_POINT('Ctrl Pts',(-43.6735798167939,30.0952766307242,
-37.3666166666667));
#257615=CARTESIAN_POINT('Ctrl Pts',(-42.8392071752677,30.5770018999139,
-37.3082833333333));
#257616=CARTESIAN_POINT('Ctrl Pts',(-42.8392071752677,31.5404524382931,
-37.24995));
#257617=CARTESIAN_POINT('Ctrl Pts',(-42.8392071752677,32.5039029766724,
-37.1916166666667));
#257618=CARTESIAN_POINT('Ctrl Pts',(-43.6735798167939,32.985628245862,-37.1332833333334));
#257619=CARTESIAN_POINT('Ctrl Pts',(-44.5079524583201,33.4673535150516,
-37.07495));
#257620=CARTESIAN_POINT('Ctrl Pts',(-45.3423250998464,32.985628245862,-37.0166166666667));
#257621=CARTESIAN_POINT('Ctrl Pts',(-45.4506530446704,32.9230850777571,
-37.0090431559831));
#257622=CARTESIAN_POINT('Ctrl Pts',(-45.5484465834729,32.8450913903532,
-37.0009024189827));
#257623=CARTESIAN_POINT('Ctrl Pts',(-46.5766932247455,31.5404524382932,
-53.2308875));
#257624=CARTESIAN_POINT('Ctrl Pts',(-46.5766932247455,30.3460643999139,
-53.1725541666667));
#257625=CARTESIAN_POINT('Ctrl Pts',(-45.5423228415329,29.7488703807243,
-53.1142208333334));
#257626=CARTESIAN_POINT('Ctrl Pts',(-44.5079524583202,29.1516763615346,
-53.0558875000001));
#257627=CARTESIAN_POINT('Ctrl Pts',(-43.4735820751074,29.7488703807243,
-52.9975541666667));
#257628=CARTESIAN_POINT('Ctrl Pts',(-42.4392116918948,30.3460643999138,
-52.9392208333334));
#257629=CARTESIAN_POINT('Ctrl Pts',(-42.4392116918948,31.5404524382931,
-52.8808875));
#257630=CARTESIAN_POINT('Ctrl Pts',(-42.4392116918947,32.7348404766723,
-52.8225541666667));
#257631=CARTESIAN_POINT('Ctrl Pts',(-43.4735820751074,33.332034495862,-52.7642208333334));
#257632=CARTESIAN_POINT('Ctrl Pts',(-44.5079524583201,33.9292285150516,
-52.7058875));
#257633=CARTESIAN_POINT('Ctrl Pts',(-45.5423228415328,33.332034495862,-52.6475541666667));
#257634=CARTESIAN_POINT('Ctrl Pts',(-46.5766932247455,32.7348404766724,
-52.5892208333333));
#257635=CARTESIAN_POINT('Ctrl Pts',(-46.5766932247455,31.5404524382932,
-52.5308875));
#257636=CARTESIAN_POINT('Ctrl Pts',(-46.5766932247455,30.3460643999139,
-52.4725541666667));
#257637=CARTESIAN_POINT('Ctrl Pts',(-45.5423228415329,29.7488703807243,
-52.4142208333333));
#257638=CARTESIAN_POINT('Ctrl Pts',(-44.5079524583202,29.1516763615346,
-52.3558875000001));
#257639=CARTESIAN_POINT('Ctrl Pts',(-43.4735820751074,29.7488703807243,
-52.2975541666667));
#257640=CARTESIAN_POINT('Ctrl Pts',(-42.4392116918948,30.3460643999138,
-52.2392208333334));
#257641=CARTESIAN_POINT('Ctrl Pts',(-42.4392116918948,31.5404524382931,
-52.1808875));
#257642=CARTESIAN_POINT('Ctrl Pts',(-42.4392116918947,32.7348404766723,
-52.1225541666667));
#257643=CARTESIAN_POINT('Ctrl Pts',(-43.4735820751074,33.332034495862,-52.0642208333334));
#257644=CARTESIAN_POINT('Ctrl Pts',(-44.5079524583201,33.9292285150516,
-52.0058875));
#257645=CARTESIAN_POINT('Ctrl Pts',(-45.5423228415328,33.332034495862,-51.9475541666667));
#257646=CARTESIAN_POINT('Ctrl Pts',(-46.5766932247455,32.7348404766724,
-51.8892208333334));
#257647=CARTESIAN_POINT('Ctrl Pts',(-46.5766932247455,31.5404524382932,
-51.8308875));
#257648=CARTESIAN_POINT('Ctrl Pts',(-46.5766932247455,30.3460643999139,
-51.7725541666667));
#257649=CARTESIAN_POINT('Ctrl Pts',(-45.5423228415329,29.7488703807243,
-51.7142208333334));
#257650=CARTESIAN_POINT('Ctrl Pts',(-44.5079524583202,29.1516763615346,
-51.6558875));
#257651=CARTESIAN_POINT('Ctrl Pts',(-43.4735820751074,29.7488703807243,
-51.5975541666667));
#257652=CARTESIAN_POINT('Ctrl Pts',(-42.4392116918948,30.3460643999138,
-51.5392208333333));
#257653=CARTESIAN_POINT('Ctrl Pts',(-42.4392116918948,31.5404524382931,
-51.4808875));
#257654=CARTESIAN_POINT('Ctrl Pts',(-42.4392116918947,32.7348404766723,
-51.4225541666667));
#257655=CARTESIAN_POINT('Ctrl Pts',(-43.4735820751074,33.332034495862,-51.3642208333334));
#257656=CARTESIAN_POINT('Ctrl Pts',(-44.5079524583201,33.9292285150516,
-51.3058875));
#257657=CARTESIAN_POINT('Ctrl Pts',(-45.5423228415328,33.332034495862,-51.2475541666667));
#257658=CARTESIAN_POINT('Ctrl Pts',(-46.5766932247455,32.7348404766724,
-51.1892208333333));
#257659=CARTESIAN_POINT('Ctrl Pts',(-46.5766932247455,31.5404524382932,
-51.1308875));
#257660=CARTESIAN_POINT('Ctrl Pts',(-46.5766932247455,30.3460643999139,
-51.0725541666667));
#257661=CARTESIAN_POINT('Ctrl Pts',(-45.5423228415329,29.7488703807243,
-51.0142208333334));
#257662=CARTESIAN_POINT('Ctrl Pts',(-44.5079524583202,29.1516763615346,
-50.9558875));
#257663=CARTESIAN_POINT('Ctrl Pts',(-43.4735820751074,29.7488703807243,
-50.8975541666667));
#257664=CARTESIAN_POINT('Ctrl Pts',(-42.4392116918948,30.3460643999138,
-50.8392208333333));
#257665=CARTESIAN_POINT('Ctrl Pts',(-42.4392116918948,31.5404524382931,
-50.7808875));
#257666=CARTESIAN_POINT('Ctrl Pts',(-42.4392116918947,32.7348404766723,
-50.7225541666666));
#257667=CARTESIAN_POINT('Ctrl Pts',(-43.4735820751074,33.332034495862,-50.6642208333333));
#257668=CARTESIAN_POINT('Ctrl Pts',(-44.5079524583201,33.9292285150516,
-50.6058875));
#257669=CARTESIAN_POINT('Ctrl Pts',(-45.5423228415328,33.332034495862,-50.5475541666667));
#257670=CARTESIAN_POINT('Ctrl Pts',(-46.5766932247455,32.7348404766724,
-50.4892208333333));
#257671=CARTESIAN_POINT('Ctrl Pts',(-46.5766932247455,31.5404524382932,
-50.4308875));
#257672=CARTESIAN_POINT('Ctrl Pts',(-46.5766932247455,30.3460643999139,
-50.3725541666667));
#257673=CARTESIAN_POINT('Ctrl Pts',(-45.5423228415329,29.7488703807243,
-50.3142208333334));
#257674=CARTESIAN_POINT('Ctrl Pts',(-44.5079524583202,29.1516763615346,
-50.2558875));
#257675=CARTESIAN_POINT('Ctrl Pts',(-43.4735820751074,29.7488703807243,
-50.1975541666667));
#257676=CARTESIAN_POINT('Ctrl Pts',(-42.4392116918948,30.3460643999138,
-50.1392208333333));
#257677=CARTESIAN_POINT('Ctrl Pts',(-42.4392116918948,31.5404524382931,
-50.0808875));
#257678=CARTESIAN_POINT('Ctrl Pts',(-42.4392116918947,32.7348404766723,
-50.0225541666667));
#257679=CARTESIAN_POINT('Ctrl Pts',(-43.4735820751074,33.332034495862,-49.9642208333334));
#257680=CARTESIAN_POINT('Ctrl Pts',(-44.5079524583201,33.9292285150516,
-49.9058875));
#257681=CARTESIAN_POINT('Ctrl Pts',(-45.5423228415328,33.332034495862,-49.8475541666667));
#257682=CARTESIAN_POINT('Ctrl Pts',(-46.5766932247455,32.7348404766724,
-49.7892208333333));
#257683=CARTESIAN_POINT('Ctrl Pts',(-46.5766932247455,31.5404524382932,
-49.7308875));
#257684=CARTESIAN_POINT('Ctrl Pts',(-46.5766932247455,30.3460643999139,
-49.6725541666667));
#257685=CARTESIAN_POINT('Ctrl Pts',(-45.5423228415329,29.7488703807243,
-49.6142208333334));
#257686=CARTESIAN_POINT('Ctrl Pts',(-44.5079524583202,29.1516763615346,
-49.5558875));
#257687=CARTESIAN_POINT('Ctrl Pts',(-43.4735820751074,29.7488703807243,
-49.4975541666667));
#257688=CARTESIAN_POINT('Ctrl Pts',(-42.4392116918948,30.3460643999138,
-49.4392208333333));
#257689=CARTESIAN_POINT('Ctrl Pts',(-42.4392116918948,31.5404524382931,
-49.3808875));
#257690=CARTESIAN_POINT('Ctrl Pts',(-42.4392116918947,32.7348404766723,
-49.3225541666667));
#257691=CARTESIAN_POINT('Ctrl Pts',(-43.4735820751074,33.332034495862,-49.2642208333334));
#257692=CARTESIAN_POINT('Ctrl Pts',(-44.5079524583201,33.9292285150516,
-49.2058875));
#257693=CARTESIAN_POINT('Ctrl Pts',(-45.5423228415328,33.332034495862,-49.1475541666667));
#257694=CARTESIAN_POINT('Ctrl Pts',(-46.5766932247455,32.7348404766724,
-49.0892208333333));
#257695=CARTESIAN_POINT('Ctrl Pts',(-46.5766932247455,31.5404524382932,
-49.0308875));
#257696=CARTESIAN_POINT('Ctrl Pts',(-46.5766932247455,30.3460643999139,
-48.9725541666667));
#257697=CARTESIAN_POINT('Ctrl Pts',(-45.5423228415329,29.7488703807243,
-48.9142208333333));
#257698=CARTESIAN_POINT('Ctrl Pts',(-44.5079524583202,29.1516763615346,
-48.8558875));
#257699=CARTESIAN_POINT('Ctrl Pts',(-43.4735820751074,29.7488703807243,
-48.7975541666667));
#257700=CARTESIAN_POINT('Ctrl Pts',(-42.4392116918948,30.3460643999138,
-48.7392208333334));
#257701=CARTESIAN_POINT('Ctrl Pts',(-42.4392116918948,31.5404524382931,
-48.6808875));
#257702=CARTESIAN_POINT('Ctrl Pts',(-42.4392116918947,32.7348404766723,
-48.6225541666667));
#257703=CARTESIAN_POINT('Ctrl Pts',(-43.4735820751074,33.332034495862,-48.5642208333334));
#257704=CARTESIAN_POINT('Ctrl Pts',(-44.5079524583201,33.9292285150516,
-48.5058875));
#257705=CARTESIAN_POINT('Ctrl Pts',(-45.5423228415328,33.332034495862,-48.4475541666667));
#257706=CARTESIAN_POINT('Ctrl Pts',(-46.5766932247455,32.7348404766724,
-48.3892208333334));
#257707=CARTESIAN_POINT('Ctrl Pts',(-46.5766932247455,31.5404524382932,
-48.3308875));
#257708=CARTESIAN_POINT('Ctrl Pts',(-46.5766932247455,30.3460643999139,
-48.2725541666667));
#257709=CARTESIAN_POINT('Ctrl Pts',(-45.5423228415329,29.7488703807243,
-48.2142208333334));
#257710=CARTESIAN_POINT('Ctrl Pts',(-44.5079524583202,29.1516763615346,
-48.1558875));
#257711=CARTESIAN_POINT('Ctrl Pts',(-43.4735820751074,29.7488703807243,
-48.0975541666667));
#257712=CARTESIAN_POINT('Ctrl Pts',(-42.4392116918948,30.3460643999138,
-48.0392208333334));
#257713=CARTESIAN_POINT('Ctrl Pts',(-42.4392116918948,31.5404524382931,
-47.9808875));
#257714=CARTESIAN_POINT('Ctrl Pts',(-42.4392116918947,32.7348404766723,
-47.9225541666667));
#257715=CARTESIAN_POINT('Ctrl Pts',(-43.4735820751074,33.332034495862,-47.8642208333334));
#257716=CARTESIAN_POINT('Ctrl Pts',(-44.5079524583201,33.9292285150516,
-47.8058875000001));
#257717=CARTESIAN_POINT('Ctrl Pts',(-45.5423228415328,33.332034495862,-47.7475541666667));
#257718=CARTESIAN_POINT('Ctrl Pts',(-46.5766932247455,32.7348404766724,
-47.6892208333334));
#257719=CARTESIAN_POINT('Ctrl Pts',(-46.5766932247455,31.5404524382932,
-47.6308875));
#257720=CARTESIAN_POINT('Ctrl Pts',(-46.5766932247455,30.3460643999139,
-47.5725541666667));
#257721=CARTESIAN_POINT('Ctrl Pts',(-45.5423228415329,29.7488703807243,
-47.5142208333333));
#257722=CARTESIAN_POINT('Ctrl Pts',(-44.5079524583202,29.1516763615346,
-47.4558875));
#257723=CARTESIAN_POINT('Ctrl Pts',(-43.4735820751074,29.7488703807243,
-47.3975541666667));
#257724=CARTESIAN_POINT('Ctrl Pts',(-42.4392116918948,30.3460643999138,
-47.3392208333333));
#257725=CARTESIAN_POINT('Ctrl Pts',(-42.4392116918948,31.5404524382931,
-47.2808875));
#257726=CARTESIAN_POINT('Ctrl Pts',(-42.4392116918947,32.7348404766723,
-47.2225541666667));
#257727=CARTESIAN_POINT('Ctrl Pts',(-43.4735820751074,33.332034495862,-47.1642208333334));
#257728=CARTESIAN_POINT('Ctrl Pts',(-44.5079524583201,33.9292285150516,
-47.1058875));
#257729=CARTESIAN_POINT('Ctrl Pts',(-45.5423228415328,33.332034495862,-47.0475541666667));
#257730=CARTESIAN_POINT('Ctrl Pts',(-46.5766932247455,32.7348404766724,
-46.9892208333334));
#257731=CARTESIAN_POINT('Ctrl Pts',(-46.5766932247455,31.5404524382932,
-46.9308875));
#257732=CARTESIAN_POINT('Ctrl Pts',(-46.5766932247455,30.3460643999139,
-46.8725541666667));
#257733=CARTESIAN_POINT('Ctrl Pts',(-45.5423228415329,29.7488703807243,
-46.8142208333334));
#257734=CARTESIAN_POINT('Ctrl Pts',(-44.5079524583202,29.1516763615346,
-46.7558875));
#257735=CARTESIAN_POINT('Ctrl Pts',(-43.4735820751074,29.7488703807243,
-46.6975541666667));
#257736=CARTESIAN_POINT('Ctrl Pts',(-42.4392116918948,30.3460643999138,
-46.6392208333333));
#257737=CARTESIAN_POINT('Ctrl Pts',(-42.4392116918948,31.5404524382931,
-46.5808875));
#257738=CARTESIAN_POINT('Ctrl Pts',(-42.4392116918948,32.7348404766723,
-46.5225541666667));
#257739=CARTESIAN_POINT('Ctrl Pts',(-43.4735820751074,33.332034495862,-46.4642208333334));
#257740=CARTESIAN_POINT('Ctrl Pts',(-44.5079524583201,33.9292285150516,
-46.4058875));
#257741=CARTESIAN_POINT('Ctrl Pts',(-45.5423228415328,33.332034495862,-46.3475541666667));
#257742=CARTESIAN_POINT('Ctrl Pts',(-46.5766932247455,32.7348404766724,
-46.2892208333334));
#257743=CARTESIAN_POINT('Ctrl Pts',(-46.5766932247455,31.5404524382932,
-46.2308875));
#257744=CARTESIAN_POINT('Ctrl Pts',(-46.5766932247455,30.3460643999139,
-46.1725541666667));
#257745=CARTESIAN_POINT('Ctrl Pts',(-45.5423228415329,29.7488703807243,
-46.1142208333334));
#257746=CARTESIAN_POINT('Ctrl Pts',(-44.5079524583202,29.1516763615346,
-46.0558875));
#257747=CARTESIAN_POINT('Ctrl Pts',(-43.4735820751074,29.7488703807243,
-45.9975541666667));
#257748=CARTESIAN_POINT('Ctrl Pts',(-42.4392116918948,30.3460643999138,
-45.9392208333333));
#257749=CARTESIAN_POINT('Ctrl Pts',(-42.4392116918948,31.5404524382931,
-45.8808875));
#257750=CARTESIAN_POINT('Ctrl Pts',(-42.4392116918948,32.7348404766723,
-45.8225541666667));
#257751=CARTESIAN_POINT('Ctrl Pts',(-43.4735820751074,33.332034495862,-45.7642208333334));
#257752=CARTESIAN_POINT('Ctrl Pts',(-44.5079524583201,33.9292285150516,
-45.7058875));
#257753=CARTESIAN_POINT('Ctrl Pts',(-45.5423228415328,33.332034495862,-45.6475541666667));
#257754=CARTESIAN_POINT('Ctrl Pts',(-46.5766932247455,32.7348404766724,
-45.5892208333333));
#257755=CARTESIAN_POINT('Ctrl Pts',(-46.5766932247455,31.5404524382932,
-45.5308875));
#257756=CARTESIAN_POINT('Ctrl Pts',(-46.5766932247455,30.3460643999139,
-45.4725541666667));
#257757=CARTESIAN_POINT('Ctrl Pts',(-45.5423228415329,29.7488703807243,
-45.4142208333334));
#257758=CARTESIAN_POINT('Ctrl Pts',(-44.5079524583202,29.1516763615346,
-45.3558875));
#257759=CARTESIAN_POINT('Ctrl Pts',(-43.4735820751074,29.7488703807243,
-45.2975541666667));
#257760=CARTESIAN_POINT('Ctrl Pts',(-42.4392116918948,30.3460643999138,
-45.2392208333333));
#257761=CARTESIAN_POINT('Ctrl Pts',(-42.4392116918948,31.5404524382931,
-45.1808875));
#257762=CARTESIAN_POINT('Ctrl Pts',(-42.4392116918948,32.7348404766723,
-45.1225541666667));
#257763=CARTESIAN_POINT('Ctrl Pts',(-43.4735820751074,33.332034495862,-45.0642208333334));
#257764=CARTESIAN_POINT('Ctrl Pts',(-44.5079524583201,33.9292285150516,
-45.0058875));
#257765=CARTESIAN_POINT('Ctrl Pts',(-45.5423228415328,33.332034495862,-44.9475541666667));
#257766=CARTESIAN_POINT('Ctrl Pts',(-46.5766932247455,32.7348404766724,
-44.8892208333333));
#257767=CARTESIAN_POINT('Ctrl Pts',(-46.5766932247455,31.5404524382932,
-44.8308875));
#257768=CARTESIAN_POINT('Ctrl Pts',(-46.5766932247455,30.3460643999139,
-44.7725541666666));
#257769=CARTESIAN_POINT('Ctrl Pts',(-45.5423228415329,29.7488703807243,
-44.7142208333334));
#257770=CARTESIAN_POINT('Ctrl Pts',(-44.5079524583202,29.1516763615346,
-44.6558875));
#257771=CARTESIAN_POINT('Ctrl Pts',(-43.4735820751074,29.7488703807243,
-44.5975541666667));
#257772=CARTESIAN_POINT('Ctrl Pts',(-42.4392116918948,30.3460643999138,
-44.5392208333333));
#257773=CARTESIAN_POINT('Ctrl Pts',(-42.4392116918948,31.5404524382931,
-44.4808875));
#257774=CARTESIAN_POINT('Ctrl Pts',(-42.4392116918948,32.7348404766723,
-44.4225541666667));
#257775=CARTESIAN_POINT('Ctrl Pts',(-43.4735820751074,33.332034495862,-44.3642208333333));
#257776=CARTESIAN_POINT('Ctrl Pts',(-44.5079524583201,33.9292285150516,
-44.3058875));
#257777=CARTESIAN_POINT('Ctrl Pts',(-45.5423228415328,33.332034495862,-44.2475541666667));
#257778=CARTESIAN_POINT('Ctrl Pts',(-46.5766932247455,32.7348404766724,
-44.1892208333334));
#257779=CARTESIAN_POINT('Ctrl Pts',(-46.5766932247455,31.5404524382932,
-44.1308875));
#257780=CARTESIAN_POINT('Ctrl Pts',(-46.5766932247455,30.3460643999139,
-44.0725541666667));
#257781=CARTESIAN_POINT('Ctrl Pts',(-45.5423228415329,29.7488703807243,
-44.0142208333334));
#257782=CARTESIAN_POINT('Ctrl Pts',(-44.5079524583202,29.1516763615346,
-43.9558875));
#257783=CARTESIAN_POINT('Ctrl Pts',(-43.4735820751074,29.7488703807243,
-43.8975541666667));
#257784=CARTESIAN_POINT('Ctrl Pts',(-42.4392116918948,30.3460643999138,
-43.8392208333333));
#257785=CARTESIAN_POINT('Ctrl Pts',(-42.4392116918948,31.5404524382931,
-43.7808875));
#257786=CARTESIAN_POINT('Ctrl Pts',(-42.4392116918948,32.7348404766723,
-43.7225541666667));
#257787=CARTESIAN_POINT('Ctrl Pts',(-43.4735820751074,33.332034495862,-43.6642208333334));
#257788=CARTESIAN_POINT('Ctrl Pts',(-44.5079524583201,33.9292285150516,
-43.6058875));
#257789=CARTESIAN_POINT('Ctrl Pts',(-45.5423228415328,33.332034495862,-43.5475541666667));
#257790=CARTESIAN_POINT('Ctrl Pts',(-46.5766932247455,32.7348404766724,
-43.4892208333333));
#257791=CARTESIAN_POINT('Ctrl Pts',(-46.5766932247455,31.5404524382932,
-43.4308875));
#257792=CARTESIAN_POINT('Ctrl Pts',(-46.5766932247455,30.3460643999139,
-43.3725541666667));
#257793=CARTESIAN_POINT('Ctrl Pts',(-45.5423228415329,29.7488703807243,
-43.3142208333334));
#257794=CARTESIAN_POINT('Ctrl Pts',(-44.5079524583202,29.1516763615346,
-43.2558875));
#257795=CARTESIAN_POINT('Ctrl Pts',(-43.4735820751074,29.7488703807243,
-43.1975541666667));
#257796=CARTESIAN_POINT('Ctrl Pts',(-42.4392116918948,30.3460643999138,
-43.1392208333334));
#257797=CARTESIAN_POINT('Ctrl Pts',(-42.4392116918948,31.5404524382931,
-43.0808875));
#257798=CARTESIAN_POINT('Ctrl Pts',(-42.4392116918948,32.7348404766723,
-43.0225541666667));
#257799=CARTESIAN_POINT('Ctrl Pts',(-43.4735820751074,33.332034495862,-42.9642208333334));
#257800=CARTESIAN_POINT('Ctrl Pts',(-44.5079524583201,33.9292285150516,
-42.9058875));
#257801=CARTESIAN_POINT('Ctrl Pts',(-45.5423228415328,33.332034495862,-42.8475541666667));
#257802=CARTESIAN_POINT('Ctrl Pts',(-46.5766932247455,32.7348404766724,
-42.7892208333334));
#257803=CARTESIAN_POINT('Ctrl Pts',(-46.5766932247455,31.5404524382932,
-42.7308875));
#257804=CARTESIAN_POINT('Ctrl Pts',(-46.5766932247455,30.3460643999139,
-42.6725541666667));
#257805=CARTESIAN_POINT('Ctrl Pts',(-45.5423228415329,29.7488703807243,
-42.6142208333334));
#257806=CARTESIAN_POINT('Ctrl Pts',(-44.5079524583202,29.1516763615346,
-42.5558875));
#257807=CARTESIAN_POINT('Ctrl Pts',(-43.4735820751074,29.7488703807243,
-42.4975541666667));
#257808=CARTESIAN_POINT('Ctrl Pts',(-42.4392116918948,30.3460643999138,
-42.4392208333334));
#257809=CARTESIAN_POINT('Ctrl Pts',(-42.4392116918948,31.5404524382931,
-42.3808875));
#257810=CARTESIAN_POINT('Ctrl Pts',(-42.4392116918948,32.7348404766723,
-42.3225541666667));
#257811=CARTESIAN_POINT('Ctrl Pts',(-43.4735820751074,33.332034495862,-42.2642208333334));
#257812=CARTESIAN_POINT('Ctrl Pts',(-44.5079524583201,33.9292285150516,
-42.2058875));
#257813=CARTESIAN_POINT('Ctrl Pts',(-45.5423228415328,33.332034495862,-42.1475541666667));
#257814=CARTESIAN_POINT('Ctrl Pts',(-46.5766932247455,32.7348404766724,
-42.0892208333333));
#257815=CARTESIAN_POINT('Ctrl Pts',(-46.5766932247455,31.5404524382932,
-42.0308875));
#257816=CARTESIAN_POINT('Ctrl Pts',(-46.5766932247455,30.3460643999139,
-41.9725541666667));
#257817=CARTESIAN_POINT('Ctrl Pts',(-45.5423228415329,29.7488703807243,
-41.9142208333334));
#257818=CARTESIAN_POINT('Ctrl Pts',(-44.5079524583202,29.1516763615346,
-41.8558875));
#257819=CARTESIAN_POINT('Ctrl Pts',(-43.4735820751074,29.7488703807243,
-41.7975541666667));
#257820=CARTESIAN_POINT('Ctrl Pts',(-42.4392116918948,30.3460643999138,
-41.7392208333333));
#257821=CARTESIAN_POINT('Ctrl Pts',(-42.4392116918948,31.5404524382931,
-41.6808875));
#257822=CARTESIAN_POINT('Ctrl Pts',(-42.4392116918948,32.7348404766723,
-41.6225541666667));
#257823=CARTESIAN_POINT('Ctrl Pts',(-43.4735820751074,33.332034495862,-41.5642208333334));
#257824=CARTESIAN_POINT('Ctrl Pts',(-44.5079524583201,33.9292285150516,
-41.5058875));
#257825=CARTESIAN_POINT('Ctrl Pts',(-45.5423228415328,33.332034495862,-41.4475541666667));
#257826=CARTESIAN_POINT('Ctrl Pts',(-46.5766932247455,32.7348404766724,
-41.3892208333333));
#257827=CARTESIAN_POINT('Ctrl Pts',(-46.5766932247455,31.5404524382932,
-41.3308875));
#257828=CARTESIAN_POINT('Ctrl Pts',(-46.5766932247455,30.3460643999139,
-41.2725541666667));
#257829=CARTESIAN_POINT('Ctrl Pts',(-45.5423228415329,29.7488703807243,
-41.2142208333333));
#257830=CARTESIAN_POINT('Ctrl Pts',(-44.5079524583202,29.1516763615346,
-41.1558875));
#257831=CARTESIAN_POINT('Ctrl Pts',(-43.4735820751074,29.7488703807243,
-41.0975541666667));
#257832=CARTESIAN_POINT('Ctrl Pts',(-42.4392116918948,30.3460643999138,
-41.0392208333333));
#257833=CARTESIAN_POINT('Ctrl Pts',(-42.4392116918948,31.5404524382931,
-40.9808875));
#257834=CARTESIAN_POINT('Ctrl Pts',(-42.4392116918948,32.7348404766723,
-40.9225541666667));
#257835=CARTESIAN_POINT('Ctrl Pts',(-43.4735820751074,33.332034495862,-40.8642208333334));
#257836=CARTESIAN_POINT('Ctrl Pts',(-44.5079524583201,33.9292285150516,
-40.8058875));
#257837=CARTESIAN_POINT('Ctrl Pts',(-45.5423228415328,33.332034495862,-40.7475541666667));
#257838=CARTESIAN_POINT('Ctrl Pts',(-46.5766932247455,32.7348404766724,
-40.6892208333333));
#257839=CARTESIAN_POINT('Ctrl Pts',(-46.5766932247455,31.5404524382932,
-40.6308875));
#257840=CARTESIAN_POINT('Ctrl Pts',(-46.5766932247455,30.3460643999139,
-40.5725541666667));
#257841=CARTESIAN_POINT('Ctrl Pts',(-45.5423228415329,29.7488703807243,
-40.5142208333333));
#257842=CARTESIAN_POINT('Ctrl Pts',(-44.5079524583202,29.1516763615346,
-40.4558875));
#257843=CARTESIAN_POINT('Ctrl Pts',(-43.4735820751074,29.7488703807243,
-40.3975541666667));
#257844=CARTESIAN_POINT('Ctrl Pts',(-42.4392116918948,30.3460643999138,
-40.3392208333333));
#257845=CARTESIAN_POINT('Ctrl Pts',(-42.4392116918948,31.5404524382931,
-40.2808875));
#257846=CARTESIAN_POINT('Ctrl Pts',(-42.4392116918948,32.7348404766723,
-40.2225541666667));
#257847=CARTESIAN_POINT('Ctrl Pts',(-43.4735820751074,33.332034495862,-40.1642208333333));
#257848=CARTESIAN_POINT('Ctrl Pts',(-44.5079524583201,33.9292285150516,
-40.1058875));
#257849=CARTESIAN_POINT('Ctrl Pts',(-45.5423228415328,33.332034495862,-40.0475541666667));
#257850=CARTESIAN_POINT('Ctrl Pts',(-46.5766932247455,32.7348404766724,
-39.9892208333333));
#257851=CARTESIAN_POINT('Ctrl Pts',(-46.5766932247455,31.5404524382932,
-39.9308875));
#257852=CARTESIAN_POINT('Ctrl Pts',(-46.5766932247455,30.3460643999139,
-39.8725541666667));
#257853=CARTESIAN_POINT('Ctrl Pts',(-45.5423228415329,29.7488703807243,
-39.8142208333334));
#257854=CARTESIAN_POINT('Ctrl Pts',(-44.5079524583202,29.1516763615346,
-39.7558875));
#257855=CARTESIAN_POINT('Ctrl Pts',(-43.4735820751074,29.7488703807243,
-39.6975541666667));
#257856=CARTESIAN_POINT('Ctrl Pts',(-42.4392116918948,30.3460643999138,
-39.6392208333334));
#257857=CARTESIAN_POINT('Ctrl Pts',(-42.4392116918948,31.5404524382931,
-39.5808875));
#257858=CARTESIAN_POINT('Ctrl Pts',(-42.4392116918948,32.7348404766723,
-39.5225541666667));
#257859=CARTESIAN_POINT('Ctrl Pts',(-43.4735820751074,33.332034495862,-39.4642208333333));
#257860=CARTESIAN_POINT('Ctrl Pts',(-44.5079524583201,33.9292285150516,
-39.4058875));
#257861=CARTESIAN_POINT('Ctrl Pts',(-45.5423228415328,33.332034495862,-39.3475541666667));
#257862=CARTESIAN_POINT('Ctrl Pts',(-46.5766932247455,32.7348404766724,
-39.2892208333334));
#257863=CARTESIAN_POINT('Ctrl Pts',(-46.5766932247455,31.5404524382932,
-39.2308875));
#257864=CARTESIAN_POINT('Ctrl Pts',(-46.5766932247455,30.3460643999139,
-39.1725541666667));
#257865=CARTESIAN_POINT('Ctrl Pts',(-45.5423228415329,29.7488703807243,
-39.1142208333333));
#257866=CARTESIAN_POINT('Ctrl Pts',(-44.5079524583202,29.1516763615346,
-39.0558875));
#257867=CARTESIAN_POINT('Ctrl Pts',(-43.4735820751074,29.7488703807243,
-38.9975541666667));
#257868=CARTESIAN_POINT('Ctrl Pts',(-42.4392116918948,30.3460643999138,
-38.9392208333334));
#257869=CARTESIAN_POINT('Ctrl Pts',(-42.4392116918948,31.5404524382931,
-38.8808875));
#257870=CARTESIAN_POINT('Ctrl Pts',(-42.4392116918948,32.7348404766723,
-38.8225541666667));
#257871=CARTESIAN_POINT('Ctrl Pts',(-43.4735820751074,33.332034495862,-38.7642208333333));
#257872=CARTESIAN_POINT('Ctrl Pts',(-44.5079524583201,33.9292285150516,
-38.7058875));
#257873=CARTESIAN_POINT('Ctrl Pts',(-45.5423228415328,33.332034495862,-38.6475541666667));
#257874=CARTESIAN_POINT('Ctrl Pts',(-46.5766932247455,32.7348404766724,
-38.5892208333334));
#257875=CARTESIAN_POINT('Ctrl Pts',(-46.5766932247455,31.5404524382932,
-38.5308875));
#257876=CARTESIAN_POINT('Ctrl Pts',(-46.5766932247455,30.3460643999139,
-38.4725541666667));
#257877=CARTESIAN_POINT('Ctrl Pts',(-45.5423228415329,29.7488703807243,
-38.4142208333334));
#257878=CARTESIAN_POINT('Ctrl Pts',(-44.5079524583202,29.1516763615346,
-38.3558875));
#257879=CARTESIAN_POINT('Ctrl Pts',(-43.4735820751074,29.7488703807243,
-38.2975541666667));
#257880=CARTESIAN_POINT('Ctrl Pts',(-42.4392116918948,30.3460643999138,
-38.2392208333333));
#257881=CARTESIAN_POINT('Ctrl Pts',(-42.4392116918948,31.5404524382931,
-38.1808875));
#257882=CARTESIAN_POINT('Ctrl Pts',(-42.4392116918948,32.7348404766723,
-38.1225541666667));
#257883=CARTESIAN_POINT('Ctrl Pts',(-43.4735820751074,33.332034495862,-38.0642208333334));
#257884=CARTESIAN_POINT('Ctrl Pts',(-44.5079524583201,33.9292285150516,
-38.0058875));
#257885=CARTESIAN_POINT('Ctrl Pts',(-45.5423228415328,33.332034495862,-37.9475541666667));
#257886=CARTESIAN_POINT('Ctrl Pts',(-46.5766932247455,32.7348404766724,
-37.8892208333334));
#257887=CARTESIAN_POINT('Ctrl Pts',(-46.5766932247455,31.5404524382932,
-37.8308875));
#257888=CARTESIAN_POINT('Ctrl Pts',(-46.5766932247455,30.3460643999139,
-37.7725541666667));
#257889=CARTESIAN_POINT('Ctrl Pts',(-45.5423228415329,29.7488703807243,
-37.7142208333333));
#257890=CARTESIAN_POINT('Ctrl Pts',(-44.5079524583202,29.1516763615346,
-37.6558875));
#257891=CARTESIAN_POINT('Ctrl Pts',(-43.4735820751074,29.7488703807243,
-37.5975541666667));
#257892=CARTESIAN_POINT('Ctrl Pts',(-42.4392116918948,30.3460643999138,
-37.5392208333334));
#257893=CARTESIAN_POINT('Ctrl Pts',(-42.4392116918948,31.5404524382931,
-37.4808875));
#257894=CARTESIAN_POINT('Ctrl Pts',(-42.4392116918948,32.7348404766723,
-37.4225541666667));
#257895=CARTESIAN_POINT('Ctrl Pts',(-43.4735820751074,33.332034495862,-37.3642208333333));
#257896=CARTESIAN_POINT('Ctrl Pts',(-44.5079524583201,33.9292285150516,
-37.3058875));
#257897=CARTESIAN_POINT('Ctrl Pts',(-45.5423228415328,33.332034495862,-37.2475541666667));
#257898=CARTESIAN_POINT('Ctrl Pts',(-45.6766168155003,33.2544998338414,
-37.239980655983));
#257899=CARTESIAN_POINT('Ctrl Pts',(-45.7978513037523,33.1578111886089,
-37.2318399189827));
#257900=CARTESIAN_POINT('Ctrl Pts',(-46.5057015041446,31.6353141793171,
-39.8960578923557));
#257901=CARTESIAN_POINT('Ctrl Pts',(-46.5119689182291,31.50332502993,-39.889207245322));
#257902=CARTESIAN_POINT('Ctrl Pts',(-46.5051456084936,31.3710593016932,
-39.8825607059083));
#257903=CARTESIAN_POINT('Ctrl Pts',(-46.4647767050806,31.1050578555559,
-39.8679453789873));
#257904=CARTESIAN_POINT('Ctrl Pts',(-46.4304101376052,30.9722276023654,
-39.8602326823062));
#257905=CARTESIAN_POINT('Ctrl Pts',(-46.2910712917496,30.5971572052441,
-39.8372207705955));
#257906=CARTESIAN_POINT('Ctrl Pts',(-46.1515432444974,30.3708657627987,
-39.8217193778446));
#257907=CARTESIAN_POINT('Ctrl Pts',(-45.7937945447006,29.986360537189,-39.7918605486601));
#257908=CARTESIAN_POINT('Ctrl Pts',(-45.5795141212975,29.83155817775,-39.7787077636743));
#257909=CARTESIAN_POINT('Ctrl Pts',(-45.1083142701796,29.6155194738802,
-39.7512211056924));
#257910=CARTESIAN_POINT('Ctrl Pts',(-44.8567670881079,29.5544784081473,
-39.7365475200715));
#257911=CARTESIAN_POINT('Ctrl Pts',(-44.5697046391987,29.5411668093911,
-39.7198022105518));
#257912=CARTESIAN_POINT('Ctrl Pts',(-44.5388151356,29.5404524382925,-39.7180003228417));
#257913=CARTESIAN_POINT('Ctrl Pts',(-44.5079524583208,29.5404524382925,
-39.7162000000005));
#257914=CARTESIAN_POINT('',(-46.2580162608798,30.7712606105792,-39.7946023861626));
#257915=CARTESIAN_POINT('Ctrl Pts',(-46.2580162608798,30.7712606105792,
-39.7946023861626));
#257916=CARTESIAN_POINT('Ctrl Pts',(-46.3359857239729,30.9069849161725,
-39.8137239675819));
#257917=CARTESIAN_POINT('Ctrl Pts',(-46.396731144117,31.0517787814577,-39.8323019201559));
#257918=CARTESIAN_POINT('Ctrl Pts',(-46.4779237668435,31.3431553140667,
-39.8662996885231));
#257919=CARTESIAN_POINT('Ctrl Pts',(-46.5007939700139,31.4890814765333,
-39.8816624604009));
#257920=CARTESIAN_POINT('Ctrl Pts',(-46.5057020315789,31.6353141675789,
-39.896058194301));
#257921=CARTESIAN_POINT('Ctrl Pts',(-42.7562642394046,32.2382933072411,
-39.4336017780242));
#257922=CARTESIAN_POINT('Ctrl Pts',(-42.7061752771237,32.0303939840906,
-39.4290050783144));
#257923=CARTESIAN_POINT('Ctrl Pts',(-42.6879554887345,31.8161871839669,
-39.4265147261078));
#257924=CARTESIAN_POINT('Ctrl Pts',(-42.722826451042,31.3151915282915,-39.4248348087752));
#257925=CARTESIAN_POINT('Ctrl Pts',(-42.7978352817771,31.0971672163081,
-39.4293776397756));
#257926=CARTESIAN_POINT('Ctrl Pts',(-42.9440228306321,30.7609930563022,
-39.4392856099245));
#257927=CARTESIAN_POINT('Ctrl Pts',(-43.0567852873963,30.5852973811317,
-39.4475010921534));
#257928=CARTESIAN_POINT('Ctrl Pts',(-43.2774600503745,30.3411850111334,
-39.4631783255256));
#257929=CARTESIAN_POINT('Ctrl Pts',(-43.3671859662176,30.2593637739806,
-39.4694819317037));
#257930=CARTESIAN_POINT('Ctrl Pts',(-43.4669086721409,30.1846213999269,
-39.4763662142424));
#257931=CARTESIAN_POINT('Ctrl Pts',(-43.4696440671836,30.1825827861219,
-39.4765549614359));
#257932=CARTESIAN_POINT('Ctrl Pts',(-43.4751302568142,30.1785171929352,
-39.476933339386));
#257933=CARTESIAN_POINT('Ctrl Pts',(-43.4778810222449,30.1764902718028,
-39.477122967848));
#257934=CARTESIAN_POINT('Ctrl Pts',(-43.486189072521,30.1704031945995,-39.4776954266054));
#257935=CARTESIAN_POINT('Ctrl Pts',(-43.4917628814586,30.1663661255867,
-39.478079121429));
#257936=CARTESIAN_POINT('Ctrl Pts',(-43.6119452918925,30.0803173607471,
-39.486344690909));
#257937=CARTESIAN_POINT('Ctrl Pts',(-43.7365211293469,30.0105461443142,
-39.4945972457688));
#257938=CARTESIAN_POINT('Ctrl Pts',(-44.1000414214535,29.8596150599266,
-39.5217363802476));
#257939=CARTESIAN_POINT('Ctrl Pts',(-44.348728581181,29.8115394459938,-39.5427431282814));
#257940=CARTESIAN_POINT('Ctrl Pts',(-44.8440271149477,29.8137267466852,
-39.5899036033774));
#257941=CARTESIAN_POINT('Ctrl Pts',(-45.0860786710093,29.861506312415,-39.6155008436718));
#257942=CARTESIAN_POINT('Ctrl Pts',(-45.5020085767912,30.0282049213117,
-39.6643839318259));
#257943=CARTESIAN_POINT('Ctrl Pts',(-45.6748667889198,30.1313751697612,
-39.6873672741751));
#257944=CARTESIAN_POINT('Ctrl Pts',(-46.0013454707669,30.4043598575736,
-39.7391811305329));
#257945=CARTESIAN_POINT('Ctrl Pts',(-46.1464934812618,30.5771288156309,
-39.767252038655));
#257946=CARTESIAN_POINT('Ctrl Pts',(-46.2580162608798,30.7712606105792,
-39.7946023861626));
#257947=CARTESIAN_POINT('Ctrl Pts',(-46.1766977413726,31.5404524382932,
-52.99995));
#257948=CARTESIAN_POINT('Ctrl Pts',(-46.1766977413726,30.5770018999139,
-52.9416166666667));
#257949=CARTESIAN_POINT('Ctrl Pts',(-45.3423250998464,30.0952766307242,
-52.8832833333334));
#257950=CARTESIAN_POINT('Ctrl Pts',(-44.5079524583202,29.6135513615346,
-52.82495));
#257951=CARTESIAN_POINT('Ctrl Pts',(-43.6735798167939,30.0952766307242,
-52.7666166666667));
#257952=CARTESIAN_POINT('Ctrl Pts',(-42.8392071752677,30.5770018999139,
-52.7082833333333));
#257953=CARTESIAN_POINT('Ctrl Pts',(-42.8392071752677,31.5404524382931,
-52.64995));
#257954=CARTESIAN_POINT('Ctrl Pts',(-42.8392071752677,32.5039029766724,
-52.5916166666666));
#257955=CARTESIAN_POINT('Ctrl Pts',(-43.6735798167939,32.985628245862,-52.5332833333334));
#257956=CARTESIAN_POINT('Ctrl Pts',(-44.5079524583201,33.4673535150516,
-52.4749500000001));
#257957=CARTESIAN_POINT('Ctrl Pts',(-45.3423250998464,32.985628245862,-52.4166166666667));
#257958=CARTESIAN_POINT('Ctrl Pts',(-46.1766977413726,32.5039029766724,
-52.3582833333334));
#257959=CARTESIAN_POINT('Ctrl Pts',(-46.1766977413726,31.5404524382932,
-52.29995));
#257960=CARTESIAN_POINT('Ctrl Pts',(-46.1766977413726,30.5770018999139,
-52.2416166666667));
#257961=CARTESIAN_POINT('Ctrl Pts',(-45.3423250998464,30.0952766307242,
-52.1832833333333));
#257962=CARTESIAN_POINT('Ctrl Pts',(-44.5079524583202,29.6135513615346,
-52.12495));
#257963=CARTESIAN_POINT('Ctrl Pts',(-43.6735798167939,30.0952766307242,
-52.0666166666667));
#257964=CARTESIAN_POINT('Ctrl Pts',(-42.8392071752677,30.5770018999139,
-52.0082833333333));
#257965=CARTESIAN_POINT('Ctrl Pts',(-42.8392071752677,31.5404524382931,
-51.94995));
#257966=CARTESIAN_POINT('Ctrl Pts',(-42.8392071752677,32.5039029766724,
-51.8916166666667));
#257967=CARTESIAN_POINT('Ctrl Pts',(-43.6735798167939,32.985628245862,-51.8332833333333));
#257968=CARTESIAN_POINT('Ctrl Pts',(-44.5079524583201,33.4673535150516,
-51.77495));
#257969=CARTESIAN_POINT('Ctrl Pts',(-45.3423250998464,32.985628245862,-51.7166166666667));
#257970=CARTESIAN_POINT('Ctrl Pts',(-46.1766977413726,32.5039029766724,
-51.6582833333333));
#257971=CARTESIAN_POINT('Ctrl Pts',(-46.1766977413726,31.5404524382932,
-51.59995));
#257972=CARTESIAN_POINT('Ctrl Pts',(-46.1766977413726,30.5770018999139,
-51.5416166666667));
#257973=CARTESIAN_POINT('Ctrl Pts',(-45.3423250998464,30.0952766307242,
-51.4832833333333));
#257974=CARTESIAN_POINT('Ctrl Pts',(-44.5079524583202,29.6135513615346,
-51.42495));
#257975=CARTESIAN_POINT('Ctrl Pts',(-43.6735798167939,30.0952766307242,
-51.3666166666667));
#257976=CARTESIAN_POINT('Ctrl Pts',(-42.8392071752677,30.5770018999139,
-51.3082833333333));
#257977=CARTESIAN_POINT('Ctrl Pts',(-42.8392071752677,31.5404524382931,
-51.24995));
#257978=CARTESIAN_POINT('Ctrl Pts',(-42.8392071752677,32.5039029766724,
-51.1916166666666));
#257979=CARTESIAN_POINT('Ctrl Pts',(-43.6735798167939,32.985628245862,-51.1332833333333));
#257980=CARTESIAN_POINT('Ctrl Pts',(-44.5079524583201,33.4673535150516,
-51.07495));
#257981=CARTESIAN_POINT('Ctrl Pts',(-45.3423250998464,32.985628245862,-51.0166166666667));
#257982=CARTESIAN_POINT('Ctrl Pts',(-46.1766977413726,32.5039029766724,
-50.9582833333334));
#257983=CARTESIAN_POINT('Ctrl Pts',(-46.1766977413726,31.5404524382932,
-50.89995));
#257984=CARTESIAN_POINT('Ctrl Pts',(-46.1766977413726,30.5770018999139,
-50.8416166666667));
#257985=CARTESIAN_POINT('Ctrl Pts',(-45.3423250998464,30.0952766307242,
-50.7832833333333));
#257986=CARTESIAN_POINT('Ctrl Pts',(-44.5079524583202,29.6135513615346,
-50.72495));
#257987=CARTESIAN_POINT('Ctrl Pts',(-43.6735798167939,30.0952766307242,
-50.6666166666667));
#257988=CARTESIAN_POINT('Ctrl Pts',(-42.8392071752677,30.5770018999139,
-50.6082833333334));
#257989=CARTESIAN_POINT('Ctrl Pts',(-42.8392071752677,31.5404524382931,
-50.54995));
#257990=CARTESIAN_POINT('Ctrl Pts',(-42.8392071752677,32.5039029766724,
-50.4916166666667));
#257991=CARTESIAN_POINT('Ctrl Pts',(-43.6735798167939,32.985628245862,-50.4332833333333));
#257992=CARTESIAN_POINT('Ctrl Pts',(-44.5079524583201,33.4673535150516,
-50.37495));
#257993=CARTESIAN_POINT('Ctrl Pts',(-45.3423250998464,32.985628245862,-50.3166166666667));
#257994=CARTESIAN_POINT('Ctrl Pts',(-46.1766977413726,32.5039029766724,
-50.2582833333334));
#257995=CARTESIAN_POINT('Ctrl Pts',(-46.1766977413726,31.5404524382932,
-50.19995));
#257996=CARTESIAN_POINT('Ctrl Pts',(-46.1766977413726,30.5770018999139,
-50.1416166666667));
#257997=CARTESIAN_POINT('Ctrl Pts',(-45.3423250998464,30.0952766307242,
-50.0832833333333));
#257998=CARTESIAN_POINT('Ctrl Pts',(-44.5079524583202,29.6135513615346,
-50.02495));
#257999=CARTESIAN_POINT('Ctrl Pts',(-43.6735798167939,30.0952766307242,
-49.9666166666667));
#258000=CARTESIAN_POINT('Ctrl Pts',(-42.8392071752677,30.5770018999139,
-49.9082833333334));
#258001=CARTESIAN_POINT('Ctrl Pts',(-42.8392071752677,31.5404524382931,
-49.84995));
#258002=CARTESIAN_POINT('Ctrl Pts',(-42.8392071752677,32.5039029766724,
-49.7916166666667));
#258003=CARTESIAN_POINT('Ctrl Pts',(-43.6735798167939,32.985628245862,-49.7332833333333));
#258004=CARTESIAN_POINT('Ctrl Pts',(-44.5079524583201,33.4673535150516,
-49.67495));
#258005=CARTESIAN_POINT('Ctrl Pts',(-45.3423250998464,32.985628245862,-49.6166166666667));
#258006=CARTESIAN_POINT('Ctrl Pts',(-46.1766977413726,32.5039029766724,
-49.5582833333334));
#258007=CARTESIAN_POINT('Ctrl Pts',(-46.1766977413726,31.5404524382932,
-49.49995));
#258008=CARTESIAN_POINT('Ctrl Pts',(-46.1766977413726,30.5770018999139,
-49.4416166666667));
#258009=CARTESIAN_POINT('Ctrl Pts',(-45.3423250998464,30.0952766307242,
-49.3832833333334));
#258010=CARTESIAN_POINT('Ctrl Pts',(-44.5079524583202,29.6135513615346,
-49.32495));
#258011=CARTESIAN_POINT('Ctrl Pts',(-43.6735798167939,30.0952766307242,
-49.2666166666667));
#258012=CARTESIAN_POINT('Ctrl Pts',(-42.8392071752677,30.5770018999139,
-49.2082833333334));
#258013=CARTESIAN_POINT('Ctrl Pts',(-42.8392071752677,31.5404524382931,
-49.14995));
#258014=CARTESIAN_POINT('Ctrl Pts',(-42.8392071752677,32.5039029766724,
-49.0916166666667));
#258015=CARTESIAN_POINT('Ctrl Pts',(-43.6735798167939,32.985628245862,-49.0332833333333));
#258016=CARTESIAN_POINT('Ctrl Pts',(-44.5079524583201,33.4673535150516,
-48.97495));
#258017=CARTESIAN_POINT('Ctrl Pts',(-45.3423250998464,32.985628245862,-48.9166166666667));
#258018=CARTESIAN_POINT('Ctrl Pts',(-46.1766977413726,32.5039029766724,
-48.8582833333333));
#258019=CARTESIAN_POINT('Ctrl Pts',(-46.1766977413726,31.5404524382932,
-48.79995));
#258020=CARTESIAN_POINT('Ctrl Pts',(-46.1766977413726,30.5770018999139,
-48.7416166666667));
#258021=CARTESIAN_POINT('Ctrl Pts',(-45.3423250998464,30.0952766307242,
-48.6832833333333));
#258022=CARTESIAN_POINT('Ctrl Pts',(-44.5079524583202,29.6135513615346,
-48.62495));
#258023=CARTESIAN_POINT('Ctrl Pts',(-43.6735798167939,30.0952766307242,
-48.5666166666667));
#258024=CARTESIAN_POINT('Ctrl Pts',(-42.8392071752677,30.5770018999139,
-48.5082833333333));
#258025=CARTESIAN_POINT('Ctrl Pts',(-42.8392071752677,31.5404524382931,
-48.44995));
#258026=CARTESIAN_POINT('Ctrl Pts',(-42.8392071752677,32.5039029766724,
-48.3916166666667));
#258027=CARTESIAN_POINT('Ctrl Pts',(-43.6735798167939,32.985628245862,-48.3332833333333));
#258028=CARTESIAN_POINT('Ctrl Pts',(-44.5079524583201,33.4673535150516,
-48.27495));
#258029=CARTESIAN_POINT('Ctrl Pts',(-45.3423250998464,32.985628245862,-48.2166166666667));
#258030=CARTESIAN_POINT('Ctrl Pts',(-46.1766977413726,32.5039029766724,
-48.1582833333333));
#258031=CARTESIAN_POINT('Ctrl Pts',(-46.1766977413726,31.5404524382932,
-48.09995));
#258032=CARTESIAN_POINT('Ctrl Pts',(-46.1766977413726,30.5770018999139,
-48.0416166666667));
#258033=CARTESIAN_POINT('Ctrl Pts',(-45.3423250998464,30.0952766307242,
-47.9832833333334));
#258034=CARTESIAN_POINT('Ctrl Pts',(-44.5079524583202,29.6135513615346,
-47.92495));
#258035=CARTESIAN_POINT('Ctrl Pts',(-43.6735798167939,30.0952766307242,
-47.8666166666667));
#258036=CARTESIAN_POINT('Ctrl Pts',(-42.8392071752677,30.5770018999139,
-47.8082833333333));
#258037=CARTESIAN_POINT('Ctrl Pts',(-42.8392071752677,31.5404524382931,
-47.74995));
#258038=CARTESIAN_POINT('Ctrl Pts',(-42.8392071752677,32.5039029766724,
-47.6916166666667));
#258039=CARTESIAN_POINT('Ctrl Pts',(-43.6735798167939,32.985628245862,-47.6332833333333));
#258040=CARTESIAN_POINT('Ctrl Pts',(-44.5079524583201,33.4673535150516,
-47.57495));
#258041=CARTESIAN_POINT('Ctrl Pts',(-45.3423250998464,32.985628245862,-47.5166166666667));
#258042=CARTESIAN_POINT('Ctrl Pts',(-46.1766977413726,32.5039029766724,
-47.4582833333333));
#258043=CARTESIAN_POINT('Ctrl Pts',(-46.1766977413726,31.5404524382932,
-47.39995));
#258044=CARTESIAN_POINT('Ctrl Pts',(-46.1766977413726,30.5770018999139,
-47.3416166666666));
#258045=CARTESIAN_POINT('Ctrl Pts',(-45.3423250998464,30.0952766307242,
-47.2832833333333));
#258046=CARTESIAN_POINT('Ctrl Pts',(-44.5079524583202,29.6135513615346,
-47.22495));
#258047=CARTESIAN_POINT('Ctrl Pts',(-43.6735798167939,30.0952766307242,
-47.1666166666667));
#258048=CARTESIAN_POINT('Ctrl Pts',(-42.8392071752677,30.5770018999139,
-47.1082833333333));
#258049=CARTESIAN_POINT('Ctrl Pts',(-42.8392071752677,31.5404524382931,
-47.04995));
#258050=CARTESIAN_POINT('Ctrl Pts',(-42.8392071752677,32.5039029766724,
-46.9916166666667));
#258051=CARTESIAN_POINT('Ctrl Pts',(-43.6735798167939,32.985628245862,-46.9332833333333));
#258052=CARTESIAN_POINT('Ctrl Pts',(-44.5079524583201,33.4673535150516,
-46.87495));
#258053=CARTESIAN_POINT('Ctrl Pts',(-45.3423250998464,32.985628245862,-46.8166166666667));
#258054=CARTESIAN_POINT('Ctrl Pts',(-46.1766977413726,32.5039029766724,
-46.7582833333333));
#258055=CARTESIAN_POINT('Ctrl Pts',(-46.1766977413726,31.5404524382932,
-46.69995));
#258056=CARTESIAN_POINT('Ctrl Pts',(-46.1766977413726,30.5770018999139,
-46.6416166666666));
#258057=CARTESIAN_POINT('Ctrl Pts',(-45.3423250998464,30.0952766307242,
-46.5832833333334));
#258058=CARTESIAN_POINT('Ctrl Pts',(-44.5079524583202,29.6135513615346,
-46.52495));
#258059=CARTESIAN_POINT('Ctrl Pts',(-43.6735798167939,30.0952766307242,
-46.4666166666667));
#258060=CARTESIAN_POINT('Ctrl Pts',(-42.8392071752677,30.5770018999139,
-46.4082833333334));
#258061=CARTESIAN_POINT('Ctrl Pts',(-42.8392071752677,31.5404524382931,
-46.34995));
#258062=CARTESIAN_POINT('Ctrl Pts',(-42.8392071752677,32.5039029766724,
-46.2916166666667));
#258063=CARTESIAN_POINT('Ctrl Pts',(-43.6735798167939,32.985628245862,-46.2332833333334));
#258064=CARTESIAN_POINT('Ctrl Pts',(-44.5079524583201,33.4673535150516,
-46.17495));
#258065=CARTESIAN_POINT('Ctrl Pts',(-45.3423250998464,32.985628245862,-46.1166166666667));
#258066=CARTESIAN_POINT('Ctrl Pts',(-46.1766977413726,32.5039029766724,
-46.0582833333333));
#258067=CARTESIAN_POINT('Ctrl Pts',(-46.1766977413726,31.5404524382932,
-45.99995));
#258068=CARTESIAN_POINT('Ctrl Pts',(-46.1766977413726,30.5770018999139,
-45.9416166666667));
#258069=CARTESIAN_POINT('Ctrl Pts',(-45.3423250998464,30.0952766307242,
-45.8832833333333));
#258070=CARTESIAN_POINT('Ctrl Pts',(-44.5079524583202,29.6135513615346,
-45.82495));
#258071=CARTESIAN_POINT('Ctrl Pts',(-43.6735798167939,30.0952766307242,
-45.7666166666667));
#258072=CARTESIAN_POINT('Ctrl Pts',(-42.8392071752677,30.5770018999139,
-45.7082833333333));
#258073=CARTESIAN_POINT('Ctrl Pts',(-42.8392071752677,31.5404524382931,
-45.64995));
#258074=CARTESIAN_POINT('Ctrl Pts',(-42.8392071752677,32.5039029766724,
-45.5916166666667));
#258075=CARTESIAN_POINT('Ctrl Pts',(-43.6735798167939,32.985628245862,-45.5332833333333));
#258076=CARTESIAN_POINT('Ctrl Pts',(-44.5079524583201,33.4673535150516,
-45.47495));
#258077=CARTESIAN_POINT('Ctrl Pts',(-45.3423250998464,32.985628245862,-45.4166166666667));
#258078=CARTESIAN_POINT('Ctrl Pts',(-46.1766977413726,32.5039029766724,
-45.3582833333333));
#258079=CARTESIAN_POINT('Ctrl Pts',(-46.1766977413726,31.5404524382932,
-45.29995));
#258080=CARTESIAN_POINT('Ctrl Pts',(-46.1766977413726,30.5770018999139,
-45.2416166666667));
#258081=CARTESIAN_POINT('Ctrl Pts',(-45.3423250998464,30.0952766307242,
-45.1832833333333));
#258082=CARTESIAN_POINT('Ctrl Pts',(-44.5079524583202,29.6135513615346,
-45.12495));
#258083=CARTESIAN_POINT('Ctrl Pts',(-43.6735798167939,30.0952766307242,
-45.0666166666667));
#258084=CARTESIAN_POINT('Ctrl Pts',(-42.8392071752677,30.5770018999139,
-45.0082833333334));
#258085=CARTESIAN_POINT('Ctrl Pts',(-42.8392071752677,31.5404524382931,
-44.94995));
#258086=CARTESIAN_POINT('Ctrl Pts',(-42.8392071752677,32.5039029766724,
-44.8916166666667));
#258087=CARTESIAN_POINT('Ctrl Pts',(-43.6735798167939,32.985628245862,-44.8332833333334));
#258088=CARTESIAN_POINT('Ctrl Pts',(-44.5079524583201,33.4673535150516,
-44.77495));
#258089=CARTESIAN_POINT('Ctrl Pts',(-45.3423250998464,32.985628245862,-44.7166166666667));
#258090=CARTESIAN_POINT('Ctrl Pts',(-46.1766977413726,32.5039029766724,
-44.6582833333333));
#258091=CARTESIAN_POINT('Ctrl Pts',(-46.1766977413726,31.5404524382932,
-44.59995));
#258092=CARTESIAN_POINT('Ctrl Pts',(-46.1766977413726,30.5770018999139,
-44.5416166666667));
#258093=CARTESIAN_POINT('Ctrl Pts',(-45.3423250998464,30.0952766307242,
-44.4832833333334));
#258094=CARTESIAN_POINT('Ctrl Pts',(-44.5079524583202,29.6135513615346,
-44.42495));
#258095=CARTESIAN_POINT('Ctrl Pts',(-43.6735798167939,30.0952766307242,
-44.3666166666667));
#258096=CARTESIAN_POINT('Ctrl Pts',(-42.8392071752677,30.5770018999139,
-44.3082833333334));
#258097=CARTESIAN_POINT('Ctrl Pts',(-42.8392071752677,31.5404524382931,
-44.24995));
#258098=CARTESIAN_POINT('Ctrl Pts',(-42.8392071752677,32.5039029766724,
-44.1916166666667));
#258099=CARTESIAN_POINT('Ctrl Pts',(-43.6735798167939,32.985628245862,-44.1332833333334));
#258100=CARTESIAN_POINT('Ctrl Pts',(-44.5079524583201,33.4673535150516,
-44.07495));
#258101=CARTESIAN_POINT('Ctrl Pts',(-45.3423250998464,32.985628245862,-44.0166166666667));
#258102=CARTESIAN_POINT('Ctrl Pts',(-46.1766977413726,32.5039029766724,
-43.9582833333334));
#258103=CARTESIAN_POINT('Ctrl Pts',(-46.1766977413726,31.5404524382932,
-43.89995));
#258104=CARTESIAN_POINT('Ctrl Pts',(-46.1766977413726,30.5770018999139,
-43.8416166666667));
#258105=CARTESIAN_POINT('Ctrl Pts',(-45.3423250998464,30.0952766307242,
-43.7832833333334));
#258106=CARTESIAN_POINT('Ctrl Pts',(-44.5079524583202,29.6135513615346,
-43.72495));
#258107=CARTESIAN_POINT('Ctrl Pts',(-43.6735798167939,30.0952766307242,
-43.6666166666667));
#258108=CARTESIAN_POINT('Ctrl Pts',(-42.8392071752677,30.5770018999139,
-43.6082833333333));
#258109=CARTESIAN_POINT('Ctrl Pts',(-42.8392071752677,31.5404524382931,
-43.54995));
#258110=CARTESIAN_POINT('Ctrl Pts',(-42.8392071752677,32.5039029766724,
-43.4916166666667));
#258111=CARTESIAN_POINT('Ctrl Pts',(-43.6735798167939,32.985628245862,-43.4332833333333));
#258112=CARTESIAN_POINT('Ctrl Pts',(-44.5079524583201,33.4673535150516,
-43.37495));
#258113=CARTESIAN_POINT('Ctrl Pts',(-45.3423250998464,32.985628245862,-43.3166166666667));
#258114=CARTESIAN_POINT('Ctrl Pts',(-46.1766977413726,32.5039029766724,
-43.2582833333333));
#258115=CARTESIAN_POINT('Ctrl Pts',(-46.1766977413726,31.5404524382932,
-43.19995));
#258116=CARTESIAN_POINT('Ctrl Pts',(-46.1766977413726,30.5770018999139,
-43.1416166666666));
#258117=CARTESIAN_POINT('Ctrl Pts',(-45.3423250998464,30.0952766307242,
-43.0832833333333));
#258118=CARTESIAN_POINT('Ctrl Pts',(-44.5079524583202,29.6135513615346,
-43.02495));
#258119=CARTESIAN_POINT('Ctrl Pts',(-43.6735798167939,30.0952766307242,
-42.9666166666667));
#258120=CARTESIAN_POINT('Ctrl Pts',(-42.8392071752677,30.5770018999139,
-42.9082833333333));
#258121=CARTESIAN_POINT('Ctrl Pts',(-42.8392071752677,31.5404524382931,
-42.84995));
#258122=CARTESIAN_POINT('Ctrl Pts',(-42.8392071752677,32.5039029766724,
-42.7916166666667));
#258123=CARTESIAN_POINT('Ctrl Pts',(-43.6735798167939,32.985628245862,-42.7332833333334));
#258124=CARTESIAN_POINT('Ctrl Pts',(-44.5079524583201,33.4673535150516,
-42.67495));
#258125=CARTESIAN_POINT('Ctrl Pts',(-45.3423250998464,32.985628245862,-42.6166166666667));
#258126=CARTESIAN_POINT('Ctrl Pts',(-46.1766977413726,32.5039029766724,
-42.5582833333333));
#258127=CARTESIAN_POINT('Ctrl Pts',(-46.1766977413726,31.5404524382932,
-42.49995));
#258128=CARTESIAN_POINT('Ctrl Pts',(-46.1766977413726,30.5770018999139,
-42.4416166666667));
#258129=CARTESIAN_POINT('Ctrl Pts',(-45.3423250998464,30.0952766307242,
-42.3832833333333));
#258130=CARTESIAN_POINT('Ctrl Pts',(-44.5079524583202,29.6135513615346,
-42.32495));
#258131=CARTESIAN_POINT('Ctrl Pts',(-43.6735798167939,30.0952766307242,
-42.2666166666667));
#258132=CARTESIAN_POINT('Ctrl Pts',(-42.8392071752677,30.5770018999139,
-42.2082833333333));
#258133=CARTESIAN_POINT('Ctrl Pts',(-42.8392071752677,31.5404524382931,
-42.14995));
#258134=CARTESIAN_POINT('Ctrl Pts',(-42.8392071752677,32.5039029766724,
-42.0916166666667));
#258135=CARTESIAN_POINT('Ctrl Pts',(-43.6735798167939,32.985628245862,-42.0332833333334));
#258136=CARTESIAN_POINT('Ctrl Pts',(-44.5079524583201,33.4673535150516,
-41.97495));
#258137=CARTESIAN_POINT('Ctrl Pts',(-45.3423250998464,32.985628245862,-41.9166166666666));
#258138=CARTESIAN_POINT('Ctrl Pts',(-46.1766977413726,32.5039029766724,
-41.8582833333333));
#258139=CARTESIAN_POINT('Ctrl Pts',(-46.1766977413726,31.5404524382932,
-41.79995));
#258140=CARTESIAN_POINT('Ctrl Pts',(-46.1766977413726,30.5770018999139,
-41.7416166666667));
#258141=CARTESIAN_POINT('Ctrl Pts',(-45.3423250998464,30.0952766307242,
-41.6832833333333));
#258142=CARTESIAN_POINT('Ctrl Pts',(-44.5079524583202,29.6135513615346,
-41.62495));
#258143=CARTESIAN_POINT('Ctrl Pts',(-43.6735798167939,30.0952766307242,
-41.5666166666667));
#258144=CARTESIAN_POINT('Ctrl Pts',(-42.8392071752677,30.5770018999139,
-41.5082833333334));
#258145=CARTESIAN_POINT('Ctrl Pts',(-42.8392071752677,31.5404524382931,
-41.44995));
#258146=CARTESIAN_POINT('Ctrl Pts',(-42.8392071752677,32.5039029766724,
-41.3916166666667));
#258147=CARTESIAN_POINT('Ctrl Pts',(-43.6735798167939,32.985628245862,-41.3332833333334));
#258148=CARTESIAN_POINT('Ctrl Pts',(-44.5079524583201,33.4673535150516,
-41.27495));
#258149=CARTESIAN_POINT('Ctrl Pts',(-45.3423250998464,32.985628245862,-41.2166166666667));
#258150=CARTESIAN_POINT('Ctrl Pts',(-46.1766977413726,32.5039029766724,
-41.1582833333333));
#258151=CARTESIAN_POINT('Ctrl Pts',(-46.1766977413726,31.5404524382932,
-41.09995));
#258152=CARTESIAN_POINT('Ctrl Pts',(-46.1766977413726,30.5770018999139,
-41.0416166666667));
#258153=CARTESIAN_POINT('Ctrl Pts',(-45.3423250998464,30.0952766307242,
-40.9832833333333));
#258154=CARTESIAN_POINT('Ctrl Pts',(-44.5079524583202,29.6135513615346,
-40.92495));
#258155=CARTESIAN_POINT('Ctrl Pts',(-43.6735798167939,30.0952766307242,
-40.8666166666667));
#258156=CARTESIAN_POINT('Ctrl Pts',(-42.8392071752677,30.5770018999139,
-40.8082833333334));
#258157=CARTESIAN_POINT('Ctrl Pts',(-42.8392071752677,31.5404524382931,
-40.74995));
#258158=CARTESIAN_POINT('Ctrl Pts',(-42.8392071752677,32.5039029766724,
-40.6916166666667));
#258159=CARTESIAN_POINT('Ctrl Pts',(-43.6735798167939,32.985628245862,-40.6332833333334));
#258160=CARTESIAN_POINT('Ctrl Pts',(-44.5079524583201,33.4673535150516,
-40.57495));
#258161=CARTESIAN_POINT('Ctrl Pts',(-45.3423250998464,32.985628245862,-40.5166166666666));
#258162=CARTESIAN_POINT('Ctrl Pts',(-46.1766977413726,32.5039029766724,
-40.4582833333333));
#258163=CARTESIAN_POINT('Ctrl Pts',(-46.1766977413726,31.5404524382932,
-40.39995));
#258164=CARTESIAN_POINT('Ctrl Pts',(-46.1766977413726,30.5770018999139,
-40.3416166666667));
#258165=CARTESIAN_POINT('Ctrl Pts',(-45.3423250998464,30.0952766307242,
-40.2832833333334));
#258166=CARTESIAN_POINT('Ctrl Pts',(-44.5079524583202,29.6135513615346,
-40.22495));
#258167=CARTESIAN_POINT('Ctrl Pts',(-43.6735798167939,30.0952766307242,
-40.1666166666667));
#258168=CARTESIAN_POINT('Ctrl Pts',(-42.8392071752677,30.5770018999139,
-40.1082833333334));
#258169=CARTESIAN_POINT('Ctrl Pts',(-42.8392071752677,31.5404524382931,
-40.04995));
#258170=CARTESIAN_POINT('Ctrl Pts',(-42.8392071752677,32.5039029766724,
-39.9916166666667));
#258171=CARTESIAN_POINT('Ctrl Pts',(-43.6735798167939,32.985628245862,-39.9332833333333));
#258172=CARTESIAN_POINT('Ctrl Pts',(-44.5079524583201,33.4673535150516,
-39.87495));
#258173=CARTESIAN_POINT('Ctrl Pts',(-45.3423250998464,32.985628245862,-39.8166166666667));
#258174=CARTESIAN_POINT('Ctrl Pts',(-46.1766977413726,32.5039029766724,
-39.7582833333334));
#258175=CARTESIAN_POINT('Ctrl Pts',(-46.1766977413726,31.5404524382932,
-39.69995));
#258176=CARTESIAN_POINT('Ctrl Pts',(-46.1766977413726,30.5770018999139,
-39.6416166666667));
#258177=CARTESIAN_POINT('Ctrl Pts',(-45.3423250998464,30.0952766307242,
-39.5832833333333));
#258178=CARTESIAN_POINT('Ctrl Pts',(-44.5079524583202,29.6135513615346,
-39.52495));
#258179=CARTESIAN_POINT('Ctrl Pts',(-43.6735798167939,30.0952766307242,
-39.4666166666667));
#258180=CARTESIAN_POINT('Ctrl Pts',(-42.8392071752677,30.5770018999139,
-39.4082833333333));
#258181=CARTESIAN_POINT('Ctrl Pts',(-42.8392071752677,31.5404524382931,
-39.34995));
#258182=CARTESIAN_POINT('Ctrl Pts',(-42.8392071752677,32.5039029766724,
-39.2916166666667));
#258183=CARTESIAN_POINT('Ctrl Pts',(-43.6735798167939,32.985628245862,-39.2332833333333));
#258184=CARTESIAN_POINT('Ctrl Pts',(-44.5079524583201,33.4673535150516,
-39.17495));
#258185=CARTESIAN_POINT('Ctrl Pts',(-45.3423250998464,32.985628245862,-39.1166166666667));
#258186=CARTESIAN_POINT('Ctrl Pts',(-46.1766977413726,32.5039029766724,
-39.0582833333333));
#258187=CARTESIAN_POINT('Ctrl Pts',(-46.1766977413726,31.5404524382932,
-38.99995));
#258188=CARTESIAN_POINT('Ctrl Pts',(-46.1766977413726,30.5770018999139,
-38.9416166666667));
#258189=CARTESIAN_POINT('Ctrl Pts',(-45.3423250998464,30.0952766307242,
-38.8832833333334));
#258190=CARTESIAN_POINT('Ctrl Pts',(-44.5079524583202,29.6135513615346,
-38.82495));
#258191=CARTESIAN_POINT('Ctrl Pts',(-43.6735798167939,30.0952766307242,
-38.7666166666667));
#258192=CARTESIAN_POINT('Ctrl Pts',(-42.8392071752677,30.5770018999139,
-38.7082833333333));
#258193=CARTESIAN_POINT('Ctrl Pts',(-42.8392071752677,31.5404524382931,
-38.64995));
#258194=CARTESIAN_POINT('Ctrl Pts',(-42.8392071752677,32.5039029766724,
-38.5916166666667));
#258195=CARTESIAN_POINT('Ctrl Pts',(-43.6735798167939,32.985628245862,-38.5332833333334));
#258196=CARTESIAN_POINT('Ctrl Pts',(-44.5079524583201,33.4673535150516,
-38.47495));
#258197=CARTESIAN_POINT('Ctrl Pts',(-45.3423250998464,32.985628245862,-38.4166166666667));
#258198=CARTESIAN_POINT('Ctrl Pts',(-46.1766977413726,32.5039029766724,
-38.3582833333333));
#258199=CARTESIAN_POINT('Ctrl Pts',(-46.1766977413726,31.5404524382932,
-38.29995));
#258200=CARTESIAN_POINT('Ctrl Pts',(-46.1766977413726,30.5770018999139,
-38.2416166666667));
#258201=CARTESIAN_POINT('Ctrl Pts',(-45.3423250998464,30.0952766307242,
-38.1832833333333));
#258202=CARTESIAN_POINT('Ctrl Pts',(-44.5079524583202,29.6135513615346,
-38.12495));
#258203=CARTESIAN_POINT('Ctrl Pts',(-43.6735798167939,30.0952766307242,
-38.0666166666667));
#258204=CARTESIAN_POINT('Ctrl Pts',(-42.8392071752677,30.5770018999139,
-38.0082833333333));
#258205=CARTESIAN_POINT('Ctrl Pts',(-42.8392071752677,31.5404524382931,
-37.94995));
#258206=CARTESIAN_POINT('Ctrl Pts',(-42.8392071752677,32.5039029766724,
-37.8916166666667));
#258207=CARTESIAN_POINT('Ctrl Pts',(-43.6735798167939,32.985628245862,-37.8332833333334));
#258208=CARTESIAN_POINT('Ctrl Pts',(-44.5079524583201,33.4673535150516,
-37.77495));
#258209=CARTESIAN_POINT('Ctrl Pts',(-45.3423250998464,32.985628245862,-37.7166166666667));
#258210=CARTESIAN_POINT('Ctrl Pts',(-46.1766977413726,32.5039029766724,
-37.6582833333333));
#258211=CARTESIAN_POINT('Ctrl Pts',(-46.1766977413726,31.5404524382932,
-37.59995));
#258212=CARTESIAN_POINT('Ctrl Pts',(-46.1766977413726,30.5770018999139,
-37.5416166666667));
#258213=CARTESIAN_POINT('Ctrl Pts',(-45.3423250998464,30.0952766307242,
-37.4832833333334));
#258214=CARTESIAN_POINT('Ctrl Pts',(-44.5079524583202,29.6135513615346,
-37.42495));
#258215=CARTESIAN_POINT('Ctrl Pts',(-43.6735798167939,30.0952766307242,
-37.3666166666667));
#258216=CARTESIAN_POINT('Ctrl Pts',(-42.8392071752677,30.5770018999139,
-37.3082833333333));
#258217=CARTESIAN_POINT('Ctrl Pts',(-42.8392071752677,31.5404524382931,
-37.24995));
#258218=CARTESIAN_POINT('Ctrl Pts',(-42.8392071752677,32.5039029766724,
-37.1916166666667));
#258219=CARTESIAN_POINT('Ctrl Pts',(-43.6735798167939,32.985628245862,-37.1332833333334));
#258220=CARTESIAN_POINT('Ctrl Pts',(-44.5079524583201,33.4673535150516,
-37.07495));
#258221=CARTESIAN_POINT('Ctrl Pts',(-45.3423250998464,32.985628245862,-37.0166166666667));
#258222=CARTESIAN_POINT('Ctrl Pts',(-45.4506530446704,32.9230850777571,
-37.0090431559831));
#258223=CARTESIAN_POINT('Ctrl Pts',(-45.5484465834729,32.8450913903532,
-37.0009024189827));
#258224=CARTESIAN_POINT('Ctrl Pts',(-46.5766932247455,31.5404524382932,
-53.2308875));
#258225=CARTESIAN_POINT('Ctrl Pts',(-46.5766932247455,30.3460643999139,
-53.1725541666667));
#258226=CARTESIAN_POINT('Ctrl Pts',(-45.5423228415329,29.7488703807243,
-53.1142208333334));
#258227=CARTESIAN_POINT('Ctrl Pts',(-44.5079524583202,29.1516763615346,
-53.0558875000001));
#258228=CARTESIAN_POINT('Ctrl Pts',(-43.4735820751074,29.7488703807243,
-52.9975541666667));
#258229=CARTESIAN_POINT('Ctrl Pts',(-42.4392116918948,30.3460643999138,
-52.9392208333334));
#258230=CARTESIAN_POINT('Ctrl Pts',(-42.4392116918948,31.5404524382931,
-52.8808875));
#258231=CARTESIAN_POINT('Ctrl Pts',(-42.4392116918947,32.7348404766723,
-52.8225541666667));
#258232=CARTESIAN_POINT('Ctrl Pts',(-43.4735820751074,33.332034495862,-52.7642208333334));
#258233=CARTESIAN_POINT('Ctrl Pts',(-44.5079524583201,33.9292285150516,
-52.7058875));
#258234=CARTESIAN_POINT('Ctrl Pts',(-45.5423228415328,33.332034495862,-52.6475541666667));
#258235=CARTESIAN_POINT('Ctrl Pts',(-46.5766932247455,32.7348404766724,
-52.5892208333333));
#258236=CARTESIAN_POINT('Ctrl Pts',(-46.5766932247455,31.5404524382932,
-52.5308875));
#258237=CARTESIAN_POINT('Ctrl Pts',(-46.5766932247455,30.3460643999139,
-52.4725541666667));
#258238=CARTESIAN_POINT('Ctrl Pts',(-45.5423228415329,29.7488703807243,
-52.4142208333333));
#258239=CARTESIAN_POINT('Ctrl Pts',(-44.5079524583202,29.1516763615346,
-52.3558875000001));
#258240=CARTESIAN_POINT('Ctrl Pts',(-43.4735820751074,29.7488703807243,
-52.2975541666667));
#258241=CARTESIAN_POINT('Ctrl Pts',(-42.4392116918948,30.3460643999138,
-52.2392208333334));
#258242=CARTESIAN_POINT('Ctrl Pts',(-42.4392116918948,31.5404524382931,
-52.1808875));
#258243=CARTESIAN_POINT('Ctrl Pts',(-42.4392116918947,32.7348404766723,
-52.1225541666667));
#258244=CARTESIAN_POINT('Ctrl Pts',(-43.4735820751074,33.332034495862,-52.0642208333334));
#258245=CARTESIAN_POINT('Ctrl Pts',(-44.5079524583201,33.9292285150516,
-52.0058875));
#258246=CARTESIAN_POINT('Ctrl Pts',(-45.5423228415328,33.332034495862,-51.9475541666667));
#258247=CARTESIAN_POINT('Ctrl Pts',(-46.5766932247455,32.7348404766724,
-51.8892208333334));
#258248=CARTESIAN_POINT('Ctrl Pts',(-46.5766932247455,31.5404524382932,
-51.8308875));
#258249=CARTESIAN_POINT('Ctrl Pts',(-46.5766932247455,30.3460643999139,
-51.7725541666667));
#258250=CARTESIAN_POINT('Ctrl Pts',(-45.5423228415329,29.7488703807243,
-51.7142208333334));
#258251=CARTESIAN_POINT('Ctrl Pts',(-44.5079524583202,29.1516763615346,
-51.6558875));
#258252=CARTESIAN_POINT('Ctrl Pts',(-43.4735820751074,29.7488703807243,
-51.5975541666667));
#258253=CARTESIAN_POINT('Ctrl Pts',(-42.4392116918948,30.3460643999138,
-51.5392208333333));
#258254=CARTESIAN_POINT('Ctrl Pts',(-42.4392116918948,31.5404524382931,
-51.4808875));
#258255=CARTESIAN_POINT('Ctrl Pts',(-42.4392116918947,32.7348404766723,
-51.4225541666667));
#258256=CARTESIAN_POINT('Ctrl Pts',(-43.4735820751074,33.332034495862,-51.3642208333334));
#258257=CARTESIAN_POINT('Ctrl Pts',(-44.5079524583201,33.9292285150516,
-51.3058875));
#258258=CARTESIAN_POINT('Ctrl Pts',(-45.5423228415328,33.332034495862,-51.2475541666667));
#258259=CARTESIAN_POINT('Ctrl Pts',(-46.5766932247455,32.7348404766724,
-51.1892208333333));
#258260=CARTESIAN_POINT('Ctrl Pts',(-46.5766932247455,31.5404524382932,
-51.1308875));
#258261=CARTESIAN_POINT('Ctrl Pts',(-46.5766932247455,30.3460643999139,
-51.0725541666667));
#258262=CARTESIAN_POINT('Ctrl Pts',(-45.5423228415329,29.7488703807243,
-51.0142208333334));
#258263=CARTESIAN_POINT('Ctrl Pts',(-44.5079524583202,29.1516763615346,
-50.9558875));
#258264=CARTESIAN_POINT('Ctrl Pts',(-43.4735820751074,29.7488703807243,
-50.8975541666667));
#258265=CARTESIAN_POINT('Ctrl Pts',(-42.4392116918948,30.3460643999138,
-50.8392208333333));
#258266=CARTESIAN_POINT('Ctrl Pts',(-42.4392116918948,31.5404524382931,
-50.7808875));
#258267=CARTESIAN_POINT('Ctrl Pts',(-42.4392116918947,32.7348404766723,
-50.7225541666666));
#258268=CARTESIAN_POINT('Ctrl Pts',(-43.4735820751074,33.332034495862,-50.6642208333333));
#258269=CARTESIAN_POINT('Ctrl Pts',(-44.5079524583201,33.9292285150516,
-50.6058875));
#258270=CARTESIAN_POINT('Ctrl Pts',(-45.5423228415328,33.332034495862,-50.5475541666667));
#258271=CARTESIAN_POINT('Ctrl Pts',(-46.5766932247455,32.7348404766724,
-50.4892208333333));
#258272=CARTESIAN_POINT('Ctrl Pts',(-46.5766932247455,31.5404524382932,
-50.4308875));
#258273=CARTESIAN_POINT('Ctrl Pts',(-46.5766932247455,30.3460643999139,
-50.3725541666667));
#258274=CARTESIAN_POINT('Ctrl Pts',(-45.5423228415329,29.7488703807243,
-50.3142208333334));
#258275=CARTESIAN_POINT('Ctrl Pts',(-44.5079524583202,29.1516763615346,
-50.2558875));
#258276=CARTESIAN_POINT('Ctrl Pts',(-43.4735820751074,29.7488703807243,
-50.1975541666667));
#258277=CARTESIAN_POINT('Ctrl Pts',(-42.4392116918948,30.3460643999138,
-50.1392208333333));
#258278=CARTESIAN_POINT('Ctrl Pts',(-42.4392116918948,31.5404524382931,
-50.0808875));
#258279=CARTESIAN_POINT('Ctrl Pts',(-42.4392116918947,32.7348404766723,
-50.0225541666667));
#258280=CARTESIAN_POINT('Ctrl Pts',(-43.4735820751074,33.332034495862,-49.9642208333334));
#258281=CARTESIAN_POINT('Ctrl Pts',(-44.5079524583201,33.9292285150516,
-49.9058875));
#258282=CARTESIAN_POINT('Ctrl Pts',(-45.5423228415328,33.332034495862,-49.8475541666667));
#258283=CARTESIAN_POINT('Ctrl Pts',(-46.5766932247455,32.7348404766724,
-49.7892208333333));
#258284=CARTESIAN_POINT('Ctrl Pts',(-46.5766932247455,31.5404524382932,
-49.7308875));
#258285=CARTESIAN_POINT('Ctrl Pts',(-46.5766932247455,30.3460643999139,
-49.6725541666667));
#258286=CARTESIAN_POINT('Ctrl Pts',(-45.5423228415329,29.7488703807243,
-49.6142208333334));
#258287=CARTESIAN_POINT('Ctrl Pts',(-44.5079524583202,29.1516763615346,
-49.5558875));
#258288=CARTESIAN_POINT('Ctrl Pts',(-43.4735820751074,29.7488703807243,
-49.4975541666667));
#258289=CARTESIAN_POINT('Ctrl Pts',(-42.4392116918948,30.3460643999138,
-49.4392208333333));
#258290=CARTESIAN_POINT('Ctrl Pts',(-42.4392116918948,31.5404524382931,
-49.3808875));
#258291=CARTESIAN_POINT('Ctrl Pts',(-42.4392116918947,32.7348404766723,
-49.3225541666667));
#258292=CARTESIAN_POINT('Ctrl Pts',(-43.4735820751074,33.332034495862,-49.2642208333334));
#258293=CARTESIAN_POINT('Ctrl Pts',(-44.5079524583201,33.9292285150516,
-49.2058875));
#258294=CARTESIAN_POINT('Ctrl Pts',(-45.5423228415328,33.332034495862,-49.1475541666667));
#258295=CARTESIAN_POINT('Ctrl Pts',(-46.5766932247455,32.7348404766724,
-49.0892208333333));
#258296=CARTESIAN_POINT('Ctrl Pts',(-46.5766932247455,31.5404524382932,
-49.0308875));
#258297=CARTESIAN_POINT('Ctrl Pts',(-46.5766932247455,30.3460643999139,
-48.9725541666667));
#258298=CARTESIAN_POINT('Ctrl Pts',(-45.5423228415329,29.7488703807243,
-48.9142208333333));
#258299=CARTESIAN_POINT('Ctrl Pts',(-44.5079524583202,29.1516763615346,
-48.8558875));
#258300=CARTESIAN_POINT('Ctrl Pts',(-43.4735820751074,29.7488703807243,
-48.7975541666667));
#258301=CARTESIAN_POINT('Ctrl Pts',(-42.4392116918948,30.3460643999138,
-48.7392208333334));
#258302=CARTESIAN_POINT('Ctrl Pts',(-42.4392116918948,31.5404524382931,
-48.6808875));
#258303=CARTESIAN_POINT('Ctrl Pts',(-42.4392116918947,32.7348404766723,
-48.6225541666667));
#258304=CARTESIAN_POINT('Ctrl Pts',(-43.4735820751074,33.332034495862,-48.5642208333334));
#258305=CARTESIAN_POINT('Ctrl Pts',(-44.5079524583201,33.9292285150516,
-48.5058875));
#258306=CARTESIAN_POINT('Ctrl Pts',(-45.5423228415328,33.332034495862,-48.4475541666667));
#258307=CARTESIAN_POINT('Ctrl Pts',(-46.5766932247455,32.7348404766724,
-48.3892208333334));
#258308=CARTESIAN_POINT('Ctrl Pts',(-46.5766932247455,31.5404524382932,
-48.3308875));
#258309=CARTESIAN_POINT('Ctrl Pts',(-46.5766932247455,30.3460643999139,
-48.2725541666667));
#258310=CARTESIAN_POINT('Ctrl Pts',(-45.5423228415329,29.7488703807243,
-48.2142208333334));
#258311=CARTESIAN_POINT('Ctrl Pts',(-44.5079524583202,29.1516763615346,
-48.1558875));
#258312=CARTESIAN_POINT('Ctrl Pts',(-43.4735820751074,29.7488703807243,
-48.0975541666667));
#258313=CARTESIAN_POINT('Ctrl Pts',(-42.4392116918948,30.3460643999138,
-48.0392208333334));
#258314=CARTESIAN_POINT('Ctrl Pts',(-42.4392116918948,31.5404524382931,
-47.9808875));
#258315=CARTESIAN_POINT('Ctrl Pts',(-42.4392116918947,32.7348404766723,
-47.9225541666667));
#258316=CARTESIAN_POINT('Ctrl Pts',(-43.4735820751074,33.332034495862,-47.8642208333334));
#258317=CARTESIAN_POINT('Ctrl Pts',(-44.5079524583201,33.9292285150516,
-47.8058875000001));
#258318=CARTESIAN_POINT('Ctrl Pts',(-45.5423228415328,33.332034495862,-47.7475541666667));
#258319=CARTESIAN_POINT('Ctrl Pts',(-46.5766932247455,32.7348404766724,
-47.6892208333334));
#258320=CARTESIAN_POINT('Ctrl Pts',(-46.5766932247455,31.5404524382932,
-47.6308875));
#258321=CARTESIAN_POINT('Ctrl Pts',(-46.5766932247455,30.3460643999139,
-47.5725541666667));
#258322=CARTESIAN_POINT('Ctrl Pts',(-45.5423228415329,29.7488703807243,
-47.5142208333333));
#258323=CARTESIAN_POINT('Ctrl Pts',(-44.5079524583202,29.1516763615346,
-47.4558875));
#258324=CARTESIAN_POINT('Ctrl Pts',(-43.4735820751074,29.7488703807243,
-47.3975541666667));
#258325=CARTESIAN_POINT('Ctrl Pts',(-42.4392116918948,30.3460643999138,
-47.3392208333333));
#258326=CARTESIAN_POINT('Ctrl Pts',(-42.4392116918948,31.5404524382931,
-47.2808875));
#258327=CARTESIAN_POINT('Ctrl Pts',(-42.4392116918947,32.7348404766723,
-47.2225541666667));
#258328=CARTESIAN_POINT('Ctrl Pts',(-43.4735820751074,33.332034495862,-47.1642208333334));
#258329=CARTESIAN_POINT('Ctrl Pts',(-44.5079524583201,33.9292285150516,
-47.1058875));
#258330=CARTESIAN_POINT('Ctrl Pts',(-45.5423228415328,33.332034495862,-47.0475541666667));
#258331=CARTESIAN_POINT('Ctrl Pts',(-46.5766932247455,32.7348404766724,
-46.9892208333334));
#258332=CARTESIAN_POINT('Ctrl Pts',(-46.5766932247455,31.5404524382932,
-46.9308875));
#258333=CARTESIAN_POINT('Ctrl Pts',(-46.5766932247455,30.3460643999139,
-46.8725541666667));
#258334=CARTESIAN_POINT('Ctrl Pts',(-45.5423228415329,29.7488703807243,
-46.8142208333334));
#258335=CARTESIAN_POINT('Ctrl Pts',(-44.5079524583202,29.1516763615346,
-46.7558875));
#258336=CARTESIAN_POINT('Ctrl Pts',(-43.4735820751074,29.7488703807243,
-46.6975541666667));
#258337=CARTESIAN_POINT('Ctrl Pts',(-42.4392116918948,30.3460643999138,
-46.6392208333333));
#258338=CARTESIAN_POINT('Ctrl Pts',(-42.4392116918948,31.5404524382931,
-46.5808875));
#258339=CARTESIAN_POINT('Ctrl Pts',(-42.4392116918948,32.7348404766723,
-46.5225541666667));
#258340=CARTESIAN_POINT('Ctrl Pts',(-43.4735820751074,33.332034495862,-46.4642208333334));
#258341=CARTESIAN_POINT('Ctrl Pts',(-44.5079524583201,33.9292285150516,
-46.4058875));
#258342=CARTESIAN_POINT('Ctrl Pts',(-45.5423228415328,33.332034495862,-46.3475541666667));
#258343=CARTESIAN_POINT('Ctrl Pts',(-46.5766932247455,32.7348404766724,
-46.2892208333334));
#258344=CARTESIAN_POINT('Ctrl Pts',(-46.5766932247455,31.5404524382932,
-46.2308875));
#258345=CARTESIAN_POINT('Ctrl Pts',(-46.5766932247455,30.3460643999139,
-46.1725541666667));
#258346=CARTESIAN_POINT('Ctrl Pts',(-45.5423228415329,29.7488703807243,
-46.1142208333334));
#258347=CARTESIAN_POINT('Ctrl Pts',(-44.5079524583202,29.1516763615346,
-46.0558875));
#258348=CARTESIAN_POINT('Ctrl Pts',(-43.4735820751074,29.7488703807243,
-45.9975541666667));
#258349=CARTESIAN_POINT('Ctrl Pts',(-42.4392116918948,30.3460643999138,
-45.9392208333333));
#258350=CARTESIAN_POINT('Ctrl Pts',(-42.4392116918948,31.5404524382931,
-45.8808875));
#258351=CARTESIAN_POINT('Ctrl Pts',(-42.4392116918948,32.7348404766723,
-45.8225541666667));
#258352=CARTESIAN_POINT('Ctrl Pts',(-43.4735820751074,33.332034495862,-45.7642208333334));
#258353=CARTESIAN_POINT('Ctrl Pts',(-44.5079524583201,33.9292285150516,
-45.7058875));
#258354=CARTESIAN_POINT('Ctrl Pts',(-45.5423228415328,33.332034495862,-45.6475541666667));
#258355=CARTESIAN_POINT('Ctrl Pts',(-46.5766932247455,32.7348404766724,
-45.5892208333333));
#258356=CARTESIAN_POINT('Ctrl Pts',(-46.5766932247455,31.5404524382932,
-45.5308875));
#258357=CARTESIAN_POINT('Ctrl Pts',(-46.5766932247455,30.3460643999139,
-45.4725541666667));
#258358=CARTESIAN_POINT('Ctrl Pts',(-45.5423228415329,29.7488703807243,
-45.4142208333334));
#258359=CARTESIAN_POINT('Ctrl Pts',(-44.5079524583202,29.1516763615346,
-45.3558875));
#258360=CARTESIAN_POINT('Ctrl Pts',(-43.4735820751074,29.7488703807243,
-45.2975541666667));
#258361=CARTESIAN_POINT('Ctrl Pts',(-42.4392116918948,30.3460643999138,
-45.2392208333333));
#258362=CARTESIAN_POINT('Ctrl Pts',(-42.4392116918948,31.5404524382931,
-45.1808875));
#258363=CARTESIAN_POINT('Ctrl Pts',(-42.4392116918948,32.7348404766723,
-45.1225541666667));
#258364=CARTESIAN_POINT('Ctrl Pts',(-43.4735820751074,33.332034495862,-45.0642208333334));
#258365=CARTESIAN_POINT('Ctrl Pts',(-44.5079524583201,33.9292285150516,
-45.0058875));
#258366=CARTESIAN_POINT('Ctrl Pts',(-45.5423228415328,33.332034495862,-44.9475541666667));
#258367=CARTESIAN_POINT('Ctrl Pts',(-46.5766932247455,32.7348404766724,
-44.8892208333333));
#258368=CARTESIAN_POINT('Ctrl Pts',(-46.5766932247455,31.5404524382932,
-44.8308875));
#258369=CARTESIAN_POINT('Ctrl Pts',(-46.5766932247455,30.3460643999139,
-44.7725541666666));
#258370=CARTESIAN_POINT('Ctrl Pts',(-45.5423228415329,29.7488703807243,
-44.7142208333334));
#258371=CARTESIAN_POINT('Ctrl Pts',(-44.5079524583202,29.1516763615346,
-44.6558875));
#258372=CARTESIAN_POINT('Ctrl Pts',(-43.4735820751074,29.7488703807243,
-44.5975541666667));
#258373=CARTESIAN_POINT('Ctrl Pts',(-42.4392116918948,30.3460643999138,
-44.5392208333333));
#258374=CARTESIAN_POINT('Ctrl Pts',(-42.4392116918948,31.5404524382931,
-44.4808875));
#258375=CARTESIAN_POINT('Ctrl Pts',(-42.4392116918948,32.7348404766723,
-44.4225541666667));
#258376=CARTESIAN_POINT('Ctrl Pts',(-43.4735820751074,33.332034495862,-44.3642208333333));
#258377=CARTESIAN_POINT('Ctrl Pts',(-44.5079524583201,33.9292285150516,
-44.3058875));
#258378=CARTESIAN_POINT('Ctrl Pts',(-45.5423228415328,33.332034495862,-44.2475541666667));
#258379=CARTESIAN_POINT('Ctrl Pts',(-46.5766932247455,32.7348404766724,
-44.1892208333334));
#258380=CARTESIAN_POINT('Ctrl Pts',(-46.5766932247455,31.5404524382932,
-44.1308875));
#258381=CARTESIAN_POINT('Ctrl Pts',(-46.5766932247455,30.3460643999139,
-44.0725541666667));
#258382=CARTESIAN_POINT('Ctrl Pts',(-45.5423228415329,29.7488703807243,
-44.0142208333334));
#258383=CARTESIAN_POINT('Ctrl Pts',(-44.5079524583202,29.1516763615346,
-43.9558875));
#258384=CARTESIAN_POINT('Ctrl Pts',(-43.4735820751074,29.7488703807243,
-43.8975541666667));
#258385=CARTESIAN_POINT('Ctrl Pts',(-42.4392116918948,30.3460643999138,
-43.8392208333333));
#258386=CARTESIAN_POINT('Ctrl Pts',(-42.4392116918948,31.5404524382931,
-43.7808875));
#258387=CARTESIAN_POINT('Ctrl Pts',(-42.4392116918948,32.7348404766723,
-43.7225541666667));
#258388=CARTESIAN_POINT('Ctrl Pts',(-43.4735820751074,33.332034495862,-43.6642208333334));
#258389=CARTESIAN_POINT('Ctrl Pts',(-44.5079524583201,33.9292285150516,
-43.6058875));
#258390=CARTESIAN_POINT('Ctrl Pts',(-45.5423228415328,33.332034495862,-43.5475541666667));
#258391=CARTESIAN_POINT('Ctrl Pts',(-46.5766932247455,32.7348404766724,
-43.4892208333333));
#258392=CARTESIAN_POINT('Ctrl Pts',(-46.5766932247455,31.5404524382932,
-43.4308875));
#258393=CARTESIAN_POINT('Ctrl Pts',(-46.5766932247455,30.3460643999139,
-43.3725541666667));
#258394=CARTESIAN_POINT('Ctrl Pts',(-45.5423228415329,29.7488703807243,
-43.3142208333334));
#258395=CARTESIAN_POINT('Ctrl Pts',(-44.5079524583202,29.1516763615346,
-43.2558875));
#258396=CARTESIAN_POINT('Ctrl Pts',(-43.4735820751074,29.7488703807243,
-43.1975541666667));
#258397=CARTESIAN_POINT('Ctrl Pts',(-42.4392116918948,30.3460643999138,
-43.1392208333334));
#258398=CARTESIAN_POINT('Ctrl Pts',(-42.4392116918948,31.5404524382931,
-43.0808875));
#258399=CARTESIAN_POINT('Ctrl Pts',(-42.4392116918948,32.7348404766723,
-43.0225541666667));
#258400=CARTESIAN_POINT('Ctrl Pts',(-43.4735820751074,33.332034495862,-42.9642208333334));
#258401=CARTESIAN_POINT('Ctrl Pts',(-44.5079524583201,33.9292285150516,
-42.9058875));
#258402=CARTESIAN_POINT('Ctrl Pts',(-45.5423228415328,33.332034495862,-42.8475541666667));
#258403=CARTESIAN_POINT('Ctrl Pts',(-46.5766932247455,32.7348404766724,
-42.7892208333334));
#258404=CARTESIAN_POINT('Ctrl Pts',(-46.5766932247455,31.5404524382932,
-42.7308875));
#258405=CARTESIAN_POINT('Ctrl Pts',(-46.5766932247455,30.3460643999139,
-42.6725541666667));
#258406=CARTESIAN_POINT('Ctrl Pts',(-45.5423228415329,29.7488703807243,
-42.6142208333334));
#258407=CARTESIAN_POINT('Ctrl Pts',(-44.5079524583202,29.1516763615346,
-42.5558875));
#258408=CARTESIAN_POINT('Ctrl Pts',(-43.4735820751074,29.7488703807243,
-42.4975541666667));
#258409=CARTESIAN_POINT('Ctrl Pts',(-42.4392116918948,30.3460643999138,
-42.4392208333334));
#258410=CARTESIAN_POINT('Ctrl Pts',(-42.4392116918948,31.5404524382931,
-42.3808875));
#258411=CARTESIAN_POINT('Ctrl Pts',(-42.4392116918948,32.7348404766723,
-42.3225541666667));
#258412=CARTESIAN_POINT('Ctrl Pts',(-43.4735820751074,33.332034495862,-42.2642208333334));
#258413=CARTESIAN_POINT('Ctrl Pts',(-44.5079524583201,33.9292285150516,
-42.2058875));
#258414=CARTESIAN_POINT('Ctrl Pts',(-45.5423228415328,33.332034495862,-42.1475541666667));
#258415=CARTESIAN_POINT('Ctrl Pts',(-46.5766932247455,32.7348404766724,
-42.0892208333333));
#258416=CARTESIAN_POINT('Ctrl Pts',(-46.5766932247455,31.5404524382932,
-42.0308875));
#258417=CARTESIAN_POINT('Ctrl Pts',(-46.5766932247455,30.3460643999139,
-41.9725541666667));
#258418=CARTESIAN_POINT('Ctrl Pts',(-45.5423228415329,29.7488703807243,
-41.9142208333334));
#258419=CARTESIAN_POINT('Ctrl Pts',(-44.5079524583202,29.1516763615346,
-41.8558875));
#258420=CARTESIAN_POINT('Ctrl Pts',(-43.4735820751074,29.7488703807243,
-41.7975541666667));
#258421=CARTESIAN_POINT('Ctrl Pts',(-42.4392116918948,30.3460643999138,
-41.7392208333333));
#258422=CARTESIAN_POINT('Ctrl Pts',(-42.4392116918948,31.5404524382931,
-41.6808875));
#258423=CARTESIAN_POINT('Ctrl Pts',(-42.4392116918948,32.7348404766723,
-41.6225541666667));
#258424=CARTESIAN_POINT('Ctrl Pts',(-43.4735820751074,33.332034495862,-41.5642208333334));
#258425=CARTESIAN_POINT('Ctrl Pts',(-44.5079524583201,33.9292285150516,
-41.5058875));
#258426=CARTESIAN_POINT('Ctrl Pts',(-45.5423228415328,33.332034495862,-41.4475541666667));
#258427=CARTESIAN_POINT('Ctrl Pts',(-46.5766932247455,32.7348404766724,
-41.3892208333333));
#258428=CARTESIAN_POINT('Ctrl Pts',(-46.5766932247455,31.5404524382932,
-41.3308875));
#258429=CARTESIAN_POINT('Ctrl Pts',(-46.5766932247455,30.3460643999139,
-41.2725541666667));
#258430=CARTESIAN_POINT('Ctrl Pts',(-45.5423228415329,29.7488703807243,
-41.2142208333333));
#258431=CARTESIAN_POINT('Ctrl Pts',(-44.5079524583202,29.1516763615346,
-41.1558875));
#258432=CARTESIAN_POINT('Ctrl Pts',(-43.4735820751074,29.7488703807243,
-41.0975541666667));
#258433=CARTESIAN_POINT('Ctrl Pts',(-42.4392116918948,30.3460643999138,
-41.0392208333333));
#258434=CARTESIAN_POINT('Ctrl Pts',(-42.4392116918948,31.5404524382931,
-40.9808875));
#258435=CARTESIAN_POINT('Ctrl Pts',(-42.4392116918948,32.7348404766723,
-40.9225541666667));
#258436=CARTESIAN_POINT('Ctrl Pts',(-43.4735820751074,33.332034495862,-40.8642208333334));
#258437=CARTESIAN_POINT('Ctrl Pts',(-44.5079524583201,33.9292285150516,
-40.8058875));
#258438=CARTESIAN_POINT('Ctrl Pts',(-45.5423228415328,33.332034495862,-40.7475541666667));
#258439=CARTESIAN_POINT('Ctrl Pts',(-46.5766932247455,32.7348404766724,
-40.6892208333333));
#258440=CARTESIAN_POINT('Ctrl Pts',(-46.5766932247455,31.5404524382932,
-40.6308875));
#258441=CARTESIAN_POINT('Ctrl Pts',(-46.5766932247455,30.3460643999139,
-40.5725541666667));
#258442=CARTESIAN_POINT('Ctrl Pts',(-45.5423228415329,29.7488703807243,
-40.5142208333333));
#258443=CARTESIAN_POINT('Ctrl Pts',(-44.5079524583202,29.1516763615346,
-40.4558875));
#258444=CARTESIAN_POINT('Ctrl Pts',(-43.4735820751074,29.7488703807243,
-40.3975541666667));
#258445=CARTESIAN_POINT('Ctrl Pts',(-42.4392116918948,30.3460643999138,
-40.3392208333333));
#258446=CARTESIAN_POINT('Ctrl Pts',(-42.4392116918948,31.5404524382931,
-40.2808875));
#258447=CARTESIAN_POINT('Ctrl Pts',(-42.4392116918948,32.7348404766723,
-40.2225541666667));
#258448=CARTESIAN_POINT('Ctrl Pts',(-43.4735820751074,33.332034495862,-40.1642208333333));
#258449=CARTESIAN_POINT('Ctrl Pts',(-44.5079524583201,33.9292285150516,
-40.1058875));
#258450=CARTESIAN_POINT('Ctrl Pts',(-45.5423228415328,33.332034495862,-40.0475541666667));
#258451=CARTESIAN_POINT('Ctrl Pts',(-46.5766932247455,32.7348404766724,
-39.9892208333333));
#258452=CARTESIAN_POINT('Ctrl Pts',(-46.5766932247455,31.5404524382932,
-39.9308875));
#258453=CARTESIAN_POINT('Ctrl Pts',(-46.5766932247455,30.3460643999139,
-39.8725541666667));
#258454=CARTESIAN_POINT('Ctrl Pts',(-45.5423228415329,29.7488703807243,
-39.8142208333334));
#258455=CARTESIAN_POINT('Ctrl Pts',(-44.5079524583202,29.1516763615346,
-39.7558875));
#258456=CARTESIAN_POINT('Ctrl Pts',(-43.4735820751074,29.7488703807243,
-39.6975541666667));
#258457=CARTESIAN_POINT('Ctrl Pts',(-42.4392116918948,30.3460643999138,
-39.6392208333334));
#258458=CARTESIAN_POINT('Ctrl Pts',(-42.4392116918948,31.5404524382931,
-39.5808875));
#258459=CARTESIAN_POINT('Ctrl Pts',(-42.4392116918948,32.7348404766723,
-39.5225541666667));
#258460=CARTESIAN_POINT('Ctrl Pts',(-43.4735820751074,33.332034495862,-39.4642208333333));
#258461=CARTESIAN_POINT('Ctrl Pts',(-44.5079524583201,33.9292285150516,
-39.4058875));
#258462=CARTESIAN_POINT('Ctrl Pts',(-45.5423228415328,33.332034495862,-39.3475541666667));
#258463=CARTESIAN_POINT('Ctrl Pts',(-46.5766932247455,32.7348404766724,
-39.2892208333334));
#258464=CARTESIAN_POINT('Ctrl Pts',(-46.5766932247455,31.5404524382932,
-39.2308875));
#258465=CARTESIAN_POINT('Ctrl Pts',(-46.5766932247455,30.3460643999139,
-39.1725541666667));
#258466=CARTESIAN_POINT('Ctrl Pts',(-45.5423228415329,29.7488703807243,
-39.1142208333333));
#258467=CARTESIAN_POINT('Ctrl Pts',(-44.5079524583202,29.1516763615346,
-39.0558875));
#258468=CARTESIAN_POINT('Ctrl Pts',(-43.4735820751074,29.7488703807243,
-38.9975541666667));
#258469=CARTESIAN_POINT('Ctrl Pts',(-42.4392116918948,30.3460643999138,
-38.9392208333334));
#258470=CARTESIAN_POINT('Ctrl Pts',(-42.4392116918948,31.5404524382931,
-38.8808875));
#258471=CARTESIAN_POINT('Ctrl Pts',(-42.4392116918948,32.7348404766723,
-38.8225541666667));
#258472=CARTESIAN_POINT('Ctrl Pts',(-43.4735820751074,33.332034495862,-38.7642208333333));
#258473=CARTESIAN_POINT('Ctrl Pts',(-44.5079524583201,33.9292285150516,
-38.7058875));
#258474=CARTESIAN_POINT('Ctrl Pts',(-45.5423228415328,33.332034495862,-38.6475541666667));
#258475=CARTESIAN_POINT('Ctrl Pts',(-46.5766932247455,32.7348404766724,
-38.5892208333334));
#258476=CARTESIAN_POINT('Ctrl Pts',(-46.5766932247455,31.5404524382932,
-38.5308875));
#258477=CARTESIAN_POINT('Ctrl Pts',(-46.5766932247455,30.3460643999139,
-38.4725541666667));
#258478=CARTESIAN_POINT('Ctrl Pts',(-45.5423228415329,29.7488703807243,
-38.4142208333334));
#258479=CARTESIAN_POINT('Ctrl Pts',(-44.5079524583202,29.1516763615346,
-38.3558875));
#258480=CARTESIAN_POINT('Ctrl Pts',(-43.4735820751074,29.7488703807243,
-38.2975541666667));
#258481=CARTESIAN_POINT('Ctrl Pts',(-42.4392116918948,30.3460643999138,
-38.2392208333333));
#258482=CARTESIAN_POINT('Ctrl Pts',(-42.4392116918948,31.5404524382931,
-38.1808875));
#258483=CARTESIAN_POINT('Ctrl Pts',(-42.4392116918948,32.7348404766723,
-38.1225541666667));
#258484=CARTESIAN_POINT('Ctrl Pts',(-43.4735820751074,33.332034495862,-38.0642208333334));
#258485=CARTESIAN_POINT('Ctrl Pts',(-44.5079524583201,33.9292285150516,
-38.0058875));
#258486=CARTESIAN_POINT('Ctrl Pts',(-45.5423228415328,33.332034495862,-37.9475541666667));
#258487=CARTESIAN_POINT('Ctrl Pts',(-46.5766932247455,32.7348404766724,
-37.8892208333334));
#258488=CARTESIAN_POINT('Ctrl Pts',(-46.5766932247455,31.5404524382932,
-37.8308875));
#258489=CARTESIAN_POINT('Ctrl Pts',(-46.5766932247455,30.3460643999139,
-37.7725541666667));
#258490=CARTESIAN_POINT('Ctrl Pts',(-45.5423228415329,29.7488703807243,
-37.7142208333333));
#258491=CARTESIAN_POINT('Ctrl Pts',(-44.5079524583202,29.1516763615346,
-37.6558875));
#258492=CARTESIAN_POINT('Ctrl Pts',(-43.4735820751074,29.7488703807243,
-37.5975541666667));
#258493=CARTESIAN_POINT('Ctrl Pts',(-42.4392116918948,30.3460643999138,
-37.5392208333334));
#258494=CARTESIAN_POINT('Ctrl Pts',(-42.4392116918948,31.5404524382931,
-37.4808875));
#258495=CARTESIAN_POINT('Ctrl Pts',(-42.4392116918948,32.7348404766723,
-37.4225541666667));
#258496=CARTESIAN_POINT('Ctrl Pts',(-43.4735820751074,33.332034495862,-37.3642208333333));
#258497=CARTESIAN_POINT('Ctrl Pts',(-44.5079524583201,33.9292285150516,
-37.3058875));
#258498=CARTESIAN_POINT('Ctrl Pts',(-45.5423228415328,33.332034495862,-37.2475541666667));
#258499=CARTESIAN_POINT('Ctrl Pts',(-45.6766168155003,33.2544998338414,
-37.239980655983));
#258500=CARTESIAN_POINT('Ctrl Pts',(-45.7978513037523,33.1578111886089,
-37.2318399189827));
#258501=CARTESIAN_POINT('Ctrl Pts',(-42.8392071752677,31.5404524382931,
-52.64995));
#258502=CARTESIAN_POINT('Ctrl Pts',(-42.8226659458705,31.698184429907,-52.64995));
#258503=CARTESIAN_POINT('Ctrl Pts',(-42.8274712764285,31.857393032193,-52.64995));
#258504=CARTESIAN_POINT('Ctrl Pts',(-42.8786574174946,32.1643235021153,
-52.64995));
#258505=CARTESIAN_POINT('Ctrl Pts',(-42.9232286878865,32.3108921662114,
-52.64995));
#258506=CARTESIAN_POINT('Ctrl Pts',(-43.0750368173286,32.6461601401754,
-52.64995));
#258507=CARTESIAN_POINT('Ctrl Pts',(-43.199204951854,32.8244027472953,-52.64995));
#258508=CARTESIAN_POINT('Ctrl Pts',(-43.5542933457999,33.1754582937784,
-52.64995));
#258509=CARTESIAN_POINT('Ctrl Pts',(-43.7742269286882,33.2962963987312,
-52.64995));
#258510=CARTESIAN_POINT('Ctrl Pts',(-44.079508833452,33.4246330791964,-52.64995));
#258511=CARTESIAN_POINT('Ctrl Pts',(-44.2169771822674,33.4654712631672,
-52.64995));
#258512=CARTESIAN_POINT('Ctrl Pts',(-44.4991010430727,33.5166685395148,
-52.64995));
#258513=CARTESIAN_POINT('Ctrl Pts',(-44.6429009445464,33.526707841618,-52.64995));
#258514=CARTESIAN_POINT('Ctrl Pts',(-44.7865238868864,33.5209569091753,
-52.64995));
#258515=CARTESIAN_POINT('Ctrl Pts',(-45.4138902596022,33.323505073581,-40.0133536282584));
#258516=CARTESIAN_POINT('Ctrl Pts',(-45.2343960628182,33.4147029298636,
-40.0238241230707));
#258517=CARTESIAN_POINT('Ctrl Pts',(-45.0421833621338,33.4782627639555,
-40.0350365306106));
#258518=CARTESIAN_POINT('Ctrl Pts',(-44.6401461563769,33.546739741288,-40.0584887009463));
#258519=CARTESIAN_POINT('Ctrl Pts',(-44.4323784874203,33.5496690225212,
-40.0706084816355));
#258520=CARTESIAN_POINT('Ctrl Pts',(-43.965283865819,33.4836041701764,-40.0978556678955));
#258521=CARTESIAN_POINT('Ctrl Pts',(-43.7127963349201,33.3946236208596,
-40.1123894250198));
#258522=CARTESIAN_POINT('Ctrl Pts',(-43.2663921378172,33.1289396202989,
-40.1388314112441));
#258523=CARTESIAN_POINT('Ctrl Pts',(-43.0745867349475,32.9582604222257,
-40.1530481325778));
#258524=CARTESIAN_POINT('Ctrl Pts',(-42.7592677610395,32.5464128492502,
-40.1830507128567));
#258525=CARTESIAN_POINT('Ctrl Pts',(-42.6417717032953,32.3067654968633,
-40.1985842217561));
#258526=CARTESIAN_POINT('Ctrl Pts',(-42.5080675690629,31.8005712300943,
-40.2280559228371));
#258527=CARTESIAN_POINT('Ctrl Pts',(-42.491225438116,31.539507602342,-40.24075985994));
#258528=CARTESIAN_POINT('Ctrl Pts',(-42.5578673808582,31.0271940342069,
-40.2685847162115));
#258529=CARTESIAN_POINT('Ctrl Pts',(-42.6400423036273,30.7807512666597,
-40.2834313171333));
#258530=CARTESIAN_POINT('Ctrl Pts',(-42.8982610531121,30.3236941111856,
-40.3140523786047));
#258531=CARTESIAN_POINT('Ctrl Pts',(-43.0753335831877,30.1194513548329,
-40.3295349599719));
#258532=CARTESIAN_POINT('Ctrl Pts',(-43.4885359770171,29.801119579637,-40.3576682283675));
#258533=CARTESIAN_POINT('Ctrl Pts',(-43.7173503770357,29.6858775233593,
-40.3700815452588));
#258534=CARTESIAN_POINT('Ctrl Pts',(-44.1397209055691,29.5659481498849,
-40.39471982609));
#258535=CARTESIAN_POINT('Ctrl Pts',(-44.3235830214837,29.5404524382925,
-40.4054451161849));
#258536=CARTESIAN_POINT('Ctrl Pts',(-44.5079524583208,29.5404524382925,
-40.4162000000005));
#258537=CARTESIAN_POINT('Origin',(-44.5079524583206,-57.475452478349,235.35105));
#258538=CARTESIAN_POINT('',(-44.2366247616132,-55.4939425958135,-39.0141962777036));
#258539=CARTESIAN_POINT('Ctrl Pts',(-44.2366247583656,-55.4939426255002,
-39.0141963182746));
#258540=CARTESIAN_POINT('Ctrl Pts',(-44.2338595158803,-55.4943212705074,
-39.0136979066985));
#258541=CARTESIAN_POINT('Ctrl Pts',(-44.2310952123238,-55.494705686492,
-39.0132009363795));
#258542=CARTESIAN_POINT('Ctrl Pts',(-44.1959512291589,-55.4996679139964,
-39.0068980480834));
#258543=CARTESIAN_POINT('Ctrl Pts',(-44.1637009035284,-55.5050310901567,
-39.0012798595208));
#258544=CARTESIAN_POINT('Ctrl Pts',(-44.0994607677182,-55.5173400934252,
-38.9904230184279));
#258545=CARTESIAN_POINT('Ctrl Pts',(-44.0674709555852,-55.5242859080952,
-38.9851843621813));
#258546=CARTESIAN_POINT('Ctrl Pts',(-44.0037536572564,-55.5397721100658,
-38.9750906394313));
#258547=CARTESIAN_POINT('Ctrl Pts',(-43.9720261650696,-55.5483124604321,
-38.9702355633813));
#258548=CARTESIAN_POINT('Ctrl Pts',(-43.9088372843841,-55.5670115927043,
-38.9609158992096));
#258549=CARTESIAN_POINT('Ctrl Pts',(-43.877363149692,-55.5771759127617,
-38.9564497975263));
#258550=CARTESIAN_POINT('Ctrl Pts',(-43.8147378173409,-55.5991372642861,
-38.9479240409952));
#258551=CARTESIAN_POINT('Ctrl Pts',(-43.783451665776,-55.6109933882688,
-38.943848461355));
#258552=CARTESIAN_POINT('Ctrl Pts',(-43.7218906736911,-55.6361026235129,
-38.9361997181442));
#258553=CARTESIAN_POINT('Ctrl Pts',(-43.6915050002909,-55.6493890121587,
-38.9326103047847));
#258554=CARTESIAN_POINT('Ctrl Pts',(-43.631563048157,-55.6773880028563,
-38.9259028928878));
#258555=CARTESIAN_POINT('Ctrl Pts',(-43.601998052992,-55.6921031576597,
-38.9227836015923));
#258556=CARTESIAN_POINT('Ctrl Pts',(-43.5179303005816,-55.7365693660334,
-38.914462897476));
#258557=CARTESIAN_POINT('Ctrl Pts',(-43.4644496898179,-55.7681223775077,
-38.909852823657));
#258558=CARTESIAN_POINT('Ctrl Pts',(-43.412401760938,-55.8022014933363,
-38.9060754072981));
#258559=CARTESIAN_POINT('',(-42.599626743264,-58.0740282963067,-39.2098669215977));
#258560=CARTESIAN_POINT('Ctrl Pts',(-44.2366247692744,-55.4939426503596,
-39.0141962812275));
#258561=CARTESIAN_POINT('Ctrl Pts',(-44.1816234426521,-55.5014739795454,
-39.0171945157568));
#258562=CARTESIAN_POINT('Ctrl Pts',(-44.1264848220931,-55.511360891976,
-39.0202683895418));
#258563=CARTESIAN_POINT('Ctrl Pts',(-44.0715088992886,-55.5236541187052,
-39.0234042273537));
#258564=CARTESIAN_POINT('Ctrl Pts',(-44.016932191927,-55.5358580764289,
-39.0265172938357));
#258565=CARTESIAN_POINT('Ctrl Pts',(-43.9625165190864,-55.550433742495,
-39.0296913990414));
#258566=CARTESIAN_POINT('Ctrl Pts',(-43.9085673130736,-55.567380883633,
-39.0329111064327));
#258567=CARTESIAN_POINT('Ctrl Pts',(-43.8549038016002,-55.5842382791373,
-39.0361137634745));
#258568=CARTESIAN_POINT('Ctrl Pts',(-43.801702557357,-55.6034421513973,
-39.0393615057487));
#258569=CARTESIAN_POINT('Ctrl Pts',(-43.749265424276,-55.6249407308052,
-39.0426375748536));
#258570=CARTESIAN_POINT('Ctrl Pts',(-43.6969997422626,-55.6463690173848,
-39.0459029323596));
#258571=CARTESIAN_POINT('Ctrl Pts',(-43.645493907733,-55.6700769138001,
-39.0491963917554));
#258572=CARTESIAN_POINT('Ctrl Pts',(-43.5950371540441,-55.6959622708899,
-39.0525003623023));
#258573=CARTESIAN_POINT('Ctrl Pts',(-43.5446118156451,-55.7218315112868,
-39.0558022757373));
#258574=CARTESIAN_POINT('Ctrl Pts',(-43.4952349376079,-55.7498752261513,
-39.0591146445718));
#258575=CARTESIAN_POINT('Ctrl Pts',(-43.4471749346482,-55.7799434619491,
-39.0624195354973));
#258576=CARTESIAN_POINT('Ctrl Pts',(-43.3990613691433,-55.8100452085905,
-39.0657281097011));
#258577=CARTESIAN_POINT('Ctrl Pts',(-43.3522682206211,-55.8421755622777,
-39.069029146243));
#258578=CARTESIAN_POINT('Ctrl Pts',(-43.3070347303892,-55.8761412415753,
-39.0723049218769));
#258579=CARTESIAN_POINT('Ctrl Pts',(-43.2616720745725,-55.9102039108864,
-39.0755900515862));
#258580=CARTESIAN_POINT('Ctrl Pts',(-43.2178784859956,-55.9461118443527,
-39.0788497349381));
#258581=CARTESIAN_POINT('Ctrl Pts',(-43.1758567523826,-55.983634493292,
-39.0820670033003));
#258582=CARTESIAN_POINT('Ctrl Pts',(-43.1334622507125,-56.0214899996301,
-39.0853128115339));
#258583=CARTESIAN_POINT('Ctrl Pts',(-43.0928715614086,-56.0609883511961,
-39.0885154107999));
#258584=CARTESIAN_POINT('Ctrl Pts',(-43.0542470912624,-56.1018657043628,
-39.0916589013438));
#258585=CARTESIAN_POINT('Ctrl Pts',(-43.0154024605019,-56.1429760596432,
-39.0948203098761));
#258586=CARTESIAN_POINT('Ctrl Pts',(-42.9785467086067,-56.1854804548215,
-39.0979219035787));
#258587=CARTESIAN_POINT('Ctrl Pts',(-42.9437946423332,-56.2290936658421,
-39.1009495637756));
#258588=CARTESIAN_POINT('Ctrl Pts',(-42.9085901815573,-56.273274623734,
-39.104016637365));
#258589=CARTESIAN_POINT('Ctrl Pts',(-42.8755445902652,-56.318592705421,
-39.1070078153198));
#258590=CARTESIAN_POINT('Ctrl Pts',(-42.8447237362775,-56.3647454016771,
-39.10991094713));
#258591=CARTESIAN_POINT('Ctrl Pts',(-42.8203947202628,-56.4011768933802,
-39.1122025883782));
#258592=CARTESIAN_POINT('Ctrl Pts',(-42.7974508292817,-56.4381282062735,
-39.1144394174622));
#258593=CARTESIAN_POINT('Ctrl Pts',(-42.7759016507517,-56.4754524783487,
-39.1166166666666));
#258594=CARTESIAN_POINT('Ctrl Pts',(-42.7485194349713,-56.5228798673043,
-39.1193832643557));
#258595=CARTESIAN_POINT('Ctrl Pts',(-42.7227853156708,-56.5719579455147,
-39.1222461525621));
#258596=CARTESIAN_POINT('Ctrl Pts',(-42.6989483896267,-56.6225138678289,
-39.1251952485667));
#258597=CARTESIAN_POINT('Ctrl Pts',(-42.6753690419702,-56.6725234901324,
-39.128112477065));
#258598=CARTESIAN_POINT('Ctrl Pts',(-42.6536467732358,-56.7239789270653,
-39.1311140449706));
#258599=CARTESIAN_POINT('Ctrl Pts',(-42.6339995794796,-56.7766673996404,
-39.134187540091));
#258600=CARTESIAN_POINT('Ctrl Pts',(-42.6145810488471,-56.828742659414,
-39.1372252644543));
#258601=CARTESIAN_POINT('Ctrl Pts',(-42.597190147,-56.8820219948949,-39.1403332266998));
#258602=CARTESIAN_POINT('Ctrl Pts',(-42.5820054437861,-56.9362604394896,
-39.1434971370248));
#258603=CARTESIAN_POINT('Ctrl Pts',(-42.5669079416121,-56.9901874095233,
-39.1466428779944));
#258604=CARTESIAN_POINT('Ctrl Pts',(-42.5539918645355,-57.0450619765139,
-39.1498438955004));
#258605=CARTESIAN_POINT('Ctrl Pts',(-42.543392993098,-57.1006111214144,
-39.1530842633456));
#258606=CARTESIAN_POINT('Ctrl Pts',(-42.532836604651,-57.155937611119,-39.1563116429668));
#258607=CARTESIAN_POINT('Ctrl Pts',(-42.5245792445104,-57.2119326478768,
-39.1595780211275));
#258608=CARTESIAN_POINT('Ctrl Pts',(-42.518709123124,-57.2683030915222,
-39.1628662978962));
#258609=CARTESIAN_POINT('Ctrl Pts',(-42.5128523366118,-57.3245454811242,
-39.1661471048438));
#258610=CARTESIAN_POINT('Ctrl Pts',(-42.509372161352,-57.3811608687148,
-39.1694496698809));
#258611=CARTESIAN_POINT('Ctrl Pts',(-42.5083060983997,-57.4378448214745,
-39.1727562343354));
#258612=CARTESIAN_POINT('Ctrl Pts',(-42.5072390574213,-57.4945807771591,
-39.1760658322944));
#258613=CARTESIAN_POINT('Ctrl Pts',(-42.5085906099458,-57.5513846843009,
-39.1793793938705));
#258614=CARTESIAN_POINT('Ctrl Pts',(-42.5123461307596,-57.6079488207989,
-39.1826789685134));
#258615=CARTESIAN_POINT('Ctrl Pts',(-42.5161064641788,-57.6645854428161,
-39.1859827714784));
#258616=CARTESIAN_POINT('Ctrl Pts',(-42.5222767953613,-57.7209809488454,
-39.1892725090309));
#258617=CARTESIAN_POINT('Ctrl Pts',(-42.5307907462682,-57.7768350714559,
-39.1925306654734));
#258618=CARTESIAN_POINT('Ctrl Pts',(-42.5393557389353,-57.8330240436285,
-39.1958083548028));
#258619=CARTESIAN_POINT('Ctrl Pts',(-42.5502922560484,-57.8886644282291,
-39.1990540427749));
#258620=CARTESIAN_POINT('Ctrl Pts',(-42.5634835159962,-57.9434700632674,
-39.202251036505));
#258621=CARTESIAN_POINT('Ctrl Pts',(-42.5740992219077,-57.9875750620441,
-39.2048238267748));
#258622=CARTESIAN_POINT('Ctrl Pts',(-42.5861741058487,-58.0311397239746,
-39.2073650970601));
#258623=CARTESIAN_POINT('Ctrl Pts',(-42.5996267629089,-58.0740282897704,
-39.2098669280151));
#258624=CARTESIAN_POINT('Ctrl Pts',(-42.5465468229071,-57.0844434842294,
-38.9933892973418));
#258625=CARTESIAN_POINT('Ctrl Pts',(-42.5456036161884,-57.089174404209,
-38.9941812935483));
#258626=CARTESIAN_POINT('Ctrl Pts',(-42.5446783779407,-57.0939047795968,
-38.9949768713224));
#258627=CARTESIAN_POINT('Ctrl Pts',(-42.543771399786,-57.0986331989938,
-38.9957757940657));
#258628=CARTESIAN_POINT('Ctrl Pts',(-42.5375451994903,-57.131092730784,
-39.0012602183534));
#258629=CARTESIAN_POINT('Ctrl Pts',(-42.5321429006105,-57.163596155606,
-39.0069231082391));
#258630=CARTESIAN_POINT('Ctrl Pts',(-42.5275574313231,-57.1961040632046,
-39.0127541622176));
#258631=CARTESIAN_POINT('Ctrl Pts',(-42.5229719620357,-57.2286119708033,
-39.018585216196));
#258632=CARTESIAN_POINT('Ctrl Pts',(-42.5191999190634,-57.2611374049919,
-39.0245864537587));
#258633=CARTESIAN_POINT('Ctrl Pts',(-42.5162298763662,-57.2936802127718,
-39.0307548596727));
#258634=CARTESIAN_POINT('Ctrl Pts',(-42.5102897909718,-57.3587658283315,
-39.0430916715007));
#258635=CARTESIAN_POINT('Ctrl Pts',(-42.5075526709299,-57.4239208272887,
-39.0560961189448));
#258636=CARTESIAN_POINT('Ctrl Pts',(-42.507999333869,-57.4891455421591,
-39.0697591885565));
#258637=CARTESIAN_POINT('Ctrl Pts',(-42.5082226653386,-57.5217578995943,
-39.0765907233624));
#258638=CARTESIAN_POINT('Ctrl Pts',(-42.5092432682604,-57.5543877143394,
-39.0835871924588));
#258639=CARTESIAN_POINT('Ctrl Pts',(-42.5110675613762,-57.5870352205429,
-39.0907492962697));
#258640=CARTESIAN_POINT('Ctrl Pts',(-42.512891854492,-57.6196827267464,
-39.0979114000806));
#258641=CARTESIAN_POINT('Ctrl Pts',(-42.5155178619726,-57.6523290916439,
-39.1052348221532));
#258642=CARTESIAN_POINT('Ctrl Pts',(-42.5189635766488,-57.6850311714121,
-39.1127343794571));
#258643=CARTESIAN_POINT('Ctrl Pts',(-42.5224092913251,-57.7177332511804,
-39.1202339367609));
#258644=CARTESIAN_POINT('Ctrl Pts',(-42.5266542176424,-57.7502677264705,
-39.1278590184786));
#258645=CARTESIAN_POINT('Ctrl Pts',(-42.5316660996073,-57.7825228747794,
-39.1355792827514));
#258646=CARTESIAN_POINT('Ctrl Pts',(-42.5366779815723,-57.8147780230883,
-39.1432995470241));
#258647=CARTESIAN_POINT('Ctrl Pts',(-42.5424617625837,-57.8468004016288,
-39.1511256797657));
#258648=CARTESIAN_POINT('Ctrl Pts',(-42.5490019659384,-57.8785814507583,
-39.159052225872));
#258649=CARTESIAN_POINT('Ctrl Pts',(-42.5626174009892,-57.9447434317856,
-39.1755537576797));
#258650=CARTESIAN_POINT('Ctrl Pts',(-42.5795086601173,-58.0098893460482,
-39.1924961709041));
#258651=CARTESIAN_POINT('Ctrl Pts',(-42.5996267529072,-58.0740282937004,
-39.2098669200529));
#258652=CARTESIAN_POINT('Origin',(-44.5079524583206,-57.475452478349,235.35105));
#258653=CARTESIAN_POINT('Ctrl Pts',(-44.5079524583204,-59.475452478349,
-40.0499499999999));
#258654=CARTESIAN_POINT('Ctrl Pts',(-44.6760170471088,-59.475452478349,
-40.058440311863));
#258655=CARTESIAN_POINT('Ctrl Pts',(-44.8437184416945,-59.454274826314,
-40.067529957345));
#258656=CARTESIAN_POINT('Ctrl Pts',(-45.2594552607162,-59.3471207622369,
-40.0916575385967));
#258657=CARTESIAN_POINT('Ctrl Pts',(-45.496644407017,-59.2333984614142,
-40.1069567955656));
#258658=CARTESIAN_POINT('Ctrl Pts',(-45.9176156971467,-58.9187425694116,
-40.1374009492541));
#258659=CARTESIAN_POINT('Ctrl Pts',(-46.0962927130596,-58.7194235547151,
-40.1522408525492));
#258660=CARTESIAN_POINT('Ctrl Pts',(-46.3597901723978,-58.2723890083923,
-40.1785907639449));
#258661=CARTESIAN_POINT('Ctrl Pts',(-46.4459283624828,-58.0311157161805,
-40.1925363111265));
#258662=CARTESIAN_POINT('Ctrl Pts',(-46.5247792217884,-57.5194806295679,
-40.2223816911789));
#258663=CARTESIAN_POINT('Ctrl Pts',(-46.5130120601188,-57.25347877823,-40.2378984658403));
#258664=CARTESIAN_POINT('Ctrl Pts',(-46.3876509989154,-56.7441882232003,
-40.2676070815504));
#258665=CARTESIAN_POINT('Ctrl Pts',(-46.2764125732784,-56.5056369266457,
-40.280563622792));
#258666=CARTESIAN_POINT('Ctrl Pts',(-45.9709302364628,-56.0877642162817,
-40.3081839789162));
#258667=CARTESIAN_POINT('Ctrl Pts',(-45.7808172794246,-55.9115589358159,
-40.3229274542022));
#258668=CARTESIAN_POINT('Ctrl Pts',(-45.3357905484516,-55.6353556244966,
-40.3534653106215));
#258669=CARTESIAN_POINT('Ctrl Pts',(-45.0830257677249,-55.541391309908,
-40.3689751452056));
#258670=CARTESIAN_POINT('Ctrl Pts',(-44.5678032257904,-55.4602065065838,
-40.3973711242144));
#258671=CARTESIAN_POINT('Ctrl Pts',(-44.3111368282405,-55.4689461400547,
-40.409702993038));
#258672=CARTESIAN_POINT('Ctrl Pts',(-43.8096122890819,-55.5834047199034,
-40.4383774594563));
#258673=CARTESIAN_POINT('Ctrl Pts',(-43.5699698324844,-55.6900407660986,
-40.4535939706926));
#258674=CARTESIAN_POINT('Ctrl Pts',(-43.1406185437216,-55.991989266126,
-40.4840908341309));
#258675=CARTESIAN_POINT('Ctrl Pts',(-42.9562192264815,-56.1860972069512,
-40.4990678278399));
#258676=CARTESIAN_POINT('Ctrl Pts',(-42.6801324996151,-56.6250040775835,
-40.525816668515));
#258677=CARTESIAN_POINT('Ctrl Pts',(-42.5871730365578,-56.8631930866537,
-40.5392348688177));
#258678=CARTESIAN_POINT('Ctrl Pts',(-42.4934537579717,-57.3710008542222,
-40.5688569885925));
#258679=CARTESIAN_POINT('Ctrl Pts',(-42.4971800063187,-57.6364236424564,
-40.5843399845728));
#258680=CARTESIAN_POINT('Ctrl Pts',(-42.6071199604835,-58.1507508500168,
-40.6143424050137));
#258681=CARTESIAN_POINT('Ctrl Pts',(-42.7122907149391,-58.3945581559768,
-40.6277104088922));
#258682=CARTESIAN_POINT('Ctrl Pts',(-43.0070601563209,-58.8219102326021,
-40.6550660508894));
#258683=CARTESIAN_POINT('Ctrl Pts',(-43.1916614582763,-59.0028573575633,
-40.6696693913629));
#258684=CARTESIAN_POINT('Ctrl Pts',(-43.6274028185405,-59.2907998889782,
-40.7000805619648));
#258685=CARTESIAN_POINT('Ctrl Pts',(-43.8765775868587,-59.3917624882435,
-40.7156131524052));
#258686=CARTESIAN_POINT('Ctrl Pts',(-44.2604122311971,-59.4639653632714,
-40.7371096851764));
#258687=CARTESIAN_POINT('Ctrl Pts',(-44.3841812462878,-59.475452478349,
-40.7436973075237));
#258688=CARTESIAN_POINT('Ctrl Pts',(-44.5079524583206,-59.475452478349,
-40.7499499999999));
#258689=CARTESIAN_POINT('',(-46.2909969405137,-58.3814064003432,-40.0133527207719));
#258690=CARTESIAN_POINT('Ctrl Pts',(-44.5079524583206,-59.475452478349,
-40.5912000000001));
#258691=CARTESIAN_POINT('Ctrl Pts',(-44.3712894750723,-59.475452478349,
-40.5842960391105));
#258692=CARTESIAN_POINT('Ctrl Pts',(-44.2346952893026,-59.4614482703518,
-40.5769870976757));
#258693=CARTESIAN_POINT('Ctrl Pts',(-43.8401496223421,-59.3793023154099,
-40.5546594573751));
#258694=CARTESIAN_POINT('Ctrl Pts',(-43.5934164424196,-59.2738427846152,
-40.539119050957));
#258695=CARTESIAN_POINT('Ctrl Pts',(-43.1638937079193,-58.978402858688,
-40.5088033598087));
#258696=CARTESIAN_POINT('Ctrl Pts',(-42.9829501165407,-58.7944530350421,
-40.4942972213898));
#258697=CARTESIAN_POINT('Ctrl Pts',(-42.6952377625678,-58.3609299758541,
-40.4671181033913));
#258698=CARTESIAN_POINT('Ctrl Pts',(-42.5941044680215,-58.1136062477262,
-40.4534256365473));
#258699=CARTESIAN_POINT('Ctrl Pts',(-42.4944238939425,-57.5960599864837,
-40.4232354379748));
#258700=CARTESIAN_POINT('Ctrl Pts',(-42.4959830199083,-57.331149200749,
-40.4077823088069));
#258701=CARTESIAN_POINT('Ctrl Pts',(-42.599471521949,-56.8259352812586,
-40.3783114968366));
#258702=CARTESIAN_POINT('Ctrl Pts',(-42.6969737399032,-56.5897443279571,
-40.3651874708724));
#258703=CARTESIAN_POINT('Ctrl Pts',(-42.9814317908889,-56.1563383945309,
-40.3381761704037));
#258704=CARTESIAN_POINT('Ctrl Pts',(-43.1695715019011,-55.9658105643254,
-40.3231146388194));
#258705=CARTESIAN_POINT('Ctrl Pts',(-43.6043129843349,-55.6724854920117,
-40.292596989418));
#258706=CARTESIAN_POINT('Ctrl Pts',(-43.8454807836701,-55.5706149980718,
-40.2774424159648));
#258707=CARTESIAN_POINT('Ctrl Pts',(-44.3492069523885,-55.4654949802471,
-40.248929102023));
#258708=CARTESIAN_POINT('Ctrl Pts',(-44.6066546508642,-55.461653859112,
-40.2366162077022));
#258709=CARTESIAN_POINT('Ctrl Pts',(-45.120303738751,-55.5529418352898,
-40.2080050408038));
#258710=CARTESIAN_POINT('Ctrl Pts',(-45.3707162471246,-55.6515462973986,
-40.1924787010278));
#258711=CARTESIAN_POINT('Ctrl Pts',(-45.8096388792983,-55.935542744414,
-40.1620219125873));
#258712=CARTESIAN_POINT('Ctrl Pts',(-45.9961215501845,-56.1149012768774,
-40.1473698627865));
#258713=CARTESIAN_POINT('Ctrl Pts',(-46.2945361068356,-56.5390431049575,
-40.1199237085639));
#258714=CARTESIAN_POINT('Ctrl Pts',(-46.4017791757504,-56.7810506455932,
-40.1067067735774));
#258715=CARTESIAN_POINT('Ctrl Pts',(-46.5104850354038,-57.2647523638798,
-40.0784908400107));
#258716=CARTESIAN_POINT('Ctrl Pts',(-46.5213905146943,-57.4997997300255,
-40.0647797436521));
#258717=CARTESIAN_POINT('Ctrl Pts',(-46.462284513203,-57.9578859173332,
-40.0380580493925));
#258718=CARTESIAN_POINT('Ctrl Pts',(-46.394478244912,-58.1777405942362,
-40.0252331932399));
#258719=CARTESIAN_POINT('Ctrl Pts',(-46.2909969103393,-58.3814063856342,
-40.0133526887417));
#258720=CARTESIAN_POINT('',(-44.6028144957888,-59.4732020054856,-39.8960583336497));
#258721=CARTESIAN_POINT('Ctrl Pts',(-44.6028145367817,-59.4732017575571,
-39.896058052999));
#258722=CARTESIAN_POINT('Ctrl Pts',(-44.6309237118345,-59.4718673393062,
-39.9013440349211));
#258723=CARTESIAN_POINT('Ctrl Pts',(-44.6590015032546,-59.4699391376493,
-39.9065030818641));
#258724=CARTESIAN_POINT('Ctrl Pts',(-44.7195562226364,-59.4644947877976,
-39.9173708456776));
#258725=CARTESIAN_POINT('Ctrl Pts',(-44.7520254641284,-59.4607736709145,
-39.9230368121193));
#258726=CARTESIAN_POINT('Ctrl Pts',(-44.8168752155214,-59.4517213309666,
-39.9340284833551));
#258727=CARTESIAN_POINT('Ctrl Pts',(-44.8492557303708,-59.4463901948908,
-39.9393542053395));
#258728=CARTESIAN_POINT('Ctrl Pts',(-44.9139264543873,-59.4340919253905,
-39.9496609938934));
#258729=CARTESIAN_POINT('Ctrl Pts',(-44.946215463264,-59.4271242954454,
-39.9546417246475));
#258730=CARTESIAN_POINT('Ctrl Pts',(-45.0107056952338,-59.411516304601,
-39.9642527707462));
#258731=CARTESIAN_POINT('Ctrl Pts',(-45.0429448249416,-59.4028563587456,
-39.9688866673414));
#258732=CARTESIAN_POINT('Ctrl Pts',(-45.1065152212723,-59.3840690317117,
-39.9776842198647));
#258733=CARTESIAN_POINT('Ctrl Pts',(-45.1380045334646,-59.373905450928,
-39.981871837324));
#258734=CARTESIAN_POINT('Ctrl Pts',(-45.200302444735,-59.3520826555279,
-39.9898169453504));
#258735=CARTESIAN_POINT('Ctrl Pts',(-45.2311273685557,-59.3404195858245,
-39.9935768864381));
#258736=CARTESIAN_POINT('Ctrl Pts',(-45.32263664318,-59.3031909081966,-40.0042245496825));
#258737=CARTESIAN_POINT('Ctrl Pts',(-45.3823576994497,-59.2753909454431,
-40.0104815827663));
#258738=CARTESIAN_POINT('Ctrl Pts',(-45.4699947035294,-59.2291813824217,
-40.0185985839041));
#258739=CARTESIAN_POINT('Ctrl Pts',(-45.4988824306035,-59.2130254047437,
-40.0210924810235));
#258740=CARTESIAN_POINT('Ctrl Pts',(-45.5559983886489,-59.1791841401258,
-40.0256506619548));
#258741=CARTESIAN_POINT('Ctrl Pts',(-45.5842159038049,-59.161505654346,
-40.0277141794724));
#258742=CARTESIAN_POINT('Ctrl Pts',(-45.6260683484526,-59.1337942848195,
-40.0304825527898));
#258743=CARTESIAN_POINT('Ctrl Pts',(-45.639937085558,-59.1243584137232,
-40.0313502886864));
#258744=CARTESIAN_POINT('Ctrl Pts',(-45.6673408070756,-59.1052063125898,
-40.0329654356527));
#258745=CARTESIAN_POINT('Ctrl Pts',(-45.6809062118534,-59.0954702890689,
-40.0337149272658));
#258746=CARTESIAN_POINT('Ctrl Pts',(-45.721141509693,-59.0658238467719,
-40.0357872710599));
#258747=CARTESIAN_POINT('Ctrl Pts',(-45.7474017250148,-59.0454416887883,
-40.0369374935097));
#258748=CARTESIAN_POINT('Ctrl Pts',(-45.8244369758231,-58.9825233897898,
-40.0396997359252));
#258749=CARTESIAN_POINT('Ctrl Pts',(-45.8735338613848,-58.9381770793581,
-40.0406290361817));
#258750=CARTESIAN_POINT('Ctrl Pts',(-45.9672017588149,-58.844746856131,
-40.0406755331895));
#258751=CARTESIAN_POINT('Ctrl Pts',(-46.0117880585293,-58.7956402330911,
-40.0397912781262));
#258752=CARTESIAN_POINT('Ctrl Pts',(-46.0751829525158,-58.7183959597934,
-40.03708141461));
#258753=CARTESIAN_POINT('Ctrl Pts',(-46.0957687894685,-58.6919898183277,
-40.0359425033221));
#258754=CARTESIAN_POINT('Ctrl Pts',(-46.1356388662634,-58.6381045244638,
-40.0331996147473));
#258755=CARTESIAN_POINT('Ctrl Pts',(-46.1547846879949,-58.6108153057907,
-40.0316057182764));
#258756=CARTESIAN_POINT('Ctrl Pts',(-46.191608467482,-58.5554560068352,
-40.0279771039652));
#258757=CARTESIAN_POINT('Ctrl Pts',(-46.209273608015,-58.5274033537027,
-40.025943288199));
#258758=CARTESIAN_POINT('Ctrl Pts',(-46.2431323556178,-58.4705630466323,
-40.0214426044335));
#258759=CARTESIAN_POINT('Ctrl Pts',(-46.2593259282838,-58.441775375496,
-40.0189757265311));
#258760=CARTESIAN_POINT('Ctrl Pts',(-46.2802839458637,-58.4022634681017,
-40.0153404975323));
#258761=CARTESIAN_POINT('Ctrl Pts',(-46.2856865831931,-58.3918579776286,
-40.0143602145261));
#258762=CARTESIAN_POINT('Ctrl Pts',(-46.2909969450817,-58.3814064047113,
-40.0133526947335));
#258763=CARTESIAN_POINT('Ctrl Pts',(-44.6028144943784,-59.4732015101633,
-39.8960579076686));
#258764=CARTESIAN_POINT('Ctrl Pts',(-44.5712018647696,-59.4747026188422,
-39.8944171138134));
#258765=CARTESIAN_POINT('Ctrl Pts',(-44.539572771046,-59.475452478349,-39.8927973996557));
#258766=CARTESIAN_POINT('Ctrl Pts',(-44.5079524583206,-59.475452478349,
-39.8912000000002));
#258767=CARTESIAN_POINT('Ctrl Pts',(-43.4805771074156,-59.5712767529309,
-39.2399080357013));
#258768=CARTESIAN_POINT('Ctrl Pts',(-43.4150727209207,-59.5358440364426,
-39.2223070534893));
#258769=CARTESIAN_POINT('Ctrl Pts',(-43.2883193276586,-59.4590682572254,
-39.1867578392588));
#258770=CARTESIAN_POINT('Ctrl Pts',(-43.1106712693135,-59.32658002426,-39.1324031814995));
#258771=CARTESIAN_POINT('Ctrl Pts',(-43.0005921597408,-59.2266373021163,
-39.0954660506179));
#258772=CARTESIAN_POINT('Ctrl Pts',(-42.8948534568781,-59.1207134074407,
-39.0581733199915));
#258773=CARTESIAN_POINT('Ctrl Pts',(-42.7951360401793,-59.0104958554849,
-39.0211184761739));
#258774=CARTESIAN_POINT('Ctrl Pts',(-42.6850011896347,-58.8622904152127,
-38.9753582681256));
#258775=CARTESIAN_POINT('Ctrl Pts',(-42.6055727997797,-58.7375004045667,
-38.939089851323));
#258776=CARTESIAN_POINT('Ctrl Pts',(-42.5503788594446,-58.6407591922129,
-38.9120596161462));
#258777=CARTESIAN_POINT('Ctrl Pts',(-42.5165536369311,-58.5741539171446,
-38.8941613358138));
#258778=CARTESIAN_POINT('Ctrl Pts',(-42.4842288567228,-58.5064298632496,
-38.8763157156907));
#258779=CARTESIAN_POINT('Ctrl Pts',(-42.4689425396028,-58.4722695523732,
-38.8674882509199));
#258780=CARTESIAN_POINT('Ctrl Pts',(-42.4257123024776,-58.3690064948315,
-38.8413136266604));
#258781=CARTESIAN_POINT('Ctrl Pts',(-42.3750272156063,-58.229152189777,
-38.8072100415055));
#258782=CARTESIAN_POINT('Ctrl Pts',(-42.3380647902547,-58.0850119200902,
-38.7746901633276));
#258783=CARTESIAN_POINT('Ctrl Pts',(-42.3155659796374,-57.9752818499468,
-38.7509105250088));
#258784=CARTESIAN_POINT('Ctrl Pts',(-42.3089374211558,-57.9384266221928,
-38.7430843922672));
#258785=CARTESIAN_POINT('Ctrl Pts',(-42.297458012674,-57.864178756387,-38.7276438637217));
#258786=CARTESIAN_POINT('Ctrl Pts',(-42.292601515188,-57.8267325312259,
-38.720018782004));
#258787=CARTESIAN_POINT('Ctrl Pts',(-42.2847289916893,-57.7514526301959,
-38.7050196673963));
#258788=CARTESIAN_POINT('Ctrl Pts',(-42.2817363521424,-57.7138759968928,
-38.6976962453237));
#258789=CARTESIAN_POINT('Ctrl Pts',(-42.277596992864,-57.6387184974263,
-38.6833720377019));
#258790=CARTESIAN_POINT('Ctrl Pts',(-42.2741651307842,-57.5260409596698,
-38.6623829091612));
#258791=CARTESIAN_POINT('Ctrl Pts',(-42.2805893100654,-57.3760354719141,
-38.6363740800325));
#258792=CARTESIAN_POINT('Ctrl Pts',(-42.2937061680812,-57.2637038035873,
-38.618370061439));
#258793=CARTESIAN_POINT('Ctrl Pts',(-42.3043247017591,-57.1888547452426,
-38.6067079534822));
#258794=CARTESIAN_POINT('Ctrl Pts',(-42.3105743117123,-57.1514345461221,
-38.6010450635964));
#258795=CARTESIAN_POINT('Ctrl Pts',(-42.3249704170347,-57.0766935209607,
-38.590076215021));
#258796=CARTESIAN_POINT('Ctrl Pts',(-42.3331592025312,-57.0392159768686,
-38.5847494243559));
#258797=CARTESIAN_POINT('Ctrl Pts',(-42.3512949844302,-56.9651221381903,
-38.5745673038812));
#258798=CARTESIAN_POINT('Ctrl Pts',(-42.3712216906218,-56.8916587034686,
-38.564820665347));
#258799=CARTESIAN_POINT('Ctrl Pts',(-42.4063979707918,-56.7834465224234,
-38.5515118436));
#258800=CARTESIAN_POINT('Ctrl Pts',(-42.4468320479729,-56.6771725078319,
-38.5395042677724));
#258801=CARTESIAN_POINT('Ctrl Pts',(-42.4925290654744,-56.5728473165674,
-38.5288039137004));
#258802=CARTESIAN_POINT('Ctrl Pts',(-42.5265325119253,-56.5046058456765,
-38.5225509073062));
#258803=CARTESIAN_POINT('Ctrl Pts',(-42.5623338475306,-56.4370293947697,
-38.5167461666044));
#258804=CARTESIAN_POINT('Ctrl Pts',(-42.5811223641794,-56.4035923099625,
-38.5140693065785));
#258805=CARTESIAN_POINT('Ctrl Pts',(-42.620584523009,-56.3373241998654,
-38.5091697400817));
#258806=CARTESIAN_POINT('Ctrl Pts',(-42.6411082254821,-56.3047465904101,
-38.5069659500128));
#258807=CARTESIAN_POINT('Ctrl Pts',(-42.7048067991197,-56.2090283357163,
-38.501110858935));
#258808=CARTESIAN_POINT('Ctrl Pts',(-42.7502234543428,-56.1476408662828,
-38.4981890389281));
#258809=CARTESIAN_POINT('Ctrl Pts',(-42.8467942323831,-56.0297655581676,
-38.4942910511033));
#258810=CARTESIAN_POINT('Ctrl Pts',(-42.8979715413934,-55.9732420482176,
-38.4933125989996));
#258811=CARTESIAN_POINT('Ctrl Pts',(-42.9790570553347,-55.8921695883033,
-38.4933149859729));
#258812=CARTESIAN_POINT('Ctrl Pts',(-43.0068374106561,-55.8657400908868,
-38.4935622007431));
#258813=CARTESIAN_POINT('Ctrl Pts',(-43.0495800649421,-55.8270637749536,
-38.4943063068789));
#258814=CARTESIAN_POINT('Ctrl Pts',(-43.0640222060113,-55.8143203511958,
-38.494617152342));
#258815=CARTESIAN_POINT('Ctrl Pts',(-43.0932714774893,-55.7891564261061,
-38.4953646906773));
#258816=CARTESIAN_POINT('Ctrl Pts',(-43.1080901283632,-55.7767277938553,
-38.4958020036096));
#258817=CARTESIAN_POINT('Ctrl Pts',(-43.1528523310046,-55.7401327167866,
-38.4972962980169));
#258818=CARTESIAN_POINT('Ctrl Pts',(-43.2134913856688,-55.6930468850421,
-38.4997758707861));
#258819=CARTESIAN_POINT('Ctrl Pts',(-43.3385569247743,-55.6055389451161,
-38.5066450244003));
#258820=CARTESIAN_POINT('Ctrl Pts',(-43.4691986576013,-55.5278792007279,
-38.5163302992824));
#258821=CARTESIAN_POINT('Ctrl Pts',(-43.5713395927684,-55.4769743237494,
-38.5256877381308));
#258822=CARTESIAN_POINT('Ctrl Pts',(-43.6403672861995,-55.4446857735354,
-38.5323951500278));
#258823=CARTESIAN_POINT('Ctrl Pts',(-43.6753577685123,-55.4293620157832,
-38.5359845633874));
#258824=CARTESIAN_POINT('Ctrl Pts',(-43.7462462065788,-55.4003985583156,
-38.5436333065981));
#258825=CARTESIAN_POINT('Ctrl Pts',(-43.7822717759725,-55.3867204456352,
-38.5477088862383));
#258826=CARTESIAN_POINT('Ctrl Pts',(-43.8543821738219,-55.3613797848081,
-38.5562346427694));
#258827=CARTESIAN_POINT('Ctrl Pts',(-43.890622407919,-55.349649082917,-38.5607007444526));
#258828=CARTESIAN_POINT('Ctrl Pts',(-43.9997560709039,-55.3172704656441,
-38.5746802407103));
#258829=CARTESIAN_POINT('Ctrl Pts',(-44.1098017310836,-55.290468361793,
-38.5898286859852));
#258830=CARTESIAN_POINT('Ctrl Pts',(-44.2583166685835,-55.2656490138239,
-38.612301023075));
#258831=CARTESIAN_POINT('Ctrl Pts',(-44.3705972700495,-55.2524997368729,
-38.6302900391873));
#258832=CARTESIAN_POINT('Ctrl Pts',(-44.446056048267,-55.2474029004138,
-38.6430428201589));
#258833=CARTESIAN_POINT('Ctrl Pts',(-44.5218128020516,-55.2441636366351,
-38.65617756452));
#258834=CARTESIAN_POINT('Ctrl Pts',(-44.5599089424743,-55.2434808562086,
-38.6629497802385));
#258835=CARTESIAN_POINT('Ctrl Pts',(-44.6354869543582,-55.2439911084578,
-38.6767130108817));
#258836=CARTESIAN_POINT('Ctrl Pts',(-44.6731456892459,-55.2451740103824,
-38.6837342374529));
#258837=CARTESIAN_POINT('Ctrl Pts',(-44.7481014788608,-55.2493620066237,
-38.6980304684339));
#258838=CARTESIAN_POINT('Ctrl Pts',(-44.860046548974,-55.2583760573225,
-38.7198650218829));
#258839=CARTESIAN_POINT('Ctrl Pts',(-45.0073845433675,-55.2811507310277,
-38.7505067688753));
#258840=CARTESIAN_POINT('Ctrl Pts',(-45.1528189888476,-55.3146135839333,
-38.7826550300594));
#258841=CARTESIAN_POINT('Ctrl Pts',(-45.2248832056965,-55.3349380951144,
-38.7992310848652));
#258842=CARTESIAN_POINT('Ctrl Pts',(-45.2966462681613,-55.3570913336823,
-38.8160672125853));
#258843=CARTESIAN_POINT('Ctrl Pts',(-45.3323638946335,-55.3690863290504,
-38.8246135819642));
#258844=CARTESIAN_POINT('Ctrl Pts',(-45.4027951436545,-55.3946744461232,
-38.841798196801));
#258845=CARTESIAN_POINT('Ctrl Pts',(-45.4376370321487,-55.4083060218429,
-38.85046633842));
#258846=CARTESIAN_POINT('Ctrl Pts',(-45.5409345111852,-55.4516493275196,
-38.8766665754573));
#258847=CARTESIAN_POINT('Ctrl Pts',(-45.6082182891413,-55.4838201174091,
-38.8944064774514));
#258848=CARTESIAN_POINT('Ctrl Pts',(-45.7067749877369,-55.5369855856676,
-38.9214216121435));
#258849=CARTESIAN_POINT('Ctrl Pts',(-45.7392219877795,-55.5555212114618,
-38.9304915704334));
#258850=CARTESIAN_POINT('Ctrl Pts',(-45.8033556832395,-55.5942722159849,
-38.9487787872477));
#258851=CARTESIAN_POINT('Ctrl Pts',(-45.8348443691401,-55.6143675312756,
-38.9579395118015));
#258852=CARTESIAN_POINT('Ctrl Pts',(-45.9274099842789,-55.6766589025306,
-38.9854159162723));
#258853=CARTESIAN_POINT('Ctrl Pts',(-45.9867610865919,-55.7209353156014,
-39.0037703637879));
#258854=CARTESIAN_POINT('Ctrl Pts',(-46.1007337830098,-55.8148102393793,
-39.0405190865864));
#258855=CARTESIAN_POINT('Ctrl Pts',(-46.1826971388658,-55.889219933262,
-39.0681181728269));
#258856=CARTESIAN_POINT('Ctrl Pts',(-46.259356574729,-55.9696687352924,
-39.0957737179551));
#258857=CARTESIAN_POINT('Ctrl Pts',(-46.309266807939,-56.024663053365,-39.1142236413887));
#258858=CARTESIAN_POINT('Ctrl Pts',(-46.3336138177017,-56.0528284109483,
-39.1234510495426));
#258859=CARTESIAN_POINT('Ctrl Pts',(-46.3692509284248,-56.0961546965833,
-39.1373141736981));
#258860=CARTESIAN_POINT('Ctrl Pts',(-46.3809719555493,-56.1107655250657,
-39.14193505412));
#258861=CARTESIAN_POINT('Ctrl Pts',(-46.4039850968433,-56.1401806715041,
-39.1511314768264));
#258862=CARTESIAN_POINT('Ctrl Pts',(-46.4153001903629,-56.1550126624776,
-39.1557159133813));
#258863=CARTESIAN_POINT('Ctrl Pts',(-46.4486370096885,-56.1998310060263,
-39.1694131182659));
#258864=CARTESIAN_POINT('Ctrl Pts',(-46.4700835091466,-56.2301795317326,
-39.1784826054425));
#258865=CARTESIAN_POINT('Ctrl Pts',(-46.532071913686,-56.3225583984772,
-39.2054898733524));
#258866=CARTESIAN_POINT('Ctrl Pts',(-46.5894197348374,-56.4176636744323,
-39.23211607576));
#258867=CARTESIAN_POINT('Ctrl Pts',(-46.6566074362748,-56.5498680842415,
-39.2668544229849));
#258868=CARTESIAN_POINT('Ctrl Pts',(-46.6870820302515,-56.617790568625,
-39.2839693714534));
#258869=CARTESIAN_POINT('Ctrl Pts',(-46.7159729830272,-56.6866360545619,
-39.3009558869148));
#258870=CARTESIAN_POINT('Ctrl Pts',(-46.7296188023799,-56.7214992889704,
-39.3093799218186));
#258871=CARTESIAN_POINT('Ctrl Pts',(-46.7553216997643,-56.7922546384013,
-39.3261176641085));
#258872=CARTESIAN_POINT('Ctrl Pts',(-46.7672996943011,-56.8279354881579,
-39.3343809787628));
#258873=CARTESIAN_POINT('Ctrl Pts',(-46.8004530502947,-56.9353633959568,
-39.358737163018));
#258874=CARTESIAN_POINT('Ctrl Pts',(-46.8189795501832,-57.0077635587999,
-39.3744658121213));
#258875=CARTESIAN_POINT('Ctrl Pts',(-46.848916211803,-57.1540080946302,
-39.4048998290393));
#258876=CARTESIAN_POINT('Ctrl Pts',(-46.866048617508,-57.2647966217996,
-39.4269646939479));
#258877=CARTESIAN_POINT('Ctrl Pts',(-46.875074749658,-57.3772756893033,
-39.4478819384746));
#258878=CARTESIAN_POINT('Ctrl Pts',(-46.8792542953452,-57.4526370309597,
-39.4615663943076));
#258879=CARTESIAN_POINT('Ctrl Pts',(-46.8804258736835,-57.4905390832845,
-39.4682843608713));
#258880=CARTESIAN_POINT('Ctrl Pts',(-46.8808837743635,-57.566610437341,
-39.4814341960201));
#258881=CARTESIAN_POINT('Ctrl Pts',(-46.8801708637706,-57.604491394965,
-39.4878166677226));
#258882=CARTESIAN_POINT('Ctrl Pts',(-46.8768913879562,-57.6800597985945,
-39.5002231148134));
#258883=CARTESIAN_POINT('Ctrl Pts',(-46.8691896925243,-57.7930657109158,
-39.5182849936093));
#258884=CARTESIAN_POINT('Ctrl Pts',(-46.8479069711518,-57.9423669591112,
-39.540205996752));
#258885=CARTESIAN_POINT('Ctrl Pts',(-46.8236459543104,-58.053306681129,
-39.5550278422771));
#258886=CARTESIAN_POINT('Ctrl Pts',(-46.8055990109883,-58.1270324939452,
-39.5645447403379));
#258887=CARTESIAN_POINT('Ctrl Pts',(-46.7956339676918,-58.1637938532181,
-39.5691227921436));
#258888=CARTESIAN_POINT('Ctrl Pts',(-46.7738161327052,-58.2370162077019,
-39.5779016468881));
#258889=CARTESIAN_POINT('Ctrl Pts',(-46.7619036278491,-58.2736352268715,
-39.5821192203466));
#258890=CARTESIAN_POINT('Ctrl Pts',(-46.7364059718256,-58.3458255995332,
-39.5900871854462));
#258891=CARTESIAN_POINT('Ctrl Pts',(-46.7091836493705,-58.4171862986019,
-39.5976163356366));
#258892=CARTESIAN_POINT('Ctrl Pts',(-46.663274408039,-58.5216699086648,
-39.6076014242402));
#258893=CARTESIAN_POINT('Ctrl Pts',(-46.6123207377325,-58.6236436013082,
-39.616293729045));
#258894=CARTESIAN_POINT('Ctrl Pts',(-46.5563244858032,-58.7230996041114,
-39.6236943138341));
#258895=CARTESIAN_POINT('Ctrl Pts',(-46.515607032986,-58.7877140896312,
-39.6277619492082));
#258896=CARTESIAN_POINT('Ctrl Pts',(-46.4731710833873,-58.8514710047945,
-39.6313905635194));
#258897=CARTESIAN_POINT('Ctrl Pts',(-46.4511086137465,-58.8829006319494,
-39.6329844599904));
#258898=CARTESIAN_POINT('Ctrl Pts',(-46.4051673201274,-58.9449633016888,
-39.6357273485653));
#258899=CARTESIAN_POINT('Ctrl Pts',(-46.381447994276,-58.975377588932,-39.6368662598532));
#258900=CARTESIAN_POINT('Ctrl Pts',(-46.3084068909562,-59.0643493136614,
-39.6395761233691));
#258901=CARTESIAN_POINT('Ctrl Pts',(-46.2570407846102,-59.1209150453974,
-39.6404603784325));
#258902=CARTESIAN_POINT('Ctrl Pts',(-46.1491379755941,-59.228544463199,
-39.6404138814247));
#258903=CARTESIAN_POINT('Ctrl Pts',(-46.0925836555155,-59.2796343044913,
-39.6394845811684));
#258904=CARTESIAN_POINT('Ctrl Pts',(-46.0038529437629,-59.3521266125547,
-39.6367223387528));
#258905=CARTESIAN_POINT('Ctrl Pts',(-45.9736068078661,-59.3756113554055,
-39.6355721163029));
#258906=CARTESIAN_POINT('Ctrl Pts',(-45.9272656961273,-59.4097723546528,
-39.6334997725088));
#258907=CARTESIAN_POINT('Ctrl Pts',(-45.9116419215573,-59.4209912820171,
-39.6327502808957));
#258908=CARTESIAN_POINT('Ctrl Pts',(-45.8800804794677,-59.4430610802669,
-39.6311351339295));
#258909=CARTESIAN_POINT('Ctrl Pts',(-45.8321587971618,-59.4756823489919,
-39.628531354857));
#258910=CARTESIAN_POINT('Ctrl Pts',(-45.7834097108732,-59.5062438963941,
-39.6254355071979));
#258911=CARTESIAN_POINT('Ctrl Pts',(-45.717633106262,-59.5452481912826,
-39.6208773262667));
#258912=CARTESIAN_POINT('Ctrl Pts',(-45.6178307490054,-59.601113548897,
-39.6133952897297));
#258913=CARTESIAN_POINT('Ctrl Pts',(-45.4802897643185,-59.6652183443042,
-39.6008811885904));
#258914=CARTESIAN_POINT('Ctrl Pts',(-45.3738098009101,-59.7055766782111,
-39.5896017905935));
#258915=CARTESIAN_POINT('Ctrl Pts',(-45.3020778813705,-59.7307512119865,
-39.5816566825671));
#258916=CARTESIAN_POINT('Ctrl Pts',(-45.2658207311094,-59.7424779859237,
-39.5774690651077));
#258917=CARTESIAN_POINT('Ctrl Pts',(-45.1926264675053,-59.7641596016776,
-39.5686715125846));
#258918=CARTESIAN_POINT('Ctrl Pts',(-45.1555073907618,-59.7741562512684,
-39.5640376159893));
#258919=CARTESIAN_POINT('Ctrl Pts',(-45.0441315765335,-59.8011904590316,
-39.5496210468413));
#258920=CARTESIAN_POINT('Ctrl Pts',(-44.9324484012679,-59.8224577850013,
-39.5341534065747));
#258921=CARTESIAN_POINT('Ctrl Pts',(-44.8203079610257,-59.8353953605365,
-39.5171556909205));
#258922=CARTESIAN_POINT('Ctrl Pts',(-44.7080184564226,-59.8455760612675,
-39.4996502778008));
#258923=CARTESIAN_POINT('Ctrl Pts',(-44.6329372249224,-59.8486931621852,
-39.4873001861445));
#258924=CARTESIAN_POINT('Ctrl Pts',(-44.5200834441659,-59.8478515133141,
-39.4677634802869));
#258925=CARTESIAN_POINT('Ctrl Pts',(-44.4823810871712,-59.8466449718289,
-39.4610736497974));
#258926=CARTESIAN_POINT('Ctrl Pts',(-44.4258051079382,-59.8434394706745,
-39.4507883432074));
#258927=CARTESIAN_POINT('Ctrl Pts',(-44.4069254589855,-59.8421361346926,
-39.4473147915973));
#258928=CARTESIAN_POINT('Ctrl Pts',(-44.3691376542581,-59.8390581625153,
-39.4402793331445));
#258929=CARTESIAN_POINT('Ctrl Pts',(-44.3502459350849,-59.8372838734483,
-39.4367203104461));
#258930=CARTESIAN_POINT('Ctrl Pts',(-44.2562487381671,-59.8272835659938,
-39.4188041728073));
#258931=CARTESIAN_POINT('Ctrl Pts',(-44.1080045765469,-59.8040393501646,
-39.3892226636159));
#258932=CARTESIAN_POINT('Ctrl Pts',(-43.9639303529155,-59.7668593120831,
-39.3578670379715));
#258933=CARTESIAN_POINT('Ctrl Pts',(-43.8219159040518,-59.7227861654643,
-39.3256251231267));
#258934=CARTESIAN_POINT('Ctrl Pts',(-43.7519290534068,-59.6972943066161,
-39.3090578287531));
#258935=CARTESIAN_POINT('Ctrl Pts',(-43.665783177736,-59.6610675807531,
-39.2877890488175));
#258936=CARTESIAN_POINT('Ctrl Pts',(-43.6486106666635,-59.653596197985,
-39.2835041280971));
#258937=CARTESIAN_POINT('Ctrl Pts',(-43.6144193015916,-59.6382222359849,
-39.2748825183767));
#258938=CARTESIAN_POINT('Ctrl Pts',(-43.597366582891,-59.6303022352814,
-39.2705368924251));
#258939=CARTESIAN_POINT('Ctrl Pts',(-43.5465994182959,-59.605961903298,
-39.2574616452183));
#258940=CARTESIAN_POINT('Ctrl Pts',(-43.513329300663,-59.588993111175,-39.2487085268073));
#258941=CARTESIAN_POINT('Ctrl Pts',(-43.4805771074156,-59.5712767529309,
-39.2399080357013));
#258942=CARTESIAN_POINT('Ctrl Pts',(-43.8341420587998,-57.9817357678076,
-41.1268248734572));
#258943=CARTESIAN_POINT('Ctrl Pts',(-43.8090823387197,-57.9680163597508,
-41.1092238912453));
#258944=CARTESIAN_POINT('Ctrl Pts',(-43.7605654269547,-57.9383371077444,
-41.0736746770147));
#258945=CARTESIAN_POINT('Ctrl Pts',(-43.6924895655639,-57.8872515755908,
-41.019320019256));
#258946=CARTESIAN_POINT('Ctrl Pts',(-43.6502497090231,-57.8487916199066,
-40.9823828883729));
#258947=CARTESIAN_POINT('Ctrl Pts',(-43.6096433745973,-57.8080652293815,
-40.945090157748));
#258948=CARTESIAN_POINT('Ctrl Pts',(-43.5713160673933,-57.7657212262301,
-40.9080353139296));
#258949=CARTESIAN_POINT('Ctrl Pts',(-43.5288984657655,-57.7088609123343,
-40.8622751058818));
#258950=CARTESIAN_POINT('Ctrl Pts',(-43.4982484100127,-57.6610280687967,
-40.826006689079));
#258951=CARTESIAN_POINT('Ctrl Pts',(-43.4769169762936,-57.6239677344727,
-40.798976453902));
#258952=CARTESIAN_POINT('Ctrl Pts',(-43.4638199758968,-57.5984660781933,
-40.7810781735695));
#258953=CARTESIAN_POINT('Ctrl Pts',(-43.4512904535732,-57.5725430453748,
-40.7632325534464));
#258954=CARTESIAN_POINT('Ctrl Pts',(-43.4453582046716,-57.5594707895743,
-40.7544050886758));
#258955=CARTESIAN_POINT('Ctrl Pts',(-43.4285595200757,-57.5199648485381,
-40.7282304644163));
#258956=CARTESIAN_POINT('Ctrl Pts',(-43.4088016745783,-57.4664867157472,
-40.6941268792613));
#258957=CARTESIAN_POINT('Ctrl Pts',(-43.3942530508608,-57.4114223976644,
-40.6616070010832));
#258958=CARTESIAN_POINT('Ctrl Pts',(-43.3853242538269,-57.3695231591805,
-40.6378273627645));
#258959=CARTESIAN_POINT('Ctrl Pts',(-43.3826786150667,-57.3554536366825,
-40.630001230023));
#258960=CARTESIAN_POINT('Ctrl Pts',(-43.378062215599,-57.3271160344971,
-40.6145607014775));
#258961=CARTESIAN_POINT('Ctrl Pts',(-43.3760891270041,-57.3128275119467,
-40.60693561976));
#258962=CARTESIAN_POINT('Ctrl Pts',(-43.3728422231051,-57.2841093232557,
-40.5919365051523));
#258963=CARTESIAN_POINT('Ctrl Pts',(-43.3715781643254,-57.2697777029377,
-40.5846130830795));
#258964=CARTESIAN_POINT('Ctrl Pts',(-43.3697526802575,-57.2411194243864,
-40.5702888754578));
#258965=CARTESIAN_POINT('Ctrl Pts',(-43.3680717796799,-57.1981642741791,
-40.5492997469169));
#258966=CARTESIAN_POINT('Ctrl Pts',(-43.3700185838812,-57.1410182421193,
-40.5232909177883));
#258967=CARTESIAN_POINT('Ctrl Pts',(-43.3746384661022,-57.0982543712987,
-40.505286899195));
#258968=CARTESIAN_POINT('Ctrl Pts',(-43.3784319419536,-57.0697666559562,
-40.4936247912381));
#258969=CARTESIAN_POINT('Ctrl Pts',(-43.3806866868643,-57.0555278483981,
-40.4879619013523));
#258970=CARTESIAN_POINT('Ctrl Pts',(-43.3859186984709,-57.0270949764048,
-40.476993052777));
#258971=CARTESIAN_POINT('Ctrl Pts',(-43.3889115442249,-57.0128413374093,
-40.4716662621118));
#258972=CARTESIAN_POINT('Ctrl Pts',(-43.3955695423488,-56.984668670318,
-40.4614841416371));
#258973=CARTESIAN_POINT('Ctrl Pts',(-43.4029115329907,-56.9567427536229,
-40.4517375031029));
#258974=CARTESIAN_POINT('Ctrl Pts',(-43.4159439893498,-56.915628788467,
-40.4384286813559));
#258975=CARTESIAN_POINT('Ctrl Pts',(-43.4309850942545,-56.8752725380991,
-40.4264211055283));
#258976=CARTESIAN_POINT('Ctrl Pts',(-43.4480370013178,-56.8356780486645,
-40.4157207514563));
#258977=CARTESIAN_POINT('Ctrl Pts',(-43.4607570961379,-56.8097932355363,
-40.409467745062));
#258978=CARTESIAN_POINT('Ctrl Pts',(-43.4741642201056,-56.7841683331057,
-40.4036630043601));
#258979=CARTESIAN_POINT('Ctrl Pts',(-43.4812071336048,-56.7714928975767,
-40.4009861443346));
#258980=CARTESIAN_POINT('Ctrl Pts',(-43.4960130774609,-56.7463797512019,
-40.3960865778375));
#258981=CARTESIAN_POINT('Ctrl Pts',(-43.5037198572985,-56.7340380787953,
-40.3938827877695));
#258982=CARTESIAN_POINT('Ctrl Pts',(-43.527657505214,-56.6977883833479,
-40.3880276966888));
#258983=CARTESIAN_POINT('Ctrl Pts',(-43.5447483375558,-56.6745564757614,
-40.3851058766842));
#258984=CARTESIAN_POINT('Ctrl Pts',(-43.5811328114983,-56.629979998045,
-40.3812078888591));
#258985=CARTESIAN_POINT('Ctrl Pts',(-43.6004351631962,-56.6086219171049,
-40.3802294367552));
#258986=CARTESIAN_POINT('Ctrl Pts',(-43.6310475296952,-56.578014570072,
-40.3802318237287));
#258987=CARTESIAN_POINT('Ctrl Pts',(-43.6415402048873,-56.5680413281089,
-40.3804790384992));
#258988=CARTESIAN_POINT('Ctrl Pts',(-43.6576911458811,-56.5534539772523,
-40.3812231446347));
#258989=CARTESIAN_POINT('Ctrl Pts',(-43.6631494628181,-56.5486488515781,
-40.3815339900979));
#258990=CARTESIAN_POINT('Ctrl Pts',(-43.6742063152013,-56.5391628964206,
-40.3822815284329));
#258991=CARTESIAN_POINT('Ctrl Pts',(-43.6798092119243,-56.534479009001,
-40.3827188413654));
#258992=CARTESIAN_POINT('Ctrl Pts',(-43.6967370434146,-56.5206915949946,
-40.3842131357726));
#258993=CARTESIAN_POINT('Ctrl Pts',(-43.7196778600618,-56.5029622466235,
-40.386692708542));
#258994=CARTESIAN_POINT('Ctrl Pts',(-43.7670264629127,-56.4700551612604,
-40.3935618621563));
#258995=CARTESIAN_POINT('Ctrl Pts',(-43.8165352419067,-56.4409186299576,
-40.4032471370382));
#258996=CARTESIAN_POINT('Ctrl Pts',(-43.8552784957563,-56.4218759376155,
-40.4126045758866));
#258997=CARTESIAN_POINT('Ctrl Pts',(-43.8814691350842,-56.4098116142502,
-40.4193119877837));
#258998=CARTESIAN_POINT('Ctrl Pts',(-43.8947490665381,-56.4040935548973,
-40.4229014011429));
#258999=CARTESIAN_POINT('Ctrl Pts',(-43.9216608718689,-56.3933018151258,
-40.430550144354));
#259000=CARTESIAN_POINT('Ctrl Pts',(-43.9353412421961,-56.3882139347518,
-40.434625723994));
#259001=CARTESIAN_POINT('Ctrl Pts',(-43.9627318697344,-56.3788058930362,
-40.4431514805252));
#259002=CARTESIAN_POINT('Ctrl Pts',(-43.9765011076412,-56.3744602994329,
-40.4476175822086));
#259003=CARTESIAN_POINT('Ctrl Pts',(-44.0179764085085,-56.3624961934912,
-40.4615970784657));
#259004=CARTESIAN_POINT('Ctrl Pts',(-44.0598195105868,-56.3526585058303,
-40.4767455237411));
#259005=CARTESIAN_POINT('Ctrl Pts',(-44.1163310625808,-56.3437038269143,
-40.4992178608308));
#259006=CARTESIAN_POINT('Ctrl Pts',(-44.1590753545772,-56.3390714325247,
-40.5172068769433));
#259007=CARTESIAN_POINT('Ctrl Pts',(-44.1878153726385,-56.337382052278,
-40.5299596579145));
#259008=CARTESIAN_POINT('Ctrl Pts',(-44.2166756293141,-56.3364007867548,
-40.5430944022758));
#259009=CARTESIAN_POINT('Ctrl Pts',(-44.2311921171808,-56.3362675100036,
-40.5498666179945));
#259010=CARTESIAN_POINT('Ctrl Pts',(-44.2599977007373,-56.3367129587916,
-40.5636298486377));
#259011=CARTESIAN_POINT('Ctrl Pts',(-44.2743541649932,-56.3372884158027,
-40.5706510752088));
#259012=CARTESIAN_POINT('Ctrl Pts',(-44.3029357424357,-56.3391317429585,
-40.5849473061899));
#259013=CARTESIAN_POINT('Ctrl Pts',(-44.3456316213443,-56.3429350642169,
-40.6067818596389));
#259014=CARTESIAN_POINT('Ctrl Pts',(-44.4018650235691,-56.3520939287388,
-40.6374236066311));
#259015=CARTESIAN_POINT('Ctrl Pts',(-44.4574103376146,-56.3653147883305,
-40.6695718678152));
#259016=CARTESIAN_POINT('Ctrl Pts',(-44.4849466005937,-56.3732907222196,
-40.686147922621));
#259017=CARTESIAN_POINT('Ctrl Pts',(-44.512374392093,-56.3819617528141,
-40.7029840503412));
#259018=CARTESIAN_POINT('Ctrl Pts',(-44.5260289861432,-56.3866462995878,
-40.7115304197201));
#259019=CARTESIAN_POINT('Ctrl Pts',(-44.5529609776699,-56.3966203919845,
-40.7287150345567));
#259020=CARTESIAN_POINT('Ctrl Pts',(-44.5662873943758,-56.4019250012471,
-40.737383176176));
#259021=CARTESIAN_POINT('Ctrl Pts',(-44.6058068395674,-56.4187668411382,
-40.7635834132132));
#259022=CARTESIAN_POINT('Ctrl Pts',(-44.6315615859976,-56.4312362585519,
-40.7813233152079));
#259023=CARTESIAN_POINT('Ctrl Pts',(-44.6693071486035,-56.4518014713652,
-40.8083384498991));
#259024=CARTESIAN_POINT('Ctrl Pts',(-44.6817372625133,-56.458965010373,
-40.8174084081892));
#259025=CARTESIAN_POINT('Ctrl Pts',(-44.7063132537473,-56.473929075182,
-40.8356956250034));
#259026=CARTESIAN_POINT('Ctrl Pts',(-44.7183832523531,-56.4816832398284,
-40.8448563495594));
#259027=CARTESIAN_POINT('Ctrl Pts',(-44.7538754102704,-56.505703003501,
-40.8723327540241));
#259028=CARTESIAN_POINT('Ctrl Pts',(-44.7766465418209,-56.5227549736834,
-40.8906872015444));
#259029=CARTESIAN_POINT('Ctrl Pts',(-44.8204030914552,-56.5588699415109,
-40.9274359243417));
#259030=CARTESIAN_POINT('Ctrl Pts',(-44.851893062885,-56.5874690797881,
-40.9550350105826));
#259031=CARTESIAN_POINT('Ctrl Pts',(-44.8813802932551,-56.6183507815631,
-40.982690555711));
#259032=CARTESIAN_POINT('Ctrl Pts',(-44.9005867815582,-56.6394533348067,
-41.0011404791447));
#259033=CARTESIAN_POINT('Ctrl Pts',(-44.9099603095753,-56.6502571213647,
-41.0103678872986));
#259034=CARTESIAN_POINT('Ctrl Pts',(-44.9236872082217,-56.6668706184025,
-41.0242310114538));
#259035=CARTESIAN_POINT('Ctrl Pts',(-44.9282031316495,-56.6724722064122,
-41.0288518918758));
#259036=CARTESIAN_POINT('Ctrl Pts',(-44.9370720489983,-56.6837477093971,
-41.038048314582));
#259037=CARTESIAN_POINT('Ctrl Pts',(-44.9414338933841,-56.6894322363092,
-41.0426327511372));
#259038=CARTESIAN_POINT('Ctrl Pts',(-44.9542884395491,-56.7066066663578,
-41.0563299560217));
#259039=CARTESIAN_POINT('Ctrl Pts',(-44.9625629539304,-56.7182326826763,
-41.0653994431984));
#259040=CARTESIAN_POINT('Ctrl Pts',(-44.9864941991718,-56.7536111473724,
-41.0924067111081));
#259041=CARTESIAN_POINT('Ctrl Pts',(-45.0086645271567,-56.7900134244028,
-41.1190329135161));
#259042=CARTESIAN_POINT('Ctrl Pts',(-45.034704630644,-56.8405768845403,
-41.1537712607408));
#259043=CARTESIAN_POINT('Ctrl Pts',(-45.0465408860903,-56.8665423758261,
-41.1708862092094));
#259044=CARTESIAN_POINT('Ctrl Pts',(-45.0577761134165,-56.8928546179869,
-41.1878727246706));
#259045=CARTESIAN_POINT('Ctrl Pts',(-45.0630901582258,-56.906176087846,
-41.1962967595746));
#259046=CARTESIAN_POINT('Ctrl Pts',(-45.0731156002939,-56.9332061371524,
-41.2130345018643));
#259047=CARTESIAN_POINT('Ctrl Pts',(-45.0777961712447,-56.9468340019015,
-41.2212978165198));
#259048=CARTESIAN_POINT('Ctrl Pts',(-45.0907786540592,-56.9878560258786,
-41.2456540007716));
#259049=CARTESIAN_POINT('Ctrl Pts',(-45.0980724298404,-57.0154910056487,
-41.2613826498774));
#259050=CARTESIAN_POINT('Ctrl Pts',(-45.1099506000897,-57.0712899900431,
-41.2918166667949));
#259051=CARTESIAN_POINT('Ctrl Pts',(-45.1168338059478,-57.11354441615,-41.3138815317038));
#259052=CARTESIAN_POINT('Ctrl Pts',(-45.1206309792415,-57.1564190282566,
-41.3347987762303));
#259053=CARTESIAN_POINT('Ctrl Pts',(-45.1224627479043,-57.1851396939165,
-41.3484832320635));
#259054=CARTESIAN_POINT('Ctrl Pts',(-45.1230291819396,-57.199581674993,
-41.3552011986272));
#259055=CARTESIAN_POINT('Ctrl Pts',(-45.1234439819388,-57.2285619504273,
-41.3683510337761));
#259056=CARTESIAN_POINT('Ctrl Pts',(-45.1232917301137,-57.2429904040975,
-41.3747335054784));
#259057=CARTESIAN_POINT('Ctrl Pts',(-45.122279779691,-57.2717682086368,
-41.3871399525693));
#259058=CARTESIAN_POINT('Ctrl Pts',(-45.1196997436484,-57.3147947598186,
-41.4052018313649));
#259059=CARTESIAN_POINT('Ctrl Pts',(-45.1120557453653,-57.3716084168758,
-41.4271228345082));
#259060=CARTESIAN_POINT('Ctrl Pts',(-45.1031553338884,-57.4137999065974,
-41.4419446800329));
#259061=CARTESIAN_POINT('Ctrl Pts',(-45.09650693546,-57.4418330021969,-41.4514615780937));
#259062=CARTESIAN_POINT('Ctrl Pts',(-45.092823442876,-57.4558081403435,
-41.4560396298995));
#259063=CARTESIAN_POINT('Ctrl Pts',(-45.08473584999,-57.4836385233421,-41.464818484644));
#259064=CARTESIAN_POINT('Ctrl Pts',(-45.0803094818206,-57.4975537933777,
-41.4690360581021));
#259065=CARTESIAN_POINT('Ctrl Pts',(-45.0708158371377,-57.5249803724867,
-41.4770040232021));
#259066=CARTESIAN_POINT('Ctrl Pts',(-45.060662137239,-57.5520858826269,
-41.4845331733926));
#259067=CARTESIAN_POINT('Ctrl Pts',(-45.0434887903859,-57.591755117417,
-41.4945182619959));
#259068=CARTESIAN_POINT('Ctrl Pts',(-45.0243848727922,-57.6304534586566,
-41.5032105668009));
#259069=CARTESIAN_POINT('Ctrl Pts',(-45.0033512023575,-57.6681778817651,
-41.51061115159));
#259070=CARTESIAN_POINT('Ctrl Pts',(-44.9880328234845,-57.692673879575,
-41.5146787869643));
#259071=CARTESIAN_POINT('Ctrl Pts',(-44.9720568870916,-57.7168380825906,
-41.5183074012753));
#259072=CARTESIAN_POINT('Ctrl Pts',(-44.9637457009402,-57.7287466936453,
-41.5199012977462));
#259073=CARTESIAN_POINT('Ctrl Pts',(-44.9464287138105,-57.7522550306847,
-41.5226441863212));
#259074=CARTESIAN_POINT('Ctrl Pts',(-44.9374830238235,-57.7637718882179,
-41.5237830976086));
#259075=CARTESIAN_POINT('Ctrl Pts',(-44.9099214446927,-57.7974515399035,
-41.5264929611258));
#259076=CARTESIAN_POINT('Ctrl Pts',(-44.8905204729439,-57.8188493934961,
-41.5273772161885));
#259077=CARTESIAN_POINT('Ctrl Pts',(-44.8497318000032,-57.8595330722204,
-41.5273307191807));
#259078=CARTESIAN_POINT('Ctrl Pts',(-44.8283374647208,-57.878828810327,
-41.5264014189239));
#259079=CARTESIAN_POINT('Ctrl Pts',(-44.7947479986672,-57.9061820008563,
-41.5236391765087));
#259080=CARTESIAN_POINT('Ctrl Pts',(-44.7832945060713,-57.9150388128137,
-41.5224889540588));
#259081=CARTESIAN_POINT('Ctrl Pts',(-44.7657408175914,-57.9279147771907,
-41.5204166102647));
#259082=CARTESIAN_POINT('Ctrl Pts',(-44.7598217545323,-57.9321421746299,
-41.5196671186517));
#259083=CARTESIAN_POINT('Ctrl Pts',(-44.7478629508254,-57.9404557426351,
-41.5180519716851));
#259084=CARTESIAN_POINT('Ctrl Pts',(-44.7297025277655,-57.9527400844071,
-41.5154481926132));
#259085=CARTESIAN_POINT('Ctrl Pts',(-44.711220794734,-57.9642369190977,
-41.5123523449538));
#259086=CARTESIAN_POINT('Ctrl Pts',(-44.6862770262529,-57.9788987855805,
-41.5077941640223));
#259087=CARTESIAN_POINT('Ctrl Pts',(-44.6484202704456,-57.9998814948776,
-41.5003121274858));
#259088=CARTESIAN_POINT('Ctrl Pts',(-44.5962108390282,-58.0238874022289,
-41.4877980263462));
#259089=CARTESIAN_POINT('Ctrl Pts',(-44.5557649369164,-58.0389385823793,
-41.4765186283493));
#259090=CARTESIAN_POINT('Ctrl Pts',(-44.5285120653069,-58.048310487242,
-41.4685735203231));
#259091=CARTESIAN_POINT('Ctrl Pts',(-44.5147341086114,-58.0526671867402,
-41.4643859028639));
#259092=CARTESIAN_POINT('Ctrl Pts',(-44.4869140318333,-58.0607029371288,
-41.4555883503401));
#259093=CARTESIAN_POINT('Ctrl Pts',(-44.4728027150897,-58.0643973546439,
-41.4509544537452));
#259094=CARTESIAN_POINT('Ctrl Pts',(-44.4304531283686,-58.0743536715507,
-41.4365378845966));
#259095=CARTESIAN_POINT('Ctrl Pts',(-44.3879697631396,-58.0821103913619,
-41.4210702443308));
#259096=CARTESIAN_POINT('Ctrl Pts',(-44.3452880889881,-58.0866896268435,
-41.4040725286766));
#259097=CARTESIAN_POINT('Ctrl Pts',(-44.3025416355467,-58.090217180745,
-41.3865671155567));
#259098=CARTESIAN_POINT('Ctrl Pts',(-44.2739489581488,-58.0911687787978,
-41.3742170239002));
#259099=CARTESIAN_POINT('Ctrl Pts',(-44.2309555122234,-58.090491506171,
-41.3546803180427));
#259100=CARTESIAN_POINT('Ctrl Pts',(-44.2165895018292,-58.0899123697243,
-41.347990487553));
#259101=CARTESIAN_POINT('Ctrl Pts',(-44.1950278537333,-58.0885113544661,
-41.337705180963));
#259102=CARTESIAN_POINT('Ctrl Pts',(-44.1878319550126,-58.0879547296283,
-41.3342316293533));
#259103=CARTESIAN_POINT('Ctrl Pts',(-44.1734279164018,-58.0866616594573,
-41.3271961709002));
#259104=CARTESIAN_POINT('Ctrl Pts',(-44.1662260389348,-58.0859253983809,
-41.3236371482021));
#259105=CARTESIAN_POINT('Ctrl Pts',(-44.130389101081,-58.0818150523559,
-41.3057210105631));
#259106=CARTESIAN_POINT('Ctrl Pts',(-44.073848260417,-58.0724828543971,
-41.2761395013722));
#259107=CARTESIAN_POINT('Ctrl Pts',(-44.0188545174212,-58.0578491440998,
-41.2447838757269));
#259108=CARTESIAN_POINT('Ctrl Pts',(-43.9646246641704,-58.0405931079736,
-41.2125419608827));
#259109=CARTESIAN_POINT('Ctrl Pts',(-43.9378880325505,-58.0306505669816,
-41.1959746665064));
#259110=CARTESIAN_POINT('Ctrl Pts',(-43.9049634769563,-58.0165631445999,
-41.174705886574));
#259111=CARTESIAN_POINT('Ctrl Pts',(-43.898399460067,-58.0136596367661,
-41.1704209658528));
#259112=CARTESIAN_POINT('Ctrl Pts',(-43.8853286348063,-58.0076886655405,
-41.1617993561325));
#259113=CARTESIAN_POINT('Ctrl Pts',(-43.8788088737381,-58.0046144513738,
-41.157453730181));
#259114=CARTESIAN_POINT('Ctrl Pts',(-43.8593967360427,-57.9951717320096,
-41.1443784829743));
#259115=CARTESIAN_POINT('Ctrl Pts',(-43.8466719188398,-57.9885954718361,
-41.1356253645631));
#259116=CARTESIAN_POINT('Ctrl Pts',(-43.8341420587998,-57.9817357678076,
-41.1268248734572));
#259117=CARTESIAN_POINT('Ctrl Pts',(-45.9506478428458,-58.3141066664263,
-40.3575668188428));
#259118=CARTESIAN_POINT('Ctrl Pts',(-45.9187159875041,-58.4427318713764,
-40.3284662798477));
#259119=CARTESIAN_POINT('Ctrl Pts',(-45.8662597178432,-58.5652908169572,
-40.3027297091841));
#259120=CARTESIAN_POINT('Ctrl Pts',(-45.7408073320632,-58.7557683566169,
-40.2662627946592));
#259121=CARTESIAN_POINT('Ctrl Pts',(-45.6790009363265,-58.8279963011486,
-40.2535679867602));
#259122=CARTESIAN_POINT('Ctrl Pts',(-45.5604868254795,-58.9348862510393,
-40.2365559979816));
#259123=CARTESIAN_POINT('Ctrl Pts',(-45.5089640560027,-58.9738218628677,
-40.2309032397059));
#259124=CARTESIAN_POINT('Ctrl Pts',(-45.4511612750621,-59.0101321417087,
-40.2261786038362));
#259125=CARTESIAN_POINT('Ctrl Pts',(-45.4480371162561,-59.0120733533552,
-40.225927923055));
#259126=CARTESIAN_POINT('Ctrl Pts',(-45.4417466121093,-59.015939425046,
-40.2254324787861));
#259127=CARTESIAN_POINT('Ctrl Pts',(-45.4385803758859,-59.0178639115207,
-40.2251877908802));
#259128=CARTESIAN_POINT('Ctrl Pts',(-45.4289273025488,-59.0236663554915,
-40.2244558904502));
#259129=CARTESIAN_POINT('Ctrl Pts',(-45.4224008854538,-59.0275005455267,
-40.2239803627221));
#259130=CARTESIAN_POINT('Ctrl Pts',(-45.4091894470304,-59.0350866163115,
-40.2230553863648));
#259131=CARTESIAN_POINT('Ctrl Pts',(-45.4024735404165,-59.0388524512952,
-40.2226046964558));
#259132=CARTESIAN_POINT('Ctrl Pts',(-45.3308213216707,-59.0780782303883,
-40.2180000493414));
#259133=CARTESIAN_POINT('Ctrl Pts',(-45.2626750700944,-59.1071890367889,
-40.2153702456219));
#259134=CARTESIAN_POINT('Ctrl Pts',(-45.0546969823245,-59.1736287470141,
-40.2117346205805));
#259135=CARTESIAN_POINT('Ctrl Pts',(-44.910874640258,-59.192104560712,-40.2145478148852));
#259136=CARTESIAN_POINT('Ctrl Pts',(-44.6409196303305,-59.1827735438882,
-40.2265311750986));
#259137=CARTESIAN_POINT('Ctrl Pts',(-44.5382095666334,-59.1613643120583,
-40.233858657804));
#259138=CARTESIAN_POINT('Ctrl Pts',(-44.4689492302736,-59.1437418920634,
-40.2388225645965));
#259139=CARTESIAN_POINT('Ctrl Pts',(-43.4805771074156,-59.5712767529309,
-39.2399080357013));
#259140=CARTESIAN_POINT('Ctrl Pts',(-43.4150727209207,-59.5358440364426,
-39.2223070534893));
#259141=CARTESIAN_POINT('Ctrl Pts',(-43.2883193276586,-59.4590682572254,
-39.1867578392588));
#259142=CARTESIAN_POINT('Ctrl Pts',(-43.1106712693135,-59.32658002426,-39.1324031814995));
#259143=CARTESIAN_POINT('Ctrl Pts',(-43.0005921597408,-59.2266373021163,
-39.0954660506179));
#259144=CARTESIAN_POINT('Ctrl Pts',(-42.8948534568781,-59.1207134074407,
-39.0581733199915));
#259145=CARTESIAN_POINT('Ctrl Pts',(-42.7951360401793,-59.0104958554849,
-39.0211184761739));
#259146=CARTESIAN_POINT('Ctrl Pts',(-42.6850011896347,-58.8622904152127,
-38.9753582681256));
#259147=CARTESIAN_POINT('Ctrl Pts',(-42.6055727997797,-58.7375004045667,
-38.939089851323));
#259148=CARTESIAN_POINT('Ctrl Pts',(-42.5503788594446,-58.6407591922129,
-38.9120596161462));
#259149=CARTESIAN_POINT('Ctrl Pts',(-42.5165536369311,-58.5741539171446,
-38.8941613358138));
#259150=CARTESIAN_POINT('Ctrl Pts',(-42.4842288567228,-58.5064298632496,
-38.8763157156907));
#259151=CARTESIAN_POINT('Ctrl Pts',(-42.4689425396028,-58.4722695523732,
-38.8674882509199));
#259152=CARTESIAN_POINT('Ctrl Pts',(-42.4257123024776,-58.3690064948315,
-38.8413136266604));
#259153=CARTESIAN_POINT('Ctrl Pts',(-42.3750272156063,-58.229152189777,
-38.8072100415055));
#259154=CARTESIAN_POINT('Ctrl Pts',(-42.3380647902547,-58.0850119200902,
-38.7746901633276));
#259155=CARTESIAN_POINT('Ctrl Pts',(-42.3155659796374,-57.9752818499468,
-38.7509105250088));
#259156=CARTESIAN_POINT('Ctrl Pts',(-42.3089374211558,-57.9384266221928,
-38.7430843922672));
#259157=CARTESIAN_POINT('Ctrl Pts',(-42.297458012674,-57.864178756387,-38.7276438637217));
#259158=CARTESIAN_POINT('Ctrl Pts',(-42.292601515188,-57.8267325312259,
-38.720018782004));
#259159=CARTESIAN_POINT('Ctrl Pts',(-42.2847289916893,-57.7514526301959,
-38.7050196673963));
#259160=CARTESIAN_POINT('Ctrl Pts',(-42.2817363521424,-57.7138759968928,
-38.6976962453237));
#259161=CARTESIAN_POINT('Ctrl Pts',(-42.277596992864,-57.6387184974263,
-38.6833720377019));
#259162=CARTESIAN_POINT('Ctrl Pts',(-42.2741651307842,-57.5260409596698,
-38.6623829091612));
#259163=CARTESIAN_POINT('Ctrl Pts',(-42.2805893100654,-57.3760354719141,
-38.6363740800325));
#259164=CARTESIAN_POINT('Ctrl Pts',(-42.2937061680812,-57.2637038035873,
-38.618370061439));
#259165=CARTESIAN_POINT('Ctrl Pts',(-42.3043247017591,-57.1888547452426,
-38.6067079534822));
#259166=CARTESIAN_POINT('Ctrl Pts',(-42.3105743117123,-57.1514345461221,
-38.6010450635964));
#259167=CARTESIAN_POINT('Ctrl Pts',(-42.3249704170347,-57.0766935209607,
-38.590076215021));
#259168=CARTESIAN_POINT('Ctrl Pts',(-42.3331592025312,-57.0392159768686,
-38.5847494243559));
#259169=CARTESIAN_POINT('Ctrl Pts',(-42.3512949844302,-56.9651221381903,
-38.5745673038812));
#259170=CARTESIAN_POINT('Ctrl Pts',(-42.3712216906218,-56.8916587034686,
-38.564820665347));
#259171=CARTESIAN_POINT('Ctrl Pts',(-42.4063979707918,-56.7834465224234,
-38.5515118436));
#259172=CARTESIAN_POINT('Ctrl Pts',(-42.4468320479729,-56.6771725078319,
-38.5395042677724));
#259173=CARTESIAN_POINT('Ctrl Pts',(-42.4925290654744,-56.5728473165674,
-38.5288039137004));
#259174=CARTESIAN_POINT('Ctrl Pts',(-42.5265325119253,-56.5046058456765,
-38.5225509073062));
#259175=CARTESIAN_POINT('Ctrl Pts',(-42.5623338475306,-56.4370293947697,
-38.5167461666044));
#259176=CARTESIAN_POINT('Ctrl Pts',(-42.5811223641794,-56.4035923099625,
-38.5140693065785));
#259177=CARTESIAN_POINT('Ctrl Pts',(-42.620584523009,-56.3373241998654,
-38.5091697400817));
#259178=CARTESIAN_POINT('Ctrl Pts',(-42.6411082254821,-56.3047465904101,
-38.5069659500128));
#259179=CARTESIAN_POINT('Ctrl Pts',(-42.7048067991197,-56.2090283357163,
-38.501110858935));
#259180=CARTESIAN_POINT('Ctrl Pts',(-42.7502234543428,-56.1476408662828,
-38.4981890389281));
#259181=CARTESIAN_POINT('Ctrl Pts',(-42.8467942323831,-56.0297655581676,
-38.4942910511033));
#259182=CARTESIAN_POINT('Ctrl Pts',(-42.8979715413934,-55.9732420482176,
-38.4933125989996));
#259183=CARTESIAN_POINT('Ctrl Pts',(-42.9790570553347,-55.8921695883033,
-38.4933149859729));
#259184=CARTESIAN_POINT('Ctrl Pts',(-43.0068374106561,-55.8657400908868,
-38.4935622007431));
#259185=CARTESIAN_POINT('Ctrl Pts',(-43.0495800649421,-55.8270637749536,
-38.4943063068789));
#259186=CARTESIAN_POINT('Ctrl Pts',(-43.0640222060113,-55.8143203511958,
-38.494617152342));
#259187=CARTESIAN_POINT('Ctrl Pts',(-43.0932714774893,-55.7891564261061,
-38.4953646906773));
#259188=CARTESIAN_POINT('Ctrl Pts',(-43.1080901283632,-55.7767277938553,
-38.4958020036096));
#259189=CARTESIAN_POINT('Ctrl Pts',(-43.1528523310046,-55.7401327167866,
-38.4972962980169));
#259190=CARTESIAN_POINT('Ctrl Pts',(-43.2134913856688,-55.6930468850421,
-38.4997758707861));
#259191=CARTESIAN_POINT('Ctrl Pts',(-43.3385569247743,-55.6055389451161,
-38.5066450244003));
#259192=CARTESIAN_POINT('Ctrl Pts',(-43.4691986576013,-55.5278792007279,
-38.5163302992824));
#259193=CARTESIAN_POINT('Ctrl Pts',(-43.5713395927684,-55.4769743237494,
-38.5256877381308));
#259194=CARTESIAN_POINT('Ctrl Pts',(-43.6403672861995,-55.4446857735354,
-38.5323951500278));
#259195=CARTESIAN_POINT('Ctrl Pts',(-43.6753577685123,-55.4293620157832,
-38.5359845633874));
#259196=CARTESIAN_POINT('Ctrl Pts',(-43.7462462065788,-55.4003985583156,
-38.5436333065981));
#259197=CARTESIAN_POINT('Ctrl Pts',(-43.7822717759725,-55.3867204456352,
-38.5477088862383));
#259198=CARTESIAN_POINT('Ctrl Pts',(-43.8543821738219,-55.3613797848081,
-38.5562346427694));
#259199=CARTESIAN_POINT('Ctrl Pts',(-43.890622407919,-55.349649082917,-38.5607007444526));
#259200=CARTESIAN_POINT('Ctrl Pts',(-43.9997560709039,-55.3172704656441,
-38.5746802407103));
#259201=CARTESIAN_POINT('Ctrl Pts',(-44.1098017310836,-55.290468361793,
-38.5898286859852));
#259202=CARTESIAN_POINT('Ctrl Pts',(-44.2583166685835,-55.2656490138239,
-38.612301023075));
#259203=CARTESIAN_POINT('Ctrl Pts',(-44.3705972700495,-55.2524997368729,
-38.6302900391873));
#259204=CARTESIAN_POINT('Ctrl Pts',(-44.446056048267,-55.2474029004138,
-38.6430428201589));
#259205=CARTESIAN_POINT('Ctrl Pts',(-44.5218128020516,-55.2441636366351,
-38.65617756452));
#259206=CARTESIAN_POINT('Ctrl Pts',(-44.5599089424743,-55.2434808562086,
-38.6629497802385));
#259207=CARTESIAN_POINT('Ctrl Pts',(-44.6354869543582,-55.2439911084578,
-38.6767130108817));
#259208=CARTESIAN_POINT('Ctrl Pts',(-44.6731456892459,-55.2451740103824,
-38.6837342374529));
#259209=CARTESIAN_POINT('Ctrl Pts',(-44.7481014788608,-55.2493620066237,
-38.6980304684339));
#259210=CARTESIAN_POINT('Ctrl Pts',(-44.860046548974,-55.2583760573225,
-38.7198650218829));
#259211=CARTESIAN_POINT('Ctrl Pts',(-45.0073845433675,-55.2811507310277,
-38.7505067688753));
#259212=CARTESIAN_POINT('Ctrl Pts',(-45.1528189888476,-55.3146135839333,
-38.7826550300594));
#259213=CARTESIAN_POINT('Ctrl Pts',(-45.2248832056965,-55.3349380951144,
-38.7992310848652));
#259214=CARTESIAN_POINT('Ctrl Pts',(-45.2966462681613,-55.3570913336823,
-38.8160672125853));
#259215=CARTESIAN_POINT('Ctrl Pts',(-45.3323638946335,-55.3690863290504,
-38.8246135819642));
#259216=CARTESIAN_POINT('Ctrl Pts',(-45.4027951436545,-55.3946744461232,
-38.841798196801));
#259217=CARTESIAN_POINT('Ctrl Pts',(-45.4376370321487,-55.4083060218429,
-38.85046633842));
#259218=CARTESIAN_POINT('Ctrl Pts',(-45.5409345111852,-55.4516493275196,
-38.8766665754573));
#259219=CARTESIAN_POINT('Ctrl Pts',(-45.6082182891413,-55.4838201174091,
-38.8944064774514));
#259220=CARTESIAN_POINT('Ctrl Pts',(-45.7067749877369,-55.5369855856676,
-38.9214216121435));
#259221=CARTESIAN_POINT('Ctrl Pts',(-45.7392219877795,-55.5555212114618,
-38.9304915704334));
#259222=CARTESIAN_POINT('Ctrl Pts',(-45.8033556832395,-55.5942722159849,
-38.9487787872477));
#259223=CARTESIAN_POINT('Ctrl Pts',(-45.8348443691401,-55.6143675312756,
-38.9579395118015));
#259224=CARTESIAN_POINT('Ctrl Pts',(-45.9274099842789,-55.6766589025306,
-38.9854159162723));
#259225=CARTESIAN_POINT('Ctrl Pts',(-45.9867610865919,-55.7209353156014,
-39.0037703637879));
#259226=CARTESIAN_POINT('Ctrl Pts',(-46.1007337830098,-55.8148102393793,
-39.0405190865864));
#259227=CARTESIAN_POINT('Ctrl Pts',(-46.1826971388658,-55.889219933262,
-39.0681181728269));
#259228=CARTESIAN_POINT('Ctrl Pts',(-46.259356574729,-55.9696687352924,
-39.0957737179551));
#259229=CARTESIAN_POINT('Ctrl Pts',(-46.309266807939,-56.024663053365,-39.1142236413887));
#259230=CARTESIAN_POINT('Ctrl Pts',(-46.3336138177017,-56.0528284109483,
-39.1234510495426));
#259231=CARTESIAN_POINT('Ctrl Pts',(-46.3692509284248,-56.0961546965833,
-39.1373141736981));
#259232=CARTESIAN_POINT('Ctrl Pts',(-46.3809719555493,-56.1107655250657,
-39.14193505412));
#259233=CARTESIAN_POINT('Ctrl Pts',(-46.4039850968433,-56.1401806715041,
-39.1511314768264));
#259234=CARTESIAN_POINT('Ctrl Pts',(-46.4153001903629,-56.1550126624776,
-39.1557159133813));
#259235=CARTESIAN_POINT('Ctrl Pts',(-46.4486370096885,-56.1998310060263,
-39.1694131182659));
#259236=CARTESIAN_POINT('Ctrl Pts',(-46.4700835091466,-56.2301795317326,
-39.1784826054425));
#259237=CARTESIAN_POINT('Ctrl Pts',(-46.532071913686,-56.3225583984772,
-39.2054898733524));
#259238=CARTESIAN_POINT('Ctrl Pts',(-46.5894197348374,-56.4176636744323,
-39.23211607576));
#259239=CARTESIAN_POINT('Ctrl Pts',(-46.6566074362748,-56.5498680842415,
-39.2668544229849));
#259240=CARTESIAN_POINT('Ctrl Pts',(-46.6870820302515,-56.617790568625,
-39.2839693714534));
#259241=CARTESIAN_POINT('Ctrl Pts',(-46.7159729830272,-56.6866360545619,
-39.3009558869148));
#259242=CARTESIAN_POINT('Ctrl Pts',(-46.7296188023799,-56.7214992889704,
-39.3093799218186));
#259243=CARTESIAN_POINT('Ctrl Pts',(-46.7553216997643,-56.7922546384013,
-39.3261176641085));
#259244=CARTESIAN_POINT('Ctrl Pts',(-46.7672996943011,-56.8279354881579,
-39.3343809787628));
#259245=CARTESIAN_POINT('Ctrl Pts',(-46.8004530502947,-56.9353633959568,
-39.358737163018));
#259246=CARTESIAN_POINT('Ctrl Pts',(-46.8189795501832,-57.0077635587999,
-39.3744658121213));
#259247=CARTESIAN_POINT('Ctrl Pts',(-46.848916211803,-57.1540080946302,
-39.4048998290393));
#259248=CARTESIAN_POINT('Ctrl Pts',(-46.866048617508,-57.2647966217996,
-39.4269646939479));
#259249=CARTESIAN_POINT('Ctrl Pts',(-46.875074749658,-57.3772756893033,
-39.4478819384746));
#259250=CARTESIAN_POINT('Ctrl Pts',(-46.8792542953452,-57.4526370309597,
-39.4615663943076));
#259251=CARTESIAN_POINT('Ctrl Pts',(-46.8804258736835,-57.4905390832845,
-39.4682843608713));
#259252=CARTESIAN_POINT('Ctrl Pts',(-46.8808837743635,-57.566610437341,
-39.4814341960201));
#259253=CARTESIAN_POINT('Ctrl Pts',(-46.8801708637706,-57.604491394965,
-39.4878166677226));
#259254=CARTESIAN_POINT('Ctrl Pts',(-46.8768913879562,-57.6800597985945,
-39.5002231148134));
#259255=CARTESIAN_POINT('Ctrl Pts',(-46.8691896925243,-57.7930657109158,
-39.5182849936093));
#259256=CARTESIAN_POINT('Ctrl Pts',(-46.8479069711518,-57.9423669591112,
-39.540205996752));
#259257=CARTESIAN_POINT('Ctrl Pts',(-46.8236459543104,-58.053306681129,
-39.5550278422771));
#259258=CARTESIAN_POINT('Ctrl Pts',(-46.8055990109883,-58.1270324939452,
-39.5645447403379));
#259259=CARTESIAN_POINT('Ctrl Pts',(-46.7956339676918,-58.1637938532181,
-39.5691227921436));
#259260=CARTESIAN_POINT('Ctrl Pts',(-46.7738161327052,-58.2370162077019,
-39.5779016468881));
#259261=CARTESIAN_POINT('Ctrl Pts',(-46.7619036278491,-58.2736352268715,
-39.5821192203466));
#259262=CARTESIAN_POINT('Ctrl Pts',(-46.7364059718256,-58.3458255995332,
-39.5900871854462));
#259263=CARTESIAN_POINT('Ctrl Pts',(-46.7091836493705,-58.4171862986019,
-39.5976163356366));
#259264=CARTESIAN_POINT('Ctrl Pts',(-46.663274408039,-58.5216699086648,
-39.6076014242402));
#259265=CARTESIAN_POINT('Ctrl Pts',(-46.6123207377325,-58.6236436013082,
-39.616293729045));
#259266=CARTESIAN_POINT('Ctrl Pts',(-46.5563244858032,-58.7230996041114,
-39.6236943138341));
#259267=CARTESIAN_POINT('Ctrl Pts',(-46.515607032986,-58.7877140896312,
-39.6277619492082));
#259268=CARTESIAN_POINT('Ctrl Pts',(-46.4731710833873,-58.8514710047945,
-39.6313905635194));
#259269=CARTESIAN_POINT('Ctrl Pts',(-46.4511086137465,-58.8829006319494,
-39.6329844599904));
#259270=CARTESIAN_POINT('Ctrl Pts',(-46.4051673201274,-58.9449633016888,
-39.6357273485653));
#259271=CARTESIAN_POINT('Ctrl Pts',(-46.381447994276,-58.975377588932,-39.6368662598532));
#259272=CARTESIAN_POINT('Ctrl Pts',(-46.3084068909562,-59.0643493136614,
-39.6395761233691));
#259273=CARTESIAN_POINT('Ctrl Pts',(-46.2570407846102,-59.1209150453974,
-39.6404603784325));
#259274=CARTESIAN_POINT('Ctrl Pts',(-46.1491379755941,-59.228544463199,
-39.6404138814247));
#259275=CARTESIAN_POINT('Ctrl Pts',(-46.0925836555155,-59.2796343044913,
-39.6394845811684));
#259276=CARTESIAN_POINT('Ctrl Pts',(-46.0038529437629,-59.3521266125547,
-39.6367223387528));
#259277=CARTESIAN_POINT('Ctrl Pts',(-45.9736068078661,-59.3756113554055,
-39.6355721163029));
#259278=CARTESIAN_POINT('Ctrl Pts',(-45.9272656961273,-59.4097723546528,
-39.6334997725088));
#259279=CARTESIAN_POINT('Ctrl Pts',(-45.9116419215573,-59.4209912820171,
-39.6327502808957));
#259280=CARTESIAN_POINT('Ctrl Pts',(-45.8800804794677,-59.4430610802669,
-39.6311351339295));
#259281=CARTESIAN_POINT('Ctrl Pts',(-45.8321587971618,-59.4756823489919,
-39.628531354857));
#259282=CARTESIAN_POINT('Ctrl Pts',(-45.7834097108732,-59.5062438963941,
-39.6254355071979));
#259283=CARTESIAN_POINT('Ctrl Pts',(-45.717633106262,-59.5452481912826,
-39.6208773262667));
#259284=CARTESIAN_POINT('Ctrl Pts',(-45.6178307490054,-59.601113548897,
-39.6133952897297));
#259285=CARTESIAN_POINT('Ctrl Pts',(-45.4802897643185,-59.6652183443042,
-39.6008811885904));
#259286=CARTESIAN_POINT('Ctrl Pts',(-45.3738098009101,-59.7055766782111,
-39.5896017905935));
#259287=CARTESIAN_POINT('Ctrl Pts',(-45.3020778813705,-59.7307512119865,
-39.5816566825671));
#259288=CARTESIAN_POINT('Ctrl Pts',(-45.2658207311094,-59.7424779859237,
-39.5774690651077));
#259289=CARTESIAN_POINT('Ctrl Pts',(-45.1926264675053,-59.7641596016776,
-39.5686715125846));
#259290=CARTESIAN_POINT('Ctrl Pts',(-45.1555073907618,-59.7741562512684,
-39.5640376159893));
#259291=CARTESIAN_POINT('Ctrl Pts',(-45.0441315765335,-59.8011904590316,
-39.5496210468413));
#259292=CARTESIAN_POINT('Ctrl Pts',(-44.9324484012679,-59.8224577850013,
-39.5341534065747));
#259293=CARTESIAN_POINT('Ctrl Pts',(-44.8203079610257,-59.8353953605365,
-39.5171556909205));
#259294=CARTESIAN_POINT('Ctrl Pts',(-44.7080184564226,-59.8455760612675,
-39.4996502778008));
#259295=CARTESIAN_POINT('Ctrl Pts',(-44.6329372249224,-59.8486931621852,
-39.4873001861445));
#259296=CARTESIAN_POINT('Ctrl Pts',(-44.5200834441659,-59.8478515133141,
-39.4677634802869));
#259297=CARTESIAN_POINT('Ctrl Pts',(-44.4823810871712,-59.8466449718289,
-39.4610736497974));
#259298=CARTESIAN_POINT('Ctrl Pts',(-44.4258051079382,-59.8434394706745,
-39.4507883432074));
#259299=CARTESIAN_POINT('Ctrl Pts',(-44.4069254589855,-59.8421361346926,
-39.4473147915973));
#259300=CARTESIAN_POINT('Ctrl Pts',(-44.3691376542581,-59.8390581625153,
-39.4402793331445));
#259301=CARTESIAN_POINT('Ctrl Pts',(-44.3502459350849,-59.8372838734483,
-39.4367203104461));
#259302=CARTESIAN_POINT('Ctrl Pts',(-44.2562487381671,-59.8272835659938,
-39.4188041728073));
#259303=CARTESIAN_POINT('Ctrl Pts',(-44.1080045765469,-59.8040393501646,
-39.3892226636159));
#259304=CARTESIAN_POINT('Ctrl Pts',(-43.9639303529155,-59.7668593120831,
-39.3578670379715));
#259305=CARTESIAN_POINT('Ctrl Pts',(-43.8219159040518,-59.7227861654643,
-39.3256251231267));
#259306=CARTESIAN_POINT('Ctrl Pts',(-43.7519290534068,-59.6972943066161,
-39.3090578287531));
#259307=CARTESIAN_POINT('Ctrl Pts',(-43.665783177736,-59.6610675807531,
-39.2877890488175));
#259308=CARTESIAN_POINT('Ctrl Pts',(-43.6486106666635,-59.653596197985,
-39.2835041280971));
#259309=CARTESIAN_POINT('Ctrl Pts',(-43.6144193015916,-59.6382222359849,
-39.2748825183767));
#259310=CARTESIAN_POINT('Ctrl Pts',(-43.597366582891,-59.6303022352814,
-39.2705368924251));
#259311=CARTESIAN_POINT('Ctrl Pts',(-43.5465994182959,-59.605961903298,
-39.2574616452183));
#259312=CARTESIAN_POINT('Ctrl Pts',(-43.513329300663,-59.588993111175,-39.2487085268073));
#259313=CARTESIAN_POINT('Ctrl Pts',(-43.4805771074156,-59.5712767529309,
-39.2399080357013));
#259314=CARTESIAN_POINT('Ctrl Pts',(-43.8341420587998,-57.9817357678076,
-41.1268248734572));
#259315=CARTESIAN_POINT('Ctrl Pts',(-43.8090823387197,-57.9680163597508,
-41.1092238912453));
#259316=CARTESIAN_POINT('Ctrl Pts',(-43.7605654269547,-57.9383371077444,
-41.0736746770147));
#259317=CARTESIAN_POINT('Ctrl Pts',(-43.6924895655639,-57.8872515755908,
-41.019320019256));
#259318=CARTESIAN_POINT('Ctrl Pts',(-43.6502497090231,-57.8487916199066,
-40.9823828883729));
#259319=CARTESIAN_POINT('Ctrl Pts',(-43.6096433745973,-57.8080652293815,
-40.945090157748));
#259320=CARTESIAN_POINT('Ctrl Pts',(-43.5713160673933,-57.7657212262301,
-40.9080353139296));
#259321=CARTESIAN_POINT('Ctrl Pts',(-43.5288984657655,-57.7088609123343,
-40.8622751058818));
#259322=CARTESIAN_POINT('Ctrl Pts',(-43.4982484100127,-57.6610280687967,
-40.826006689079));
#259323=CARTESIAN_POINT('Ctrl Pts',(-43.4769169762936,-57.6239677344727,
-40.798976453902));
#259324=CARTESIAN_POINT('Ctrl Pts',(-43.4638199758968,-57.5984660781933,
-40.7810781735695));
#259325=CARTESIAN_POINT('Ctrl Pts',(-43.4512904535732,-57.5725430453748,
-40.7632325534464));
#259326=CARTESIAN_POINT('Ctrl Pts',(-43.4453582046716,-57.5594707895743,
-40.7544050886758));
#259327=CARTESIAN_POINT('Ctrl Pts',(-43.4285595200757,-57.5199648485381,
-40.7282304644163));
#259328=CARTESIAN_POINT('Ctrl Pts',(-43.4088016745783,-57.4664867157472,
-40.6941268792613));
#259329=CARTESIAN_POINT('Ctrl Pts',(-43.3942530508608,-57.4114223976644,
-40.6616070010832));
#259330=CARTESIAN_POINT('Ctrl Pts',(-43.3853242538269,-57.3695231591805,
-40.6378273627645));
#259331=CARTESIAN_POINT('Ctrl Pts',(-43.3826786150667,-57.3554536366825,
-40.630001230023));
#259332=CARTESIAN_POINT('Ctrl Pts',(-43.378062215599,-57.3271160344971,
-40.6145607014775));
#259333=CARTESIAN_POINT('Ctrl Pts',(-43.3760891270041,-57.3128275119467,
-40.60693561976));
#259334=CARTESIAN_POINT('Ctrl Pts',(-43.3728422231051,-57.2841093232557,
-40.5919365051523));
#259335=CARTESIAN_POINT('Ctrl Pts',(-43.3715781643254,-57.2697777029377,
-40.5846130830795));
#259336=CARTESIAN_POINT('Ctrl Pts',(-43.3697526802575,-57.2411194243864,
-40.5702888754578));
#259337=CARTESIAN_POINT('Ctrl Pts',(-43.3680717796799,-57.1981642741791,
-40.5492997469169));
#259338=CARTESIAN_POINT('Ctrl Pts',(-43.3700185838812,-57.1410182421193,
-40.5232909177883));
#259339=CARTESIAN_POINT('Ctrl Pts',(-43.3746384661022,-57.0982543712987,
-40.505286899195));
#259340=CARTESIAN_POINT('Ctrl Pts',(-43.3784319419536,-57.0697666559562,
-40.4936247912381));
#259341=CARTESIAN_POINT('Ctrl Pts',(-43.3806866868643,-57.0555278483981,
-40.4879619013523));
#259342=CARTESIAN_POINT('Ctrl Pts',(-43.3859186984709,-57.0270949764048,
-40.476993052777));
#259343=CARTESIAN_POINT('Ctrl Pts',(-43.3889115442249,-57.0128413374093,
-40.4716662621118));
#259344=CARTESIAN_POINT('Ctrl Pts',(-43.3955695423488,-56.984668670318,
-40.4614841416371));
#259345=CARTESIAN_POINT('Ctrl Pts',(-43.4029115329907,-56.9567427536229,
-40.4517375031029));
#259346=CARTESIAN_POINT('Ctrl Pts',(-43.4159439893498,-56.915628788467,
-40.4384286813559));
#259347=CARTESIAN_POINT('Ctrl Pts',(-43.4309850942545,-56.8752725380991,
-40.4264211055283));
#259348=CARTESIAN_POINT('Ctrl Pts',(-43.4480370013178,-56.8356780486645,
-40.4157207514563));
#259349=CARTESIAN_POINT('Ctrl Pts',(-43.4607570961379,-56.8097932355363,
-40.409467745062));
#259350=CARTESIAN_POINT('Ctrl Pts',(-43.4741642201056,-56.7841683331057,
-40.4036630043601));
#259351=CARTESIAN_POINT('Ctrl Pts',(-43.4812071336048,-56.7714928975767,
-40.4009861443346));
#259352=CARTESIAN_POINT('Ctrl Pts',(-43.4960130774609,-56.7463797512019,
-40.3960865778375));
#259353=CARTESIAN_POINT('Ctrl Pts',(-43.5037198572985,-56.7340380787953,
-40.3938827877695));
#259354=CARTESIAN_POINT('Ctrl Pts',(-43.527657505214,-56.6977883833479,
-40.3880276966888));
#259355=CARTESIAN_POINT('Ctrl Pts',(-43.5447483375558,-56.6745564757614,
-40.3851058766842));
#259356=CARTESIAN_POINT('Ctrl Pts',(-43.5811328114983,-56.629979998045,
-40.3812078888591));
#259357=CARTESIAN_POINT('Ctrl Pts',(-43.6004351631962,-56.6086219171049,
-40.3802294367552));
#259358=CARTESIAN_POINT('Ctrl Pts',(-43.6310475296952,-56.578014570072,
-40.3802318237287));
#259359=CARTESIAN_POINT('Ctrl Pts',(-43.6415402048873,-56.5680413281089,
-40.3804790384992));
#259360=CARTESIAN_POINT('Ctrl Pts',(-43.6576911458811,-56.5534539772523,
-40.3812231446347));
#259361=CARTESIAN_POINT('Ctrl Pts',(-43.6631494628181,-56.5486488515781,
-40.3815339900979));
#259362=CARTESIAN_POINT('Ctrl Pts',(-43.6742063152013,-56.5391628964206,
-40.3822815284329));
#259363=CARTESIAN_POINT('Ctrl Pts',(-43.6798092119243,-56.534479009001,
-40.3827188413654));
#259364=CARTESIAN_POINT('Ctrl Pts',(-43.6967370434146,-56.5206915949946,
-40.3842131357726));
#259365=CARTESIAN_POINT('Ctrl Pts',(-43.7196778600618,-56.5029622466235,
-40.386692708542));
#259366=CARTESIAN_POINT('Ctrl Pts',(-43.7670264629127,-56.4700551612604,
-40.3935618621563));
#259367=CARTESIAN_POINT('Ctrl Pts',(-43.8165352419067,-56.4409186299576,
-40.4032471370382));
#259368=CARTESIAN_POINT('Ctrl Pts',(-43.8552784957563,-56.4218759376155,
-40.4126045758866));
#259369=CARTESIAN_POINT('Ctrl Pts',(-43.8814691350842,-56.4098116142502,
-40.4193119877837));
#259370=CARTESIAN_POINT('Ctrl Pts',(-43.8947490665381,-56.4040935548973,
-40.4229014011429));
#259371=CARTESIAN_POINT('Ctrl Pts',(-43.9216608718689,-56.3933018151258,
-40.430550144354));
#259372=CARTESIAN_POINT('Ctrl Pts',(-43.9353412421961,-56.3882139347518,
-40.434625723994));
#259373=CARTESIAN_POINT('Ctrl Pts',(-43.9627318697344,-56.3788058930362,
-40.4431514805252));
#259374=CARTESIAN_POINT('Ctrl Pts',(-43.9765011076412,-56.3744602994329,
-40.4476175822086));
#259375=CARTESIAN_POINT('Ctrl Pts',(-44.0179764085085,-56.3624961934912,
-40.4615970784657));
#259376=CARTESIAN_POINT('Ctrl Pts',(-44.0598195105868,-56.3526585058303,
-40.4767455237411));
#259377=CARTESIAN_POINT('Ctrl Pts',(-44.1163310625808,-56.3437038269143,
-40.4992178608308));
#259378=CARTESIAN_POINT('Ctrl Pts',(-44.1590753545772,-56.3390714325247,
-40.5172068769433));
#259379=CARTESIAN_POINT('Ctrl Pts',(-44.1878153726385,-56.337382052278,
-40.5299596579145));
#259380=CARTESIAN_POINT('Ctrl Pts',(-44.2166756293141,-56.3364007867548,
-40.5430944022758));
#259381=CARTESIAN_POINT('Ctrl Pts',(-44.2311921171808,-56.3362675100036,
-40.5498666179945));
#259382=CARTESIAN_POINT('Ctrl Pts',(-44.2599977007373,-56.3367129587916,
-40.5636298486377));
#259383=CARTESIAN_POINT('Ctrl Pts',(-44.2743541649932,-56.3372884158027,
-40.5706510752088));
#259384=CARTESIAN_POINT('Ctrl Pts',(-44.3029357424357,-56.3391317429585,
-40.5849473061899));
#259385=CARTESIAN_POINT('Ctrl Pts',(-44.3456316213443,-56.3429350642169,
-40.6067818596389));
#259386=CARTESIAN_POINT('Ctrl Pts',(-44.4018650235691,-56.3520939287388,
-40.6374236066311));
#259387=CARTESIAN_POINT('Ctrl Pts',(-44.4574103376146,-56.3653147883305,
-40.6695718678152));
#259388=CARTESIAN_POINT('Ctrl Pts',(-44.4849466005937,-56.3732907222196,
-40.686147922621));
#259389=CARTESIAN_POINT('Ctrl Pts',(-44.512374392093,-56.3819617528141,
-40.7029840503412));
#259390=CARTESIAN_POINT('Ctrl Pts',(-44.5260289861432,-56.3866462995878,
-40.7115304197201));
#259391=CARTESIAN_POINT('Ctrl Pts',(-44.5529609776699,-56.3966203919845,
-40.7287150345567));
#259392=CARTESIAN_POINT('Ctrl Pts',(-44.5662873943758,-56.4019250012471,
-40.737383176176));
#259393=CARTESIAN_POINT('Ctrl Pts',(-44.6058068395674,-56.4187668411382,
-40.7635834132132));
#259394=CARTESIAN_POINT('Ctrl Pts',(-44.6315615859976,-56.4312362585519,
-40.7813233152079));
#259395=CARTESIAN_POINT('Ctrl Pts',(-44.6693071486035,-56.4518014713652,
-40.8083384498991));
#259396=CARTESIAN_POINT('Ctrl Pts',(-44.6817372625133,-56.458965010373,
-40.8174084081892));
#259397=CARTESIAN_POINT('Ctrl Pts',(-44.7063132537473,-56.473929075182,
-40.8356956250034));
#259398=CARTESIAN_POINT('Ctrl Pts',(-44.7183832523531,-56.4816832398284,
-40.8448563495594));
#259399=CARTESIAN_POINT('Ctrl Pts',(-44.7538754102704,-56.505703003501,
-40.8723327540241));
#259400=CARTESIAN_POINT('Ctrl Pts',(-44.7766465418209,-56.5227549736834,
-40.8906872015444));
#259401=CARTESIAN_POINT('Ctrl Pts',(-44.8204030914552,-56.5588699415109,
-40.9274359243417));
#259402=CARTESIAN_POINT('Ctrl Pts',(-44.851893062885,-56.5874690797881,
-40.9550350105826));
#259403=CARTESIAN_POINT('Ctrl Pts',(-44.8813802932551,-56.6183507815631,
-40.982690555711));
#259404=CARTESIAN_POINT('Ctrl Pts',(-44.9005867815582,-56.6394533348067,
-41.0011404791447));
#259405=CARTESIAN_POINT('Ctrl Pts',(-44.9099603095753,-56.6502571213647,
-41.0103678872986));
#259406=CARTESIAN_POINT('Ctrl Pts',(-44.9236872082217,-56.6668706184025,
-41.0242310114538));
#259407=CARTESIAN_POINT('Ctrl Pts',(-44.9282031316495,-56.6724722064122,
-41.0288518918758));
#259408=CARTESIAN_POINT('Ctrl Pts',(-44.9370720489983,-56.6837477093971,
-41.038048314582));
#259409=CARTESIAN_POINT('Ctrl Pts',(-44.9414338933841,-56.6894322363092,
-41.0426327511372));
#259410=CARTESIAN_POINT('Ctrl Pts',(-44.9542884395491,-56.7066066663578,
-41.0563299560217));
#259411=CARTESIAN_POINT('Ctrl Pts',(-44.9625629539304,-56.7182326826763,
-41.0653994431984));
#259412=CARTESIAN_POINT('Ctrl Pts',(-44.9864941991718,-56.7536111473724,
-41.0924067111081));
#259413=CARTESIAN_POINT('Ctrl Pts',(-45.0086645271567,-56.7900134244028,
-41.1190329135161));
#259414=CARTESIAN_POINT('Ctrl Pts',(-45.034704630644,-56.8405768845403,
-41.1537712607408));
#259415=CARTESIAN_POINT('Ctrl Pts',(-45.0465408860903,-56.8665423758261,
-41.1708862092094));
#259416=CARTESIAN_POINT('Ctrl Pts',(-45.0577761134165,-56.8928546179869,
-41.1878727246706));
#259417=CARTESIAN_POINT('Ctrl Pts',(-45.0630901582258,-56.906176087846,
-41.1962967595746));
#259418=CARTESIAN_POINT('Ctrl Pts',(-45.0731156002939,-56.9332061371524,
-41.2130345018643));
#259419=CARTESIAN_POINT('Ctrl Pts',(-45.0777961712447,-56.9468340019015,
-41.2212978165198));
#259420=CARTESIAN_POINT('Ctrl Pts',(-45.0907786540592,-56.9878560258786,
-41.2456540007716));
#259421=CARTESIAN_POINT('Ctrl Pts',(-45.0980724298404,-57.0154910056487,
-41.2613826498774));
#259422=CARTESIAN_POINT('Ctrl Pts',(-45.1099506000897,-57.0712899900431,
-41.2918166667949));
#259423=CARTESIAN_POINT('Ctrl Pts',(-45.1168338059478,-57.11354441615,-41.3138815317038));
#259424=CARTESIAN_POINT('Ctrl Pts',(-45.1206309792415,-57.1564190282566,
-41.3347987762303));
#259425=CARTESIAN_POINT('Ctrl Pts',(-45.1224627479043,-57.1851396939165,
-41.3484832320635));
#259426=CARTESIAN_POINT('Ctrl Pts',(-45.1230291819396,-57.199581674993,
-41.3552011986272));
#259427=CARTESIAN_POINT('Ctrl Pts',(-45.1234439819388,-57.2285619504273,
-41.3683510337761));
#259428=CARTESIAN_POINT('Ctrl Pts',(-45.1232917301137,-57.2429904040975,
-41.3747335054784));
#259429=CARTESIAN_POINT('Ctrl Pts',(-45.122279779691,-57.2717682086368,
-41.3871399525693));
#259430=CARTESIAN_POINT('Ctrl Pts',(-45.1196997436484,-57.3147947598186,
-41.4052018313649));
#259431=CARTESIAN_POINT('Ctrl Pts',(-45.1120557453653,-57.3716084168758,
-41.4271228345082));
#259432=CARTESIAN_POINT('Ctrl Pts',(-45.1031553338884,-57.4137999065974,
-41.4419446800329));
#259433=CARTESIAN_POINT('Ctrl Pts',(-45.09650693546,-57.4418330021969,-41.4514615780937));
#259434=CARTESIAN_POINT('Ctrl Pts',(-45.092823442876,-57.4558081403435,
-41.4560396298995));
#259435=CARTESIAN_POINT('Ctrl Pts',(-45.08473584999,-57.4836385233421,-41.464818484644));
#259436=CARTESIAN_POINT('Ctrl Pts',(-45.0803094818206,-57.4975537933777,
-41.4690360581021));
#259437=CARTESIAN_POINT('Ctrl Pts',(-45.0708158371377,-57.5249803724867,
-41.4770040232021));
#259438=CARTESIAN_POINT('Ctrl Pts',(-45.060662137239,-57.5520858826269,
-41.4845331733926));
#259439=CARTESIAN_POINT('Ctrl Pts',(-45.0434887903859,-57.591755117417,
-41.4945182619959));
#259440=CARTESIAN_POINT('Ctrl Pts',(-45.0243848727922,-57.6304534586566,
-41.5032105668009));
#259441=CARTESIAN_POINT('Ctrl Pts',(-45.0033512023575,-57.6681778817651,
-41.51061115159));
#259442=CARTESIAN_POINT('Ctrl Pts',(-44.9880328234845,-57.692673879575,
-41.5146787869643));
#259443=CARTESIAN_POINT('Ctrl Pts',(-44.9720568870916,-57.7168380825906,
-41.5183074012753));
#259444=CARTESIAN_POINT('Ctrl Pts',(-44.9637457009402,-57.7287466936453,
-41.5199012977462));
#259445=CARTESIAN_POINT('Ctrl Pts',(-44.9464287138105,-57.7522550306847,
-41.5226441863212));
#259446=CARTESIAN_POINT('Ctrl Pts',(-44.9374830238235,-57.7637718882179,
-41.5237830976086));
#259447=CARTESIAN_POINT('Ctrl Pts',(-44.9099214446927,-57.7974515399035,
-41.5264929611258));
#259448=CARTESIAN_POINT('Ctrl Pts',(-44.8905204729439,-57.8188493934961,
-41.5273772161885));
#259449=CARTESIAN_POINT('Ctrl Pts',(-44.8497318000032,-57.8595330722204,
-41.5273307191807));
#259450=CARTESIAN_POINT('Ctrl Pts',(-44.8283374647208,-57.878828810327,
-41.5264014189239));
#259451=CARTESIAN_POINT('Ctrl Pts',(-44.7947479986672,-57.9061820008563,
-41.5236391765087));
#259452=CARTESIAN_POINT('Ctrl Pts',(-44.7832945060713,-57.9150388128137,
-41.5224889540588));
#259453=CARTESIAN_POINT('Ctrl Pts',(-44.7657408175914,-57.9279147771907,
-41.5204166102647));
#259454=CARTESIAN_POINT('Ctrl Pts',(-44.7598217545323,-57.9321421746299,
-41.5196671186517));
#259455=CARTESIAN_POINT('Ctrl Pts',(-44.7478629508254,-57.9404557426351,
-41.5180519716851));
#259456=CARTESIAN_POINT('Ctrl Pts',(-44.7297025277655,-57.9527400844071,
-41.5154481926132));
#259457=CARTESIAN_POINT('Ctrl Pts',(-44.711220794734,-57.9642369190977,
-41.5123523449538));
#259458=CARTESIAN_POINT('Ctrl Pts',(-44.6862770262529,-57.9788987855805,
-41.5077941640223));
#259459=CARTESIAN_POINT('Ctrl Pts',(-44.6484202704456,-57.9998814948776,
-41.5003121274858));
#259460=CARTESIAN_POINT('Ctrl Pts',(-44.5962108390282,-58.0238874022289,
-41.4877980263462));
#259461=CARTESIAN_POINT('Ctrl Pts',(-44.5557649369164,-58.0389385823793,
-41.4765186283493));
#259462=CARTESIAN_POINT('Ctrl Pts',(-44.5285120653069,-58.048310487242,
-41.4685735203231));
#259463=CARTESIAN_POINT('Ctrl Pts',(-44.5147341086114,-58.0526671867402,
-41.4643859028639));
#259464=CARTESIAN_POINT('Ctrl Pts',(-44.4869140318333,-58.0607029371288,
-41.4555883503401));
#259465=CARTESIAN_POINT('Ctrl Pts',(-44.4728027150897,-58.0643973546439,
-41.4509544537452));
#259466=CARTESIAN_POINT('Ctrl Pts',(-44.4304531283686,-58.0743536715507,
-41.4365378845966));
#259467=CARTESIAN_POINT('Ctrl Pts',(-44.3879697631396,-58.0821103913619,
-41.4210702443308));
#259468=CARTESIAN_POINT('Ctrl Pts',(-44.3452880889881,-58.0866896268435,
-41.4040725286766));
#259469=CARTESIAN_POINT('Ctrl Pts',(-44.3025416355467,-58.090217180745,
-41.3865671155567));
#259470=CARTESIAN_POINT('Ctrl Pts',(-44.2739489581488,-58.0911687787978,
-41.3742170239002));
#259471=CARTESIAN_POINT('Ctrl Pts',(-44.2309555122234,-58.090491506171,
-41.3546803180427));
#259472=CARTESIAN_POINT('Ctrl Pts',(-44.2165895018292,-58.0899123697243,
-41.347990487553));
#259473=CARTESIAN_POINT('Ctrl Pts',(-44.1950278537333,-58.0885113544661,
-41.337705180963));
#259474=CARTESIAN_POINT('Ctrl Pts',(-44.1878319550126,-58.0879547296283,
-41.3342316293533));
#259475=CARTESIAN_POINT('Ctrl Pts',(-44.1734279164018,-58.0866616594573,
-41.3271961709002));
#259476=CARTESIAN_POINT('Ctrl Pts',(-44.1662260389348,-58.0859253983809,
-41.3236371482021));
#259477=CARTESIAN_POINT('Ctrl Pts',(-44.130389101081,-58.0818150523559,
-41.3057210105631));
#259478=CARTESIAN_POINT('Ctrl Pts',(-44.073848260417,-58.0724828543971,
-41.2761395013722));
#259479=CARTESIAN_POINT('Ctrl Pts',(-44.0188545174212,-58.0578491440998,
-41.2447838757269));
#259480=CARTESIAN_POINT('Ctrl Pts',(-43.9646246641704,-58.0405931079736,
-41.2125419608827));
#259481=CARTESIAN_POINT('Ctrl Pts',(-43.9378880325505,-58.0306505669816,
-41.1959746665064));
#259482=CARTESIAN_POINT('Ctrl Pts',(-43.9049634769563,-58.0165631445999,
-41.174705886574));
#259483=CARTESIAN_POINT('Ctrl Pts',(-43.898399460067,-58.0136596367661,
-41.1704209658528));
#259484=CARTESIAN_POINT('Ctrl Pts',(-43.8853286348063,-58.0076886655405,
-41.1617993561325));
#259485=CARTESIAN_POINT('Ctrl Pts',(-43.8788088737381,-58.0046144513738,
-41.157453730181));
#259486=CARTESIAN_POINT('Ctrl Pts',(-43.8593967360427,-57.9951717320096,
-41.1443784829743));
#259487=CARTESIAN_POINT('Ctrl Pts',(-43.8466719188398,-57.9885954718361,
-41.1356253645631));
#259488=CARTESIAN_POINT('Ctrl Pts',(-43.8341420587998,-57.9817357678076,
-41.1268248734572));
#259489=CARTESIAN_POINT('Ctrl Pts',(-46.1726021405987,-56.3668761797815,
-39.5898551158851));
#259490=CARTESIAN_POINT('Ctrl Pts',(-46.2069057047429,-56.4183864095348,
-39.607121781657));
#259491=CARTESIAN_POINT('Ctrl Pts',(-46.2553082908951,-56.4989321412679,
-39.6330245761036));
#259492=CARTESIAN_POINT('Ctrl Pts',(-46.3126017708591,-56.6115274351852,
-39.6670695777419));
#259493=CARTESIAN_POINT('Ctrl Pts',(-46.3391231723103,-56.6705508392544,
-39.6841845262104));
#259494=CARTESIAN_POINT('Ctrl Pts',(-46.3642693448436,-56.7303750220794,
-39.7011710416717));
#259495=CARTESIAN_POINT('Ctrl Pts',(-46.3761479944029,-56.76066924716,-39.7095950765756));
#259496=CARTESIAN_POINT('Ctrl Pts',(-46.3985257027381,-56.8221504582685,
-39.7263328188654));
#259497=CARTESIAN_POINT('Ctrl Pts',(-46.4089559133708,-56.8531538688126,
-39.73459613352));
#259498=CARTESIAN_POINT('Ctrl Pts',(-46.437831026164,-56.9464970853635,
-39.7589523177745));
#259499=CARTESIAN_POINT('Ctrl Pts',(-46.4539750647129,-57.0094025506593,
-39.7746809668783));
#259500=CARTESIAN_POINT('Ctrl Pts',(-46.4800815194185,-57.1364635805498,
-39.8051149837962));
#259501=CARTESIAN_POINT('Ctrl Pts',(-46.4950400693282,-57.232716021489,
-39.8271798487049));
#259502=CARTESIAN_POINT('Ctrl Pts',(-46.5029571390459,-57.3304319805551,
-39.8480970932315));
#259503=CARTESIAN_POINT('Ctrl Pts',(-46.5066387211099,-57.3959008325223,
-39.8617815490646));
#259504=CARTESIAN_POINT('Ctrl Pts',(-46.5076819483115,-57.4288270025733,
-39.8684995156283));
#259505=CARTESIAN_POINT('Ctrl Pts',(-46.508130707335,-57.4949103365212,
-39.8816493507771));
#259506=CARTESIAN_POINT('Ctrl Pts',(-46.5075367124945,-57.527817016895,
-39.8880318224796));
#259507=CARTESIAN_POINT('Ctrl Pts',(-46.504738178928,-57.5934611321397,
-39.9004382695704));
#259508=CARTESIAN_POINT('Ctrl Pts',(-46.4981227877063,-57.6916244184968,
-39.9185001483662));
#259509=CARTESIAN_POINT('Ctrl Pts',(-46.4797328401766,-57.8213090440304,
-39.940421151509));
#259510=CARTESIAN_POINT('Ctrl Pts',(-46.4587298084939,-57.9176672625727,
-39.9552429970341));
#259511=CARTESIAN_POINT('Ctrl Pts',(-46.4431004971084,-57.9817016478038,
-39.9647598950948));
#259512=CARTESIAN_POINT('Ctrl Pts',(-46.4344677710292,-58.0136300484471,
-39.9693379469006));
#259513=CARTESIAN_POINT('Ctrl Pts',(-46.4155621210723,-58.0772247635304,
-39.9781168016451));
#259514=CARTESIAN_POINT('Ctrl Pts',(-46.4052374261782,-58.109028316384,
-39.9823343751034));
#259515=CARTESIAN_POINT('Ctrl Pts',(-46.3831342217529,-58.1717242862158,
-39.9903023402032));
#259516=CARTESIAN_POINT('Ctrl Pts',(-46.3595321549874,-58.2336984575206,
-39.9978314903936));
#259517=CARTESIAN_POINT('Ctrl Pts',(-46.3244338236407,-58.3136871658631,
-40.0066338415421));
#259518=CARTESIAN_POINT('Ctrl Pts',(-46.3006305954557,-58.3624460386648,
-40.0115250278133));
#259519=CARTESIAN_POINT('Ctrl Pts',(-46.2909969450817,-58.3814064047113,
-40.0133526947335));
#259520=CARTESIAN_POINT('Ctrl Pts',(-46.2909969422729,-58.3814064027011,
-40.013352709603));
#259521=CARTESIAN_POINT('Ctrl Pts',(-46.3693097501125,-58.1875098833917,
-40.0137875322504));
#259522=CARTESIAN_POINT('Ctrl Pts',(-46.411278999678,-57.9809289977677,
-40.0118819906088));
#259523=CARTESIAN_POINT('Ctrl Pts',(-46.4191068837893,-57.5991845865335,
-40.0050928659256));
#259524=CARTESIAN_POINT('Ctrl Pts',(-46.3968688023029,-57.4268964497847,
-40.0008179121686));
#259525=CARTESIAN_POINT('Ctrl Pts',(-46.2946092803027,-57.0638316879311,
-39.9897515821211));
#259526=CARTESIAN_POINT('Ctrl Pts',(-46.2056470788626,-56.8783069534362,
-39.9827369701668));
#259527=CARTESIAN_POINT('Ctrl Pts',(-45.9855349754196,-56.5673096976623,
-39.9689716167871));
#259528=CARTESIAN_POINT('Ctrl Pts',(-45.8629979265771,-56.4391204389221,
-39.9626060055202));
#259529=CARTESIAN_POINT('Ctrl Pts',(-45.7222549758842,-56.3308214393021,
-39.9581073668549));
#259530=CARTESIAN_POINT('Ctrl Pts',(-45.3258935545055,-56.0209136569754,
-39.8341888326825));
#259531=CARTESIAN_POINT('Ctrl Pts',(-45.4764270023181,-56.0526141472619,
-39.797283341326));
#259532=CARTESIAN_POINT('Ctrl Pts',(-45.6236924541279,-56.098325931019,
-39.7577446198746));
#259533=CARTESIAN_POINT('Ctrl Pts',(-45.9074046606253,-56.214732273663,
-39.6755637187821));
#259534=CARTESIAN_POINT('Ctrl Pts',(-46.0434656100389,-56.2851743761681,
-39.6330616925565));
#259535=CARTESIAN_POINT('Ctrl Pts',(-46.1726021442766,-56.3668761803699,
-39.5898551239125));
#259536=CARTESIAN_POINT('Ctrl Pts',(-43.4805771074156,-59.5712767529309,
-39.2399080357013));
#259537=CARTESIAN_POINT('Ctrl Pts',(-43.4150727209207,-59.5358440364426,
-39.2223070534893));
#259538=CARTESIAN_POINT('Ctrl Pts',(-43.2883193276586,-59.4590682572254,
-39.1867578392588));
#259539=CARTESIAN_POINT('Ctrl Pts',(-43.1106712693135,-59.32658002426,-39.1324031814995));
#259540=CARTESIAN_POINT('Ctrl Pts',(-43.0005921597408,-59.2266373021163,
-39.0954660506179));
#259541=CARTESIAN_POINT('Ctrl Pts',(-42.8948534568781,-59.1207134074407,
-39.0581733199915));
#259542=CARTESIAN_POINT('Ctrl Pts',(-42.7951360401793,-59.0104958554849,
-39.0211184761739));
#259543=CARTESIAN_POINT('Ctrl Pts',(-42.6850011896347,-58.8622904152127,
-38.9753582681256));
#259544=CARTESIAN_POINT('Ctrl Pts',(-42.6055727997797,-58.7375004045667,
-38.939089851323));
#259545=CARTESIAN_POINT('Ctrl Pts',(-42.5503788594446,-58.6407591922129,
-38.9120596161462));
#259546=CARTESIAN_POINT('Ctrl Pts',(-42.5165536369311,-58.5741539171446,
-38.8941613358138));
#259547=CARTESIAN_POINT('Ctrl Pts',(-42.4842288567228,-58.5064298632496,
-38.8763157156907));
#259548=CARTESIAN_POINT('Ctrl Pts',(-42.4689425396028,-58.4722695523732,
-38.8674882509199));
#259549=CARTESIAN_POINT('Ctrl Pts',(-42.4257123024776,-58.3690064948315,
-38.8413136266604));
#259550=CARTESIAN_POINT('Ctrl Pts',(-42.3750272156063,-58.229152189777,
-38.8072100415055));
#259551=CARTESIAN_POINT('Ctrl Pts',(-42.3380647902547,-58.0850119200902,
-38.7746901633276));
#259552=CARTESIAN_POINT('Ctrl Pts',(-42.3155659796374,-57.9752818499468,
-38.7509105250088));
#259553=CARTESIAN_POINT('Ctrl Pts',(-42.3089374211558,-57.9384266221928,
-38.7430843922672));
#259554=CARTESIAN_POINT('Ctrl Pts',(-42.297458012674,-57.864178756387,-38.7276438637217));
#259555=CARTESIAN_POINT('Ctrl Pts',(-42.292601515188,-57.8267325312259,
-38.720018782004));
#259556=CARTESIAN_POINT('Ctrl Pts',(-42.2847289916893,-57.7514526301959,
-38.7050196673963));
#259557=CARTESIAN_POINT('Ctrl Pts',(-42.2817363521424,-57.7138759968928,
-38.6976962453237));
#259558=CARTESIAN_POINT('Ctrl Pts',(-42.277596992864,-57.6387184974263,
-38.6833720377019));
#259559=CARTESIAN_POINT('Ctrl Pts',(-42.2741651307842,-57.5260409596698,
-38.6623829091612));
#259560=CARTESIAN_POINT('Ctrl Pts',(-42.2805893100654,-57.3760354719141,
-38.6363740800325));
#259561=CARTESIAN_POINT('Ctrl Pts',(-42.2937061680812,-57.2637038035873,
-38.618370061439));
#259562=CARTESIAN_POINT('Ctrl Pts',(-42.3043247017591,-57.1888547452426,
-38.6067079534822));
#259563=CARTESIAN_POINT('Ctrl Pts',(-42.3105743117123,-57.1514345461221,
-38.6010450635964));
#259564=CARTESIAN_POINT('Ctrl Pts',(-42.3249704170347,-57.0766935209607,
-38.590076215021));
#259565=CARTESIAN_POINT('Ctrl Pts',(-42.3331592025312,-57.0392159768686,
-38.5847494243559));
#259566=CARTESIAN_POINT('Ctrl Pts',(-42.3512949844302,-56.9651221381903,
-38.5745673038812));
#259567=CARTESIAN_POINT('Ctrl Pts',(-42.3712216906218,-56.8916587034686,
-38.564820665347));
#259568=CARTESIAN_POINT('Ctrl Pts',(-42.4063979707918,-56.7834465224234,
-38.5515118436));
#259569=CARTESIAN_POINT('Ctrl Pts',(-42.4468320479729,-56.6771725078319,
-38.5395042677724));
#259570=CARTESIAN_POINT('Ctrl Pts',(-42.4925290654744,-56.5728473165674,
-38.5288039137004));
#259571=CARTESIAN_POINT('Ctrl Pts',(-42.5265325119253,-56.5046058456765,
-38.5225509073062));
#259572=CARTESIAN_POINT('Ctrl Pts',(-42.5623338475306,-56.4370293947697,
-38.5167461666044));
#259573=CARTESIAN_POINT('Ctrl Pts',(-42.5811223641794,-56.4035923099625,
-38.5140693065785));
#259574=CARTESIAN_POINT('Ctrl Pts',(-42.620584523009,-56.3373241998654,
-38.5091697400817));
#259575=CARTESIAN_POINT('Ctrl Pts',(-42.6411082254821,-56.3047465904101,
-38.5069659500128));
#259576=CARTESIAN_POINT('Ctrl Pts',(-42.7048067991197,-56.2090283357163,
-38.501110858935));
#259577=CARTESIAN_POINT('Ctrl Pts',(-42.7502234543428,-56.1476408662828,
-38.4981890389281));
#259578=CARTESIAN_POINT('Ctrl Pts',(-42.8467942323831,-56.0297655581676,
-38.4942910511033));
#259579=CARTESIAN_POINT('Ctrl Pts',(-42.8979715413934,-55.9732420482176,
-38.4933125989996));
#259580=CARTESIAN_POINT('Ctrl Pts',(-42.9790570553347,-55.8921695883033,
-38.4933149859729));
#259581=CARTESIAN_POINT('Ctrl Pts',(-43.0068374106561,-55.8657400908868,
-38.4935622007431));
#259582=CARTESIAN_POINT('Ctrl Pts',(-43.0495800649421,-55.8270637749536,
-38.4943063068789));
#259583=CARTESIAN_POINT('Ctrl Pts',(-43.0640222060113,-55.8143203511958,
-38.494617152342));
#259584=CARTESIAN_POINT('Ctrl Pts',(-43.0932714774893,-55.7891564261061,
-38.4953646906773));
#259585=CARTESIAN_POINT('Ctrl Pts',(-43.1080901283632,-55.7767277938553,
-38.4958020036096));
#259586=CARTESIAN_POINT('Ctrl Pts',(-43.1528523310046,-55.7401327167866,
-38.4972962980169));
#259587=CARTESIAN_POINT('Ctrl Pts',(-43.2134913856688,-55.6930468850421,
-38.4997758707861));
#259588=CARTESIAN_POINT('Ctrl Pts',(-43.3385569247743,-55.6055389451161,
-38.5066450244003));
#259589=CARTESIAN_POINT('Ctrl Pts',(-43.4691986576013,-55.5278792007279,
-38.5163302992824));
#259590=CARTESIAN_POINT('Ctrl Pts',(-43.5713395927684,-55.4769743237494,
-38.5256877381308));
#259591=CARTESIAN_POINT('Ctrl Pts',(-43.6403672861995,-55.4446857735354,
-38.5323951500278));
#259592=CARTESIAN_POINT('Ctrl Pts',(-43.6753577685123,-55.4293620157832,
-38.5359845633874));
#259593=CARTESIAN_POINT('Ctrl Pts',(-43.7462462065788,-55.4003985583156,
-38.5436333065981));
#259594=CARTESIAN_POINT('Ctrl Pts',(-43.7822717759725,-55.3867204456352,
-38.5477088862383));
#259595=CARTESIAN_POINT('Ctrl Pts',(-43.8543821738219,-55.3613797848081,
-38.5562346427694));
#259596=CARTESIAN_POINT('Ctrl Pts',(-43.890622407919,-55.349649082917,-38.5607007444526));
#259597=CARTESIAN_POINT('Ctrl Pts',(-43.9997560709039,-55.3172704656441,
-38.5746802407103));
#259598=CARTESIAN_POINT('Ctrl Pts',(-44.1098017310836,-55.290468361793,
-38.5898286859852));
#259599=CARTESIAN_POINT('Ctrl Pts',(-44.2583166685835,-55.2656490138239,
-38.612301023075));
#259600=CARTESIAN_POINT('Ctrl Pts',(-44.3705972700495,-55.2524997368729,
-38.6302900391873));
#259601=CARTESIAN_POINT('Ctrl Pts',(-44.446056048267,-55.2474029004138,
-38.6430428201589));
#259602=CARTESIAN_POINT('Ctrl Pts',(-44.5218128020516,-55.2441636366351,
-38.65617756452));
#259603=CARTESIAN_POINT('Ctrl Pts',(-44.5599089424743,-55.2434808562086,
-38.6629497802385));
#259604=CARTESIAN_POINT('Ctrl Pts',(-44.6354869543582,-55.2439911084578,
-38.6767130108817));
#259605=CARTESIAN_POINT('Ctrl Pts',(-44.6731456892459,-55.2451740103824,
-38.6837342374529));
#259606=CARTESIAN_POINT('Ctrl Pts',(-44.7481014788608,-55.2493620066237,
-38.6980304684339));
#259607=CARTESIAN_POINT('Ctrl Pts',(-44.860046548974,-55.2583760573225,
-38.7198650218829));
#259608=CARTESIAN_POINT('Ctrl Pts',(-45.0073845433675,-55.2811507310277,
-38.7505067688753));
#259609=CARTESIAN_POINT('Ctrl Pts',(-45.1528189888476,-55.3146135839333,
-38.7826550300594));
#259610=CARTESIAN_POINT('Ctrl Pts',(-45.2248832056965,-55.3349380951144,
-38.7992310848652));
#259611=CARTESIAN_POINT('Ctrl Pts',(-45.2966462681613,-55.3570913336823,
-38.8160672125853));
#259612=CARTESIAN_POINT('Ctrl Pts',(-45.3323638946335,-55.3690863290504,
-38.8246135819642));
#259613=CARTESIAN_POINT('Ctrl Pts',(-45.4027951436545,-55.3946744461232,
-38.841798196801));
#259614=CARTESIAN_POINT('Ctrl Pts',(-45.4376370321487,-55.4083060218429,
-38.85046633842));
#259615=CARTESIAN_POINT('Ctrl Pts',(-45.5409345111852,-55.4516493275196,
-38.8766665754573));
#259616=CARTESIAN_POINT('Ctrl Pts',(-45.6082182891413,-55.4838201174091,
-38.8944064774514));
#259617=CARTESIAN_POINT('Ctrl Pts',(-45.7067749877369,-55.5369855856676,
-38.9214216121435));
#259618=CARTESIAN_POINT('Ctrl Pts',(-45.7392219877795,-55.5555212114618,
-38.9304915704334));
#259619=CARTESIAN_POINT('Ctrl Pts',(-45.8033556832395,-55.5942722159849,
-38.9487787872477));
#259620=CARTESIAN_POINT('Ctrl Pts',(-45.8348443691401,-55.6143675312756,
-38.9579395118015));
#259621=CARTESIAN_POINT('Ctrl Pts',(-45.9274099842789,-55.6766589025306,
-38.9854159162723));
#259622=CARTESIAN_POINT('Ctrl Pts',(-45.9867610865919,-55.7209353156014,
-39.0037703637879));
#259623=CARTESIAN_POINT('Ctrl Pts',(-46.1007337830098,-55.8148102393793,
-39.0405190865864));
#259624=CARTESIAN_POINT('Ctrl Pts',(-46.1826971388658,-55.889219933262,
-39.0681181728269));
#259625=CARTESIAN_POINT('Ctrl Pts',(-46.259356574729,-55.9696687352924,
-39.0957737179551));
#259626=CARTESIAN_POINT('Ctrl Pts',(-46.309266807939,-56.024663053365,-39.1142236413887));
#259627=CARTESIAN_POINT('Ctrl Pts',(-46.3336138177017,-56.0528284109483,
-39.1234510495426));
#259628=CARTESIAN_POINT('Ctrl Pts',(-46.3692509284248,-56.0961546965833,
-39.1373141736981));
#259629=CARTESIAN_POINT('Ctrl Pts',(-46.3809719555493,-56.1107655250657,
-39.14193505412));
#259630=CARTESIAN_POINT('Ctrl Pts',(-46.4039850968433,-56.1401806715041,
-39.1511314768264));
#259631=CARTESIAN_POINT('Ctrl Pts',(-46.4153001903629,-56.1550126624776,
-39.1557159133813));
#259632=CARTESIAN_POINT('Ctrl Pts',(-46.4486370096885,-56.1998310060263,
-39.1694131182659));
#259633=CARTESIAN_POINT('Ctrl Pts',(-46.4700835091466,-56.2301795317326,
-39.1784826054425));
#259634=CARTESIAN_POINT('Ctrl Pts',(-46.532071913686,-56.3225583984772,
-39.2054898733524));
#259635=CARTESIAN_POINT('Ctrl Pts',(-46.5894197348374,-56.4176636744323,
-39.23211607576));
#259636=CARTESIAN_POINT('Ctrl Pts',(-46.6566074362748,-56.5498680842415,
-39.2668544229849));
#259637=CARTESIAN_POINT('Ctrl Pts',(-46.6870820302515,-56.617790568625,
-39.2839693714534));
#259638=CARTESIAN_POINT('Ctrl Pts',(-46.7159729830272,-56.6866360545619,
-39.3009558869148));
#259639=CARTESIAN_POINT('Ctrl Pts',(-46.7296188023799,-56.7214992889704,
-39.3093799218186));
#259640=CARTESIAN_POINT('Ctrl Pts',(-46.7553216997643,-56.7922546384013,
-39.3261176641085));
#259641=CARTESIAN_POINT('Ctrl Pts',(-46.7672996943011,-56.8279354881579,
-39.3343809787628));
#259642=CARTESIAN_POINT('Ctrl Pts',(-46.8004530502947,-56.9353633959568,
-39.358737163018));
#259643=CARTESIAN_POINT('Ctrl Pts',(-46.8189795501832,-57.0077635587999,
-39.3744658121213));
#259644=CARTESIAN_POINT('Ctrl Pts',(-46.848916211803,-57.1540080946302,
-39.4048998290393));
#259645=CARTESIAN_POINT('Ctrl Pts',(-46.866048617508,-57.2647966217996,
-39.4269646939479));
#259646=CARTESIAN_POINT('Ctrl Pts',(-46.875074749658,-57.3772756893033,
-39.4478819384746));
#259647=CARTESIAN_POINT('Ctrl Pts',(-46.8792542953452,-57.4526370309597,
-39.4615663943076));
#259648=CARTESIAN_POINT('Ctrl Pts',(-46.8804258736835,-57.4905390832845,
-39.4682843608713));
#259649=CARTESIAN_POINT('Ctrl Pts',(-46.8808837743635,-57.566610437341,
-39.4814341960201));
#259650=CARTESIAN_POINT('Ctrl Pts',(-46.8801708637706,-57.604491394965,
-39.4878166677226));
#259651=CARTESIAN_POINT('Ctrl Pts',(-46.8768913879562,-57.6800597985945,
-39.5002231148134));
#259652=CARTESIAN_POINT('Ctrl Pts',(-46.8691896925243,-57.7930657109158,
-39.5182849936093));
#259653=CARTESIAN_POINT('Ctrl Pts',(-46.8479069711518,-57.9423669591112,
-39.540205996752));
#259654=CARTESIAN_POINT('Ctrl Pts',(-46.8236459543104,-58.053306681129,
-39.5550278422771));
#259655=CARTESIAN_POINT('Ctrl Pts',(-46.8055990109883,-58.1270324939452,
-39.5645447403379));
#259656=CARTESIAN_POINT('Ctrl Pts',(-46.7956339676918,-58.1637938532181,
-39.5691227921436));
#259657=CARTESIAN_POINT('Ctrl Pts',(-46.7738161327052,-58.2370162077019,
-39.5779016468881));
#259658=CARTESIAN_POINT('Ctrl Pts',(-46.7619036278491,-58.2736352268715,
-39.5821192203466));
#259659=CARTESIAN_POINT('Ctrl Pts',(-46.7364059718256,-58.3458255995332,
-39.5900871854462));
#259660=CARTESIAN_POINT('Ctrl Pts',(-46.7091836493705,-58.4171862986019,
-39.5976163356366));
#259661=CARTESIAN_POINT('Ctrl Pts',(-46.663274408039,-58.5216699086648,
-39.6076014242402));
#259662=CARTESIAN_POINT('Ctrl Pts',(-46.6123207377325,-58.6236436013082,
-39.616293729045));
#259663=CARTESIAN_POINT('Ctrl Pts',(-46.5563244858032,-58.7230996041114,
-39.6236943138341));
#259664=CARTESIAN_POINT('Ctrl Pts',(-46.515607032986,-58.7877140896312,
-39.6277619492082));
#259665=CARTESIAN_POINT('Ctrl Pts',(-46.4731710833873,-58.8514710047945,
-39.6313905635194));
#259666=CARTESIAN_POINT('Ctrl Pts',(-46.4511086137465,-58.8829006319494,
-39.6329844599904));
#259667=CARTESIAN_POINT('Ctrl Pts',(-46.4051673201274,-58.9449633016888,
-39.6357273485653));
#259668=CARTESIAN_POINT('Ctrl Pts',(-46.381447994276,-58.975377588932,-39.6368662598532));
#259669=CARTESIAN_POINT('Ctrl Pts',(-46.3084068909562,-59.0643493136614,
-39.6395761233691));
#259670=CARTESIAN_POINT('Ctrl Pts',(-46.2570407846102,-59.1209150453974,
-39.6404603784325));
#259671=CARTESIAN_POINT('Ctrl Pts',(-46.1491379755941,-59.228544463199,
-39.6404138814247));
#259672=CARTESIAN_POINT('Ctrl Pts',(-46.0925836555155,-59.2796343044913,
-39.6394845811684));
#259673=CARTESIAN_POINT('Ctrl Pts',(-46.0038529437629,-59.3521266125547,
-39.6367223387528));
#259674=CARTESIAN_POINT('Ctrl Pts',(-45.9736068078661,-59.3756113554055,
-39.6355721163029));
#259675=CARTESIAN_POINT('Ctrl Pts',(-45.9272656961273,-59.4097723546528,
-39.6334997725088));
#259676=CARTESIAN_POINT('Ctrl Pts',(-45.9116419215573,-59.4209912820171,
-39.6327502808957));
#259677=CARTESIAN_POINT('Ctrl Pts',(-45.8800804794677,-59.4430610802669,
-39.6311351339295));
#259678=CARTESIAN_POINT('Ctrl Pts',(-45.8321587971618,-59.4756823489919,
-39.628531354857));
#259679=CARTESIAN_POINT('Ctrl Pts',(-45.7834097108732,-59.5062438963941,
-39.6254355071979));
#259680=CARTESIAN_POINT('Ctrl Pts',(-45.717633106262,-59.5452481912826,
-39.6208773262667));
#259681=CARTESIAN_POINT('Ctrl Pts',(-45.6178307490054,-59.601113548897,
-39.6133952897297));
#259682=CARTESIAN_POINT('Ctrl Pts',(-45.4802897643185,-59.6652183443042,
-39.6008811885904));
#259683=CARTESIAN_POINT('Ctrl Pts',(-45.3738098009101,-59.7055766782111,
-39.5896017905935));
#259684=CARTESIAN_POINT('Ctrl Pts',(-45.3020778813705,-59.7307512119865,
-39.5816566825671));
#259685=CARTESIAN_POINT('Ctrl Pts',(-45.2658207311094,-59.7424779859237,
-39.5774690651077));
#259686=CARTESIAN_POINT('Ctrl Pts',(-45.1926264675053,-59.7641596016776,
-39.5686715125846));
#259687=CARTESIAN_POINT('Ctrl Pts',(-45.1555073907618,-59.7741562512684,
-39.5640376159893));
#259688=CARTESIAN_POINT('Ctrl Pts',(-45.0441315765335,-59.8011904590316,
-39.5496210468413));
#259689=CARTESIAN_POINT('Ctrl Pts',(-44.9324484012679,-59.8224577850013,
-39.5341534065747));
#259690=CARTESIAN_POINT('Ctrl Pts',(-44.8203079610257,-59.8353953605365,
-39.5171556909205));
#259691=CARTESIAN_POINT('Ctrl Pts',(-44.7080184564226,-59.8455760612675,
-39.4996502778008));
#259692=CARTESIAN_POINT('Ctrl Pts',(-44.6329372249224,-59.8486931621852,
-39.4873001861445));
#259693=CARTESIAN_POINT('Ctrl Pts',(-44.5200834441659,-59.8478515133141,
-39.4677634802869));
#259694=CARTESIAN_POINT('Ctrl Pts',(-44.4823810871712,-59.8466449718289,
-39.4610736497974));
#259695=CARTESIAN_POINT('Ctrl Pts',(-44.4258051079382,-59.8434394706745,
-39.4507883432074));
#259696=CARTESIAN_POINT('Ctrl Pts',(-44.4069254589855,-59.8421361346926,
-39.4473147915973));
#259697=CARTESIAN_POINT('Ctrl Pts',(-44.3691376542581,-59.8390581625153,
-39.4402793331445));
#259698=CARTESIAN_POINT('Ctrl Pts',(-44.3502459350849,-59.8372838734483,
-39.4367203104461));
#259699=CARTESIAN_POINT('Ctrl Pts',(-44.2562487381671,-59.8272835659938,
-39.4188041728073));
#259700=CARTESIAN_POINT('Ctrl Pts',(-44.1080045765469,-59.8040393501646,
-39.3892226636159));
#259701=CARTESIAN_POINT('Ctrl Pts',(-43.9639303529155,-59.7668593120831,
-39.3578670379715));
#259702=CARTESIAN_POINT('Ctrl Pts',(-43.8219159040518,-59.7227861654643,
-39.3256251231267));
#259703=CARTESIAN_POINT('Ctrl Pts',(-43.7519290534068,-59.6972943066161,
-39.3090578287531));
#259704=CARTESIAN_POINT('Ctrl Pts',(-43.665783177736,-59.6610675807531,
-39.2877890488175));
#259705=CARTESIAN_POINT('Ctrl Pts',(-43.6486106666635,-59.653596197985,
-39.2835041280971));
#259706=CARTESIAN_POINT('Ctrl Pts',(-43.6144193015916,-59.6382222359849,
-39.2748825183767));
#259707=CARTESIAN_POINT('Ctrl Pts',(-43.597366582891,-59.6303022352814,
-39.2705368924251));
#259708=CARTESIAN_POINT('Ctrl Pts',(-43.5465994182959,-59.605961903298,
-39.2574616452183));
#259709=CARTESIAN_POINT('Ctrl Pts',(-43.513329300663,-59.588993111175,-39.2487085268073));
#259710=CARTESIAN_POINT('Ctrl Pts',(-43.4805771074156,-59.5712767529309,
-39.2399080357013));
#259711=CARTESIAN_POINT('Ctrl Pts',(-43.8341420587998,-57.9817357678076,
-41.1268248734572));
#259712=CARTESIAN_POINT('Ctrl Pts',(-43.8090823387197,-57.9680163597508,
-41.1092238912453));
#259713=CARTESIAN_POINT('Ctrl Pts',(-43.7605654269547,-57.9383371077444,
-41.0736746770147));
#259714=CARTESIAN_POINT('Ctrl Pts',(-43.6924895655639,-57.8872515755908,
-41.019320019256));
#259715=CARTESIAN_POINT('Ctrl Pts',(-43.6502497090231,-57.8487916199066,
-40.9823828883729));
#259716=CARTESIAN_POINT('Ctrl Pts',(-43.6096433745973,-57.8080652293815,
-40.945090157748));
#259717=CARTESIAN_POINT('Ctrl Pts',(-43.5713160673933,-57.7657212262301,
-40.9080353139296));
#259718=CARTESIAN_POINT('Ctrl Pts',(-43.5288984657655,-57.7088609123343,
-40.8622751058818));
#259719=CARTESIAN_POINT('Ctrl Pts',(-43.4982484100127,-57.6610280687967,
-40.826006689079));
#259720=CARTESIAN_POINT('Ctrl Pts',(-43.4769169762936,-57.6239677344727,
-40.798976453902));
#259721=CARTESIAN_POINT('Ctrl Pts',(-43.4638199758968,-57.5984660781933,
-40.7810781735695));
#259722=CARTESIAN_POINT('Ctrl Pts',(-43.4512904535732,-57.5725430453748,
-40.7632325534464));
#259723=CARTESIAN_POINT('Ctrl Pts',(-43.4453582046716,-57.5594707895743,
-40.7544050886758));
#259724=CARTESIAN_POINT('Ctrl Pts',(-43.4285595200757,-57.5199648485381,
-40.7282304644163));
#259725=CARTESIAN_POINT('Ctrl Pts',(-43.4088016745783,-57.4664867157472,
-40.6941268792613));
#259726=CARTESIAN_POINT('Ctrl Pts',(-43.3942530508608,-57.4114223976644,
-40.6616070010832));
#259727=CARTESIAN_POINT('Ctrl Pts',(-43.3853242538269,-57.3695231591805,
-40.6378273627645));
#259728=CARTESIAN_POINT('Ctrl Pts',(-43.3826786150667,-57.3554536366825,
-40.630001230023));
#259729=CARTESIAN_POINT('Ctrl Pts',(-43.378062215599,-57.3271160344971,
-40.6145607014775));
#259730=CARTESIAN_POINT('Ctrl Pts',(-43.3760891270041,-57.3128275119467,
-40.60693561976));
#259731=CARTESIAN_POINT('Ctrl Pts',(-43.3728422231051,-57.2841093232557,
-40.5919365051523));
#259732=CARTESIAN_POINT('Ctrl Pts',(-43.3715781643254,-57.2697777029377,
-40.5846130830795));
#259733=CARTESIAN_POINT('Ctrl Pts',(-43.3697526802575,-57.2411194243864,
-40.5702888754578));
#259734=CARTESIAN_POINT('Ctrl Pts',(-43.3680717796799,-57.1981642741791,
-40.5492997469169));
#259735=CARTESIAN_POINT('Ctrl Pts',(-43.3700185838812,-57.1410182421193,
-40.5232909177883));
#259736=CARTESIAN_POINT('Ctrl Pts',(-43.3746384661022,-57.0982543712987,
-40.505286899195));
#259737=CARTESIAN_POINT('Ctrl Pts',(-43.3784319419536,-57.0697666559562,
-40.4936247912381));
#259738=CARTESIAN_POINT('Ctrl Pts',(-43.3806866868643,-57.0555278483981,
-40.4879619013523));
#259739=CARTESIAN_POINT('Ctrl Pts',(-43.3859186984709,-57.0270949764048,
-40.476993052777));
#259740=CARTESIAN_POINT('Ctrl Pts',(-43.3889115442249,-57.0128413374093,
-40.4716662621118));
#259741=CARTESIAN_POINT('Ctrl Pts',(-43.3955695423488,-56.984668670318,
-40.4614841416371));
#259742=CARTESIAN_POINT('Ctrl Pts',(-43.4029115329907,-56.9567427536229,
-40.4517375031029));
#259743=CARTESIAN_POINT('Ctrl Pts',(-43.4159439893498,-56.915628788467,
-40.4384286813559));
#259744=CARTESIAN_POINT('Ctrl Pts',(-43.4309850942545,-56.8752725380991,
-40.4264211055283));
#259745=CARTESIAN_POINT('Ctrl Pts',(-43.4480370013178,-56.8356780486645,
-40.4157207514563));
#259746=CARTESIAN_POINT('Ctrl Pts',(-43.4607570961379,-56.8097932355363,
-40.409467745062));
#259747=CARTESIAN_POINT('Ctrl Pts',(-43.4741642201056,-56.7841683331057,
-40.4036630043601));
#259748=CARTESIAN_POINT('Ctrl Pts',(-43.4812071336048,-56.7714928975767,
-40.4009861443346));
#259749=CARTESIAN_POINT('Ctrl Pts',(-43.4960130774609,-56.7463797512019,
-40.3960865778375));
#259750=CARTESIAN_POINT('Ctrl Pts',(-43.5037198572985,-56.7340380787953,
-40.3938827877695));
#259751=CARTESIAN_POINT('Ctrl Pts',(-43.527657505214,-56.6977883833479,
-40.3880276966888));
#259752=CARTESIAN_POINT('Ctrl Pts',(-43.5447483375558,-56.6745564757614,
-40.3851058766842));
#259753=CARTESIAN_POINT('Ctrl Pts',(-43.5811328114983,-56.629979998045,
-40.3812078888591));
#259754=CARTESIAN_POINT('Ctrl Pts',(-43.6004351631962,-56.6086219171049,
-40.3802294367552));
#259755=CARTESIAN_POINT('Ctrl Pts',(-43.6310475296952,-56.578014570072,
-40.3802318237287));
#259756=CARTESIAN_POINT('Ctrl Pts',(-43.6415402048873,-56.5680413281089,
-40.3804790384992));
#259757=CARTESIAN_POINT('Ctrl Pts',(-43.6576911458811,-56.5534539772523,
-40.3812231446347));
#259758=CARTESIAN_POINT('Ctrl Pts',(-43.6631494628181,-56.5486488515781,
-40.3815339900979));
#259759=CARTESIAN_POINT('Ctrl Pts',(-43.6742063152013,-56.5391628964206,
-40.3822815284329));
#259760=CARTESIAN_POINT('Ctrl Pts',(-43.6798092119243,-56.534479009001,
-40.3827188413654));
#259761=CARTESIAN_POINT('Ctrl Pts',(-43.6967370434146,-56.5206915949946,
-40.3842131357726));
#259762=CARTESIAN_POINT('Ctrl Pts',(-43.7196778600618,-56.5029622466235,
-40.386692708542));
#259763=CARTESIAN_POINT('Ctrl Pts',(-43.7670264629127,-56.4700551612604,
-40.3935618621563));
#259764=CARTESIAN_POINT('Ctrl Pts',(-43.8165352419067,-56.4409186299576,
-40.4032471370382));
#259765=CARTESIAN_POINT('Ctrl Pts',(-43.8552784957563,-56.4218759376155,
-40.4126045758866));
#259766=CARTESIAN_POINT('Ctrl Pts',(-43.8814691350842,-56.4098116142502,
-40.4193119877837));
#259767=CARTESIAN_POINT('Ctrl Pts',(-43.8947490665381,-56.4040935548973,
-40.4229014011429));
#259768=CARTESIAN_POINT('Ctrl Pts',(-43.9216608718689,-56.3933018151258,
-40.430550144354));
#259769=CARTESIAN_POINT('Ctrl Pts',(-43.9353412421961,-56.3882139347518,
-40.434625723994));
#259770=CARTESIAN_POINT('Ctrl Pts',(-43.9627318697344,-56.3788058930362,
-40.4431514805252));
#259771=CARTESIAN_POINT('Ctrl Pts',(-43.9765011076412,-56.3744602994329,
-40.4476175822086));
#259772=CARTESIAN_POINT('Ctrl Pts',(-44.0179764085085,-56.3624961934912,
-40.4615970784657));
#259773=CARTESIAN_POINT('Ctrl Pts',(-44.0598195105868,-56.3526585058303,
-40.4767455237411));
#259774=CARTESIAN_POINT('Ctrl Pts',(-44.1163310625808,-56.3437038269143,
-40.4992178608308));
#259775=CARTESIAN_POINT('Ctrl Pts',(-44.1590753545772,-56.3390714325247,
-40.5172068769433));
#259776=CARTESIAN_POINT('Ctrl Pts',(-44.1878153726385,-56.337382052278,
-40.5299596579145));
#259777=CARTESIAN_POINT('Ctrl Pts',(-44.2166756293141,-56.3364007867548,
-40.5430944022758));
#259778=CARTESIAN_POINT('Ctrl Pts',(-44.2311921171808,-56.3362675100036,
-40.5498666179945));
#259779=CARTESIAN_POINT('Ctrl Pts',(-44.2599977007373,-56.3367129587916,
-40.5636298486377));
#259780=CARTESIAN_POINT('Ctrl Pts',(-44.2743541649932,-56.3372884158027,
-40.5706510752088));
#259781=CARTESIAN_POINT('Ctrl Pts',(-44.3029357424357,-56.3391317429585,
-40.5849473061899));
#259782=CARTESIAN_POINT('Ctrl Pts',(-44.3456316213443,-56.3429350642169,
-40.6067818596389));
#259783=CARTESIAN_POINT('Ctrl Pts',(-44.4018650235691,-56.3520939287388,
-40.6374236066311));
#259784=CARTESIAN_POINT('Ctrl Pts',(-44.4574103376146,-56.3653147883305,
-40.6695718678152));
#259785=CARTESIAN_POINT('Ctrl Pts',(-44.4849466005937,-56.3732907222196,
-40.686147922621));
#259786=CARTESIAN_POINT('Ctrl Pts',(-44.512374392093,-56.3819617528141,
-40.7029840503412));
#259787=CARTESIAN_POINT('Ctrl Pts',(-44.5260289861432,-56.3866462995878,
-40.7115304197201));
#259788=CARTESIAN_POINT('Ctrl Pts',(-44.5529609776699,-56.3966203919845,
-40.7287150345567));
#259789=CARTESIAN_POINT('Ctrl Pts',(-44.5662873943758,-56.4019250012471,
-40.737383176176));
#259790=CARTESIAN_POINT('Ctrl Pts',(-44.6058068395674,-56.4187668411382,
-40.7635834132132));
#259791=CARTESIAN_POINT('Ctrl Pts',(-44.6315615859976,-56.4312362585519,
-40.7813233152079));
#259792=CARTESIAN_POINT('Ctrl Pts',(-44.6693071486035,-56.4518014713652,
-40.8083384498991));
#259793=CARTESIAN_POINT('Ctrl Pts',(-44.6817372625133,-56.458965010373,
-40.8174084081892));
#259794=CARTESIAN_POINT('Ctrl Pts',(-44.7063132537473,-56.473929075182,
-40.8356956250034));
#259795=CARTESIAN_POINT('Ctrl Pts',(-44.7183832523531,-56.4816832398284,
-40.8448563495594));
#259796=CARTESIAN_POINT('Ctrl Pts',(-44.7538754102704,-56.505703003501,
-40.8723327540241));
#259797=CARTESIAN_POINT('Ctrl Pts',(-44.7766465418209,-56.5227549736834,
-40.8906872015444));
#259798=CARTESIAN_POINT('Ctrl Pts',(-44.8204030914552,-56.5588699415109,
-40.9274359243417));
#259799=CARTESIAN_POINT('Ctrl Pts',(-44.851893062885,-56.5874690797881,
-40.9550350105826));
#259800=CARTESIAN_POINT('Ctrl Pts',(-44.8813802932551,-56.6183507815631,
-40.982690555711));
#259801=CARTESIAN_POINT('Ctrl Pts',(-44.9005867815582,-56.6394533348067,
-41.0011404791447));
#259802=CARTESIAN_POINT('Ctrl Pts',(-44.9099603095753,-56.6502571213647,
-41.0103678872986));
#259803=CARTESIAN_POINT('Ctrl Pts',(-44.9236872082217,-56.6668706184025,
-41.0242310114538));
#259804=CARTESIAN_POINT('Ctrl Pts',(-44.9282031316495,-56.6724722064122,
-41.0288518918758));
#259805=CARTESIAN_POINT('Ctrl Pts',(-44.9370720489983,-56.6837477093971,
-41.038048314582));
#259806=CARTESIAN_POINT('Ctrl Pts',(-44.9414338933841,-56.6894322363092,
-41.0426327511372));
#259807=CARTESIAN_POINT('Ctrl Pts',(-44.9542884395491,-56.7066066663578,
-41.0563299560217));
#259808=CARTESIAN_POINT('Ctrl Pts',(-44.9625629539304,-56.7182326826763,
-41.0653994431984));
#259809=CARTESIAN_POINT('Ctrl Pts',(-44.9864941991718,-56.7536111473724,
-41.0924067111081));
#259810=CARTESIAN_POINT('Ctrl Pts',(-45.0086645271567,-56.7900134244028,
-41.1190329135161));
#259811=CARTESIAN_POINT('Ctrl Pts',(-45.034704630644,-56.8405768845403,
-41.1537712607408));
#259812=CARTESIAN_POINT('Ctrl Pts',(-45.0465408860903,-56.8665423758261,
-41.1708862092094));
#259813=CARTESIAN_POINT('Ctrl Pts',(-45.0577761134165,-56.8928546179869,
-41.1878727246706));
#259814=CARTESIAN_POINT('Ctrl Pts',(-45.0630901582258,-56.906176087846,
-41.1962967595746));
#259815=CARTESIAN_POINT('Ctrl Pts',(-45.0731156002939,-56.9332061371524,
-41.2130345018643));
#259816=CARTESIAN_POINT('Ctrl Pts',(-45.0777961712447,-56.9468340019015,
-41.2212978165198));
#259817=CARTESIAN_POINT('Ctrl Pts',(-45.0907786540592,-56.9878560258786,
-41.2456540007716));
#259818=CARTESIAN_POINT('Ctrl Pts',(-45.0980724298404,-57.0154910056487,
-41.2613826498774));
#259819=CARTESIAN_POINT('Ctrl Pts',(-45.1099506000897,-57.0712899900431,
-41.2918166667949));
#259820=CARTESIAN_POINT('Ctrl Pts',(-45.1168338059478,-57.11354441615,-41.3138815317038));
#259821=CARTESIAN_POINT('Ctrl Pts',(-45.1206309792415,-57.1564190282566,
-41.3347987762303));
#259822=CARTESIAN_POINT('Ctrl Pts',(-45.1224627479043,-57.1851396939165,
-41.3484832320635));
#259823=CARTESIAN_POINT('Ctrl Pts',(-45.1230291819396,-57.199581674993,
-41.3552011986272));
#259824=CARTESIAN_POINT('Ctrl Pts',(-45.1234439819388,-57.2285619504273,
-41.3683510337761));
#259825=CARTESIAN_POINT('Ctrl Pts',(-45.1232917301137,-57.2429904040975,
-41.3747335054784));
#259826=CARTESIAN_POINT('Ctrl Pts',(-45.122279779691,-57.2717682086368,
-41.3871399525693));
#259827=CARTESIAN_POINT('Ctrl Pts',(-45.1196997436484,-57.3147947598186,
-41.4052018313649));
#259828=CARTESIAN_POINT('Ctrl Pts',(-45.1120557453653,-57.3716084168758,
-41.4271228345082));
#259829=CARTESIAN_POINT('Ctrl Pts',(-45.1031553338884,-57.4137999065974,
-41.4419446800329));
#259830=CARTESIAN_POINT('Ctrl Pts',(-45.09650693546,-57.4418330021969,-41.4514615780937));
#259831=CARTESIAN_POINT('Ctrl Pts',(-45.092823442876,-57.4558081403435,
-41.4560396298995));
#259832=CARTESIAN_POINT('Ctrl Pts',(-45.08473584999,-57.4836385233421,-41.464818484644));
#259833=CARTESIAN_POINT('Ctrl Pts',(-45.0803094818206,-57.4975537933777,
-41.4690360581021));
#259834=CARTESIAN_POINT('Ctrl Pts',(-45.0708158371377,-57.5249803724867,
-41.4770040232021));
#259835=CARTESIAN_POINT('Ctrl Pts',(-45.060662137239,-57.5520858826269,
-41.4845331733926));
#259836=CARTESIAN_POINT('Ctrl Pts',(-45.0434887903859,-57.591755117417,
-41.4945182619959));
#259837=CARTESIAN_POINT('Ctrl Pts',(-45.0243848727922,-57.6304534586566,
-41.5032105668009));
#259838=CARTESIAN_POINT('Ctrl Pts',(-45.0033512023575,-57.6681778817651,
-41.51061115159));
#259839=CARTESIAN_POINT('Ctrl Pts',(-44.9880328234845,-57.692673879575,
-41.5146787869643));
#259840=CARTESIAN_POINT('Ctrl Pts',(-44.9720568870916,-57.7168380825906,
-41.5183074012753));
#259841=CARTESIAN_POINT('Ctrl Pts',(-44.9637457009402,-57.7287466936453,
-41.5199012977462));
#259842=CARTESIAN_POINT('Ctrl Pts',(-44.9464287138105,-57.7522550306847,
-41.5226441863212));
#259843=CARTESIAN_POINT('Ctrl Pts',(-44.9374830238235,-57.7637718882179,
-41.5237830976086));
#259844=CARTESIAN_POINT('Ctrl Pts',(-44.9099214446927,-57.7974515399035,
-41.5264929611258));
#259845=CARTESIAN_POINT('Ctrl Pts',(-44.8905204729439,-57.8188493934961,
-41.5273772161885));
#259846=CARTESIAN_POINT('Ctrl Pts',(-44.8497318000032,-57.8595330722204,
-41.5273307191807));
#259847=CARTESIAN_POINT('Ctrl Pts',(-44.8283374647208,-57.878828810327,
-41.5264014189239));
#259848=CARTESIAN_POINT('Ctrl Pts',(-44.7947479986672,-57.9061820008563,
-41.5236391765087));
#259849=CARTESIAN_POINT('Ctrl Pts',(-44.7832945060713,-57.9150388128137,
-41.5224889540588));
#259850=CARTESIAN_POINT('Ctrl Pts',(-44.7657408175914,-57.9279147771907,
-41.5204166102647));
#259851=CARTESIAN_POINT('Ctrl Pts',(-44.7598217545323,-57.9321421746299,
-41.5196671186517));
#259852=CARTESIAN_POINT('Ctrl Pts',(-44.7478629508254,-57.9404557426351,
-41.5180519716851));
#259853=CARTESIAN_POINT('Ctrl Pts',(-44.7297025277655,-57.9527400844071,
-41.5154481926132));
#259854=CARTESIAN_POINT('Ctrl Pts',(-44.711220794734,-57.9642369190977,
-41.5123523449538));
#259855=CARTESIAN_POINT('Ctrl Pts',(-44.6862770262529,-57.9788987855805,
-41.5077941640223));
#259856=CARTESIAN_POINT('Ctrl Pts',(-44.6484202704456,-57.9998814948776,
-41.5003121274858));
#259857=CARTESIAN_POINT('Ctrl Pts',(-44.5962108390282,-58.0238874022289,
-41.4877980263462));
#259858=CARTESIAN_POINT('Ctrl Pts',(-44.5557649369164,-58.0389385823793,
-41.4765186283493));
#259859=CARTESIAN_POINT('Ctrl Pts',(-44.5285120653069,-58.048310487242,
-41.4685735203231));
#259860=CARTESIAN_POINT('Ctrl Pts',(-44.5147341086114,-58.0526671867402,
-41.4643859028639));
#259861=CARTESIAN_POINT('Ctrl Pts',(-44.4869140318333,-58.0607029371288,
-41.4555883503401));
#259862=CARTESIAN_POINT('Ctrl Pts',(-44.4728027150897,-58.0643973546439,
-41.4509544537452));
#259863=CARTESIAN_POINT('Ctrl Pts',(-44.4304531283686,-58.0743536715507,
-41.4365378845966));
#259864=CARTESIAN_POINT('Ctrl Pts',(-44.3879697631396,-58.0821103913619,
-41.4210702443308));
#259865=CARTESIAN_POINT('Ctrl Pts',(-44.3452880889881,-58.0866896268435,
-41.4040725286766));
#259866=CARTESIAN_POINT('Ctrl Pts',(-44.3025416355467,-58.090217180745,
-41.3865671155567));
#259867=CARTESIAN_POINT('Ctrl Pts',(-44.2739489581488,-58.0911687787978,
-41.3742170239002));
#259868=CARTESIAN_POINT('Ctrl Pts',(-44.2309555122234,-58.090491506171,
-41.3546803180427));
#259869=CARTESIAN_POINT('Ctrl Pts',(-44.2165895018292,-58.0899123697243,
-41.347990487553));
#259870=CARTESIAN_POINT('Ctrl Pts',(-44.1950278537333,-58.0885113544661,
-41.337705180963));
#259871=CARTESIAN_POINT('Ctrl Pts',(-44.1878319550126,-58.0879547296283,
-41.3342316293533));
#259872=CARTESIAN_POINT('Ctrl Pts',(-44.1734279164018,-58.0866616594573,
-41.3271961709002));
#259873=CARTESIAN_POINT('Ctrl Pts',(-44.1662260389348,-58.0859253983809,
-41.3236371482021));
#259874=CARTESIAN_POINT('Ctrl Pts',(-44.130389101081,-58.0818150523559,
-41.3057210105631));
#259875=CARTESIAN_POINT('Ctrl Pts',(-44.073848260417,-58.0724828543971,
-41.2761395013722));
#259876=CARTESIAN_POINT('Ctrl Pts',(-44.0188545174212,-58.0578491440998,
-41.2447838757269));
#259877=CARTESIAN_POINT('Ctrl Pts',(-43.9646246641704,-58.0405931079736,
-41.2125419608827));
#259878=CARTESIAN_POINT('Ctrl Pts',(-43.9378880325505,-58.0306505669816,
-41.1959746665064));
#259879=CARTESIAN_POINT('Ctrl Pts',(-43.9049634769563,-58.0165631445999,
-41.174705886574));
#259880=CARTESIAN_POINT('Ctrl Pts',(-43.898399460067,-58.0136596367661,
-41.1704209658528));
#259881=CARTESIAN_POINT('Ctrl Pts',(-43.8853286348063,-58.0076886655405,
-41.1617993561325));
#259882=CARTESIAN_POINT('Ctrl Pts',(-43.8788088737381,-58.0046144513738,
-41.157453730181));
#259883=CARTESIAN_POINT('Ctrl Pts',(-43.8593967360427,-57.9951717320096,
-41.1443784829743));
#259884=CARTESIAN_POINT('Ctrl Pts',(-43.8466719188398,-57.9885954718361,
-41.1356253645631));
#259885=CARTESIAN_POINT('Ctrl Pts',(-43.8341420587998,-57.9817357678076,
-41.1268248734572));
#259886=CARTESIAN_POINT('',(-45.4581751231188,-55.7156010961851,-39.3126317220031));
#259887=CARTESIAN_POINT('',(-45.3904396609892,-55.7772425608068,-39.4382820396906));
#259888=CARTESIAN_POINT('',(-45.4581751231188,-55.7156010961851,-39.3126317220031));
#259889=CARTESIAN_POINT('Origin',(-44.3987054398481,-57.592449415963,-39.4571364862761));
#259890=CARTESIAN_POINT('Ctrl Pts',(-45.8699710781849,-56.0109010507348,
-39.4567769182892));
#259891=CARTESIAN_POINT('Ctrl Pts',(-45.8053259834915,-55.968605507759,
-39.4535705001808));
#259892=CARTESIAN_POINT('Ctrl Pts',(-45.7383889969054,-55.9298524990358,
-39.4505766434469));
#259893=CARTESIAN_POINT('Ctrl Pts',(-45.5794955533779,-55.8490954403259,
-39.4442200262513));
#259894=CARTESIAN_POINT('Ctrl Pts',(-45.4862186035378,-55.809766049426,
-39.4410295384064));
#259895=CARTESIAN_POINT('Ctrl Pts',(-45.3904396609892,-55.7772425608068,
-39.4382820396906));
#259896=CARTESIAN_POINT('Ctrl Pts',(-45.6739227548714,-55.5192637629146,
-38.912416567246));
#259897=CARTESIAN_POINT('Ctrl Pts',(-45.7067749877366,-55.5369855856674,
-38.9214216121434));
#259898=CARTESIAN_POINT('Ctrl Pts',(-45.7392219877792,-55.5555212114617,
-38.9304915704333));
#259899=CARTESIAN_POINT('Ctrl Pts',(-45.8033556832395,-55.5942722159849,
-38.9487787872477));
#259900=CARTESIAN_POINT('Ctrl Pts',(-45.8348443691401,-55.6143675312756,
-38.9579395118016));
#259901=CARTESIAN_POINT('Ctrl Pts',(-45.9274099842789,-55.6766589025305,
-38.9854159162722));
#259902=CARTESIAN_POINT('Ctrl Pts',(-45.9867610865919,-55.7209353156014,
-39.0037703637879));
#259903=CARTESIAN_POINT('Ctrl Pts',(-46.1007337830098,-55.8148102393793,
-39.0405190865864));
#259904=CARTESIAN_POINT('Ctrl Pts',(-46.155375425224,-55.8644173763685,
-39.0589184916404));
#259905=CARTESIAN_POINT('Ctrl Pts',(-46.2338037269528,-55.9428521307486,
-39.0865551957989));
#259906=CARTESIAN_POINT('Ctrl Pts',(-46.259356574729,-55.9696687352924,
-39.0957737179551));
#259907=CARTESIAN_POINT('Ctrl Pts',(-46.309266807939,-56.024663053365,-39.1142236413887));
#259908=CARTESIAN_POINT('Ctrl Pts',(-46.3336138177017,-56.0528284109483,
-39.1234510495426));
#259909=CARTESIAN_POINT('Ctrl Pts',(-46.3692509284248,-56.0961546965834,
-39.1373141736981));
#259910=CARTESIAN_POINT('Ctrl Pts',(-46.3809719555493,-56.1107655250657,
-39.14193505412));
#259911=CARTESIAN_POINT('Ctrl Pts',(-46.4039850968433,-56.1401806715041,
-39.1511314768264));
#259912=CARTESIAN_POINT('Ctrl Pts',(-46.4153001903629,-56.1550126624777,
-39.1557159133814));
#259913=CARTESIAN_POINT('Ctrl Pts',(-46.4486370096884,-56.1998310060262,
-39.1694131182658));
#259914=CARTESIAN_POINT('Ctrl Pts',(-46.4700835091466,-56.2301795317326,
-39.1784826054425));
#259915=CARTESIAN_POINT('Ctrl Pts',(-46.5320719136859,-56.3225583984772,
-39.2054898733524));
#259916=CARTESIAN_POINT('Ctrl Pts',(-46.5703035947222,-56.3859631579321,
-39.2232408562602));
#259917=CARTESIAN_POINT('Ctrl Pts',(-46.6230137301682,-56.4837650915426,
-39.2494851373609));
#259918=CARTESIAN_POINT('Ctrl Pts',(-46.6398105780351,-56.5168167317113,
-39.2581698041384));
#259919=CARTESIAN_POINT('Ctrl Pts',(-46.6718446885168,-56.5838294931519,
-39.2754119185794));
#259920=CARTESIAN_POINT('Ctrl Pts',(-46.6870820302515,-56.617790568625,
-39.2839693714534));
#259921=CARTESIAN_POINT('Ctrl Pts',(-46.7159729830272,-56.6866360545619,
-39.3009558869148));
#259922=CARTESIAN_POINT('Ctrl Pts',(-46.7296188023799,-56.7214992889704,
-39.3093799218186));
#259923=CARTESIAN_POINT('Ctrl Pts',(-46.7553216997642,-56.7922546384013,
-39.3261176641085));
#259924=CARTESIAN_POINT('Ctrl Pts',(-46.7672996943011,-56.8279354881579,
-39.3343809787628));
#259925=CARTESIAN_POINT('Ctrl Pts',(-46.8004530502947,-56.9353633959568,
-39.358737163018));
#259926=CARTESIAN_POINT('Ctrl Pts',(-46.8189795501832,-57.0077635587999,
-39.3744658121213));
#259927=CARTESIAN_POINT('Ctrl Pts',(-46.848916211803,-57.1540080946302,
-39.4048998290393));
#259928=CARTESIAN_POINT('Ctrl Pts',(-46.8603369445408,-57.2278698672909,
-39.4196100581687));
#259929=CARTESIAN_POINT('Ctrl Pts',(-46.8720664744741,-57.3397812895282,
-39.4409093640372));
#259930=CARTESIAN_POINT('Ctrl Pts',(-46.875074749658,-57.3772756893033,
-39.4478819384746));
#259931=CARTESIAN_POINT('Ctrl Pts',(-46.8792542953452,-57.4526370309597,
-39.4615663943076));
#259932=CARTESIAN_POINT('Ctrl Pts',(-46.8804258736835,-57.4905390832846,
-39.4682843608713));
#259933=CARTESIAN_POINT('Ctrl Pts',(-46.8808837743635,-57.5666104373409,
-39.4814341960201));
#259934=CARTESIAN_POINT('Ctrl Pts',(-46.8801708637706,-57.604491394965,
-39.4878166677226));
#259935=CARTESIAN_POINT('Ctrl Pts',(-46.8768913879562,-57.6800597985945,
-39.5002231148134));
#259936=CARTESIAN_POINT('Ctrl Pts',(-46.8743246637802,-57.7177284992744,
-39.5062438407196));
#259937=CARTESIAN_POINT('Ctrl Pts',(-46.863867568228,-57.8303908432586,
-39.5237649596504));
#259938=CARTESIAN_POINT('Ctrl Pts',(-46.8532263654434,-57.9050414873811,
-39.5347254895779));
#259939=CARTESIAN_POINT('Ctrl Pts',(-46.8317335315027,-58.0163268447592,
-39.5500873410526));
#259940=CARTESIAN_POINT('Ctrl Pts',(-46.8236459543104,-58.0533066811291,
-39.5550278422771));
#259941=CARTESIAN_POINT('Ctrl Pts',(-46.8055990109883,-58.1270324939451,
-39.5645447403379));
#259942=CARTESIAN_POINT('Ctrl Pts',(-46.7956339676918,-58.1637938532181,
-39.5691227921436));
#259943=CARTESIAN_POINT('Ctrl Pts',(-46.7738161327052,-58.2370162077018,
-39.5779016468881));
#259944=CARTESIAN_POINT('Ctrl Pts',(-46.7619036278491,-58.2736352268715,
-39.5821192203466));
#259945=CARTESIAN_POINT('Ctrl Pts',(-46.7364059718256,-58.3458255995332,
-39.5900871854462));
#259946=CARTESIAN_POINT('Ctrl Pts',(-46.7227943874693,-58.3815079294473,
-39.593852026583));
#259947=CARTESIAN_POINT('Ctrl Pts',(-46.6938810604275,-58.4520118571144,
-39.6009443874688));
#259948=CARTESIAN_POINT('Ctrl Pts',(-46.6785776252269,-58.4868413763864,
-39.6042729713841));
#259949=CARTESIAN_POINT('Ctrl Pts',(-46.6462897337504,-58.5556617200885,
-39.6104989383907));
#259950=CARTESIAN_POINT('Ctrl Pts',(-46.629305264578,-58.5896525381261,
-39.6133963175589));
#259951=CARTESIAN_POINT('Ctrl Pts',(-46.5936553532051,-58.6567954587996,
-39.6187605717742));
#259952=CARTESIAN_POINT('Ctrl Pts',(-46.5749899237926,-58.6899475678396,
-39.6212274496765));
#259953=CARTESIAN_POINT('Ctrl Pts',(-46.5359657438849,-58.7554068733743,
-39.6257281334421));
#259954=CARTESIAN_POINT('Ctrl Pts',(-46.515607032986,-58.7877140896313,
-39.6277619492082));
#259955=CARTESIAN_POINT('Ctrl Pts',(-46.4731710833873,-58.8514710047945,
-39.6313905635194));
#259956=CARTESIAN_POINT('Ctrl Pts',(-46.4511086137466,-58.8829006319494,
-39.6329844599904));
#259957=CARTESIAN_POINT('Ctrl Pts',(-46.4051673201273,-58.9449633016888,
-39.6357273485653));
#259958=CARTESIAN_POINT('Ctrl Pts',(-46.381447994276,-58.975377588932,-39.6368662598532));
#259959=CARTESIAN_POINT('Ctrl Pts',(-46.3084068909562,-59.0643493136613,
-39.639576123369));
#259960=CARTESIAN_POINT('Ctrl Pts',(-46.2570407846103,-59.1209150453975,
-39.6404603784326));
#259961=CARTESIAN_POINT('Ctrl Pts',(-46.1491379755941,-59.228544463199,
-39.6404138814247));
#259962=CARTESIAN_POINT('Ctrl Pts',(-46.0925836555154,-59.2796343044913,
-39.6394845811683));
#259963=CARTESIAN_POINT('Ctrl Pts',(-46.003852943763,-59.3521266125548,
-39.6367223387528));
#259964=CARTESIAN_POINT('Ctrl Pts',(-45.9736068078661,-59.3756113554054,
-39.6355721163029));
#259965=CARTESIAN_POINT('Ctrl Pts',(-45.9272656961273,-59.4097723546528,
-39.6334997725088));
#259966=CARTESIAN_POINT('Ctrl Pts',(-45.9116419215573,-59.4209912820171,
-39.6327502808957));
#259967=CARTESIAN_POINT('Ctrl Pts',(-45.8800804794677,-59.4430610802668,
-39.6311351339295));
#259968=CARTESIAN_POINT('Ctrl Pts',(-45.8641077773929,-59.4539347618601,
-39.6302673980329));
#259969=CARTESIAN_POINT('Ctrl Pts',(-45.8159067176779,-59.4858696807562,
-39.6274990247155));
#259970=CARTESIAN_POINT('Ctrl Pts',(-45.7834097108732,-59.5062438963941,
-39.6254355071979));
#259971=CARTESIAN_POINT('Ctrl Pts',(-45.717633106262,-59.5452481912826,
-39.6208773262667));
#259972=CARTESIAN_POINT('Ctrl Pts',(-45.6843658495255,-59.5638704323978,
-39.6183834291471));
#259973=CARTESIAN_POINT('Ctrl Pts',(-45.5834449288538,-59.6171384125673,
-39.6102664280093));
#259974=CARTESIAN_POINT('Ctrl Pts',(-45.5146744626452,-59.6491908713697,
-39.6040093949256));
#259975=CARTESIAN_POINT('Ctrl Pts',(-45.409303365533,-59.6921244665012,
-39.5933617316812));
#259976=CARTESIAN_POINT('Ctrl Pts',(-45.3738098009101,-59.7055766782111,
-39.5896017905935));
#259977=CARTESIAN_POINT('Ctrl Pts',(-45.3020778813705,-59.7307512119864,
-39.5816566825671));
#259978=CARTESIAN_POINT('Ctrl Pts',(-45.2658207311094,-59.7424779859238,
-39.5774690651077));
#259979=CARTESIAN_POINT('Ctrl Pts',(-45.1926264675053,-59.7641596016776,
-39.5686715125846));
#259980=CARTESIAN_POINT('Ctrl Pts',(-45.1555073907618,-59.7741562512685,
-39.5640376159893));
#259981=CARTESIAN_POINT('Ctrl Pts',(-45.0812568479429,-59.7921790564438,
-39.5544265698906));
#259982=CARTESIAN_POINT('Ctrl Pts',(-45.04408172978,-59.8002277891036,-39.5494458391365));
#259983=CARTESIAN_POINT('Ctrl Pts',(-44.9696261062542,-59.8144410677077,
-39.5391390505826));
#259984=CARTESIAN_POINT('Ctrl Pts',(-44.9323469822025,-59.8206061841119,
-39.5338133285981));
#259985=CARTESIAN_POINT('Ctrl Pts',(-44.8576879123993,-59.8310833805954,
-39.5228216573624));
#259986=CARTESIAN_POINT('Ctrl Pts',(-44.8203079610257,-59.8353953605365,
-39.5171556909205));
#259987=CARTESIAN_POINT('Ctrl Pts',(-44.7080184564225,-59.8455760612674,
-39.4996502778007));
#259988=CARTESIAN_POINT('Ctrl Pts',(-44.6329372249224,-59.8486931621852,
-39.4873001861445));
#259989=CARTESIAN_POINT('Ctrl Pts',(-44.5200834441659,-59.8478515133141,
-39.4677634802869));
#259990=CARTESIAN_POINT('Ctrl Pts',(-44.4823810871712,-59.8466449718289,
-39.4610736497973));
#259991=CARTESIAN_POINT('Ctrl Pts',(-44.4258051079382,-59.8434394706745,
-39.4507883432074));
#259992=CARTESIAN_POINT('Ctrl Pts',(-44.4069254589855,-59.8421361346926,
-39.4473147915973));
#259993=CARTESIAN_POINT('Ctrl Pts',(-44.3691376542581,-59.8390581625153,
-39.4402793331445));
#259994=CARTESIAN_POINT('Ctrl Pts',(-44.3502459350849,-59.8372838734483,
-39.4367203104461));
#259995=CARTESIAN_POINT('Ctrl Pts',(-44.2938476169342,-59.8312836889756,
-39.4259706278629));
#259996=CARTESIAN_POINT('Ctrl Pts',(-44.2565162762141,-59.8263768596807,
-39.4186892629542));
#259997=CARTESIAN_POINT('Ctrl Pts',(-44.1823865424055,-59.8147890207299,
-39.4039021619013));
#259998=CARTESIAN_POINT('Ctrl Pts',(-44.14558648486,-59.8081083758143,-39.3963962058824));
#259999=CARTESIAN_POINT('Ctrl Pts',(-44.0359682134124,-59.785449432176,
-39.3735449917432));
#260000=CARTESIAN_POINT('Ctrl Pts',(-43.9639303529155,-59.7668593120831,
-39.3578670379715));
#260001=CARTESIAN_POINT('Ctrl Pts',(-43.8219159040518,-59.7227861654644,
-39.3256251231267));
#260002=CARTESIAN_POINT('Ctrl Pts',(-43.7519290534068,-59.6972943066161,
-39.3090578287532));
#260003=CARTESIAN_POINT('Ctrl Pts',(-43.665783177736,-59.6610675807532,
-39.2877890488175));
#260004=CARTESIAN_POINT('Ctrl Pts',(-43.6486106666635,-59.653596197985,
-39.2835041280971));
#260005=CARTESIAN_POINT('Ctrl Pts',(-43.6144193015917,-59.6382222359849,
-39.2748825183767));
#260006=CARTESIAN_POINT('Ctrl Pts',(-43.597366582891,-59.6303022352814,
-39.2705368924251));
#260007=CARTESIAN_POINT('Ctrl Pts',(-43.5465994182958,-59.6059619032979,
-39.2574616452183));
#260008=CARTESIAN_POINT('Ctrl Pts',(-43.5133293006631,-59.588993111175,
-39.2487085268073));
#260009=CARTESIAN_POINT('Ctrl Pts',(-43.4805771074156,-59.5712767529309,
-39.2399080357013));
#260010=CARTESIAN_POINT('Ctrl Pts',(-45.4581748301254,-55.7156013628182,
-39.3126322655097));
#260011=CARTESIAN_POINT('Ctrl Pts',(-45.4867277088334,-55.7310183438428,
-39.321637310407));
#260012=CARTESIAN_POINT('Ctrl Pts',(-45.51492912057,-55.7471419461907,-39.330707268697));
#260013=CARTESIAN_POINT('Ctrl Pts',(-45.5706726136103,-55.7808477327706,
-39.3489944855113));
#260014=CARTESIAN_POINT('Ctrl Pts',(-45.5980425893803,-55.7983254858436,
-39.3581552100656));
#260015=CARTESIAN_POINT('Ctrl Pts',(-45.6785029049759,-55.8524994362108,
-39.3856316145351));
#260016=CARTESIAN_POINT('Ctrl Pts',(-45.7300953831417,-55.8910015357548,
-39.4039860620517));
#260017=CARTESIAN_POINT('Ctrl Pts',(-45.8291752111236,-55.9726255533772,
-39.4407347848499));
#260018=CARTESIAN_POINT('Ctrl Pts',(-45.876679984022,-56.0157549785288,
-39.459134189904));
#260019=CARTESIAN_POINT('Ctrl Pts',(-45.9448695334179,-56.0839422557895,
-39.4867708940624));
#260020=CARTESIAN_POINT('Ctrl Pts',(-45.9670873402583,-56.1072544162851,
-39.4959894162187));
#260021=CARTESIAN_POINT('Ctrl Pts',(-46.0104852988087,-56.1550602795965,
-39.5144393396524));
#260022=CARTESIAN_POINT('Ctrl Pts',(-46.0316564280385,-56.1795432421045,
-39.5236667478063));
#260023=CARTESIAN_POINT('Ctrl Pts',(-46.0626463753838,-56.2172037362606,
-39.5375298719617));
#260024=CARTESIAN_POINT('Ctrl Pts',(-46.072839197582,-56.2299037017973,
-39.5421507523836));
#260025=CARTESIAN_POINT('Ctrl Pts',(-46.0928523442025,-56.2554714237357,
-39.55134717509));
#260026=CARTESIAN_POINT('Ctrl Pts',(-46.1026926512335,-56.268363234494,
-39.555931611645));
#260027=CARTESIAN_POINT('Ctrl Pts',(-46.1316851735074,-56.3073182946572,
-39.5696288165295));
#260028=CARTESIAN_POINT('Ctrl Pts',(-46.1503378904843,-56.3336957698022,
-39.5786983037061));
#260029=CARTESIAN_POINT('Ctrl Pts',(-46.2042543586894,-56.4139848320304,
-39.605705571616));
#260030=CARTESIAN_POINT('Ctrl Pts',(-46.2375119613918,-56.4690888109481,
-39.6234565545238));
#260031=CARTESIAN_POINT('Ctrl Pts',(-46.2833712877372,-56.5540826662774,
-39.6497008356246));
#260032=CARTESIAN_POINT('Ctrl Pts',(-46.2979862913122,-56.5828052175225,
-39.658385502402));
#260033=CARTESIAN_POINT('Ctrl Pts',(-46.3258619629745,-56.6410393597078,
-39.6756276168431));
#260034=CARTESIAN_POINT('Ctrl Pts',(-46.3391226997695,-56.6705509109048,
-39.684185069717));
#260035=CARTESIAN_POINT('Ctrl Pts',(-46.3642688672173,-56.7303750814786,
-39.7011715851784));
#260036=CARTESIAN_POINT('Ctrl Pts',(-46.3761475143767,-56.7606693003541,
-39.7095956200823));
#260037=CARTESIAN_POINT('Ctrl Pts',(-46.3985252181961,-56.8221504988681,
-39.7263333623721));
#260038=CARTESIAN_POINT('Ctrl Pts',(-46.408955426727,-56.8531539030601,
-39.7345966770267));
#260039=CARTESIAN_POINT('Ctrl Pts',(-46.43783053371,-56.9464971004833,-39.7589528612811));
#260040=CARTESIAN_POINT('Ctrl Pts',(-46.4539745690236,-57.0094025528851,
-39.774681510385));
#260041=CARTESIAN_POINT('Ctrl Pts',(-46.4800810185276,-57.1364635567237,
-39.8051155273028));
#260042=CARTESIAN_POINT('Ctrl Pts',(-46.4900526283019,-57.200634229788,
-39.8198257564322));
#260043=CARTESIAN_POINT('Ctrl Pts',(-46.5003179883916,-57.2978587411347,
-39.8411250623009));
#260044=CARTESIAN_POINT('Ctrl Pts',(-46.5029566336967,-57.3304319169396,
-39.8480976367382));
#260045=CARTESIAN_POINT('Ctrl Pts',(-46.5066382150844,-57.3959007554725,
-39.8617820925713));
#260046=CARTESIAN_POINT('Ctrl Pts',(-46.5076814421117,-57.4288269187661,
-39.8685000591349));
#260047=CARTESIAN_POINT('Ctrl Pts',(-46.5081302011228,-57.4949102391499,
-39.8816498942838));
#260048=CARTESIAN_POINT('Ctrl Pts',(-46.5075362064438,-57.5278169127684,
-39.8880323659863));
#260049=CARTESIAN_POINT('Ctrl Pts',(-46.5047376735305,-57.5934610145355,
-39.900438813077));
#260050=CARTESIAN_POINT('Ctrl Pts',(-46.5025329846453,-57.6261821585506,
-39.9064595389832));
#260051=CARTESIAN_POINT('Ctrl Pts',(-46.4935235433768,-57.7240452733633,
-39.923980657914));
#260052=CARTESIAN_POINT('Ctrl Pts',(-46.4843287087445,-57.788887590308,
-39.9349411878415));
#260053=CARTESIAN_POINT('Ctrl Pts',(-46.4657308186056,-57.885547740833,
-39.9503030393162));
#260054=CARTESIAN_POINT('Ctrl Pts',(-46.4587293129245,-57.9176670783696,
-39.9552435405408));
#260055=CARTESIAN_POINT('Ctrl Pts',(-46.4431000048223,-57.9817014504392,
-39.9647604386015));
#260056=CARTESIAN_POINT('Ctrl Pts',(-46.4344672805524,-58.0136298445192,
-39.9693384904073));
#260057=CARTESIAN_POINT('Ctrl Pts',(-46.4155616345504,-58.0772245465278,
-39.9781173451517));
#260058=CARTESIAN_POINT('Ctrl Pts',(-46.4052369418127,-58.1090280928419,
-39.9823349186101));
#260059=CARTESIAN_POINT('Ctrl Pts',(-46.383133741997,-58.1717240497799,
-39.9903028837099));
#260060=CARTESIAN_POINT('Ctrl Pts',(-46.3713323447936,-58.2027128491507,
-39.9940677248466));
#260061=CARTESIAN_POINT('Ctrl Pts',(-46.3462606561336,-58.263941687033,
-40.0011600857324));
#260062=CARTESIAN_POINT('Ctrl Pts',(-46.3329888995612,-58.2941886059125,
-40.0044886696476));
#260063=CARTESIAN_POINT('Ctrl Pts',(-46.3049844543585,-58.3539528281862,
-40.0107146366544));
#260064=CARTESIAN_POINT('Ctrl Pts',(-46.2902517545131,-58.3834701260217,
-40.0136120158225));
#260065=CARTESIAN_POINT('Ctrl Pts',(-46.2593254742523,-58.4417750834909,
-40.0189762700378));
#260066=CARTESIAN_POINT('Ctrl Pts',(-46.2431319049432,-58.4705627487002,
-40.0214431479402));
#260067=CARTESIAN_POINT('Ctrl Pts',(-46.2092731643552,-58.5274030440657,
-40.0259438317057));
#260068=CARTESIAN_POINT('Ctrl Pts',(-46.1916080274801,-58.5554556914203,
-40.0279776474719));
#260069=CARTESIAN_POINT('Ctrl Pts',(-46.1547842556146,-58.6108149789715,
-40.0316062617831));
#260070=CARTESIAN_POINT('Ctrl Pts',(-46.1356384378441,-58.6381041920218,
-40.033200158254));
#260071=CARTESIAN_POINT('Ctrl Pts',(-46.0957683692941,-58.6919894747804,
-40.0359430468289));
#260072=CARTESIAN_POINT('Ctrl Pts',(-46.0751825365968,-58.718395610803,
-40.0370819581167));
#260073=CARTESIAN_POINT('Ctrl Pts',(-46.0117876557102,-58.7956398681744,
-40.0397918216329));
#260074=CARTESIAN_POINT('Ctrl Pts',(-45.967201365203,-58.8447464810846,
-40.0406760766962));
#260075=CARTESIAN_POINT('Ctrl Pts',(-45.8735334871044,-58.9381766850286,
-40.0406295796883));
#260076=CARTESIAN_POINT('Ctrl Pts',(-45.8244366116702,-58.9825229863024,
-40.0397002794319));
#260077=CARTESIAN_POINT('Ctrl Pts',(-45.7474013767448,-59.045441272299,
-40.0369380370164));
#260078=CARTESIAN_POINT('Ctrl Pts',(-45.721141166836,-59.0658234260692,
-40.0357878145665));
#260079=CARTESIAN_POINT('Ctrl Pts',(-45.6809058772882,-59.0954698622353,
-40.0337154707725));
#260080=CARTESIAN_POINT('Ctrl Pts',(-45.6673404753058,-59.1052058837424,
-40.0329659791594));
#260081=CARTESIAN_POINT('Ctrl Pts',(-45.6399367594346,-59.1243579809134,
-40.0313508321932));
#260082=CARTESIAN_POINT('Ctrl Pts',(-45.6260680251864,-59.1337938500571,
-40.0304830962965));
#260083=CARTESIAN_POINT('Ctrl Pts',(-45.5842155891604,-59.1615052138478,
-40.0277147229792));
#260084=CARTESIAN_POINT('Ctrl Pts',(-45.5559980798161,-59.1791836959668,
-40.0256512054615));
#260085=CARTESIAN_POINT('Ctrl Pts',(-45.4988821335321,-59.2130249535731,
-40.0210930245302));
#260086=CARTESIAN_POINT('Ctrl Pts',(-45.4699944124056,-59.2291809279018,
-40.0185991274108));
#260087=CARTESIAN_POINT('Ctrl Pts',(-45.382357426366,-59.2753904813377,
-40.010482126273));
#260088=CARTESIAN_POINT('Ctrl Pts',(-45.3226363823857,-59.3031904383161,
-40.0042250931893));
#260089=CARTESIAN_POINT('Ctrl Pts',(-45.2311271265862,-59.3404191081965,
-39.9935774299448));
#260090=CARTESIAN_POINT('Ctrl Pts',(-45.2003022091057,-59.3520821754701,
-39.9898174888571));
#260091=CARTESIAN_POINT('Ctrl Pts',(-45.1380043106471,-59.3739049663185,
-39.9818723808308));
#260092=CARTESIAN_POINT('Ctrl Pts',(-45.1065150049296,-59.3840685449793,
-39.9776847633714));
#260093=CARTESIAN_POINT('Ctrl Pts',(-45.0429446216685,-59.4028558680827,
-39.9688872108481));
#260094=CARTESIAN_POINT('Ctrl Pts',(-45.0107054985878,-59.4115158121228,
-39.9642533142529));
#260095=CARTESIAN_POINT('Ctrl Pts',(-44.9462152798728,-59.4271237996878,
-39.9546422681542));
#260096=CARTESIAN_POINT('Ctrl Pts',(-44.9139262776317,-59.4340914281647,
-39.9496615374001));
#260097=CARTESIAN_POINT('Ctrl Pts',(-44.8492555669035,-59.4463896950644,
-39.9393547488463));
#260098=CARTESIAN_POINT('Ctrl Pts',(-44.8168750587066,-59.4517208300076,
-39.9340290268618));
#260099=CARTESIAN_POINT('Ctrl Pts',(-44.7520253206349,-59.4607731680205,
-39.923037355626));
#260100=CARTESIAN_POINT('Ctrl Pts',(-44.7195560858118,-59.4644942841012,
-39.9173713891842));
#260101=CARTESIAN_POINT('Ctrl Pts',(-44.6220166858359,-59.4732638501436,
-39.8998659760644));
#260102=CARTESIAN_POINT('Ctrl Pts',(-44.5567956923543,-59.4759216471728,
-39.8875158844081));
#260103=CARTESIAN_POINT('Ctrl Pts',(-44.4587593121986,-59.4751148625585,
-39.8679791785505));
#260104=CARTESIAN_POINT('Ctrl Pts',(-44.4260066021956,-59.4740413938938,
-39.861289348061));
#260105=CARTESIAN_POINT('Ctrl Pts',(-44.3768571744168,-59.4712186248072,
-39.8510040414711));
#260106=CARTESIAN_POINT('Ctrl Pts',(-44.3604556528324,-59.470073666511,
-39.8475304898609));
#260107=CARTESIAN_POINT('Ctrl Pts',(-44.3276275527921,-59.4673742726518,
-39.8404950314082));
#260108=CARTESIAN_POINT('Ctrl Pts',(-44.3112152529909,-59.465820149672,
-39.8369360087098));
#260109=CARTESIAN_POINT('Ctrl Pts',(-44.2622184211888,-59.4605695228838,
-39.8261863261265));
#260110=CARTESIAN_POINT('Ctrl Pts',(-44.2297857112555,-59.4562815511248,
-39.8189049612177));
#260111=CARTESIAN_POINT('Ctrl Pts',(-44.1653821501578,-59.4461645800485,
-39.804117860165));
#260112=CARTESIAN_POINT('Ctrl Pts',(-44.1334098533119,-59.4403358965057,
-39.796611904146));
#260113=CARTESIAN_POINT('Ctrl Pts',(-44.0381705489761,-59.4205767439822,
-39.7737606900069));
#260114=CARTESIAN_POINT('Ctrl Pts',(-43.9755797867482,-59.404377678535,
-39.758082736235));
#260115=CARTESIAN_POINT('Ctrl Pts',(-43.8521844802478,-59.3659924501046,
-39.7258408213904));
#260116=CARTESIAN_POINT('Ctrl Pts',(-43.7913710156582,-59.3437986068227,
-39.7092735270162));
#260117=CARTESIAN_POINT('Ctrl Pts',(-43.7165133999419,-59.3122676347018,
-39.6880047470813));
#260118=CARTESIAN_POINT('Ctrl Pts',(-43.7015909540668,-59.3057650997492,
-39.6837198263607));
#260119=CARTESIAN_POINT('Ctrl Pts',(-43.6718792626187,-59.2923855152665,
-39.6750982166404));
#260120=CARTESIAN_POINT('Ctrl Pts',(-43.6570605877876,-59.2854933075233,
-39.6707525906888));
#260121=CARTESIAN_POINT('Ctrl Pts',(-43.6129438349825,-59.2643127642054,
-39.657677343482));
#260122=CARTESIAN_POINT('Ctrl Pts',(-43.5840313825064,-59.2495482316173,
-39.6489242250709));
#260123=CARTESIAN_POINT('Ctrl Pts',(-43.5555683529588,-59.2341345733972,
-39.6401237339649));
#260124=CARTESIAN_POINT('',(-45.6739227569384,-55.519263759503,-38.9124165664198));
#260125=CARTESIAN_POINT('',(-45.6739227548714,-55.5192637629146,-38.912416567246));
#260126=CARTESIAN_POINT('',(-43.4805771074159,-59.5712767529304,-39.2399080357012));
#260127=CARTESIAN_POINT('Ctrl Pts',(-45.6739227574752,-55.5192637582493,
-38.9124165669282));
#260128=CARTESIAN_POINT('Ctrl Pts',(-45.7067749877369,-55.5369855856676,
-38.9214216121435));
#260129=CARTESIAN_POINT('Ctrl Pts',(-45.7392219877795,-55.5555212114618,
-38.9304915704334));
#260130=CARTESIAN_POINT('Ctrl Pts',(-45.8033556832395,-55.5942722159849,
-38.9487787872477));
#260131=CARTESIAN_POINT('Ctrl Pts',(-45.8348443691401,-55.6143675312756,
-38.9579395118016));
#260132=CARTESIAN_POINT('Ctrl Pts',(-45.9274099842789,-55.6766589025305,
-38.9854159162722));
#260133=CARTESIAN_POINT('Ctrl Pts',(-45.9867610865919,-55.7209353156014,
-39.0037703637879));
#260134=CARTESIAN_POINT('Ctrl Pts',(-46.1007337830098,-55.8148102393793,
-39.0405190865864));
#260135=CARTESIAN_POINT('Ctrl Pts',(-46.155375425224,-55.8644173763685,
-39.0589184916404));
#260136=CARTESIAN_POINT('Ctrl Pts',(-46.2338037269528,-55.9428521307486,
-39.0865551957989));
#260137=CARTESIAN_POINT('Ctrl Pts',(-46.259356574729,-55.9696687352924,
-39.0957737179551));
#260138=CARTESIAN_POINT('Ctrl Pts',(-46.309266807939,-56.024663053365,-39.1142236413887));
#260139=CARTESIAN_POINT('Ctrl Pts',(-46.3336138177017,-56.0528284109483,
-39.1234510495426));
#260140=CARTESIAN_POINT('Ctrl Pts',(-46.3692509284248,-56.0961546965834,
-39.1373141736981));
#260141=CARTESIAN_POINT('Ctrl Pts',(-46.3809719555493,-56.1107655250657,
-39.14193505412));
#260142=CARTESIAN_POINT('Ctrl Pts',(-46.4039850968433,-56.1401806715041,
-39.1511314768264));
#260143=CARTESIAN_POINT('Ctrl Pts',(-46.4153001903629,-56.1550126624777,
-39.1557159133814));
#260144=CARTESIAN_POINT('Ctrl Pts',(-46.4486370096884,-56.1998310060262,
-39.1694131182658));
#260145=CARTESIAN_POINT('Ctrl Pts',(-46.4700835091466,-56.2301795317326,
-39.1784826054425));
#260146=CARTESIAN_POINT('Ctrl Pts',(-46.5320719136859,-56.3225583984772,
-39.2054898733524));
#260147=CARTESIAN_POINT('Ctrl Pts',(-46.5703035947222,-56.3859631579321,
-39.2232408562602));
#260148=CARTESIAN_POINT('Ctrl Pts',(-46.6230137301682,-56.4837650915426,
-39.2494851373609));
#260149=CARTESIAN_POINT('Ctrl Pts',(-46.6398105780351,-56.5168167317113,
-39.2581698041384));
#260150=CARTESIAN_POINT('Ctrl Pts',(-46.6718446885168,-56.5838294931519,
-39.2754119185794));
#260151=CARTESIAN_POINT('Ctrl Pts',(-46.6870820302515,-56.617790568625,
-39.2839693714534));
#260152=CARTESIAN_POINT('Ctrl Pts',(-46.7159729830272,-56.6866360545619,
-39.3009558869148));
#260153=CARTESIAN_POINT('Ctrl Pts',(-46.7296188023799,-56.7214992889704,
-39.3093799218186));
#260154=CARTESIAN_POINT('Ctrl Pts',(-46.7553216997642,-56.7922546384013,
-39.3261176641085));
#260155=CARTESIAN_POINT('Ctrl Pts',(-46.7672996943011,-56.8279354881579,
-39.3343809787628));
#260156=CARTESIAN_POINT('Ctrl Pts',(-46.8004530502947,-56.9353633959568,
-39.358737163018));
#260157=CARTESIAN_POINT('Ctrl Pts',(-46.8189795501832,-57.0077635587999,
-39.3744658121213));
#260158=CARTESIAN_POINT('Ctrl Pts',(-46.848916211803,-57.1540080946302,
-39.4048998290393));
#260159=CARTESIAN_POINT('Ctrl Pts',(-46.8603369445408,-57.2278698672909,
-39.4196100581687));
#260160=CARTESIAN_POINT('Ctrl Pts',(-46.8720664744741,-57.3397812895282,
-39.4409093640372));
#260161=CARTESIAN_POINT('Ctrl Pts',(-46.875074749658,-57.3772756893033,
-39.4478819384746));
#260162=CARTESIAN_POINT('Ctrl Pts',(-46.8792542953452,-57.4526370309597,
-39.4615663943076));
#260163=CARTESIAN_POINT('Ctrl Pts',(-46.8804258736835,-57.4905390832846,
-39.4682843608713));
#260164=CARTESIAN_POINT('Ctrl Pts',(-46.8808837743635,-57.5666104373409,
-39.4814341960201));
#260165=CARTESIAN_POINT('Ctrl Pts',(-46.8801708637706,-57.604491394965,
-39.4878166677226));
#260166=CARTESIAN_POINT('Ctrl Pts',(-46.8768913879562,-57.6800597985945,
-39.5002231148134));
#260167=CARTESIAN_POINT('Ctrl Pts',(-46.8743246637802,-57.7177284992744,
-39.5062438407196));
#260168=CARTESIAN_POINT('Ctrl Pts',(-46.863867568228,-57.8303908432586,
-39.5237649596504));
#260169=CARTESIAN_POINT('Ctrl Pts',(-46.8532263654434,-57.9050414873811,
-39.5347254895779));
#260170=CARTESIAN_POINT('Ctrl Pts',(-46.8317335315027,-58.0163268447592,
-39.5500873410526));
#260171=CARTESIAN_POINT('Ctrl Pts',(-46.8236459543104,-58.0533066811291,
-39.5550278422771));
#260172=CARTESIAN_POINT('Ctrl Pts',(-46.8055990109883,-58.1270324939451,
-39.5645447403379));
#260173=CARTESIAN_POINT('Ctrl Pts',(-46.7956339676918,-58.1637938532181,
-39.5691227921436));
#260174=CARTESIAN_POINT('Ctrl Pts',(-46.7738161327052,-58.2370162077018,
-39.5779016468881));
#260175=CARTESIAN_POINT('Ctrl Pts',(-46.7619036278491,-58.2736352268715,
-39.5821192203466));
#260176=CARTESIAN_POINT('Ctrl Pts',(-46.7364059718256,-58.3458255995332,
-39.5900871854462));
#260177=CARTESIAN_POINT('Ctrl Pts',(-46.7227943874693,-58.3815079294473,
-39.593852026583));
#260178=CARTESIAN_POINT('Ctrl Pts',(-46.6938810604275,-58.4520118571144,
-39.6009443874688));
#260179=CARTESIAN_POINT('Ctrl Pts',(-46.6785776252269,-58.4868413763864,
-39.6042729713841));
#260180=CARTESIAN_POINT('Ctrl Pts',(-46.6462897337504,-58.5556617200885,
-39.6104989383907));
#260181=CARTESIAN_POINT('Ctrl Pts',(-46.629305264578,-58.5896525381261,
-39.6133963175589));
#260182=CARTESIAN_POINT('Ctrl Pts',(-46.5936553532051,-58.6567954587996,
-39.6187605717742));
#260183=CARTESIAN_POINT('Ctrl Pts',(-46.5749899237926,-58.6899475678396,
-39.6212274496765));
#260184=CARTESIAN_POINT('Ctrl Pts',(-46.5359657438849,-58.7554068733743,
-39.6257281334421));
#260185=CARTESIAN_POINT('Ctrl Pts',(-46.515607032986,-58.7877140896313,
-39.6277619492082));
#260186=CARTESIAN_POINT('Ctrl Pts',(-46.4731710833873,-58.8514710047945,
-39.6313905635194));
#260187=CARTESIAN_POINT('Ctrl Pts',(-46.4511086137466,-58.8829006319494,
-39.6329844599904));
#260188=CARTESIAN_POINT('Ctrl Pts',(-46.4051673201273,-58.9449633016888,
-39.6357273485653));
#260189=CARTESIAN_POINT('Ctrl Pts',(-46.381447994276,-58.975377588932,-39.6368662598532));
#260190=CARTESIAN_POINT('Ctrl Pts',(-46.3084068909562,-59.0643493136613,
-39.639576123369));
#260191=CARTESIAN_POINT('Ctrl Pts',(-46.2570407846103,-59.1209150453975,
-39.6404603784326));
#260192=CARTESIAN_POINT('Ctrl Pts',(-46.1491379755941,-59.228544463199,
-39.6404138814247));
#260193=CARTESIAN_POINT('Ctrl Pts',(-46.0925836555154,-59.2796343044913,
-39.6394845811683));
#260194=CARTESIAN_POINT('Ctrl Pts',(-46.003852943763,-59.3521266125548,
-39.6367223387528));
#260195=CARTESIAN_POINT('Ctrl Pts',(-45.9736068078661,-59.3756113554054,
-39.6355721163029));
#260196=CARTESIAN_POINT('Ctrl Pts',(-45.9272656961273,-59.4097723546528,
-39.6334997725088));
#260197=CARTESIAN_POINT('Ctrl Pts',(-45.9116419215573,-59.4209912820171,
-39.6327502808957));
#260198=CARTESIAN_POINT('Ctrl Pts',(-45.8800804794677,-59.4430610802668,
-39.6311351339295));
#260199=CARTESIAN_POINT('Ctrl Pts',(-45.8641077773929,-59.4539347618601,
-39.6302673980329));
#260200=CARTESIAN_POINT('Ctrl Pts',(-45.8159067176779,-59.4858696807562,
-39.6274990247155));
#260201=CARTESIAN_POINT('Ctrl Pts',(-45.7834097108732,-59.5062438963941,
-39.6254355071979));
#260202=CARTESIAN_POINT('Ctrl Pts',(-45.717633106262,-59.5452481912826,
-39.6208773262667));
#260203=CARTESIAN_POINT('Ctrl Pts',(-45.6843658495255,-59.5638704323978,
-39.6183834291471));
#260204=CARTESIAN_POINT('Ctrl Pts',(-45.5834449288538,-59.6171384125673,
-39.6102664280093));
#260205=CARTESIAN_POINT('Ctrl Pts',(-45.5146744626452,-59.6491908713697,
-39.6040093949256));
#260206=CARTESIAN_POINT('Ctrl Pts',(-45.409303365533,-59.6921244665012,
-39.5933617316812));
#260207=CARTESIAN_POINT('Ctrl Pts',(-45.3738098009101,-59.7055766782111,
-39.5896017905935));
#260208=CARTESIAN_POINT('Ctrl Pts',(-45.3020778813705,-59.7307512119864,
-39.5816566825671));
#260209=CARTESIAN_POINT('Ctrl Pts',(-45.2658207311094,-59.7424779859238,
-39.5774690651077));
#260210=CARTESIAN_POINT('Ctrl Pts',(-45.1926264675053,-59.7641596016776,
-39.5686715125846));
#260211=CARTESIAN_POINT('Ctrl Pts',(-45.1555073907618,-59.7741562512685,
-39.5640376159893));
#260212=CARTESIAN_POINT('Ctrl Pts',(-45.0812568479429,-59.7921790564438,
-39.5544265698906));
#260213=CARTESIAN_POINT('Ctrl Pts',(-45.04408172978,-59.8002277891036,-39.5494458391365));
#260214=CARTESIAN_POINT('Ctrl Pts',(-44.9696261062542,-59.8144410677077,
-39.5391390505826));
#260215=CARTESIAN_POINT('Ctrl Pts',(-44.9323469822025,-59.8206061841119,
-39.5338133285981));
#260216=CARTESIAN_POINT('Ctrl Pts',(-44.8576879123993,-59.8310833805954,
-39.5228216573624));
#260217=CARTESIAN_POINT('Ctrl Pts',(-44.8203079610257,-59.8353953605365,
-39.5171556909205));
#260218=CARTESIAN_POINT('Ctrl Pts',(-44.7080184564225,-59.8455760612674,
-39.4996502778007));
#260219=CARTESIAN_POINT('Ctrl Pts',(-44.6329372249224,-59.8486931621852,
-39.4873001861445));
#260220=CARTESIAN_POINT('Ctrl Pts',(-44.5200834441659,-59.8478515133141,
-39.4677634802869));
#260221=CARTESIAN_POINT('Ctrl Pts',(-44.4823810871712,-59.8466449718289,
-39.4610736497973));
#260222=CARTESIAN_POINT('Ctrl Pts',(-44.4258051079382,-59.8434394706745,
-39.4507883432074));
#260223=CARTESIAN_POINT('Ctrl Pts',(-44.4069254589855,-59.8421361346926,
-39.4473147915973));
#260224=CARTESIAN_POINT('Ctrl Pts',(-44.3691376542581,-59.8390581625153,
-39.4402793331445));
#260225=CARTESIAN_POINT('Ctrl Pts',(-44.3502459350849,-59.8372838734483,
-39.4367203104461));
#260226=CARTESIAN_POINT('Ctrl Pts',(-44.2938476169342,-59.8312836889756,
-39.4259706278629));
#260227=CARTESIAN_POINT('Ctrl Pts',(-44.2565162762141,-59.8263768596807,
-39.4186892629542));
#260228=CARTESIAN_POINT('Ctrl Pts',(-44.1823865424055,-59.8147890207299,
-39.4039021619013));
#260229=CARTESIAN_POINT('Ctrl Pts',(-44.14558648486,-59.8081083758143,-39.3963962058824));
#260230=CARTESIAN_POINT('Ctrl Pts',(-44.0359682134124,-59.785449432176,
-39.3735449917432));
#260231=CARTESIAN_POINT('Ctrl Pts',(-43.9639303529155,-59.7668593120831,
-39.3578670379715));
#260232=CARTESIAN_POINT('Ctrl Pts',(-43.8219159040518,-59.7227861654644,
-39.3256251231267));
#260233=CARTESIAN_POINT('Ctrl Pts',(-43.7519290534068,-59.6972943066161,
-39.3090578287532));
#260234=CARTESIAN_POINT('Ctrl Pts',(-43.665783177736,-59.6610675807532,
-39.2877890488175));
#260235=CARTESIAN_POINT('Ctrl Pts',(-43.6486106666635,-59.653596197985,
-39.2835041280971));
#260236=CARTESIAN_POINT('Ctrl Pts',(-43.6144193015917,-59.6382222359849,
-39.2748825183767));
#260237=CARTESIAN_POINT('Ctrl Pts',(-43.597366582891,-59.6303022352814,
-39.2705368924251));
#260238=CARTESIAN_POINT('Ctrl Pts',(-43.5465994182958,-59.6059619032979,
-39.2574616452183));
#260239=CARTESIAN_POINT('Ctrl Pts',(-43.5133293006631,-59.588993111175,
-39.2487085268073));
#260240=CARTESIAN_POINT('Ctrl Pts',(-43.4805771074159,-59.5712767529304,
-39.2399080357012));
#260241=CARTESIAN_POINT('',(-43.5555682511181,-59.2341350312479,-39.6401231904583));
#260242=CARTESIAN_POINT('',(-43.4805771074159,-59.5712767529304,-39.2399080357012));
#260243=CARTESIAN_POINT('Ctrl Pts',(-44.6028144607067,-59.4732023778567,
-39.8960586142665));
#260244=CARTESIAN_POINT('Ctrl Pts',(-44.5657362830796,-59.4749625407307,
-39.8890876965807));
#260245=CARTESIAN_POINT('Ctrl Pts',(-44.5286093371808,-59.4756901946432,
-39.8818983399833));
#260246=CARTESIAN_POINT('Ctrl Pts',(-44.4914381955716,-59.4753842969682,
-39.8744908703297));
#260247=CARTESIAN_POINT('Ctrl Pts',(-44.4587593954789,-59.4751153687477,
-39.8679786350438));
#260248=CARTESIAN_POINT('Ctrl Pts',(-44.4260066787541,-59.4740418999023,
-39.8612888045543));
#260249=CARTESIAN_POINT('Ctrl Pts',(-44.3932403868445,-59.4721600534981,
-39.8544319334943));
#260250=CARTESIAN_POINT('Ctrl Pts',(-44.3768572408897,-59.4712191302959,
-39.8510034979643));
#260251=CARTESIAN_POINT('Ctrl Pts',(-44.36045571594,-59.4700741717846,-39.8475299463542));
#260252=CARTESIAN_POINT('Ctrl Pts',(-44.3440416625521,-59.468724474598,
-39.8440122171279));
#260253=CARTESIAN_POINT('Ctrl Pts',(-44.3276276091642,-59.4673747774113,
-39.8404944879015));
#260254=CARTESIAN_POINT('Ctrl Pts',(-44.3112153059959,-59.4658206541325,
-39.8369354652031));
#260255=CARTESIAN_POINT('Ctrl Pts',(-44.2948830253781,-59.4640704448638,
-39.8333522376753));
#260256=CARTESIAN_POINT('Ctrl Pts',(-44.2622183820993,-59.4605700175345,
-39.8261857646199));
#260257=CARTESIAN_POINT('Ctrl Pts',(-44.2297857475685,-59.4562820537288,
-39.8189044177111));
#260258=CARTESIAN_POINT('Ctrl Pts',(-44.1975839604555,-59.4512235680695,
-39.8115108662318));
#260259=CARTESIAN_POINT('Ctrl Pts',(-44.1653823351036,-59.4461651078207,
-39.804117351893));
#260260=CARTESIAN_POINT('Ctrl Pts',(-44.1334101092193,-59.4403364490933,
-39.7966114142227));
#260261=CARTESIAN_POINT('Ctrl Pts',(-44.1016634287012,-59.4337500174524,
-39.7889942816371));
#260262=CARTESIAN_POINT('Ctrl Pts',(-44.0381699081893,-59.4205771210844,
-39.7737599782022));
#260263=CARTESIAN_POINT('Ctrl Pts',(-43.9755797709279,-59.4043781707976,
-39.7580821927283));
#260264=CARTESIAN_POINT('Ctrl Pts',(-43.913882105035,-59.3851855527201,
-39.741961235306));
#260265=CARTESIAN_POINT('Ctrl Pts',(-43.8521844391421,-59.3659929346427,
-39.7258402778837));
#260266=CARTESIAN_POINT('Ctrl Pts',(-43.7913709620947,-59.343799086882,
-39.7092729835095));
#260267=CARTESIAN_POINT('Ctrl Pts',(-43.7314848572577,-59.3185743040837,
-39.6922579595616));
#260268=CARTESIAN_POINT('Ctrl Pts',(-43.7165133310485,-59.3122681083841,
-39.6880042035746));
#260269=CARTESIAN_POINT('Ctrl Pts',(-43.7015908821177,-59.3057655721158,
-39.6837192828541));
#260270=CARTESIAN_POINT('Ctrl Pts',(-43.6867350333519,-59.2990757785203,
-39.6794084779939));
#260271=CARTESIAN_POINT('Ctrl Pts',(-43.671879184586,-59.2923859849247,
-39.6750976731337));
#260272=CARTESIAN_POINT('Ctrl Pts',(-43.657060506721,-59.2854937757857,
-39.6707520471821));
#260273=CARTESIAN_POINT('Ctrl Pts',(-43.6423549194422,-59.2784335932494,
-39.6663936314465));
#260274=CARTESIAN_POINT('Ctrl Pts',(-43.6129437448845,-59.2643132281768,
-39.6576767999753));
#260275=CARTESIAN_POINT('Ctrl Pts',(-43.5840312864905,-59.2495486925951,
-39.6489236815642));
#260276=CARTESIAN_POINT('Ctrl Pts',(-43.5555682511181,-59.2341350312479,
-39.6401231904583));
#260277=CARTESIAN_POINT('Origin',(-44.5079524583207,-57.4754524783487,-52.920575));
#260278=CARTESIAN_POINT('Ctrl Pts',(-44.5079524583208,-55.8067071952963,
-52.4912));
#260279=CARTESIAN_POINT('Ctrl Pts',(-45.4714029967,-55.8067071952963,-52.4328666666667));
#260280=CARTESIAN_POINT('Ctrl Pts',(-45.9531282658897,-56.6410798368225,
-52.3745333333334));
#260281=CARTESIAN_POINT('Ctrl Pts',(-46.4348535350793,-57.4754524783487,
-52.3162000000001));
#260282=CARTESIAN_POINT('Ctrl Pts',(-45.9531282658897,-58.309825119875,
-52.2578666666667));
#260283=CARTESIAN_POINT('Ctrl Pts',(-45.4714029967,-59.1441977614012,-52.1995333333334));
#260284=CARTESIAN_POINT('Ctrl Pts',(-44.5079524583208,-59.1441977614012,
-52.1412));
#260285=CARTESIAN_POINT('Ctrl Pts',(-43.5445019199415,-59.1441977614012,
-52.0828666666667));
#260286=CARTESIAN_POINT('Ctrl Pts',(-43.0627766507519,-58.309825119875,
-52.0245333333333));
#260287=CARTESIAN_POINT('Ctrl Pts',(-42.5810513815623,-57.4754524783487,
-51.9662));
#260288=CARTESIAN_POINT('Ctrl Pts',(-43.0627766507519,-56.6410798368225,
-51.9078666666667));
#260289=CARTESIAN_POINT('Ctrl Pts',(-43.5445019199415,-55.8067071952963,
-51.8495333333334));
#260290=CARTESIAN_POINT('Ctrl Pts',(-44.5079524583208,-55.8067071952963,
-51.7912));
#260291=CARTESIAN_POINT('Ctrl Pts',(-44.5079524583208,-55.8067071952963,
-52.64995));
#260292=CARTESIAN_POINT('Ctrl Pts',(-45.4714029967001,-55.8067071952964,
-52.5916166666668));
#260293=CARTESIAN_POINT('Ctrl Pts',(-45.9531282658897,-56.6410798368225,
-52.5332833333334));
#260294=CARTESIAN_POINT('Ctrl Pts',(-46.4348535350793,-57.4754524783487,
-52.4749500000001));
#260295=CARTESIAN_POINT('Ctrl Pts',(-45.9531282658897,-58.309825119875,
-52.4166166666667));
#260296=CARTESIAN_POINT('Ctrl Pts',(-45.4714029967,-59.1441977614012,-52.3582833333334));
#260297=CARTESIAN_POINT('Ctrl Pts',(-44.5079524583208,-59.1441977614012,
-52.29995));
#260298=CARTESIAN_POINT('Ctrl Pts',(-43.5445019199415,-59.1441977614012,
-52.2416166666667));
#260299=CARTESIAN_POINT('Ctrl Pts',(-43.0627766507519,-58.309825119875,
-52.1832833333333));
#260300=CARTESIAN_POINT('Ctrl Pts',(-42.5810513815623,-57.4754524783487,
-52.12495));
#260301=CARTESIAN_POINT('Ctrl Pts',(-43.0627766507519,-56.6410798368225,
-52.0666166666667));
#260302=CARTESIAN_POINT('Ctrl Pts',(-43.5445019199415,-55.8067071952963,
-52.0082833333333));
#260303=CARTESIAN_POINT('Ctrl Pts',(-44.5079524583208,-55.8067071952963,
-51.94995));
#260304=CARTESIAN_POINT('Ctrl Pts',(-44.5079524583208,-59.5441932447742,
-52.6102625));
#260305=CARTESIAN_POINT('Ctrl Pts',(-43.3135644199415,-59.5441932447742,
-52.5519291666666));
#260306=CARTESIAN_POINT('Ctrl Pts',(-42.7163704007519,-58.5098228615615,
-52.4935958333333));
#260307=CARTESIAN_POINT('Ctrl Pts',(-42.1191763815623,-57.4754524783487,
-52.4352625000001));
#260308=CARTESIAN_POINT('Ctrl Pts',(-42.7163704007519,-56.4410820951361,
-52.3769291666667));
#260309=CARTESIAN_POINT('Ctrl Pts',(-43.3135644199415,-55.4067117119233,
-52.3185958333334));
#260310=CARTESIAN_POINT('Ctrl Pts',(-44.5079524583208,-55.4067117119234,
-52.2602625));
#260311=CARTESIAN_POINT('Ctrl Pts',(-45.7023404967,-55.4067117119233,-52.2019291666667));
#260312=CARTESIAN_POINT('Ctrl Pts',(-46.2995345158897,-56.4410820951361,
-52.1435958333333));
#260313=CARTESIAN_POINT('Ctrl Pts',(-46.8967285350793,-57.4754524783487,
-52.0852625));
#260314=CARTESIAN_POINT('Ctrl Pts',(-46.2995345158897,-58.5098228615615,
-52.0269291666667));
#260315=CARTESIAN_POINT('Ctrl Pts',(-45.7023404967,-59.5441932447742,-51.9685958333333));
#260316=CARTESIAN_POINT('Ctrl Pts',(-44.5079524583208,-59.5441932447742,
-51.9102625));
#260317=CARTESIAN_POINT('Ctrl Pts',(-43.3135644199415,-59.5441932447742,
-51.8519291666667));
#260318=CARTESIAN_POINT('Ctrl Pts',(-42.7163704007519,-58.5098228615615,
-51.7935958333333));
#260319=CARTESIAN_POINT('Ctrl Pts',(-42.1191763815623,-57.4754524783487,
-51.7352625));
#260320=CARTESIAN_POINT('Ctrl Pts',(-42.7163704007519,-56.4410820951361,
-51.6769291666667));
#260321=CARTESIAN_POINT('Ctrl Pts',(-43.3135644199415,-55.4067117119233,
-51.6185958333333));
#260322=CARTESIAN_POINT('Ctrl Pts',(-44.5079524583208,-55.4067117119234,
-51.5602625));
#260323=CARTESIAN_POINT('Ctrl Pts',(-45.7023404967,-55.4067117119233,-51.5019291666666));
#260324=CARTESIAN_POINT('Ctrl Pts',(-46.2995345158897,-56.4410820951361,
-51.4435958333333));
#260325=CARTESIAN_POINT('Ctrl Pts',(-46.8967285350793,-57.4754524783487,
-51.3852625));
#260326=CARTESIAN_POINT('Ctrl Pts',(-46.2995345158897,-58.5098228615615,
-51.3269291666667));
#260327=CARTESIAN_POINT('Ctrl Pts',(-45.7023404967,-59.5441932447742,-51.2685958333333));
#260328=CARTESIAN_POINT('Ctrl Pts',(-44.5079524583208,-59.5441932447742,
-51.2102625));
#260329=CARTESIAN_POINT('Ctrl Pts',(-43.3135644199415,-59.5441932447742,
-51.1519291666666));
#260330=CARTESIAN_POINT('Ctrl Pts',(-42.7163704007519,-58.5098228615615,
-51.0935958333334));
#260331=CARTESIAN_POINT('Ctrl Pts',(-42.1191763815623,-57.4754524783487,
-51.0352625));
#260332=CARTESIAN_POINT('Ctrl Pts',(-42.7163704007519,-56.4410820951361,
-50.9769291666667));
#260333=CARTESIAN_POINT('Ctrl Pts',(-43.3135644199415,-55.4067117119233,
-50.9185958333333));
#260334=CARTESIAN_POINT('Ctrl Pts',(-44.5079524583208,-55.4067117119234,
-50.8602625));
#260335=CARTESIAN_POINT('Ctrl Pts',(-45.7023404967,-55.4067117119233,-50.8019291666667));
#260336=CARTESIAN_POINT('Ctrl Pts',(-46.2995345158897,-56.4410820951361,
-50.7435958333333));
#260337=CARTESIAN_POINT('Ctrl Pts',(-46.8967285350793,-57.4754524783487,
-50.6852625));
#260338=CARTESIAN_POINT('Ctrl Pts',(-46.2995345158897,-58.5098228615615,
-50.6269291666667));
#260339=CARTESIAN_POINT('Ctrl Pts',(-45.7023404967,-59.5441932447742,-50.5685958333333));
#260340=CARTESIAN_POINT('Ctrl Pts',(-44.5079524583208,-59.5441932447742,
-50.5102625));
#260341=CARTESIAN_POINT('Ctrl Pts',(-43.3135644199415,-59.5441932447742,
-50.4519291666667));
#260342=CARTESIAN_POINT('Ctrl Pts',(-42.7163704007519,-58.5098228615615,
-50.3935958333333));
#260343=CARTESIAN_POINT('Ctrl Pts',(-42.1191763815623,-57.4754524783487,
-50.3352625));
#260344=CARTESIAN_POINT('Ctrl Pts',(-42.7163704007519,-56.4410820951361,
-50.2769291666667));
#260345=CARTESIAN_POINT('Ctrl Pts',(-43.3135644199415,-55.4067117119233,
-50.2185958333333));
#260346=CARTESIAN_POINT('Ctrl Pts',(-44.5079524583208,-55.4067117119234,
-50.1602625));
#260347=CARTESIAN_POINT('Ctrl Pts',(-45.7023404967,-55.4067117119233,-50.1019291666667));
#260348=CARTESIAN_POINT('Ctrl Pts',(-46.2995345158897,-56.4410820951361,
-50.0435958333333));
#260349=CARTESIAN_POINT('Ctrl Pts',(-46.8967285350793,-57.4754524783487,
-49.9852625));
#260350=CARTESIAN_POINT('Ctrl Pts',(-46.2995345158897,-58.5098228615615,
-49.9269291666667));
#260351=CARTESIAN_POINT('Ctrl Pts',(-45.7023404967,-59.5441932447742,-49.8685958333333));
#260352=CARTESIAN_POINT('Ctrl Pts',(-44.5079524583208,-59.5441932447742,
-49.8102625));
#260353=CARTESIAN_POINT('Ctrl Pts',(-43.3135644199415,-59.5441932447742,
-49.7519291666667));
#260354=CARTESIAN_POINT('Ctrl Pts',(-42.7163704007519,-58.5098228615615,
-49.6935958333334));
#260355=CARTESIAN_POINT('Ctrl Pts',(-42.1191763815623,-57.4754524783487,
-49.6352625));
#260356=CARTESIAN_POINT('Ctrl Pts',(-42.7163704007519,-56.4410820951361,
-49.5769291666667));
#260357=CARTESIAN_POINT('Ctrl Pts',(-43.3135644199415,-55.4067117119233,
-49.5185958333334));
#260358=CARTESIAN_POINT('Ctrl Pts',(-44.5079524583208,-55.4067117119234,
-49.4602625));
#260359=CARTESIAN_POINT('Ctrl Pts',(-45.7023404967,-55.4067117119233,-49.4019291666667));
#260360=CARTESIAN_POINT('Ctrl Pts',(-46.2995345158897,-56.4410820951361,
-49.3435958333333));
#260361=CARTESIAN_POINT('Ctrl Pts',(-46.8967285350793,-57.4754524783487,
-49.2852625));
#260362=CARTESIAN_POINT('Ctrl Pts',(-46.2995345158897,-58.5098228615615,
-49.2269291666667));
#260363=CARTESIAN_POINT('Ctrl Pts',(-45.7023404967,-59.5441932447742,-49.1685958333334));
#260364=CARTESIAN_POINT('Ctrl Pts',(-44.5079524583208,-59.5441932447742,
-49.1102625));
#260365=CARTESIAN_POINT('Ctrl Pts',(-43.3135644199415,-59.5441932447742,
-49.0519291666667));
#260366=CARTESIAN_POINT('Ctrl Pts',(-42.7163704007519,-58.5098228615615,
-48.9935958333333));
#260367=CARTESIAN_POINT('Ctrl Pts',(-42.1191763815623,-57.4754524783487,
-48.9352625));
#260368=CARTESIAN_POINT('Ctrl Pts',(-42.7163704007519,-56.4410820951361,
-48.8769291666667));
#260369=CARTESIAN_POINT('Ctrl Pts',(-43.3135644199415,-55.4067117119233,
-48.8185958333334));
#260370=CARTESIAN_POINT('Ctrl Pts',(-44.5079524583208,-55.4067117119234,
-48.7602625));
#260371=CARTESIAN_POINT('Ctrl Pts',(-45.7023404967,-55.4067117119233,-48.7019291666667));
#260372=CARTESIAN_POINT('Ctrl Pts',(-46.2995345158897,-56.4410820951361,
-48.6435958333333));
#260373=CARTESIAN_POINT('Ctrl Pts',(-46.8967285350793,-57.4754524783487,
-48.5852625));
#260374=CARTESIAN_POINT('Ctrl Pts',(-46.2995345158897,-58.5098228615615,
-48.5269291666667));
#260375=CARTESIAN_POINT('Ctrl Pts',(-45.7023404967,-59.5441932447742,-48.4685958333333));
#260376=CARTESIAN_POINT('Ctrl Pts',(-44.5079524583208,-59.5441932447742,
-48.4102625));
#260377=CARTESIAN_POINT('Ctrl Pts',(-43.3135644199415,-59.5441932447742,
-48.3519291666667));
#260378=CARTESIAN_POINT('Ctrl Pts',(-42.7163704007519,-58.5098228615615,
-48.2935958333334));
#260379=CARTESIAN_POINT('Ctrl Pts',(-42.1191763815623,-57.4754524783487,
-48.2352625));
#260380=CARTESIAN_POINT('Ctrl Pts',(-42.7163704007519,-56.4410820951361,
-48.1769291666667));
#260381=CARTESIAN_POINT('Ctrl Pts',(-43.3135644199415,-55.4067117119233,
-48.1185958333334));
#260382=CARTESIAN_POINT('Ctrl Pts',(-44.5079524583208,-55.4067117119234,
-48.0602625));
#260383=CARTESIAN_POINT('Ctrl Pts',(-45.7023404967,-55.4067117119233,-48.0019291666667));
#260384=CARTESIAN_POINT('Ctrl Pts',(-46.2995345158897,-56.4410820951361,
-47.9435958333334));
#260385=CARTESIAN_POINT('Ctrl Pts',(-46.8967285350793,-57.4754524783487,
-47.8852625));
#260386=CARTESIAN_POINT('Ctrl Pts',(-46.2995345158897,-58.5098228615615,
-47.8269291666667));
#260387=CARTESIAN_POINT('Ctrl Pts',(-45.7023404967,-59.5441932447742,-47.7685958333333));
#260388=CARTESIAN_POINT('Ctrl Pts',(-44.5079524583208,-59.5441932447742,
-47.7102625));
#260389=CARTESIAN_POINT('Ctrl Pts',(-43.3135644199415,-59.5441932447742,
-47.6519291666667));
#260390=CARTESIAN_POINT('Ctrl Pts',(-42.7163704007519,-58.5098228615615,
-47.5935958333333));
#260391=CARTESIAN_POINT('Ctrl Pts',(-42.1191763815623,-57.4754524783487,
-47.5352625));
#260392=CARTESIAN_POINT('Ctrl Pts',(-42.7163704007519,-56.4410820951361,
-47.4769291666667));
#260393=CARTESIAN_POINT('Ctrl Pts',(-43.3135644199415,-55.4067117119233,
-47.4185958333333));
#260394=CARTESIAN_POINT('Ctrl Pts',(-44.5079524583208,-55.4067117119234,
-47.3602625));
#260395=CARTESIAN_POINT('Ctrl Pts',(-45.7023404967,-55.4067117119233,-47.3019291666666));
#260396=CARTESIAN_POINT('Ctrl Pts',(-46.2995345158897,-56.4410820951361,
-47.2435958333334));
#260397=CARTESIAN_POINT('Ctrl Pts',(-46.8967285350793,-57.4754524783487,
-47.1852625));
#260398=CARTESIAN_POINT('Ctrl Pts',(-46.2995345158897,-58.5098228615615,
-47.1269291666667));
#260399=CARTESIAN_POINT('Ctrl Pts',(-45.7023404967,-59.5441932447742,-47.0685958333333));
#260400=CARTESIAN_POINT('Ctrl Pts',(-44.5079524583208,-59.5441932447742,
-47.0102625));
#260401=CARTESIAN_POINT('Ctrl Pts',(-43.3135644199415,-59.5441932447742,
-46.9519291666667));
#260402=CARTESIAN_POINT('Ctrl Pts',(-42.7163704007519,-58.5098228615615,
-46.8935958333333));
#260403=CARTESIAN_POINT('Ctrl Pts',(-42.1191763815623,-57.4754524783487,
-46.8352625));
#260404=CARTESIAN_POINT('Ctrl Pts',(-42.7163704007519,-56.4410820951361,
-46.7769291666667));
#260405=CARTESIAN_POINT('Ctrl Pts',(-43.3135644199415,-55.4067117119233,
-46.7185958333333));
#260406=CARTESIAN_POINT('Ctrl Pts',(-44.5079524583208,-55.4067117119234,
-46.6602625));
#260407=CARTESIAN_POINT('Ctrl Pts',(-45.7023404967,-55.4067117119233,-46.6019291666667));
#260408=CARTESIAN_POINT('Ctrl Pts',(-46.2995345158897,-56.4410820951361,
-46.5435958333334));
#260409=CARTESIAN_POINT('Ctrl Pts',(-46.8967285350793,-57.4754524783487,
-46.4852625));
#260410=CARTESIAN_POINT('Ctrl Pts',(-46.2995345158897,-58.5098228615615,
-46.4269291666667));
#260411=CARTESIAN_POINT('Ctrl Pts',(-45.7023404967,-59.5441932447742,-46.3685958333333));
#260412=CARTESIAN_POINT('Ctrl Pts',(-44.5079524583208,-59.5441932447742,
-46.3102625));
#260413=CARTESIAN_POINT('Ctrl Pts',(-43.3135644199415,-59.5441932447742,
-46.2519291666667));
#260414=CARTESIAN_POINT('Ctrl Pts',(-42.7163704007519,-58.5098228615615,
-46.1935958333333));
#260415=CARTESIAN_POINT('Ctrl Pts',(-42.1191763815623,-57.4754524783487,
-46.1352625));
#260416=CARTESIAN_POINT('Ctrl Pts',(-42.7163704007519,-56.4410820951361,
-46.0769291666667));
#260417=CARTESIAN_POINT('Ctrl Pts',(-43.3135644199415,-55.4067117119233,
-46.0185958333334));
#260418=CARTESIAN_POINT('Ctrl Pts',(-44.5079524583208,-55.4067117119234,
-45.9602625));
#260419=CARTESIAN_POINT('Ctrl Pts',(-45.7023404967,-55.4067117119233,-45.9019291666667));
#260420=CARTESIAN_POINT('Ctrl Pts',(-46.2995345158897,-56.4410820951361,
-45.8435958333333));
#260421=CARTESIAN_POINT('Ctrl Pts',(-46.8967285350793,-57.4754524783487,
-45.7852625));
#260422=CARTESIAN_POINT('Ctrl Pts',(-46.2995345158897,-58.5098228615615,
-45.7269291666667));
#260423=CARTESIAN_POINT('Ctrl Pts',(-45.7023404967,-59.5441932447742,-45.6685958333334));
#260424=CARTESIAN_POINT('Ctrl Pts',(-44.5079524583208,-59.5441932447742,
-45.6102625));
#260425=CARTESIAN_POINT('Ctrl Pts',(-43.3135644199415,-59.5441932447742,
-45.5519291666667));
#260426=CARTESIAN_POINT('Ctrl Pts',(-42.7163704007519,-58.5098228615615,
-45.4935958333333));
#260427=CARTESIAN_POINT('Ctrl Pts',(-42.1191763815623,-57.4754524783487,
-45.4352625));
#260428=CARTESIAN_POINT('Ctrl Pts',(-42.7163704007519,-56.4410820951361,
-45.3769291666667));
#260429=CARTESIAN_POINT('Ctrl Pts',(-43.3135644199415,-55.4067117119233,
-45.3185958333333));
#260430=CARTESIAN_POINT('Ctrl Pts',(-44.5079524583208,-55.4067117119234,
-45.2602625));
#260431=CARTESIAN_POINT('Ctrl Pts',(-45.7023404967,-55.4067117119233,-45.2019291666667));
#260432=CARTESIAN_POINT('Ctrl Pts',(-46.2995345158897,-56.4410820951361,
-45.1435958333334));
#260433=CARTESIAN_POINT('Ctrl Pts',(-46.8967285350793,-57.4754524783487,
-45.0852625));
#260434=CARTESIAN_POINT('Ctrl Pts',(-46.2995345158897,-58.5098228615615,
-45.0269291666667));
#260435=CARTESIAN_POINT('Ctrl Pts',(-45.7023404967,-59.5441932447742,-44.9685958333334));
#260436=CARTESIAN_POINT('Ctrl Pts',(-44.5079524583208,-59.5441932447742,
-44.9102625));
#260437=CARTESIAN_POINT('Ctrl Pts',(-43.3135644199415,-59.5441932447742,
-44.8519291666667));
#260438=CARTESIAN_POINT('Ctrl Pts',(-42.7163704007519,-58.5098228615615,
-44.7935958333333));
#260439=CARTESIAN_POINT('Ctrl Pts',(-42.1191763815623,-57.4754524783487,
-44.7352625));
#260440=CARTESIAN_POINT('Ctrl Pts',(-42.7163704007519,-56.4410820951361,
-44.6769291666667));
#260441=CARTESIAN_POINT('Ctrl Pts',(-43.3135644199415,-55.4067117119233,
-44.6185958333334));
#260442=CARTESIAN_POINT('Ctrl Pts',(-44.5079524583208,-55.4067117119234,
-44.5602625));
#260443=CARTESIAN_POINT('Ctrl Pts',(-45.7023404967,-55.4067117119233,-44.5019291666667));
#260444=CARTESIAN_POINT('Ctrl Pts',(-46.2995345158897,-56.4410820951361,
-44.4435958333333));
#260445=CARTESIAN_POINT('Ctrl Pts',(-46.8967285350793,-57.4754524783487,
-44.3852625));
#260446=CARTESIAN_POINT('Ctrl Pts',(-46.2995345158897,-58.5098228615615,
-44.3269291666667));
#260447=CARTESIAN_POINT('Ctrl Pts',(-45.7023404967,-59.5441932447742,-44.2685958333334));
#260448=CARTESIAN_POINT('Ctrl Pts',(-44.5079524583208,-59.5441932447742,
-44.2102625));
#260449=CARTESIAN_POINT('Ctrl Pts',(-43.3135644199415,-59.5441932447742,
-44.1519291666667));
#260450=CARTESIAN_POINT('Ctrl Pts',(-42.7163704007519,-58.5098228615615,
-44.0935958333334));
#260451=CARTESIAN_POINT('Ctrl Pts',(-42.1191763815623,-57.4754524783487,
-44.0352625));
#260452=CARTESIAN_POINT('Ctrl Pts',(-42.7163704007519,-56.4410820951361,
-43.9769291666667));
#260453=CARTESIAN_POINT('Ctrl Pts',(-43.3135644199415,-55.4067117119233,
-43.9185958333334));
#260454=CARTESIAN_POINT('Ctrl Pts',(-44.5079524583208,-55.4067117119234,
-43.8602625));
#260455=CARTESIAN_POINT('Ctrl Pts',(-45.7023404967,-55.4067117119233,-43.8019291666667));
#260456=CARTESIAN_POINT('Ctrl Pts',(-46.2995345158897,-56.4410820951361,
-43.7435958333334));
#260457=CARTESIAN_POINT('Ctrl Pts',(-46.8967285350793,-57.4754524783487,
-43.6852625));
#260458=CARTESIAN_POINT('Ctrl Pts',(-46.2995345158897,-58.5098228615615,
-43.6269291666667));
#260459=CARTESIAN_POINT('Ctrl Pts',(-45.7023404967,-59.5441932447742,-43.5685958333334));
#260460=CARTESIAN_POINT('Ctrl Pts',(-44.5079524583208,-59.5441932447742,
-43.5102625));
#260461=CARTESIAN_POINT('Ctrl Pts',(-43.3135644199415,-59.5441932447742,
-43.4519291666667));
#260462=CARTESIAN_POINT('Ctrl Pts',(-42.7163704007519,-58.5098228615615,
-43.3935958333334));
#260463=CARTESIAN_POINT('Ctrl Pts',(-42.1191763815623,-57.4754524783487,
-43.3352625));
#260464=CARTESIAN_POINT('Ctrl Pts',(-42.7163704007519,-56.4410820951361,
-43.2769291666667));
#260465=CARTESIAN_POINT('Ctrl Pts',(-43.3135644199415,-55.4067117119233,
-43.2185958333334));
#260466=CARTESIAN_POINT('Ctrl Pts',(-44.5079524583208,-55.4067117119234,
-43.1602625));
#260467=CARTESIAN_POINT('Ctrl Pts',(-45.7023404967,-55.4067117119233,-43.1019291666667));
#260468=CARTESIAN_POINT('Ctrl Pts',(-46.2995345158897,-56.4410820951361,
-43.0435958333334));
#260469=CARTESIAN_POINT('Ctrl Pts',(-46.8967285350793,-57.4754524783487,
-42.9852625));
#260470=CARTESIAN_POINT('Ctrl Pts',(-46.2995345158897,-58.5098228615615,
-42.9269291666667));
#260471=CARTESIAN_POINT('Ctrl Pts',(-45.7023404967,-59.5441932447742,-42.8685958333333));
#260472=CARTESIAN_POINT('Ctrl Pts',(-44.5079524583208,-59.5441932447742,
-42.8102625));
#260473=CARTESIAN_POINT('Ctrl Pts',(-43.3135644199415,-59.5441932447742,
-42.7519291666667));
#260474=CARTESIAN_POINT('Ctrl Pts',(-42.7163704007519,-58.5098228615615,
-42.6935958333333));
#260475=CARTESIAN_POINT('Ctrl Pts',(-42.1191763815623,-57.4754524783487,
-42.6352625));
#260476=CARTESIAN_POINT('Ctrl Pts',(-42.7163704007519,-56.4410820951361,
-42.5769291666667));
#260477=CARTESIAN_POINT('Ctrl Pts',(-43.3135644199415,-55.4067117119233,
-42.5185958333333));
#260478=CARTESIAN_POINT('Ctrl Pts',(-44.5079524583208,-55.4067117119234,
-42.4602625));
#260479=CARTESIAN_POINT('Ctrl Pts',(-45.7023404967,-55.4067117119233,-42.4019291666666));
#260480=CARTESIAN_POINT('Ctrl Pts',(-46.2995345158897,-56.4410820951361,
-42.3435958333334));
#260481=CARTESIAN_POINT('Ctrl Pts',(-46.8967285350793,-57.4754524783487,
-42.2852625));
#260482=CARTESIAN_POINT('Ctrl Pts',(-46.2995345158897,-58.5098228615615,
-42.2269291666667));
#260483=CARTESIAN_POINT('Ctrl Pts',(-45.7023404967,-59.5441932447742,-42.1685958333333));
#260484=CARTESIAN_POINT('Ctrl Pts',(-44.5079524583208,-59.5441932447742,
-42.1102625));
#260485=CARTESIAN_POINT('Ctrl Pts',(-43.3135644199415,-59.5441932447742,
-42.0519291666667));
#260486=CARTESIAN_POINT('Ctrl Pts',(-42.7163704007519,-58.5098228615615,
-41.9935958333334));
#260487=CARTESIAN_POINT('Ctrl Pts',(-42.1191763815623,-57.4754524783487,
-41.9352625));
#260488=CARTESIAN_POINT('Ctrl Pts',(-42.7163704007519,-56.4410820951361,
-41.8769291666667));
#260489=CARTESIAN_POINT('Ctrl Pts',(-43.3135644199415,-55.4067117119233,
-41.8185958333333));
#260490=CARTESIAN_POINT('Ctrl Pts',(-44.5079524583208,-55.4067117119234,
-41.7602625));
#260491=CARTESIAN_POINT('Ctrl Pts',(-45.7023404967,-55.4067117119233,-41.7019291666667));
#260492=CARTESIAN_POINT('Ctrl Pts',(-46.2995345158897,-56.4410820951361,
-41.6435958333334));
#260493=CARTESIAN_POINT('Ctrl Pts',(-46.8967285350793,-57.4754524783487,
-41.5852625));
#260494=CARTESIAN_POINT('Ctrl Pts',(-46.2995345158897,-58.5098228615615,
-41.5269291666667));
#260495=CARTESIAN_POINT('Ctrl Pts',(-45.7023404967,-59.5441932447742,-41.4685958333333));
#260496=CARTESIAN_POINT('Ctrl Pts',(-44.5079524583208,-59.5441932447742,
-41.4102625));
#260497=CARTESIAN_POINT('Ctrl Pts',(-43.3135644199415,-59.5441932447742,
-41.3519291666666));
#260498=CARTESIAN_POINT('Ctrl Pts',(-42.7163704007519,-58.5098228615615,
-41.2935958333334));
#260499=CARTESIAN_POINT('Ctrl Pts',(-42.1191763815623,-57.4754524783487,
-41.2352625));
#260500=CARTESIAN_POINT('Ctrl Pts',(-42.7163704007519,-56.4410820951361,
-41.1769291666667));
#260501=CARTESIAN_POINT('Ctrl Pts',(-43.3135644199415,-55.4067117119233,
-41.1185958333333));
#260502=CARTESIAN_POINT('Ctrl Pts',(-44.5079524583208,-55.4067117119234,
-41.0602625));
#260503=CARTESIAN_POINT('Ctrl Pts',(-45.7023404967,-55.4067117119233,-41.0019291666666));
#260504=CARTESIAN_POINT('Ctrl Pts',(-46.2995345158897,-56.4410820951361,
-40.9435958333334));
#260505=CARTESIAN_POINT('Ctrl Pts',(-46.8967285350793,-57.4754524783487,
-40.8852625));
#260506=CARTESIAN_POINT('Ctrl Pts',(-46.2995345158897,-58.5098228615615,
-40.8269291666667));
#260507=CARTESIAN_POINT('Ctrl Pts',(-45.7023404967,-59.5441932447742,-40.7685958333333));
#260508=CARTESIAN_POINT('Ctrl Pts',(-44.5079524583208,-59.5441932447742,
-40.7102625));
#260509=CARTESIAN_POINT('Ctrl Pts',(-43.3135644199415,-59.5441932447742,
-40.6519291666667));
#260510=CARTESIAN_POINT('Ctrl Pts',(-42.7163704007519,-58.5098228615615,
-40.5935958333334));
#260511=CARTESIAN_POINT('Ctrl Pts',(-42.1191763815623,-57.4754524783487,
-40.5352625));
#260512=CARTESIAN_POINT('Ctrl Pts',(-42.7163704007519,-56.4410820951361,
-40.4769291666667));
#260513=CARTESIAN_POINT('Ctrl Pts',(-43.3135644199415,-55.4067117119233,
-40.4185958333333));
#260514=CARTESIAN_POINT('Ctrl Pts',(-44.5079524583208,-55.4067117119234,
-40.3602625));
#260515=CARTESIAN_POINT('Ctrl Pts',(-45.7023404967,-55.4067117119233,-40.3019291666667));
#260516=CARTESIAN_POINT('Ctrl Pts',(-46.2995345158897,-56.4410820951361,
-40.2435958333334));
#260517=CARTESIAN_POINT('Ctrl Pts',(-46.8967285350793,-57.4754524783487,
-40.1852625));
#260518=CARTESIAN_POINT('Ctrl Pts',(-46.2995345158897,-58.5098228615615,
-40.1269291666666));
#260519=CARTESIAN_POINT('Ctrl Pts',(-45.7023404967,-59.5441932447742,-40.0685958333333));
#260520=CARTESIAN_POINT('Ctrl Pts',(-44.5079524583208,-59.5441932447742,
-40.0102625));
#260521=CARTESIAN_POINT('Ctrl Pts',(-43.3135644199415,-59.5441932447742,
-39.9519291666667));
#260522=CARTESIAN_POINT('Ctrl Pts',(-42.7163704007519,-58.5098228615615,
-39.8935958333334));
#260523=CARTESIAN_POINT('Ctrl Pts',(-42.1191763815623,-57.4754524783487,
-39.8352625));
#260524=CARTESIAN_POINT('Ctrl Pts',(-42.7163704007519,-56.4410820951361,
-39.7769291666667));
#260525=CARTESIAN_POINT('Ctrl Pts',(-43.3135644199415,-55.4067117119233,
-39.7185958333334));
#260526=CARTESIAN_POINT('Ctrl Pts',(-44.5079524583208,-55.4067117119234,
-39.6602625));
#260527=CARTESIAN_POINT('Ctrl Pts',(-45.7023404967,-55.4067117119233,-39.6019291666667));
#260528=CARTESIAN_POINT('Ctrl Pts',(-46.2995345158897,-56.4410820951361,
-39.5435958333333));
#260529=CARTESIAN_POINT('Ctrl Pts',(-46.8967285350793,-57.4754524783487,
-39.4852625));
#260530=CARTESIAN_POINT('Ctrl Pts',(-46.2995345158897,-58.5098228615615,
-39.4269291666667));
#260531=CARTESIAN_POINT('Ctrl Pts',(-45.7023404967,-59.5441932447742,-39.3685958333334));
#260532=CARTESIAN_POINT('Ctrl Pts',(-44.5079524583208,-59.5441932447742,
-39.3102625));
#260533=CARTESIAN_POINT('Ctrl Pts',(-43.3135644199415,-59.5441932447742,
-39.2519291666667));
#260534=CARTESIAN_POINT('Ctrl Pts',(-42.7163704007519,-58.5098228615615,
-39.1935958333334));
#260535=CARTESIAN_POINT('Ctrl Pts',(-42.1191763815623,-57.4754524783487,
-39.1352625));
#260536=CARTESIAN_POINT('Ctrl Pts',(-42.7163704007519,-56.4410820951361,
-39.0769291666667));
#260537=CARTESIAN_POINT('Ctrl Pts',(-43.3135644199415,-55.4067117119233,
-39.0185958333334));
#260538=CARTESIAN_POINT('Ctrl Pts',(-44.5079524583208,-55.4067117119234,
-38.9602625));
#260539=CARTESIAN_POINT('Ctrl Pts',(-45.7023404967,-55.4067117119233,-38.9019291666667));
#260540=CARTESIAN_POINT('Ctrl Pts',(-46.2995345158897,-56.4410820951361,
-38.8435958333333));
#260541=CARTESIAN_POINT('Ctrl Pts',(-46.8967285350793,-57.4754524783487,
-38.7852625));
#260542=CARTESIAN_POINT('Ctrl Pts',(-46.2995345158897,-58.5098228615615,
-38.7269291666667));
#260543=CARTESIAN_POINT('Ctrl Pts',(-45.7023404967,-59.5441932447742,-38.6685958333334));
#260544=CARTESIAN_POINT('Ctrl Pts',(-44.5079524583208,-59.5441932447742,
-38.6102625));
#260545=CARTESIAN_POINT('Ctrl Pts',(-43.3135644199415,-59.5441932447742,
-38.5519291666667));
#260546=CARTESIAN_POINT('Ctrl Pts',(-42.7163704007519,-58.5098228615615,
-38.4935958333334));
#260547=CARTESIAN_POINT('Ctrl Pts',(-42.1191763815623,-57.4754524783487,
-38.4352625));
#260548=CARTESIAN_POINT('Ctrl Pts',(-42.7163704007519,-56.4410820951361,
-38.3769291666667));
#260549=CARTESIAN_POINT('Ctrl Pts',(-43.3135644199415,-55.4067117119233,
-38.3185958333333));
#260550=CARTESIAN_POINT('Ctrl Pts',(-44.5079524583208,-55.4067117119234,
-38.2602625));
#260551=CARTESIAN_POINT('Ctrl Pts',(-45.7023404967,-55.4067117119233,-38.2019291666667));
#260552=CARTESIAN_POINT('Ctrl Pts',(-46.2995345158897,-56.4410820951361,
-38.1435958333334));
#260553=CARTESIAN_POINT('Ctrl Pts',(-46.8967285350793,-57.4754524783487,
-38.0852625));
#260554=CARTESIAN_POINT('Ctrl Pts',(-46.2995345158897,-58.5098228615615,
-38.0269291666667));
#260555=CARTESIAN_POINT('Ctrl Pts',(-45.7023404967,-59.5441932447742,-37.9685958333333));
#260556=CARTESIAN_POINT('Ctrl Pts',(-44.5079524583208,-59.5441932447742,
-37.9102625));
#260557=CARTESIAN_POINT('Ctrl Pts',(-43.3135644199415,-59.5441932447742,
-37.8519291666667));
#260558=CARTESIAN_POINT('Ctrl Pts',(-42.7163704007519,-58.5098228615615,
-37.7935958333334));
#260559=CARTESIAN_POINT('Ctrl Pts',(-42.1191763815623,-57.4754524783487,
-37.7352625));
#260560=CARTESIAN_POINT('Ctrl Pts',(-42.7163704007519,-56.4410820951361,
-37.6769291666667));
#260561=CARTESIAN_POINT('Ctrl Pts',(-43.3135644199415,-55.4067117119233,
-37.6185958333333));
#260562=CARTESIAN_POINT('Ctrl Pts',(-44.5079524583208,-55.4067117119234,
-37.5602625));
#260563=CARTESIAN_POINT('Ctrl Pts',(-45.7023404967,-55.4067117119233,-37.5019291666667));
#260564=CARTESIAN_POINT('Ctrl Pts',(-46.2995345158897,-56.4410820951361,
-37.4435958333333));
#260565=CARTESIAN_POINT('Ctrl Pts',(-46.8967285350793,-57.4754524783487,
-37.3852625));
#260566=CARTESIAN_POINT('Ctrl Pts',(-46.2995345158897,-58.5098228615615,
-37.3269291666667));
#260567=CARTESIAN_POINT('Ctrl Pts',(-45.7023404967,-59.5441932447742,-37.2685958333333));
#260568=CARTESIAN_POINT('Ctrl Pts',(-44.5079524583208,-59.5441932447742,
-37.2102625));
#260569=CARTESIAN_POINT('Ctrl Pts',(-43.3135644199415,-59.5441932447742,
-37.1519291666667));
#260570=CARTESIAN_POINT('Ctrl Pts',(-42.7163704007519,-58.5098228615615,
-37.0935958333333));
#260571=CARTESIAN_POINT('Ctrl Pts',(-42.1191763815623,-57.4754524783487,
-37.0352625));
#260572=CARTESIAN_POINT('Ctrl Pts',(-42.7163704007519,-56.4410820951361,
-36.9769291666667));
#260573=CARTESIAN_POINT('Ctrl Pts',(-43.3135644199415,-55.4067117119233,
-36.9185958333333));
#260574=CARTESIAN_POINT('Ctrl Pts',(-44.5079524583208,-55.4067117119234,
-36.8602625));
#260575=CARTESIAN_POINT('Ctrl Pts',(-45.7023404967,-55.4067117119233,-36.8019291666666));
#260576=CARTESIAN_POINT('Ctrl Pts',(-46.2995345158897,-56.4410820951361,
-36.7435958333334));
#260577=CARTESIAN_POINT('Ctrl Pts',(-46.8967285350793,-57.4754524783487,
-36.6852625));
#260578=CARTESIAN_POINT('Ctrl Pts',(-46.2995345158897,-58.5098228615615,
-36.6269291666667));
#260579=CARTESIAN_POINT('Ctrl Pts',(-46.222006582932,-58.64410518045,-36.6193563132714));
#260580=CARTESIAN_POINT('Ctrl Pts',(-46.1253278975281,-58.7653303978899,
-36.611216324118));
#260581=CARTESIAN_POINT('Ctrl Pts',(-44.5079524583208,-59.1441977614012,
-52.8412));
#260582=CARTESIAN_POINT('Ctrl Pts',(-43.5445019199415,-59.1441977614012,
-52.7828666666667));
#260583=CARTESIAN_POINT('Ctrl Pts',(-43.0627766507519,-58.309825119875,
-52.7245333333334));
#260584=CARTESIAN_POINT('Ctrl Pts',(-42.5810513815623,-57.4754524783487,
-52.6662));
#260585=CARTESIAN_POINT('Ctrl Pts',(-43.0627766507519,-56.6410798368225,
-52.6078666666667));
#260586=CARTESIAN_POINT('Ctrl Pts',(-43.5445019199415,-55.8067071952963,
-52.5495333333333));
#260587=CARTESIAN_POINT('Ctrl Pts',(-44.5079524583208,-55.8067071952963,
-52.4912));
#260588=CARTESIAN_POINT('Ctrl Pts',(-45.4714029967,-55.8067071952963,-52.4328666666667));
#260589=CARTESIAN_POINT('Ctrl Pts',(-45.9531282658897,-56.6410798368225,
-52.3745333333334));
#260590=CARTESIAN_POINT('Ctrl Pts',(-46.4348535350793,-57.4754524783487,
-52.3162000000001));
#260591=CARTESIAN_POINT('Ctrl Pts',(-45.9531282658897,-58.309825119875,
-52.2578666666667));
#260592=CARTESIAN_POINT('Ctrl Pts',(-45.4714029967,-59.1441977614012,-52.1995333333334));
#260593=CARTESIAN_POINT('Ctrl Pts',(-44.5079524583208,-59.1441977614012,
-52.1412));
#260594=CARTESIAN_POINT('Ctrl Pts',(-43.5445019199415,-59.1441977614012,
-52.0828666666667));
#260595=CARTESIAN_POINT('Ctrl Pts',(-43.0627766507519,-58.309825119875,
-52.0245333333333));
#260596=CARTESIAN_POINT('Ctrl Pts',(-42.5810513815623,-57.4754524783487,
-51.9662));
#260597=CARTESIAN_POINT('Ctrl Pts',(-43.0627766507519,-56.6410798368225,
-51.9078666666667));
#260598=CARTESIAN_POINT('Ctrl Pts',(-43.5445019199415,-55.8067071952963,
-51.8495333333334));
#260599=CARTESIAN_POINT('Ctrl Pts',(-44.5079524583208,-55.8067071952963,
-51.7912));
#260600=CARTESIAN_POINT('Ctrl Pts',(-45.4714029967,-55.8067071952963,-51.7328666666667));
#260601=CARTESIAN_POINT('Ctrl Pts',(-45.9531282658897,-56.6410798368225,
-51.6745333333334));
#260602=CARTESIAN_POINT('Ctrl Pts',(-46.4348535350793,-57.4754524783487,
-51.6162));
#260603=CARTESIAN_POINT('Ctrl Pts',(-45.9531282658897,-58.309825119875,
-51.5578666666667));
#260604=CARTESIAN_POINT('Ctrl Pts',(-45.4714029967,-59.1441977614012,-51.4995333333334));
#260605=CARTESIAN_POINT('Ctrl Pts',(-44.5079524583208,-59.1441977614012,
-51.4412));
#260606=CARTESIAN_POINT('Ctrl Pts',(-43.5445019199415,-59.1441977614012,
-51.3828666666667));
#260607=CARTESIAN_POINT('Ctrl Pts',(-43.0627766507519,-58.309825119875,
-51.3245333333334));
#260608=CARTESIAN_POINT('Ctrl Pts',(-42.5810513815623,-57.4754524783487,
-51.2662));
#260609=CARTESIAN_POINT('Ctrl Pts',(-43.0627766507519,-56.6410798368225,
-51.2078666666667));
#260610=CARTESIAN_POINT('Ctrl Pts',(-43.5445019199415,-55.8067071952963,
-51.1495333333334));
#260611=CARTESIAN_POINT('Ctrl Pts',(-44.5079524583208,-55.8067071952963,
-51.0912));
#260612=CARTESIAN_POINT('Ctrl Pts',(-45.4714029967,-55.8067071952963,-51.0328666666667));
#260613=CARTESIAN_POINT('Ctrl Pts',(-45.9531282658897,-56.6410798368225,
-50.9745333333333));
#260614=CARTESIAN_POINT('Ctrl Pts',(-46.4348535350793,-57.4754524783487,
-50.9162));
#260615=CARTESIAN_POINT('Ctrl Pts',(-45.9531282658897,-58.309825119875,
-50.8578666666667));
#260616=CARTESIAN_POINT('Ctrl Pts',(-45.4714029967,-59.1441977614012,-50.7995333333334));
#260617=CARTESIAN_POINT('Ctrl Pts',(-44.5079524583208,-59.1441977614012,
-50.7412));
#260618=CARTESIAN_POINT('Ctrl Pts',(-43.5445019199415,-59.1441977614012,
-50.6828666666667));
#260619=CARTESIAN_POINT('Ctrl Pts',(-43.0627766507519,-58.309825119875,
-50.6245333333333));
#260620=CARTESIAN_POINT('Ctrl Pts',(-42.5810513815623,-57.4754524783487,
-50.5662));
#260621=CARTESIAN_POINT('Ctrl Pts',(-43.0627766507519,-56.6410798368225,
-50.5078666666667));
#260622=CARTESIAN_POINT('Ctrl Pts',(-43.5445019199415,-55.8067071952963,
-50.4495333333333));
#260623=CARTESIAN_POINT('Ctrl Pts',(-44.5079524583208,-55.8067071952963,
-50.3912));
#260624=CARTESIAN_POINT('Ctrl Pts',(-45.4714029967,-55.8067071952963,-50.3328666666667));
#260625=CARTESIAN_POINT('Ctrl Pts',(-45.9531282658897,-56.6410798368225,
-50.2745333333334));
#260626=CARTESIAN_POINT('Ctrl Pts',(-46.4348535350793,-57.4754524783487,
-50.2162));
#260627=CARTESIAN_POINT('Ctrl Pts',(-45.9531282658897,-58.309825119875,
-50.1578666666667));
#260628=CARTESIAN_POINT('Ctrl Pts',(-45.4714029967,-59.1441977614012,-50.0995333333333));
#260629=CARTESIAN_POINT('Ctrl Pts',(-44.5079524583208,-59.1441977614012,
-50.0412));
#260630=CARTESIAN_POINT('Ctrl Pts',(-43.5445019199415,-59.1441977614012,
-49.9828666666667));
#260631=CARTESIAN_POINT('Ctrl Pts',(-43.0627766507519,-58.309825119875,
-49.9245333333334));
#260632=CARTESIAN_POINT('Ctrl Pts',(-42.5810513815623,-57.4754524783487,
-49.8662));
#260633=CARTESIAN_POINT('Ctrl Pts',(-43.0627766507519,-56.6410798368225,
-49.8078666666667));
#260634=CARTESIAN_POINT('Ctrl Pts',(-43.5445019199415,-55.8067071952963,
-49.7495333333333));
#260635=CARTESIAN_POINT('Ctrl Pts',(-44.5079524583208,-55.8067071952963,
-49.6912));
#260636=CARTESIAN_POINT('Ctrl Pts',(-45.4714029967,-55.8067071952963,-49.6328666666667));
#260637=CARTESIAN_POINT('Ctrl Pts',(-45.9531282658897,-56.6410798368225,
-49.5745333333334));
#260638=CARTESIAN_POINT('Ctrl Pts',(-46.4348535350793,-57.4754524783487,
-49.5162));
#260639=CARTESIAN_POINT('Ctrl Pts',(-45.9531282658897,-58.309825119875,
-49.4578666666667));
#260640=CARTESIAN_POINT('Ctrl Pts',(-45.4714029967,-59.1441977614012,-49.3995333333333));
#260641=CARTESIAN_POINT('Ctrl Pts',(-44.5079524583208,-59.1441977614012,
-49.3412));
#260642=CARTESIAN_POINT('Ctrl Pts',(-43.5445019199415,-59.1441977614012,
-49.2828666666666));
#260643=CARTESIAN_POINT('Ctrl Pts',(-43.0627766507519,-58.309825119875,
-49.2245333333334));
#260644=CARTESIAN_POINT('Ctrl Pts',(-42.5810513815623,-57.4754524783487,
-49.1662));
#260645=CARTESIAN_POINT('Ctrl Pts',(-43.0627766507519,-56.6410798368225,
-49.1078666666667));
#260646=CARTESIAN_POINT('Ctrl Pts',(-43.5445019199415,-55.8067071952963,
-49.0495333333334));
#260647=CARTESIAN_POINT('Ctrl Pts',(-44.5079524583208,-55.8067071952963,
-48.9912));
#260648=CARTESIAN_POINT('Ctrl Pts',(-45.4714029967,-55.8067071952963,-48.9328666666667));
#260649=CARTESIAN_POINT('Ctrl Pts',(-45.9531282658897,-56.6410798368225,
-48.8745333333334));
#260650=CARTESIAN_POINT('Ctrl Pts',(-46.4348535350793,-57.4754524783487,
-48.8162));
#260651=CARTESIAN_POINT('Ctrl Pts',(-45.9531282658897,-58.309825119875,
-48.7578666666667));
#260652=CARTESIAN_POINT('Ctrl Pts',(-45.4714029967,-59.1441977614012,-48.6995333333334));
#260653=CARTESIAN_POINT('Ctrl Pts',(-44.5079524583208,-59.1441977614012,
-48.6412));
#260654=CARTESIAN_POINT('Ctrl Pts',(-43.5445019199415,-59.1441977614012,
-48.5828666666667));
#260655=CARTESIAN_POINT('Ctrl Pts',(-43.0627766507519,-58.309825119875,
-48.5245333333334));
#260656=CARTESIAN_POINT('Ctrl Pts',(-42.5810513815623,-57.4754524783487,
-48.4662));
#260657=CARTESIAN_POINT('Ctrl Pts',(-43.0627766507519,-56.6410798368225,
-48.4078666666667));
#260658=CARTESIAN_POINT('Ctrl Pts',(-43.5445019199415,-55.8067071952963,
-48.3495333333333));
#260659=CARTESIAN_POINT('Ctrl Pts',(-44.5079524583208,-55.8067071952963,
-48.2912));
#260660=CARTESIAN_POINT('Ctrl Pts',(-45.4714029967,-55.8067071952963,-48.2328666666667));
#260661=CARTESIAN_POINT('Ctrl Pts',(-45.9531282658897,-56.6410798368225,
-48.1745333333334));
#260662=CARTESIAN_POINT('Ctrl Pts',(-46.4348535350793,-57.4754524783487,
-48.1162));
#260663=CARTESIAN_POINT('Ctrl Pts',(-45.9531282658897,-58.309825119875,
-48.0578666666667));
#260664=CARTESIAN_POINT('Ctrl Pts',(-45.4714029967,-59.1441977614012,-47.9995333333334));
#260665=CARTESIAN_POINT('Ctrl Pts',(-44.5079524583208,-59.1441977614012,
-47.9412));
#260666=CARTESIAN_POINT('Ctrl Pts',(-43.5445019199415,-59.1441977614012,
-47.8828666666667));
#260667=CARTESIAN_POINT('Ctrl Pts',(-43.0627766507519,-58.309825119875,
-47.8245333333333));
#260668=CARTESIAN_POINT('Ctrl Pts',(-42.5810513815623,-57.4754524783487,
-47.7662));
#260669=CARTESIAN_POINT('Ctrl Pts',(-43.0627766507519,-56.6410798368225,
-47.7078666666667));
#260670=CARTESIAN_POINT('Ctrl Pts',(-43.5445019199415,-55.8067071952963,
-47.6495333333334));
#260671=CARTESIAN_POINT('Ctrl Pts',(-44.5079524583208,-55.8067071952963,
-47.5912));
#260672=CARTESIAN_POINT('Ctrl Pts',(-45.4714029967,-55.8067071952963,-47.5328666666667));
#260673=CARTESIAN_POINT('Ctrl Pts',(-45.9531282658897,-56.6410798368225,
-47.4745333333334));
#260674=CARTESIAN_POINT('Ctrl Pts',(-46.4348535350793,-57.4754524783487,
-47.4162));
#260675=CARTESIAN_POINT('Ctrl Pts',(-45.9531282658897,-58.309825119875,
-47.3578666666667));
#260676=CARTESIAN_POINT('Ctrl Pts',(-45.4714029967,-59.1441977614012,-47.2995333333334));
#260677=CARTESIAN_POINT('Ctrl Pts',(-44.5079524583208,-59.1441977614012,
-47.2412));
#260678=CARTESIAN_POINT('Ctrl Pts',(-43.5445019199415,-59.1441977614012,
-47.1828666666667));
#260679=CARTESIAN_POINT('Ctrl Pts',(-43.0627766507519,-58.309825119875,
-47.1245333333333));
#260680=CARTESIAN_POINT('Ctrl Pts',(-42.5810513815623,-57.4754524783487,
-47.0662));
#260681=CARTESIAN_POINT('Ctrl Pts',(-43.0627766507519,-56.6410798368225,
-47.0078666666667));
#260682=CARTESIAN_POINT('Ctrl Pts',(-43.5445019199415,-55.8067071952963,
-46.9495333333334));
#260683=CARTESIAN_POINT('Ctrl Pts',(-44.5079524583208,-55.8067071952963,
-46.8912));
#260684=CARTESIAN_POINT('Ctrl Pts',(-45.4714029967,-55.8067071952963,-46.8328666666667));
#260685=CARTESIAN_POINT('Ctrl Pts',(-45.9531282658897,-56.6410798368225,
-46.7745333333334));
#260686=CARTESIAN_POINT('Ctrl Pts',(-46.4348535350793,-57.4754524783487,
-46.7162));
#260687=CARTESIAN_POINT('Ctrl Pts',(-45.9531282658897,-58.309825119875,
-46.6578666666667));
#260688=CARTESIAN_POINT('Ctrl Pts',(-45.4714029967,-59.1441977614012,-46.5995333333334));
#260689=CARTESIAN_POINT('Ctrl Pts',(-44.5079524583208,-59.1441977614012,
-46.5412));
#260690=CARTESIAN_POINT('Ctrl Pts',(-43.5445019199415,-59.1441977614012,
-46.4828666666667));
#260691=CARTESIAN_POINT('Ctrl Pts',(-43.0627766507519,-58.309825119875,
-46.4245333333334));
#260692=CARTESIAN_POINT('Ctrl Pts',(-42.5810513815623,-57.4754524783487,
-46.3662));
#260693=CARTESIAN_POINT('Ctrl Pts',(-43.0627766507519,-56.6410798368225,
-46.3078666666667));
#260694=CARTESIAN_POINT('Ctrl Pts',(-43.5445019199415,-55.8067071952963,
-46.2495333333334));
#260695=CARTESIAN_POINT('Ctrl Pts',(-44.5079524583208,-55.8067071952963,
-46.1912));
#260696=CARTESIAN_POINT('Ctrl Pts',(-45.4714029967,-55.8067071952963,-46.1328666666667));
#260697=CARTESIAN_POINT('Ctrl Pts',(-45.9531282658897,-56.6410798368225,
-46.0745333333334));
#260698=CARTESIAN_POINT('Ctrl Pts',(-46.4348535350793,-57.4754524783487,
-46.0162));
#260699=CARTESIAN_POINT('Ctrl Pts',(-45.9531282658897,-58.309825119875,
-45.9578666666667));
#260700=CARTESIAN_POINT('Ctrl Pts',(-45.4714029967,-59.1441977614012,-45.8995333333333));
#260701=CARTESIAN_POINT('Ctrl Pts',(-44.5079524583208,-59.1441977614012,
-45.8412));
#260702=CARTESIAN_POINT('Ctrl Pts',(-43.5445019199415,-59.1441977614012,
-45.7828666666667));
#260703=CARTESIAN_POINT('Ctrl Pts',(-43.0627766507519,-58.309825119875,
-45.7245333333333));
#260704=CARTESIAN_POINT('Ctrl Pts',(-42.5810513815623,-57.4754524783487,
-45.6662));
#260705=CARTESIAN_POINT('Ctrl Pts',(-43.0627766507519,-56.6410798368225,
-45.6078666666667));
#260706=CARTESIAN_POINT('Ctrl Pts',(-43.5445019199415,-55.8067071952963,
-45.5495333333333));
#260707=CARTESIAN_POINT('Ctrl Pts',(-44.5079524583208,-55.8067071952963,
-45.4912));
#260708=CARTESIAN_POINT('Ctrl Pts',(-45.4714029967,-55.8067071952963,-45.4328666666666));
#260709=CARTESIAN_POINT('Ctrl Pts',(-45.9531282658897,-56.6410798368225,
-45.3745333333334));
#260710=CARTESIAN_POINT('Ctrl Pts',(-46.4348535350793,-57.4754524783487,
-45.3162));
#260711=CARTESIAN_POINT('Ctrl Pts',(-45.9531282658897,-58.309825119875,
-45.2578666666667));
#260712=CARTESIAN_POINT('Ctrl Pts',(-45.4714029967,-59.1441977614012,-45.1995333333333));
#260713=CARTESIAN_POINT('Ctrl Pts',(-44.5079524583208,-59.1441977614012,
-45.1412));
#260714=CARTESIAN_POINT('Ctrl Pts',(-43.5445019199415,-59.1441977614012,
-45.0828666666667));
#260715=CARTESIAN_POINT('Ctrl Pts',(-43.0627766507519,-58.309825119875,
-45.0245333333334));
#260716=CARTESIAN_POINT('Ctrl Pts',(-42.5810513815623,-57.4754524783487,
-44.9662));
#260717=CARTESIAN_POINT('Ctrl Pts',(-43.0627766507519,-56.6410798368225,
-44.9078666666667));
#260718=CARTESIAN_POINT('Ctrl Pts',(-43.5445019199415,-55.8067071952963,
-44.8495333333333));
#260719=CARTESIAN_POINT('Ctrl Pts',(-44.5079524583208,-55.8067071952963,
-44.7912));
#260720=CARTESIAN_POINT('Ctrl Pts',(-45.4714029967,-55.8067071952963,-44.7328666666667));
#260721=CARTESIAN_POINT('Ctrl Pts',(-45.9531282658897,-56.6410798368225,
-44.6745333333334));
#260722=CARTESIAN_POINT('Ctrl Pts',(-46.4348535350793,-57.4754524783487,
-44.6162));
#260723=CARTESIAN_POINT('Ctrl Pts',(-45.9531282658897,-58.309825119875,
-44.5578666666667));
#260724=CARTESIAN_POINT('Ctrl Pts',(-45.4714029967,-59.1441977614012,-44.4995333333333));
#260725=CARTESIAN_POINT('Ctrl Pts',(-44.5079524583208,-59.1441977614012,
-44.4412));
#260726=CARTESIAN_POINT('Ctrl Pts',(-43.5445019199415,-59.1441977614012,
-44.3828666666667));
#260727=CARTESIAN_POINT('Ctrl Pts',(-43.0627766507519,-58.309825119875,
-44.3245333333334));
#260728=CARTESIAN_POINT('Ctrl Pts',(-42.5810513815623,-57.4754524783487,
-44.2662));
#260729=CARTESIAN_POINT('Ctrl Pts',(-43.0627766507519,-56.6410798368225,
-44.2078666666667));
#260730=CARTESIAN_POINT('Ctrl Pts',(-43.5445019199415,-55.8067071952963,
-44.1495333333334));
#260731=CARTESIAN_POINT('Ctrl Pts',(-44.5079524583208,-55.8067071952963,
-44.0912));
#260732=CARTESIAN_POINT('Ctrl Pts',(-45.4714029967,-55.8067071952963,-44.0328666666667));
#260733=CARTESIAN_POINT('Ctrl Pts',(-45.9531282658897,-56.6410798368225,
-43.9745333333333));
#260734=CARTESIAN_POINT('Ctrl Pts',(-46.4348535350793,-57.4754524783487,
-43.9162));
#260735=CARTESIAN_POINT('Ctrl Pts',(-45.9531282658897,-58.309825119875,
-43.8578666666667));
#260736=CARTESIAN_POINT('Ctrl Pts',(-45.4714029967,-59.1441977614012,-43.7995333333334));
#260737=CARTESIAN_POINT('Ctrl Pts',(-44.5079524583208,-59.1441977614012,
-43.7412));
#260738=CARTESIAN_POINT('Ctrl Pts',(-43.5445019199415,-59.1441977614012,
-43.6828666666667));
#260739=CARTESIAN_POINT('Ctrl Pts',(-43.0627766507519,-58.309825119875,
-43.6245333333333));
#260740=CARTESIAN_POINT('Ctrl Pts',(-42.5810513815623,-57.4754524783487,
-43.5662));
#260741=CARTESIAN_POINT('Ctrl Pts',(-43.0627766507519,-56.6410798368225,
-43.5078666666667));
#260742=CARTESIAN_POINT('Ctrl Pts',(-43.5445019199415,-55.8067071952963,
-43.4495333333334));
#260743=CARTESIAN_POINT('Ctrl Pts',(-44.5079524583208,-55.8067071952963,
-43.3912));
#260744=CARTESIAN_POINT('Ctrl Pts',(-45.4714029967,-55.8067071952963,-43.3328666666667));
#260745=CARTESIAN_POINT('Ctrl Pts',(-45.9531282658897,-56.6410798368225,
-43.2745333333334));
#260746=CARTESIAN_POINT('Ctrl Pts',(-46.4348535350793,-57.4754524783487,
-43.2162));
#260747=CARTESIAN_POINT('Ctrl Pts',(-45.9531282658897,-58.309825119875,
-43.1578666666667));
#260748=CARTESIAN_POINT('Ctrl Pts',(-45.4714029967,-59.1441977614012,-43.0995333333334));
#260749=CARTESIAN_POINT('Ctrl Pts',(-44.5079524583208,-59.1441977614012,
-43.0412));
#260750=CARTESIAN_POINT('Ctrl Pts',(-43.5445019199415,-59.1441977614012,
-42.9828666666667));
#260751=CARTESIAN_POINT('Ctrl Pts',(-43.0627766507519,-58.309825119875,
-42.9245333333334));
#260752=CARTESIAN_POINT('Ctrl Pts',(-42.5810513815623,-57.4754524783487,
-42.8662));
#260753=CARTESIAN_POINT('Ctrl Pts',(-43.0627766507519,-56.6410798368225,
-42.8078666666667));
#260754=CARTESIAN_POINT('Ctrl Pts',(-43.5445019199415,-55.8067071952963,
-42.7495333333334));
#260755=CARTESIAN_POINT('Ctrl Pts',(-44.5079524583208,-55.8067071952963,
-42.6912));
#260756=CARTESIAN_POINT('Ctrl Pts',(-45.4714029967,-55.8067071952963,-42.6328666666667));
#260757=CARTESIAN_POINT('Ctrl Pts',(-45.9531282658897,-56.6410798368225,
-42.5745333333333));
#260758=CARTESIAN_POINT('Ctrl Pts',(-46.4348535350793,-57.4754524783487,
-42.5162));
#260759=CARTESIAN_POINT('Ctrl Pts',(-45.9531282658897,-58.309825119875,
-42.4578666666667));
#260760=CARTESIAN_POINT('Ctrl Pts',(-45.4714029967,-59.1441977614012,-42.3995333333334));
#260761=CARTESIAN_POINT('Ctrl Pts',(-44.5079524583208,-59.1441977614012,
-42.3412));
#260762=CARTESIAN_POINT('Ctrl Pts',(-43.5445019199415,-59.1441977614012,
-42.2828666666667));
#260763=CARTESIAN_POINT('Ctrl Pts',(-43.0627766507519,-58.309825119875,
-42.2245333333333));
#260764=CARTESIAN_POINT('Ctrl Pts',(-42.5810513815623,-57.4754524783487,
-42.1662));
#260765=CARTESIAN_POINT('Ctrl Pts',(-43.0627766507519,-56.6410798368225,
-42.1078666666667));
#260766=CARTESIAN_POINT('Ctrl Pts',(-43.5445019199415,-55.8067071952963,
-42.0495333333334));
#260767=CARTESIAN_POINT('Ctrl Pts',(-44.5079524583208,-55.8067071952963,
-41.9912));
#260768=CARTESIAN_POINT('Ctrl Pts',(-45.4714029967,-55.8067071952963,-41.9328666666667));
#260769=CARTESIAN_POINT('Ctrl Pts',(-45.9531282658897,-56.6410798368225,
-41.8745333333334));
#260770=CARTESIAN_POINT('Ctrl Pts',(-46.4348535350793,-57.4754524783487,
-41.8162));
#260771=CARTESIAN_POINT('Ctrl Pts',(-45.9531282658897,-58.309825119875,
-41.7578666666667));
#260772=CARTESIAN_POINT('Ctrl Pts',(-45.4714029967,-59.1441977614012,-41.6995333333334));
#260773=CARTESIAN_POINT('Ctrl Pts',(-44.5079524583208,-59.1441977614012,
-41.6412));
#260774=CARTESIAN_POINT('Ctrl Pts',(-43.5445019199415,-59.1441977614012,
-41.5828666666667));
#260775=CARTESIAN_POINT('Ctrl Pts',(-43.0627766507519,-58.309825119875,
-41.5245333333334));
#260776=CARTESIAN_POINT('Ctrl Pts',(-42.5810513815623,-57.4754524783487,
-41.4662));
#260777=CARTESIAN_POINT('Ctrl Pts',(-43.0627766507519,-56.6410798368225,
-41.4078666666667));
#260778=CARTESIAN_POINT('Ctrl Pts',(-43.5445019199415,-55.8067071952963,
-41.3495333333333));
#260779=CARTESIAN_POINT('Ctrl Pts',(-44.5079524583208,-55.8067071952963,
-41.2912));
#260780=CARTESIAN_POINT('Ctrl Pts',(-45.4714029967,-55.8067071952963,-41.2328666666667));
#260781=CARTESIAN_POINT('Ctrl Pts',(-45.9531282658897,-56.6410798368225,
-41.1745333333334));
#260782=CARTESIAN_POINT('Ctrl Pts',(-46.4348535350793,-57.4754524783487,
-41.1162));
#260783=CARTESIAN_POINT('Ctrl Pts',(-45.9531282658897,-58.309825119875,
-41.0578666666667));
#260784=CARTESIAN_POINT('Ctrl Pts',(-45.4714029967,-59.1441977614012,-40.9995333333333));
#260785=CARTESIAN_POINT('Ctrl Pts',(-44.5079524583208,-59.1441977614012,
-40.9412));
#260786=CARTESIAN_POINT('Ctrl Pts',(-43.5445019199415,-59.1441977614012,
-40.8828666666667));
#260787=CARTESIAN_POINT('Ctrl Pts',(-43.0627766507519,-58.309825119875,
-40.8245333333333));
#260788=CARTESIAN_POINT('Ctrl Pts',(-42.5810513815623,-57.4754524783487,
-40.7662));
#260789=CARTESIAN_POINT('Ctrl Pts',(-43.0627766507519,-56.6410798368225,
-40.7078666666667));
#260790=CARTESIAN_POINT('Ctrl Pts',(-43.5445019199415,-55.8067071952963,
-40.6495333333334));
#260791=CARTESIAN_POINT('Ctrl Pts',(-44.5079524583208,-55.8067071952963,
-40.5912));
#260792=CARTESIAN_POINT('Ctrl Pts',(-45.4714029967,-55.8067071952963,-40.5328666666667));
#260793=CARTESIAN_POINT('Ctrl Pts',(-45.9531282658897,-56.6410798368225,
-40.4745333333334));
#260794=CARTESIAN_POINT('Ctrl Pts',(-46.4348535350793,-57.4754524783487,
-40.4162));
#260795=CARTESIAN_POINT('Ctrl Pts',(-45.9531282658897,-58.309825119875,
-40.3578666666667));
#260796=CARTESIAN_POINT('Ctrl Pts',(-45.4714029967,-59.1441977614012,-40.2995333333333));
#260797=CARTESIAN_POINT('Ctrl Pts',(-44.5079524583208,-59.1441977614012,
-40.2412));
#260798=CARTESIAN_POINT('Ctrl Pts',(-43.5445019199415,-59.1441977614012,
-40.1828666666667));
#260799=CARTESIAN_POINT('Ctrl Pts',(-43.0627766507519,-58.309825119875,
-40.1245333333334));
#260800=CARTESIAN_POINT('Ctrl Pts',(-42.5810513815623,-57.4754524783487,
-40.0662));
#260801=CARTESIAN_POINT('Ctrl Pts',(-43.0627766507519,-56.6410798368225,
-40.0078666666667));
#260802=CARTESIAN_POINT('Ctrl Pts',(-43.5445019199415,-55.8067071952963,
-39.9495333333333));
#260803=CARTESIAN_POINT('Ctrl Pts',(-44.5079524583208,-55.8067071952963,
-39.8912));
#260804=CARTESIAN_POINT('Ctrl Pts',(-45.4714029967,-55.8067071952963,-39.8328666666666));
#260805=CARTESIAN_POINT('Ctrl Pts',(-45.9531282658897,-56.6410798368225,
-39.7745333333334));
#260806=CARTESIAN_POINT('Ctrl Pts',(-46.4348535350793,-57.4754524783487,
-39.7162));
#260807=CARTESIAN_POINT('Ctrl Pts',(-45.9531282658897,-58.309825119875,
-39.6578666666667));
#260808=CARTESIAN_POINT('Ctrl Pts',(-45.4714029967,-59.1441977614012,-39.5995333333333));
#260809=CARTESIAN_POINT('Ctrl Pts',(-44.5079524583208,-59.1441977614012,
-39.5412));
#260810=CARTESIAN_POINT('Ctrl Pts',(-43.5445019199415,-59.1441977614012,
-39.4828666666666));
#260811=CARTESIAN_POINT('Ctrl Pts',(-43.0627766507519,-58.309825119875,
-39.4245333333334));
#260812=CARTESIAN_POINT('Ctrl Pts',(-42.5810513815623,-57.4754524783487,
-39.3662));
#260813=CARTESIAN_POINT('Ctrl Pts',(-43.0627766507519,-56.6410798368225,
-39.3078666666667));
#260814=CARTESIAN_POINT('Ctrl Pts',(-43.5445019199415,-55.8067071952963,
-39.2495333333333));
#260815=CARTESIAN_POINT('Ctrl Pts',(-44.5079524583208,-55.8067071952963,
-39.1912));
#260816=CARTESIAN_POINT('Ctrl Pts',(-45.4714029967,-55.8067071952963,-39.1328666666667));
#260817=CARTESIAN_POINT('Ctrl Pts',(-45.9531282658897,-56.6410798368225,
-39.0745333333333));
#260818=CARTESIAN_POINT('Ctrl Pts',(-46.4348535350793,-57.4754524783487,
-39.0162));
#260819=CARTESIAN_POINT('Ctrl Pts',(-45.9531282658897,-58.309825119875,
-38.9578666666667));
#260820=CARTESIAN_POINT('Ctrl Pts',(-45.4714029967,-59.1441977614012,-38.8995333333334));
#260821=CARTESIAN_POINT('Ctrl Pts',(-44.5079524583208,-59.1441977614012,
-38.8412));
#260822=CARTESIAN_POINT('Ctrl Pts',(-43.5445019199415,-59.1441977614012,
-38.7828666666667));
#260823=CARTESIAN_POINT('Ctrl Pts',(-43.0627766507519,-58.309825119875,
-38.7245333333334));
#260824=CARTESIAN_POINT('Ctrl Pts',(-42.5810513815623,-57.4754524783487,
-38.6662));
#260825=CARTESIAN_POINT('Ctrl Pts',(-43.0627766507519,-56.6410798368225,
-38.6078666666667));
#260826=CARTESIAN_POINT('Ctrl Pts',(-43.5445019199415,-55.8067071952963,
-38.5495333333334));
#260827=CARTESIAN_POINT('Ctrl Pts',(-44.5079524583208,-55.8067071952963,
-38.4912));
#260828=CARTESIAN_POINT('Ctrl Pts',(-45.4714029967,-55.8067071952963,-38.4328666666667));
#260829=CARTESIAN_POINT('Ctrl Pts',(-45.9531282658897,-56.6410798368225,
-38.3745333333333));
#260830=CARTESIAN_POINT('Ctrl Pts',(-46.4348535350793,-57.4754524783487,
-38.3162));
#260831=CARTESIAN_POINT('Ctrl Pts',(-45.9531282658897,-58.309825119875,
-38.2578666666667));
#260832=CARTESIAN_POINT('Ctrl Pts',(-45.4714029967,-59.1441977614012,-38.1995333333333));
#260833=CARTESIAN_POINT('Ctrl Pts',(-44.5079524583208,-59.1441977614012,
-38.1412));
#260834=CARTESIAN_POINT('Ctrl Pts',(-43.5445019199415,-59.1441977614012,
-38.0828666666667));
#260835=CARTESIAN_POINT('Ctrl Pts',(-43.0627766507519,-58.309825119875,
-38.0245333333334));
#260836=CARTESIAN_POINT('Ctrl Pts',(-42.5810513815623,-57.4754524783487,
-37.9662));
#260837=CARTESIAN_POINT('Ctrl Pts',(-43.0627766507519,-56.6410798368225,
-37.9078666666667));
#260838=CARTESIAN_POINT('Ctrl Pts',(-43.5445019199415,-55.8067071952963,
-37.8495333333334));
#260839=CARTESIAN_POINT('Ctrl Pts',(-44.5079524583208,-55.8067071952963,
-37.7912));
#260840=CARTESIAN_POINT('Ctrl Pts',(-45.4714029967,-55.8067071952963,-37.7328666666667));
#260841=CARTESIAN_POINT('Ctrl Pts',(-45.9531282658897,-56.6410798368225,
-37.6745333333334));
#260842=CARTESIAN_POINT('Ctrl Pts',(-46.4348535350793,-57.4754524783487,
-37.6162));
#260843=CARTESIAN_POINT('Ctrl Pts',(-45.9531282658897,-58.309825119875,
-37.5578666666667));
#260844=CARTESIAN_POINT('Ctrl Pts',(-45.4714029967,-59.1441977614012,-37.4995333333334));
#260845=CARTESIAN_POINT('Ctrl Pts',(-44.5079524583208,-59.1441977614012,
-37.4412));
#260846=CARTESIAN_POINT('Ctrl Pts',(-43.5445019199415,-59.1441977614012,
-37.3828666666667));
#260847=CARTESIAN_POINT('Ctrl Pts',(-43.0627766507519,-58.309825119875,
-37.3245333333333));
#260848=CARTESIAN_POINT('Ctrl Pts',(-42.5810513815623,-57.4754524783487,
-37.2662));
#260849=CARTESIAN_POINT('Ctrl Pts',(-43.0627766507519,-56.6410798368225,
-37.2078666666667));
#260850=CARTESIAN_POINT('Ctrl Pts',(-43.5445019199415,-55.8067071952963,
-37.1495333333334));
#260851=CARTESIAN_POINT('Ctrl Pts',(-44.5079524583208,-55.8067071952963,
-37.0912));
#260852=CARTESIAN_POINT('Ctrl Pts',(-45.4714029967,-55.8067071952963,-37.0328666666667));
#260853=CARTESIAN_POINT('Ctrl Pts',(-45.9531282658897,-56.6410798368225,
-36.9745333333333));
#260854=CARTESIAN_POINT('Ctrl Pts',(-46.4348535350793,-57.4754524783487,
-36.9162));
#260855=CARTESIAN_POINT('Ctrl Pts',(-45.9531282658897,-58.309825119875,
-36.8578666666667));
#260856=CARTESIAN_POINT('Ctrl Pts',(-45.8905905257689,-58.4181436631548,
-36.8502938132714));
#260857=CARTESIAN_POINT('Ctrl Pts',(-45.8126048724392,-58.5159297236766,
-36.8421538241181));
#260858=CARTESIAN_POINT('Ctrl Pts',(-42.5996267014623,-58.0740282996226,
-39.2098668919623));
#260859=CARTESIAN_POINT('Ctrl Pts',(-42.5725778614496,-57.8429829953309,
-39.2221682992926));
#260860=CARTESIAN_POINT('Ctrl Pts',(-42.5746974198402,-57.610126621336,
-39.227083277036));
#260861=CARTESIAN_POINT('Ctrl Pts',(-42.6405003904691,-57.1745640350164,
-39.2256289192332));
#260862=CARTESIAN_POINT('Ctrl Pts',(-42.6977550170523,-56.9733387116817,
-39.2204303507015));
#260863=CARTESIAN_POINT('Ctrl Pts',(-42.8283324794819,-56.6773258608037,
-39.2079085695582));
#260864=CARTESIAN_POINT('Ctrl Pts',(-42.8824025719944,-56.5767100388546,
-39.2029307320589));
#260865=CARTESIAN_POINT('Ctrl Pts',(-42.9551055667509,-56.4626324221248,
-39.1954338390341));
#260866=CARTESIAN_POINT('Ctrl Pts',(-42.9664620034791,-56.4453286852025,
-39.1942364504284));
#260867=CARTESIAN_POINT('Ctrl Pts',(-42.9795523961031,-56.4259574076604,
-39.1928277088137));
#260868=CARTESIAN_POINT('Ctrl Pts',(-42.9809760143693,-56.4238580974341,
-39.192674110711));
#260869=CARTESIAN_POINT('Ctrl Pts',(-42.9838312438709,-56.419662423705,
-39.1923652757117));
#260870=CARTESIAN_POINT('Ctrl Pts',(-42.9852628470618,-56.4175660843538,
-39.1922100390342));
#260871=CARTESIAN_POINT('Ctrl Pts',(-43.0379271161551,-56.3407179277042,
-39.1864853162508));
#260872=CARTESIAN_POINT('Ctrl Pts',(-43.093260109904,-56.269324547675,-39.1800000400795));
#260873=CARTESIAN_POINT('Ctrl Pts',(-43.2395455298464,-56.1018453733189,
-39.1619525260045));
#260874=CARTESIAN_POINT('Ctrl Pts',(-43.334446313922,-56.0103462780516,
-39.1495099323279));
#260875=CARTESIAN_POINT('Ctrl Pts',(-43.6658508016362,-55.7405007337001,
-39.103943047775));
#260876=CARTESIAN_POINT('Ctrl Pts',(-43.9263559243168,-55.5998720026574,
-39.0651121378969));
#260877=CARTESIAN_POINT('Ctrl Pts',(-44.2150213622831,-55.5011028009662,
-39.0177579842635));
#260878=CARTESIAN_POINT('Ctrl Pts',(-44.225814020228,-55.4974873478956,
-39.0159815752866));
#260879=CARTESIAN_POINT('Ctrl Pts',(-44.236624711623,-55.4939424893001,
-39.0141961864886));
#260880=CARTESIAN_POINT('Ctrl Pts',(-44.5079524583208,-59.5441932447742,
-52.6102625));
#260881=CARTESIAN_POINT('Ctrl Pts',(-43.3135644199415,-59.5441932447742,
-52.5519291666666));
#260882=CARTESIAN_POINT('Ctrl Pts',(-42.7163704007519,-58.5098228615615,
-52.4935958333333));
#260883=CARTESIAN_POINT('Ctrl Pts',(-42.1191763815623,-57.4754524783487,
-52.4352625000001));
#260884=CARTESIAN_POINT('Ctrl Pts',(-42.7163704007519,-56.4410820951361,
-52.3769291666667));
#260885=CARTESIAN_POINT('Ctrl Pts',(-43.3135644199415,-55.4067117119233,
-52.3185958333334));
#260886=CARTESIAN_POINT('Ctrl Pts',(-44.5079524583208,-55.4067117119234,
-52.2602625));
#260887=CARTESIAN_POINT('Ctrl Pts',(-45.7023404967,-55.4067117119233,-52.2019291666667));
#260888=CARTESIAN_POINT('Ctrl Pts',(-46.2995345158897,-56.4410820951361,
-52.1435958333333));
#260889=CARTESIAN_POINT('Ctrl Pts',(-46.8967285350793,-57.4754524783487,
-52.0852625));
#260890=CARTESIAN_POINT('Ctrl Pts',(-46.2995345158897,-58.5098228615615,
-52.0269291666667));
#260891=CARTESIAN_POINT('Ctrl Pts',(-45.7023404967,-59.5441932447742,-51.9685958333333));
#260892=CARTESIAN_POINT('Ctrl Pts',(-44.5079524583208,-59.5441932447742,
-51.9102625));
#260893=CARTESIAN_POINT('Ctrl Pts',(-43.3135644199415,-59.5441932447742,
-51.8519291666667));
#260894=CARTESIAN_POINT('Ctrl Pts',(-42.7163704007519,-58.5098228615615,
-51.7935958333333));
#260895=CARTESIAN_POINT('Ctrl Pts',(-42.1191763815623,-57.4754524783487,
-51.7352625));
#260896=CARTESIAN_POINT('Ctrl Pts',(-42.7163704007519,-56.4410820951361,
-51.6769291666667));
#260897=CARTESIAN_POINT('Ctrl Pts',(-43.3135644199415,-55.4067117119233,
-51.6185958333333));
#260898=CARTESIAN_POINT('Ctrl Pts',(-44.5079524583208,-55.4067117119234,
-51.5602625));
#260899=CARTESIAN_POINT('Ctrl Pts',(-45.7023404967,-55.4067117119233,-51.5019291666666));
#260900=CARTESIAN_POINT('Ctrl Pts',(-46.2995345158897,-56.4410820951361,
-51.4435958333333));
#260901=CARTESIAN_POINT('Ctrl Pts',(-46.8967285350793,-57.4754524783487,
-51.3852625));
#260902=CARTESIAN_POINT('Ctrl Pts',(-46.2995345158897,-58.5098228615615,
-51.3269291666667));
#260903=CARTESIAN_POINT('Ctrl Pts',(-45.7023404967,-59.5441932447742,-51.2685958333333));
#260904=CARTESIAN_POINT('Ctrl Pts',(-44.5079524583208,-59.5441932447742,
-51.2102625));
#260905=CARTESIAN_POINT('Ctrl Pts',(-43.3135644199415,-59.5441932447742,
-51.1519291666666));
#260906=CARTESIAN_POINT('Ctrl Pts',(-42.7163704007519,-58.5098228615615,
-51.0935958333334));
#260907=CARTESIAN_POINT('Ctrl Pts',(-42.1191763815623,-57.4754524783487,
-51.0352625));
#260908=CARTESIAN_POINT('Ctrl Pts',(-42.7163704007519,-56.4410820951361,
-50.9769291666667));
#260909=CARTESIAN_POINT('Ctrl Pts',(-43.3135644199415,-55.4067117119233,
-50.9185958333333));
#260910=CARTESIAN_POINT('Ctrl Pts',(-44.5079524583208,-55.4067117119234,
-50.8602625));
#260911=CARTESIAN_POINT('Ctrl Pts',(-45.7023404967,-55.4067117119233,-50.8019291666667));
#260912=CARTESIAN_POINT('Ctrl Pts',(-46.2995345158897,-56.4410820951361,
-50.7435958333333));
#260913=CARTESIAN_POINT('Ctrl Pts',(-46.8967285350793,-57.4754524783487,
-50.6852625));
#260914=CARTESIAN_POINT('Ctrl Pts',(-46.2995345158897,-58.5098228615615,
-50.6269291666667));
#260915=CARTESIAN_POINT('Ctrl Pts',(-45.7023404967,-59.5441932447742,-50.5685958333333));
#260916=CARTESIAN_POINT('Ctrl Pts',(-44.5079524583208,-59.5441932447742,
-50.5102625));
#260917=CARTESIAN_POINT('Ctrl Pts',(-43.3135644199415,-59.5441932447742,
-50.4519291666667));
#260918=CARTESIAN_POINT('Ctrl Pts',(-42.7163704007519,-58.5098228615615,
-50.3935958333333));
#260919=CARTESIAN_POINT('Ctrl Pts',(-42.1191763815623,-57.4754524783487,
-50.3352625));
#260920=CARTESIAN_POINT('Ctrl Pts',(-42.7163704007519,-56.4410820951361,
-50.2769291666667));
#260921=CARTESIAN_POINT('Ctrl Pts',(-43.3135644199415,-55.4067117119233,
-50.2185958333333));
#260922=CARTESIAN_POINT('Ctrl Pts',(-44.5079524583208,-55.4067117119234,
-50.1602625));
#260923=CARTESIAN_POINT('Ctrl Pts',(-45.7023404967,-55.4067117119233,-50.1019291666667));
#260924=CARTESIAN_POINT('Ctrl Pts',(-46.2995345158897,-56.4410820951361,
-50.0435958333333));
#260925=CARTESIAN_POINT('Ctrl Pts',(-46.8967285350793,-57.4754524783487,
-49.9852625));
#260926=CARTESIAN_POINT('Ctrl Pts',(-46.2995345158897,-58.5098228615615,
-49.9269291666667));
#260927=CARTESIAN_POINT('Ctrl Pts',(-45.7023404967,-59.5441932447742,-49.8685958333333));
#260928=CARTESIAN_POINT('Ctrl Pts',(-44.5079524583208,-59.5441932447742,
-49.8102625));
#260929=CARTESIAN_POINT('Ctrl Pts',(-43.3135644199415,-59.5441932447742,
-49.7519291666667));
#260930=CARTESIAN_POINT('Ctrl Pts',(-42.7163704007519,-58.5098228615615,
-49.6935958333334));
#260931=CARTESIAN_POINT('Ctrl Pts',(-42.1191763815623,-57.4754524783487,
-49.6352625));
#260932=CARTESIAN_POINT('Ctrl Pts',(-42.7163704007519,-56.4410820951361,
-49.5769291666667));
#260933=CARTESIAN_POINT('Ctrl Pts',(-43.3135644199415,-55.4067117119233,
-49.5185958333334));
#260934=CARTESIAN_POINT('Ctrl Pts',(-44.5079524583208,-55.4067117119234,
-49.4602625));
#260935=CARTESIAN_POINT('Ctrl Pts',(-45.7023404967,-55.4067117119233,-49.4019291666667));
#260936=CARTESIAN_POINT('Ctrl Pts',(-46.2995345158897,-56.4410820951361,
-49.3435958333333));
#260937=CARTESIAN_POINT('Ctrl Pts',(-46.8967285350793,-57.4754524783487,
-49.2852625));
#260938=CARTESIAN_POINT('Ctrl Pts',(-46.2995345158897,-58.5098228615615,
-49.2269291666667));
#260939=CARTESIAN_POINT('Ctrl Pts',(-45.7023404967,-59.5441932447742,-49.1685958333334));
#260940=CARTESIAN_POINT('Ctrl Pts',(-44.5079524583208,-59.5441932447742,
-49.1102625));
#260941=CARTESIAN_POINT('Ctrl Pts',(-43.3135644199415,-59.5441932447742,
-49.0519291666667));
#260942=CARTESIAN_POINT('Ctrl Pts',(-42.7163704007519,-58.5098228615615,
-48.9935958333333));
#260943=CARTESIAN_POINT('Ctrl Pts',(-42.1191763815623,-57.4754524783487,
-48.9352625));
#260944=CARTESIAN_POINT('Ctrl Pts',(-42.7163704007519,-56.4410820951361,
-48.8769291666667));
#260945=CARTESIAN_POINT('Ctrl Pts',(-43.3135644199415,-55.4067117119233,
-48.8185958333334));
#260946=CARTESIAN_POINT('Ctrl Pts',(-44.5079524583208,-55.4067117119234,
-48.7602625));
#260947=CARTESIAN_POINT('Ctrl Pts',(-45.7023404967,-55.4067117119233,-48.7019291666667));
#260948=CARTESIAN_POINT('Ctrl Pts',(-46.2995345158897,-56.4410820951361,
-48.6435958333333));
#260949=CARTESIAN_POINT('Ctrl Pts',(-46.8967285350793,-57.4754524783487,
-48.5852625));
#260950=CARTESIAN_POINT('Ctrl Pts',(-46.2995345158897,-58.5098228615615,
-48.5269291666667));
#260951=CARTESIAN_POINT('Ctrl Pts',(-45.7023404967,-59.5441932447742,-48.4685958333333));
#260952=CARTESIAN_POINT('Ctrl Pts',(-44.5079524583208,-59.5441932447742,
-48.4102625));
#260953=CARTESIAN_POINT('Ctrl Pts',(-43.3135644199415,-59.5441932447742,
-48.3519291666667));
#260954=CARTESIAN_POINT('Ctrl Pts',(-42.7163704007519,-58.5098228615615,
-48.2935958333334));
#260955=CARTESIAN_POINT('Ctrl Pts',(-42.1191763815623,-57.4754524783487,
-48.2352625));
#260956=CARTESIAN_POINT('Ctrl Pts',(-42.7163704007519,-56.4410820951361,
-48.1769291666667));
#260957=CARTESIAN_POINT('Ctrl Pts',(-43.3135644199415,-55.4067117119233,
-48.1185958333334));
#260958=CARTESIAN_POINT('Ctrl Pts',(-44.5079524583208,-55.4067117119234,
-48.0602625));
#260959=CARTESIAN_POINT('Ctrl Pts',(-45.7023404967,-55.4067117119233,-48.0019291666667));
#260960=CARTESIAN_POINT('Ctrl Pts',(-46.2995345158897,-56.4410820951361,
-47.9435958333334));
#260961=CARTESIAN_POINT('Ctrl Pts',(-46.8967285350793,-57.4754524783487,
-47.8852625));
#260962=CARTESIAN_POINT('Ctrl Pts',(-46.2995345158897,-58.5098228615615,
-47.8269291666667));
#260963=CARTESIAN_POINT('Ctrl Pts',(-45.7023404967,-59.5441932447742,-47.7685958333333));
#260964=CARTESIAN_POINT('Ctrl Pts',(-44.5079524583208,-59.5441932447742,
-47.7102625));
#260965=CARTESIAN_POINT('Ctrl Pts',(-43.3135644199415,-59.5441932447742,
-47.6519291666667));
#260966=CARTESIAN_POINT('Ctrl Pts',(-42.7163704007519,-58.5098228615615,
-47.5935958333333));
#260967=CARTESIAN_POINT('Ctrl Pts',(-42.1191763815623,-57.4754524783487,
-47.5352625));
#260968=CARTESIAN_POINT('Ctrl Pts',(-42.7163704007519,-56.4410820951361,
-47.4769291666667));
#260969=CARTESIAN_POINT('Ctrl Pts',(-43.3135644199415,-55.4067117119233,
-47.4185958333333));
#260970=CARTESIAN_POINT('Ctrl Pts',(-44.5079524583208,-55.4067117119234,
-47.3602625));
#260971=CARTESIAN_POINT('Ctrl Pts',(-45.7023404967,-55.4067117119233,-47.3019291666666));
#260972=CARTESIAN_POINT('Ctrl Pts',(-46.2995345158897,-56.4410820951361,
-47.2435958333334));
#260973=CARTESIAN_POINT('Ctrl Pts',(-46.8967285350793,-57.4754524783487,
-47.1852625));
#260974=CARTESIAN_POINT('Ctrl Pts',(-46.2995345158897,-58.5098228615615,
-47.1269291666667));
#260975=CARTESIAN_POINT('Ctrl Pts',(-45.7023404967,-59.5441932447742,-47.0685958333333));
#260976=CARTESIAN_POINT('Ctrl Pts',(-44.5079524583208,-59.5441932447742,
-47.0102625));
#260977=CARTESIAN_POINT('Ctrl Pts',(-43.3135644199415,-59.5441932447742,
-46.9519291666667));
#260978=CARTESIAN_POINT('Ctrl Pts',(-42.7163704007519,-58.5098228615615,
-46.8935958333333));
#260979=CARTESIAN_POINT('Ctrl Pts',(-42.1191763815623,-57.4754524783487,
-46.8352625));
#260980=CARTESIAN_POINT('Ctrl Pts',(-42.7163704007519,-56.4410820951361,
-46.7769291666667));
#260981=CARTESIAN_POINT('Ctrl Pts',(-43.3135644199415,-55.4067117119233,
-46.7185958333333));
#260982=CARTESIAN_POINT('Ctrl Pts',(-44.5079524583208,-55.4067117119234,
-46.6602625));
#260983=CARTESIAN_POINT('Ctrl Pts',(-45.7023404967,-55.4067117119233,-46.6019291666667));
#260984=CARTESIAN_POINT('Ctrl Pts',(-46.2995345158897,-56.4410820951361,
-46.5435958333334));
#260985=CARTESIAN_POINT('Ctrl Pts',(-46.8967285350793,-57.4754524783487,
-46.4852625));
#260986=CARTESIAN_POINT('Ctrl Pts',(-46.2995345158897,-58.5098228615615,
-46.4269291666667));
#260987=CARTESIAN_POINT('Ctrl Pts',(-45.7023404967,-59.5441932447742,-46.3685958333333));
#260988=CARTESIAN_POINT('Ctrl Pts',(-44.5079524583208,-59.5441932447742,
-46.3102625));
#260989=CARTESIAN_POINT('Ctrl Pts',(-43.3135644199415,-59.5441932447742,
-46.2519291666667));
#260990=CARTESIAN_POINT('Ctrl Pts',(-42.7163704007519,-58.5098228615615,
-46.1935958333333));
#260991=CARTESIAN_POINT('Ctrl Pts',(-42.1191763815623,-57.4754524783487,
-46.1352625));
#260992=CARTESIAN_POINT('Ctrl Pts',(-42.7163704007519,-56.4410820951361,
-46.0769291666667));
#260993=CARTESIAN_POINT('Ctrl Pts',(-43.3135644199415,-55.4067117119233,
-46.0185958333334));
#260994=CARTESIAN_POINT('Ctrl Pts',(-44.5079524583208,-55.4067117119234,
-45.9602625));
#260995=CARTESIAN_POINT('Ctrl Pts',(-45.7023404967,-55.4067117119233,-45.9019291666667));
#260996=CARTESIAN_POINT('Ctrl Pts',(-46.2995345158897,-56.4410820951361,
-45.8435958333333));
#260997=CARTESIAN_POINT('Ctrl Pts',(-46.8967285350793,-57.4754524783487,
-45.7852625));
#260998=CARTESIAN_POINT('Ctrl Pts',(-46.2995345158897,-58.5098228615615,
-45.7269291666667));
#260999=CARTESIAN_POINT('Ctrl Pts',(-45.7023404967,-59.5441932447742,-45.6685958333334));
#261000=CARTESIAN_POINT('Ctrl Pts',(-44.5079524583208,-59.5441932447742,
-45.6102625));
#261001=CARTESIAN_POINT('Ctrl Pts',(-43.3135644199415,-59.5441932447742,
-45.5519291666667));
#261002=CARTESIAN_POINT('Ctrl Pts',(-42.7163704007519,-58.5098228615615,
-45.4935958333333));
#261003=CARTESIAN_POINT('Ctrl Pts',(-42.1191763815623,-57.4754524783487,
-45.4352625));
#261004=CARTESIAN_POINT('Ctrl Pts',(-42.7163704007519,-56.4410820951361,
-45.3769291666667));
#261005=CARTESIAN_POINT('Ctrl Pts',(-43.3135644199415,-55.4067117119233,
-45.3185958333333));
#261006=CARTESIAN_POINT('Ctrl Pts',(-44.5079524583208,-55.4067117119234,
-45.2602625));
#261007=CARTESIAN_POINT('Ctrl Pts',(-45.7023404967,-55.4067117119233,-45.2019291666667));
#261008=CARTESIAN_POINT('Ctrl Pts',(-46.2995345158897,-56.4410820951361,
-45.1435958333334));
#261009=CARTESIAN_POINT('Ctrl Pts',(-46.8967285350793,-57.4754524783487,
-45.0852625));
#261010=CARTESIAN_POINT('Ctrl Pts',(-46.2995345158897,-58.5098228615615,
-45.0269291666667));
#261011=CARTESIAN_POINT('Ctrl Pts',(-45.7023404967,-59.5441932447742,-44.9685958333334));
#261012=CARTESIAN_POINT('Ctrl Pts',(-44.5079524583208,-59.5441932447742,
-44.9102625));
#261013=CARTESIAN_POINT('Ctrl Pts',(-43.3135644199415,-59.5441932447742,
-44.8519291666667));
#261014=CARTESIAN_POINT('Ctrl Pts',(-42.7163704007519,-58.5098228615615,
-44.7935958333333));
#261015=CARTESIAN_POINT('Ctrl Pts',(-42.1191763815623,-57.4754524783487,
-44.7352625));
#261016=CARTESIAN_POINT('Ctrl Pts',(-42.7163704007519,-56.4410820951361,
-44.6769291666667));
#261017=CARTESIAN_POINT('Ctrl Pts',(-43.3135644199415,-55.4067117119233,
-44.6185958333334));
#261018=CARTESIAN_POINT('Ctrl Pts',(-44.5079524583208,-55.4067117119234,
-44.5602625));
#261019=CARTESIAN_POINT('Ctrl Pts',(-45.7023404967,-55.4067117119233,-44.5019291666667));
#261020=CARTESIAN_POINT('Ctrl Pts',(-46.2995345158897,-56.4410820951361,
-44.4435958333333));
#261021=CARTESIAN_POINT('Ctrl Pts',(-46.8967285350793,-57.4754524783487,
-44.3852625));
#261022=CARTESIAN_POINT('Ctrl Pts',(-46.2995345158897,-58.5098228615615,
-44.3269291666667));
#261023=CARTESIAN_POINT('Ctrl Pts',(-45.7023404967,-59.5441932447742,-44.2685958333334));
#261024=CARTESIAN_POINT('Ctrl Pts',(-44.5079524583208,-59.5441932447742,
-44.2102625));
#261025=CARTESIAN_POINT('Ctrl Pts',(-43.3135644199415,-59.5441932447742,
-44.1519291666667));
#261026=CARTESIAN_POINT('Ctrl Pts',(-42.7163704007519,-58.5098228615615,
-44.0935958333334));
#261027=CARTESIAN_POINT('Ctrl Pts',(-42.1191763815623,-57.4754524783487,
-44.0352625));
#261028=CARTESIAN_POINT('Ctrl Pts',(-42.7163704007519,-56.4410820951361,
-43.9769291666667));
#261029=CARTESIAN_POINT('Ctrl Pts',(-43.3135644199415,-55.4067117119233,
-43.9185958333334));
#261030=CARTESIAN_POINT('Ctrl Pts',(-44.5079524583208,-55.4067117119234,
-43.8602625));
#261031=CARTESIAN_POINT('Ctrl Pts',(-45.7023404967,-55.4067117119233,-43.8019291666667));
#261032=CARTESIAN_POINT('Ctrl Pts',(-46.2995345158897,-56.4410820951361,
-43.7435958333334));
#261033=CARTESIAN_POINT('Ctrl Pts',(-46.8967285350793,-57.4754524783487,
-43.6852625));
#261034=CARTESIAN_POINT('Ctrl Pts',(-46.2995345158897,-58.5098228615615,
-43.6269291666667));
#261035=CARTESIAN_POINT('Ctrl Pts',(-45.7023404967,-59.5441932447742,-43.5685958333334));
#261036=CARTESIAN_POINT('Ctrl Pts',(-44.5079524583208,-59.5441932447742,
-43.5102625));
#261037=CARTESIAN_POINT('Ctrl Pts',(-43.3135644199415,-59.5441932447742,
-43.4519291666667));
#261038=CARTESIAN_POINT('Ctrl Pts',(-42.7163704007519,-58.5098228615615,
-43.3935958333334));
#261039=CARTESIAN_POINT('Ctrl Pts',(-42.1191763815623,-57.4754524783487,
-43.3352625));
#261040=CARTESIAN_POINT('Ctrl Pts',(-42.7163704007519,-56.4410820951361,
-43.2769291666667));
#261041=CARTESIAN_POINT('Ctrl Pts',(-43.3135644199415,-55.4067117119233,
-43.2185958333334));
#261042=CARTESIAN_POINT('Ctrl Pts',(-44.5079524583208,-55.4067117119234,
-43.1602625));
#261043=CARTESIAN_POINT('Ctrl Pts',(-45.7023404967,-55.4067117119233,-43.1019291666667));
#261044=CARTESIAN_POINT('Ctrl Pts',(-46.2995345158897,-56.4410820951361,
-43.0435958333334));
#261045=CARTESIAN_POINT('Ctrl Pts',(-46.8967285350793,-57.4754524783487,
-42.9852625));
#261046=CARTESIAN_POINT('Ctrl Pts',(-46.2995345158897,-58.5098228615615,
-42.9269291666667));
#261047=CARTESIAN_POINT('Ctrl Pts',(-45.7023404967,-59.5441932447742,-42.8685958333333));
#261048=CARTESIAN_POINT('Ctrl Pts',(-44.5079524583208,-59.5441932447742,
-42.8102625));
#261049=CARTESIAN_POINT('Ctrl Pts',(-43.3135644199415,-59.5441932447742,
-42.7519291666667));
#261050=CARTESIAN_POINT('Ctrl Pts',(-42.7163704007519,-58.5098228615615,
-42.6935958333333));
#261051=CARTESIAN_POINT('Ctrl Pts',(-42.1191763815623,-57.4754524783487,
-42.6352625));
#261052=CARTESIAN_POINT('Ctrl Pts',(-42.7163704007519,-56.4410820951361,
-42.5769291666667));
#261053=CARTESIAN_POINT('Ctrl Pts',(-43.3135644199415,-55.4067117119233,
-42.5185958333333));
#261054=CARTESIAN_POINT('Ctrl Pts',(-44.5079524583208,-55.4067117119234,
-42.4602625));
#261055=CARTESIAN_POINT('Ctrl Pts',(-45.7023404967,-55.4067117119233,-42.4019291666666));
#261056=CARTESIAN_POINT('Ctrl Pts',(-46.2995345158897,-56.4410820951361,
-42.3435958333334));
#261057=CARTESIAN_POINT('Ctrl Pts',(-46.8967285350793,-57.4754524783487,
-42.2852625));
#261058=CARTESIAN_POINT('Ctrl Pts',(-46.2995345158897,-58.5098228615615,
-42.2269291666667));
#261059=CARTESIAN_POINT('Ctrl Pts',(-45.7023404967,-59.5441932447742,-42.1685958333333));
#261060=CARTESIAN_POINT('Ctrl Pts',(-44.5079524583208,-59.5441932447742,
-42.1102625));
#261061=CARTESIAN_POINT('Ctrl Pts',(-43.3135644199415,-59.5441932447742,
-42.0519291666667));
#261062=CARTESIAN_POINT('Ctrl Pts',(-42.7163704007519,-58.5098228615615,
-41.9935958333334));
#261063=CARTESIAN_POINT('Ctrl Pts',(-42.1191763815623,-57.4754524783487,
-41.9352625));
#261064=CARTESIAN_POINT('Ctrl Pts',(-42.7163704007519,-56.4410820951361,
-41.8769291666667));
#261065=CARTESIAN_POINT('Ctrl Pts',(-43.3135644199415,-55.4067117119233,
-41.8185958333333));
#261066=CARTESIAN_POINT('Ctrl Pts',(-44.5079524583208,-55.4067117119234,
-41.7602625));
#261067=CARTESIAN_POINT('Ctrl Pts',(-45.7023404967,-55.4067117119233,-41.7019291666667));
#261068=CARTESIAN_POINT('Ctrl Pts',(-46.2995345158897,-56.4410820951361,
-41.6435958333334));
#261069=CARTESIAN_POINT('Ctrl Pts',(-46.8967285350793,-57.4754524783487,
-41.5852625));
#261070=CARTESIAN_POINT('Ctrl Pts',(-46.2995345158897,-58.5098228615615,
-41.5269291666667));
#261071=CARTESIAN_POINT('Ctrl Pts',(-45.7023404967,-59.5441932447742,-41.4685958333333));
#261072=CARTESIAN_POINT('Ctrl Pts',(-44.5079524583208,-59.5441932447742,
-41.4102625));
#261073=CARTESIAN_POINT('Ctrl Pts',(-43.3135644199415,-59.5441932447742,
-41.3519291666666));
#261074=CARTESIAN_POINT('Ctrl Pts',(-42.7163704007519,-58.5098228615615,
-41.2935958333334));
#261075=CARTESIAN_POINT('Ctrl Pts',(-42.1191763815623,-57.4754524783487,
-41.2352625));
#261076=CARTESIAN_POINT('Ctrl Pts',(-42.7163704007519,-56.4410820951361,
-41.1769291666667));
#261077=CARTESIAN_POINT('Ctrl Pts',(-43.3135644199415,-55.4067117119233,
-41.1185958333333));
#261078=CARTESIAN_POINT('Ctrl Pts',(-44.5079524583208,-55.4067117119234,
-41.0602625));
#261079=CARTESIAN_POINT('Ctrl Pts',(-45.7023404967,-55.4067117119233,-41.0019291666666));
#261080=CARTESIAN_POINT('Ctrl Pts',(-46.2995345158897,-56.4410820951361,
-40.9435958333334));
#261081=CARTESIAN_POINT('Ctrl Pts',(-46.8967285350793,-57.4754524783487,
-40.8852625));
#261082=CARTESIAN_POINT('Ctrl Pts',(-46.2995345158897,-58.5098228615615,
-40.8269291666667));
#261083=CARTESIAN_POINT('Ctrl Pts',(-45.7023404967,-59.5441932447742,-40.7685958333333));
#261084=CARTESIAN_POINT('Ctrl Pts',(-44.5079524583208,-59.5441932447742,
-40.7102625));
#261085=CARTESIAN_POINT('Ctrl Pts',(-43.3135644199415,-59.5441932447742,
-40.6519291666667));
#261086=CARTESIAN_POINT('Ctrl Pts',(-42.7163704007519,-58.5098228615615,
-40.5935958333334));
#261087=CARTESIAN_POINT('Ctrl Pts',(-42.1191763815623,-57.4754524783487,
-40.5352625));
#261088=CARTESIAN_POINT('Ctrl Pts',(-42.7163704007519,-56.4410820951361,
-40.4769291666667));
#261089=CARTESIAN_POINT('Ctrl Pts',(-43.3135644199415,-55.4067117119233,
-40.4185958333333));
#261090=CARTESIAN_POINT('Ctrl Pts',(-44.5079524583208,-55.4067117119234,
-40.3602625));
#261091=CARTESIAN_POINT('Ctrl Pts',(-45.7023404967,-55.4067117119233,-40.3019291666667));
#261092=CARTESIAN_POINT('Ctrl Pts',(-46.2995345158897,-56.4410820951361,
-40.2435958333334));
#261093=CARTESIAN_POINT('Ctrl Pts',(-46.8967285350793,-57.4754524783487,
-40.1852625));
#261094=CARTESIAN_POINT('Ctrl Pts',(-46.2995345158897,-58.5098228615615,
-40.1269291666666));
#261095=CARTESIAN_POINT('Ctrl Pts',(-45.7023404967,-59.5441932447742,-40.0685958333333));
#261096=CARTESIAN_POINT('Ctrl Pts',(-44.5079524583208,-59.5441932447742,
-40.0102625));
#261097=CARTESIAN_POINT('Ctrl Pts',(-43.3135644199415,-59.5441932447742,
-39.9519291666667));
#261098=CARTESIAN_POINT('Ctrl Pts',(-42.7163704007519,-58.5098228615615,
-39.8935958333334));
#261099=CARTESIAN_POINT('Ctrl Pts',(-42.1191763815623,-57.4754524783487,
-39.8352625));
#261100=CARTESIAN_POINT('Ctrl Pts',(-42.7163704007519,-56.4410820951361,
-39.7769291666667));
#261101=CARTESIAN_POINT('Ctrl Pts',(-43.3135644199415,-55.4067117119233,
-39.7185958333334));
#261102=CARTESIAN_POINT('Ctrl Pts',(-44.5079524583208,-55.4067117119234,
-39.6602625));
#261103=CARTESIAN_POINT('Ctrl Pts',(-45.7023404967,-55.4067117119233,-39.6019291666667));
#261104=CARTESIAN_POINT('Ctrl Pts',(-46.2995345158897,-56.4410820951361,
-39.5435958333333));
#261105=CARTESIAN_POINT('Ctrl Pts',(-46.8967285350793,-57.4754524783487,
-39.4852625));
#261106=CARTESIAN_POINT('Ctrl Pts',(-46.2995345158897,-58.5098228615615,
-39.4269291666667));
#261107=CARTESIAN_POINT('Ctrl Pts',(-45.7023404967,-59.5441932447742,-39.3685958333334));
#261108=CARTESIAN_POINT('Ctrl Pts',(-44.5079524583208,-59.5441932447742,
-39.3102625));
#261109=CARTESIAN_POINT('Ctrl Pts',(-43.3135644199415,-59.5441932447742,
-39.2519291666667));
#261110=CARTESIAN_POINT('Ctrl Pts',(-42.7163704007519,-58.5098228615615,
-39.1935958333334));
#261111=CARTESIAN_POINT('Ctrl Pts',(-42.1191763815623,-57.4754524783487,
-39.1352625));
#261112=CARTESIAN_POINT('Ctrl Pts',(-42.7163704007519,-56.4410820951361,
-39.0769291666667));
#261113=CARTESIAN_POINT('Ctrl Pts',(-43.3135644199415,-55.4067117119233,
-39.0185958333334));
#261114=CARTESIAN_POINT('Ctrl Pts',(-44.5079524583208,-55.4067117119234,
-38.9602625));
#261115=CARTESIAN_POINT('Ctrl Pts',(-45.7023404967,-55.4067117119233,-38.9019291666667));
#261116=CARTESIAN_POINT('Ctrl Pts',(-46.2995345158897,-56.4410820951361,
-38.8435958333333));
#261117=CARTESIAN_POINT('Ctrl Pts',(-46.8967285350793,-57.4754524783487,
-38.7852625));
#261118=CARTESIAN_POINT('Ctrl Pts',(-46.2995345158897,-58.5098228615615,
-38.7269291666667));
#261119=CARTESIAN_POINT('Ctrl Pts',(-45.7023404967,-59.5441932447742,-38.6685958333334));
#261120=CARTESIAN_POINT('Ctrl Pts',(-44.5079524583208,-59.5441932447742,
-38.6102625));
#261121=CARTESIAN_POINT('Ctrl Pts',(-43.3135644199415,-59.5441932447742,
-38.5519291666667));
#261122=CARTESIAN_POINT('Ctrl Pts',(-42.7163704007519,-58.5098228615615,
-38.4935958333334));
#261123=CARTESIAN_POINT('Ctrl Pts',(-42.1191763815623,-57.4754524783487,
-38.4352625));
#261124=CARTESIAN_POINT('Ctrl Pts',(-42.7163704007519,-56.4410820951361,
-38.3769291666667));
#261125=CARTESIAN_POINT('Ctrl Pts',(-43.3135644199415,-55.4067117119233,
-38.3185958333333));
#261126=CARTESIAN_POINT('Ctrl Pts',(-44.5079524583208,-55.4067117119234,
-38.2602625));
#261127=CARTESIAN_POINT('Ctrl Pts',(-45.7023404967,-55.4067117119233,-38.2019291666667));
#261128=CARTESIAN_POINT('Ctrl Pts',(-46.2995345158897,-56.4410820951361,
-38.1435958333334));
#261129=CARTESIAN_POINT('Ctrl Pts',(-46.8967285350793,-57.4754524783487,
-38.0852625));
#261130=CARTESIAN_POINT('Ctrl Pts',(-46.2995345158897,-58.5098228615615,
-38.0269291666667));
#261131=CARTESIAN_POINT('Ctrl Pts',(-45.7023404967,-59.5441932447742,-37.9685958333333));
#261132=CARTESIAN_POINT('Ctrl Pts',(-44.5079524583208,-59.5441932447742,
-37.9102625));
#261133=CARTESIAN_POINT('Ctrl Pts',(-43.3135644199415,-59.5441932447742,
-37.8519291666667));
#261134=CARTESIAN_POINT('Ctrl Pts',(-42.7163704007519,-58.5098228615615,
-37.7935958333334));
#261135=CARTESIAN_POINT('Ctrl Pts',(-42.1191763815623,-57.4754524783487,
-37.7352625));
#261136=CARTESIAN_POINT('Ctrl Pts',(-42.7163704007519,-56.4410820951361,
-37.6769291666667));
#261137=CARTESIAN_POINT('Ctrl Pts',(-43.3135644199415,-55.4067117119233,
-37.6185958333333));
#261138=CARTESIAN_POINT('Ctrl Pts',(-44.5079524583208,-55.4067117119234,
-37.5602625));
#261139=CARTESIAN_POINT('Ctrl Pts',(-45.7023404967,-55.4067117119233,-37.5019291666667));
#261140=CARTESIAN_POINT('Ctrl Pts',(-46.2995345158897,-56.4410820951361,
-37.4435958333333));
#261141=CARTESIAN_POINT('Ctrl Pts',(-46.8967285350793,-57.4754524783487,
-37.3852625));
#261142=CARTESIAN_POINT('Ctrl Pts',(-46.2995345158897,-58.5098228615615,
-37.3269291666667));
#261143=CARTESIAN_POINT('Ctrl Pts',(-45.7023404967,-59.5441932447742,-37.2685958333333));
#261144=CARTESIAN_POINT('Ctrl Pts',(-44.5079524583208,-59.5441932447742,
-37.2102625));
#261145=CARTESIAN_POINT('Ctrl Pts',(-43.3135644199415,-59.5441932447742,
-37.1519291666667));
#261146=CARTESIAN_POINT('Ctrl Pts',(-42.7163704007519,-58.5098228615615,
-37.0935958333333));
#261147=CARTESIAN_POINT('Ctrl Pts',(-42.1191763815623,-57.4754524783487,
-37.0352625));
#261148=CARTESIAN_POINT('Ctrl Pts',(-42.7163704007519,-56.4410820951361,
-36.9769291666667));
#261149=CARTESIAN_POINT('Ctrl Pts',(-43.3135644199415,-55.4067117119233,
-36.9185958333333));
#261150=CARTESIAN_POINT('Ctrl Pts',(-44.5079524583208,-55.4067117119234,
-36.8602625));
#261151=CARTESIAN_POINT('Ctrl Pts',(-45.7023404967,-55.4067117119233,-36.8019291666666));
#261152=CARTESIAN_POINT('Ctrl Pts',(-46.2995345158897,-56.4410820951361,
-36.7435958333334));
#261153=CARTESIAN_POINT('Ctrl Pts',(-46.8967285350793,-57.4754524783487,
-36.6852625));
#261154=CARTESIAN_POINT('Ctrl Pts',(-46.2995345158897,-58.5098228615615,
-36.6269291666667));
#261155=CARTESIAN_POINT('Ctrl Pts',(-46.222006582932,-58.64410518045,-36.6193563132714));
#261156=CARTESIAN_POINT('Ctrl Pts',(-46.1253278975281,-58.7653303978899,
-36.611216324118));
#261157=CARTESIAN_POINT('Ctrl Pts',(-44.5079524583208,-59.1441976086192,
-52.8412000882087));
#261158=CARTESIAN_POINT('Ctrl Pts',(-43.5445020081503,-59.1441976086192,
-52.7828667548754));
#261159=CARTESIAN_POINT('Ctrl Pts',(-43.062776783065,-58.309825043484,-52.7245334215421));
#261160=CARTESIAN_POINT('Ctrl Pts',(-42.5810515579797,-57.4754524783487,
-52.6662000882087));
#261161=CARTESIAN_POINT('Ctrl Pts',(-43.062776783065,-56.6410799132135,
-52.6078667548754));
#261162=CARTESIAN_POINT('Ctrl Pts',(-43.5445020081503,-55.8067073480783,
-52.549533421542));
#261163=CARTESIAN_POINT('Ctrl Pts',(-44.5079524583208,-55.8067073480783,
-52.4912000882087));
#261164=CARTESIAN_POINT('Ctrl Pts',(-45.4714029084913,-55.8067073480783,
-52.4328667548755));
#261165=CARTESIAN_POINT('Ctrl Pts',(-45.9531281335766,-56.6410799132135,
-52.3745334215421));
#261166=CARTESIAN_POINT('Ctrl Pts',(-46.4348533586618,-57.4754524783487,
-52.3162000882088));
#261167=CARTESIAN_POINT('Ctrl Pts',(-45.9531281335766,-58.309825043484,
-52.2578667548754));
#261168=CARTESIAN_POINT('Ctrl Pts',(-45.4714029084913,-59.1441976086192,
-52.1995334215421));
#261169=CARTESIAN_POINT('Ctrl Pts',(-44.5079524583208,-59.1441976086192,
-52.1412000882087));
#261170=CARTESIAN_POINT('Ctrl Pts',(-43.5445020081503,-59.1441976086192,
-52.0828667548754));
#261171=CARTESIAN_POINT('Ctrl Pts',(-43.062776783065,-58.309825043484,-52.024533421542));
#261172=CARTESIAN_POINT('Ctrl Pts',(-42.5810515579797,-57.4754524783487,
-51.9662000882087));
#261173=CARTESIAN_POINT('Ctrl Pts',(-43.062776783065,-56.6410799132135,
-51.9078667548754));
#261174=CARTESIAN_POINT('Ctrl Pts',(-43.5445020081503,-55.8067073480783,
-51.8495334215421));
#261175=CARTESIAN_POINT('Ctrl Pts',(-44.5079524583208,-55.8067073480783,
-51.7912000882087));
#261176=CARTESIAN_POINT('Ctrl Pts',(-45.4714029084913,-55.8067073480783,
-51.7328667548754));
#261177=CARTESIAN_POINT('Ctrl Pts',(-45.9531281335766,-56.6410799132135,
-51.6745334215421));
#261178=CARTESIAN_POINT('Ctrl Pts',(-46.4348533586618,-57.4754524783487,
-51.6162000882087));
#261179=CARTESIAN_POINT('Ctrl Pts',(-45.9531281335766,-58.309825043484,
-51.5578667548754));
#261180=CARTESIAN_POINT('Ctrl Pts',(-45.4714029084913,-59.1441976086192,
-51.4995334215421));
#261181=CARTESIAN_POINT('Ctrl Pts',(-44.5079524583208,-59.1441976086192,
-51.4412000882087));
#261182=CARTESIAN_POINT('Ctrl Pts',(-43.5445020081503,-59.1441976086192,
-51.3828667548754));
#261183=CARTESIAN_POINT('Ctrl Pts',(-43.062776783065,-58.309825043484,-51.3245334215421));
#261184=CARTESIAN_POINT('Ctrl Pts',(-42.5810515579797,-57.4754524783487,
-51.2662000882087));
#261185=CARTESIAN_POINT('Ctrl Pts',(-43.062776783065,-56.6410799132135,
-51.2078667548754));
#261186=CARTESIAN_POINT('Ctrl Pts',(-43.5445020081503,-55.8067073480783,
-51.1495334215421));
#261187=CARTESIAN_POINT('Ctrl Pts',(-44.5079524583208,-55.8067073480783,
-51.0912000882087));
#261188=CARTESIAN_POINT('Ctrl Pts',(-45.4714029084913,-55.8067073480783,
-51.0328667548754));
#261189=CARTESIAN_POINT('Ctrl Pts',(-45.9531281335766,-56.6410799132135,
-50.974533421542));
#261190=CARTESIAN_POINT('Ctrl Pts',(-46.4348533586618,-57.4754524783487,
-50.9162000882087));
#261191=CARTESIAN_POINT('Ctrl Pts',(-45.9531281335766,-58.309825043484,
-50.8578667548754));
#261192=CARTESIAN_POINT('Ctrl Pts',(-45.4714029084913,-59.1441976086192,
-50.7995334215421));
#261193=CARTESIAN_POINT('Ctrl Pts',(-44.5079524583208,-59.1441976086192,
-50.7412000882087));
#261194=CARTESIAN_POINT('Ctrl Pts',(-43.5445020081503,-59.1441976086192,
-50.6828667548754));
#261195=CARTESIAN_POINT('Ctrl Pts',(-43.062776783065,-58.309825043484,-50.624533421542));
#261196=CARTESIAN_POINT('Ctrl Pts',(-42.5810515579797,-57.4754524783487,
-50.5662000882087));
#261197=CARTESIAN_POINT('Ctrl Pts',(-43.062776783065,-56.6410799132135,
-50.5078667548754));
#261198=CARTESIAN_POINT('Ctrl Pts',(-43.5445020081503,-55.8067073480783,
-50.4495334215421));
#261199=CARTESIAN_POINT('Ctrl Pts',(-44.5079524583208,-55.8067073480783,
-50.3912000882087));
#261200=CARTESIAN_POINT('Ctrl Pts',(-45.4714029084913,-55.8067073480783,
-50.3328667548754));
#261201=CARTESIAN_POINT('Ctrl Pts',(-45.9531281335766,-56.6410799132135,
-50.2745334215421));
#261202=CARTESIAN_POINT('Ctrl Pts',(-46.4348533586618,-57.4754524783487,
-50.2162000882088));
#261203=CARTESIAN_POINT('Ctrl Pts',(-45.9531281335766,-58.309825043484,
-50.1578667548754));
#261204=CARTESIAN_POINT('Ctrl Pts',(-45.4714029084913,-59.1441976086192,
-50.0995334215421));
#261205=CARTESIAN_POINT('Ctrl Pts',(-44.5079524583208,-59.1441976086192,
-50.0412000882087));
#261206=CARTESIAN_POINT('Ctrl Pts',(-43.5445020081503,-59.1441976086192,
-49.9828667548755));
#261207=CARTESIAN_POINT('Ctrl Pts',(-43.062776783065,-58.309825043484,-49.9245334215421));
#261208=CARTESIAN_POINT('Ctrl Pts',(-42.5810515579797,-57.4754524783487,
-49.8662000882087));
#261209=CARTESIAN_POINT('Ctrl Pts',(-43.062776783065,-56.6410799132135,
-49.8078667548754));
#261210=CARTESIAN_POINT('Ctrl Pts',(-43.5445020081503,-55.8067073480783,
-49.7495334215421));
#261211=CARTESIAN_POINT('Ctrl Pts',(-44.5079524583208,-55.8067073480783,
-49.6912000882087));
#261212=CARTESIAN_POINT('Ctrl Pts',(-45.4714029084913,-55.8067073480783,
-49.6328667548754));
#261213=CARTESIAN_POINT('Ctrl Pts',(-45.9531281335766,-56.6410799132135,
-49.5745334215421));
#261214=CARTESIAN_POINT('Ctrl Pts',(-46.4348533586618,-57.4754524783487,
-49.5162000882088));
#261215=CARTESIAN_POINT('Ctrl Pts',(-45.9531281335766,-58.309825043484,
-49.4578667548754));
#261216=CARTESIAN_POINT('Ctrl Pts',(-45.4714029084913,-59.1441976086192,
-49.3995334215421));
#261217=CARTESIAN_POINT('Ctrl Pts',(-44.5079524583208,-59.1441976086192,
-49.3412000882087));
#261218=CARTESIAN_POINT('Ctrl Pts',(-43.5445020081503,-59.1441976086192,
-49.2828667548754));
#261219=CARTESIAN_POINT('Ctrl Pts',(-43.062776783065,-58.309825043484,-49.2245334215421));
#261220=CARTESIAN_POINT('Ctrl Pts',(-42.5810515579797,-57.4754524783487,
-49.1662000882087));
#261221=CARTESIAN_POINT('Ctrl Pts',(-43.062776783065,-56.6410799132135,
-49.1078667548754));
#261222=CARTESIAN_POINT('Ctrl Pts',(-43.5445020081503,-55.8067073480783,
-49.0495334215421));
#261223=CARTESIAN_POINT('Ctrl Pts',(-44.5079524583208,-55.8067073480783,
-48.9912000882087));
#261224=CARTESIAN_POINT('Ctrl Pts',(-45.4714029084913,-55.8067073480783,
-48.9328667548754));
#261225=CARTESIAN_POINT('Ctrl Pts',(-45.9531281335766,-56.6410799132135,
-48.8745334215421));
#261226=CARTESIAN_POINT('Ctrl Pts',(-46.4348533586618,-57.4754524783487,
-48.8162000882088));
#261227=CARTESIAN_POINT('Ctrl Pts',(-45.9531281335766,-58.309825043484,
-48.7578667548754));
#261228=CARTESIAN_POINT('Ctrl Pts',(-45.4714029084913,-59.1441976086192,
-48.6995334215421));
#261229=CARTESIAN_POINT('Ctrl Pts',(-44.5079524583208,-59.1441976086192,
-48.6412000882087));
#261230=CARTESIAN_POINT('Ctrl Pts',(-43.5445020081503,-59.1441976086192,
-48.5828667548754));
#261231=CARTESIAN_POINT('Ctrl Pts',(-43.062776783065,-58.309825043484,-48.5245334215421));
#261232=CARTESIAN_POINT('Ctrl Pts',(-42.5810515579797,-57.4754524783487,
-48.4662000882088));
#261233=CARTESIAN_POINT('Ctrl Pts',(-43.062776783065,-56.6410799132135,
-48.4078667548754));
#261234=CARTESIAN_POINT('Ctrl Pts',(-43.5445020081503,-55.8067073480783,
-48.3495334215421));
#261235=CARTESIAN_POINT('Ctrl Pts',(-44.5079524583208,-55.8067073480783,
-48.2912000882087));
#261236=CARTESIAN_POINT('Ctrl Pts',(-45.4714029084913,-55.8067073480783,
-48.2328667548754));
#261237=CARTESIAN_POINT('Ctrl Pts',(-45.9531281335766,-56.6410799132135,
-48.1745334215421));
#261238=CARTESIAN_POINT('Ctrl Pts',(-46.4348533586618,-57.4754524783487,
-48.1162000882087));
#261239=CARTESIAN_POINT('Ctrl Pts',(-45.9531281335766,-58.309825043484,
-48.0578667548754));
#261240=CARTESIAN_POINT('Ctrl Pts',(-45.4714029084913,-59.1441976086192,
-47.9995334215421));
#261241=CARTESIAN_POINT('Ctrl Pts',(-44.5079524583208,-59.1441976086192,
-47.9412000882087));
#261242=CARTESIAN_POINT('Ctrl Pts',(-43.5445020081503,-59.1441976086192,
-47.8828667548754));
#261243=CARTESIAN_POINT('Ctrl Pts',(-43.062776783065,-58.309825043484,-47.824533421542));
#261244=CARTESIAN_POINT('Ctrl Pts',(-42.5810515579797,-57.4754524783487,
-47.7662000882088));
#261245=CARTESIAN_POINT('Ctrl Pts',(-43.062776783065,-56.6410799132135,
-47.7078667548754));
#261246=CARTESIAN_POINT('Ctrl Pts',(-43.5445020081503,-55.8067073480783,
-47.6495334215421));
#261247=CARTESIAN_POINT('Ctrl Pts',(-44.5079524583208,-55.8067073480783,
-47.5912000882087));
#261248=CARTESIAN_POINT('Ctrl Pts',(-45.4714029084913,-55.8067073480783,
-47.5328667548754));
#261249=CARTESIAN_POINT('Ctrl Pts',(-45.9531281335766,-56.6410799132135,
-47.4745334215421));
#261250=CARTESIAN_POINT('Ctrl Pts',(-46.4348533586618,-57.4754524783487,
-47.4162000882087));
#261251=CARTESIAN_POINT('Ctrl Pts',(-45.9531281335766,-58.309825043484,
-47.3578667548754));
#261252=CARTESIAN_POINT('Ctrl Pts',(-45.4714029084913,-59.1441976086192,
-47.2995334215421));
#261253=CARTESIAN_POINT('Ctrl Pts',(-44.5079524583208,-59.1441976086192,
-47.2412000882087));
#261254=CARTESIAN_POINT('Ctrl Pts',(-43.5445020081503,-59.1441976086192,
-47.1828667548754));
#261255=CARTESIAN_POINT('Ctrl Pts',(-43.062776783065,-58.309825043484,-47.124533421542));
#261256=CARTESIAN_POINT('Ctrl Pts',(-42.5810515579797,-57.4754524783487,
-47.0662000882087));
#261257=CARTESIAN_POINT('Ctrl Pts',(-43.062776783065,-56.6410799132135,
-47.0078667548754));
#261258=CARTESIAN_POINT('Ctrl Pts',(-43.5445020081503,-55.8067073480783,
-46.9495334215421));
#261259=CARTESIAN_POINT('Ctrl Pts',(-44.5079524583208,-55.8067073480783,
-46.8912000882087));
#261260=CARTESIAN_POINT('Ctrl Pts',(-45.4714029084913,-55.8067073480783,
-46.8328667548754));
#261261=CARTESIAN_POINT('Ctrl Pts',(-45.9531281335766,-56.6410799132135,
-46.7745334215421));
#261262=CARTESIAN_POINT('Ctrl Pts',(-46.4348533586618,-57.4754524783487,
-46.7162000882087));
#261263=CARTESIAN_POINT('Ctrl Pts',(-45.9531281335766,-58.309825043484,
-46.6578667548754));
#261264=CARTESIAN_POINT('Ctrl Pts',(-45.4714029084913,-59.1441976086192,
-46.5995334215421));
#261265=CARTESIAN_POINT('Ctrl Pts',(-44.5079524583208,-59.1441976086192,
-46.5412000882087));
#261266=CARTESIAN_POINT('Ctrl Pts',(-43.5445020081503,-59.1441976086192,
-46.4828667548754));
#261267=CARTESIAN_POINT('Ctrl Pts',(-43.062776783065,-58.309825043484,-46.4245334215421));
#261268=CARTESIAN_POINT('Ctrl Pts',(-42.5810515579797,-57.4754524783487,
-46.3662000882087));
#261269=CARTESIAN_POINT('Ctrl Pts',(-43.062776783065,-56.6410799132135,
-46.3078667548754));
#261270=CARTESIAN_POINT('Ctrl Pts',(-43.5445020081503,-55.8067073480783,
-46.2495334215421));
#261271=CARTESIAN_POINT('Ctrl Pts',(-44.5079524583208,-55.8067073480783,
-46.1912000882087));
#261272=CARTESIAN_POINT('Ctrl Pts',(-45.4714029084913,-55.8067073480783,
-46.1328667548754));
#261273=CARTESIAN_POINT('Ctrl Pts',(-45.9531281335766,-56.6410799132135,
-46.0745334215421));
#261274=CARTESIAN_POINT('Ctrl Pts',(-46.4348533586618,-57.4754524783487,
-46.0162000882087));
#261275=CARTESIAN_POINT('Ctrl Pts',(-45.9531281335766,-58.309825043484,
-45.9578667548754));
#261276=CARTESIAN_POINT('Ctrl Pts',(-45.4714029084913,-59.1441976086192,
-45.8995334215421));
#261277=CARTESIAN_POINT('Ctrl Pts',(-44.5079524583208,-59.1441976086192,
-45.8412000882087));
#261278=CARTESIAN_POINT('Ctrl Pts',(-43.5445020081503,-59.1441976086192,
-45.7828667548754));
#261279=CARTESIAN_POINT('Ctrl Pts',(-43.062776783065,-58.309825043484,-45.724533421542));
#261280=CARTESIAN_POINT('Ctrl Pts',(-42.5810515579797,-57.4754524783487,
-45.6662000882087));
#261281=CARTESIAN_POINT('Ctrl Pts',(-43.062776783065,-56.6410799132135,
-45.6078667548754));
#261282=CARTESIAN_POINT('Ctrl Pts',(-43.5445020081503,-55.8067073480783,
-45.5495334215421));
#261283=CARTESIAN_POINT('Ctrl Pts',(-44.5079524583208,-55.8067073480783,
-45.4912000882087));
#261284=CARTESIAN_POINT('Ctrl Pts',(-45.4714029084913,-55.8067073480783,
-45.4328667548754));
#261285=CARTESIAN_POINT('Ctrl Pts',(-45.9531281335766,-56.6410799132135,
-45.3745334215421));
#261286=CARTESIAN_POINT('Ctrl Pts',(-46.4348533586618,-57.4754524783487,
-45.3162000882088));
#261287=CARTESIAN_POINT('Ctrl Pts',(-45.9531281335766,-58.309825043484,
-45.2578667548754));
#261288=CARTESIAN_POINT('Ctrl Pts',(-45.4714029084913,-59.1441976086192,
-45.1995334215421));
#261289=CARTESIAN_POINT('Ctrl Pts',(-44.5079524583208,-59.1441976086192,
-45.1412000882087));
#261290=CARTESIAN_POINT('Ctrl Pts',(-43.5445020081503,-59.1441976086192,
-45.0828667548754));
#261291=CARTESIAN_POINT('Ctrl Pts',(-43.062776783065,-58.309825043484,-45.0245334215421));
#261292=CARTESIAN_POINT('Ctrl Pts',(-42.5810515579797,-57.4754524783487,
-44.9662000882088));
#261293=CARTESIAN_POINT('Ctrl Pts',(-43.062776783065,-56.6410799132135,
-44.9078667548754));
#261294=CARTESIAN_POINT('Ctrl Pts',(-43.5445020081503,-55.8067073480783,
-44.8495334215421));
#261295=CARTESIAN_POINT('Ctrl Pts',(-44.5079524583208,-55.8067073480783,
-44.7912000882087));
#261296=CARTESIAN_POINT('Ctrl Pts',(-45.4714029084913,-55.8067073480783,
-44.7328667548754));
#261297=CARTESIAN_POINT('Ctrl Pts',(-45.9531281335766,-56.6410799132135,
-44.6745334215421));
#261298=CARTESIAN_POINT('Ctrl Pts',(-46.4348533586618,-57.4754524783487,
-44.6162000882088));
#261299=CARTESIAN_POINT('Ctrl Pts',(-45.9531281335766,-58.309825043484,
-44.5578667548754));
#261300=CARTESIAN_POINT('Ctrl Pts',(-45.4714029084913,-59.1441976086192,
-44.4995334215421));
#261301=CARTESIAN_POINT('Ctrl Pts',(-44.5079524583208,-59.1441976086192,
-44.4412000882087));
#261302=CARTESIAN_POINT('Ctrl Pts',(-43.5445020081503,-59.1441976086192,
-44.3828667548754));
#261303=CARTESIAN_POINT('Ctrl Pts',(-43.062776783065,-58.309825043484,-44.3245334215421));
#261304=CARTESIAN_POINT('Ctrl Pts',(-42.5810515579797,-57.4754524783487,
-44.2662000882088));
#261305=CARTESIAN_POINT('Ctrl Pts',(-43.062776783065,-56.6410799132135,
-44.2078667548754));
#261306=CARTESIAN_POINT('Ctrl Pts',(-43.5445020081503,-55.8067073480783,
-44.1495334215421));
#261307=CARTESIAN_POINT('Ctrl Pts',(-44.5079524583208,-55.8067073480783,
-44.0912000882087));
#261308=CARTESIAN_POINT('Ctrl Pts',(-45.4714029084913,-55.8067073480783,
-44.0328667548754));
#261309=CARTESIAN_POINT('Ctrl Pts',(-45.9531281335766,-56.6410799132135,
-43.9745334215421));
#261310=CARTESIAN_POINT('Ctrl Pts',(-46.4348533586618,-57.4754524783487,
-43.9162000882088));
#261311=CARTESIAN_POINT('Ctrl Pts',(-45.9531281335766,-58.309825043484,
-43.8578667548754));
#261312=CARTESIAN_POINT('Ctrl Pts',(-45.4714029084913,-59.1441976086192,
-43.7995334215421));
#261313=CARTESIAN_POINT('Ctrl Pts',(-44.5079524583208,-59.1441976086192,
-43.7412000882087));
#261314=CARTESIAN_POINT('Ctrl Pts',(-43.5445020081503,-59.1441976086192,
-43.6828667548754));
#261315=CARTESIAN_POINT('Ctrl Pts',(-43.062776783065,-58.309825043484,-43.6245334215421));
#261316=CARTESIAN_POINT('Ctrl Pts',(-42.5810515579797,-57.4754524783487,
-43.5662000882088));
#261317=CARTESIAN_POINT('Ctrl Pts',(-43.062776783065,-56.6410799132135,
-43.5078667548754));
#261318=CARTESIAN_POINT('Ctrl Pts',(-43.5445020081503,-55.8067073480783,
-43.4495334215421));
#261319=CARTESIAN_POINT('Ctrl Pts',(-44.5079524583208,-55.8067073480783,
-43.3912000882087));
#261320=CARTESIAN_POINT('Ctrl Pts',(-45.4714029084913,-55.8067073480783,
-43.3328667548754));
#261321=CARTESIAN_POINT('Ctrl Pts',(-45.9531281335766,-56.6410799132135,
-43.2745334215421));
#261322=CARTESIAN_POINT('Ctrl Pts',(-46.4348533586618,-57.4754524783487,
-43.2162000882088));
#261323=CARTESIAN_POINT('Ctrl Pts',(-45.9531281335766,-58.309825043484,
-43.1578667548754));
#261324=CARTESIAN_POINT('Ctrl Pts',(-45.4714029084913,-59.1441976086192,
-43.0995334215421));
#261325=CARTESIAN_POINT('Ctrl Pts',(-44.5079524583208,-59.1441976086192,
-43.0412000882087));
#261326=CARTESIAN_POINT('Ctrl Pts',(-43.5445020081503,-59.1441976086192,
-42.9828667548754));
#261327=CARTESIAN_POINT('Ctrl Pts',(-43.062776783065,-58.309825043484,-42.9245334215421));
#261328=CARTESIAN_POINT('Ctrl Pts',(-42.5810515579797,-57.4754524783487,
-42.8662000882087));
#261329=CARTESIAN_POINT('Ctrl Pts',(-43.062776783065,-56.6410799132135,
-42.8078667548754));
#261330=CARTESIAN_POINT('Ctrl Pts',(-43.5445020081503,-55.8067073480783,
-42.7495334215421));
#261331=CARTESIAN_POINT('Ctrl Pts',(-44.5079524583208,-55.8067073480783,
-42.6912000882087));
#261332=CARTESIAN_POINT('Ctrl Pts',(-45.4714029084913,-55.8067073480783,
-42.6328667548754));
#261333=CARTESIAN_POINT('Ctrl Pts',(-45.9531281335766,-56.6410799132135,
-42.5745334215421));
#261334=CARTESIAN_POINT('Ctrl Pts',(-46.4348533586618,-57.4754524783487,
-42.5162000882087));
#261335=CARTESIAN_POINT('Ctrl Pts',(-45.9531281335766,-58.309825043484,
-42.4578667548754));
#261336=CARTESIAN_POINT('Ctrl Pts',(-45.4714029084913,-59.1441976086192,
-42.3995334215421));
#261337=CARTESIAN_POINT('Ctrl Pts',(-44.5079524583208,-59.1441976086192,
-42.3412000882087));
#261338=CARTESIAN_POINT('Ctrl Pts',(-43.5445020081503,-59.1441976086192,
-42.2828667548754));
#261339=CARTESIAN_POINT('Ctrl Pts',(-43.062776783065,-58.309825043484,-42.2245334215421));
#261340=CARTESIAN_POINT('Ctrl Pts',(-42.5810515579797,-57.4754524783487,
-42.1662000882087));
#261341=CARTESIAN_POINT('Ctrl Pts',(-43.062776783065,-56.6410799132135,
-42.1078667548754));
#261342=CARTESIAN_POINT('Ctrl Pts',(-43.5445020081503,-55.8067073480783,
-42.0495334215421));
#261343=CARTESIAN_POINT('Ctrl Pts',(-44.5079524583208,-55.8067073480783,
-41.9912000882087));
#261344=CARTESIAN_POINT('Ctrl Pts',(-45.4714029084913,-55.8067073480783,
-41.9328667548754));
#261345=CARTESIAN_POINT('Ctrl Pts',(-45.9531281335766,-56.6410799132135,
-41.8745334215421));
#261346=CARTESIAN_POINT('Ctrl Pts',(-46.4348533586618,-57.4754524783487,
-41.8162000882087));
#261347=CARTESIAN_POINT('Ctrl Pts',(-45.9531281335766,-58.309825043484,
-41.7578667548754));
#261348=CARTESIAN_POINT('Ctrl Pts',(-45.4714029084913,-59.1441976086192,
-41.6995334215421));
#261349=CARTESIAN_POINT('Ctrl Pts',(-44.5079524583208,-59.1441976086192,
-41.6412000882087));
#261350=CARTESIAN_POINT('Ctrl Pts',(-43.5445020081503,-59.1441976086192,
-41.5828667548754));
#261351=CARTESIAN_POINT('Ctrl Pts',(-43.062776783065,-58.309825043484,-41.5245334215421));
#261352=CARTESIAN_POINT('Ctrl Pts',(-42.5810515579797,-57.4754524783487,
-41.4662000882087));
#261353=CARTESIAN_POINT('Ctrl Pts',(-43.062776783065,-56.6410799132135,
-41.4078667548754));
#261354=CARTESIAN_POINT('Ctrl Pts',(-43.5445020081503,-55.8067073480783,
-41.349533421542));
#261355=CARTESIAN_POINT('Ctrl Pts',(-44.5079524583208,-55.8067073480783,
-41.2912000882087));
#261356=CARTESIAN_POINT('Ctrl Pts',(-45.4714029084913,-55.8067073480783,
-41.2328667548754));
#261357=CARTESIAN_POINT('Ctrl Pts',(-45.9531281335766,-56.6410799132135,
-41.1745334215421));
#261358=CARTESIAN_POINT('Ctrl Pts',(-46.4348533586618,-57.4754524783487,
-41.1162000882087));
#261359=CARTESIAN_POINT('Ctrl Pts',(-45.9531281335766,-58.309825043484,
-41.0578667548754));
#261360=CARTESIAN_POINT('Ctrl Pts',(-45.4714029084913,-59.1441976086192,
-40.9995334215421));
#261361=CARTESIAN_POINT('Ctrl Pts',(-44.5079524583208,-59.1441976086192,
-40.9412000882087));
#261362=CARTESIAN_POINT('Ctrl Pts',(-43.5445020081503,-59.1441976086192,
-40.8828667548755));
#261363=CARTESIAN_POINT('Ctrl Pts',(-43.062776783065,-58.309825043484,-40.8245334215421));
#261364=CARTESIAN_POINT('Ctrl Pts',(-42.5810515579797,-57.4754524783487,
-40.7662000882087));
#261365=CARTESIAN_POINT('Ctrl Pts',(-43.062776783065,-56.6410799132135,
-40.7078667548754));
#261366=CARTESIAN_POINT('Ctrl Pts',(-43.5445020081503,-55.8067073480783,
-40.6495334215421));
#261367=CARTESIAN_POINT('Ctrl Pts',(-44.5079524583208,-55.8067073480783,
-40.5912000882087));
#261368=CARTESIAN_POINT('Ctrl Pts',(-45.4714029084913,-55.8067073480783,
-40.5328667548754));
#261369=CARTESIAN_POINT('Ctrl Pts',(-45.9531281335766,-56.6410799132135,
-40.4745334215421));
#261370=CARTESIAN_POINT('Ctrl Pts',(-46.4348533586618,-57.4754524783487,
-40.4162000882087));
#261371=CARTESIAN_POINT('Ctrl Pts',(-45.9531281335766,-58.309825043484,
-40.3578667548754));
#261372=CARTESIAN_POINT('Ctrl Pts',(-45.4714029084913,-59.1441976086192,
-40.2995334215421));
#261373=CARTESIAN_POINT('Ctrl Pts',(-44.5079524583208,-59.1441976086192,
-40.2412000882087));
#261374=CARTESIAN_POINT('Ctrl Pts',(-43.5445020081503,-59.1441976086192,
-40.1828667548754));
#261375=CARTESIAN_POINT('Ctrl Pts',(-43.062776783065,-58.309825043484,-40.1245334215421));
#261376=CARTESIAN_POINT('Ctrl Pts',(-42.5810515579797,-57.4754524783487,
-40.0662000882088));
#261377=CARTESIAN_POINT('Ctrl Pts',(-43.062776783065,-56.6410799132135,
-40.0078667548754));
#261378=CARTESIAN_POINT('Ctrl Pts',(-43.5445020081503,-55.8067073480783,
-39.9495334215421));
#261379=CARTESIAN_POINT('Ctrl Pts',(-44.5079524583208,-55.8067073480783,
-39.8912000882087));
#261380=CARTESIAN_POINT('Ctrl Pts',(-45.4714029084913,-55.8067073480783,
-39.8328667548754));
#261381=CARTESIAN_POINT('Ctrl Pts',(-45.9531281335766,-56.6410799132135,
-39.7745334215421));
#261382=CARTESIAN_POINT('Ctrl Pts',(-46.4348533586618,-57.4754524783487,
-39.7162000882088));
#261383=CARTESIAN_POINT('Ctrl Pts',(-45.9531281335766,-58.309825043484,
-39.6578667548754));
#261384=CARTESIAN_POINT('Ctrl Pts',(-45.4714029084913,-59.1441976086192,
-39.5995334215421));
#261385=CARTESIAN_POINT('Ctrl Pts',(-44.5079524583208,-59.1441976086192,
-39.5412000882087));
#261386=CARTESIAN_POINT('Ctrl Pts',(-43.5445020081503,-59.1441976086192,
-39.4828667548754));
#261387=CARTESIAN_POINT('Ctrl Pts',(-43.062776783065,-58.309825043484,-39.4245334215421));
#261388=CARTESIAN_POINT('Ctrl Pts',(-42.5810515579797,-57.4754524783487,
-39.3662000882088));
#261389=CARTESIAN_POINT('Ctrl Pts',(-43.062776783065,-56.6410799132135,
-39.3078667548754));
#261390=CARTESIAN_POINT('Ctrl Pts',(-43.5445020081503,-55.8067073480783,
-39.2495334215421));
#261391=CARTESIAN_POINT('Ctrl Pts',(-44.5079524583208,-55.8067073480783,
-39.1912000882087));
#261392=CARTESIAN_POINT('Ctrl Pts',(-45.4714029084913,-55.8067073480783,
-39.1328667548754));
#261393=CARTESIAN_POINT('Ctrl Pts',(-45.9531281335766,-56.6410799132135,
-39.0745334215421));
#261394=CARTESIAN_POINT('Ctrl Pts',(-46.4348533586618,-57.4754524783487,
-39.0162000882088));
#261395=CARTESIAN_POINT('Ctrl Pts',(-45.9531281335766,-58.309825043484,
-38.9578667548754));
#261396=CARTESIAN_POINT('Ctrl Pts',(-45.4714029084913,-59.1441976086192,
-38.8995334215421));
#261397=CARTESIAN_POINT('Ctrl Pts',(-44.5079524583208,-59.1441976086192,
-38.8412000882087));
#261398=CARTESIAN_POINT('Ctrl Pts',(-43.5445020081503,-59.1441976086192,
-38.7828667548754));
#261399=CARTESIAN_POINT('Ctrl Pts',(-43.062776783065,-58.309825043484,-38.7245334215421));
#261400=CARTESIAN_POINT('Ctrl Pts',(-42.5810515579797,-57.4754524783487,
-38.6662000882088));
#261401=CARTESIAN_POINT('Ctrl Pts',(-43.062776783065,-56.6410799132135,
-38.6078667548754));
#261402=CARTESIAN_POINT('Ctrl Pts',(-43.5445020081503,-55.8067073480783,
-38.5495334215421));
#261403=CARTESIAN_POINT('Ctrl Pts',(-44.5079524583208,-55.8067073480783,
-38.4912000882087));
#261404=CARTESIAN_POINT('Ctrl Pts',(-45.4714029084913,-55.8067073480783,
-38.4328667548754));
#261405=CARTESIAN_POINT('Ctrl Pts',(-45.9531281335766,-56.6410799132135,
-38.3745334215421));
#261406=CARTESIAN_POINT('Ctrl Pts',(-46.4348533586618,-57.4754524783487,
-38.3162000882087));
#261407=CARTESIAN_POINT('Ctrl Pts',(-45.9531281335766,-58.309825043484,
-38.2578667548754));
#261408=CARTESIAN_POINT('Ctrl Pts',(-45.4714029084913,-59.1441976086192,
-38.1995334215421));
#261409=CARTESIAN_POINT('Ctrl Pts',(-44.5079524583208,-59.1441976086192,
-38.1412000882087));
#261410=CARTESIAN_POINT('Ctrl Pts',(-43.5445020081503,-59.1441976086192,
-38.0828667548754));
#261411=CARTESIAN_POINT('Ctrl Pts',(-43.062776783065,-58.309825043484,-38.0245334215421));
#261412=CARTESIAN_POINT('Ctrl Pts',(-42.5810515579797,-57.4754524783487,
-37.9662000882088));
#261413=CARTESIAN_POINT('Ctrl Pts',(-43.062776783065,-56.6410799132135,
-37.9078667548754));
#261414=CARTESIAN_POINT('Ctrl Pts',(-43.5445020081503,-55.8067073480783,
-37.8495334215421));
#261415=CARTESIAN_POINT('Ctrl Pts',(-44.5079524583208,-55.8067073480783,
-37.7912000882087));
#261416=CARTESIAN_POINT('Ctrl Pts',(-45.4714029084913,-55.8067073480783,
-37.7328667548754));
#261417=CARTESIAN_POINT('Ctrl Pts',(-45.9531281335766,-56.6410799132135,
-37.6745334215421));
#261418=CARTESIAN_POINT('Ctrl Pts',(-46.4348533586618,-57.4754524783487,
-37.6162000882088));
#261419=CARTESIAN_POINT('Ctrl Pts',(-45.9531281335766,-58.309825043484,
-37.5578667548754));
#261420=CARTESIAN_POINT('Ctrl Pts',(-45.4714029084913,-59.1441976086192,
-37.4995334215421));
#261421=CARTESIAN_POINT('Ctrl Pts',(-44.5079524583208,-59.1441976086192,
-37.4412000882087));
#261422=CARTESIAN_POINT('Ctrl Pts',(-43.5445020081503,-59.1441976086192,
-37.3828667548754));
#261423=CARTESIAN_POINT('Ctrl Pts',(-43.062776783065,-58.309825043484,-37.3245334215421));
#261424=CARTESIAN_POINT('Ctrl Pts',(-42.5810515579797,-57.4754524783487,
-37.2662000882087));
#261425=CARTESIAN_POINT('Ctrl Pts',(-43.062776783065,-56.6410799132135,
-37.2078667548754));
#261426=CARTESIAN_POINT('Ctrl Pts',(-43.5445020081503,-55.8067073480783,
-37.1495334215421));
#261427=CARTESIAN_POINT('Ctrl Pts',(-44.5079524583208,-55.8067073480783,
-37.0912000882087));
#261428=CARTESIAN_POINT('Ctrl Pts',(-45.4714029084913,-55.8067073480783,
-37.0328667548754));
#261429=CARTESIAN_POINT('Ctrl Pts',(-45.9531281335766,-56.6410799132135,
-36.9745334215421));
#261430=CARTESIAN_POINT('Ctrl Pts',(-46.4348533586618,-57.4754524783487,
-36.9162000882087));
#261431=CARTESIAN_POINT('Ctrl Pts',(-45.9531281335766,-58.309825043484,
-36.8578667548754));
#261432=CARTESIAN_POINT('Ctrl Pts',(-45.8905903991815,-58.4181435768467,
-36.8502939014801));
#261433=CARTESIAN_POINT('Ctrl Pts',(-45.8126047529917,-58.5159296284157,
-36.8421539123268));
#261434=CARTESIAN_POINT('Ctrl Pts',(-44.5079524583208,-59.4754524783488,
-52.64995));
#261435=CARTESIAN_POINT('Ctrl Pts',(-44.3600617863357,-59.4625120445501,
-52.64995));
#261436=CARTESIAN_POINT('Ctrl Pts',(-44.2142042532552,-59.4322659035397,
-52.64995));
#261437=CARTESIAN_POINT('Ctrl Pts',(-43.9445256487742,-59.3423033429062,
-52.64995));
#261438=CARTESIAN_POINT('Ctrl Pts',(-43.8206799356501,-59.2855753019495,
-52.64995));
#261439=CARTESIAN_POINT('Ctrl Pts',(-43.4951040594959,-59.0916199608506,
-52.64995));
#261440=CARTESIAN_POINT('Ctrl Pts',(-43.3122546189713,-58.9280617429974,
-52.6499500000001));
#261441=CARTESIAN_POINT('Ctrl Pts',(-43.0527600317383,-58.5856631129985,
-52.6499500000001));
#261442=CARTESIAN_POINT('Ctrl Pts',(-42.923716913873,-58.371224501979,-52.6499500000282));
#261443=CARTESIAN_POINT('Ctrl Pts',(-42.815884786658,-57.953786980419,-52.6499500000282));
#261444=CARTESIAN_POINT('Ctrl Pts',(-42.7978378140676,-57.8061017722689,
-52.64995));
#261445=CARTESIAN_POINT('Ctrl Pts',(-42.8007193914761,-57.5178390254165,
-52.64995));
#261446=CARTESIAN_POINT('Ctrl Pts',(-42.8195756983132,-57.3784642494499,
-52.64995));
#261447=CARTESIAN_POINT('Ctrl Pts',(-42.8554737113965,-57.2430200996376,
-52.64995));
#261448=CARTESIAN_POINT('Ctrl Pts',(-44.5079524583208,-59.1441977614012,
-52.99995));
#261449=CARTESIAN_POINT('Ctrl Pts',(-43.5445019199415,-59.1441977614012,
-52.9416166666667));
#261450=CARTESIAN_POINT('Ctrl Pts',(-43.0627766507519,-58.309825119875,
-52.8832833333334));
#261451=CARTESIAN_POINT('Ctrl Pts',(-42.5810513815623,-57.4754524783487,
-52.82495));
#261452=CARTESIAN_POINT('Ctrl Pts',(-43.0627766507519,-56.6410798368225,
-52.7666166666667));
#261453=CARTESIAN_POINT('Ctrl Pts',(-43.5445019199415,-55.8067071952963,
-52.7082833333333));
#261454=CARTESIAN_POINT('Ctrl Pts',(-44.5079524583208,-55.8067071952963,
-52.64995));
#261455=CARTESIAN_POINT('Ctrl Pts',(-45.4714029967,-55.8067071952963,-52.5916166666666));
#261456=CARTESIAN_POINT('Ctrl Pts',(-45.9531282658897,-56.6410798368225,
-52.5332833333334));
#261457=CARTESIAN_POINT('Ctrl Pts',(-46.4348535350793,-57.4754524783487,
-52.4749500000001));
#261458=CARTESIAN_POINT('Ctrl Pts',(-45.9531282658897,-58.309825119875,
-52.4166166666667));
#261459=CARTESIAN_POINT('Ctrl Pts',(-45.4714029967,-59.1441977614012,-52.3582833333334));
#261460=CARTESIAN_POINT('Ctrl Pts',(-44.5079524583208,-59.1441977614012,
-52.29995));
#261461=CARTESIAN_POINT('Ctrl Pts',(-43.5445019199415,-59.1441977614012,
-52.2416166666667));
#261462=CARTESIAN_POINT('Ctrl Pts',(-43.0627766507519,-58.309825119875,
-52.1832833333333));
#261463=CARTESIAN_POINT('Ctrl Pts',(-42.5810513815623,-57.4754524783487,
-52.12495));
#261464=CARTESIAN_POINT('Ctrl Pts',(-43.0627766507519,-56.6410798368225,
-52.0666166666667));
#261465=CARTESIAN_POINT('Ctrl Pts',(-43.5445019199415,-55.8067071952963,
-52.0082833333333));
#261466=CARTESIAN_POINT('Ctrl Pts',(-44.5079524583208,-55.8067071952963,
-51.94995));
#261467=CARTESIAN_POINT('Ctrl Pts',(-45.4714029967,-55.8067071952963,-51.8916166666667));
#261468=CARTESIAN_POINT('Ctrl Pts',(-45.9531282658897,-56.6410798368225,
-51.8332833333334));
#261469=CARTESIAN_POINT('Ctrl Pts',(-46.4348535350793,-57.4754524783487,
-51.77495));
#261470=CARTESIAN_POINT('Ctrl Pts',(-45.9531282658897,-58.309825119875,
-51.7166166666667));
#261471=CARTESIAN_POINT('Ctrl Pts',(-45.4714029967,-59.1441977614012,-51.6582833333333));
#261472=CARTESIAN_POINT('Ctrl Pts',(-44.5079524583208,-59.1441977614012,
-51.59995));
#261473=CARTESIAN_POINT('Ctrl Pts',(-43.5445019199415,-59.1441977614012,
-51.5416166666667));
#261474=CARTESIAN_POINT('Ctrl Pts',(-43.0627766507519,-58.309825119875,
-51.4832833333334));
#261475=CARTESIAN_POINT('Ctrl Pts',(-42.5810513815623,-57.4754524783487,
-51.42495));
#261476=CARTESIAN_POINT('Ctrl Pts',(-43.0627766507519,-56.6410798368225,
-51.3666166666667));
#261477=CARTESIAN_POINT('Ctrl Pts',(-43.5445019199415,-55.8067071952963,
-51.3082833333333));
#261478=CARTESIAN_POINT('Ctrl Pts',(-44.5079524583208,-55.8067071952963,
-51.24995));
#261479=CARTESIAN_POINT('Ctrl Pts',(-45.4714029967,-55.8067071952963,-51.1916166666667));
#261480=CARTESIAN_POINT('Ctrl Pts',(-45.9531282658897,-56.6410798368225,
-51.1332833333334));
#261481=CARTESIAN_POINT('Ctrl Pts',(-46.4348535350793,-57.4754524783487,
-51.07495));
#261482=CARTESIAN_POINT('Ctrl Pts',(-45.9531282658897,-58.309825119875,
-51.0166166666667));
#261483=CARTESIAN_POINT('Ctrl Pts',(-45.4714029967,-59.1441977614012,-50.9582833333334));
#261484=CARTESIAN_POINT('Ctrl Pts',(-44.5079524583208,-59.1441977614012,
-50.89995));
#261485=CARTESIAN_POINT('Ctrl Pts',(-43.5445019199415,-59.1441977614012,
-50.8416166666667));
#261486=CARTESIAN_POINT('Ctrl Pts',(-43.0627766507519,-58.309825119875,
-50.7832833333333));
#261487=CARTESIAN_POINT('Ctrl Pts',(-42.5810513815623,-57.4754524783487,
-50.72495));
#261488=CARTESIAN_POINT('Ctrl Pts',(-43.0627766507519,-56.6410798368225,
-50.6666166666667));
#261489=CARTESIAN_POINT('Ctrl Pts',(-43.5445019199415,-55.8067071952963,
-50.6082833333334));
#261490=CARTESIAN_POINT('Ctrl Pts',(-44.5079524583208,-55.8067071952963,
-50.54995));
#261491=CARTESIAN_POINT('Ctrl Pts',(-45.4714029967,-55.8067071952963,-50.4916166666667));
#261492=CARTESIAN_POINT('Ctrl Pts',(-45.9531282658897,-56.6410798368225,
-50.4332833333333));
#261493=CARTESIAN_POINT('Ctrl Pts',(-46.4348535350793,-57.4754524783487,
-50.37495));
#261494=CARTESIAN_POINT('Ctrl Pts',(-45.9531282658897,-58.309825119875,
-50.3166166666667));
#261495=CARTESIAN_POINT('Ctrl Pts',(-45.4714029967,-59.1441977614012,-50.2582833333334));
#261496=CARTESIAN_POINT('Ctrl Pts',(-44.5079524583208,-59.1441977614012,
-50.19995));
#261497=CARTESIAN_POINT('Ctrl Pts',(-43.5445019199415,-59.1441977614012,
-50.1416166666667));
#261498=CARTESIAN_POINT('Ctrl Pts',(-43.0627766507519,-58.309825119875,
-50.0832833333334));
#261499=CARTESIAN_POINT('Ctrl Pts',(-42.5810513815623,-57.4754524783487,
-50.02495));
#261500=CARTESIAN_POINT('Ctrl Pts',(-43.0627766507519,-56.6410798368225,
-49.9666166666667));
#261501=CARTESIAN_POINT('Ctrl Pts',(-43.5445019199415,-55.8067071952963,
-49.9082833333334));
#261502=CARTESIAN_POINT('Ctrl Pts',(-44.5079524583208,-55.8067071952963,
-49.84995));
#261503=CARTESIAN_POINT('Ctrl Pts',(-45.4714029967,-55.8067071952963,-49.7916166666667));
#261504=CARTESIAN_POINT('Ctrl Pts',(-45.9531282658897,-56.6410798368225,
-49.7332833333334));
#261505=CARTESIAN_POINT('Ctrl Pts',(-46.4348535350793,-57.4754524783487,
-49.67495));
#261506=CARTESIAN_POINT('Ctrl Pts',(-45.9531282658897,-58.309825119875,
-49.6166166666667));
#261507=CARTESIAN_POINT('Ctrl Pts',(-45.4714029967,-59.1441977614012,-49.5582833333334));
#261508=CARTESIAN_POINT('Ctrl Pts',(-44.5079524583208,-59.1441977614012,
-49.49995));
#261509=CARTESIAN_POINT('Ctrl Pts',(-43.5445019199415,-59.1441977614012,
-49.4416166666667));
#261510=CARTESIAN_POINT('Ctrl Pts',(-43.0627766507519,-58.309825119875,
-49.3832833333334));
#261511=CARTESIAN_POINT('Ctrl Pts',(-42.5810513815623,-57.4754524783487,
-49.32495));
#261512=CARTESIAN_POINT('Ctrl Pts',(-43.0627766507519,-56.6410798368225,
-49.2666166666667));
#261513=CARTESIAN_POINT('Ctrl Pts',(-43.5445019199415,-55.8067071952963,
-49.2082833333334));
#261514=CARTESIAN_POINT('Ctrl Pts',(-44.5079524583208,-55.8067071952963,
-49.14995));
#261515=CARTESIAN_POINT('Ctrl Pts',(-45.4714029967,-55.8067071952963,-49.0916166666667));
#261516=CARTESIAN_POINT('Ctrl Pts',(-45.9531282658897,-56.6410798368225,
-49.0332833333333));
#261517=CARTESIAN_POINT('Ctrl Pts',(-46.4348535350793,-57.4754524783487,
-48.97495));
#261518=CARTESIAN_POINT('Ctrl Pts',(-45.9531282658897,-58.309825119875,
-48.9166166666667));
#261519=CARTESIAN_POINT('Ctrl Pts',(-45.4714029967,-59.1441977614012,-48.8582833333333));
#261520=CARTESIAN_POINT('Ctrl Pts',(-44.5079524583208,-59.1441977614012,
-48.79995));
#261521=CARTESIAN_POINT('Ctrl Pts',(-43.5445019199415,-59.1441977614012,
-48.7416166666667));
#261522=CARTESIAN_POINT('Ctrl Pts',(-43.0627766507519,-58.309825119875,
-48.6832833333334));
#261523=CARTESIAN_POINT('Ctrl Pts',(-42.5810513815623,-57.4754524783487,
-48.62495));
#261524=CARTESIAN_POINT('Ctrl Pts',(-43.0627766507519,-56.6410798368225,
-48.5666166666667));
#261525=CARTESIAN_POINT('Ctrl Pts',(-43.5445019199415,-55.8067071952963,
-48.5082833333334));
#261526=CARTESIAN_POINT('Ctrl Pts',(-44.5079524583208,-55.8067071952963,
-48.44995));
#261527=CARTESIAN_POINT('Ctrl Pts',(-45.4714029967,-55.8067071952963,-48.3916166666667));
#261528=CARTESIAN_POINT('Ctrl Pts',(-45.9531282658897,-56.6410798368225,
-48.3332833333334));
#261529=CARTESIAN_POINT('Ctrl Pts',(-46.4348535350793,-57.4754524783487,
-48.27495));
#261530=CARTESIAN_POINT('Ctrl Pts',(-45.9531282658897,-58.309825119875,
-48.2166166666667));
#261531=CARTESIAN_POINT('Ctrl Pts',(-45.4714029967,-59.1441977614012,-48.1582833333334));
#261532=CARTESIAN_POINT('Ctrl Pts',(-44.5079524583208,-59.1441977614012,
-48.09995));
#261533=CARTESIAN_POINT('Ctrl Pts',(-43.5445019199415,-59.1441977614012,
-48.0416166666667));
#261534=CARTESIAN_POINT('Ctrl Pts',(-43.0627766507519,-58.309825119875,
-47.9832833333334));
#261535=CARTESIAN_POINT('Ctrl Pts',(-42.5810513815623,-57.4754524783487,
-47.92495));
#261536=CARTESIAN_POINT('Ctrl Pts',(-43.0627766507519,-56.6410798368225,
-47.8666166666667));
#261537=CARTESIAN_POINT('Ctrl Pts',(-43.5445019199415,-55.8067071952963,
-47.8082833333333));
#261538=CARTESIAN_POINT('Ctrl Pts',(-44.5079524583208,-55.8067071952963,
-47.74995));
#261539=CARTESIAN_POINT('Ctrl Pts',(-45.4714029967,-55.8067071952963,-47.6916166666667));
#261540=CARTESIAN_POINT('Ctrl Pts',(-45.9531282658897,-56.6410798368225,
-47.6332833333333));
#261541=CARTESIAN_POINT('Ctrl Pts',(-46.4348535350793,-57.4754524783487,
-47.57495));
#261542=CARTESIAN_POINT('Ctrl Pts',(-45.9531282658897,-58.309825119875,
-47.5166166666667));
#261543=CARTESIAN_POINT('Ctrl Pts',(-45.4714029967,-59.1441977614012,-47.4582833333333));
#261544=CARTESIAN_POINT('Ctrl Pts',(-44.5079524583208,-59.1441977614012,
-47.39995));
#261545=CARTESIAN_POINT('Ctrl Pts',(-43.5445019199415,-59.1441977614012,
-47.3416166666666));
#261546=CARTESIAN_POINT('Ctrl Pts',(-43.0627766507519,-58.309825119875,
-47.2832833333333));
#261547=CARTESIAN_POINT('Ctrl Pts',(-42.5810513815623,-57.4754524783487,
-47.22495));
#261548=CARTESIAN_POINT('Ctrl Pts',(-43.0627766507519,-56.6410798368225,
-47.1666166666667));
#261549=CARTESIAN_POINT('Ctrl Pts',(-43.5445019199415,-55.8067071952963,
-47.1082833333333));
#261550=CARTESIAN_POINT('Ctrl Pts',(-44.5079524583208,-55.8067071952963,
-47.04995));
#261551=CARTESIAN_POINT('Ctrl Pts',(-45.4714029967,-55.8067071952963,-46.9916166666667));
#261552=CARTESIAN_POINT('Ctrl Pts',(-45.9531282658897,-56.6410798368225,
-46.9332833333334));
#261553=CARTESIAN_POINT('Ctrl Pts',(-46.4348535350793,-57.4754524783487,
-46.87495));
#261554=CARTESIAN_POINT('Ctrl Pts',(-45.9531282658897,-58.309825119875,
-46.8166166666667));
#261555=CARTESIAN_POINT('Ctrl Pts',(-45.4714029967,-59.1441977614012,-46.7582833333333));
#261556=CARTESIAN_POINT('Ctrl Pts',(-44.5079524583208,-59.1441977614012,
-46.69995));
#261557=CARTESIAN_POINT('Ctrl Pts',(-43.5445019199415,-59.1441977614012,
-46.6416166666666));
#261558=CARTESIAN_POINT('Ctrl Pts',(-43.0627766507519,-58.309825119875,
-46.5832833333334));
#261559=CARTESIAN_POINT('Ctrl Pts',(-42.5810513815623,-57.4754524783487,
-46.52495));
#261560=CARTESIAN_POINT('Ctrl Pts',(-43.0627766507519,-56.6410798368225,
-46.4666166666667));
#261561=CARTESIAN_POINT('Ctrl Pts',(-43.5445019199415,-55.8067071952963,
-46.4082833333333));
#261562=CARTESIAN_POINT('Ctrl Pts',(-44.5079524583208,-55.8067071952963,
-46.34995));
#261563=CARTESIAN_POINT('Ctrl Pts',(-45.4714029967,-55.8067071952963,-46.2916166666667));
#261564=CARTESIAN_POINT('Ctrl Pts',(-45.9531282658897,-56.6410798368225,
-46.2332833333334));
#261565=CARTESIAN_POINT('Ctrl Pts',(-46.4348535350793,-57.4754524783487,
-46.17495));
#261566=CARTESIAN_POINT('Ctrl Pts',(-45.9531282658897,-58.309825119875,
-46.1166166666667));
#261567=CARTESIAN_POINT('Ctrl Pts',(-45.4714029967,-59.1441977614012,-46.0582833333333));
#261568=CARTESIAN_POINT('Ctrl Pts',(-44.5079524583208,-59.1441977614012,
-45.99995));
#261569=CARTESIAN_POINT('Ctrl Pts',(-43.5445019199415,-59.1441977614012,
-45.9416166666667));
#261570=CARTESIAN_POINT('Ctrl Pts',(-43.0627766507519,-58.309825119875,
-45.8832833333333));
#261571=CARTESIAN_POINT('Ctrl Pts',(-42.5810513815623,-57.4754524783487,
-45.82495));
#261572=CARTESIAN_POINT('Ctrl Pts',(-43.0627766507519,-56.6410798368225,
-45.7666166666667));
#261573=CARTESIAN_POINT('Ctrl Pts',(-43.5445019199415,-55.8067071952963,
-45.7082833333333));
#261574=CARTESIAN_POINT('Ctrl Pts',(-44.5079524583208,-55.8067071952963,
-45.64995));
#261575=CARTESIAN_POINT('Ctrl Pts',(-45.4714029967,-55.8067071952963,-45.5916166666667));
#261576=CARTESIAN_POINT('Ctrl Pts',(-45.9531282658897,-56.6410798368225,
-45.5332833333333));
#261577=CARTESIAN_POINT('Ctrl Pts',(-46.4348535350793,-57.4754524783487,
-45.47495));
#261578=CARTESIAN_POINT('Ctrl Pts',(-45.9531282658897,-58.309825119875,
-45.4166166666667));
#261579=CARTESIAN_POINT('Ctrl Pts',(-45.4714029967,-59.1441977614012,-45.3582833333333));
#261580=CARTESIAN_POINT('Ctrl Pts',(-44.5079524583208,-59.1441977614012,
-45.29995));
#261581=CARTESIAN_POINT('Ctrl Pts',(-43.5445019199415,-59.1441977614012,
-45.2416166666667));
#261582=CARTESIAN_POINT('Ctrl Pts',(-43.0627766507519,-58.309825119875,
-45.1832833333334));
#261583=CARTESIAN_POINT('Ctrl Pts',(-42.5810513815623,-57.4754524783487,
-45.12495));
#261584=CARTESIAN_POINT('Ctrl Pts',(-43.0627766507519,-56.6410798368225,
-45.0666166666667));
#261585=CARTESIAN_POINT('Ctrl Pts',(-43.5445019199415,-55.8067071952963,
-45.0082833333334));
#261586=CARTESIAN_POINT('Ctrl Pts',(-44.5079524583208,-55.8067071952963,
-44.94995));
#261587=CARTESIAN_POINT('Ctrl Pts',(-45.4714029967,-55.8067071952963,-44.8916166666667));
#261588=CARTESIAN_POINT('Ctrl Pts',(-45.9531282658897,-56.6410798368225,
-44.8332833333334));
#261589=CARTESIAN_POINT('Ctrl Pts',(-46.4348535350793,-57.4754524783487,
-44.77495));
#261590=CARTESIAN_POINT('Ctrl Pts',(-45.9531282658897,-58.309825119875,
-44.7166166666667));
#261591=CARTESIAN_POINT('Ctrl Pts',(-45.4714029967,-59.1441977614012,-44.6582833333334));
#261592=CARTESIAN_POINT('Ctrl Pts',(-44.5079524583208,-59.1441977614012,
-44.59995));
#261593=CARTESIAN_POINT('Ctrl Pts',(-43.5445019199415,-59.1441977614012,
-44.5416166666667));
#261594=CARTESIAN_POINT('Ctrl Pts',(-43.0627766507519,-58.309825119875,
-44.4832833333334));
#261595=CARTESIAN_POINT('Ctrl Pts',(-42.5810513815623,-57.4754524783487,
-44.42495));
#261596=CARTESIAN_POINT('Ctrl Pts',(-43.0627766507519,-56.6410798368225,
-44.3666166666667));
#261597=CARTESIAN_POINT('Ctrl Pts',(-43.5445019199415,-55.8067071952963,
-44.3082833333334));
#261598=CARTESIAN_POINT('Ctrl Pts',(-44.5079524583208,-55.8067071952963,
-44.24995));
#261599=CARTESIAN_POINT('Ctrl Pts',(-45.4714029967,-55.8067071952963,-44.1916166666667));
#261600=CARTESIAN_POINT('Ctrl Pts',(-45.9531282658897,-56.6410798368225,
-44.1332833333334));
#261601=CARTESIAN_POINT('Ctrl Pts',(-46.4348535350793,-57.4754524783487,
-44.07495));
#261602=CARTESIAN_POINT('Ctrl Pts',(-45.9531282658897,-58.309825119875,
-44.0166166666667));
#261603=CARTESIAN_POINT('Ctrl Pts',(-45.4714029967,-59.1441977614012,-43.9582833333334));
#261604=CARTESIAN_POINT('Ctrl Pts',(-44.5079524583208,-59.1441977614012,
-43.89995));
#261605=CARTESIAN_POINT('Ctrl Pts',(-43.5445019199415,-59.1441977614012,
-43.8416166666667));
#261606=CARTESIAN_POINT('Ctrl Pts',(-43.0627766507519,-58.309825119875,
-43.7832833333334));
#261607=CARTESIAN_POINT('Ctrl Pts',(-42.5810513815623,-57.4754524783487,
-43.72495));
#261608=CARTESIAN_POINT('Ctrl Pts',(-43.0627766507519,-56.6410798368225,
-43.6666166666667));
#261609=CARTESIAN_POINT('Ctrl Pts',(-43.5445019199415,-55.8067071952963,
-43.6082833333333));
#261610=CARTESIAN_POINT('Ctrl Pts',(-44.5079524583208,-55.8067071952963,
-43.54995));
#261611=CARTESIAN_POINT('Ctrl Pts',(-45.4714029967,-55.8067071952963,-43.4916166666667));
#261612=CARTESIAN_POINT('Ctrl Pts',(-45.9531282658897,-56.6410798368225,
-43.4332833333333));
#261613=CARTESIAN_POINT('Ctrl Pts',(-46.4348535350793,-57.4754524783487,
-43.37495));
#261614=CARTESIAN_POINT('Ctrl Pts',(-45.9531282658897,-58.309825119875,
-43.3166166666667));
#261615=CARTESIAN_POINT('Ctrl Pts',(-45.4714029967,-59.1441977614012,-43.2582833333333));
#261616=CARTESIAN_POINT('Ctrl Pts',(-44.5079524583208,-59.1441977614012,
-43.19995));
#261617=CARTESIAN_POINT('Ctrl Pts',(-43.5445019199415,-59.1441977614012,
-43.1416166666667));
#261618=CARTESIAN_POINT('Ctrl Pts',(-43.0627766507519,-58.309825119875,
-43.0832833333333));
#261619=CARTESIAN_POINT('Ctrl Pts',(-42.5810513815623,-57.4754524783487,
-43.02495));
#261620=CARTESIAN_POINT('Ctrl Pts',(-43.0627766507519,-56.6410798368225,
-42.9666166666667));
#261621=CARTESIAN_POINT('Ctrl Pts',(-43.5445019199415,-55.8067071952963,
-42.9082833333333));
#261622=CARTESIAN_POINT('Ctrl Pts',(-44.5079524583208,-55.8067071952963,
-42.84995));
#261623=CARTESIAN_POINT('Ctrl Pts',(-45.4714029967,-55.8067071952963,-42.7916166666667));
#261624=CARTESIAN_POINT('Ctrl Pts',(-45.9531282658897,-56.6410798368225,
-42.7332833333334));
#261625=CARTESIAN_POINT('Ctrl Pts',(-46.4348535350793,-57.4754524783487,
-42.67495));
#261626=CARTESIAN_POINT('Ctrl Pts',(-45.9531282658897,-58.309825119875,
-42.6166166666667));
#261627=CARTESIAN_POINT('Ctrl Pts',(-45.4714029967,-59.1441977614012,-42.5582833333333));
#261628=CARTESIAN_POINT('Ctrl Pts',(-44.5079524583208,-59.1441977614012,
-42.49995));
#261629=CARTESIAN_POINT('Ctrl Pts',(-43.5445019199415,-59.1441977614012,
-42.4416166666667));
#261630=CARTESIAN_POINT('Ctrl Pts',(-43.0627766507519,-58.309825119875,
-42.3832833333333));
#261631=CARTESIAN_POINT('Ctrl Pts',(-42.5810513815623,-57.4754524783487,
-42.32495));
#261632=CARTESIAN_POINT('Ctrl Pts',(-43.0627766507519,-56.6410798368225,
-42.2666166666667));
#261633=CARTESIAN_POINT('Ctrl Pts',(-43.5445019199415,-55.8067071952963,
-42.2082833333333));
#261634=CARTESIAN_POINT('Ctrl Pts',(-44.5079524583208,-55.8067071952963,
-42.14995));
#261635=CARTESIAN_POINT('Ctrl Pts',(-45.4714029967,-55.8067071952963,-42.0916166666667));
#261636=CARTESIAN_POINT('Ctrl Pts',(-45.9531282658897,-56.6410798368225,
-42.0332833333334));
#261637=CARTESIAN_POINT('Ctrl Pts',(-46.4348535350793,-57.4754524783487,
-41.97495));
#261638=CARTESIAN_POINT('Ctrl Pts',(-45.9531282658897,-58.309825119875,
-41.9166166666667));
#261639=CARTESIAN_POINT('Ctrl Pts',(-45.4714029967,-59.1441977614012,-41.8582833333333));
#261640=CARTESIAN_POINT('Ctrl Pts',(-44.5079524583208,-59.1441977614012,
-41.79995));
#261641=CARTESIAN_POINT('Ctrl Pts',(-43.5445019199415,-59.1441977614012,
-41.7416166666667));
#261642=CARTESIAN_POINT('Ctrl Pts',(-43.0627766507519,-58.309825119875,
-41.6832833333333));
#261643=CARTESIAN_POINT('Ctrl Pts',(-42.5810513815623,-57.4754524783487,
-41.62495));
#261644=CARTESIAN_POINT('Ctrl Pts',(-43.0627766507519,-56.6410798368225,
-41.5666166666667));
#261645=CARTESIAN_POINT('Ctrl Pts',(-43.5445019199415,-55.8067071952963,
-41.5082833333334));
#261646=CARTESIAN_POINT('Ctrl Pts',(-44.5079524583208,-55.8067071952963,
-41.44995));
#261647=CARTESIAN_POINT('Ctrl Pts',(-45.4714029967,-55.8067071952963,-41.3916166666667));
#261648=CARTESIAN_POINT('Ctrl Pts',(-45.9531282658897,-56.6410798368225,
-41.3332833333334));
#261649=CARTESIAN_POINT('Ctrl Pts',(-46.4348535350793,-57.4754524783487,
-41.27495));
#261650=CARTESIAN_POINT('Ctrl Pts',(-45.9531282658897,-58.309825119875,
-41.2166166666667));
#261651=CARTESIAN_POINT('Ctrl Pts',(-45.4714029967,-59.1441977614012,-41.1582833333333));
#261652=CARTESIAN_POINT('Ctrl Pts',(-44.5079524583208,-59.1441977614012,
-41.09995));
#261653=CARTESIAN_POINT('Ctrl Pts',(-43.5445019199415,-59.1441977614012,
-41.0416166666667));
#261654=CARTESIAN_POINT('Ctrl Pts',(-43.0627766507519,-58.309825119875,
-40.9832833333333));
#261655=CARTESIAN_POINT('Ctrl Pts',(-42.5810513815623,-57.4754524783487,
-40.92495));
#261656=CARTESIAN_POINT('Ctrl Pts',(-43.0627766507519,-56.6410798368225,
-40.8666166666667));
#261657=CARTESIAN_POINT('Ctrl Pts',(-43.5445019199415,-55.8067071952963,
-40.8082833333334));
#261658=CARTESIAN_POINT('Ctrl Pts',(-44.5079524583208,-55.8067071952963,
-40.74995));
#261659=CARTESIAN_POINT('Ctrl Pts',(-45.4714029967,-55.8067071952963,-40.6916166666667));
#261660=CARTESIAN_POINT('Ctrl Pts',(-45.9531282658897,-56.6410798368225,
-40.6332833333334));
#261661=CARTESIAN_POINT('Ctrl Pts',(-46.4348535350793,-57.4754524783487,
-40.57495));
#261662=CARTESIAN_POINT('Ctrl Pts',(-45.9531282658897,-58.309825119875,
-40.5166166666667));
#261663=CARTESIAN_POINT('Ctrl Pts',(-45.4714029967,-59.1441977614012,-40.4582833333333));
#261664=CARTESIAN_POINT('Ctrl Pts',(-44.5079524583208,-59.1441977614012,
-40.39995));
#261665=CARTESIAN_POINT('Ctrl Pts',(-43.5445019199415,-59.1441977614012,
-40.3416166666667));
#261666=CARTESIAN_POINT('Ctrl Pts',(-43.0627766507519,-58.309825119875,
-40.2832833333334));
#261667=CARTESIAN_POINT('Ctrl Pts',(-42.5810513815623,-57.4754524783487,
-40.22495));
#261668=CARTESIAN_POINT('Ctrl Pts',(-43.0627766507519,-56.6410798368225,
-40.1666166666667));
#261669=CARTESIAN_POINT('Ctrl Pts',(-43.5445019199415,-55.8067071952963,
-40.1082833333334));
#261670=CARTESIAN_POINT('Ctrl Pts',(-44.5079524583208,-55.8067071952963,
-40.04995));
#261671=CARTESIAN_POINT('Ctrl Pts',(-45.4714029967,-55.8067071952963,-39.9916166666667));
#261672=CARTESIAN_POINT('Ctrl Pts',(-45.9531282658897,-56.6410798368225,
-39.9332833333333));
#261673=CARTESIAN_POINT('Ctrl Pts',(-46.4348535350793,-57.4754524783487,
-39.87495));
#261674=CARTESIAN_POINT('Ctrl Pts',(-45.9531282658897,-58.309825119875,
-39.8166166666667));
#261675=CARTESIAN_POINT('Ctrl Pts',(-45.4714029967,-59.1441977614012,-39.7582833333334));
#261676=CARTESIAN_POINT('Ctrl Pts',(-44.5079524583208,-59.1441977614012,
-39.69995));
#261677=CARTESIAN_POINT('Ctrl Pts',(-43.5445019199415,-59.1441977614012,
-39.6416166666667));
#261678=CARTESIAN_POINT('Ctrl Pts',(-43.0627766507519,-58.309825119875,
-39.5832833333333));
#261679=CARTESIAN_POINT('Ctrl Pts',(-42.5810513815623,-57.4754524783487,
-39.52495));
#261680=CARTESIAN_POINT('Ctrl Pts',(-43.0627766507519,-56.6410798368225,
-39.4666166666667));
#261681=CARTESIAN_POINT('Ctrl Pts',(-43.5445019199415,-55.8067071952963,
-39.4082833333334));
#261682=CARTESIAN_POINT('Ctrl Pts',(-44.5079524583208,-55.8067071952963,
-39.34995));
#261683=CARTESIAN_POINT('Ctrl Pts',(-45.4714029967,-55.8067071952963,-39.2916166666667));
#261684=CARTESIAN_POINT('Ctrl Pts',(-45.9531282658897,-56.6410798368225,
-39.2332833333333));
#261685=CARTESIAN_POINT('Ctrl Pts',(-46.4348535350793,-57.4754524783487,
-39.17495));
#261686=CARTESIAN_POINT('Ctrl Pts',(-45.9531282658897,-58.309825119875,
-39.1166166666667));
#261687=CARTESIAN_POINT('Ctrl Pts',(-45.4714029967,-59.1441977614012,-39.0582833333334));
#261688=CARTESIAN_POINT('Ctrl Pts',(-44.5079524583208,-59.1441977614012,
-38.99995));
#261689=CARTESIAN_POINT('Ctrl Pts',(-43.5445019199415,-59.1441977614012,
-38.9416166666667));
#261690=CARTESIAN_POINT('Ctrl Pts',(-43.0627766507519,-58.309825119875,
-38.8832833333334));
#261691=CARTESIAN_POINT('Ctrl Pts',(-42.5810513815623,-57.4754524783487,
-38.82495));
#261692=CARTESIAN_POINT('Ctrl Pts',(-43.0627766507519,-56.6410798368225,
-38.7666166666667));
#261693=CARTESIAN_POINT('Ctrl Pts',(-43.5445019199415,-55.8067071952963,
-38.7082833333334));
#261694=CARTESIAN_POINT('Ctrl Pts',(-44.5079524583208,-55.8067071952963,
-38.64995));
#261695=CARTESIAN_POINT('Ctrl Pts',(-45.4714029967,-55.8067071952963,-38.5916166666667));
#261696=CARTESIAN_POINT('Ctrl Pts',(-45.9531282658897,-56.6410798368225,
-38.5332833333334));
#261697=CARTESIAN_POINT('Ctrl Pts',(-46.4348535350793,-57.4754524783487,
-38.47495));
#261698=CARTESIAN_POINT('Ctrl Pts',(-45.9531282658897,-58.309825119875,
-38.4166166666667));
#261699=CARTESIAN_POINT('Ctrl Pts',(-45.4714029967,-59.1441977614012,-38.3582833333333));
#261700=CARTESIAN_POINT('Ctrl Pts',(-44.5079524583208,-59.1441977614012,
-38.29995));
#261701=CARTESIAN_POINT('Ctrl Pts',(-43.5445019199415,-59.1441977614012,
-38.2416166666667));
#261702=CARTESIAN_POINT('Ctrl Pts',(-43.0627766507519,-58.309825119875,
-38.1832833333333));
#261703=CARTESIAN_POINT('Ctrl Pts',(-42.5810513815623,-57.4754524783487,
-38.12495));
#261704=CARTESIAN_POINT('Ctrl Pts',(-43.0627766507519,-56.6410798368225,
-38.0666166666667));
#261705=CARTESIAN_POINT('Ctrl Pts',(-43.5445019199415,-55.8067071952963,
-38.0082833333333));
#261706=CARTESIAN_POINT('Ctrl Pts',(-44.5079524583208,-55.8067071952963,
-37.94995));
#261707=CARTESIAN_POINT('Ctrl Pts',(-45.4714029967,-55.8067071952963,-37.8916166666667));
#261708=CARTESIAN_POINT('Ctrl Pts',(-45.9531282658897,-56.6410798368225,
-37.8332833333334));
#261709=CARTESIAN_POINT('Ctrl Pts',(-46.4348535350793,-57.4754524783487,
-37.77495));
#261710=CARTESIAN_POINT('Ctrl Pts',(-45.9531282658897,-58.309825119875,
-37.7166166666667));
#261711=CARTESIAN_POINT('Ctrl Pts',(-45.4714029967,-59.1441977614012,-37.6582833333333));
#261712=CARTESIAN_POINT('Ctrl Pts',(-44.5079524583208,-59.1441977614012,
-37.59995));
#261713=CARTESIAN_POINT('Ctrl Pts',(-43.5445019199415,-59.1441977614012,
-37.5416166666667));
#261714=CARTESIAN_POINT('Ctrl Pts',(-43.0627766507519,-58.309825119875,
-37.4832833333334));
#261715=CARTESIAN_POINT('Ctrl Pts',(-42.5810513815623,-57.4754524783487,
-37.42495));
#261716=CARTESIAN_POINT('Ctrl Pts',(-43.0627766507519,-56.6410798368225,
-37.3666166666667));
#261717=CARTESIAN_POINT('Ctrl Pts',(-43.5445019199415,-55.8067071952963,
-37.3082833333333));
#261718=CARTESIAN_POINT('Ctrl Pts',(-44.5079524583208,-55.8067071952963,
-37.24995));
#261719=CARTESIAN_POINT('Ctrl Pts',(-45.4714029967,-55.8067071952963,-37.1916166666667));
#261720=CARTESIAN_POINT('Ctrl Pts',(-45.9531282658897,-56.6410798368225,
-37.1332833333334));
#261721=CARTESIAN_POINT('Ctrl Pts',(-46.4348535350793,-57.4754524783487,
-37.07495));
#261722=CARTESIAN_POINT('Ctrl Pts',(-45.9531282658897,-58.309825119875,
-37.0166166666667));
#261723=CARTESIAN_POINT('Ctrl Pts',(-45.8905850977848,-58.418153064699,
-37.0090431559831));
#261724=CARTESIAN_POINT('Ctrl Pts',(-45.8125914103809,-58.5159466035015,
-37.0009024189827));
#261725=CARTESIAN_POINT('Ctrl Pts',(-44.5079524583208,-59.5441932447742,
-53.2308875));
#261726=CARTESIAN_POINT('Ctrl Pts',(-43.3135644199415,-59.5441932447742,
-53.1725541666667));
#261727=CARTESIAN_POINT('Ctrl Pts',(-42.7163704007519,-58.5098228615615,
-53.1142208333334));
#261728=CARTESIAN_POINT('Ctrl Pts',(-42.1191763815623,-57.4754524783487,
-53.0558875000001));
#261729=CARTESIAN_POINT('Ctrl Pts',(-42.7163704007519,-56.4410820951361,
-52.9975541666667));
#261730=CARTESIAN_POINT('Ctrl Pts',(-43.3135644199415,-55.4067117119233,
-52.9392208333334));
#261731=CARTESIAN_POINT('Ctrl Pts',(-44.5079524583208,-55.4067117119234,
-52.8808875));
#261732=CARTESIAN_POINT('Ctrl Pts',(-45.7023404967,-55.4067117119233,-52.8225541666667));
#261733=CARTESIAN_POINT('Ctrl Pts',(-46.2995345158897,-56.4410820951361,
-52.7642208333334));
#261734=CARTESIAN_POINT('Ctrl Pts',(-46.8967285350793,-57.4754524783487,
-52.7058875));
#261735=CARTESIAN_POINT('Ctrl Pts',(-46.2995345158897,-58.5098228615615,
-52.6475541666667));
#261736=CARTESIAN_POINT('Ctrl Pts',(-45.7023404967,-59.5441932447742,-52.5892208333333));
#261737=CARTESIAN_POINT('Ctrl Pts',(-44.5079524583208,-59.5441932447742,
-52.5308875));
#261738=CARTESIAN_POINT('Ctrl Pts',(-43.3135644199415,-59.5441932447742,
-52.4725541666667));
#261739=CARTESIAN_POINT('Ctrl Pts',(-42.7163704007519,-58.5098228615615,
-52.4142208333334));
#261740=CARTESIAN_POINT('Ctrl Pts',(-42.1191763815623,-57.4754524783487,
-52.3558875000001));
#261741=CARTESIAN_POINT('Ctrl Pts',(-42.7163704007519,-56.4410820951361,
-52.2975541666667));
#261742=CARTESIAN_POINT('Ctrl Pts',(-43.3135644199415,-55.4067117119233,
-52.2392208333334));
#261743=CARTESIAN_POINT('Ctrl Pts',(-44.5079524583208,-55.4067117119234,
-52.1808875));
#261744=CARTESIAN_POINT('Ctrl Pts',(-45.7023404967,-55.4067117119233,-52.1225541666667));
#261745=CARTESIAN_POINT('Ctrl Pts',(-46.2995345158897,-56.4410820951361,
-52.0642208333334));
#261746=CARTESIAN_POINT('Ctrl Pts',(-46.8967285350793,-57.4754524783487,
-52.0058875));
#261747=CARTESIAN_POINT('Ctrl Pts',(-46.2995345158897,-58.5098228615615,
-51.9475541666667));
#261748=CARTESIAN_POINT('Ctrl Pts',(-45.7023404967,-59.5441932447742,-51.8892208333334));
#261749=CARTESIAN_POINT('Ctrl Pts',(-44.5079524583208,-59.5441932447742,
-51.8308875));
#261750=CARTESIAN_POINT('Ctrl Pts',(-43.3135644199415,-59.5441932447742,
-51.7725541666667));
#261751=CARTESIAN_POINT('Ctrl Pts',(-42.7163704007519,-58.5098228615615,
-51.7142208333334));
#261752=CARTESIAN_POINT('Ctrl Pts',(-42.1191763815623,-57.4754524783487,
-51.6558875));
#261753=CARTESIAN_POINT('Ctrl Pts',(-42.7163704007519,-56.4410820951361,
-51.5975541666667));
#261754=CARTESIAN_POINT('Ctrl Pts',(-43.3135644199415,-55.4067117119233,
-51.5392208333333));
#261755=CARTESIAN_POINT('Ctrl Pts',(-44.5079524583208,-55.4067117119234,
-51.4808875));
#261756=CARTESIAN_POINT('Ctrl Pts',(-45.7023404967,-55.4067117119233,-51.4225541666667));
#261757=CARTESIAN_POINT('Ctrl Pts',(-46.2995345158897,-56.4410820951361,
-51.3642208333334));
#261758=CARTESIAN_POINT('Ctrl Pts',(-46.8967285350793,-57.4754524783487,
-51.3058875));
#261759=CARTESIAN_POINT('Ctrl Pts',(-46.2995345158897,-58.5098228615615,
-51.2475541666667));
#261760=CARTESIAN_POINT('Ctrl Pts',(-45.7023404967,-59.5441932447742,-51.1892208333334));
#261761=CARTESIAN_POINT('Ctrl Pts',(-44.5079524583208,-59.5441932447742,
-51.1308875));
#261762=CARTESIAN_POINT('Ctrl Pts',(-43.3135644199415,-59.5441932447742,
-51.0725541666667));
#261763=CARTESIAN_POINT('Ctrl Pts',(-42.7163704007519,-58.5098228615615,
-51.0142208333334));
#261764=CARTESIAN_POINT('Ctrl Pts',(-42.1191763815623,-57.4754524783487,
-50.9558875));
#261765=CARTESIAN_POINT('Ctrl Pts',(-42.7163704007519,-56.4410820951361,
-50.8975541666667));
#261766=CARTESIAN_POINT('Ctrl Pts',(-43.3135644199415,-55.4067117119233,
-50.8392208333333));
#261767=CARTESIAN_POINT('Ctrl Pts',(-44.5079524583208,-55.4067117119234,
-50.7808875));
#261768=CARTESIAN_POINT('Ctrl Pts',(-45.7023404967,-55.4067117119233,-50.7225541666667));
#261769=CARTESIAN_POINT('Ctrl Pts',(-46.2995345158897,-56.4410820951361,
-50.6642208333333));
#261770=CARTESIAN_POINT('Ctrl Pts',(-46.8967285350793,-57.4754524783487,
-50.6058875));
#261771=CARTESIAN_POINT('Ctrl Pts',(-46.2995345158897,-58.5098228615615,
-50.5475541666667));
#261772=CARTESIAN_POINT('Ctrl Pts',(-45.7023404967,-59.5441932447742,-50.4892208333333));
#261773=CARTESIAN_POINT('Ctrl Pts',(-44.5079524583208,-59.5441932447742,
-50.4308875));
#261774=CARTESIAN_POINT('Ctrl Pts',(-43.3135644199415,-59.5441932447742,
-50.3725541666667));
#261775=CARTESIAN_POINT('Ctrl Pts',(-42.7163704007519,-58.5098228615615,
-50.3142208333334));
#261776=CARTESIAN_POINT('Ctrl Pts',(-42.1191763815623,-57.4754524783487,
-50.2558875));
#261777=CARTESIAN_POINT('Ctrl Pts',(-42.7163704007519,-56.4410820951361,
-50.1975541666667));
#261778=CARTESIAN_POINT('Ctrl Pts',(-43.3135644199415,-55.4067117119233,
-50.1392208333333));
#261779=CARTESIAN_POINT('Ctrl Pts',(-44.5079524583208,-55.4067117119234,
-50.0808875));
#261780=CARTESIAN_POINT('Ctrl Pts',(-45.7023404967,-55.4067117119233,-50.0225541666667));
#261781=CARTESIAN_POINT('Ctrl Pts',(-46.2995345158897,-56.4410820951361,
-49.9642208333334));
#261782=CARTESIAN_POINT('Ctrl Pts',(-46.8967285350793,-57.4754524783487,
-49.9058875));
#261783=CARTESIAN_POINT('Ctrl Pts',(-46.2995345158897,-58.5098228615615,
-49.8475541666667));
#261784=CARTESIAN_POINT('Ctrl Pts',(-45.7023404967,-59.5441932447742,-49.7892208333333));
#261785=CARTESIAN_POINT('Ctrl Pts',(-44.5079524583208,-59.5441932447742,
-49.7308875));
#261786=CARTESIAN_POINT('Ctrl Pts',(-43.3135644199415,-59.5441932447742,
-49.6725541666667));
#261787=CARTESIAN_POINT('Ctrl Pts',(-42.7163704007519,-58.5098228615615,
-49.6142208333334));
#261788=CARTESIAN_POINT('Ctrl Pts',(-42.1191763815623,-57.4754524783487,
-49.5558875));
#261789=CARTESIAN_POINT('Ctrl Pts',(-42.7163704007519,-56.4410820951361,
-49.4975541666667));
#261790=CARTESIAN_POINT('Ctrl Pts',(-43.3135644199415,-55.4067117119233,
-49.4392208333333));
#261791=CARTESIAN_POINT('Ctrl Pts',(-44.5079524583208,-55.4067117119234,
-49.3808875));
#261792=CARTESIAN_POINT('Ctrl Pts',(-45.7023404967,-55.4067117119233,-49.3225541666667));
#261793=CARTESIAN_POINT('Ctrl Pts',(-46.2995345158897,-56.4410820951361,
-49.2642208333334));
#261794=CARTESIAN_POINT('Ctrl Pts',(-46.8967285350793,-57.4754524783487,
-49.2058875));
#261795=CARTESIAN_POINT('Ctrl Pts',(-46.2995345158897,-58.5098228615615,
-49.1475541666667));
#261796=CARTESIAN_POINT('Ctrl Pts',(-45.7023404967,-59.5441932447742,-49.0892208333333));
#261797=CARTESIAN_POINT('Ctrl Pts',(-44.5079524583208,-59.5441932447742,
-49.0308875));
#261798=CARTESIAN_POINT('Ctrl Pts',(-43.3135644199415,-59.5441932447742,
-48.9725541666667));
#261799=CARTESIAN_POINT('Ctrl Pts',(-42.7163704007519,-58.5098228615615,
-48.9142208333334));
#261800=CARTESIAN_POINT('Ctrl Pts',(-42.1191763815623,-57.4754524783487,
-48.8558875));
#261801=CARTESIAN_POINT('Ctrl Pts',(-42.7163704007519,-56.4410820951361,
-48.7975541666667));
#261802=CARTESIAN_POINT('Ctrl Pts',(-43.3135644199415,-55.4067117119233,
-48.7392208333334));
#261803=CARTESIAN_POINT('Ctrl Pts',(-44.5079524583208,-55.4067117119234,
-48.6808875));
#261804=CARTESIAN_POINT('Ctrl Pts',(-45.7023404967,-55.4067117119233,-48.6225541666667));
#261805=CARTESIAN_POINT('Ctrl Pts',(-46.2995345158897,-56.4410820951361,
-48.5642208333334));
#261806=CARTESIAN_POINT('Ctrl Pts',(-46.8967285350793,-57.4754524783487,
-48.5058875));
#261807=CARTESIAN_POINT('Ctrl Pts',(-46.2995345158897,-58.5098228615615,
-48.4475541666667));
#261808=CARTESIAN_POINT('Ctrl Pts',(-45.7023404967,-59.5441932447742,-48.3892208333334));
#261809=CARTESIAN_POINT('Ctrl Pts',(-44.5079524583208,-59.5441932447742,
-48.3308875));
#261810=CARTESIAN_POINT('Ctrl Pts',(-43.3135644199415,-59.5441932447742,
-48.2725541666667));
#261811=CARTESIAN_POINT('Ctrl Pts',(-42.7163704007519,-58.5098228615615,
-48.2142208333334));
#261812=CARTESIAN_POINT('Ctrl Pts',(-42.1191763815623,-57.4754524783487,
-48.1558875));
#261813=CARTESIAN_POINT('Ctrl Pts',(-42.7163704007519,-56.4410820951361,
-48.0975541666667));
#261814=CARTESIAN_POINT('Ctrl Pts',(-43.3135644199415,-55.4067117119233,
-48.0392208333334));
#261815=CARTESIAN_POINT('Ctrl Pts',(-44.5079524583208,-55.4067117119234,
-47.9808875));
#261816=CARTESIAN_POINT('Ctrl Pts',(-45.7023404967,-55.4067117119233,-47.9225541666667));
#261817=CARTESIAN_POINT('Ctrl Pts',(-46.2995345158897,-56.4410820951361,
-47.8642208333334));
#261818=CARTESIAN_POINT('Ctrl Pts',(-46.8967285350793,-57.4754524783487,
-47.8058875000001));
#261819=CARTESIAN_POINT('Ctrl Pts',(-46.2995345158897,-58.5098228615615,
-47.7475541666667));
#261820=CARTESIAN_POINT('Ctrl Pts',(-45.7023404967,-59.5441932447742,-47.6892208333334));
#261821=CARTESIAN_POINT('Ctrl Pts',(-44.5079524583208,-59.5441932447742,
-47.6308875));
#261822=CARTESIAN_POINT('Ctrl Pts',(-43.3135644199415,-59.5441932447742,
-47.5725541666667));
#261823=CARTESIAN_POINT('Ctrl Pts',(-42.7163704007519,-58.5098228615615,
-47.5142208333333));
#261824=CARTESIAN_POINT('Ctrl Pts',(-42.1191763815623,-57.4754524783487,
-47.4558875));
#261825=CARTESIAN_POINT('Ctrl Pts',(-42.7163704007519,-56.4410820951361,
-47.3975541666667));
#261826=CARTESIAN_POINT('Ctrl Pts',(-43.3135644199415,-55.4067117119233,
-47.3392208333334));
#261827=CARTESIAN_POINT('Ctrl Pts',(-44.5079524583208,-55.4067117119234,
-47.2808875));
#261828=CARTESIAN_POINT('Ctrl Pts',(-45.7023404967,-55.4067117119233,-47.2225541666667));
#261829=CARTESIAN_POINT('Ctrl Pts',(-46.2995345158897,-56.4410820951361,
-47.1642208333334));
#261830=CARTESIAN_POINT('Ctrl Pts',(-46.8967285350793,-57.4754524783487,
-47.1058875));
#261831=CARTESIAN_POINT('Ctrl Pts',(-46.2995345158897,-58.5098228615615,
-47.0475541666667));
#261832=CARTESIAN_POINT('Ctrl Pts',(-45.7023404967,-59.5441932447742,-46.9892208333334));
#261833=CARTESIAN_POINT('Ctrl Pts',(-44.5079524583208,-59.5441932447742,
-46.9308875));
#261834=CARTESIAN_POINT('Ctrl Pts',(-43.3135644199415,-59.5441932447742,
-46.8725541666667));
#261835=CARTESIAN_POINT('Ctrl Pts',(-42.7163704007519,-58.5098228615615,
-46.8142208333334));
#261836=CARTESIAN_POINT('Ctrl Pts',(-42.1191763815623,-57.4754524783487,
-46.7558875));
#261837=CARTESIAN_POINT('Ctrl Pts',(-42.7163704007519,-56.4410820951361,
-46.6975541666667));
#261838=CARTESIAN_POINT('Ctrl Pts',(-43.3135644199415,-55.4067117119233,
-46.6392208333334));
#261839=CARTESIAN_POINT('Ctrl Pts',(-44.5079524583208,-55.4067117119234,
-46.5808875));
#261840=CARTESIAN_POINT('Ctrl Pts',(-45.7023404967,-55.4067117119233,-46.5225541666667));
#261841=CARTESIAN_POINT('Ctrl Pts',(-46.2995345158897,-56.4410820951361,
-46.4642208333334));
#261842=CARTESIAN_POINT('Ctrl Pts',(-46.8967285350793,-57.4754524783487,
-46.4058875));
#261843=CARTESIAN_POINT('Ctrl Pts',(-46.2995345158897,-58.5098228615615,
-46.3475541666667));
#261844=CARTESIAN_POINT('Ctrl Pts',(-45.7023404967,-59.5441932447742,-46.2892208333334));
#261845=CARTESIAN_POINT('Ctrl Pts',(-44.5079524583208,-59.5441932447742,
-46.2308875));
#261846=CARTESIAN_POINT('Ctrl Pts',(-43.3135644199415,-59.5441932447742,
-46.1725541666667));
#261847=CARTESIAN_POINT('Ctrl Pts',(-42.7163704007519,-58.5098228615615,
-46.1142208333334));
#261848=CARTESIAN_POINT('Ctrl Pts',(-42.1191763815623,-57.4754524783487,
-46.0558875));
#261849=CARTESIAN_POINT('Ctrl Pts',(-42.7163704007519,-56.4410820951361,
-45.9975541666667));
#261850=CARTESIAN_POINT('Ctrl Pts',(-43.3135644199415,-55.4067117119233,
-45.9392208333333));
#261851=CARTESIAN_POINT('Ctrl Pts',(-44.5079524583208,-55.4067117119234,
-45.8808875));
#261852=CARTESIAN_POINT('Ctrl Pts',(-45.7023404967,-55.4067117119233,-45.8225541666667));
#261853=CARTESIAN_POINT('Ctrl Pts',(-46.2995345158897,-56.4410820951361,
-45.7642208333334));
#261854=CARTESIAN_POINT('Ctrl Pts',(-46.8967285350793,-57.4754524783487,
-45.7058875));
#261855=CARTESIAN_POINT('Ctrl Pts',(-46.2995345158897,-58.5098228615615,
-45.6475541666667));
#261856=CARTESIAN_POINT('Ctrl Pts',(-45.7023404967,-59.5441932447742,-45.5892208333334));
#261857=CARTESIAN_POINT('Ctrl Pts',(-44.5079524583208,-59.5441932447742,
-45.5308875));
#261858=CARTESIAN_POINT('Ctrl Pts',(-43.3135644199415,-59.5441932447742,
-45.4725541666667));
#261859=CARTESIAN_POINT('Ctrl Pts',(-42.7163704007519,-58.5098228615615,
-45.4142208333334));
#261860=CARTESIAN_POINT('Ctrl Pts',(-42.1191763815623,-57.4754524783487,
-45.3558875));
#261861=CARTESIAN_POINT('Ctrl Pts',(-42.7163704007519,-56.4410820951361,
-45.2975541666667));
#261862=CARTESIAN_POINT('Ctrl Pts',(-43.3135644199415,-55.4067117119233,
-45.2392208333333));
#261863=CARTESIAN_POINT('Ctrl Pts',(-44.5079524583208,-55.4067117119234,
-45.1808875));
#261864=CARTESIAN_POINT('Ctrl Pts',(-45.7023404967,-55.4067117119233,-45.1225541666667));
#261865=CARTESIAN_POINT('Ctrl Pts',(-46.2995345158897,-56.4410820951361,
-45.0642208333334));
#261866=CARTESIAN_POINT('Ctrl Pts',(-46.8967285350793,-57.4754524783487,
-45.0058875));
#261867=CARTESIAN_POINT('Ctrl Pts',(-46.2995345158897,-58.5098228615615,
-44.9475541666667));
#261868=CARTESIAN_POINT('Ctrl Pts',(-45.7023404967,-59.5441932447742,-44.8892208333333));
#261869=CARTESIAN_POINT('Ctrl Pts',(-44.5079524583208,-59.5441932447742,
-44.8308875));
#261870=CARTESIAN_POINT('Ctrl Pts',(-43.3135644199415,-59.5441932447742,
-44.7725541666667));
#261871=CARTESIAN_POINT('Ctrl Pts',(-42.7163704007519,-58.5098228615615,
-44.7142208333334));
#261872=CARTESIAN_POINT('Ctrl Pts',(-42.1191763815623,-57.4754524783487,
-44.6558875));
#261873=CARTESIAN_POINT('Ctrl Pts',(-42.7163704007519,-56.4410820951361,
-44.5975541666667));
#261874=CARTESIAN_POINT('Ctrl Pts',(-43.3135644199415,-55.4067117119233,
-44.5392208333333));
#261875=CARTESIAN_POINT('Ctrl Pts',(-44.5079524583208,-55.4067117119234,
-44.4808875000001));
#261876=CARTESIAN_POINT('Ctrl Pts',(-45.7023404967,-55.4067117119233,-44.4225541666667));
#261877=CARTESIAN_POINT('Ctrl Pts',(-46.2995345158897,-56.4410820951361,
-44.3642208333333));
#261878=CARTESIAN_POINT('Ctrl Pts',(-46.8967285350793,-57.4754524783487,
-44.3058875));
#261879=CARTESIAN_POINT('Ctrl Pts',(-46.2995345158897,-58.5098228615615,
-44.2475541666667));
#261880=CARTESIAN_POINT('Ctrl Pts',(-45.7023404967,-59.5441932447742,-44.1892208333334));
#261881=CARTESIAN_POINT('Ctrl Pts',(-44.5079524583208,-59.5441932447742,
-44.1308875000001));
#261882=CARTESIAN_POINT('Ctrl Pts',(-43.3135644199415,-59.5441932447742,
-44.0725541666667));
#261883=CARTESIAN_POINT('Ctrl Pts',(-42.7163704007519,-58.5098228615615,
-44.0142208333334));
#261884=CARTESIAN_POINT('Ctrl Pts',(-42.1191763815623,-57.4754524783487,
-43.9558875));
#261885=CARTESIAN_POINT('Ctrl Pts',(-42.7163704007519,-56.4410820951361,
-43.8975541666667));
#261886=CARTESIAN_POINT('Ctrl Pts',(-43.3135644199415,-55.4067117119233,
-43.8392208333333));
#261887=CARTESIAN_POINT('Ctrl Pts',(-44.5079524583208,-55.4067117119234,
-43.7808875));
#261888=CARTESIAN_POINT('Ctrl Pts',(-45.7023404967,-55.4067117119233,-43.7225541666667));
#261889=CARTESIAN_POINT('Ctrl Pts',(-46.2995345158897,-56.4410820951361,
-43.6642208333334));
#261890=CARTESIAN_POINT('Ctrl Pts',(-46.8967285350793,-57.4754524783487,
-43.6058875));
#261891=CARTESIAN_POINT('Ctrl Pts',(-46.2995345158897,-58.5098228615615,
-43.5475541666667));
#261892=CARTESIAN_POINT('Ctrl Pts',(-45.7023404967,-59.5441932447742,-43.4892208333333));
#261893=CARTESIAN_POINT('Ctrl Pts',(-44.5079524583208,-59.5441932447742,
-43.4308875));
#261894=CARTESIAN_POINT('Ctrl Pts',(-43.3135644199415,-59.5441932447742,
-43.3725541666667));
#261895=CARTESIAN_POINT('Ctrl Pts',(-42.7163704007519,-58.5098228615615,
-43.3142208333334));
#261896=CARTESIAN_POINT('Ctrl Pts',(-42.1191763815623,-57.4754524783487,
-43.2558875));
#261897=CARTESIAN_POINT('Ctrl Pts',(-42.7163704007519,-56.4410820951361,
-43.1975541666667));
#261898=CARTESIAN_POINT('Ctrl Pts',(-43.3135644199415,-55.4067117119233,
-43.1392208333334));
#261899=CARTESIAN_POINT('Ctrl Pts',(-44.5079524583208,-55.4067117119234,
-43.0808875));
#261900=CARTESIAN_POINT('Ctrl Pts',(-45.7023404967,-55.4067117119233,-43.0225541666667));
#261901=CARTESIAN_POINT('Ctrl Pts',(-46.2995345158897,-56.4410820951361,
-42.9642208333334));
#261902=CARTESIAN_POINT('Ctrl Pts',(-46.8967285350793,-57.4754524783487,
-42.9058875));
#261903=CARTESIAN_POINT('Ctrl Pts',(-46.2995345158897,-58.5098228615615,
-42.8475541666667));
#261904=CARTESIAN_POINT('Ctrl Pts',(-45.7023404967,-59.5441932447742,-42.7892208333334));
#261905=CARTESIAN_POINT('Ctrl Pts',(-44.5079524583208,-59.5441932447742,
-42.7308875000001));
#261906=CARTESIAN_POINT('Ctrl Pts',(-43.3135644199415,-59.5441932447742,
-42.6725541666667));
#261907=CARTESIAN_POINT('Ctrl Pts',(-42.7163704007519,-58.5098228615615,
-42.6142208333334));
#261908=CARTESIAN_POINT('Ctrl Pts',(-42.1191763815623,-57.4754524783487,
-42.5558875));
#261909=CARTESIAN_POINT('Ctrl Pts',(-42.7163704007519,-56.4410820951361,
-42.4975541666667));
#261910=CARTESIAN_POINT('Ctrl Pts',(-43.3135644199415,-55.4067117119233,
-42.4392208333334));
#261911=CARTESIAN_POINT('Ctrl Pts',(-44.5079524583208,-55.4067117119234,
-42.3808875000001));
#261912=CARTESIAN_POINT('Ctrl Pts',(-45.7023404967,-55.4067117119233,-42.3225541666667));
#261913=CARTESIAN_POINT('Ctrl Pts',(-46.2995345158897,-56.4410820951361,
-42.2642208333334));
#261914=CARTESIAN_POINT('Ctrl Pts',(-46.8967285350793,-57.4754524783487,
-42.2058875));
#261915=CARTESIAN_POINT('Ctrl Pts',(-46.2995345158897,-58.5098228615615,
-42.1475541666667));
#261916=CARTESIAN_POINT('Ctrl Pts',(-45.7023404967,-59.5441932447742,-42.0892208333334));
#261917=CARTESIAN_POINT('Ctrl Pts',(-44.5079524583208,-59.5441932447742,
-42.0308875000001));
#261918=CARTESIAN_POINT('Ctrl Pts',(-43.3135644199415,-59.5441932447742,
-41.9725541666667));
#261919=CARTESIAN_POINT('Ctrl Pts',(-42.7163704007519,-58.5098228615615,
-41.9142208333334));
#261920=CARTESIAN_POINT('Ctrl Pts',(-42.1191763815623,-57.4754524783487,
-41.8558875));
#261921=CARTESIAN_POINT('Ctrl Pts',(-42.7163704007519,-56.4410820951361,
-41.7975541666667));
#261922=CARTESIAN_POINT('Ctrl Pts',(-43.3135644199415,-55.4067117119233,
-41.7392208333334));
#261923=CARTESIAN_POINT('Ctrl Pts',(-44.5079524583208,-55.4067117119234,
-41.6808875000001));
#261924=CARTESIAN_POINT('Ctrl Pts',(-45.7023404967,-55.4067117119233,-41.6225541666667));
#261925=CARTESIAN_POINT('Ctrl Pts',(-46.2995345158897,-56.4410820951361,
-41.5642208333334));
#261926=CARTESIAN_POINT('Ctrl Pts',(-46.8967285350793,-57.4754524783487,
-41.5058875));
#261927=CARTESIAN_POINT('Ctrl Pts',(-46.2995345158897,-58.5098228615615,
-41.4475541666667));
#261928=CARTESIAN_POINT('Ctrl Pts',(-45.7023404967,-59.5441932447742,-41.3892208333334));
#261929=CARTESIAN_POINT('Ctrl Pts',(-44.5079524583208,-59.5441932447742,
-41.3308875000001));
#261930=CARTESIAN_POINT('Ctrl Pts',(-43.3135644199415,-59.5441932447742,
-41.2725541666667));
#261931=CARTESIAN_POINT('Ctrl Pts',(-42.7163704007519,-58.5098228615615,
-41.2142208333333));
#261932=CARTESIAN_POINT('Ctrl Pts',(-42.1191763815623,-57.4754524783487,
-41.1558875));
#261933=CARTESIAN_POINT('Ctrl Pts',(-42.7163704007519,-56.4410820951361,
-41.0975541666667));
#261934=CARTESIAN_POINT('Ctrl Pts',(-43.3135644199415,-55.4067117119233,
-41.0392208333333));
#261935=CARTESIAN_POINT('Ctrl Pts',(-44.5079524583208,-55.4067117119234,
-40.9808875000001));
#261936=CARTESIAN_POINT('Ctrl Pts',(-45.7023404967,-55.4067117119233,-40.9225541666667));
#261937=CARTESIAN_POINT('Ctrl Pts',(-46.2995345158897,-56.4410820951361,
-40.8642208333334));
#261938=CARTESIAN_POINT('Ctrl Pts',(-46.8967285350793,-57.4754524783487,
-40.8058875));
#261939=CARTESIAN_POINT('Ctrl Pts',(-46.2995345158897,-58.5098228615615,
-40.7475541666667));
#261940=CARTESIAN_POINT('Ctrl Pts',(-45.7023404967,-59.5441932447742,-40.6892208333333));
#261941=CARTESIAN_POINT('Ctrl Pts',(-44.5079524583208,-59.5441932447742,
-40.6308875));
#261942=CARTESIAN_POINT('Ctrl Pts',(-43.3135644199415,-59.5441932447742,
-40.5725541666667));
#261943=CARTESIAN_POINT('Ctrl Pts',(-42.7163704007519,-58.5098228615615,
-40.5142208333333));
#261944=CARTESIAN_POINT('Ctrl Pts',(-42.1191763815623,-57.4754524783487,
-40.4558875));
#261945=CARTESIAN_POINT('Ctrl Pts',(-42.7163704007519,-56.4410820951361,
-40.3975541666667));
#261946=CARTESIAN_POINT('Ctrl Pts',(-43.3135644199415,-55.4067117119233,
-40.3392208333333));
#261947=CARTESIAN_POINT('Ctrl Pts',(-44.5079524583208,-55.4067117119234,
-40.2808875));
#261948=CARTESIAN_POINT('Ctrl Pts',(-45.7023404967,-55.4067117119233,-40.2225541666667));
#261949=CARTESIAN_POINT('Ctrl Pts',(-46.2995345158897,-56.4410820951361,
-40.1642208333333));
#261950=CARTESIAN_POINT('Ctrl Pts',(-46.8967285350793,-57.4754524783487,
-40.1058875));
#261951=CARTESIAN_POINT('Ctrl Pts',(-46.2995345158897,-58.5098228615615,
-40.0475541666667));
#261952=CARTESIAN_POINT('Ctrl Pts',(-45.7023404967,-59.5441932447742,-39.9892208333333));
#261953=CARTESIAN_POINT('Ctrl Pts',(-44.5079524583208,-59.5441932447742,
-39.9308875));
#261954=CARTESIAN_POINT('Ctrl Pts',(-43.3135644199415,-59.5441932447742,
-39.8725541666667));
#261955=CARTESIAN_POINT('Ctrl Pts',(-42.7163704007519,-58.5098228615615,
-39.8142208333334));
#261956=CARTESIAN_POINT('Ctrl Pts',(-42.1191763815623,-57.4754524783487,
-39.7558875));
#261957=CARTESIAN_POINT('Ctrl Pts',(-42.7163704007519,-56.4410820951361,
-39.6975541666667));
#261958=CARTESIAN_POINT('Ctrl Pts',(-43.3135644199415,-55.4067117119233,
-39.6392208333334));
#261959=CARTESIAN_POINT('Ctrl Pts',(-44.5079524583208,-55.4067117119234,
-39.5808875000001));
#261960=CARTESIAN_POINT('Ctrl Pts',(-45.7023404967,-55.4067117119233,-39.5225541666667));
#261961=CARTESIAN_POINT('Ctrl Pts',(-46.2995345158897,-56.4410820951361,
-39.4642208333333));
#261962=CARTESIAN_POINT('Ctrl Pts',(-46.8967285350793,-57.4754524783487,
-39.4058875));
#261963=CARTESIAN_POINT('Ctrl Pts',(-46.2995345158897,-58.5098228615615,
-39.3475541666667));
#261964=CARTESIAN_POINT('Ctrl Pts',(-45.7023404967,-59.5441932447742,-39.2892208333334));
#261965=CARTESIAN_POINT('Ctrl Pts',(-44.5079524583208,-59.5441932447742,
-39.2308875));
#261966=CARTESIAN_POINT('Ctrl Pts',(-43.3135644199415,-59.5441932447742,
-39.1725541666667));
#261967=CARTESIAN_POINT('Ctrl Pts',(-42.7163704007519,-58.5098228615615,
-39.1142208333333));
#261968=CARTESIAN_POINT('Ctrl Pts',(-42.1191763815623,-57.4754524783487,
-39.0558875));
#261969=CARTESIAN_POINT('Ctrl Pts',(-42.7163704007519,-56.4410820951361,
-38.9975541666667));
#261970=CARTESIAN_POINT('Ctrl Pts',(-43.3135644199415,-55.4067117119233,
-38.9392208333334));
#261971=CARTESIAN_POINT('Ctrl Pts',(-44.5079524583208,-55.4067117119234,
-38.8808875));
#261972=CARTESIAN_POINT('Ctrl Pts',(-45.7023404967,-55.4067117119233,-38.8225541666667));
#261973=CARTESIAN_POINT('Ctrl Pts',(-46.2995345158897,-56.4410820951361,
-38.7642208333333));
#261974=CARTESIAN_POINT('Ctrl Pts',(-46.8967285350793,-57.4754524783487,
-38.7058875));
#261975=CARTESIAN_POINT('Ctrl Pts',(-46.2995345158897,-58.5098228615615,
-38.6475541666667));
#261976=CARTESIAN_POINT('Ctrl Pts',(-45.7023404967,-59.5441932447742,-38.5892208333334));
#261977=CARTESIAN_POINT('Ctrl Pts',(-44.5079524583208,-59.5441932447742,
-38.5308875));
#261978=CARTESIAN_POINT('Ctrl Pts',(-43.3135644199415,-59.5441932447742,
-38.4725541666667));
#261979=CARTESIAN_POINT('Ctrl Pts',(-42.7163704007519,-58.5098228615615,
-38.4142208333334));
#261980=CARTESIAN_POINT('Ctrl Pts',(-42.1191763815623,-57.4754524783487,
-38.3558875));
#261981=CARTESIAN_POINT('Ctrl Pts',(-42.7163704007519,-56.4410820951361,
-38.2975541666667));
#261982=CARTESIAN_POINT('Ctrl Pts',(-43.3135644199415,-55.4067117119233,
-38.2392208333333));
#261983=CARTESIAN_POINT('Ctrl Pts',(-44.5079524583208,-55.4067117119234,
-38.1808875000001));
#261984=CARTESIAN_POINT('Ctrl Pts',(-45.7023404967,-55.4067117119233,-38.1225541666667));
#261985=CARTESIAN_POINT('Ctrl Pts',(-46.2995345158897,-56.4410820951361,
-38.0642208333334));
#261986=CARTESIAN_POINT('Ctrl Pts',(-46.8967285350793,-57.4754524783487,
-38.0058875));
#261987=CARTESIAN_POINT('Ctrl Pts',(-46.2995345158897,-58.5098228615615,
-37.9475541666667));
#261988=CARTESIAN_POINT('Ctrl Pts',(-45.7023404967,-59.5441932447742,-37.8892208333334));
#261989=CARTESIAN_POINT('Ctrl Pts',(-44.5079524583208,-59.5441932447742,
-37.8308875));
#261990=CARTESIAN_POINT('Ctrl Pts',(-43.3135644199415,-59.5441932447742,
-37.7725541666667));
#261991=CARTESIAN_POINT('Ctrl Pts',(-42.7163704007519,-58.5098228615615,
-37.7142208333333));
#261992=CARTESIAN_POINT('Ctrl Pts',(-42.1191763815623,-57.4754524783487,
-37.6558875));
#261993=CARTESIAN_POINT('Ctrl Pts',(-42.7163704007519,-56.4410820951361,
-37.5975541666667));
#261994=CARTESIAN_POINT('Ctrl Pts',(-43.3135644199415,-55.4067117119233,
-37.5392208333334));
#261995=CARTESIAN_POINT('Ctrl Pts',(-44.5079524583208,-55.4067117119234,
-37.4808875));
#261996=CARTESIAN_POINT('Ctrl Pts',(-45.7023404967,-55.4067117119233,-37.4225541666667));
#261997=CARTESIAN_POINT('Ctrl Pts',(-46.2995345158897,-56.4410820951361,
-37.3642208333333));
#261998=CARTESIAN_POINT('Ctrl Pts',(-46.8967285350793,-57.4754524783487,
-37.3058875));
#261999=CARTESIAN_POINT('Ctrl Pts',(-46.2995345158897,-58.5098228615615,
-37.2475541666667));
#262000=CARTESIAN_POINT('Ctrl Pts',(-46.2219998538691,-58.6441168355289,
-37.239980655983));
#262001=CARTESIAN_POINT('Ctrl Pts',(-46.1253112086366,-58.7653513237809,
-37.2318399189827));
#262002=CARTESIAN_POINT('',(-43.5801633933645,-59.1235613262403,-39.7713833389821));
#262003=CARTESIAN_POINT('Ctrl Pts',(-43.5801633933644,-59.1235613262403,
-39.7713833389821));
#262004=CARTESIAN_POINT('Ctrl Pts',(-43.7343054498627,-59.2338784870309,
-39.7948518398299));
#262005=CARTESIAN_POINT('Ctrl Pts',(-43.9040124134241,-59.3204101936929,
-39.8178912026959));
#262006=CARTESIAN_POINT('Ctrl Pts',(-44.2515556962439,-59.4355123678575,
-39.8599414219136));
#262007=CARTESIAN_POINT('Ctrl Pts',(-44.4268269797126,-59.467295367295,
-39.8787333172327));
#262008=CARTESIAN_POINT('Ctrl Pts',(-44.6028144650695,-59.4732025036409,
-39.8960584758442));
#262009=CARTESIAN_POINT('Ctrl Pts',(-45.3904396609892,-55.7772425608068,
-39.4382820396906));
#262010=CARTESIAN_POINT('Ctrl Pts',(-45.127863070379,-55.6880798854926,
-39.4307498115588));
#262011=CARTESIAN_POINT('Ctrl Pts',(-44.8501824314513,-55.65124567929,-39.4267602137955));
#262012=CARTESIAN_POINT('Ctrl Pts',(-44.272714170611,-55.6905726318167,
-39.4247756080659));
#262013=CARTESIAN_POINT('Ctrl Pts',(-44.0459076609694,-55.7713412684499,
-39.429749730603));
#262014=CARTESIAN_POINT('Ctrl Pts',(-43.7113885810197,-55.9220046278699,
-39.4400449959408));
#262015=CARTESIAN_POINT('Ctrl Pts',(-43.5414996037919,-56.0332426275574,
-39.4481441882684));
#262016=CARTESIAN_POINT('Ctrl Pts',(-43.3043122263345,-56.2496978707112,
-39.463510471409));
#262017=CARTESIAN_POINT('Ctrl Pts',(-43.2243163532729,-56.3378976358391,
-39.4697052531975));
#262018=CARTESIAN_POINT('Ctrl Pts',(-43.1510722028329,-56.4358173812626,
-39.4764626542922));
#262019=CARTESIAN_POINT('Ctrl Pts',(-43.1490501437171,-56.4385358974063,
-39.4766501743115));
#262020=CARTESIAN_POINT('Ctrl Pts',(-43.1429859160015,-56.4467348329594,
-39.477215478004));
#262021=CARTESIAN_POINT('Ctrl Pts',(-43.1389661987681,-56.4522315327458,
-39.4775941325867));
#262022=CARTESIAN_POINT('Ctrl Pts',(-43.1268675096469,-56.4689648450911,
-39.4787458758348));
#262023=CARTESIAN_POINT('Ctrl Pts',(-43.1188830933565,-56.4802673936354,
-39.4795224926569));
#262024=CARTESIAN_POINT('Ctrl Pts',(-43.0947203700718,-56.5152795267588,
-39.4819247606914));
#262025=CARTESIAN_POINT('Ctrl Pts',(-43.0789875520127,-56.5392273724946,
-39.4835617361158));
#262026=CARTESIAN_POINT('Ctrl Pts',(-43.0434745327861,-56.5960535881947,
-39.4874324719544));
#262027=CARTESIAN_POINT('Ctrl Pts',(-43.0238940213821,-56.6295843258748,
-39.489685078298));
#262028=CARTESIAN_POINT('Ctrl Pts',(-42.8971332874247,-56.8634741974343,
-39.505873075687));
#262029=CARTESIAN_POINT('Ctrl Pts',(-42.8269092740029,-57.0813286464389,
-39.5229511009414));
#262030=CARTESIAN_POINT('Ctrl Pts',(-42.7655858512823,-57.540255899092,
-39.5633280588462));
#262031=CARTESIAN_POINT('Ctrl Pts',(-42.7783791664303,-57.7782929357622,
-39.5865645306336));
#262032=CARTESIAN_POINT('Ctrl Pts',(-42.8697928172135,-58.1607402986936,
-39.6279729382228));
#262033=CARTESIAN_POINT('Ctrl Pts',(-42.9407328612678,-58.3782873632772,
-39.6516656052854));
#262034=CARTESIAN_POINT('Ctrl Pts',(-43.2188700913275,-58.8092261000328,
-39.7119082485011));
#262035=CARTESIAN_POINT('Ctrl Pts',(-43.3855231146887,-58.9842601944999,
-39.741748885875));
#262036=CARTESIAN_POINT('Ctrl Pts',(-43.5801633933645,-59.1235613262403,
-39.7713833389821));
#262037=CARTESIAN_POINT('Ctrl Pts',(-44.5079524583208,-59.1441977614012,
-52.99995));
#262038=CARTESIAN_POINT('Ctrl Pts',(-43.5445019199415,-59.1441977614012,
-52.9416166666667));
#262039=CARTESIAN_POINT('Ctrl Pts',(-43.0627766507519,-58.309825119875,
-52.8832833333334));
#262040=CARTESIAN_POINT('Ctrl Pts',(-42.5810513815623,-57.4754524783487,
-52.82495));
#262041=CARTESIAN_POINT('Ctrl Pts',(-43.0627766507519,-56.6410798368225,
-52.7666166666667));
#262042=CARTESIAN_POINT('Ctrl Pts',(-43.5445019199415,-55.8067071952963,
-52.7082833333333));
#262043=CARTESIAN_POINT('Ctrl Pts',(-44.5079524583208,-55.8067071952963,
-52.64995));
#262044=CARTESIAN_POINT('Ctrl Pts',(-45.4714029967,-55.8067071952963,-52.5916166666666));
#262045=CARTESIAN_POINT('Ctrl Pts',(-45.9531282658897,-56.6410798368225,
-52.5332833333334));
#262046=CARTESIAN_POINT('Ctrl Pts',(-46.4348535350793,-57.4754524783487,
-52.4749500000001));
#262047=CARTESIAN_POINT('Ctrl Pts',(-45.9531282658897,-58.309825119875,
-52.4166166666667));
#262048=CARTESIAN_POINT('Ctrl Pts',(-45.4714029967,-59.1441977614012,-52.3582833333334));
#262049=CARTESIAN_POINT('Ctrl Pts',(-44.5079524583208,-59.1441977614012,
-52.29995));
#262050=CARTESIAN_POINT('Ctrl Pts',(-43.5445019199415,-59.1441977614012,
-52.2416166666667));
#262051=CARTESIAN_POINT('Ctrl Pts',(-43.0627766507519,-58.309825119875,
-52.1832833333333));
#262052=CARTESIAN_POINT('Ctrl Pts',(-42.5810513815623,-57.4754524783487,
-52.12495));
#262053=CARTESIAN_POINT('Ctrl Pts',(-43.0627766507519,-56.6410798368225,
-52.0666166666667));
#262054=CARTESIAN_POINT('Ctrl Pts',(-43.5445019199415,-55.8067071952963,
-52.0082833333333));
#262055=CARTESIAN_POINT('Ctrl Pts',(-44.5079524583208,-55.8067071952963,
-51.94995));
#262056=CARTESIAN_POINT('Ctrl Pts',(-45.4714029967,-55.8067071952963,-51.8916166666667));
#262057=CARTESIAN_POINT('Ctrl Pts',(-45.9531282658897,-56.6410798368225,
-51.8332833333334));
#262058=CARTESIAN_POINT('Ctrl Pts',(-46.4348535350793,-57.4754524783487,
-51.77495));
#262059=CARTESIAN_POINT('Ctrl Pts',(-45.9531282658897,-58.309825119875,
-51.7166166666667));
#262060=CARTESIAN_POINT('Ctrl Pts',(-45.4714029967,-59.1441977614012,-51.6582833333333));
#262061=CARTESIAN_POINT('Ctrl Pts',(-44.5079524583208,-59.1441977614012,
-51.59995));
#262062=CARTESIAN_POINT('Ctrl Pts',(-43.5445019199415,-59.1441977614012,
-51.5416166666667));
#262063=CARTESIAN_POINT('Ctrl Pts',(-43.0627766507519,-58.309825119875,
-51.4832833333334));
#262064=CARTESIAN_POINT('Ctrl Pts',(-42.5810513815623,-57.4754524783487,
-51.42495));
#262065=CARTESIAN_POINT('Ctrl Pts',(-43.0627766507519,-56.6410798368225,
-51.3666166666667));
#262066=CARTESIAN_POINT('Ctrl Pts',(-43.5445019199415,-55.8067071952963,
-51.3082833333333));
#262067=CARTESIAN_POINT('Ctrl Pts',(-44.5079524583208,-55.8067071952963,
-51.24995));
#262068=CARTESIAN_POINT('Ctrl Pts',(-45.4714029967,-55.8067071952963,-51.1916166666667));
#262069=CARTESIAN_POINT('Ctrl Pts',(-45.9531282658897,-56.6410798368225,
-51.1332833333334));
#262070=CARTESIAN_POINT('Ctrl Pts',(-46.4348535350793,-57.4754524783487,
-51.07495));
#262071=CARTESIAN_POINT('Ctrl Pts',(-45.9531282658897,-58.309825119875,
-51.0166166666667));
#262072=CARTESIAN_POINT('Ctrl Pts',(-45.4714029967,-59.1441977614012,-50.9582833333334));
#262073=CARTESIAN_POINT('Ctrl Pts',(-44.5079524583208,-59.1441977614012,
-50.89995));
#262074=CARTESIAN_POINT('Ctrl Pts',(-43.5445019199415,-59.1441977614012,
-50.8416166666667));
#262075=CARTESIAN_POINT('Ctrl Pts',(-43.0627766507519,-58.309825119875,
-50.7832833333333));
#262076=CARTESIAN_POINT('Ctrl Pts',(-42.5810513815623,-57.4754524783487,
-50.72495));
#262077=CARTESIAN_POINT('Ctrl Pts',(-43.0627766507519,-56.6410798368225,
-50.6666166666667));
#262078=CARTESIAN_POINT('Ctrl Pts',(-43.5445019199415,-55.8067071952963,
-50.6082833333334));
#262079=CARTESIAN_POINT('Ctrl Pts',(-44.5079524583208,-55.8067071952963,
-50.54995));
#262080=CARTESIAN_POINT('Ctrl Pts',(-45.4714029967,-55.8067071952963,-50.4916166666667));
#262081=CARTESIAN_POINT('Ctrl Pts',(-45.9531282658897,-56.6410798368225,
-50.4332833333333));
#262082=CARTESIAN_POINT('Ctrl Pts',(-46.4348535350793,-57.4754524783487,
-50.37495));
#262083=CARTESIAN_POINT('Ctrl Pts',(-45.9531282658897,-58.309825119875,
-50.3166166666667));
#262084=CARTESIAN_POINT('Ctrl Pts',(-45.4714029967,-59.1441977614012,-50.2582833333334));
#262085=CARTESIAN_POINT('Ctrl Pts',(-44.5079524583208,-59.1441977614012,
-50.19995));
#262086=CARTESIAN_POINT('Ctrl Pts',(-43.5445019199415,-59.1441977614012,
-50.1416166666667));
#262087=CARTESIAN_POINT('Ctrl Pts',(-43.0627766507519,-58.309825119875,
-50.0832833333334));
#262088=CARTESIAN_POINT('Ctrl Pts',(-42.5810513815623,-57.4754524783487,
-50.02495));
#262089=CARTESIAN_POINT('Ctrl Pts',(-43.0627766507519,-56.6410798368225,
-49.9666166666667));
#262090=CARTESIAN_POINT('Ctrl Pts',(-43.5445019199415,-55.8067071952963,
-49.9082833333334));
#262091=CARTESIAN_POINT('Ctrl Pts',(-44.5079524583208,-55.8067071952963,
-49.84995));
#262092=CARTESIAN_POINT('Ctrl Pts',(-45.4714029967,-55.8067071952963,-49.7916166666667));
#262093=CARTESIAN_POINT('Ctrl Pts',(-45.9531282658897,-56.6410798368225,
-49.7332833333334));
#262094=CARTESIAN_POINT('Ctrl Pts',(-46.4348535350793,-57.4754524783487,
-49.67495));
#262095=CARTESIAN_POINT('Ctrl Pts',(-45.9531282658897,-58.309825119875,
-49.6166166666667));
#262096=CARTESIAN_POINT('Ctrl Pts',(-45.4714029967,-59.1441977614012,-49.5582833333334));
#262097=CARTESIAN_POINT('Ctrl Pts',(-44.5079524583208,-59.1441977614012,
-49.49995));
#262098=CARTESIAN_POINT('Ctrl Pts',(-43.5445019199415,-59.1441977614012,
-49.4416166666667));
#262099=CARTESIAN_POINT('Ctrl Pts',(-43.0627766507519,-58.309825119875,
-49.3832833333334));
#262100=CARTESIAN_POINT('Ctrl Pts',(-42.5810513815623,-57.4754524783487,
-49.32495));
#262101=CARTESIAN_POINT('Ctrl Pts',(-43.0627766507519,-56.6410798368225,
-49.2666166666667));
#262102=CARTESIAN_POINT('Ctrl Pts',(-43.5445019199415,-55.8067071952963,
-49.2082833333334));
#262103=CARTESIAN_POINT('Ctrl Pts',(-44.5079524583208,-55.8067071952963,
-49.14995));
#262104=CARTESIAN_POINT('Ctrl Pts',(-45.4714029967,-55.8067071952963,-49.0916166666667));
#262105=CARTESIAN_POINT('Ctrl Pts',(-45.9531282658897,-56.6410798368225,
-49.0332833333333));
#262106=CARTESIAN_POINT('Ctrl Pts',(-46.4348535350793,-57.4754524783487,
-48.97495));
#262107=CARTESIAN_POINT('Ctrl Pts',(-45.9531282658897,-58.309825119875,
-48.9166166666667));
#262108=CARTESIAN_POINT('Ctrl Pts',(-45.4714029967,-59.1441977614012,-48.8582833333333));
#262109=CARTESIAN_POINT('Ctrl Pts',(-44.5079524583208,-59.1441977614012,
-48.79995));
#262110=CARTESIAN_POINT('Ctrl Pts',(-43.5445019199415,-59.1441977614012,
-48.7416166666667));
#262111=CARTESIAN_POINT('Ctrl Pts',(-43.0627766507519,-58.309825119875,
-48.6832833333334));
#262112=CARTESIAN_POINT('Ctrl Pts',(-42.5810513815623,-57.4754524783487,
-48.62495));
#262113=CARTESIAN_POINT('Ctrl Pts',(-43.0627766507519,-56.6410798368225,
-48.5666166666667));
#262114=CARTESIAN_POINT('Ctrl Pts',(-43.5445019199415,-55.8067071952963,
-48.5082833333334));
#262115=CARTESIAN_POINT('Ctrl Pts',(-44.5079524583208,-55.8067071952963,
-48.44995));
#262116=CARTESIAN_POINT('Ctrl Pts',(-45.4714029967,-55.8067071952963,-48.3916166666667));
#262117=CARTESIAN_POINT('Ctrl Pts',(-45.9531282658897,-56.6410798368225,
-48.3332833333334));
#262118=CARTESIAN_POINT('Ctrl Pts',(-46.4348535350793,-57.4754524783487,
-48.27495));
#262119=CARTESIAN_POINT('Ctrl Pts',(-45.9531282658897,-58.309825119875,
-48.2166166666667));
#262120=CARTESIAN_POINT('Ctrl Pts',(-45.4714029967,-59.1441977614012,-48.1582833333334));
#262121=CARTESIAN_POINT('Ctrl Pts',(-44.5079524583208,-59.1441977614012,
-48.09995));
#262122=CARTESIAN_POINT('Ctrl Pts',(-43.5445019199415,-59.1441977614012,
-48.0416166666667));
#262123=CARTESIAN_POINT('Ctrl Pts',(-43.0627766507519,-58.309825119875,
-47.9832833333334));
#262124=CARTESIAN_POINT('Ctrl Pts',(-42.5810513815623,-57.4754524783487,
-47.92495));
#262125=CARTESIAN_POINT('Ctrl Pts',(-43.0627766507519,-56.6410798368225,
-47.8666166666667));
#262126=CARTESIAN_POINT('Ctrl Pts',(-43.5445019199415,-55.8067071952963,
-47.8082833333333));
#262127=CARTESIAN_POINT('Ctrl Pts',(-44.5079524583208,-55.8067071952963,
-47.74995));
#262128=CARTESIAN_POINT('Ctrl Pts',(-45.4714029967,-55.8067071952963,-47.6916166666667));
#262129=CARTESIAN_POINT('Ctrl Pts',(-45.9531282658897,-56.6410798368225,
-47.6332833333333));
#262130=CARTESIAN_POINT('Ctrl Pts',(-46.4348535350793,-57.4754524783487,
-47.57495));
#262131=CARTESIAN_POINT('Ctrl Pts',(-45.9531282658897,-58.309825119875,
-47.5166166666667));
#262132=CARTESIAN_POINT('Ctrl Pts',(-45.4714029967,-59.1441977614012,-47.4582833333333));
#262133=CARTESIAN_POINT('Ctrl Pts',(-44.5079524583208,-59.1441977614012,
-47.39995));
#262134=CARTESIAN_POINT('Ctrl Pts',(-43.5445019199415,-59.1441977614012,
-47.3416166666666));
#262135=CARTESIAN_POINT('Ctrl Pts',(-43.0627766507519,-58.309825119875,
-47.2832833333333));
#262136=CARTESIAN_POINT('Ctrl Pts',(-42.5810513815623,-57.4754524783487,
-47.22495));
#262137=CARTESIAN_POINT('Ctrl Pts',(-43.0627766507519,-56.6410798368225,
-47.1666166666667));
#262138=CARTESIAN_POINT('Ctrl Pts',(-43.5445019199415,-55.8067071952963,
-47.1082833333333));
#262139=CARTESIAN_POINT('Ctrl Pts',(-44.5079524583208,-55.8067071952963,
-47.04995));
#262140=CARTESIAN_POINT('Ctrl Pts',(-45.4714029967,-55.8067071952963,-46.9916166666667));
#262141=CARTESIAN_POINT('Ctrl Pts',(-45.9531282658897,-56.6410798368225,
-46.9332833333334));
#262142=CARTESIAN_POINT('Ctrl Pts',(-46.4348535350793,-57.4754524783487,
-46.87495));
#262143=CARTESIAN_POINT('Ctrl Pts',(-45.9531282658897,-58.309825119875,
-46.8166166666667));
#262144=CARTESIAN_POINT('Ctrl Pts',(-45.4714029967,-59.1441977614012,-46.7582833333333));
#262145=CARTESIAN_POINT('Ctrl Pts',(-44.5079524583208,-59.1441977614012,
-46.69995));
#262146=CARTESIAN_POINT('Ctrl Pts',(-43.5445019199415,-59.1441977614012,
-46.6416166666666));
#262147=CARTESIAN_POINT('Ctrl Pts',(-43.0627766507519,-58.309825119875,
-46.5832833333334));
#262148=CARTESIAN_POINT('Ctrl Pts',(-42.5810513815623,-57.4754524783487,
-46.52495));
#262149=CARTESIAN_POINT('Ctrl Pts',(-43.0627766507519,-56.6410798368225,
-46.4666166666667));
#262150=CARTESIAN_POINT('Ctrl Pts',(-43.5445019199415,-55.8067071952963,
-46.4082833333333));
#262151=CARTESIAN_POINT('Ctrl Pts',(-44.5079524583208,-55.8067071952963,
-46.34995));
#262152=CARTESIAN_POINT('Ctrl Pts',(-45.4714029967,-55.8067071952963,-46.2916166666667));
#262153=CARTESIAN_POINT('Ctrl Pts',(-45.9531282658897,-56.6410798368225,
-46.2332833333334));
#262154=CARTESIAN_POINT('Ctrl Pts',(-46.4348535350793,-57.4754524783487,
-46.17495));
#262155=CARTESIAN_POINT('Ctrl Pts',(-45.9531282658897,-58.309825119875,
-46.1166166666667));
#262156=CARTESIAN_POINT('Ctrl Pts',(-45.4714029967,-59.1441977614012,-46.0582833333333));
#262157=CARTESIAN_POINT('Ctrl Pts',(-44.5079524583208,-59.1441977614012,
-45.99995));
#262158=CARTESIAN_POINT('Ctrl Pts',(-43.5445019199415,-59.1441977614012,
-45.9416166666667));
#262159=CARTESIAN_POINT('Ctrl Pts',(-43.0627766507519,-58.309825119875,
-45.8832833333333));
#262160=CARTESIAN_POINT('Ctrl Pts',(-42.5810513815623,-57.4754524783487,
-45.82495));
#262161=CARTESIAN_POINT('Ctrl Pts',(-43.0627766507519,-56.6410798368225,
-45.7666166666667));
#262162=CARTESIAN_POINT('Ctrl Pts',(-43.5445019199415,-55.8067071952963,
-45.7082833333333));
#262163=CARTESIAN_POINT('Ctrl Pts',(-44.5079524583208,-55.8067071952963,
-45.64995));
#262164=CARTESIAN_POINT('Ctrl Pts',(-45.4714029967,-55.8067071952963,-45.5916166666667));
#262165=CARTESIAN_POINT('Ctrl Pts',(-45.9531282658897,-56.6410798368225,
-45.5332833333333));
#262166=CARTESIAN_POINT('Ctrl Pts',(-46.4348535350793,-57.4754524783487,
-45.47495));
#262167=CARTESIAN_POINT('Ctrl Pts',(-45.9531282658897,-58.309825119875,
-45.4166166666667));
#262168=CARTESIAN_POINT('Ctrl Pts',(-45.4714029967,-59.1441977614012,-45.3582833333333));
#262169=CARTESIAN_POINT('Ctrl Pts',(-44.5079524583208,-59.1441977614012,
-45.29995));
#262170=CARTESIAN_POINT('Ctrl Pts',(-43.5445019199415,-59.1441977614012,
-45.2416166666667));
#262171=CARTESIAN_POINT('Ctrl Pts',(-43.0627766507519,-58.309825119875,
-45.1832833333334));
#262172=CARTESIAN_POINT('Ctrl Pts',(-42.5810513815623,-57.4754524783487,
-45.12495));
#262173=CARTESIAN_POINT('Ctrl Pts',(-43.0627766507519,-56.6410798368225,
-45.0666166666667));
#262174=CARTESIAN_POINT('Ctrl Pts',(-43.5445019199415,-55.8067071952963,
-45.0082833333334));
#262175=CARTESIAN_POINT('Ctrl Pts',(-44.5079524583208,-55.8067071952963,
-44.94995));
#262176=CARTESIAN_POINT('Ctrl Pts',(-45.4714029967,-55.8067071952963,-44.8916166666667));
#262177=CARTESIAN_POINT('Ctrl Pts',(-45.9531282658897,-56.6410798368225,
-44.8332833333334));
#262178=CARTESIAN_POINT('Ctrl Pts',(-46.4348535350793,-57.4754524783487,
-44.77495));
#262179=CARTESIAN_POINT('Ctrl Pts',(-45.9531282658897,-58.309825119875,
-44.7166166666667));
#262180=CARTESIAN_POINT('Ctrl Pts',(-45.4714029967,-59.1441977614012,-44.6582833333334));
#262181=CARTESIAN_POINT('Ctrl Pts',(-44.5079524583208,-59.1441977614012,
-44.59995));
#262182=CARTESIAN_POINT('Ctrl Pts',(-43.5445019199415,-59.1441977614012,
-44.5416166666667));
#262183=CARTESIAN_POINT('Ctrl Pts',(-43.0627766507519,-58.309825119875,
-44.4832833333334));
#262184=CARTESIAN_POINT('Ctrl Pts',(-42.5810513815623,-57.4754524783487,
-44.42495));
#262185=CARTESIAN_POINT('Ctrl Pts',(-43.0627766507519,-56.6410798368225,
-44.3666166666667));
#262186=CARTESIAN_POINT('Ctrl Pts',(-43.5445019199415,-55.8067071952963,
-44.3082833333334));
#262187=CARTESIAN_POINT('Ctrl Pts',(-44.5079524583208,-55.8067071952963,
-44.24995));
#262188=CARTESIAN_POINT('Ctrl Pts',(-45.4714029967,-55.8067071952963,-44.1916166666667));
#262189=CARTESIAN_POINT('Ctrl Pts',(-45.9531282658897,-56.6410798368225,
-44.1332833333334));
#262190=CARTESIAN_POINT('Ctrl Pts',(-46.4348535350793,-57.4754524783487,
-44.07495));
#262191=CARTESIAN_POINT('Ctrl Pts',(-45.9531282658897,-58.309825119875,
-44.0166166666667));
#262192=CARTESIAN_POINT('Ctrl Pts',(-45.4714029967,-59.1441977614012,-43.9582833333334));
#262193=CARTESIAN_POINT('Ctrl Pts',(-44.5079524583208,-59.1441977614012,
-43.89995));
#262194=CARTESIAN_POINT('Ctrl Pts',(-43.5445019199415,-59.1441977614012,
-43.8416166666667));
#262195=CARTESIAN_POINT('Ctrl Pts',(-43.0627766507519,-58.309825119875,
-43.7832833333334));
#262196=CARTESIAN_POINT('Ctrl Pts',(-42.5810513815623,-57.4754524783487,
-43.72495));
#262197=CARTESIAN_POINT('Ctrl Pts',(-43.0627766507519,-56.6410798368225,
-43.6666166666667));
#262198=CARTESIAN_POINT('Ctrl Pts',(-43.5445019199415,-55.8067071952963,
-43.6082833333333));
#262199=CARTESIAN_POINT('Ctrl Pts',(-44.5079524583208,-55.8067071952963,
-43.54995));
#262200=CARTESIAN_POINT('Ctrl Pts',(-45.4714029967,-55.8067071952963,-43.4916166666667));
#262201=CARTESIAN_POINT('Ctrl Pts',(-45.9531282658897,-56.6410798368225,
-43.4332833333333));
#262202=CARTESIAN_POINT('Ctrl Pts',(-46.4348535350793,-57.4754524783487,
-43.37495));
#262203=CARTESIAN_POINT('Ctrl Pts',(-45.9531282658897,-58.309825119875,
-43.3166166666667));
#262204=CARTESIAN_POINT('Ctrl Pts',(-45.4714029967,-59.1441977614012,-43.2582833333333));
#262205=CARTESIAN_POINT('Ctrl Pts',(-44.5079524583208,-59.1441977614012,
-43.19995));
#262206=CARTESIAN_POINT('Ctrl Pts',(-43.5445019199415,-59.1441977614012,
-43.1416166666667));
#262207=CARTESIAN_POINT('Ctrl Pts',(-43.0627766507519,-58.309825119875,
-43.0832833333333));
#262208=CARTESIAN_POINT('Ctrl Pts',(-42.5810513815623,-57.4754524783487,
-43.02495));
#262209=CARTESIAN_POINT('Ctrl Pts',(-43.0627766507519,-56.6410798368225,
-42.9666166666667));
#262210=CARTESIAN_POINT('Ctrl Pts',(-43.5445019199415,-55.8067071952963,
-42.9082833333333));
#262211=CARTESIAN_POINT('Ctrl Pts',(-44.5079524583208,-55.8067071952963,
-42.84995));
#262212=CARTESIAN_POINT('Ctrl Pts',(-45.4714029967,-55.8067071952963,-42.7916166666667));
#262213=CARTESIAN_POINT('Ctrl Pts',(-45.9531282658897,-56.6410798368225,
-42.7332833333334));
#262214=CARTESIAN_POINT('Ctrl Pts',(-46.4348535350793,-57.4754524783487,
-42.67495));
#262215=CARTESIAN_POINT('Ctrl Pts',(-45.9531282658897,-58.309825119875,
-42.6166166666667));
#262216=CARTESIAN_POINT('Ctrl Pts',(-45.4714029967,-59.1441977614012,-42.5582833333333));
#262217=CARTESIAN_POINT('Ctrl Pts',(-44.5079524583208,-59.1441977614012,
-42.49995));
#262218=CARTESIAN_POINT('Ctrl Pts',(-43.5445019199415,-59.1441977614012,
-42.4416166666667));
#262219=CARTESIAN_POINT('Ctrl Pts',(-43.0627766507519,-58.309825119875,
-42.3832833333333));
#262220=CARTESIAN_POINT('Ctrl Pts',(-42.5810513815623,-57.4754524783487,
-42.32495));
#262221=CARTESIAN_POINT('Ctrl Pts',(-43.0627766507519,-56.6410798368225,
-42.2666166666667));
#262222=CARTESIAN_POINT('Ctrl Pts',(-43.5445019199415,-55.8067071952963,
-42.2082833333333));
#262223=CARTESIAN_POINT('Ctrl Pts',(-44.5079524583208,-55.8067071952963,
-42.14995));
#262224=CARTESIAN_POINT('Ctrl Pts',(-45.4714029967,-55.8067071952963,-42.0916166666667));
#262225=CARTESIAN_POINT('Ctrl Pts',(-45.9531282658897,-56.6410798368225,
-42.0332833333334));
#262226=CARTESIAN_POINT('Ctrl Pts',(-46.4348535350793,-57.4754524783487,
-41.97495));
#262227=CARTESIAN_POINT('Ctrl Pts',(-45.9531282658897,-58.309825119875,
-41.9166166666667));
#262228=CARTESIAN_POINT('Ctrl Pts',(-45.4714029967,-59.1441977614012,-41.8582833333333));
#262229=CARTESIAN_POINT('Ctrl Pts',(-44.5079524583208,-59.1441977614012,
-41.79995));
#262230=CARTESIAN_POINT('Ctrl Pts',(-43.5445019199415,-59.1441977614012,
-41.7416166666667));
#262231=CARTESIAN_POINT('Ctrl Pts',(-43.0627766507519,-58.309825119875,
-41.6832833333333));
#262232=CARTESIAN_POINT('Ctrl Pts',(-42.5810513815623,-57.4754524783487,
-41.62495));
#262233=CARTESIAN_POINT('Ctrl Pts',(-43.0627766507519,-56.6410798368225,
-41.5666166666667));
#262234=CARTESIAN_POINT('Ctrl Pts',(-43.5445019199415,-55.8067071952963,
-41.5082833333334));
#262235=CARTESIAN_POINT('Ctrl Pts',(-44.5079524583208,-55.8067071952963,
-41.44995));
#262236=CARTESIAN_POINT('Ctrl Pts',(-45.4714029967,-55.8067071952963,-41.3916166666667));
#262237=CARTESIAN_POINT('Ctrl Pts',(-45.9531282658897,-56.6410798368225,
-41.3332833333334));
#262238=CARTESIAN_POINT('Ctrl Pts',(-46.4348535350793,-57.4754524783487,
-41.27495));
#262239=CARTESIAN_POINT('Ctrl Pts',(-45.9531282658897,-58.309825119875,
-41.2166166666667));
#262240=CARTESIAN_POINT('Ctrl Pts',(-45.4714029967,-59.1441977614012,-41.1582833333333));
#262241=CARTESIAN_POINT('Ctrl Pts',(-44.5079524583208,-59.1441977614012,
-41.09995));
#262242=CARTESIAN_POINT('Ctrl Pts',(-43.5445019199415,-59.1441977614012,
-41.0416166666667));
#262243=CARTESIAN_POINT('Ctrl Pts',(-43.0627766507519,-58.309825119875,
-40.9832833333333));
#262244=CARTESIAN_POINT('Ctrl Pts',(-42.5810513815623,-57.4754524783487,
-40.92495));
#262245=CARTESIAN_POINT('Ctrl Pts',(-43.0627766507519,-56.6410798368225,
-40.8666166666667));
#262246=CARTESIAN_POINT('Ctrl Pts',(-43.5445019199415,-55.8067071952963,
-40.8082833333334));
#262247=CARTESIAN_POINT('Ctrl Pts',(-44.5079524583208,-55.8067071952963,
-40.74995));
#262248=CARTESIAN_POINT('Ctrl Pts',(-45.4714029967,-55.8067071952963,-40.6916166666667));
#262249=CARTESIAN_POINT('Ctrl Pts',(-45.9531282658897,-56.6410798368225,
-40.6332833333334));
#262250=CARTESIAN_POINT('Ctrl Pts',(-46.4348535350793,-57.4754524783487,
-40.57495));
#262251=CARTESIAN_POINT('Ctrl Pts',(-45.9531282658897,-58.309825119875,
-40.5166166666667));
#262252=CARTESIAN_POINT('Ctrl Pts',(-45.4714029967,-59.1441977614012,-40.4582833333333));
#262253=CARTESIAN_POINT('Ctrl Pts',(-44.5079524583208,-59.1441977614012,
-40.39995));
#262254=CARTESIAN_POINT('Ctrl Pts',(-43.5445019199415,-59.1441977614012,
-40.3416166666667));
#262255=CARTESIAN_POINT('Ctrl Pts',(-43.0627766507519,-58.309825119875,
-40.2832833333334));
#262256=CARTESIAN_POINT('Ctrl Pts',(-42.5810513815623,-57.4754524783487,
-40.22495));
#262257=CARTESIAN_POINT('Ctrl Pts',(-43.0627766507519,-56.6410798368225,
-40.1666166666667));
#262258=CARTESIAN_POINT('Ctrl Pts',(-43.5445019199415,-55.8067071952963,
-40.1082833333334));
#262259=CARTESIAN_POINT('Ctrl Pts',(-44.5079524583208,-55.8067071952963,
-40.04995));
#262260=CARTESIAN_POINT('Ctrl Pts',(-45.4714029967,-55.8067071952963,-39.9916166666667));
#262261=CARTESIAN_POINT('Ctrl Pts',(-45.9531282658897,-56.6410798368225,
-39.9332833333333));
#262262=CARTESIAN_POINT('Ctrl Pts',(-46.4348535350793,-57.4754524783487,
-39.87495));
#262263=CARTESIAN_POINT('Ctrl Pts',(-45.9531282658897,-58.309825119875,
-39.8166166666667));
#262264=CARTESIAN_POINT('Ctrl Pts',(-45.4714029967,-59.1441977614012,-39.7582833333334));
#262265=CARTESIAN_POINT('Ctrl Pts',(-44.5079524583208,-59.1441977614012,
-39.69995));
#262266=CARTESIAN_POINT('Ctrl Pts',(-43.5445019199415,-59.1441977614012,
-39.6416166666667));
#262267=CARTESIAN_POINT('Ctrl Pts',(-43.0627766507519,-58.309825119875,
-39.5832833333333));
#262268=CARTESIAN_POINT('Ctrl Pts',(-42.5810513815623,-57.4754524783487,
-39.52495));
#262269=CARTESIAN_POINT('Ctrl Pts',(-43.0627766507519,-56.6410798368225,
-39.4666166666667));
#262270=CARTESIAN_POINT('Ctrl Pts',(-43.5445019199415,-55.8067071952963,
-39.4082833333334));
#262271=CARTESIAN_POINT('Ctrl Pts',(-44.5079524583208,-55.8067071952963,
-39.34995));
#262272=CARTESIAN_POINT('Ctrl Pts',(-45.4714029967,-55.8067071952963,-39.2916166666667));
#262273=CARTESIAN_POINT('Ctrl Pts',(-45.9531282658897,-56.6410798368225,
-39.2332833333333));
#262274=CARTESIAN_POINT('Ctrl Pts',(-46.4348535350793,-57.4754524783487,
-39.17495));
#262275=CARTESIAN_POINT('Ctrl Pts',(-45.9531282658897,-58.309825119875,
-39.1166166666667));
#262276=CARTESIAN_POINT('Ctrl Pts',(-45.4714029967,-59.1441977614012,-39.0582833333334));
#262277=CARTESIAN_POINT('Ctrl Pts',(-44.5079524583208,-59.1441977614012,
-38.99995));
#262278=CARTESIAN_POINT('Ctrl Pts',(-43.5445019199415,-59.1441977614012,
-38.9416166666667));
#262279=CARTESIAN_POINT('Ctrl Pts',(-43.0627766507519,-58.309825119875,
-38.8832833333334));
#262280=CARTESIAN_POINT('Ctrl Pts',(-42.5810513815623,-57.4754524783487,
-38.82495));
#262281=CARTESIAN_POINT('Ctrl Pts',(-43.0627766507519,-56.6410798368225,
-38.7666166666667));
#262282=CARTESIAN_POINT('Ctrl Pts',(-43.5445019199415,-55.8067071952963,
-38.7082833333334));
#262283=CARTESIAN_POINT('Ctrl Pts',(-44.5079524583208,-55.8067071952963,
-38.64995));
#262284=CARTESIAN_POINT('Ctrl Pts',(-45.4714029967,-55.8067071952963,-38.5916166666667));
#262285=CARTESIAN_POINT('Ctrl Pts',(-45.9531282658897,-56.6410798368225,
-38.5332833333334));
#262286=CARTESIAN_POINT('Ctrl Pts',(-46.4348535350793,-57.4754524783487,
-38.47495));
#262287=CARTESIAN_POINT('Ctrl Pts',(-45.9531282658897,-58.309825119875,
-38.4166166666667));
#262288=CARTESIAN_POINT('Ctrl Pts',(-45.4714029967,-59.1441977614012,-38.3582833333333));
#262289=CARTESIAN_POINT('Ctrl Pts',(-44.5079524583208,-59.1441977614012,
-38.29995));
#262290=CARTESIAN_POINT('Ctrl Pts',(-43.5445019199415,-59.1441977614012,
-38.2416166666667));
#262291=CARTESIAN_POINT('Ctrl Pts',(-43.0627766507519,-58.309825119875,
-38.1832833333333));
#262292=CARTESIAN_POINT('Ctrl Pts',(-42.5810513815623,-57.4754524783487,
-38.12495));
#262293=CARTESIAN_POINT('Ctrl Pts',(-43.0627766507519,-56.6410798368225,
-38.0666166666667));
#262294=CARTESIAN_POINT('Ctrl Pts',(-43.5445019199415,-55.8067071952963,
-38.0082833333333));
#262295=CARTESIAN_POINT('Ctrl Pts',(-44.5079524583208,-55.8067071952963,
-37.94995));
#262296=CARTESIAN_POINT('Ctrl Pts',(-45.4714029967,-55.8067071952963,-37.8916166666667));
#262297=CARTESIAN_POINT('Ctrl Pts',(-45.9531282658897,-56.6410798368225,
-37.8332833333334));
#262298=CARTESIAN_POINT('Ctrl Pts',(-46.4348535350793,-57.4754524783487,
-37.77495));
#262299=CARTESIAN_POINT('Ctrl Pts',(-45.9531282658897,-58.309825119875,
-37.7166166666667));
#262300=CARTESIAN_POINT('Ctrl Pts',(-45.4714029967,-59.1441977614012,-37.6582833333333));
#262301=CARTESIAN_POINT('Ctrl Pts',(-44.5079524583208,-59.1441977614012,
-37.59995));
#262302=CARTESIAN_POINT('Ctrl Pts',(-43.5445019199415,-59.1441977614012,
-37.5416166666667));
#262303=CARTESIAN_POINT('Ctrl Pts',(-43.0627766507519,-58.309825119875,
-37.4832833333334));
#262304=CARTESIAN_POINT('Ctrl Pts',(-42.5810513815623,-57.4754524783487,
-37.42495));
#262305=CARTESIAN_POINT('Ctrl Pts',(-43.0627766507519,-56.6410798368225,
-37.3666166666667));
#262306=CARTESIAN_POINT('Ctrl Pts',(-43.5445019199415,-55.8067071952963,
-37.3082833333333));
#262307=CARTESIAN_POINT('Ctrl Pts',(-44.5079524583208,-55.8067071952963,
-37.24995));
#262308=CARTESIAN_POINT('Ctrl Pts',(-45.4714029967,-55.8067071952963,-37.1916166666667));
#262309=CARTESIAN_POINT('Ctrl Pts',(-45.9531282658897,-56.6410798368225,
-37.1332833333334));
#262310=CARTESIAN_POINT('Ctrl Pts',(-46.4348535350793,-57.4754524783487,
-37.07495));
#262311=CARTESIAN_POINT('Ctrl Pts',(-45.9531282658897,-58.309825119875,
-37.0166166666667));
#262312=CARTESIAN_POINT('Ctrl Pts',(-45.8905850977848,-58.418153064699,
-37.0090431559831));
#262313=CARTESIAN_POINT('Ctrl Pts',(-45.8125914103809,-58.5159466035015,
-37.0009024189827));
#262314=CARTESIAN_POINT('Ctrl Pts',(-44.5079524583208,-59.5441932447742,
-53.2308875));
#262315=CARTESIAN_POINT('Ctrl Pts',(-43.3135644199415,-59.5441932447742,
-53.1725541666667));
#262316=CARTESIAN_POINT('Ctrl Pts',(-42.7163704007519,-58.5098228615615,
-53.1142208333334));
#262317=CARTESIAN_POINT('Ctrl Pts',(-42.1191763815623,-57.4754524783487,
-53.0558875000001));
#262318=CARTESIAN_POINT('Ctrl Pts',(-42.7163704007519,-56.4410820951361,
-52.9975541666667));
#262319=CARTESIAN_POINT('Ctrl Pts',(-43.3135644199415,-55.4067117119233,
-52.9392208333334));
#262320=CARTESIAN_POINT('Ctrl Pts',(-44.5079524583208,-55.4067117119234,
-52.8808875));
#262321=CARTESIAN_POINT('Ctrl Pts',(-45.7023404967,-55.4067117119233,-52.8225541666667));
#262322=CARTESIAN_POINT('Ctrl Pts',(-46.2995345158897,-56.4410820951361,
-52.7642208333334));
#262323=CARTESIAN_POINT('Ctrl Pts',(-46.8967285350793,-57.4754524783487,
-52.7058875));
#262324=CARTESIAN_POINT('Ctrl Pts',(-46.2995345158897,-58.5098228615615,
-52.6475541666667));
#262325=CARTESIAN_POINT('Ctrl Pts',(-45.7023404967,-59.5441932447742,-52.5892208333333));
#262326=CARTESIAN_POINT('Ctrl Pts',(-44.5079524583208,-59.5441932447742,
-52.5308875));
#262327=CARTESIAN_POINT('Ctrl Pts',(-43.3135644199415,-59.5441932447742,
-52.4725541666667));
#262328=CARTESIAN_POINT('Ctrl Pts',(-42.7163704007519,-58.5098228615615,
-52.4142208333334));
#262329=CARTESIAN_POINT('Ctrl Pts',(-42.1191763815623,-57.4754524783487,
-52.3558875000001));
#262330=CARTESIAN_POINT('Ctrl Pts',(-42.7163704007519,-56.4410820951361,
-52.2975541666667));
#262331=CARTESIAN_POINT('Ctrl Pts',(-43.3135644199415,-55.4067117119233,
-52.2392208333334));
#262332=CARTESIAN_POINT('Ctrl Pts',(-44.5079524583208,-55.4067117119234,
-52.1808875));
#262333=CARTESIAN_POINT('Ctrl Pts',(-45.7023404967,-55.4067117119233,-52.1225541666667));
#262334=CARTESIAN_POINT('Ctrl Pts',(-46.2995345158897,-56.4410820951361,
-52.0642208333334));
#262335=CARTESIAN_POINT('Ctrl Pts',(-46.8967285350793,-57.4754524783487,
-52.0058875));
#262336=CARTESIAN_POINT('Ctrl Pts',(-46.2995345158897,-58.5098228615615,
-51.9475541666667));
#262337=CARTESIAN_POINT('Ctrl Pts',(-45.7023404967,-59.5441932447742,-51.8892208333334));
#262338=CARTESIAN_POINT('Ctrl Pts',(-44.5079524583208,-59.5441932447742,
-51.8308875));
#262339=CARTESIAN_POINT('Ctrl Pts',(-43.3135644199415,-59.5441932447742,
-51.7725541666667));
#262340=CARTESIAN_POINT('Ctrl Pts',(-42.7163704007519,-58.5098228615615,
-51.7142208333334));
#262341=CARTESIAN_POINT('Ctrl Pts',(-42.1191763815623,-57.4754524783487,
-51.6558875));
#262342=CARTESIAN_POINT('Ctrl Pts',(-42.7163704007519,-56.4410820951361,
-51.5975541666667));
#262343=CARTESIAN_POINT('Ctrl Pts',(-43.3135644199415,-55.4067117119233,
-51.5392208333333));
#262344=CARTESIAN_POINT('Ctrl Pts',(-44.5079524583208,-55.4067117119234,
-51.4808875));
#262345=CARTESIAN_POINT('Ctrl Pts',(-45.7023404967,-55.4067117119233,-51.4225541666667));
#262346=CARTESIAN_POINT('Ctrl Pts',(-46.2995345158897,-56.4410820951361,
-51.3642208333334));
#262347=CARTESIAN_POINT('Ctrl Pts',(-46.8967285350793,-57.4754524783487,
-51.3058875));
#262348=CARTESIAN_POINT('Ctrl Pts',(-46.2995345158897,-58.5098228615615,
-51.2475541666667));
#262349=CARTESIAN_POINT('Ctrl Pts',(-45.7023404967,-59.5441932447742,-51.1892208333334));
#262350=CARTESIAN_POINT('Ctrl Pts',(-44.5079524583208,-59.5441932447742,
-51.1308875));
#262351=CARTESIAN_POINT('Ctrl Pts',(-43.3135644199415,-59.5441932447742,
-51.0725541666667));
#262352=CARTESIAN_POINT('Ctrl Pts',(-42.7163704007519,-58.5098228615615,
-51.0142208333334));
#262353=CARTESIAN_POINT('Ctrl Pts',(-42.1191763815623,-57.4754524783487,
-50.9558875));
#262354=CARTESIAN_POINT('Ctrl Pts',(-42.7163704007519,-56.4410820951361,
-50.8975541666667));
#262355=CARTESIAN_POINT('Ctrl Pts',(-43.3135644199415,-55.4067117119233,
-50.8392208333333));
#262356=CARTESIAN_POINT('Ctrl Pts',(-44.5079524583208,-55.4067117119234,
-50.7808875));
#262357=CARTESIAN_POINT('Ctrl Pts',(-45.7023404967,-55.4067117119233,-50.7225541666667));
#262358=CARTESIAN_POINT('Ctrl Pts',(-46.2995345158897,-56.4410820951361,
-50.6642208333333));
#262359=CARTESIAN_POINT('Ctrl Pts',(-46.8967285350793,-57.4754524783487,
-50.6058875));
#262360=CARTESIAN_POINT('Ctrl Pts',(-46.2995345158897,-58.5098228615615,
-50.5475541666667));
#262361=CARTESIAN_POINT('Ctrl Pts',(-45.7023404967,-59.5441932447742,-50.4892208333333));
#262362=CARTESIAN_POINT('Ctrl Pts',(-44.5079524583208,-59.5441932447742,
-50.4308875));
#262363=CARTESIAN_POINT('Ctrl Pts',(-43.3135644199415,-59.5441932447742,
-50.3725541666667));
#262364=CARTESIAN_POINT('Ctrl Pts',(-42.7163704007519,-58.5098228615615,
-50.3142208333334));
#262365=CARTESIAN_POINT('Ctrl Pts',(-42.1191763815623,-57.4754524783487,
-50.2558875));
#262366=CARTESIAN_POINT('Ctrl Pts',(-42.7163704007519,-56.4410820951361,
-50.1975541666667));
#262367=CARTESIAN_POINT('Ctrl Pts',(-43.3135644199415,-55.4067117119233,
-50.1392208333333));
#262368=CARTESIAN_POINT('Ctrl Pts',(-44.5079524583208,-55.4067117119234,
-50.0808875));
#262369=CARTESIAN_POINT('Ctrl Pts',(-45.7023404967,-55.4067117119233,-50.0225541666667));
#262370=CARTESIAN_POINT('Ctrl Pts',(-46.2995345158897,-56.4410820951361,
-49.9642208333334));
#262371=CARTESIAN_POINT('Ctrl Pts',(-46.8967285350793,-57.4754524783487,
-49.9058875));
#262372=CARTESIAN_POINT('Ctrl Pts',(-46.2995345158897,-58.5098228615615,
-49.8475541666667));
#262373=CARTESIAN_POINT('Ctrl Pts',(-45.7023404967,-59.5441932447742,-49.7892208333333));
#262374=CARTESIAN_POINT('Ctrl Pts',(-44.5079524583208,-59.5441932447742,
-49.7308875));
#262375=CARTESIAN_POINT('Ctrl Pts',(-43.3135644199415,-59.5441932447742,
-49.6725541666667));
#262376=CARTESIAN_POINT('Ctrl Pts',(-42.7163704007519,-58.5098228615615,
-49.6142208333334));
#262377=CARTESIAN_POINT('Ctrl Pts',(-42.1191763815623,-57.4754524783487,
-49.5558875));
#262378=CARTESIAN_POINT('Ctrl Pts',(-42.7163704007519,-56.4410820951361,
-49.4975541666667));
#262379=CARTESIAN_POINT('Ctrl Pts',(-43.3135644199415,-55.4067117119233,
-49.4392208333333));
#262380=CARTESIAN_POINT('Ctrl Pts',(-44.5079524583208,-55.4067117119234,
-49.3808875));
#262381=CARTESIAN_POINT('Ctrl Pts',(-45.7023404967,-55.4067117119233,-49.3225541666667));
#262382=CARTESIAN_POINT('Ctrl Pts',(-46.2995345158897,-56.4410820951361,
-49.2642208333334));
#262383=CARTESIAN_POINT('Ctrl Pts',(-46.8967285350793,-57.4754524783487,
-49.2058875));
#262384=CARTESIAN_POINT('Ctrl Pts',(-46.2995345158897,-58.5098228615615,
-49.1475541666667));
#262385=CARTESIAN_POINT('Ctrl Pts',(-45.7023404967,-59.5441932447742,-49.0892208333333));
#262386=CARTESIAN_POINT('Ctrl Pts',(-44.5079524583208,-59.5441932447742,
-49.0308875));
#262387=CARTESIAN_POINT('Ctrl Pts',(-43.3135644199415,-59.5441932447742,
-48.9725541666667));
#262388=CARTESIAN_POINT('Ctrl Pts',(-42.7163704007519,-58.5098228615615,
-48.9142208333334));
#262389=CARTESIAN_POINT('Ctrl Pts',(-42.1191763815623,-57.4754524783487,
-48.8558875));
#262390=CARTESIAN_POINT('Ctrl Pts',(-42.7163704007519,-56.4410820951361,
-48.7975541666667));
#262391=CARTESIAN_POINT('Ctrl Pts',(-43.3135644199415,-55.4067117119233,
-48.7392208333334));
#262392=CARTESIAN_POINT('Ctrl Pts',(-44.5079524583208,-55.4067117119234,
-48.6808875));
#262393=CARTESIAN_POINT('Ctrl Pts',(-45.7023404967,-55.4067117119233,-48.6225541666667));
#262394=CARTESIAN_POINT('Ctrl Pts',(-46.2995345158897,-56.4410820951361,
-48.5642208333334));
#262395=CARTESIAN_POINT('Ctrl Pts',(-46.8967285350793,-57.4754524783487,
-48.5058875));
#262396=CARTESIAN_POINT('Ctrl Pts',(-46.2995345158897,-58.5098228615615,
-48.4475541666667));
#262397=CARTESIAN_POINT('Ctrl Pts',(-45.7023404967,-59.5441932447742,-48.3892208333334));
#262398=CARTESIAN_POINT('Ctrl Pts',(-44.5079524583208,-59.5441932447742,
-48.3308875));
#262399=CARTESIAN_POINT('Ctrl Pts',(-43.3135644199415,-59.5441932447742,
-48.2725541666667));
#262400=CARTESIAN_POINT('Ctrl Pts',(-42.7163704007519,-58.5098228615615,
-48.2142208333334));
#262401=CARTESIAN_POINT('Ctrl Pts',(-42.1191763815623,-57.4754524783487,
-48.1558875));
#262402=CARTESIAN_POINT('Ctrl Pts',(-42.7163704007519,-56.4410820951361,
-48.0975541666667));
#262403=CARTESIAN_POINT('Ctrl Pts',(-43.3135644199415,-55.4067117119233,
-48.0392208333334));
#262404=CARTESIAN_POINT('Ctrl Pts',(-44.5079524583208,-55.4067117119234,
-47.9808875));
#262405=CARTESIAN_POINT('Ctrl Pts',(-45.7023404967,-55.4067117119233,-47.9225541666667));
#262406=CARTESIAN_POINT('Ctrl Pts',(-46.2995345158897,-56.4410820951361,
-47.8642208333334));
#262407=CARTESIAN_POINT('Ctrl Pts',(-46.8967285350793,-57.4754524783487,
-47.8058875000001));
#262408=CARTESIAN_POINT('Ctrl Pts',(-46.2995345158897,-58.5098228615615,
-47.7475541666667));
#262409=CARTESIAN_POINT('Ctrl Pts',(-45.7023404967,-59.5441932447742,-47.6892208333334));
#262410=CARTESIAN_POINT('Ctrl Pts',(-44.5079524583208,-59.5441932447742,
-47.6308875));
#262411=CARTESIAN_POINT('Ctrl Pts',(-43.3135644199415,-59.5441932447742,
-47.5725541666667));
#262412=CARTESIAN_POINT('Ctrl Pts',(-42.7163704007519,-58.5098228615615,
-47.5142208333333));
#262413=CARTESIAN_POINT('Ctrl Pts',(-42.1191763815623,-57.4754524783487,
-47.4558875));
#262414=CARTESIAN_POINT('Ctrl Pts',(-42.7163704007519,-56.4410820951361,
-47.3975541666667));
#262415=CARTESIAN_POINT('Ctrl Pts',(-43.3135644199415,-55.4067117119233,
-47.3392208333334));
#262416=CARTESIAN_POINT('Ctrl Pts',(-44.5079524583208,-55.4067117119234,
-47.2808875));
#262417=CARTESIAN_POINT('Ctrl Pts',(-45.7023404967,-55.4067117119233,-47.2225541666667));
#262418=CARTESIAN_POINT('Ctrl Pts',(-46.2995345158897,-56.4410820951361,
-47.1642208333334));
#262419=CARTESIAN_POINT('Ctrl Pts',(-46.8967285350793,-57.4754524783487,
-47.1058875));
#262420=CARTESIAN_POINT('Ctrl Pts',(-46.2995345158897,-58.5098228615615,
-47.0475541666667));
#262421=CARTESIAN_POINT('Ctrl Pts',(-45.7023404967,-59.5441932447742,-46.9892208333334));
#262422=CARTESIAN_POINT('Ctrl Pts',(-44.5079524583208,-59.5441932447742,
-46.9308875));
#262423=CARTESIAN_POINT('Ctrl Pts',(-43.3135644199415,-59.5441932447742,
-46.8725541666667));
#262424=CARTESIAN_POINT('Ctrl Pts',(-42.7163704007519,-58.5098228615615,
-46.8142208333334));
#262425=CARTESIAN_POINT('Ctrl Pts',(-42.1191763815623,-57.4754524783487,
-46.7558875));
#262426=CARTESIAN_POINT('Ctrl Pts',(-42.7163704007519,-56.4410820951361,
-46.6975541666667));
#262427=CARTESIAN_POINT('Ctrl Pts',(-43.3135644199415,-55.4067117119233,
-46.6392208333334));
#262428=CARTESIAN_POINT('Ctrl Pts',(-44.5079524583208,-55.4067117119234,
-46.5808875));
#262429=CARTESIAN_POINT('Ctrl Pts',(-45.7023404967,-55.4067117119233,-46.5225541666667));
#262430=CARTESIAN_POINT('Ctrl Pts',(-46.2995345158897,-56.4410820951361,
-46.4642208333334));
#262431=CARTESIAN_POINT('Ctrl Pts',(-46.8967285350793,-57.4754524783487,
-46.4058875));
#262432=CARTESIAN_POINT('Ctrl Pts',(-46.2995345158897,-58.5098228615615,
-46.3475541666667));
#262433=CARTESIAN_POINT('Ctrl Pts',(-45.7023404967,-59.5441932447742,-46.2892208333334));
#262434=CARTESIAN_POINT('Ctrl Pts',(-44.5079524583208,-59.5441932447742,
-46.2308875));
#262435=CARTESIAN_POINT('Ctrl Pts',(-43.3135644199415,-59.5441932447742,
-46.1725541666667));
#262436=CARTESIAN_POINT('Ctrl Pts',(-42.7163704007519,-58.5098228615615,
-46.1142208333334));
#262437=CARTESIAN_POINT('Ctrl Pts',(-42.1191763815623,-57.4754524783487,
-46.0558875));
#262438=CARTESIAN_POINT('Ctrl Pts',(-42.7163704007519,-56.4410820951361,
-45.9975541666667));
#262439=CARTESIAN_POINT('Ctrl Pts',(-43.3135644199415,-55.4067117119233,
-45.9392208333333));
#262440=CARTESIAN_POINT('Ctrl Pts',(-44.5079524583208,-55.4067117119234,
-45.8808875));
#262441=CARTESIAN_POINT('Ctrl Pts',(-45.7023404967,-55.4067117119233,-45.8225541666667));
#262442=CARTESIAN_POINT('Ctrl Pts',(-46.2995345158897,-56.4410820951361,
-45.7642208333334));
#262443=CARTESIAN_POINT('Ctrl Pts',(-46.8967285350793,-57.4754524783487,
-45.7058875));
#262444=CARTESIAN_POINT('Ctrl Pts',(-46.2995345158897,-58.5098228615615,
-45.6475541666667));
#262445=CARTESIAN_POINT('Ctrl Pts',(-45.7023404967,-59.5441932447742,-45.5892208333334));
#262446=CARTESIAN_POINT('Ctrl Pts',(-44.5079524583208,-59.5441932447742,
-45.5308875));
#262447=CARTESIAN_POINT('Ctrl Pts',(-43.3135644199415,-59.5441932447742,
-45.4725541666667));
#262448=CARTESIAN_POINT('Ctrl Pts',(-42.7163704007519,-58.5098228615615,
-45.4142208333334));
#262449=CARTESIAN_POINT('Ctrl Pts',(-42.1191763815623,-57.4754524783487,
-45.3558875));
#262450=CARTESIAN_POINT('Ctrl Pts',(-42.7163704007519,-56.4410820951361,
-45.2975541666667));
#262451=CARTESIAN_POINT('Ctrl Pts',(-43.3135644199415,-55.4067117119233,
-45.2392208333333));
#262452=CARTESIAN_POINT('Ctrl Pts',(-44.5079524583208,-55.4067117119234,
-45.1808875));
#262453=CARTESIAN_POINT('Ctrl Pts',(-45.7023404967,-55.4067117119233,-45.1225541666667));
#262454=CARTESIAN_POINT('Ctrl Pts',(-46.2995345158897,-56.4410820951361,
-45.0642208333334));
#262455=CARTESIAN_POINT('Ctrl Pts',(-46.8967285350793,-57.4754524783487,
-45.0058875));
#262456=CARTESIAN_POINT('Ctrl Pts',(-46.2995345158897,-58.5098228615615,
-44.9475541666667));
#262457=CARTESIAN_POINT('Ctrl Pts',(-45.7023404967,-59.5441932447742,-44.8892208333333));
#262458=CARTESIAN_POINT('Ctrl Pts',(-44.5079524583208,-59.5441932447742,
-44.8308875));
#262459=CARTESIAN_POINT('Ctrl Pts',(-43.3135644199415,-59.5441932447742,
-44.7725541666667));
#262460=CARTESIAN_POINT('Ctrl Pts',(-42.7163704007519,-58.5098228615615,
-44.7142208333334));
#262461=CARTESIAN_POINT('Ctrl Pts',(-42.1191763815623,-57.4754524783487,
-44.6558875));
#262462=CARTESIAN_POINT('Ctrl Pts',(-42.7163704007519,-56.4410820951361,
-44.5975541666667));
#262463=CARTESIAN_POINT('Ctrl Pts',(-43.3135644199415,-55.4067117119233,
-44.5392208333333));
#262464=CARTESIAN_POINT('Ctrl Pts',(-44.5079524583208,-55.4067117119234,
-44.4808875000001));
#262465=CARTESIAN_POINT('Ctrl Pts',(-45.7023404967,-55.4067117119233,-44.4225541666667));
#262466=CARTESIAN_POINT('Ctrl Pts',(-46.2995345158897,-56.4410820951361,
-44.3642208333333));
#262467=CARTESIAN_POINT('Ctrl Pts',(-46.8967285350793,-57.4754524783487,
-44.3058875));
#262468=CARTESIAN_POINT('Ctrl Pts',(-46.2995345158897,-58.5098228615615,
-44.2475541666667));
#262469=CARTESIAN_POINT('Ctrl Pts',(-45.7023404967,-59.5441932447742,-44.1892208333334));
#262470=CARTESIAN_POINT('Ctrl Pts',(-44.5079524583208,-59.5441932447742,
-44.1308875000001));
#262471=CARTESIAN_POINT('Ctrl Pts',(-43.3135644199415,-59.5441932447742,
-44.0725541666667));
#262472=CARTESIAN_POINT('Ctrl Pts',(-42.7163704007519,-58.5098228615615,
-44.0142208333334));
#262473=CARTESIAN_POINT('Ctrl Pts',(-42.1191763815623,-57.4754524783487,
-43.9558875));
#262474=CARTESIAN_POINT('Ctrl Pts',(-42.7163704007519,-56.4410820951361,
-43.8975541666667));
#262475=CARTESIAN_POINT('Ctrl Pts',(-43.3135644199415,-55.4067117119233,
-43.8392208333333));
#262476=CARTESIAN_POINT('Ctrl Pts',(-44.5079524583208,-55.4067117119234,
-43.7808875));
#262477=CARTESIAN_POINT('Ctrl Pts',(-45.7023404967,-55.4067117119233,-43.7225541666667));
#262478=CARTESIAN_POINT('Ctrl Pts',(-46.2995345158897,-56.4410820951361,
-43.6642208333334));
#262479=CARTESIAN_POINT('Ctrl Pts',(-46.8967285350793,-57.4754524783487,
-43.6058875));
#262480=CARTESIAN_POINT('Ctrl Pts',(-46.2995345158897,-58.5098228615615,
-43.5475541666667));
#262481=CARTESIAN_POINT('Ctrl Pts',(-45.7023404967,-59.5441932447742,-43.4892208333333));
#262482=CARTESIAN_POINT('Ctrl Pts',(-44.5079524583208,-59.5441932447742,
-43.4308875));
#262483=CARTESIAN_POINT('Ctrl Pts',(-43.3135644199415,-59.5441932447742,
-43.3725541666667));
#262484=CARTESIAN_POINT('Ctrl Pts',(-42.7163704007519,-58.5098228615615,
-43.3142208333334));
#262485=CARTESIAN_POINT('Ctrl Pts',(-42.1191763815623,-57.4754524783487,
-43.2558875));
#262486=CARTESIAN_POINT('Ctrl Pts',(-42.7163704007519,-56.4410820951361,
-43.1975541666667));
#262487=CARTESIAN_POINT('Ctrl Pts',(-43.3135644199415,-55.4067117119233,
-43.1392208333334));
#262488=CARTESIAN_POINT('Ctrl Pts',(-44.5079524583208,-55.4067117119234,
-43.0808875));
#262489=CARTESIAN_POINT('Ctrl Pts',(-45.7023404967,-55.4067117119233,-43.0225541666667));
#262490=CARTESIAN_POINT('Ctrl Pts',(-46.2995345158897,-56.4410820951361,
-42.9642208333334));
#262491=CARTESIAN_POINT('Ctrl Pts',(-46.8967285350793,-57.4754524783487,
-42.9058875));
#262492=CARTESIAN_POINT('Ctrl Pts',(-46.2995345158897,-58.5098228615615,
-42.8475541666667));
#262493=CARTESIAN_POINT('Ctrl Pts',(-45.7023404967,-59.5441932447742,-42.7892208333334));
#262494=CARTESIAN_POINT('Ctrl Pts',(-44.5079524583208,-59.5441932447742,
-42.7308875000001));
#262495=CARTESIAN_POINT('Ctrl Pts',(-43.3135644199415,-59.5441932447742,
-42.6725541666667));
#262496=CARTESIAN_POINT('Ctrl Pts',(-42.7163704007519,-58.5098228615615,
-42.6142208333334));
#262497=CARTESIAN_POINT('Ctrl Pts',(-42.1191763815623,-57.4754524783487,
-42.5558875));
#262498=CARTESIAN_POINT('Ctrl Pts',(-42.7163704007519,-56.4410820951361,
-42.4975541666667));
#262499=CARTESIAN_POINT('Ctrl Pts',(-43.3135644199415,-55.4067117119233,
-42.4392208333334));
#262500=CARTESIAN_POINT('Ctrl Pts',(-44.5079524583208,-55.4067117119234,
-42.3808875000001));
#262501=CARTESIAN_POINT('Ctrl Pts',(-45.7023404967,-55.4067117119233,-42.3225541666667));
#262502=CARTESIAN_POINT('Ctrl Pts',(-46.2995345158897,-56.4410820951361,
-42.2642208333334));
#262503=CARTESIAN_POINT('Ctrl Pts',(-46.8967285350793,-57.4754524783487,
-42.2058875));
#262504=CARTESIAN_POINT('Ctrl Pts',(-46.2995345158897,-58.5098228615615,
-42.1475541666667));
#262505=CARTESIAN_POINT('Ctrl Pts',(-45.7023404967,-59.5441932447742,-42.0892208333334));
#262506=CARTESIAN_POINT('Ctrl Pts',(-44.5079524583208,-59.5441932447742,
-42.0308875000001));
#262507=CARTESIAN_POINT('Ctrl Pts',(-43.3135644199415,-59.5441932447742,
-41.9725541666667));
#262508=CARTESIAN_POINT('Ctrl Pts',(-42.7163704007519,-58.5098228615615,
-41.9142208333334));
#262509=CARTESIAN_POINT('Ctrl Pts',(-42.1191763815623,-57.4754524783487,
-41.8558875));
#262510=CARTESIAN_POINT('Ctrl Pts',(-42.7163704007519,-56.4410820951361,
-41.7975541666667));
#262511=CARTESIAN_POINT('Ctrl Pts',(-43.3135644199415,-55.4067117119233,
-41.7392208333334));
#262512=CARTESIAN_POINT('Ctrl Pts',(-44.5079524583208,-55.4067117119234,
-41.6808875000001));
#262513=CARTESIAN_POINT('Ctrl Pts',(-45.7023404967,-55.4067117119233,-41.6225541666667));
#262514=CARTESIAN_POINT('Ctrl Pts',(-46.2995345158897,-56.4410820951361,
-41.5642208333334));
#262515=CARTESIAN_POINT('Ctrl Pts',(-46.8967285350793,-57.4754524783487,
-41.5058875));
#262516=CARTESIAN_POINT('Ctrl Pts',(-46.2995345158897,-58.5098228615615,
-41.4475541666667));
#262517=CARTESIAN_POINT('Ctrl Pts',(-45.7023404967,-59.5441932447742,-41.3892208333334));
#262518=CARTESIAN_POINT('Ctrl Pts',(-44.5079524583208,-59.5441932447742,
-41.3308875000001));
#262519=CARTESIAN_POINT('Ctrl Pts',(-43.3135644199415,-59.5441932447742,
-41.2725541666667));
#262520=CARTESIAN_POINT('Ctrl Pts',(-42.7163704007519,-58.5098228615615,
-41.2142208333333));
#262521=CARTESIAN_POINT('Ctrl Pts',(-42.1191763815623,-57.4754524783487,
-41.1558875));
#262522=CARTESIAN_POINT('Ctrl Pts',(-42.7163704007519,-56.4410820951361,
-41.0975541666667));
#262523=CARTESIAN_POINT('Ctrl Pts',(-43.3135644199415,-55.4067117119233,
-41.0392208333333));
#262524=CARTESIAN_POINT('Ctrl Pts',(-44.5079524583208,-55.4067117119234,
-40.9808875000001));
#262525=CARTESIAN_POINT('Ctrl Pts',(-45.7023404967,-55.4067117119233,-40.9225541666667));
#262526=CARTESIAN_POINT('Ctrl Pts',(-46.2995345158897,-56.4410820951361,
-40.8642208333334));
#262527=CARTESIAN_POINT('Ctrl Pts',(-46.8967285350793,-57.4754524783487,
-40.8058875));
#262528=CARTESIAN_POINT('Ctrl Pts',(-46.2995345158897,-58.5098228615615,
-40.7475541666667));
#262529=CARTESIAN_POINT('Ctrl Pts',(-45.7023404967,-59.5441932447742,-40.6892208333333));
#262530=CARTESIAN_POINT('Ctrl Pts',(-44.5079524583208,-59.5441932447742,
-40.6308875));
#262531=CARTESIAN_POINT('Ctrl Pts',(-43.3135644199415,-59.5441932447742,
-40.5725541666667));
#262532=CARTESIAN_POINT('Ctrl Pts',(-42.7163704007519,-58.5098228615615,
-40.5142208333333));
#262533=CARTESIAN_POINT('Ctrl Pts',(-42.1191763815623,-57.4754524783487,
-40.4558875));
#262534=CARTESIAN_POINT('Ctrl Pts',(-42.7163704007519,-56.4410820951361,
-40.3975541666667));
#262535=CARTESIAN_POINT('Ctrl Pts',(-43.3135644199415,-55.4067117119233,
-40.3392208333333));
#262536=CARTESIAN_POINT('Ctrl Pts',(-44.5079524583208,-55.4067117119234,
-40.2808875));
#262537=CARTESIAN_POINT('Ctrl Pts',(-45.7023404967,-55.4067117119233,-40.2225541666667));
#262538=CARTESIAN_POINT('Ctrl Pts',(-46.2995345158897,-56.4410820951361,
-40.1642208333333));
#262539=CARTESIAN_POINT('Ctrl Pts',(-46.8967285350793,-57.4754524783487,
-40.1058875));
#262540=CARTESIAN_POINT('Ctrl Pts',(-46.2995345158897,-58.5098228615615,
-40.0475541666667));
#262541=CARTESIAN_POINT('Ctrl Pts',(-45.7023404967,-59.5441932447742,-39.9892208333333));
#262542=CARTESIAN_POINT('Ctrl Pts',(-44.5079524583208,-59.5441932447742,
-39.9308875));
#262543=CARTESIAN_POINT('Ctrl Pts',(-43.3135644199415,-59.5441932447742,
-39.8725541666667));
#262544=CARTESIAN_POINT('Ctrl Pts',(-42.7163704007519,-58.5098228615615,
-39.8142208333334));
#262545=CARTESIAN_POINT('Ctrl Pts',(-42.1191763815623,-57.4754524783487,
-39.7558875));
#262546=CARTESIAN_POINT('Ctrl Pts',(-42.7163704007519,-56.4410820951361,
-39.6975541666667));
#262547=CARTESIAN_POINT('Ctrl Pts',(-43.3135644199415,-55.4067117119233,
-39.6392208333334));
#262548=CARTESIAN_POINT('Ctrl Pts',(-44.5079524583208,-55.4067117119234,
-39.5808875000001));
#262549=CARTESIAN_POINT('Ctrl Pts',(-45.7023404967,-55.4067117119233,-39.5225541666667));
#262550=CARTESIAN_POINT('Ctrl Pts',(-46.2995345158897,-56.4410820951361,
-39.4642208333333));
#262551=CARTESIAN_POINT('Ctrl Pts',(-46.8967285350793,-57.4754524783487,
-39.4058875));
#262552=CARTESIAN_POINT('Ctrl Pts',(-46.2995345158897,-58.5098228615615,
-39.3475541666667));
#262553=CARTESIAN_POINT('Ctrl Pts',(-45.7023404967,-59.5441932447742,-39.2892208333334));
#262554=CARTESIAN_POINT('Ctrl Pts',(-44.5079524583208,-59.5441932447742,
-39.2308875));
#262555=CARTESIAN_POINT('Ctrl Pts',(-43.3135644199415,-59.5441932447742,
-39.1725541666667));
#262556=CARTESIAN_POINT('Ctrl Pts',(-42.7163704007519,-58.5098228615615,
-39.1142208333333));
#262557=CARTESIAN_POINT('Ctrl Pts',(-42.1191763815623,-57.4754524783487,
-39.0558875));
#262558=CARTESIAN_POINT('Ctrl Pts',(-42.7163704007519,-56.4410820951361,
-38.9975541666667));
#262559=CARTESIAN_POINT('Ctrl Pts',(-43.3135644199415,-55.4067117119233,
-38.9392208333334));
#262560=CARTESIAN_POINT('Ctrl Pts',(-44.5079524583208,-55.4067117119234,
-38.8808875));
#262561=CARTESIAN_POINT('Ctrl Pts',(-45.7023404967,-55.4067117119233,-38.8225541666667));
#262562=CARTESIAN_POINT('Ctrl Pts',(-46.2995345158897,-56.4410820951361,
-38.7642208333333));
#262563=CARTESIAN_POINT('Ctrl Pts',(-46.8967285350793,-57.4754524783487,
-38.7058875));
#262564=CARTESIAN_POINT('Ctrl Pts',(-46.2995345158897,-58.5098228615615,
-38.6475541666667));
#262565=CARTESIAN_POINT('Ctrl Pts',(-45.7023404967,-59.5441932447742,-38.5892208333334));
#262566=CARTESIAN_POINT('Ctrl Pts',(-44.5079524583208,-59.5441932447742,
-38.5308875));
#262567=CARTESIAN_POINT('Ctrl Pts',(-43.3135644199415,-59.5441932447742,
-38.4725541666667));
#262568=CARTESIAN_POINT('Ctrl Pts',(-42.7163704007519,-58.5098228615615,
-38.4142208333334));
#262569=CARTESIAN_POINT('Ctrl Pts',(-42.1191763815623,-57.4754524783487,
-38.3558875));
#262570=CARTESIAN_POINT('Ctrl Pts',(-42.7163704007519,-56.4410820951361,
-38.2975541666667));
#262571=CARTESIAN_POINT('Ctrl Pts',(-43.3135644199415,-55.4067117119233,
-38.2392208333333));
#262572=CARTESIAN_POINT('Ctrl Pts',(-44.5079524583208,-55.4067117119234,
-38.1808875000001));
#262573=CARTESIAN_POINT('Ctrl Pts',(-45.7023404967,-55.4067117119233,-38.1225541666667));
#262574=CARTESIAN_POINT('Ctrl Pts',(-46.2995345158897,-56.4410820951361,
-38.0642208333334));
#262575=CARTESIAN_POINT('Ctrl Pts',(-46.8967285350793,-57.4754524783487,
-38.0058875));
#262576=CARTESIAN_POINT('Ctrl Pts',(-46.2995345158897,-58.5098228615615,
-37.9475541666667));
#262577=CARTESIAN_POINT('Ctrl Pts',(-45.7023404967,-59.5441932447742,-37.8892208333334));
#262578=CARTESIAN_POINT('Ctrl Pts',(-44.5079524583208,-59.5441932447742,
-37.8308875));
#262579=CARTESIAN_POINT('Ctrl Pts',(-43.3135644199415,-59.5441932447742,
-37.7725541666667));
#262580=CARTESIAN_POINT('Ctrl Pts',(-42.7163704007519,-58.5098228615615,
-37.7142208333333));
#262581=CARTESIAN_POINT('Ctrl Pts',(-42.1191763815623,-57.4754524783487,
-37.6558875));
#262582=CARTESIAN_POINT('Ctrl Pts',(-42.7163704007519,-56.4410820951361,
-37.5975541666667));
#262583=CARTESIAN_POINT('Ctrl Pts',(-43.3135644199415,-55.4067117119233,
-37.5392208333334));
#262584=CARTESIAN_POINT('Ctrl Pts',(-44.5079524583208,-55.4067117119234,
-37.4808875));
#262585=CARTESIAN_POINT('Ctrl Pts',(-45.7023404967,-55.4067117119233,-37.4225541666667));
#262586=CARTESIAN_POINT('Ctrl Pts',(-46.2995345158897,-56.4410820951361,
-37.3642208333333));
#262587=CARTESIAN_POINT('Ctrl Pts',(-46.8967285350793,-57.4754524783487,
-37.3058875));
#262588=CARTESIAN_POINT('Ctrl Pts',(-46.2995345158897,-58.5098228615615,
-37.2475541666667));
#262589=CARTESIAN_POINT('Ctrl Pts',(-46.2219998538691,-58.6441168355289,
-37.239980655983));
#262590=CARTESIAN_POINT('Ctrl Pts',(-46.1253112086366,-58.7653513237809,
-37.2318399189827));
#262591=CARTESIAN_POINT('Ctrl Pts',(-44.5079524583208,-55.8067071952963,
-52.64995));
#262592=CARTESIAN_POINT('Ctrl Pts',(-44.6656844499352,-55.7901659658991,
-52.64995));
#262593=CARTESIAN_POINT('Ctrl Pts',(-44.8248930522219,-55.7949712964571,
-52.64995));
#262594=CARTESIAN_POINT('Ctrl Pts',(-45.1318235221455,-55.8461574375238,
-52.64995));
#262595=CARTESIAN_POINT('Ctrl Pts',(-45.2783921862421,-55.8907287079161,
-52.64995));
#262596=CARTESIAN_POINT('Ctrl Pts',(-45.613660160206,-56.0425368373591,
-52.64995));
#262597=CARTESIAN_POINT('Ctrl Pts',(-45.7919027673255,-56.1667049718845,
-52.64995));
#262598=CARTESIAN_POINT('Ctrl Pts',(-46.1429583138082,-56.5217933658313,
-52.64995));
#262599=CARTESIAN_POINT('Ctrl Pts',(-46.2637964187606,-56.7417269487201,
-52.64995));
#262600=CARTESIAN_POINT('Ctrl Pts',(-46.392133099223,-57.0470088534789,
-52.64995));
#262601=CARTESIAN_POINT('Ctrl Pts',(-46.4329712831928,-57.1844772022895,
-52.64995));
#262602=CARTESIAN_POINT('Ctrl Pts',(-46.4841685595404,-57.4666010630848,
-52.64995));
#262603=CARTESIAN_POINT('Ctrl Pts',(-46.4942078616446,-57.6104009645534,
-52.64995));
#262604=CARTESIAN_POINT('Ctrl Pts',(-46.4884569292041,-57.7540239068882,
-52.64995));
#262605=CARTESIAN_POINT('Origin',(44.5079524583206,-57.475452478349,235.35105));
#262606=CARTESIAN_POINT('',(45.1065281918136,-55.5671267379762,-39.2098669225693));
#262607=CARTESIAN_POINT('Ctrl Pts',(44.1169605019967,-55.5140434720247,
-38.9933921946761));
#262608=CARTESIAN_POINT('Ctrl Pts',(44.2022887299052,-55.4970339392592,
-39.0076769808271));
#262609=CARTESIAN_POINT('Ctrl Pts',(44.2884091944078,-55.4856555995933,
-39.023286029138));
#262610=CARTESIAN_POINT('Ctrl Pts',(44.4991063316471,-55.4715934716373,
-39.0642737523148));
#262611=CARTESIAN_POINT('Ctrl Pts',(44.6234934076874,-55.4749641540851,
-39.0908460389324));
#262612=CARTESIAN_POINT('Ctrl Pts',(44.8688808688308,-55.504420058799,-39.1478511670598));
#262613=CARTESIAN_POINT('Ctrl Pts',(44.9894084334508,-55.5303903344848,
-39.1781481007446));
#262614=CARTESIAN_POINT('Ctrl Pts',(45.106528182368,-55.567126745519,-39.2098669533806));
#262615=CARTESIAN_POINT('',(42.5264426591671,-57.204124658128,-39.0141963127215));
#262616=CARTESIAN_POINT('Ctrl Pts',(42.8346993804887,-56.3799036982206,
-38.9060738903536));
#262617=CARTESIAN_POINT('Ctrl Pts',(42.8191079311706,-56.4037152169138,
-38.9078025937102));
#262618=CARTESIAN_POINT('Ctrl Pts',(42.8039043779996,-56.4280492827628,
-38.9097224693021));
#262619=CARTESIAN_POINT('Ctrl Pts',(42.7891466755666,-56.4528544726931,
-38.9118346780871));
#262620=CARTESIAN_POINT('Ctrl Pts',(42.7721187707309,-56.4814754870741,
-38.9142718115331));
#262621=CARTESIAN_POINT('Ctrl Pts',(42.7558136628821,-56.5105053677241,
-38.9169462637683));
#262622=CARTESIAN_POINT('Ctrl Pts',(42.7402073536177,-56.5399968434849,
-38.9198636917123));
#262623=CARTESIAN_POINT('Ctrl Pts',(42.7247612337211,-56.5691856070041,
-38.922751174015));
#262624=CARTESIAN_POINT('Ctrl Pts',(42.7100090032885,-56.5988107367616,
-38.9258753161839));
#262625=CARTESIAN_POINT('Ctrl Pts',(42.6959610908403,-56.6288786279515,
-38.9292392096901));
#262626=CARTESIAN_POINT('Ctrl Pts',(42.6820564045184,-56.6586399605976,
-38.932568806468));
#262627=CARTESIAN_POINT('Ctrl Pts',(42.6688417582775,-56.688835076219,-38.9361332943689));
#262628=CARTESIAN_POINT('Ctrl Pts',(42.6563331490267,-56.719472363895,-38.9399372898989));
#262629=CARTESIAN_POINT('Ctrl Pts',(42.6439511930279,-56.7497994402564,
-38.9437027688844));
#262630=CARTESIAN_POINT('Ctrl Pts',(42.6322610361143,-56.7805597750077,
-38.9477029270453));
#262631=CARTESIAN_POINT('Ctrl Pts',(42.6212841673493,-56.8117637261139,
-38.9519438796553));
#262632=CARTESIAN_POINT('Ctrl Pts',(42.610417657956,-56.8426539585708,-38.9561421945263));
#262633=CARTESIAN_POINT('Ctrl Pts',(42.6002501306032,-56.8739789188314,
-38.9605764771568));
#262634=CARTESIAN_POINT('Ctrl Pts',(42.5908086952621,-56.9057509847877,
-38.9652543723165));
#262635=CARTESIAN_POINT('Ctrl Pts',(42.5814614976865,-56.9372059243332,
-38.9698855760176));
#262636=CARTESIAN_POINT('Ctrl Pts',(42.5728249837433,-56.9691068258,-38.9747569641089));
#262637=CARTESIAN_POINT('Ctrl Pts',(42.5649349981973,-57.0014449365778,
-38.9798735188755));
#262638=CARTESIAN_POINT('Ctrl Pts',(42.5571231858622,-57.0334626444927,
-38.9849393793142));
#262639=CARTESIAN_POINT('Ctrl Pts',(42.5500285451438,-57.0660123389163,
-38.9902641114435));
#262640=CARTESIAN_POINT('Ctrl Pts',(42.543771399786,-57.0986331989938,-38.9957757940657));
#262641=CARTESIAN_POINT('Ctrl Pts',(42.5370689667629,-57.1335755117135,
-39.001679713746));
#262642=CARTESIAN_POINT('Ctrl Pts',(42.5312861876561,-57.1687524789562,
-39.007821532343));
#262643=CARTESIAN_POINT('Ctrl Pts',(42.5264426092999,-57.2041247208502,
-39.0141962424421));
#262644=CARTESIAN_POINT('Ctrl Pts',(42.5264426283417,-57.2041246439921,
-39.0141962764686));
#262645=CARTESIAN_POINT('Ctrl Pts',(42.5450760563286,-57.0680445370257,
-39.0216142665105));
#262646=CARTESIAN_POINT('Ctrl Pts',(42.5776734710537,-56.9342676048075,
-39.0293231873749));
#262647=CARTESIAN_POINT('Ctrl Pts',(42.6706416925213,-56.6730323503409,
-39.0452318818938));
#262648=CARTESIAN_POINT('Ctrl Pts',(42.7312783272647,-56.5464660127888,
-39.0533943474495));
#262649=CARTESIAN_POINT('Ctrl Pts',(42.9435983774129,-56.201438833693,-39.0770171498676));
#262650=CARTESIAN_POINT('Ctrl Pts',(43.1261253028118,-56.0054501928792,
-39.0922418351299));
#262651=CARTESIAN_POINT('Ctrl Pts',(43.5474287173053,-55.7029969267937,
-39.1198092304128));
#262652=CARTESIAN_POINT('Ctrl Pts',(43.7794584498512,-55.5956854299055,
-39.1324545161726));
#262653=CARTESIAN_POINT('Ctrl Pts',(44.278976126795,-55.4714954972292,-39.1615930473276));
#262654=CARTESIAN_POINT('Ctrl Pts',(44.5424550156973,-55.4587534023231,
-39.1769626491803));
#262655=CARTESIAN_POINT('Ctrl Pts',(44.904456701214,-55.5123578192425,-39.1980794141687));
#262656=CARTESIAN_POINT('Ctrl Pts',(45.0066424797803,-55.5357960578388,
-39.2040402512518));
#262657=CARTESIAN_POINT('Ctrl Pts',(45.1065281894683,-55.5671267477461,
-39.2098669176502));
#262658=CARTESIAN_POINT('Origin',(44.5079524583206,-57.475452478349,235.35105));
#262659=CARTESIAN_POINT('Ctrl Pts',(44.5079524583206,-59.475452478349,-40.22495));
#262660=CARTESIAN_POINT('Ctrl Pts',(44.3134064919888,-59.475452478349,-40.2362985147027));
#262661=CARTESIAN_POINT('Ctrl Pts',(44.1195072893019,-59.4470642229361,
-40.2476093015263));
#262662=CARTESIAN_POINT('Ctrl Pts',(43.6856583461661,-59.3167143014365,
-40.2729171565426));
#262663=CARTESIAN_POINT('Ctrl Pts',(43.4555514926831,-59.1955857510714,
-40.2854137466271));
#262664=CARTESIAN_POINT('Ctrl Pts',(43.0536254671757,-58.8724196322647,
-40.3134623430353));
#262665=CARTESIAN_POINT('Ctrl Pts',(42.8857301827636,-58.6733468203936,
-40.3284160787138));
#262666=CARTESIAN_POINT('Ctrl Pts',(42.6313500986315,-58.2161860031401,
-40.3589304159134));
#262667=CARTESIAN_POINT('Ctrl Pts',(42.5497586678929,-57.961082232183,-40.3741975361746));
#262668=CARTESIAN_POINT('Ctrl Pts',(42.4921679449883,-57.4454909452804,
-40.4019239828176));
#262669=CARTESIAN_POINT('Ctrl Pts',(42.5121837301983,-57.1904786222485,
-40.4144697636932));
#262670=CARTESIAN_POINT('Ctrl Pts',(42.6484151609807,-56.6942789617644,
-40.4435102685851));
#262671=CARTESIAN_POINT('Ctrl Pts',(42.7661045739579,-56.4585617254506,
-40.4588508748245));
#262672=CARTESIAN_POINT('Ctrl Pts',(43.0879308195211,-56.042323041325,-40.489265081332));
#262673=CARTESIAN_POINT('Ctrl Pts',(43.2901830524831,-55.8669604384183,
-40.5039134513263));
#262674=CARTESIAN_POINT('Ctrl Pts',(43.7417978374699,-55.6105947638857,
-40.5302576471172));
#262675=CARTESIAN_POINT('Ctrl Pts',(43.9848712519941,-55.5283968064006,
-40.5444369296311));
#262676=CARTESIAN_POINT('Ctrl Pts',(44.4984615764082,-55.4581084733143,
-40.5743963652219));
#262677=CARTESIAN_POINT('Ctrl Pts',(44.7646876495702,-55.4744865525067,
-40.5899262194896));
#262678=CARTESIAN_POINT('Ctrl Pts',(45.2710162925252,-55.6085985558055,
-40.6194620569953));
#262679=CARTESIAN_POINT('Ctrl Pts',(45.5066033452955,-55.7232847031097,
-40.6322277122423));
#262680=CARTESIAN_POINT('Ctrl Pts',(45.918984247136,-56.034904349389,-40.659997936129));
#262681=CARTESIAN_POINT('Ctrl Pts',(46.0923733852973,-56.2281484516539,
-40.6748174535908));
#262682=CARTESIAN_POINT('Ctrl Pts',(46.361658910303,-56.6784022072892,-40.705417600851));
#262683=CARTESIAN_POINT('Ctrl Pts',(46.4515224045839,-56.9331562661353,
-40.7209083228238));
#262684=CARTESIAN_POINT('Ctrl Pts',(46.5238640803581,-57.4496948924172,
-40.7491128634236));
#262685=CARTESIAN_POINT('Ctrl Pts',(46.5108390657226,-57.705708271998,-40.7614979036731));
#262686=CARTESIAN_POINT('Ctrl Pts',(46.3881487371309,-58.2052515427372,
-40.7903123727508));
#262687=CARTESIAN_POINT('Ctrl Pts',(46.2773227653104,-58.4434704448938,
-40.8055791748165));
#262688=CARTESIAN_POINT('Ctrl Pts',(45.9678438328221,-58.8679200514476,
-40.8360480519584));
#262689=CARTESIAN_POINT('Ctrl Pts',(45.7706383033074,-59.0489592653161,
-40.8509456458029));
#262690=CARTESIAN_POINT('Ctrl Pts',(45.3269190694736,-59.3176237716168,
-40.8774598902303));
#262691=CARTESIAN_POINT('Ctrl Pts',(45.0869234570947,-59.4065609629546,
-40.8911766917383));
#262692=CARTESIAN_POINT('Ctrl Pts',(44.7277496182526,-59.4664001015449,
-40.9121284990041));
#262693=CARTESIAN_POINT('Ctrl Pts',(44.6178162529024,-59.475452478349,-40.9185412786495));
#262694=CARTESIAN_POINT('Ctrl Pts',(44.5079524583206,-59.475452478349,-40.9249500000001));
#262695=CARTESIAN_POINT('Ctrl Pts',(44.5079524583207,-59.475452478349,-40.7662));
#262696=CARTESIAN_POINT('Ctrl Pts',(44.5083775298429,-59.475452478349,-40.7661752041612));
#262697=CARTESIAN_POINT('Ctrl Pts',(44.5088026080816,-59.4754523428346,
-40.7661504079305));
#262698=CARTESIAN_POINT('Ctrl Pts',(44.7668034260579,-59.4752878370093,
-40.7511003602152));
#262699=CARTESIAN_POINT('Ctrl Pts',(45.0219684864269,-59.4253661652626,
-40.7362157316937));
#262700=CARTESIAN_POINT('Ctrl Pts',(45.500302270728,-59.2310567042668,-40.7083129276095));
#262701=CARTESIAN_POINT('Ctrl Pts',(45.7187606546021,-59.0881700738478,
-40.6956896013403));
#262702=CARTESIAN_POINT('Ctrl Pts',(46.0934420241406,-58.7229365286537,
-40.6663104722357));
#262703=CARTESIAN_POINT('Ctrl Pts',(46.2443678867435,-58.5025073402031,
-40.650772793422));
#262704=CARTESIAN_POINT('Ctrl Pts',(46.4477890250889,-58.0248714647437,
-40.6207103967757));
#262705=CARTESIAN_POINT('Ctrl Pts',(46.5019285880958,-57.7736673579108,
-40.6064409598016));
#262706=CARTESIAN_POINT('Ctrl Pts',(46.5132520993636,-57.2540501555927,
-40.579860591705));
#262707=CARTESIAN_POINT('Ctrl Pts',(46.4663000604843,-56.9904652730994,
-40.5654844827148));
#262708=CARTESIAN_POINT('Ctrl Pts',(46.273636796699,-56.5004392710753,-40.5351099311555));
#262709=CARTESIAN_POINT('Ctrl Pts',(46.1312667756054,-56.2783098828283,
-40.5197359067732));
#262710=CARTESIAN_POINT('Ctrl Pts',(45.7746433882416,-55.9071055070085,
-40.4905818335068));
#262711=CARTESIAN_POINT('Ctrl Pts',(45.5659936742326,-55.7594271642448,
-40.4779190709282));
#262712=CARTESIAN_POINT('Ctrl Pts',(45.093845544046,-55.5448874669513,-40.4503770966673));
#262713=CARTESIAN_POINT('Ctrl Pts',(44.8329702931349,-55.4843029305355,
-40.4351593736975));
#262714=CARTESIAN_POINT('Ctrl Pts',(44.3097029112295,-55.4686054722672,
-40.4046354430863));
#262715=CARTESIAN_POINT('Ctrl Pts',(44.0523852487196,-55.51096207822,-40.3896252461066));
#262716=CARTESIAN_POINT('Ctrl Pts',(43.5694318290431,-55.6907401383014,
-40.3614529632921));
#262717=CARTESIAN_POINT('Ctrl Pts',(43.3481921407017,-55.8259134639983,
-40.3490386477088));
#262718=CARTESIAN_POINT('Ctrl Pts',(42.9626483577539,-56.1783496732344,
-40.3199891959321));
#262719=CARTESIAN_POINT('Ctrl Pts',(42.8043598248836,-56.39462241756,-40.3044467484306));
#262720=CARTESIAN_POINT('Ctrl Pts',(42.585649810967,-56.8672048416347,-40.2741937172546));
#262721=CARTESIAN_POINT('Ctrl Pts',(42.5237503418946,-57.1174066419007,
-40.259748584359));
#262722=CARTESIAN_POINT('Ctrl Pts',(42.4969324210317,-57.6377858849942,
-40.2326777990934));
#262723=CARTESIAN_POINT('Ctrl Pts',(42.5362357228956,-57.9031746362469,
-40.2187673399372));
#262724=CARTESIAN_POINT('Ctrl Pts',(42.7150872537481,-58.3997422547582,
-40.1884651602349));
#262725=CARTESIAN_POINT('Ctrl Pts',(42.8514932711515,-58.6264621509445,
-40.1730331819982));
#262726=CARTESIAN_POINT('Ctrl Pts',(43.1980642286301,-59.007884642095,-40.1436561043353));
#262727=CARTESIAN_POINT('Ctrl Pts',(43.4024115098283,-59.1612444110393,
-40.1306898886619));
#262728=CARTESIAN_POINT('Ctrl Pts',(43.868198574263,-59.3888396055522,-40.1035189765699));
#262729=CARTESIAN_POINT('Ctrl Pts',(44.127238048215,-59.4567017443637,-40.0884083405893));
#262730=CARTESIAN_POINT('Ctrl Pts',(44.4305845724308,-59.4743307533407,
-40.0707131266768));
#262731=CARTESIAN_POINT('Ctrl Pts',(44.4692789444141,-59.475452478349,-40.0684559549778));
#262732=CARTESIAN_POINT('Ctrl Pts',(44.5079524583206,-59.475452478349,-40.0662));
#262733=CARTESIAN_POINT('Ctrl Pts',(43.4805771074156,-59.5712767529309,
-39.2399080357013));
#262734=CARTESIAN_POINT('Ctrl Pts',(43.4150727209207,-59.5358440364426,
-39.2223070534893));
#262735=CARTESIAN_POINT('Ctrl Pts',(43.2883193276586,-59.4590682572254,
-39.1867578392588));
#262736=CARTESIAN_POINT('Ctrl Pts',(43.1106712693135,-59.32658002426,-39.1324031814995));
#262737=CARTESIAN_POINT('Ctrl Pts',(43.0005921597408,-59.2266373021163,
-39.0954660506179));
#262738=CARTESIAN_POINT('Ctrl Pts',(42.8948534568781,-59.1207134074407,
-39.0581733199915));
#262739=CARTESIAN_POINT('Ctrl Pts',(42.7951360401793,-59.0104958554849,
-39.0211184761739));
#262740=CARTESIAN_POINT('Ctrl Pts',(42.6850011896347,-58.8622904152127,
-38.9753582681256));
#262741=CARTESIAN_POINT('Ctrl Pts',(42.6055727997797,-58.7375004045667,
-38.939089851323));
#262742=CARTESIAN_POINT('Ctrl Pts',(42.5503788594446,-58.6407591922129,
-38.9120596161462));
#262743=CARTESIAN_POINT('Ctrl Pts',(42.5165536369311,-58.5741539171446,
-38.8941613358138));
#262744=CARTESIAN_POINT('Ctrl Pts',(42.4842288567228,-58.5064298632496,
-38.8763157156907));
#262745=CARTESIAN_POINT('Ctrl Pts',(42.4689425396028,-58.4722695523732,
-38.8674882509199));
#262746=CARTESIAN_POINT('Ctrl Pts',(42.4257123024776,-58.3690064948315,
-38.8413136266604));
#262747=CARTESIAN_POINT('Ctrl Pts',(42.3750272156063,-58.229152189777,-38.8072100415055));
#262748=CARTESIAN_POINT('Ctrl Pts',(42.3380647902547,-58.0850119200902,
-38.7746901633276));
#262749=CARTESIAN_POINT('Ctrl Pts',(42.3155659796374,-57.9752818499468,
-38.7509105250088));
#262750=CARTESIAN_POINT('Ctrl Pts',(42.3089374211558,-57.9384266221928,
-38.7430843922672));
#262751=CARTESIAN_POINT('Ctrl Pts',(42.297458012674,-57.864178756387,-38.7276438637217));
#262752=CARTESIAN_POINT('Ctrl Pts',(42.292601515188,-57.8267325312259,-38.720018782004));
#262753=CARTESIAN_POINT('Ctrl Pts',(42.2847289916893,-57.7514526301959,
-38.7050196673963));
#262754=CARTESIAN_POINT('Ctrl Pts',(42.2817363521424,-57.7138759968928,
-38.6976962453237));
#262755=CARTESIAN_POINT('Ctrl Pts',(42.277596992864,-57.6387184974263,-38.6833720377019));
#262756=CARTESIAN_POINT('Ctrl Pts',(42.2741651307842,-57.5260409596698,
-38.6623829091612));
#262757=CARTESIAN_POINT('Ctrl Pts',(42.2805893100654,-57.3760354719141,
-38.6363740800325));
#262758=CARTESIAN_POINT('Ctrl Pts',(42.2937061680812,-57.2637038035873,
-38.618370061439));
#262759=CARTESIAN_POINT('Ctrl Pts',(42.3043247017591,-57.1888547452426,
-38.6067079534822));
#262760=CARTESIAN_POINT('Ctrl Pts',(42.3105743117123,-57.1514345461221,
-38.6010450635964));
#262761=CARTESIAN_POINT('Ctrl Pts',(42.3249704170347,-57.0766935209607,
-38.590076215021));
#262762=CARTESIAN_POINT('Ctrl Pts',(42.3331592025312,-57.0392159768686,
-38.5847494243559));
#262763=CARTESIAN_POINT('Ctrl Pts',(42.3512949844302,-56.9651221381903,
-38.5745673038812));
#262764=CARTESIAN_POINT('Ctrl Pts',(42.3712216906218,-56.8916587034686,
-38.564820665347));
#262765=CARTESIAN_POINT('Ctrl Pts',(42.4063979707918,-56.7834465224234,
-38.5515118436));
#262766=CARTESIAN_POINT('Ctrl Pts',(42.4468320479729,-56.6771725078319,
-38.5395042677724));
#262767=CARTESIAN_POINT('Ctrl Pts',(42.4925290654744,-56.5728473165674,
-38.5288039137004));
#262768=CARTESIAN_POINT('Ctrl Pts',(42.5265325119253,-56.5046058456765,
-38.5225509073062));
#262769=CARTESIAN_POINT('Ctrl Pts',(42.5623338475306,-56.4370293947697,
-38.5167461666044));
#262770=CARTESIAN_POINT('Ctrl Pts',(42.5811223641794,-56.4035923099625,
-38.5140693065785));
#262771=CARTESIAN_POINT('Ctrl Pts',(42.620584523009,-56.3373241998654,-38.5091697400817));
#262772=CARTESIAN_POINT('Ctrl Pts',(42.6411082254821,-56.3047465904101,
-38.5069659500128));
#262773=CARTESIAN_POINT('Ctrl Pts',(42.7048067991197,-56.2090283357163,
-38.501110858935));
#262774=CARTESIAN_POINT('Ctrl Pts',(42.7502234543428,-56.1476408662828,
-38.4981890389281));
#262775=CARTESIAN_POINT('Ctrl Pts',(42.8467942323831,-56.0297655581676,
-38.4942910511033));
#262776=CARTESIAN_POINT('Ctrl Pts',(42.8979715413934,-55.9732420482176,
-38.4933125989996));
#262777=CARTESIAN_POINT('Ctrl Pts',(42.9790570553347,-55.8921695883033,
-38.4933149859729));
#262778=CARTESIAN_POINT('Ctrl Pts',(43.0068374106561,-55.8657400908868,
-38.4935622007431));
#262779=CARTESIAN_POINT('Ctrl Pts',(43.0495800649421,-55.8270637749536,
-38.4943063068789));
#262780=CARTESIAN_POINT('Ctrl Pts',(43.0640222060113,-55.8143203511958,
-38.494617152342));
#262781=CARTESIAN_POINT('Ctrl Pts',(43.0932714774893,-55.7891564261061,
-38.4953646906773));
#262782=CARTESIAN_POINT('Ctrl Pts',(43.1080901283632,-55.7767277938553,
-38.4958020036096));
#262783=CARTESIAN_POINT('Ctrl Pts',(43.1528523310046,-55.7401327167866,
-38.4972962980169));
#262784=CARTESIAN_POINT('Ctrl Pts',(43.2134913856688,-55.6930468850421,
-38.4997758707861));
#262785=CARTESIAN_POINT('Ctrl Pts',(43.3385569247743,-55.6055389451161,
-38.5066450244003));
#262786=CARTESIAN_POINT('Ctrl Pts',(43.4691986576013,-55.5278792007279,
-38.5163302992824));
#262787=CARTESIAN_POINT('Ctrl Pts',(43.5713395927684,-55.4769743237494,
-38.5256877381308));
#262788=CARTESIAN_POINT('Ctrl Pts',(43.6403672861995,-55.4446857735354,
-38.5323951500278));
#262789=CARTESIAN_POINT('Ctrl Pts',(43.6753577685123,-55.4293620157832,
-38.5359845633874));
#262790=CARTESIAN_POINT('Ctrl Pts',(43.7462462065788,-55.4003985583156,
-38.5436333065981));
#262791=CARTESIAN_POINT('Ctrl Pts',(43.7822717759725,-55.3867204456352,
-38.5477088862383));
#262792=CARTESIAN_POINT('Ctrl Pts',(43.8543821738219,-55.3613797848081,
-38.5562346427694));
#262793=CARTESIAN_POINT('Ctrl Pts',(43.890622407919,-55.349649082917,-38.5607007444526));
#262794=CARTESIAN_POINT('Ctrl Pts',(43.9997560709039,-55.3172704656441,
-38.5746802407103));
#262795=CARTESIAN_POINT('Ctrl Pts',(44.1098017310836,-55.290468361793,-38.5898286859852));
#262796=CARTESIAN_POINT('Ctrl Pts',(44.2583166685835,-55.2656490138239,
-38.612301023075));
#262797=CARTESIAN_POINT('Ctrl Pts',(44.3705972700495,-55.2524997368729,
-38.6302900391873));
#262798=CARTESIAN_POINT('Ctrl Pts',(44.446056048267,-55.2474029004138,-38.6430428201589));
#262799=CARTESIAN_POINT('Ctrl Pts',(44.5218128020516,-55.2441636366351,
-38.65617756452));
#262800=CARTESIAN_POINT('Ctrl Pts',(44.5599089424743,-55.2434808562086,
-38.6629497802385));
#262801=CARTESIAN_POINT('Ctrl Pts',(44.6354869543582,-55.2439911084578,
-38.6767130108817));
#262802=CARTESIAN_POINT('Ctrl Pts',(44.6731456892459,-55.2451740103824,
-38.6837342374529));
#262803=CARTESIAN_POINT('Ctrl Pts',(44.7481014788608,-55.2493620066237,
-38.6980304684339));
#262804=CARTESIAN_POINT('Ctrl Pts',(44.860046548974,-55.2583760573225,-38.7198650218829));
#262805=CARTESIAN_POINT('Ctrl Pts',(45.0073845433675,-55.2811507310277,
-38.7505067688753));
#262806=CARTESIAN_POINT('Ctrl Pts',(45.1528189888476,-55.3146135839333,
-38.7826550300594));
#262807=CARTESIAN_POINT('Ctrl Pts',(45.2248832056965,-55.3349380951144,
-38.7992310848652));
#262808=CARTESIAN_POINT('Ctrl Pts',(45.2966462681613,-55.3570913336823,
-38.8160672125853));
#262809=CARTESIAN_POINT('Ctrl Pts',(45.3323638946335,-55.3690863290504,
-38.8246135819642));
#262810=CARTESIAN_POINT('Ctrl Pts',(45.4027951436545,-55.3946744461232,
-38.841798196801));
#262811=CARTESIAN_POINT('Ctrl Pts',(45.4376370321487,-55.4083060218429,
-38.85046633842));
#262812=CARTESIAN_POINT('Ctrl Pts',(45.5409345111852,-55.4516493275196,
-38.8766665754573));
#262813=CARTESIAN_POINT('Ctrl Pts',(45.6082182891413,-55.4838201174091,
-38.8944064774514));
#262814=CARTESIAN_POINT('Ctrl Pts',(45.7067749877369,-55.5369855856676,
-38.9214216121435));
#262815=CARTESIAN_POINT('Ctrl Pts',(45.7392219877795,-55.5555212114618,
-38.9304915704334));
#262816=CARTESIAN_POINT('Ctrl Pts',(45.8033556832395,-55.5942722159849,
-38.9487787872477));
#262817=CARTESIAN_POINT('Ctrl Pts',(45.8348443691401,-55.6143675312756,
-38.9579395118015));
#262818=CARTESIAN_POINT('Ctrl Pts',(45.9274099842789,-55.6766589025306,
-38.9854159162723));
#262819=CARTESIAN_POINT('Ctrl Pts',(45.9867610865919,-55.7209353156014,
-39.0037703637879));
#262820=CARTESIAN_POINT('Ctrl Pts',(46.1007337830098,-55.8148102393793,
-39.0405190865864));
#262821=CARTESIAN_POINT('Ctrl Pts',(46.1826971388658,-55.889219933262,-39.0681181728269));
#262822=CARTESIAN_POINT('Ctrl Pts',(46.259356574729,-55.9696687352924,-39.0957737179551));
#262823=CARTESIAN_POINT('Ctrl Pts',(46.309266807939,-56.024663053365,-39.1142236413887));
#262824=CARTESIAN_POINT('Ctrl Pts',(46.3336138177017,-56.0528284109483,
-39.1234510495426));
#262825=CARTESIAN_POINT('Ctrl Pts',(46.3692509284248,-56.0961546965833,
-39.1373141736981));
#262826=CARTESIAN_POINT('Ctrl Pts',(46.3809719555493,-56.1107655250657,
-39.14193505412));
#262827=CARTESIAN_POINT('Ctrl Pts',(46.4039850968433,-56.1401806715041,
-39.1511314768264));
#262828=CARTESIAN_POINT('Ctrl Pts',(46.4153001903629,-56.1550126624776,
-39.1557159133813));
#262829=CARTESIAN_POINT('Ctrl Pts',(46.4486370096885,-56.1998310060263,
-39.1694131182659));
#262830=CARTESIAN_POINT('Ctrl Pts',(46.4700835091466,-56.2301795317326,
-39.1784826054425));
#262831=CARTESIAN_POINT('Ctrl Pts',(46.532071913686,-56.3225583984772,-39.2054898733524));
#262832=CARTESIAN_POINT('Ctrl Pts',(46.5894197348374,-56.4176636744323,
-39.23211607576));
#262833=CARTESIAN_POINT('Ctrl Pts',(46.6566074362748,-56.5498680842415,
-39.2668544229849));
#262834=CARTESIAN_POINT('Ctrl Pts',(46.6870820302515,-56.617790568625,-39.2839693714534));
#262835=CARTESIAN_POINT('Ctrl Pts',(46.7159729830272,-56.6866360545619,
-39.3009558869148));
#262836=CARTESIAN_POINT('Ctrl Pts',(46.7296188023799,-56.7214992889704,
-39.3093799218186));
#262837=CARTESIAN_POINT('Ctrl Pts',(46.7553216997643,-56.7922546384013,
-39.3261176641085));
#262838=CARTESIAN_POINT('Ctrl Pts',(46.7672996943011,-56.8279354881579,
-39.3343809787628));
#262839=CARTESIAN_POINT('Ctrl Pts',(46.8004530502947,-56.9353633959568,
-39.358737163018));
#262840=CARTESIAN_POINT('Ctrl Pts',(46.8189795501832,-57.0077635587999,
-39.3744658121213));
#262841=CARTESIAN_POINT('Ctrl Pts',(46.848916211803,-57.1540080946302,-39.4048998290393));
#262842=CARTESIAN_POINT('Ctrl Pts',(46.866048617508,-57.2647966217996,-39.4269646939479));
#262843=CARTESIAN_POINT('Ctrl Pts',(46.875074749658,-57.3772756893033,-39.4478819384746));
#262844=CARTESIAN_POINT('Ctrl Pts',(46.8792542953452,-57.4526370309597,
-39.4615663943076));
#262845=CARTESIAN_POINT('Ctrl Pts',(46.8804258736835,-57.4905390832845,
-39.4682843608713));
#262846=CARTESIAN_POINT('Ctrl Pts',(46.8808837743635,-57.566610437341,-39.4814341960201));
#262847=CARTESIAN_POINT('Ctrl Pts',(46.8801708637706,-57.604491394965,-39.4878166677226));
#262848=CARTESIAN_POINT('Ctrl Pts',(46.8768913879562,-57.6800597985945,
-39.5002231148134));
#262849=CARTESIAN_POINT('Ctrl Pts',(46.8691896925243,-57.7930657109158,
-39.5182849936093));
#262850=CARTESIAN_POINT('Ctrl Pts',(46.8479069711518,-57.9423669591112,
-39.540205996752));
#262851=CARTESIAN_POINT('Ctrl Pts',(46.8236459543104,-58.053306681129,-39.5550278422771));
#262852=CARTESIAN_POINT('Ctrl Pts',(46.8055990109883,-58.1270324939452,
-39.5645447403379));
#262853=CARTESIAN_POINT('Ctrl Pts',(46.7956339676918,-58.1637938532181,
-39.5691227921436));
#262854=CARTESIAN_POINT('Ctrl Pts',(46.7738161327052,-58.2370162077019,
-39.5779016468881));
#262855=CARTESIAN_POINT('Ctrl Pts',(46.7619036278491,-58.2736352268715,
-39.5821192203466));
#262856=CARTESIAN_POINT('Ctrl Pts',(46.7364059718256,-58.3458255995332,
-39.5900871854462));
#262857=CARTESIAN_POINT('Ctrl Pts',(46.7091836493705,-58.4171862986019,
-39.5976163356366));
#262858=CARTESIAN_POINT('Ctrl Pts',(46.663274408039,-58.5216699086648,-39.6076014242402));
#262859=CARTESIAN_POINT('Ctrl Pts',(46.6123207377325,-58.6236436013082,
-39.616293729045));
#262860=CARTESIAN_POINT('Ctrl Pts',(46.5563244858032,-58.7230996041114,
-39.6236943138341));
#262861=CARTESIAN_POINT('Ctrl Pts',(46.515607032986,-58.7877140896312,-39.6277619492082));
#262862=CARTESIAN_POINT('Ctrl Pts',(46.4731710833873,-58.8514710047945,
-39.6313905635194));
#262863=CARTESIAN_POINT('Ctrl Pts',(46.4511086137465,-58.8829006319494,
-39.6329844599904));
#262864=CARTESIAN_POINT('Ctrl Pts',(46.4051673201274,-58.9449633016888,
-39.6357273485653));
#262865=CARTESIAN_POINT('Ctrl Pts',(46.381447994276,-58.975377588932,-39.6368662598532));
#262866=CARTESIAN_POINT('Ctrl Pts',(46.3084068909562,-59.0643493136614,
-39.6395761233691));
#262867=CARTESIAN_POINT('Ctrl Pts',(46.2570407846102,-59.1209150453974,
-39.6404603784325));
#262868=CARTESIAN_POINT('Ctrl Pts',(46.1491379755941,-59.228544463199,-39.6404138814247));
#262869=CARTESIAN_POINT('Ctrl Pts',(46.0925836555155,-59.2796343044913,
-39.6394845811684));
#262870=CARTESIAN_POINT('Ctrl Pts',(46.0038529437629,-59.3521266125547,
-39.6367223387528));
#262871=CARTESIAN_POINT('Ctrl Pts',(45.9736068078661,-59.3756113554055,
-39.6355721163029));
#262872=CARTESIAN_POINT('Ctrl Pts',(45.9272656961273,-59.4097723546528,
-39.6334997725088));
#262873=CARTESIAN_POINT('Ctrl Pts',(45.9116419215573,-59.4209912820171,
-39.6327502808957));
#262874=CARTESIAN_POINT('Ctrl Pts',(45.8800804794677,-59.4430610802669,
-39.6311351339295));
#262875=CARTESIAN_POINT('Ctrl Pts',(45.8321587971618,-59.4756823489919,
-39.628531354857));
#262876=CARTESIAN_POINT('Ctrl Pts',(45.7834097108732,-59.5062438963941,
-39.6254355071979));
#262877=CARTESIAN_POINT('Ctrl Pts',(45.717633106262,-59.5452481912826,-39.6208773262667));
#262878=CARTESIAN_POINT('Ctrl Pts',(45.6178307490054,-59.601113548897,-39.6133952897297));
#262879=CARTESIAN_POINT('Ctrl Pts',(45.4802897643185,-59.6652183443042,
-39.6008811885904));
#262880=CARTESIAN_POINT('Ctrl Pts',(45.3738098009101,-59.7055766782111,
-39.5896017905935));
#262881=CARTESIAN_POINT('Ctrl Pts',(45.3020778813705,-59.7307512119865,
-39.5816566825671));
#262882=CARTESIAN_POINT('Ctrl Pts',(45.2658207311094,-59.7424779859237,
-39.5774690651077));
#262883=CARTESIAN_POINT('Ctrl Pts',(45.1926264675053,-59.7641596016776,
-39.5686715125846));
#262884=CARTESIAN_POINT('Ctrl Pts',(45.1555073907618,-59.7741562512684,
-39.5640376159893));
#262885=CARTESIAN_POINT('Ctrl Pts',(45.0441315765335,-59.8011904590316,
-39.5496210468413));
#262886=CARTESIAN_POINT('Ctrl Pts',(44.9324484012679,-59.8224577850013,
-39.5341534065747));
#262887=CARTESIAN_POINT('Ctrl Pts',(44.8203079610257,-59.8353953605365,
-39.5171556909205));
#262888=CARTESIAN_POINT('Ctrl Pts',(44.7080184564226,-59.8455760612675,
-39.4996502778008));
#262889=CARTESIAN_POINT('Ctrl Pts',(44.6329372249224,-59.8486931621852,
-39.4873001861445));
#262890=CARTESIAN_POINT('Ctrl Pts',(44.5200834441659,-59.8478515133141,
-39.4677634802869));
#262891=CARTESIAN_POINT('Ctrl Pts',(44.4823810871712,-59.8466449718289,
-39.4610736497974));
#262892=CARTESIAN_POINT('Ctrl Pts',(44.4258051079382,-59.8434394706745,
-39.4507883432074));
#262893=CARTESIAN_POINT('Ctrl Pts',(44.4069254589855,-59.8421361346926,
-39.4473147915973));
#262894=CARTESIAN_POINT('Ctrl Pts',(44.3691376542581,-59.8390581625153,
-39.4402793331445));
#262895=CARTESIAN_POINT('Ctrl Pts',(44.3502459350849,-59.8372838734483,
-39.4367203104461));
#262896=CARTESIAN_POINT('Ctrl Pts',(44.2562487381671,-59.8272835659938,
-39.4188041728073));
#262897=CARTESIAN_POINT('Ctrl Pts',(44.1080045765469,-59.8040393501646,
-39.3892226636159));
#262898=CARTESIAN_POINT('Ctrl Pts',(43.9639303529155,-59.7668593120831,
-39.3578670379715));
#262899=CARTESIAN_POINT('Ctrl Pts',(43.8219159040518,-59.7227861654643,
-39.3256251231267));
#262900=CARTESIAN_POINT('Ctrl Pts',(43.7519290534068,-59.6972943066161,
-39.3090578287531));
#262901=CARTESIAN_POINT('Ctrl Pts',(43.665783177736,-59.6610675807531,-39.2877890488175));
#262902=CARTESIAN_POINT('Ctrl Pts',(43.6486106666635,-59.653596197985,-39.2835041280971));
#262903=CARTESIAN_POINT('Ctrl Pts',(43.6144193015916,-59.6382222359849,
-39.2748825183767));
#262904=CARTESIAN_POINT('Ctrl Pts',(43.597366582891,-59.6303022352814,-39.2705368924251));
#262905=CARTESIAN_POINT('Ctrl Pts',(43.5465994182959,-59.605961903298,-39.2574616452183));
#262906=CARTESIAN_POINT('Ctrl Pts',(43.513329300663,-59.588993111175,-39.2487085268073));
#262907=CARTESIAN_POINT('Ctrl Pts',(43.4805771074156,-59.5712767529309,
-39.2399080357013));
#262908=CARTESIAN_POINT('Ctrl Pts',(43.8903154257419,-57.7291941381088,
-41.4266127101804));
#262909=CARTESIAN_POINT('Ctrl Pts',(43.8716814361492,-57.7189244770852,
-41.4090117279687));
#262910=CARTESIAN_POINT('Ctrl Pts',(43.8355945080866,-57.6967277837834,
-41.3734625137379));
#262911=CARTESIAN_POINT('Ctrl Pts',(43.7849271573585,-57.6585752750105,
-41.3191078559793));
#262912=CARTESIAN_POINT('Ctrl Pts',(43.753465403225,-57.62988352171,-41.2821707250961));
#262913=CARTESIAN_POINT('Ctrl Pts',(43.7232071092872,-57.5995155202448,
-41.2448779944712));
#262914=CARTESIAN_POINT('Ctrl Pts',(43.694633283399,-57.5679550683129,-41.2078231506529));
#262915=CARTESIAN_POINT('Ctrl Pts',(43.6629744005209,-57.5256074013359,
-41.162062942605));
#262916=CARTESIAN_POINT('Ctrl Pts',(43.6400741040405,-57.4900012877665,
-41.1257945258022));
#262917=CARTESIAN_POINT('Ctrl Pts',(43.624122646482,-57.4624228770549,-41.0987642906252));
#262918=CARTESIAN_POINT('Ctrl Pts',(43.6143188854815,-57.4434516436916,
-41.0808660102928));
#262919=CARTESIAN_POINT('Ctrl Pts',(43.6049343759216,-57.4241698350281,
-41.0630203901697));
#262920=CARTESIAN_POINT('Ctrl Pts',(43.6004882740613,-57.4144479878336,
-41.054192925399));
#262921=CARTESIAN_POINT('Ctrl Pts',(43.5878889573419,-57.3850715912746,
-41.0280183011396));
#262922=CARTESIAN_POINT('Ctrl Pts',(43.5730447416356,-57.3453166524842,
-40.9939147159844));
#262923=CARTESIAN_POINT('Ctrl Pts',(43.5620571572655,-57.3044044614592,
-40.9613948378065));
#262924=CARTESIAN_POINT('Ctrl Pts',(43.5552843243605,-57.2732819874194,
-40.9376151994878));
#262925=CARTESIAN_POINT('Ctrl Pts',(43.5532714802541,-57.2628325912303,
-40.9297890667463));
#262926=CARTESIAN_POINT('Ctrl Pts',(43.5497454556161,-57.2417890776549,
-40.9143485382007));
#262927=CARTESIAN_POINT('Ctrl Pts',(43.5482304746054,-57.2311797832666,
-40.9067234564832));
#262928=CARTESIAN_POINT('Ctrl Pts',(43.5457184756399,-57.2098591834555,
-40.8917243418755));
#262929=CARTESIAN_POINT('Ctrl Pts',(43.5447290487245,-57.199220662917,-40.8844009198028));
#262930=CARTESIAN_POINT('Ctrl Pts',(43.5432711863927,-57.1779500447907,
-40.8700767121812));
#262931=CARTESIAN_POINT('Ctrl Pts',(43.5418684734652,-57.1460721839032,
-40.8490875836402));
#262932=CARTESIAN_POINT('Ctrl Pts',(43.5431039253892,-57.1036793909824,
-40.8230787545116));
#262933=CARTESIAN_POINT('Ctrl Pts',(43.5463738329101,-57.0719682486671,
-40.8050747359183));
#262934=CARTESIAN_POINT('Ctrl Pts',(43.5490829635055,-57.0508462881094,
-40.7934126279614));
#262935=CARTESIAN_POINT('Ctrl Pts',(43.5507030159248,-57.0402904723448,
-40.7877497380755));
#262936=CARTESIAN_POINT('Ctrl Pts',(43.5544790630841,-57.019214904491,-40.7767808895002));
#262937=CARTESIAN_POINT('Ctrl Pts',(43.5566463931059,-57.0086510117152,
-40.7714540988351));
#262938=CARTESIAN_POINT('Ctrl Pts',(43.5614808344627,-56.9877741662596,
-40.7612719783604));
#262939=CARTESIAN_POINT('Ctrl Pts',(43.5668234022498,-56.9670831174431,
-40.7515253398262));
#262940=CARTESIAN_POINT('Ctrl Pts',(43.5763377125496,-56.9366295208774,
-40.7382165180791));
#262941=CARTESIAN_POINT('Ctrl Pts',(43.5873444561754,-56.9067460923864,
-40.7262089422516));
#262942=CARTESIAN_POINT('Ctrl Pts',(43.5998453117462,-56.8774358278222,
-40.7155085881795));
#262943=CARTESIAN_POINT('Ctrl Pts',(43.6091839698139,-56.8582805167828,
-40.7092555817853));
#262944=CARTESIAN_POINT('Ctrl Pts',(43.6190331668358,-56.8393207538612,
-40.7034508410834));
#262945=CARTESIAN_POINT('Ctrl Pts',(43.6242099732076,-56.8299438685379,
-40.7007739810578));
#262946=CARTESIAN_POINT('Ctrl Pts',(43.6350986096338,-56.8113693026126,
-40.6958744145609));
#262947=CARTESIAN_POINT('Ctrl Pts',(43.6407690742328,-56.8022426567881,
-40.6936706244929));
#262948=CARTESIAN_POINT('Ctrl Pts',(43.6583896223854,-56.7754411523649,
-40.6878155334118));
#262949=CARTESIAN_POINT('Ctrl Pts',(43.6709801307092,-56.7582712890167,
-40.6848937134075));
#262950=CARTESIAN_POINT('Ctrl Pts',(43.6978023804218,-56.725340315416,-40.6809957255822));
#262951=CARTESIAN_POINT('Ctrl Pts',(43.7120405319879,-56.7095692151415,
-40.6800172734785));
#262952=CARTESIAN_POINT('Ctrl Pts',(43.7346338722206,-56.6869796178674,
-40.680019660452));
#262953=CARTESIAN_POINT('Ctrl Pts',(43.7423799312797,-56.6796208977126,
-40.6802668752224));
#262954=CARTESIAN_POINT('Ctrl Pts',(43.7543060585229,-56.6688607312791,
-40.681010981358));
#262955=CARTESIAN_POINT('Ctrl Pts',(43.7583370517177,-56.6653168192219,
-40.6813218268212));
#262956=CARTESIAN_POINT('Ctrl Pts',(43.7665035456834,-56.6583217341419,
-40.6820693651562));
#262957=CARTESIAN_POINT('Ctrl Pts',(43.7706422703,-56.6548683091639,-40.6825066780886));
#262958=CARTESIAN_POINT('Ctrl Pts',(43.7831478581881,-56.6447045100584,
-40.6840009724959));
#262959=CARTESIAN_POINT('Ctrl Pts',(43.8000992888712,-56.6316392340345,
-40.6864805452653));
#262960=CARTESIAN_POINT('Ctrl Pts',(43.8351004518507,-56.6074069729907,
-40.6933496988796));
#262961=CARTESIAN_POINT('Ctrl Pts',(43.8717190640765,-56.5859796680779,
-40.7030349737613));
#262962=CARTESIAN_POINT('Ctrl Pts',(43.9003898794618,-56.5719991465823,
-40.7123924126099));
#262963=CARTESIAN_POINT('Ctrl Pts',(43.919774692733,-56.5631479893168,-40.719099824507));
#262964=CARTESIAN_POINT('Ctrl Pts',(43.9296053152689,-56.5589560552736,
-40.722689237866));
#262965=CARTESIAN_POINT('Ctrl Pts',(43.9495302416178,-56.551051384942,-40.7303379810773));
#262966=CARTESIAN_POINT('Ctrl Pts',(43.959660471973,-56.5473282955902,-40.7344135607172));
#262967=CARTESIAN_POINT('Ctrl Pts',(43.9799461530017,-56.5404515818703,
-40.7429393172485));
#262968=CARTESIAN_POINT('Ctrl Pts',(43.9901452646573,-56.5372793127045,
-40.7474054189318));
#262969=CARTESIAN_POINT('Ctrl Pts',(44.0208712025373,-56.5285586047056,
-40.7613849151889));
#262970=CARTESIAN_POINT('Ctrl Pts',(44.0518784813599,-56.521416173947,-40.7765333604643));
#262971=CARTESIAN_POINT('Ctrl Pts',(44.0937728041468,-56.5149820273198,
-40.799005697554));
#262972=CARTESIAN_POINT('Ctrl Pts',(44.1254693703652,-56.5117027703592,
-40.8169947136667));
#262973=CARTESIAN_POINT('Ctrl Pts',(44.1467868482481,-56.5105547568045,
-40.8297474946377));
#262974=CARTESIAN_POINT('Ctrl Pts',(44.1681963264173,-56.50993223545,-40.842882238999));
#262975=CARTESIAN_POINT('Ctrl Pts',(44.1789665479467,-56.509886262238,-40.8496544547178));
#262976=CARTESIAN_POINT('Ctrl Pts',(44.2003410646824,-56.5103214152413,
-40.8634176853611));
#262977=CARTESIAN_POINT('Ctrl Pts',(44.2109953322312,-56.5108003631786,
-40.8704389119319));
#262978=CARTESIAN_POINT('Ctrl Pts',(44.2322091102727,-56.5122711761573,
-40.8847351429132));
#262979=CARTESIAN_POINT('Ctrl Pts',(44.2639028799147,-56.5152466319394,
-40.9065696963621));
#262980=CARTESIAN_POINT('Ctrl Pts',(44.305661850593,-56.5222422564611,-40.9372114433545));
#262981=CARTESIAN_POINT('Ctrl Pts',(44.346925841944,-56.532247127269,-40.9693597045385));
#262982=CARTESIAN_POINT('Ctrl Pts',(44.3673876336497,-56.53826115526,-40.9859357593442));
#262983=CARTESIAN_POINT('Ctrl Pts',(44.3877715667723,-56.5447901720246,
-41.0027718870644));
#262984=CARTESIAN_POINT('Ctrl Pts',(44.3979208506631,-56.5483132560745,
-41.0113182564434));
#262985=CARTESIAN_POINT('Ctrl Pts',(44.4179418071922,-56.5558066378292,
-41.02850287128));
#262986=CARTESIAN_POINT('Ctrl Pts',(44.4278499085732,-56.5597882829787,
-41.0371710128992));
#262987=CARTESIAN_POINT('Ctrl Pts',(44.4572364860018,-56.5724196473794,
-41.0633712499365));
#262988=CARTESIAN_POINT('Ctrl Pts',(44.4763932211824,-56.581758968269,-41.0811111519311));
#262989=CARTESIAN_POINT('Ctrl Pts',(44.5044772880921,-56.5971447477014,
-41.1081262866225));
#262990=CARTESIAN_POINT('Ctrl Pts',(44.5137271775895,-56.6025015227711,
-41.1171962449124));
#262991=CARTESIAN_POINT('Ctrl Pts',(44.5320183562985,-56.6136863880645,
-41.1354834617267));
#262992=CARTESIAN_POINT('Ctrl Pts',(44.5410031705763,-56.6194798267371,
-41.144644186283));
#262993=CARTESIAN_POINT('Ctrl Pts',(44.5674276642847,-56.6374191091633,
-41.1721205907467));
#262994=CARTESIAN_POINT('Ctrl Pts',(44.5843870769067,-56.6501457393646,
-41.1904750382678));
#262995=CARTESIAN_POINT('Ctrl Pts',(44.616987890196,-56.6770839740703,-41.2272237610649));
#262996=CARTESIAN_POINT('Ctrl Pts',(44.640458797708,-56.6984048650555,-41.2548228473058));
#262997=CARTESIAN_POINT('Ctrl Pts',(44.6624514458289,-56.7214114906953,
-41.2824783924342));
#262998=CARTESIAN_POINT('Ctrl Pts',(44.6767798128067,-56.7371294193188,
-41.3009283158679));
#262999=CARTESIAN_POINT('Ctrl Pts',(44.683774397772,-56.7451748501741,-41.3101557240219));
#263000=CARTESIAN_POINT('Ctrl Pts',(44.6940202659092,-56.7575442973705,
-41.324018848177));
#263001=CARTESIAN_POINT('Ctrl Pts',(44.6973914635031,-56.7617145235639,
-41.328639728599));
#263002=CARTESIAN_POINT('Ctrl Pts',(44.7040131878578,-56.770108052971,-41.3378361513053));
#263003=CARTESIAN_POINT('Ctrl Pts',(44.7072703203268,-56.7743392575068,
-41.3424205878605));
#263004=CARTESIAN_POINT('Ctrl Pts',(44.7168707027477,-56.7871217033085,
-41.3561177927451));
#263005=CARTESIAN_POINT('Ctrl Pts',(44.7230524906066,-56.7957731420119,
-41.3651872799216));
#263006=CARTESIAN_POINT('Ctrl Pts',(44.7409373255192,-56.8220955492914,
-41.3921945478314));
#263007=CARTESIAN_POINT('Ctrl Pts',(44.7575187561203,-56.8491712652862,
-41.4188207502394));
#263008=CARTESIAN_POINT('Ctrl Pts',(44.7770214494108,-56.88676384976,-41.453559097464));
#263009=CARTESIAN_POINT('Ctrl Pts',(44.7858965000619,-56.9060633365117,
-41.4706740459328));
#263010=CARTESIAN_POINT('Ctrl Pts',(44.7943266372896,-56.9256180211132,
-41.4876605613939));
#263011=CARTESIAN_POINT('Ctrl Pts',(44.7983169540911,-56.9355169983302,
-41.4960845962979));
#263012=CARTESIAN_POINT('Ctrl Pts',(44.8058516078422,-56.9556000996462,
-41.5128223385875));
#263013=CARTESIAN_POINT('Ctrl Pts',(44.8093727854448,-56.9657242505397,
-41.5210856532432));
#263014=CARTESIAN_POINT('Ctrl Pts',(44.8191505788346,-56.9961959016236,
-41.5454418374945));
#263015=CARTESIAN_POINT('Ctrl Pts',(44.8246597322132,-57.0167187198372,
-41.5611704866007));
#263016=CARTESIAN_POINT('Ctrl Pts',(44.8336688220904,-57.0581479791523,
-41.5916045035181));
#263017=CARTESIAN_POINT('Ctrl Pts',(44.8389236650083,-57.0895139074259,
-41.613669368427));
#263018=CARTESIAN_POINT('Ctrl Pts',(44.8418900765893,-57.1213299669285,
-41.6345866129535));
#263019=CARTESIAN_POINT('Ctrl Pts',(44.8433488372948,-57.142640498193,-41.6482710687869));
#263020=CARTESIAN_POINT('Ctrl Pts',(44.8438191277705,-57.1533552116615,
-41.6549890353504));
#263021=CARTESIAN_POINT('Ctrl Pts',(44.8442270800594,-57.1748537940466,
-41.6681388704993));
#263022=CARTESIAN_POINT('Ctrl Pts',(44.8441639040618,-57.1855561823783,
-41.6745213422017));
#263023=CARTESIAN_POINT('Ctrl Pts',(44.8435122114514,-57.2069000331791,
-41.6869277892926));
#263024=CARTESIAN_POINT('Ctrl Pts',(44.8417458896958,-57.2388084678274,
-41.7049896680882));
#263025=CARTESIAN_POINT('Ctrl Pts',(44.8362687719071,-57.2809279665006,
-41.7269106712316));
#263026=CARTESIAN_POINT('Ctrl Pts',(44.8298088085522,-57.3121969378441,
-41.7417325167562));
#263027=CARTESIAN_POINT('Ctrl Pts',(44.8249713776488,-57.3329705079708,
-41.751249414817));
#263028=CARTESIAN_POINT('Ctrl Pts',(44.8222858794974,-57.3433254378487,
-41.7558274666229));
#263029=CARTESIAN_POINT('Ctrl Pts',(44.8163797073795,-57.3639440769784,
-41.7646063213672));
#263030=CARTESIAN_POINT('Ctrl Pts',(44.8131427147447,-57.3742522416544,
-41.7688238948253));
#263031=CARTESIAN_POINT('Ctrl Pts',(44.8061917406462,-57.3945668799698,
-41.7767918599254));
#263032=CARTESIAN_POINT('Ctrl Pts',(44.7987498536529,-57.4146412549335,
-41.7843210101159));
#263033=CARTESIAN_POINT('Ctrl Pts',(44.7861419817956,-57.4440129710611,
-41.7943060987191));
#263034=CARTESIAN_POINT('Ctrl Pts',(44.7720982599006,-57.4726583092559,
-41.8029984035242));
#263035=CARTESIAN_POINT('Ctrl Pts',(44.7566193423106,-57.5005749992605,
-41.8103989883131));
#263036=CARTESIAN_POINT('Ctrl Pts',(44.7453362941317,-57.518697088903,-41.8144666236875));
#263037=CARTESIAN_POINT('Ctrl Pts',(44.7335642473644,-57.5365709174371,
-41.8180952379985));
#263038=CARTESIAN_POINT('Ctrl Pts',(44.7274378249752,-57.5453780864623,
-41.8196891344695));
#263039=CARTESIAN_POINT('Ctrl Pts',(44.7146685840676,-57.5627610237142,
-41.8224320230444));
#263040=CARTESIAN_POINT('Ctrl Pts',(44.7080700862024,-57.5712755128024,
-41.8235709343319));
#263041=CARTESIAN_POINT('Ctrl Pts',(44.6877341610586,-57.5961705213949,
-41.8262807978491));
#263042=CARTESIAN_POINT('Ctrl Pts',(44.6734117165454,-57.6119810052107,
-41.8271650529119));
#263043=CARTESIAN_POINT('Ctrl Pts',(44.6432859415473,-57.6420285404153,
-41.827118555904));
#263044=CARTESIAN_POINT('Ctrl Pts',(44.6274777219699,-57.6562729242579,
-41.8261892556471));
#263045=CARTESIAN_POINT('Ctrl Pts',(44.6026489360012,-57.6764545436153,
-41.823427013232));
#263046=CARTESIAN_POINT('Ctrl Pts',(44.5941811636919,-57.6829873126311,
-41.8222767907821));
#263047=CARTESIAN_POINT('Ctrl Pts',(44.5812011369499,-57.6924815728277,
-41.820204446988));
#263048=CARTESIAN_POINT('Ctrl Pts',(44.5768239301145,-57.6955981764101,
-41.8194549553751));
#263049=CARTESIAN_POINT('Ctrl Pts',(44.5679795363474,-57.7017261947271,
-41.8178398084084));
#263050=CARTESIAN_POINT('Ctrl Pts',(44.554547495243,-57.7107794649358,-41.8152360293365));
#263051=CARTESIAN_POINT('Ctrl Pts',(44.5408745509057,-57.7192473537464,
-41.812140181677));
#263052=CARTESIAN_POINT('Ctrl Pts',(44.5224181841827,-57.7300417662926,
-41.8075820007456));
#263053=CARTESIAN_POINT('Ctrl Pts',(44.494403164631,-57.7454824222945,-41.8000999642091));
#263054=CARTESIAN_POINT('Ctrl Pts',(44.4557509611988,-57.7631175354143,
-41.7875858630695));
#263055=CARTESIAN_POINT('Ctrl Pts',(44.4257963579031,-57.7741479888816,
-41.7763064650726));
#263056=CARTESIAN_POINT('Ctrl Pts',(44.4056101875344,-57.781009218212,-41.7683613570464));
#263057=CARTESIAN_POINT('Ctrl Pts',(44.3954036594654,-57.7841949818065,
-41.7641737395871));
#263058=CARTESIAN_POINT('Ctrl Pts',(44.3747925009816,-57.7900627169564,
-41.7553761870634));
#263059=CARTESIAN_POINT('Ctrl Pts',(44.3643365899562,-57.7927558542442,
-41.7507422904685));
#263060=CARTESIAN_POINT('Ctrl Pts',(44.3329536886806,-57.7999988857253,
-41.7363257213199));
#263061=CARTESIAN_POINT('Ctrl Pts',(44.3014645871824,-57.8056090798854,
-41.7208580810542));
#263062=CARTESIAN_POINT('Ctrl Pts',(44.2698183189435,-57.8088603667088,
-41.7038603653999));
#263063=CARTESIAN_POINT('Ctrl Pts',(44.2381206623806,-57.8113308880715,
-41.6863549522799));
#263064=CARTESIAN_POINT('Ctrl Pts',(44.2169139506954,-57.8119384373532,
-41.6740048606234));
#263065=CARTESIAN_POINT('Ctrl Pts',(44.1850197107514,-57.811287280344,-41.6544681547659));
#263066=CARTESIAN_POINT('Ctrl Pts',(44.1743613109546,-57.8108078241776,
-41.6477783242763));
#263067=CARTESIAN_POINT('Ctrl Pts',(44.1583626375358,-57.8096935003687,
-41.6374930176863));
#263068=CARTESIAN_POINT('Ctrl Pts',(44.1530230189312,-57.809255510817,-41.6340194660765));
#263069=CARTESIAN_POINT('Ctrl Pts',(44.1423341247923,-57.8082460206643,
-41.6269840076234));
#263070=CARTESIAN_POINT('Ctrl Pts',(44.1369894952372,-57.8076746784434,
-41.6234249849254));
#263071=CARTESIAN_POINT('Ctrl Pts',(44.1103928894951,-57.8045001122898,
-41.6055088472864));
#263072=CARTESIAN_POINT('Ctrl Pts',(44.0684216046586,-57.7973782151022,
-41.5759273380954));
#263073=CARTESIAN_POINT('Ctrl Pts',(44.0275807082801,-57.78632659952,-41.5445717124501));
#263074=CARTESIAN_POINT('Ctrl Pts',(43.9872978152183,-57.7733311875938,
-41.5123297976061));
#263075=CARTESIAN_POINT('Ctrl Pts',(43.9674326520914,-57.7658590768128,
-41.4957625032292));
#263076=CARTESIAN_POINT('Ctrl Pts',(43.942963744406,-57.7552890823142,-41.4744937232973));
#263077=CARTESIAN_POINT('Ctrl Pts',(43.938085174092,-57.7531113051098,-41.4702088025761));
#263078=CARTESIAN_POINT('Ctrl Pts',(43.9283699185172,-57.7486342535987,
-41.4615871928557));
#263079=CARTESIAN_POINT('Ctrl Pts',(43.9235236029976,-57.7463299238453,
-41.4572415669043));
#263080=CARTESIAN_POINT('Ctrl Pts',(43.9090930604083,-57.739254093668,-41.4441663196977));
#263081=CARTESIAN_POINT('Ctrl Pts',(43.8996324205383,-57.7343289686206,
-41.4354132012863));
#263082=CARTESIAN_POINT('Ctrl Pts',(43.8903154257419,-57.7291941381088,
-41.4266127101804));
#263083=CARTESIAN_POINT('Ctrl Pts',(45.3466064770396,-58.9181479613239,
-40.3575668307238));
#263084=CARTESIAN_POINT('Ctrl Pts',(45.4516646101692,-58.8920684645362,
-40.3337973782014));
#263085=CARTESIAN_POINT('Ctrl Pts',(45.552602293926,-58.8523392629073,-40.3122779577289));
#263086=CARTESIAN_POINT('Ctrl Pts',(45.770110848815,-58.7283580826205,-40.2690841502618));
#263087=CARTESIAN_POINT('Ctrl Pts',(45.8536347036611,-58.6509076535168,
-40.2548720327848));
#263088=CARTESIAN_POINT('Ctrl Pts',(45.9570392315636,-58.5416230805558,
-40.2380576556195));
#263089=CARTESIAN_POINT('Ctrl Pts',(46.0024773285342,-58.4828736078693,
-40.2313880447387));
#263090=CARTESIAN_POINT('Ctrl Pts',(46.0430807877281,-58.4179319806454,
-40.2261213989136));
#263091=CARTESIAN_POINT('Ctrl Pts',(46.0442081473202,-58.4161174068685,
-40.2259758098144));
#263092=CARTESIAN_POINT('Ctrl Pts',(46.0464553681406,-58.4124772870063,
-40.2256868790796));
#263093=CARTESIAN_POINT('Ctrl Pts',(46.0475751858796,-58.4106517551719,
-40.2255435461549));
#263094=CARTESIAN_POINT('Ctrl Pts',(46.0509385616361,-58.4051335817647,
-40.2251149869642));
#263095=CARTESIAN_POINT('Ctrl Pts',(46.0531661919851,-58.4014311118043,
-40.2248337748911));
#263096=CARTESIAN_POINT('Ctrl Pts',(46.057596560155,-58.3939710903869,-40.2242797496958));
#263097=CARTESIAN_POINT('Ctrl Pts',(46.0597989224255,-58.3902134067562,
-40.2240070251327));
#263098=CARTESIAN_POINT('Ctrl Pts',(46.0664273169517,-58.3787531619006,
-40.2231943218832));
#263099=CARTESIAN_POINT('Ctrl Pts',(46.0707848097754,-58.3710107097114,
-40.2226712692112));
#263100=CARTESIAN_POINT('Ctrl Pts',(46.11569824585,-58.2889710726676,-40.2173984115144));
#263101=CARTESIAN_POINT('Ctrl Pts',(46.1479046651237,-58.2104747759277,
-40.2146562982938));
#263102=CARTESIAN_POINT('Ctrl Pts',(46.2182188782769,-57.9683633912216,
-40.2117772978026));
#263103=CARTESIAN_POINT('Ctrl Pts',(46.2306353135395,-57.7999976154122,
-40.2167399225082));
#263104=CARTESIAN_POINT('Ctrl Pts',(46.2049800979504,-57.5666578926161,
-40.2296961597013));
#263105=CARTESIAN_POINT('Ctrl Pts',(46.1928858033625,-57.5018627715142,
-40.234134296036));
#263106=CARTESIAN_POINT('Ctrl Pts',(46.1762417771239,-57.4364451908711,
-40.2388223154954));
#263107=CARTESIAN_POINT('Ctrl Pts',(43.4805771074156,-59.5712767529309,
-39.2399080357013));
#263108=CARTESIAN_POINT('Ctrl Pts',(43.4150727209207,-59.5358440364426,
-39.2223070534893));
#263109=CARTESIAN_POINT('Ctrl Pts',(43.2883193276586,-59.4590682572254,
-39.1867578392588));
#263110=CARTESIAN_POINT('Ctrl Pts',(43.1106712693135,-59.32658002426,-39.1324031814995));
#263111=CARTESIAN_POINT('Ctrl Pts',(43.0005921597408,-59.2266373021163,
-39.0954660506179));
#263112=CARTESIAN_POINT('Ctrl Pts',(42.8948534568781,-59.1207134074407,
-39.0581733199915));
#263113=CARTESIAN_POINT('Ctrl Pts',(42.7951360401793,-59.0104958554849,
-39.0211184761739));
#263114=CARTESIAN_POINT('Ctrl Pts',(42.6850011896347,-58.8622904152127,
-38.9753582681256));
#263115=CARTESIAN_POINT('Ctrl Pts',(42.6055727997797,-58.7375004045667,
-38.939089851323));
#263116=CARTESIAN_POINT('Ctrl Pts',(42.5503788594446,-58.6407591922129,
-38.9120596161462));
#263117=CARTESIAN_POINT('Ctrl Pts',(42.5165536369311,-58.5741539171446,
-38.8941613358138));
#263118=CARTESIAN_POINT('Ctrl Pts',(42.4842288567228,-58.5064298632496,
-38.8763157156907));
#263119=CARTESIAN_POINT('Ctrl Pts',(42.4689425396028,-58.4722695523732,
-38.8674882509199));
#263120=CARTESIAN_POINT('Ctrl Pts',(42.4257123024776,-58.3690064948315,
-38.8413136266604));
#263121=CARTESIAN_POINT('Ctrl Pts',(42.3750272156063,-58.229152189777,-38.8072100415055));
#263122=CARTESIAN_POINT('Ctrl Pts',(42.3380647902547,-58.0850119200902,
-38.7746901633276));
#263123=CARTESIAN_POINT('Ctrl Pts',(42.3155659796374,-57.9752818499468,
-38.7509105250088));
#263124=CARTESIAN_POINT('Ctrl Pts',(42.3089374211558,-57.9384266221928,
-38.7430843922672));
#263125=CARTESIAN_POINT('Ctrl Pts',(42.297458012674,-57.864178756387,-38.7276438637217));
#263126=CARTESIAN_POINT('Ctrl Pts',(42.292601515188,-57.8267325312259,-38.720018782004));
#263127=CARTESIAN_POINT('Ctrl Pts',(42.2847289916893,-57.7514526301959,
-38.7050196673963));
#263128=CARTESIAN_POINT('Ctrl Pts',(42.2817363521424,-57.7138759968928,
-38.6976962453237));
#263129=CARTESIAN_POINT('Ctrl Pts',(42.277596992864,-57.6387184974263,-38.6833720377019));
#263130=CARTESIAN_POINT('Ctrl Pts',(42.2741651307842,-57.5260409596698,
-38.6623829091612));
#263131=CARTESIAN_POINT('Ctrl Pts',(42.2805893100654,-57.3760354719141,
-38.6363740800325));
#263132=CARTESIAN_POINT('Ctrl Pts',(42.2937061680812,-57.2637038035873,
-38.618370061439));
#263133=CARTESIAN_POINT('Ctrl Pts',(42.3043247017591,-57.1888547452426,
-38.6067079534822));
#263134=CARTESIAN_POINT('Ctrl Pts',(42.3105743117123,-57.1514345461221,
-38.6010450635964));
#263135=CARTESIAN_POINT('Ctrl Pts',(42.3249704170347,-57.0766935209607,
-38.590076215021));
#263136=CARTESIAN_POINT('Ctrl Pts',(42.3331592025312,-57.0392159768686,
-38.5847494243559));
#263137=CARTESIAN_POINT('Ctrl Pts',(42.3512949844302,-56.9651221381903,
-38.5745673038812));
#263138=CARTESIAN_POINT('Ctrl Pts',(42.3712216906218,-56.8916587034686,
-38.564820665347));
#263139=CARTESIAN_POINT('Ctrl Pts',(42.4063979707918,-56.7834465224234,
-38.5515118436));
#263140=CARTESIAN_POINT('Ctrl Pts',(42.4468320479729,-56.6771725078319,
-38.5395042677724));
#263141=CARTESIAN_POINT('Ctrl Pts',(42.4925290654744,-56.5728473165674,
-38.5288039137004));
#263142=CARTESIAN_POINT('Ctrl Pts',(42.5265325119253,-56.5046058456765,
-38.5225509073062));
#263143=CARTESIAN_POINT('Ctrl Pts',(42.5623338475306,-56.4370293947697,
-38.5167461666044));
#263144=CARTESIAN_POINT('Ctrl Pts',(42.5811223641794,-56.4035923099625,
-38.5140693065785));
#263145=CARTESIAN_POINT('Ctrl Pts',(42.620584523009,-56.3373241998654,-38.5091697400817));
#263146=CARTESIAN_POINT('Ctrl Pts',(42.6411082254821,-56.3047465904101,
-38.5069659500128));
#263147=CARTESIAN_POINT('Ctrl Pts',(42.7048067991197,-56.2090283357163,
-38.501110858935));
#263148=CARTESIAN_POINT('Ctrl Pts',(42.7502234543428,-56.1476408662828,
-38.4981890389281));
#263149=CARTESIAN_POINT('Ctrl Pts',(42.8467942323831,-56.0297655581676,
-38.4942910511033));
#263150=CARTESIAN_POINT('Ctrl Pts',(42.8979715413934,-55.9732420482176,
-38.4933125989996));
#263151=CARTESIAN_POINT('Ctrl Pts',(42.9790570553347,-55.8921695883033,
-38.4933149859729));
#263152=CARTESIAN_POINT('Ctrl Pts',(43.0068374106561,-55.8657400908868,
-38.4935622007431));
#263153=CARTESIAN_POINT('Ctrl Pts',(43.0495800649421,-55.8270637749536,
-38.4943063068789));
#263154=CARTESIAN_POINT('Ctrl Pts',(43.0640222060113,-55.8143203511958,
-38.494617152342));
#263155=CARTESIAN_POINT('Ctrl Pts',(43.0932714774893,-55.7891564261061,
-38.4953646906773));
#263156=CARTESIAN_POINT('Ctrl Pts',(43.1080901283632,-55.7767277938553,
-38.4958020036096));
#263157=CARTESIAN_POINT('Ctrl Pts',(43.1528523310046,-55.7401327167866,
-38.4972962980169));
#263158=CARTESIAN_POINT('Ctrl Pts',(43.2134913856688,-55.6930468850421,
-38.4997758707861));
#263159=CARTESIAN_POINT('Ctrl Pts',(43.3385569247743,-55.6055389451161,
-38.5066450244003));
#263160=CARTESIAN_POINT('Ctrl Pts',(43.4691986576013,-55.5278792007279,
-38.5163302992824));
#263161=CARTESIAN_POINT('Ctrl Pts',(43.5713395927684,-55.4769743237494,
-38.5256877381308));
#263162=CARTESIAN_POINT('Ctrl Pts',(43.6403672861995,-55.4446857735354,
-38.5323951500278));
#263163=CARTESIAN_POINT('Ctrl Pts',(43.6753577685123,-55.4293620157832,
-38.5359845633874));
#263164=CARTESIAN_POINT('Ctrl Pts',(43.7462462065788,-55.4003985583156,
-38.5436333065981));
#263165=CARTESIAN_POINT('Ctrl Pts',(43.7822717759725,-55.3867204456352,
-38.5477088862383));
#263166=CARTESIAN_POINT('Ctrl Pts',(43.8543821738219,-55.3613797848081,
-38.5562346427694));
#263167=CARTESIAN_POINT('Ctrl Pts',(43.890622407919,-55.349649082917,-38.5607007444526));
#263168=CARTESIAN_POINT('Ctrl Pts',(43.9997560709039,-55.3172704656441,
-38.5746802407103));
#263169=CARTESIAN_POINT('Ctrl Pts',(44.1098017310836,-55.290468361793,-38.5898286859852));
#263170=CARTESIAN_POINT('Ctrl Pts',(44.2583166685835,-55.2656490138239,
-38.612301023075));
#263171=CARTESIAN_POINT('Ctrl Pts',(44.3705972700495,-55.2524997368729,
-38.6302900391873));
#263172=CARTESIAN_POINT('Ctrl Pts',(44.446056048267,-55.2474029004138,-38.6430428201589));
#263173=CARTESIAN_POINT('Ctrl Pts',(44.5218128020516,-55.2441636366351,
-38.65617756452));
#263174=CARTESIAN_POINT('Ctrl Pts',(44.5599089424743,-55.2434808562086,
-38.6629497802385));
#263175=CARTESIAN_POINT('Ctrl Pts',(44.6354869543582,-55.2439911084578,
-38.6767130108817));
#263176=CARTESIAN_POINT('Ctrl Pts',(44.6731456892459,-55.2451740103824,
-38.6837342374529));
#263177=CARTESIAN_POINT('Ctrl Pts',(44.7481014788608,-55.2493620066237,
-38.6980304684339));
#263178=CARTESIAN_POINT('Ctrl Pts',(44.860046548974,-55.2583760573225,-38.7198650218829));
#263179=CARTESIAN_POINT('Ctrl Pts',(45.0073845433675,-55.2811507310277,
-38.7505067688753));
#263180=CARTESIAN_POINT('Ctrl Pts',(45.1528189888476,-55.3146135839333,
-38.7826550300594));
#263181=CARTESIAN_POINT('Ctrl Pts',(45.2248832056965,-55.3349380951144,
-38.7992310848652));
#263182=CARTESIAN_POINT('Ctrl Pts',(45.2966462681613,-55.3570913336823,
-38.8160672125853));
#263183=CARTESIAN_POINT('Ctrl Pts',(45.3323638946335,-55.3690863290504,
-38.8246135819642));
#263184=CARTESIAN_POINT('Ctrl Pts',(45.4027951436545,-55.3946744461232,
-38.841798196801));
#263185=CARTESIAN_POINT('Ctrl Pts',(45.4376370321487,-55.4083060218429,
-38.85046633842));
#263186=CARTESIAN_POINT('Ctrl Pts',(45.5409345111852,-55.4516493275196,
-38.8766665754573));
#263187=CARTESIAN_POINT('Ctrl Pts',(45.6082182891413,-55.4838201174091,
-38.8944064774514));
#263188=CARTESIAN_POINT('Ctrl Pts',(45.7067749877369,-55.5369855856676,
-38.9214216121435));
#263189=CARTESIAN_POINT('Ctrl Pts',(45.7392219877795,-55.5555212114618,
-38.9304915704334));
#263190=CARTESIAN_POINT('Ctrl Pts',(45.8033556832395,-55.5942722159849,
-38.9487787872477));
#263191=CARTESIAN_POINT('Ctrl Pts',(45.8348443691401,-55.6143675312756,
-38.9579395118015));
#263192=CARTESIAN_POINT('Ctrl Pts',(45.9274099842789,-55.6766589025306,
-38.9854159162723));
#263193=CARTESIAN_POINT('Ctrl Pts',(45.9867610865919,-55.7209353156014,
-39.0037703637879));
#263194=CARTESIAN_POINT('Ctrl Pts',(46.1007337830098,-55.8148102393793,
-39.0405190865864));
#263195=CARTESIAN_POINT('Ctrl Pts',(46.1826971388658,-55.889219933262,-39.0681181728269));
#263196=CARTESIAN_POINT('Ctrl Pts',(46.259356574729,-55.9696687352924,-39.0957737179551));
#263197=CARTESIAN_POINT('Ctrl Pts',(46.309266807939,-56.024663053365,-39.1142236413887));
#263198=CARTESIAN_POINT('Ctrl Pts',(46.3336138177017,-56.0528284109483,
-39.1234510495426));
#263199=CARTESIAN_POINT('Ctrl Pts',(46.3692509284248,-56.0961546965833,
-39.1373141736981));
#263200=CARTESIAN_POINT('Ctrl Pts',(46.3809719555493,-56.1107655250657,
-39.14193505412));
#263201=CARTESIAN_POINT('Ctrl Pts',(46.4039850968433,-56.1401806715041,
-39.1511314768264));
#263202=CARTESIAN_POINT('Ctrl Pts',(46.4153001903629,-56.1550126624776,
-39.1557159133813));
#263203=CARTESIAN_POINT('Ctrl Pts',(46.4486370096885,-56.1998310060263,
-39.1694131182659));
#263204=CARTESIAN_POINT('Ctrl Pts',(46.4700835091466,-56.2301795317326,
-39.1784826054425));
#263205=CARTESIAN_POINT('Ctrl Pts',(46.532071913686,-56.3225583984772,-39.2054898733524));
#263206=CARTESIAN_POINT('Ctrl Pts',(46.5894197348374,-56.4176636744323,
-39.23211607576));
#263207=CARTESIAN_POINT('Ctrl Pts',(46.6566074362748,-56.5498680842415,
-39.2668544229849));
#263208=CARTESIAN_POINT('Ctrl Pts',(46.6870820302515,-56.617790568625,-39.2839693714534));
#263209=CARTESIAN_POINT('Ctrl Pts',(46.7159729830272,-56.6866360545619,
-39.3009558869148));
#263210=CARTESIAN_POINT('Ctrl Pts',(46.7296188023799,-56.7214992889704,
-39.3093799218186));
#263211=CARTESIAN_POINT('Ctrl Pts',(46.7553216997643,-56.7922546384013,
-39.3261176641085));
#263212=CARTESIAN_POINT('Ctrl Pts',(46.7672996943011,-56.8279354881579,
-39.3343809787628));
#263213=CARTESIAN_POINT('Ctrl Pts',(46.8004530502947,-56.9353633959568,
-39.358737163018));
#263214=CARTESIAN_POINT('Ctrl Pts',(46.8189795501832,-57.0077635587999,
-39.3744658121213));
#263215=CARTESIAN_POINT('Ctrl Pts',(46.848916211803,-57.1540080946302,-39.4048998290393));
#263216=CARTESIAN_POINT('Ctrl Pts',(46.866048617508,-57.2647966217996,-39.4269646939479));
#263217=CARTESIAN_POINT('Ctrl Pts',(46.875074749658,-57.3772756893033,-39.4478819384746));
#263218=CARTESIAN_POINT('Ctrl Pts',(46.8792542953452,-57.4526370309597,
-39.4615663943076));
#263219=CARTESIAN_POINT('Ctrl Pts',(46.8804258736835,-57.4905390832845,
-39.4682843608713));
#263220=CARTESIAN_POINT('Ctrl Pts',(46.8808837743635,-57.566610437341,-39.4814341960201));
#263221=CARTESIAN_POINT('Ctrl Pts',(46.8801708637706,-57.604491394965,-39.4878166677226));
#263222=CARTESIAN_POINT('Ctrl Pts',(46.8768913879562,-57.6800597985945,
-39.5002231148134));
#263223=CARTESIAN_POINT('Ctrl Pts',(46.8691896925243,-57.7930657109158,
-39.5182849936093));
#263224=CARTESIAN_POINT('Ctrl Pts',(46.8479069711518,-57.9423669591112,
-39.540205996752));
#263225=CARTESIAN_POINT('Ctrl Pts',(46.8236459543104,-58.053306681129,-39.5550278422771));
#263226=CARTESIAN_POINT('Ctrl Pts',(46.8055990109883,-58.1270324939452,
-39.5645447403379));
#263227=CARTESIAN_POINT('Ctrl Pts',(46.7956339676918,-58.1637938532181,
-39.5691227921436));
#263228=CARTESIAN_POINT('Ctrl Pts',(46.7738161327052,-58.2370162077019,
-39.5779016468881));
#263229=CARTESIAN_POINT('Ctrl Pts',(46.7619036278491,-58.2736352268715,
-39.5821192203466));
#263230=CARTESIAN_POINT('Ctrl Pts',(46.7364059718256,-58.3458255995332,
-39.5900871854462));
#263231=CARTESIAN_POINT('Ctrl Pts',(46.7091836493705,-58.4171862986019,
-39.5976163356366));
#263232=CARTESIAN_POINT('Ctrl Pts',(46.663274408039,-58.5216699086648,-39.6076014242402));
#263233=CARTESIAN_POINT('Ctrl Pts',(46.6123207377325,-58.6236436013082,
-39.616293729045));
#263234=CARTESIAN_POINT('Ctrl Pts',(46.5563244858032,-58.7230996041114,
-39.6236943138341));
#263235=CARTESIAN_POINT('Ctrl Pts',(46.515607032986,-58.7877140896312,-39.6277619492082));
#263236=CARTESIAN_POINT('Ctrl Pts',(46.4731710833873,-58.8514710047945,
-39.6313905635194));
#263237=CARTESIAN_POINT('Ctrl Pts',(46.4511086137465,-58.8829006319494,
-39.6329844599904));
#263238=CARTESIAN_POINT('Ctrl Pts',(46.4051673201274,-58.9449633016888,
-39.6357273485653));
#263239=CARTESIAN_POINT('Ctrl Pts',(46.381447994276,-58.975377588932,-39.6368662598532));
#263240=CARTESIAN_POINT('Ctrl Pts',(46.3084068909562,-59.0643493136614,
-39.6395761233691));
#263241=CARTESIAN_POINT('Ctrl Pts',(46.2570407846102,-59.1209150453974,
-39.6404603784325));
#263242=CARTESIAN_POINT('Ctrl Pts',(46.1491379755941,-59.228544463199,-39.6404138814247));
#263243=CARTESIAN_POINT('Ctrl Pts',(46.0925836555155,-59.2796343044913,
-39.6394845811684));
#263244=CARTESIAN_POINT('Ctrl Pts',(46.0038529437629,-59.3521266125547,
-39.6367223387528));
#263245=CARTESIAN_POINT('Ctrl Pts',(45.9736068078661,-59.3756113554055,
-39.6355721163029));
#263246=CARTESIAN_POINT('Ctrl Pts',(45.9272656961273,-59.4097723546528,
-39.6334997725088));
#263247=CARTESIAN_POINT('Ctrl Pts',(45.9116419215573,-59.4209912820171,
-39.6327502808957));
#263248=CARTESIAN_POINT('Ctrl Pts',(45.8800804794677,-59.4430610802669,
-39.6311351339295));
#263249=CARTESIAN_POINT('Ctrl Pts',(45.8321587971618,-59.4756823489919,
-39.628531354857));
#263250=CARTESIAN_POINT('Ctrl Pts',(45.7834097108732,-59.5062438963941,
-39.6254355071979));
#263251=CARTESIAN_POINT('Ctrl Pts',(45.717633106262,-59.5452481912826,-39.6208773262667));
#263252=CARTESIAN_POINT('Ctrl Pts',(45.6178307490054,-59.601113548897,-39.6133952897297));
#263253=CARTESIAN_POINT('Ctrl Pts',(45.4802897643185,-59.6652183443042,
-39.6008811885904));
#263254=CARTESIAN_POINT('Ctrl Pts',(45.3738098009101,-59.7055766782111,
-39.5896017905935));
#263255=CARTESIAN_POINT('Ctrl Pts',(45.3020778813705,-59.7307512119865,
-39.5816566825671));
#263256=CARTESIAN_POINT('Ctrl Pts',(45.2658207311094,-59.7424779859237,
-39.5774690651077));
#263257=CARTESIAN_POINT('Ctrl Pts',(45.1926264675053,-59.7641596016776,
-39.5686715125846));
#263258=CARTESIAN_POINT('Ctrl Pts',(45.1555073907618,-59.7741562512684,
-39.5640376159893));
#263259=CARTESIAN_POINT('Ctrl Pts',(45.0441315765335,-59.8011904590316,
-39.5496210468413));
#263260=CARTESIAN_POINT('Ctrl Pts',(44.9324484012679,-59.8224577850013,
-39.5341534065747));
#263261=CARTESIAN_POINT('Ctrl Pts',(44.8203079610257,-59.8353953605365,
-39.5171556909205));
#263262=CARTESIAN_POINT('Ctrl Pts',(44.7080184564226,-59.8455760612675,
-39.4996502778008));
#263263=CARTESIAN_POINT('Ctrl Pts',(44.6329372249224,-59.8486931621852,
-39.4873001861445));
#263264=CARTESIAN_POINT('Ctrl Pts',(44.5200834441659,-59.8478515133141,
-39.4677634802869));
#263265=CARTESIAN_POINT('Ctrl Pts',(44.4823810871712,-59.8466449718289,
-39.4610736497974));
#263266=CARTESIAN_POINT('Ctrl Pts',(44.4258051079382,-59.8434394706745,
-39.4507883432074));
#263267=CARTESIAN_POINT('Ctrl Pts',(44.4069254589855,-59.8421361346926,
-39.4473147915973));
#263268=CARTESIAN_POINT('Ctrl Pts',(44.3691376542581,-59.8390581625153,
-39.4402793331445));
#263269=CARTESIAN_POINT('Ctrl Pts',(44.3502459350849,-59.8372838734483,
-39.4367203104461));
#263270=CARTESIAN_POINT('Ctrl Pts',(44.2562487381671,-59.8272835659938,
-39.4188041728073));
#263271=CARTESIAN_POINT('Ctrl Pts',(44.1080045765469,-59.8040393501646,
-39.3892226636159));
#263272=CARTESIAN_POINT('Ctrl Pts',(43.9639303529155,-59.7668593120831,
-39.3578670379715));
#263273=CARTESIAN_POINT('Ctrl Pts',(43.8219159040518,-59.7227861654643,
-39.3256251231267));
#263274=CARTESIAN_POINT('Ctrl Pts',(43.7519290534068,-59.6972943066161,
-39.3090578287531));
#263275=CARTESIAN_POINT('Ctrl Pts',(43.665783177736,-59.6610675807531,-39.2877890488175));
#263276=CARTESIAN_POINT('Ctrl Pts',(43.6486106666635,-59.653596197985,-39.2835041280971));
#263277=CARTESIAN_POINT('Ctrl Pts',(43.6144193015916,-59.6382222359849,
-39.2748825183767));
#263278=CARTESIAN_POINT('Ctrl Pts',(43.597366582891,-59.6303022352814,-39.2705368924251));
#263279=CARTESIAN_POINT('Ctrl Pts',(43.5465994182959,-59.605961903298,-39.2574616452183));
#263280=CARTESIAN_POINT('Ctrl Pts',(43.513329300663,-59.588993111175,-39.2487085268073));
#263281=CARTESIAN_POINT('Ctrl Pts',(43.4805771074156,-59.5712767529309,
-39.2399080357013));
#263282=CARTESIAN_POINT('Ctrl Pts',(43.8903154257419,-57.7291941381088,
-41.4266127101804));
#263283=CARTESIAN_POINT('Ctrl Pts',(43.8716814361492,-57.7189244770852,
-41.4090117279687));
#263284=CARTESIAN_POINT('Ctrl Pts',(43.8355945080866,-57.6967277837834,
-41.3734625137379));
#263285=CARTESIAN_POINT('Ctrl Pts',(43.7849271573585,-57.6585752750105,
-41.3191078559793));
#263286=CARTESIAN_POINT('Ctrl Pts',(43.753465403225,-57.62988352171,-41.2821707250961));
#263287=CARTESIAN_POINT('Ctrl Pts',(43.7232071092872,-57.5995155202448,
-41.2448779944712));
#263288=CARTESIAN_POINT('Ctrl Pts',(43.694633283399,-57.5679550683129,-41.2078231506529));
#263289=CARTESIAN_POINT('Ctrl Pts',(43.6629744005209,-57.5256074013359,
-41.162062942605));
#263290=CARTESIAN_POINT('Ctrl Pts',(43.6400741040405,-57.4900012877665,
-41.1257945258022));
#263291=CARTESIAN_POINT('Ctrl Pts',(43.624122646482,-57.4624228770549,-41.0987642906252));
#263292=CARTESIAN_POINT('Ctrl Pts',(43.6143188854815,-57.4434516436916,
-41.0808660102928));
#263293=CARTESIAN_POINT('Ctrl Pts',(43.6049343759216,-57.4241698350281,
-41.0630203901697));
#263294=CARTESIAN_POINT('Ctrl Pts',(43.6004882740613,-57.4144479878336,
-41.054192925399));
#263295=CARTESIAN_POINT('Ctrl Pts',(43.5878889573419,-57.3850715912746,
-41.0280183011396));
#263296=CARTESIAN_POINT('Ctrl Pts',(43.5730447416356,-57.3453166524842,
-40.9939147159844));
#263297=CARTESIAN_POINT('Ctrl Pts',(43.5620571572655,-57.3044044614592,
-40.9613948378065));
#263298=CARTESIAN_POINT('Ctrl Pts',(43.5552843243605,-57.2732819874194,
-40.9376151994878));
#263299=CARTESIAN_POINT('Ctrl Pts',(43.5532714802541,-57.2628325912303,
-40.9297890667463));
#263300=CARTESIAN_POINT('Ctrl Pts',(43.5497454556161,-57.2417890776549,
-40.9143485382007));
#263301=CARTESIAN_POINT('Ctrl Pts',(43.5482304746054,-57.2311797832666,
-40.9067234564832));
#263302=CARTESIAN_POINT('Ctrl Pts',(43.5457184756399,-57.2098591834555,
-40.8917243418755));
#263303=CARTESIAN_POINT('Ctrl Pts',(43.5447290487245,-57.199220662917,-40.8844009198028));
#263304=CARTESIAN_POINT('Ctrl Pts',(43.5432711863927,-57.1779500447907,
-40.8700767121812));
#263305=CARTESIAN_POINT('Ctrl Pts',(43.5418684734652,-57.1460721839032,
-40.8490875836402));
#263306=CARTESIAN_POINT('Ctrl Pts',(43.5431039253892,-57.1036793909824,
-40.8230787545116));
#263307=CARTESIAN_POINT('Ctrl Pts',(43.5463738329101,-57.0719682486671,
-40.8050747359183));
#263308=CARTESIAN_POINT('Ctrl Pts',(43.5490829635055,-57.0508462881094,
-40.7934126279614));
#263309=CARTESIAN_POINT('Ctrl Pts',(43.5507030159248,-57.0402904723448,
-40.7877497380755));
#263310=CARTESIAN_POINT('Ctrl Pts',(43.5544790630841,-57.019214904491,-40.7767808895002));
#263311=CARTESIAN_POINT('Ctrl Pts',(43.5566463931059,-57.0086510117152,
-40.7714540988351));
#263312=CARTESIAN_POINT('Ctrl Pts',(43.5614808344627,-56.9877741662596,
-40.7612719783604));
#263313=CARTESIAN_POINT('Ctrl Pts',(43.5668234022498,-56.9670831174431,
-40.7515253398262));
#263314=CARTESIAN_POINT('Ctrl Pts',(43.5763377125496,-56.9366295208774,
-40.7382165180791));
#263315=CARTESIAN_POINT('Ctrl Pts',(43.5873444561754,-56.9067460923864,
-40.7262089422516));
#263316=CARTESIAN_POINT('Ctrl Pts',(43.5998453117462,-56.8774358278222,
-40.7155085881795));
#263317=CARTESIAN_POINT('Ctrl Pts',(43.6091839698139,-56.8582805167828,
-40.7092555817853));
#263318=CARTESIAN_POINT('Ctrl Pts',(43.6190331668358,-56.8393207538612,
-40.7034508410834));
#263319=CARTESIAN_POINT('Ctrl Pts',(43.6242099732076,-56.8299438685379,
-40.7007739810578));
#263320=CARTESIAN_POINT('Ctrl Pts',(43.6350986096338,-56.8113693026126,
-40.6958744145609));
#263321=CARTESIAN_POINT('Ctrl Pts',(43.6407690742328,-56.8022426567881,
-40.6936706244929));
#263322=CARTESIAN_POINT('Ctrl Pts',(43.6583896223854,-56.7754411523649,
-40.6878155334118));
#263323=CARTESIAN_POINT('Ctrl Pts',(43.6709801307092,-56.7582712890167,
-40.6848937134075));
#263324=CARTESIAN_POINT('Ctrl Pts',(43.6978023804218,-56.725340315416,-40.6809957255822));
#263325=CARTESIAN_POINT('Ctrl Pts',(43.7120405319879,-56.7095692151415,
-40.6800172734785));
#263326=CARTESIAN_POINT('Ctrl Pts',(43.7346338722206,-56.6869796178674,
-40.680019660452));
#263327=CARTESIAN_POINT('Ctrl Pts',(43.7423799312797,-56.6796208977126,
-40.6802668752224));
#263328=CARTESIAN_POINT('Ctrl Pts',(43.7543060585229,-56.6688607312791,
-40.681010981358));
#263329=CARTESIAN_POINT('Ctrl Pts',(43.7583370517177,-56.6653168192219,
-40.6813218268212));
#263330=CARTESIAN_POINT('Ctrl Pts',(43.7665035456834,-56.6583217341419,
-40.6820693651562));
#263331=CARTESIAN_POINT('Ctrl Pts',(43.7706422703,-56.6548683091639,-40.6825066780886));
#263332=CARTESIAN_POINT('Ctrl Pts',(43.7831478581881,-56.6447045100584,
-40.6840009724959));
#263333=CARTESIAN_POINT('Ctrl Pts',(43.8000992888712,-56.6316392340345,
-40.6864805452653));
#263334=CARTESIAN_POINT('Ctrl Pts',(43.8351004518507,-56.6074069729907,
-40.6933496988796));
#263335=CARTESIAN_POINT('Ctrl Pts',(43.8717190640765,-56.5859796680779,
-40.7030349737613));
#263336=CARTESIAN_POINT('Ctrl Pts',(43.9003898794618,-56.5719991465823,
-40.7123924126099));
#263337=CARTESIAN_POINT('Ctrl Pts',(43.919774692733,-56.5631479893168,-40.719099824507));
#263338=CARTESIAN_POINT('Ctrl Pts',(43.9296053152689,-56.5589560552736,
-40.722689237866));
#263339=CARTESIAN_POINT('Ctrl Pts',(43.9495302416178,-56.551051384942,-40.7303379810773));
#263340=CARTESIAN_POINT('Ctrl Pts',(43.959660471973,-56.5473282955902,-40.7344135607172));
#263341=CARTESIAN_POINT('Ctrl Pts',(43.9799461530017,-56.5404515818703,
-40.7429393172485));
#263342=CARTESIAN_POINT('Ctrl Pts',(43.9901452646573,-56.5372793127045,
-40.7474054189318));
#263343=CARTESIAN_POINT('Ctrl Pts',(44.0208712025373,-56.5285586047056,
-40.7613849151889));
#263344=CARTESIAN_POINT('Ctrl Pts',(44.0518784813599,-56.521416173947,-40.7765333604643));
#263345=CARTESIAN_POINT('Ctrl Pts',(44.0937728041468,-56.5149820273198,
-40.799005697554));
#263346=CARTESIAN_POINT('Ctrl Pts',(44.1254693703652,-56.5117027703592,
-40.8169947136667));
#263347=CARTESIAN_POINT('Ctrl Pts',(44.1467868482481,-56.5105547568045,
-40.8297474946377));
#263348=CARTESIAN_POINT('Ctrl Pts',(44.1681963264173,-56.50993223545,-40.842882238999));
#263349=CARTESIAN_POINT('Ctrl Pts',(44.1789665479467,-56.509886262238,-40.8496544547178));
#263350=CARTESIAN_POINT('Ctrl Pts',(44.2003410646824,-56.5103214152413,
-40.8634176853611));
#263351=CARTESIAN_POINT('Ctrl Pts',(44.2109953322312,-56.5108003631786,
-40.8704389119319));
#263352=CARTESIAN_POINT('Ctrl Pts',(44.2322091102727,-56.5122711761573,
-40.8847351429132));
#263353=CARTESIAN_POINT('Ctrl Pts',(44.2639028799147,-56.5152466319394,
-40.9065696963621));
#263354=CARTESIAN_POINT('Ctrl Pts',(44.305661850593,-56.5222422564611,-40.9372114433545));
#263355=CARTESIAN_POINT('Ctrl Pts',(44.346925841944,-56.532247127269,-40.9693597045385));
#263356=CARTESIAN_POINT('Ctrl Pts',(44.3673876336497,-56.53826115526,-40.9859357593442));
#263357=CARTESIAN_POINT('Ctrl Pts',(44.3877715667723,-56.5447901720246,
-41.0027718870644));
#263358=CARTESIAN_POINT('Ctrl Pts',(44.3979208506631,-56.5483132560745,
-41.0113182564434));
#263359=CARTESIAN_POINT('Ctrl Pts',(44.4179418071922,-56.5558066378292,
-41.02850287128));
#263360=CARTESIAN_POINT('Ctrl Pts',(44.4278499085732,-56.5597882829787,
-41.0371710128992));
#263361=CARTESIAN_POINT('Ctrl Pts',(44.4572364860018,-56.5724196473794,
-41.0633712499365));
#263362=CARTESIAN_POINT('Ctrl Pts',(44.4763932211824,-56.581758968269,-41.0811111519311));
#263363=CARTESIAN_POINT('Ctrl Pts',(44.5044772880921,-56.5971447477014,
-41.1081262866225));
#263364=CARTESIAN_POINT('Ctrl Pts',(44.5137271775895,-56.6025015227711,
-41.1171962449124));
#263365=CARTESIAN_POINT('Ctrl Pts',(44.5320183562985,-56.6136863880645,
-41.1354834617267));
#263366=CARTESIAN_POINT('Ctrl Pts',(44.5410031705763,-56.6194798267371,
-41.144644186283));
#263367=CARTESIAN_POINT('Ctrl Pts',(44.5674276642847,-56.6374191091633,
-41.1721205907467));
#263368=CARTESIAN_POINT('Ctrl Pts',(44.5843870769067,-56.6501457393646,
-41.1904750382678));
#263369=CARTESIAN_POINT('Ctrl Pts',(44.616987890196,-56.6770839740703,-41.2272237610649));
#263370=CARTESIAN_POINT('Ctrl Pts',(44.640458797708,-56.6984048650555,-41.2548228473058));
#263371=CARTESIAN_POINT('Ctrl Pts',(44.6624514458289,-56.7214114906953,
-41.2824783924342));
#263372=CARTESIAN_POINT('Ctrl Pts',(44.6767798128067,-56.7371294193188,
-41.3009283158679));
#263373=CARTESIAN_POINT('Ctrl Pts',(44.683774397772,-56.7451748501741,-41.3101557240219));
#263374=CARTESIAN_POINT('Ctrl Pts',(44.6940202659092,-56.7575442973705,
-41.324018848177));
#263375=CARTESIAN_POINT('Ctrl Pts',(44.6973914635031,-56.7617145235639,
-41.328639728599));
#263376=CARTESIAN_POINT('Ctrl Pts',(44.7040131878578,-56.770108052971,-41.3378361513053));
#263377=CARTESIAN_POINT('Ctrl Pts',(44.7072703203268,-56.7743392575068,
-41.3424205878605));
#263378=CARTESIAN_POINT('Ctrl Pts',(44.7168707027477,-56.7871217033085,
-41.3561177927451));
#263379=CARTESIAN_POINT('Ctrl Pts',(44.7230524906066,-56.7957731420119,
-41.3651872799216));
#263380=CARTESIAN_POINT('Ctrl Pts',(44.7409373255192,-56.8220955492914,
-41.3921945478314));
#263381=CARTESIAN_POINT('Ctrl Pts',(44.7575187561203,-56.8491712652862,
-41.4188207502394));
#263382=CARTESIAN_POINT('Ctrl Pts',(44.7770214494108,-56.88676384976,-41.453559097464));
#263383=CARTESIAN_POINT('Ctrl Pts',(44.7858965000619,-56.9060633365117,
-41.4706740459328));
#263384=CARTESIAN_POINT('Ctrl Pts',(44.7943266372896,-56.9256180211132,
-41.4876605613939));
#263385=CARTESIAN_POINT('Ctrl Pts',(44.7983169540911,-56.9355169983302,
-41.4960845962979));
#263386=CARTESIAN_POINT('Ctrl Pts',(44.8058516078422,-56.9556000996462,
-41.5128223385875));
#263387=CARTESIAN_POINT('Ctrl Pts',(44.8093727854448,-56.9657242505397,
-41.5210856532432));
#263388=CARTESIAN_POINT('Ctrl Pts',(44.8191505788346,-56.9961959016236,
-41.5454418374945));
#263389=CARTESIAN_POINT('Ctrl Pts',(44.8246597322132,-57.0167187198372,
-41.5611704866007));
#263390=CARTESIAN_POINT('Ctrl Pts',(44.8336688220904,-57.0581479791523,
-41.5916045035181));
#263391=CARTESIAN_POINT('Ctrl Pts',(44.8389236650083,-57.0895139074259,
-41.613669368427));
#263392=CARTESIAN_POINT('Ctrl Pts',(44.8418900765893,-57.1213299669285,
-41.6345866129535));
#263393=CARTESIAN_POINT('Ctrl Pts',(44.8433488372948,-57.142640498193,-41.6482710687869));
#263394=CARTESIAN_POINT('Ctrl Pts',(44.8438191277705,-57.1533552116615,
-41.6549890353504));
#263395=CARTESIAN_POINT('Ctrl Pts',(44.8442270800594,-57.1748537940466,
-41.6681388704993));
#263396=CARTESIAN_POINT('Ctrl Pts',(44.8441639040618,-57.1855561823783,
-41.6745213422017));
#263397=CARTESIAN_POINT('Ctrl Pts',(44.8435122114514,-57.2069000331791,
-41.6869277892926));
#263398=CARTESIAN_POINT('Ctrl Pts',(44.8417458896958,-57.2388084678274,
-41.7049896680882));
#263399=CARTESIAN_POINT('Ctrl Pts',(44.8362687719071,-57.2809279665006,
-41.7269106712316));
#263400=CARTESIAN_POINT('Ctrl Pts',(44.8298088085522,-57.3121969378441,
-41.7417325167562));
#263401=CARTESIAN_POINT('Ctrl Pts',(44.8249713776488,-57.3329705079708,
-41.751249414817));
#263402=CARTESIAN_POINT('Ctrl Pts',(44.8222858794974,-57.3433254378487,
-41.7558274666229));
#263403=CARTESIAN_POINT('Ctrl Pts',(44.8163797073795,-57.3639440769784,
-41.7646063213672));
#263404=CARTESIAN_POINT('Ctrl Pts',(44.8131427147447,-57.3742522416544,
-41.7688238948253));
#263405=CARTESIAN_POINT('Ctrl Pts',(44.8061917406462,-57.3945668799698,
-41.7767918599254));
#263406=CARTESIAN_POINT('Ctrl Pts',(44.7987498536529,-57.4146412549335,
-41.7843210101159));
#263407=CARTESIAN_POINT('Ctrl Pts',(44.7861419817956,-57.4440129710611,
-41.7943060987191));
#263408=CARTESIAN_POINT('Ctrl Pts',(44.7720982599006,-57.4726583092559,
-41.8029984035242));
#263409=CARTESIAN_POINT('Ctrl Pts',(44.7566193423106,-57.5005749992605,
-41.8103989883131));
#263410=CARTESIAN_POINT('Ctrl Pts',(44.7453362941317,-57.518697088903,-41.8144666236875));
#263411=CARTESIAN_POINT('Ctrl Pts',(44.7335642473644,-57.5365709174371,
-41.8180952379985));
#263412=CARTESIAN_POINT('Ctrl Pts',(44.7274378249752,-57.5453780864623,
-41.8196891344695));
#263413=CARTESIAN_POINT('Ctrl Pts',(44.7146685840676,-57.5627610237142,
-41.8224320230444));
#263414=CARTESIAN_POINT('Ctrl Pts',(44.7080700862024,-57.5712755128024,
-41.8235709343319));
#263415=CARTESIAN_POINT('Ctrl Pts',(44.6877341610586,-57.5961705213949,
-41.8262807978491));
#263416=CARTESIAN_POINT('Ctrl Pts',(44.6734117165454,-57.6119810052107,
-41.8271650529119));
#263417=CARTESIAN_POINT('Ctrl Pts',(44.6432859415473,-57.6420285404153,
-41.827118555904));
#263418=CARTESIAN_POINT('Ctrl Pts',(44.6274777219699,-57.6562729242579,
-41.8261892556471));
#263419=CARTESIAN_POINT('Ctrl Pts',(44.6026489360012,-57.6764545436153,
-41.823427013232));
#263420=CARTESIAN_POINT('Ctrl Pts',(44.5941811636919,-57.6829873126311,
-41.8222767907821));
#263421=CARTESIAN_POINT('Ctrl Pts',(44.5812011369499,-57.6924815728277,
-41.820204446988));
#263422=CARTESIAN_POINT('Ctrl Pts',(44.5768239301145,-57.6955981764101,
-41.8194549553751));
#263423=CARTESIAN_POINT('Ctrl Pts',(44.5679795363474,-57.7017261947271,
-41.8178398084084));
#263424=CARTESIAN_POINT('Ctrl Pts',(44.554547495243,-57.7107794649358,-41.8152360293365));
#263425=CARTESIAN_POINT('Ctrl Pts',(44.5408745509057,-57.7192473537464,
-41.812140181677));
#263426=CARTESIAN_POINT('Ctrl Pts',(44.5224181841827,-57.7300417662926,
-41.8075820007456));
#263427=CARTESIAN_POINT('Ctrl Pts',(44.494403164631,-57.7454824222945,-41.8000999642091));
#263428=CARTESIAN_POINT('Ctrl Pts',(44.4557509611988,-57.7631175354143,
-41.7875858630695));
#263429=CARTESIAN_POINT('Ctrl Pts',(44.4257963579031,-57.7741479888816,
-41.7763064650726));
#263430=CARTESIAN_POINT('Ctrl Pts',(44.4056101875344,-57.781009218212,-41.7683613570464));
#263431=CARTESIAN_POINT('Ctrl Pts',(44.3954036594654,-57.7841949818065,
-41.7641737395871));
#263432=CARTESIAN_POINT('Ctrl Pts',(44.3747925009816,-57.7900627169564,
-41.7553761870634));
#263433=CARTESIAN_POINT('Ctrl Pts',(44.3643365899562,-57.7927558542442,
-41.7507422904685));
#263434=CARTESIAN_POINT('Ctrl Pts',(44.3329536886806,-57.7999988857253,
-41.7363257213199));
#263435=CARTESIAN_POINT('Ctrl Pts',(44.3014645871824,-57.8056090798854,
-41.7208580810542));
#263436=CARTESIAN_POINT('Ctrl Pts',(44.2698183189435,-57.8088603667088,
-41.7038603653999));
#263437=CARTESIAN_POINT('Ctrl Pts',(44.2381206623806,-57.8113308880715,
-41.6863549522799));
#263438=CARTESIAN_POINT('Ctrl Pts',(44.2169139506954,-57.8119384373532,
-41.6740048606234));
#263439=CARTESIAN_POINT('Ctrl Pts',(44.1850197107514,-57.811287280344,-41.6544681547659));
#263440=CARTESIAN_POINT('Ctrl Pts',(44.1743613109546,-57.8108078241776,
-41.6477783242763));
#263441=CARTESIAN_POINT('Ctrl Pts',(44.1583626375358,-57.8096935003687,
-41.6374930176863));
#263442=CARTESIAN_POINT('Ctrl Pts',(44.1530230189312,-57.809255510817,-41.6340194660765));
#263443=CARTESIAN_POINT('Ctrl Pts',(44.1423341247923,-57.8082460206643,
-41.6269840076234));
#263444=CARTESIAN_POINT('Ctrl Pts',(44.1369894952372,-57.8076746784434,
-41.6234249849254));
#263445=CARTESIAN_POINT('Ctrl Pts',(44.1103928894951,-57.8045001122898,
-41.6055088472864));
#263446=CARTESIAN_POINT('Ctrl Pts',(44.0684216046586,-57.7973782151022,
-41.5759273380954));
#263447=CARTESIAN_POINT('Ctrl Pts',(44.0275807082801,-57.78632659952,-41.5445717124501));
#263448=CARTESIAN_POINT('Ctrl Pts',(43.9872978152183,-57.7733311875938,
-41.5123297976061));
#263449=CARTESIAN_POINT('Ctrl Pts',(43.9674326520914,-57.7658590768128,
-41.4957625032292));
#263450=CARTESIAN_POINT('Ctrl Pts',(43.942963744406,-57.7552890823142,-41.4744937232973));
#263451=CARTESIAN_POINT('Ctrl Pts',(43.938085174092,-57.7531113051098,-41.4702088025761));
#263452=CARTESIAN_POINT('Ctrl Pts',(43.9283699185172,-57.7486342535987,
-41.4615871928557));
#263453=CARTESIAN_POINT('Ctrl Pts',(43.9235236029976,-57.7463299238453,
-41.4572415669043));
#263454=CARTESIAN_POINT('Ctrl Pts',(43.9090930604083,-57.739254093668,-41.4441663196977));
#263455=CARTESIAN_POINT('Ctrl Pts',(43.8996324205383,-57.7343289686206,
-41.4354132012863));
#263456=CARTESIAN_POINT('Ctrl Pts',(43.8903154257419,-57.7291941381088,
-41.4266127101804));
#263457=CARTESIAN_POINT('',(43.5555682511181,-59.2341350312479,-39.6401231904583));
#263458=CARTESIAN_POINT('',(43.6172881206076,-58.9566576914661,-39.9695117808943));
#263459=CARTESIAN_POINT('',(43.5555682511181,-59.2341350312479,-39.6401231904583));
#263460=CARTESIAN_POINT('Ctrl Pts',(43.5555682511181,-59.2341350312479,
-39.6401231904583));
#263461=CARTESIAN_POINT('Ctrl Pts',(43.5840312864905,-59.2495486925951,
-39.6489236815643));
#263462=CARTESIAN_POINT('Ctrl Pts',(43.6129437448844,-59.2643132281768,
-39.6576767999753));
#263463=CARTESIAN_POINT('Ctrl Pts',(43.657060506721,-59.2854937757857,-39.6707520471821));
#263464=CARTESIAN_POINT('Ctrl Pts',(43.6718791845861,-59.2923859849247,
-39.6750976731336));
#263465=CARTESIAN_POINT('Ctrl Pts',(43.7015908821177,-59.3057655721158,
-39.6837192828541));
#263466=CARTESIAN_POINT('Ctrl Pts',(43.7165133310485,-59.3122681083841,
-39.6880042035746));
#263467=CARTESIAN_POINT('Ctrl Pts',(43.7913709620947,-59.3437990868819,
-39.7092729835095));
#263468=CARTESIAN_POINT('Ctrl Pts',(43.8521844391421,-59.3659929346427,
-39.7258402778837));
#263469=CARTESIAN_POINT('Ctrl Pts',(43.9755797709279,-59.4043781707975,
-39.7580821927283));
#263470=CARTESIAN_POINT('Ctrl Pts',(44.1007600202038,-59.4367761316392,
-39.7894378183729));
#263471=CARTESIAN_POINT('Ctrl Pts',(44.2295539029067,-59.457069607789,-39.8190193275642));
#263472=CARTESIAN_POINT('Ctrl Pts',(44.3112153059959,-59.4658206541325,
-39.8369354652031));
#263473=CARTESIAN_POINT('Ctrl Pts',(44.3276276091643,-59.4673747774113,
-39.8404944879015));
#263474=CARTESIAN_POINT('Ctrl Pts',(44.36045571594,-59.4700741717846,-39.8475299463542));
#263475=CARTESIAN_POINT('Ctrl Pts',(44.3768572408897,-59.4712191302958,
-39.8510034979643));
#263476=CARTESIAN_POINT('Ctrl Pts',(44.426006678754,-59.4740418999023,-39.8612888045543));
#263477=CARTESIAN_POINT('Ctrl Pts',(44.4587593954789,-59.4751153687477,
-39.8679786350438));
#263478=CARTESIAN_POINT('Ctrl Pts',(44.5567957957571,-59.4759221534093,
-39.8875153409015));
#263479=CARTESIAN_POINT('Ctrl Pts',(44.6220168026294,-59.4732643557565,
-39.8998654325577));
#263480=CARTESIAN_POINT('Ctrl Pts',(44.7195562226364,-59.4644947877976,
-39.9173708456776));
#263481=CARTESIAN_POINT('Ctrl Pts',(44.8169644551499,-59.4533300166017,
-39.9343685613317));
#263482=CARTESIAN_POINT('Ctrl Pts',(44.913970347279,-59.4349282908675,-39.9498362015981));
#263483=CARTESIAN_POINT('Ctrl Pts',(45.0107056952338,-59.411516304601,-39.9642527707462));
#263484=CARTESIAN_POINT('Ctrl Pts',(45.0429448249416,-59.4028563587456,
-39.9688866673415));
#263485=CARTESIAN_POINT('Ctrl Pts',(45.1065152212723,-59.3840690317117,
-39.9776842198647));
#263486=CARTESIAN_POINT('Ctrl Pts',(45.1380045334646,-59.373905450928,-39.9818718373241));
#263487=CARTESIAN_POINT('Ctrl Pts',(45.200302444735,-59.3520826555278,-39.9898169453504));
#263488=CARTESIAN_POINT('Ctrl Pts',(45.2833557066068,-59.320656673229,-39.9999472459813));
#263489=CARTESIAN_POINT('Ctrl Pts',(45.364075785606,-59.2838188850366,-40.0085499382911));
#263490=CARTESIAN_POINT('Ctrl Pts',(45.4139072224687,-59.2584967483865,
-40.0133526723911));
#263491=CARTESIAN_POINT('Ctrl Pts',(45.4139074558404,-59.258497391876,-40.0133531717389));
#263492=CARTESIAN_POINT('Ctrl Pts',(45.2555531699078,-59.3224601009847,
-40.0137109606119));
#263493=CARTESIAN_POINT('Ctrl Pts',(45.0886088759217,-59.362243913815,-40.0125039011494));
#263494=CARTESIAN_POINT('Ctrl Pts',(44.7703416864287,-59.3897953534914,
-40.007848919862));
#263495=CARTESIAN_POINT('Ctrl Pts',(44.6212948829819,-59.383482606722,-40.0047256760571));
#263496=CARTESIAN_POINT('Ctrl Pts',(44.3078241746654,-59.3300095393333,
-39.9965299346065));
#263497=CARTESIAN_POINT('Ctrl Pts',(44.1460848365945,-59.2776316689425,
-39.9912944612456));
#263498=CARTESIAN_POINT('Ctrl Pts',(43.8182442761428,-59.1175558791083,
-39.9789555992433));
#263499=CARTESIAN_POINT('Ctrl Pts',(43.6926832053086,-59.0208412827663,
-39.9730690294287));
#263500=CARTESIAN_POINT('Ctrl Pts',(43.6172881206077,-58.9566576914661,
-39.9695117808943));
#263501=CARTESIAN_POINT('Ctrl Pts',(43.4805771074156,-59.5712767529309,
-39.2399080357013));
#263502=CARTESIAN_POINT('Ctrl Pts',(43.4150727209207,-59.5358440364426,
-39.2223070534893));
#263503=CARTESIAN_POINT('Ctrl Pts',(43.2883193276586,-59.4590682572254,
-39.1867578392588));
#263504=CARTESIAN_POINT('Ctrl Pts',(43.1106712693135,-59.32658002426,-39.1324031814995));
#263505=CARTESIAN_POINT('Ctrl Pts',(43.0005921597408,-59.2266373021163,
-39.0954660506179));
#263506=CARTESIAN_POINT('Ctrl Pts',(42.8948534568781,-59.1207134074407,
-39.0581733199915));
#263507=CARTESIAN_POINT('Ctrl Pts',(42.7951360401793,-59.0104958554849,
-39.0211184761739));
#263508=CARTESIAN_POINT('Ctrl Pts',(42.6850011896347,-58.8622904152127,
-38.9753582681256));
#263509=CARTESIAN_POINT('Ctrl Pts',(42.6055727997797,-58.7375004045667,
-38.939089851323));
#263510=CARTESIAN_POINT('Ctrl Pts',(42.5503788594446,-58.6407591922129,
-38.9120596161462));
#263511=CARTESIAN_POINT('Ctrl Pts',(42.5165536369311,-58.5741539171446,
-38.8941613358138));
#263512=CARTESIAN_POINT('Ctrl Pts',(42.4842288567228,-58.5064298632496,
-38.8763157156907));
#263513=CARTESIAN_POINT('Ctrl Pts',(42.4689425396028,-58.4722695523732,
-38.8674882509199));
#263514=CARTESIAN_POINT('Ctrl Pts',(42.4257123024776,-58.3690064948315,
-38.8413136266604));
#263515=CARTESIAN_POINT('Ctrl Pts',(42.3750272156063,-58.229152189777,-38.8072100415055));
#263516=CARTESIAN_POINT('Ctrl Pts',(42.3380647902547,-58.0850119200902,
-38.7746901633276));
#263517=CARTESIAN_POINT('Ctrl Pts',(42.3155659796374,-57.9752818499468,
-38.7509105250088));
#263518=CARTESIAN_POINT('Ctrl Pts',(42.3089374211558,-57.9384266221928,
-38.7430843922672));
#263519=CARTESIAN_POINT('Ctrl Pts',(42.297458012674,-57.864178756387,-38.7276438637217));
#263520=CARTESIAN_POINT('Ctrl Pts',(42.292601515188,-57.8267325312259,-38.720018782004));
#263521=CARTESIAN_POINT('Ctrl Pts',(42.2847289916893,-57.7514526301959,
-38.7050196673963));
#263522=CARTESIAN_POINT('Ctrl Pts',(42.2817363521424,-57.7138759968928,
-38.6976962453237));
#263523=CARTESIAN_POINT('Ctrl Pts',(42.277596992864,-57.6387184974263,-38.6833720377019));
#263524=CARTESIAN_POINT('Ctrl Pts',(42.2741651307842,-57.5260409596698,
-38.6623829091612));
#263525=CARTESIAN_POINT('Ctrl Pts',(42.2805893100654,-57.3760354719141,
-38.6363740800325));
#263526=CARTESIAN_POINT('Ctrl Pts',(42.2937061680812,-57.2637038035873,
-38.618370061439));
#263527=CARTESIAN_POINT('Ctrl Pts',(42.3043247017591,-57.1888547452426,
-38.6067079534822));
#263528=CARTESIAN_POINT('Ctrl Pts',(42.3105743117123,-57.1514345461221,
-38.6010450635964));
#263529=CARTESIAN_POINT('Ctrl Pts',(42.3249704170347,-57.0766935209607,
-38.590076215021));
#263530=CARTESIAN_POINT('Ctrl Pts',(42.3331592025312,-57.0392159768686,
-38.5847494243559));
#263531=CARTESIAN_POINT('Ctrl Pts',(42.3512949844302,-56.9651221381903,
-38.5745673038812));
#263532=CARTESIAN_POINT('Ctrl Pts',(42.3712216906218,-56.8916587034686,
-38.564820665347));
#263533=CARTESIAN_POINT('Ctrl Pts',(42.4063979707918,-56.7834465224234,
-38.5515118436));
#263534=CARTESIAN_POINT('Ctrl Pts',(42.4468320479729,-56.6771725078319,
-38.5395042677724));
#263535=CARTESIAN_POINT('Ctrl Pts',(42.4925290654744,-56.5728473165674,
-38.5288039137004));
#263536=CARTESIAN_POINT('Ctrl Pts',(42.5265325119253,-56.5046058456765,
-38.5225509073062));
#263537=CARTESIAN_POINT('Ctrl Pts',(42.5623338475306,-56.4370293947697,
-38.5167461666044));
#263538=CARTESIAN_POINT('Ctrl Pts',(42.5811223641794,-56.4035923099625,
-38.5140693065785));
#263539=CARTESIAN_POINT('Ctrl Pts',(42.620584523009,-56.3373241998654,-38.5091697400817));
#263540=CARTESIAN_POINT('Ctrl Pts',(42.6411082254821,-56.3047465904101,
-38.5069659500128));
#263541=CARTESIAN_POINT('Ctrl Pts',(42.7048067991197,-56.2090283357163,
-38.501110858935));
#263542=CARTESIAN_POINT('Ctrl Pts',(42.7502234543428,-56.1476408662828,
-38.4981890389281));
#263543=CARTESIAN_POINT('Ctrl Pts',(42.8467942323831,-56.0297655581676,
-38.4942910511033));
#263544=CARTESIAN_POINT('Ctrl Pts',(42.8979715413934,-55.9732420482176,
-38.4933125989996));
#263545=CARTESIAN_POINT('Ctrl Pts',(42.9790570553347,-55.8921695883033,
-38.4933149859729));
#263546=CARTESIAN_POINT('Ctrl Pts',(43.0068374106561,-55.8657400908868,
-38.4935622007431));
#263547=CARTESIAN_POINT('Ctrl Pts',(43.0495800649421,-55.8270637749536,
-38.4943063068789));
#263548=CARTESIAN_POINT('Ctrl Pts',(43.0640222060113,-55.8143203511958,
-38.494617152342));
#263549=CARTESIAN_POINT('Ctrl Pts',(43.0932714774893,-55.7891564261061,
-38.4953646906773));
#263550=CARTESIAN_POINT('Ctrl Pts',(43.1080901283632,-55.7767277938553,
-38.4958020036096));
#263551=CARTESIAN_POINT('Ctrl Pts',(43.1528523310046,-55.7401327167866,
-38.4972962980169));
#263552=CARTESIAN_POINT('Ctrl Pts',(43.2134913856688,-55.6930468850421,
-38.4997758707861));
#263553=CARTESIAN_POINT('Ctrl Pts',(43.3385569247743,-55.6055389451161,
-38.5066450244003));
#263554=CARTESIAN_POINT('Ctrl Pts',(43.4691986576013,-55.5278792007279,
-38.5163302992824));
#263555=CARTESIAN_POINT('Ctrl Pts',(43.5713395927684,-55.4769743237494,
-38.5256877381308));
#263556=CARTESIAN_POINT('Ctrl Pts',(43.6403672861995,-55.4446857735354,
-38.5323951500278));
#263557=CARTESIAN_POINT('Ctrl Pts',(43.6753577685123,-55.4293620157832,
-38.5359845633874));
#263558=CARTESIAN_POINT('Ctrl Pts',(43.7462462065788,-55.4003985583156,
-38.5436333065981));
#263559=CARTESIAN_POINT('Ctrl Pts',(43.7822717759725,-55.3867204456352,
-38.5477088862383));
#263560=CARTESIAN_POINT('Ctrl Pts',(43.8543821738219,-55.3613797848081,
-38.5562346427694));
#263561=CARTESIAN_POINT('Ctrl Pts',(43.890622407919,-55.349649082917,-38.5607007444526));
#263562=CARTESIAN_POINT('Ctrl Pts',(43.9997560709039,-55.3172704656441,
-38.5746802407103));
#263563=CARTESIAN_POINT('Ctrl Pts',(44.1098017310836,-55.290468361793,-38.5898286859852));
#263564=CARTESIAN_POINT('Ctrl Pts',(44.2583166685835,-55.2656490138239,
-38.612301023075));
#263565=CARTESIAN_POINT('Ctrl Pts',(44.3705972700495,-55.2524997368729,
-38.6302900391873));
#263566=CARTESIAN_POINT('Ctrl Pts',(44.446056048267,-55.2474029004138,-38.6430428201589));
#263567=CARTESIAN_POINT('Ctrl Pts',(44.5218128020516,-55.2441636366351,
-38.65617756452));
#263568=CARTESIAN_POINT('Ctrl Pts',(44.5599089424743,-55.2434808562086,
-38.6629497802385));
#263569=CARTESIAN_POINT('Ctrl Pts',(44.6354869543582,-55.2439911084578,
-38.6767130108817));
#263570=CARTESIAN_POINT('Ctrl Pts',(44.6731456892459,-55.2451740103824,
-38.6837342374529));
#263571=CARTESIAN_POINT('Ctrl Pts',(44.7481014788608,-55.2493620066237,
-38.6980304684339));
#263572=CARTESIAN_POINT('Ctrl Pts',(44.860046548974,-55.2583760573225,-38.7198650218829));
#263573=CARTESIAN_POINT('Ctrl Pts',(45.0073845433675,-55.2811507310277,
-38.7505067688753));
#263574=CARTESIAN_POINT('Ctrl Pts',(45.1528189888476,-55.3146135839333,
-38.7826550300594));
#263575=CARTESIAN_POINT('Ctrl Pts',(45.2248832056965,-55.3349380951144,
-38.7992310848652));
#263576=CARTESIAN_POINT('Ctrl Pts',(45.2966462681613,-55.3570913336823,
-38.8160672125853));
#263577=CARTESIAN_POINT('Ctrl Pts',(45.3323638946335,-55.3690863290504,
-38.8246135819642));
#263578=CARTESIAN_POINT('Ctrl Pts',(45.4027951436545,-55.3946744461232,
-38.841798196801));
#263579=CARTESIAN_POINT('Ctrl Pts',(45.4376370321487,-55.4083060218429,
-38.85046633842));
#263580=CARTESIAN_POINT('Ctrl Pts',(45.5409345111852,-55.4516493275196,
-38.8766665754573));
#263581=CARTESIAN_POINT('Ctrl Pts',(45.6082182891413,-55.4838201174091,
-38.8944064774514));
#263582=CARTESIAN_POINT('Ctrl Pts',(45.7067749877369,-55.5369855856676,
-38.9214216121435));
#263583=CARTESIAN_POINT('Ctrl Pts',(45.7392219877795,-55.5555212114618,
-38.9304915704334));
#263584=CARTESIAN_POINT('Ctrl Pts',(45.8033556832395,-55.5942722159849,
-38.9487787872477));
#263585=CARTESIAN_POINT('Ctrl Pts',(45.8348443691401,-55.6143675312756,
-38.9579395118015));
#263586=CARTESIAN_POINT('Ctrl Pts',(45.9274099842789,-55.6766589025306,
-38.9854159162723));
#263587=CARTESIAN_POINT('Ctrl Pts',(45.9867610865919,-55.7209353156014,
-39.0037703637879));
#263588=CARTESIAN_POINT('Ctrl Pts',(46.1007337830098,-55.8148102393793,
-39.0405190865864));
#263589=CARTESIAN_POINT('Ctrl Pts',(46.1826971388658,-55.889219933262,-39.0681181728269));
#263590=CARTESIAN_POINT('Ctrl Pts',(46.259356574729,-55.9696687352924,-39.0957737179551));
#263591=CARTESIAN_POINT('Ctrl Pts',(46.309266807939,-56.024663053365,-39.1142236413887));
#263592=CARTESIAN_POINT('Ctrl Pts',(46.3336138177017,-56.0528284109483,
-39.1234510495426));
#263593=CARTESIAN_POINT('Ctrl Pts',(46.3692509284248,-56.0961546965833,
-39.1373141736981));
#263594=CARTESIAN_POINT('Ctrl Pts',(46.3809719555493,-56.1107655250657,
-39.14193505412));
#263595=CARTESIAN_POINT('Ctrl Pts',(46.4039850968433,-56.1401806715041,
-39.1511314768264));
#263596=CARTESIAN_POINT('Ctrl Pts',(46.4153001903629,-56.1550126624776,
-39.1557159133813));
#263597=CARTESIAN_POINT('Ctrl Pts',(46.4486370096885,-56.1998310060263,
-39.1694131182659));
#263598=CARTESIAN_POINT('Ctrl Pts',(46.4700835091466,-56.2301795317326,
-39.1784826054425));
#263599=CARTESIAN_POINT('Ctrl Pts',(46.532071913686,-56.3225583984772,-39.2054898733524));
#263600=CARTESIAN_POINT('Ctrl Pts',(46.5894197348374,-56.4176636744323,
-39.23211607576));
#263601=CARTESIAN_POINT('Ctrl Pts',(46.6566074362748,-56.5498680842415,
-39.2668544229849));
#263602=CARTESIAN_POINT('Ctrl Pts',(46.6870820302515,-56.617790568625,-39.2839693714534));
#263603=CARTESIAN_POINT('Ctrl Pts',(46.7159729830272,-56.6866360545619,
-39.3009558869148));
#263604=CARTESIAN_POINT('Ctrl Pts',(46.7296188023799,-56.7214992889704,
-39.3093799218186));
#263605=CARTESIAN_POINT('Ctrl Pts',(46.7553216997643,-56.7922546384013,
-39.3261176641085));
#263606=CARTESIAN_POINT('Ctrl Pts',(46.7672996943011,-56.8279354881579,
-39.3343809787628));
#263607=CARTESIAN_POINT('Ctrl Pts',(46.8004530502947,-56.9353633959568,
-39.358737163018));
#263608=CARTESIAN_POINT('Ctrl Pts',(46.8189795501832,-57.0077635587999,
-39.3744658121213));
#263609=CARTESIAN_POINT('Ctrl Pts',(46.848916211803,-57.1540080946302,-39.4048998290393));
#263610=CARTESIAN_POINT('Ctrl Pts',(46.866048617508,-57.2647966217996,-39.4269646939479));
#263611=CARTESIAN_POINT('Ctrl Pts',(46.875074749658,-57.3772756893033,-39.4478819384746));
#263612=CARTESIAN_POINT('Ctrl Pts',(46.8792542953452,-57.4526370309597,
-39.4615663943076));
#263613=CARTESIAN_POINT('Ctrl Pts',(46.8804258736835,-57.4905390832845,
-39.4682843608713));
#263614=CARTESIAN_POINT('Ctrl Pts',(46.8808837743635,-57.566610437341,-39.4814341960201));
#263615=CARTESIAN_POINT('Ctrl Pts',(46.8801708637706,-57.604491394965,-39.4878166677226));
#263616=CARTESIAN_POINT('Ctrl Pts',(46.8768913879562,-57.6800597985945,
-39.5002231148134));
#263617=CARTESIAN_POINT('Ctrl Pts',(46.8691896925243,-57.7930657109158,
-39.5182849936093));
#263618=CARTESIAN_POINT('Ctrl Pts',(46.8479069711518,-57.9423669591112,
-39.540205996752));
#263619=CARTESIAN_POINT('Ctrl Pts',(46.8236459543104,-58.053306681129,-39.5550278422771));
#263620=CARTESIAN_POINT('Ctrl Pts',(46.8055990109883,-58.1270324939452,
-39.5645447403379));
#263621=CARTESIAN_POINT('Ctrl Pts',(46.7956339676918,-58.1637938532181,
-39.5691227921436));
#263622=CARTESIAN_POINT('Ctrl Pts',(46.7738161327052,-58.2370162077019,
-39.5779016468881));
#263623=CARTESIAN_POINT('Ctrl Pts',(46.7619036278491,-58.2736352268715,
-39.5821192203466));
#263624=CARTESIAN_POINT('Ctrl Pts',(46.7364059718256,-58.3458255995332,
-39.5900871854462));
#263625=CARTESIAN_POINT('Ctrl Pts',(46.7091836493705,-58.4171862986019,
-39.5976163356366));
#263626=CARTESIAN_POINT('Ctrl Pts',(46.663274408039,-58.5216699086648,-39.6076014242402));
#263627=CARTESIAN_POINT('Ctrl Pts',(46.6123207377325,-58.6236436013082,
-39.616293729045));
#263628=CARTESIAN_POINT('Ctrl Pts',(46.5563244858032,-58.7230996041114,
-39.6236943138341));
#263629=CARTESIAN_POINT('Ctrl Pts',(46.515607032986,-58.7877140896312,-39.6277619492082));
#263630=CARTESIAN_POINT('Ctrl Pts',(46.4731710833873,-58.8514710047945,
-39.6313905635194));
#263631=CARTESIAN_POINT('Ctrl Pts',(46.4511086137465,-58.8829006319494,
-39.6329844599904));
#263632=CARTESIAN_POINT('Ctrl Pts',(46.4051673201274,-58.9449633016888,
-39.6357273485653));
#263633=CARTESIAN_POINT('Ctrl Pts',(46.381447994276,-58.975377588932,-39.6368662598532));
#263634=CARTESIAN_POINT('Ctrl Pts',(46.3084068909562,-59.0643493136614,
-39.6395761233691));
#263635=CARTESIAN_POINT('Ctrl Pts',(46.2570407846102,-59.1209150453974,
-39.6404603784325));
#263636=CARTESIAN_POINT('Ctrl Pts',(46.1491379755941,-59.228544463199,-39.6404138814247));
#263637=CARTESIAN_POINT('Ctrl Pts',(46.0925836555155,-59.2796343044913,
-39.6394845811684));
#263638=CARTESIAN_POINT('Ctrl Pts',(46.0038529437629,-59.3521266125547,
-39.6367223387528));
#263639=CARTESIAN_POINT('Ctrl Pts',(45.9736068078661,-59.3756113554055,
-39.6355721163029));
#263640=CARTESIAN_POINT('Ctrl Pts',(45.9272656961273,-59.4097723546528,
-39.6334997725088));
#263641=CARTESIAN_POINT('Ctrl Pts',(45.9116419215573,-59.4209912820171,
-39.6327502808957));
#263642=CARTESIAN_POINT('Ctrl Pts',(45.8800804794677,-59.4430610802669,
-39.6311351339295));
#263643=CARTESIAN_POINT('Ctrl Pts',(45.8321587971618,-59.4756823489919,
-39.628531354857));
#263644=CARTESIAN_POINT('Ctrl Pts',(45.7834097108732,-59.5062438963941,
-39.6254355071979));
#263645=CARTESIAN_POINT('Ctrl Pts',(45.717633106262,-59.5452481912826,-39.6208773262667));
#263646=CARTESIAN_POINT('Ctrl Pts',(45.6178307490054,-59.601113548897,-39.6133952897297));
#263647=CARTESIAN_POINT('Ctrl Pts',(45.4802897643185,-59.6652183443042,
-39.6008811885904));
#263648=CARTESIAN_POINT('Ctrl Pts',(45.3738098009101,-59.7055766782111,
-39.5896017905935));
#263649=CARTESIAN_POINT('Ctrl Pts',(45.3020778813705,-59.7307512119865,
-39.5816566825671));
#263650=CARTESIAN_POINT('Ctrl Pts',(45.2658207311094,-59.7424779859237,
-39.5774690651077));
#263651=CARTESIAN_POINT('Ctrl Pts',(45.1926264675053,-59.7641596016776,
-39.5686715125846));
#263652=CARTESIAN_POINT('Ctrl Pts',(45.1555073907618,-59.7741562512684,
-39.5640376159893));
#263653=CARTESIAN_POINT('Ctrl Pts',(45.0441315765335,-59.8011904590316,
-39.5496210468413));
#263654=CARTESIAN_POINT('Ctrl Pts',(44.9324484012679,-59.8224577850013,
-39.5341534065747));
#263655=CARTESIAN_POINT('Ctrl Pts',(44.8203079610257,-59.8353953605365,
-39.5171556909205));
#263656=CARTESIAN_POINT('Ctrl Pts',(44.7080184564226,-59.8455760612675,
-39.4996502778008));
#263657=CARTESIAN_POINT('Ctrl Pts',(44.6329372249224,-59.8486931621852,
-39.4873001861445));
#263658=CARTESIAN_POINT('Ctrl Pts',(44.5200834441659,-59.8478515133141,
-39.4677634802869));
#263659=CARTESIAN_POINT('Ctrl Pts',(44.4823810871712,-59.8466449718289,
-39.4610736497974));
#263660=CARTESIAN_POINT('Ctrl Pts',(44.4258051079382,-59.8434394706745,
-39.4507883432074));
#263661=CARTESIAN_POINT('Ctrl Pts',(44.4069254589855,-59.8421361346926,
-39.4473147915973));
#263662=CARTESIAN_POINT('Ctrl Pts',(44.3691376542581,-59.8390581625153,
-39.4402793331445));
#263663=CARTESIAN_POINT('Ctrl Pts',(44.3502459350849,-59.8372838734483,
-39.4367203104461));
#263664=CARTESIAN_POINT('Ctrl Pts',(44.2562487381671,-59.8272835659938,
-39.4188041728073));
#263665=CARTESIAN_POINT('Ctrl Pts',(44.1080045765469,-59.8040393501646,
-39.3892226636159));
#263666=CARTESIAN_POINT('Ctrl Pts',(43.9639303529155,-59.7668593120831,
-39.3578670379715));
#263667=CARTESIAN_POINT('Ctrl Pts',(43.8219159040518,-59.7227861654643,
-39.3256251231267));
#263668=CARTESIAN_POINT('Ctrl Pts',(43.7519290534068,-59.6972943066161,
-39.3090578287531));
#263669=CARTESIAN_POINT('Ctrl Pts',(43.665783177736,-59.6610675807531,-39.2877890488175));
#263670=CARTESIAN_POINT('Ctrl Pts',(43.6486106666635,-59.653596197985,-39.2835041280971));
#263671=CARTESIAN_POINT('Ctrl Pts',(43.6144193015916,-59.6382222359849,
-39.2748825183767));
#263672=CARTESIAN_POINT('Ctrl Pts',(43.597366582891,-59.6303022352814,-39.2705368924251));
#263673=CARTESIAN_POINT('Ctrl Pts',(43.5465994182959,-59.605961903298,-39.2574616452183));
#263674=CARTESIAN_POINT('Ctrl Pts',(43.513329300663,-59.588993111175,-39.2487085268073));
#263675=CARTESIAN_POINT('Ctrl Pts',(43.4805771074156,-59.5712767529309,
-39.2399080357013));
#263676=CARTESIAN_POINT('Ctrl Pts',(43.8903154257419,-57.7291941381088,
-41.4266127101804));
#263677=CARTESIAN_POINT('Ctrl Pts',(43.8716814361492,-57.7189244770852,
-41.4090117279687));
#263678=CARTESIAN_POINT('Ctrl Pts',(43.8355945080866,-57.6967277837834,
-41.3734625137379));
#263679=CARTESIAN_POINT('Ctrl Pts',(43.7849271573585,-57.6585752750105,
-41.3191078559793));
#263680=CARTESIAN_POINT('Ctrl Pts',(43.753465403225,-57.62988352171,-41.2821707250961));
#263681=CARTESIAN_POINT('Ctrl Pts',(43.7232071092872,-57.5995155202448,
-41.2448779944712));
#263682=CARTESIAN_POINT('Ctrl Pts',(43.694633283399,-57.5679550683129,-41.2078231506529));
#263683=CARTESIAN_POINT('Ctrl Pts',(43.6629744005209,-57.5256074013359,
-41.162062942605));
#263684=CARTESIAN_POINT('Ctrl Pts',(43.6400741040405,-57.4900012877665,
-41.1257945258022));
#263685=CARTESIAN_POINT('Ctrl Pts',(43.624122646482,-57.4624228770549,-41.0987642906252));
#263686=CARTESIAN_POINT('Ctrl Pts',(43.6143188854815,-57.4434516436916,
-41.0808660102928));
#263687=CARTESIAN_POINT('Ctrl Pts',(43.6049343759216,-57.4241698350281,
-41.0630203901697));
#263688=CARTESIAN_POINT('Ctrl Pts',(43.6004882740613,-57.4144479878336,
-41.054192925399));
#263689=CARTESIAN_POINT('Ctrl Pts',(43.5878889573419,-57.3850715912746,
-41.0280183011396));
#263690=CARTESIAN_POINT('Ctrl Pts',(43.5730447416356,-57.3453166524842,
-40.9939147159844));
#263691=CARTESIAN_POINT('Ctrl Pts',(43.5620571572655,-57.3044044614592,
-40.9613948378065));
#263692=CARTESIAN_POINT('Ctrl Pts',(43.5552843243605,-57.2732819874194,
-40.9376151994878));
#263693=CARTESIAN_POINT('Ctrl Pts',(43.5532714802541,-57.2628325912303,
-40.9297890667463));
#263694=CARTESIAN_POINT('Ctrl Pts',(43.5497454556161,-57.2417890776549,
-40.9143485382007));
#263695=CARTESIAN_POINT('Ctrl Pts',(43.5482304746054,-57.2311797832666,
-40.9067234564832));
#263696=CARTESIAN_POINT('Ctrl Pts',(43.5457184756399,-57.2098591834555,
-40.8917243418755));
#263697=CARTESIAN_POINT('Ctrl Pts',(43.5447290487245,-57.199220662917,-40.8844009198028));
#263698=CARTESIAN_POINT('Ctrl Pts',(43.5432711863927,-57.1779500447907,
-40.8700767121812));
#263699=CARTESIAN_POINT('Ctrl Pts',(43.5418684734652,-57.1460721839032,
-40.8490875836402));
#263700=CARTESIAN_POINT('Ctrl Pts',(43.5431039253892,-57.1036793909824,
-40.8230787545116));
#263701=CARTESIAN_POINT('Ctrl Pts',(43.5463738329101,-57.0719682486671,
-40.8050747359183));
#263702=CARTESIAN_POINT('Ctrl Pts',(43.5490829635055,-57.0508462881094,
-40.7934126279614));
#263703=CARTESIAN_POINT('Ctrl Pts',(43.5507030159248,-57.0402904723448,
-40.7877497380755));
#263704=CARTESIAN_POINT('Ctrl Pts',(43.5544790630841,-57.019214904491,-40.7767808895002));
#263705=CARTESIAN_POINT('Ctrl Pts',(43.5566463931059,-57.0086510117152,
-40.7714540988351));
#263706=CARTESIAN_POINT('Ctrl Pts',(43.5614808344627,-56.9877741662596,
-40.7612719783604));
#263707=CARTESIAN_POINT('Ctrl Pts',(43.5668234022498,-56.9670831174431,
-40.7515253398262));
#263708=CARTESIAN_POINT('Ctrl Pts',(43.5763377125496,-56.9366295208774,
-40.7382165180791));
#263709=CARTESIAN_POINT('Ctrl Pts',(43.5873444561754,-56.9067460923864,
-40.7262089422516));
#263710=CARTESIAN_POINT('Ctrl Pts',(43.5998453117462,-56.8774358278222,
-40.7155085881795));
#263711=CARTESIAN_POINT('Ctrl Pts',(43.6091839698139,-56.8582805167828,
-40.7092555817853));
#263712=CARTESIAN_POINT('Ctrl Pts',(43.6190331668358,-56.8393207538612,
-40.7034508410834));
#263713=CARTESIAN_POINT('Ctrl Pts',(43.6242099732076,-56.8299438685379,
-40.7007739810578));
#263714=CARTESIAN_POINT('Ctrl Pts',(43.6350986096338,-56.8113693026126,
-40.6958744145609));
#263715=CARTESIAN_POINT('Ctrl Pts',(43.6407690742328,-56.8022426567881,
-40.6936706244929));
#263716=CARTESIAN_POINT('Ctrl Pts',(43.6583896223854,-56.7754411523649,
-40.6878155334118));
#263717=CARTESIAN_POINT('Ctrl Pts',(43.6709801307092,-56.7582712890167,
-40.6848937134075));
#263718=CARTESIAN_POINT('Ctrl Pts',(43.6978023804218,-56.725340315416,-40.6809957255822));
#263719=CARTESIAN_POINT('Ctrl Pts',(43.7120405319879,-56.7095692151415,
-40.6800172734785));
#263720=CARTESIAN_POINT('Ctrl Pts',(43.7346338722206,-56.6869796178674,
-40.680019660452));
#263721=CARTESIAN_POINT('Ctrl Pts',(43.7423799312797,-56.6796208977126,
-40.6802668752224));
#263722=CARTESIAN_POINT('Ctrl Pts',(43.7543060585229,-56.6688607312791,
-40.681010981358));
#263723=CARTESIAN_POINT('Ctrl Pts',(43.7583370517177,-56.6653168192219,
-40.6813218268212));
#263724=CARTESIAN_POINT('Ctrl Pts',(43.7665035456834,-56.6583217341419,
-40.6820693651562));
#263725=CARTESIAN_POINT('Ctrl Pts',(43.7706422703,-56.6548683091639,-40.6825066780886));
#263726=CARTESIAN_POINT('Ctrl Pts',(43.7831478581881,-56.6447045100584,
-40.6840009724959));
#263727=CARTESIAN_POINT('Ctrl Pts',(43.8000992888712,-56.6316392340345,
-40.6864805452653));
#263728=CARTESIAN_POINT('Ctrl Pts',(43.8351004518507,-56.6074069729907,
-40.6933496988796));
#263729=CARTESIAN_POINT('Ctrl Pts',(43.8717190640765,-56.5859796680779,
-40.7030349737613));
#263730=CARTESIAN_POINT('Ctrl Pts',(43.9003898794618,-56.5719991465823,
-40.7123924126099));
#263731=CARTESIAN_POINT('Ctrl Pts',(43.919774692733,-56.5631479893168,-40.719099824507));
#263732=CARTESIAN_POINT('Ctrl Pts',(43.9296053152689,-56.5589560552736,
-40.722689237866));
#263733=CARTESIAN_POINT('Ctrl Pts',(43.9495302416178,-56.551051384942,-40.7303379810773));
#263734=CARTESIAN_POINT('Ctrl Pts',(43.959660471973,-56.5473282955902,-40.7344135607172));
#263735=CARTESIAN_POINT('Ctrl Pts',(43.9799461530017,-56.5404515818703,
-40.7429393172485));
#263736=CARTESIAN_POINT('Ctrl Pts',(43.9901452646573,-56.5372793127045,
-40.7474054189318));
#263737=CARTESIAN_POINT('Ctrl Pts',(44.0208712025373,-56.5285586047056,
-40.7613849151889));
#263738=CARTESIAN_POINT('Ctrl Pts',(44.0518784813599,-56.521416173947,-40.7765333604643));
#263739=CARTESIAN_POINT('Ctrl Pts',(44.0937728041468,-56.5149820273198,
-40.799005697554));
#263740=CARTESIAN_POINT('Ctrl Pts',(44.1254693703652,-56.5117027703592,
-40.8169947136667));
#263741=CARTESIAN_POINT('Ctrl Pts',(44.1467868482481,-56.5105547568045,
-40.8297474946377));
#263742=CARTESIAN_POINT('Ctrl Pts',(44.1681963264173,-56.50993223545,-40.842882238999));
#263743=CARTESIAN_POINT('Ctrl Pts',(44.1789665479467,-56.509886262238,-40.8496544547178));
#263744=CARTESIAN_POINT('Ctrl Pts',(44.2003410646824,-56.5103214152413,
-40.8634176853611));
#263745=CARTESIAN_POINT('Ctrl Pts',(44.2109953322312,-56.5108003631786,
-40.8704389119319));
#263746=CARTESIAN_POINT('Ctrl Pts',(44.2322091102727,-56.5122711761573,
-40.8847351429132));
#263747=CARTESIAN_POINT('Ctrl Pts',(44.2639028799147,-56.5152466319394,
-40.9065696963621));
#263748=CARTESIAN_POINT('Ctrl Pts',(44.305661850593,-56.5222422564611,-40.9372114433545));
#263749=CARTESIAN_POINT('Ctrl Pts',(44.346925841944,-56.532247127269,-40.9693597045385));
#263750=CARTESIAN_POINT('Ctrl Pts',(44.3673876336497,-56.53826115526,-40.9859357593442));
#263751=CARTESIAN_POINT('Ctrl Pts',(44.3877715667723,-56.5447901720246,
-41.0027718870644));
#263752=CARTESIAN_POINT('Ctrl Pts',(44.3979208506631,-56.5483132560745,
-41.0113182564434));
#263753=CARTESIAN_POINT('Ctrl Pts',(44.4179418071922,-56.5558066378292,
-41.02850287128));
#263754=CARTESIAN_POINT('Ctrl Pts',(44.4278499085732,-56.5597882829787,
-41.0371710128992));
#263755=CARTESIAN_POINT('Ctrl Pts',(44.4572364860018,-56.5724196473794,
-41.0633712499365));
#263756=CARTESIAN_POINT('Ctrl Pts',(44.4763932211824,-56.581758968269,-41.0811111519311));
#263757=CARTESIAN_POINT('Ctrl Pts',(44.5044772880921,-56.5971447477014,
-41.1081262866225));
#263758=CARTESIAN_POINT('Ctrl Pts',(44.5137271775895,-56.6025015227711,
-41.1171962449124));
#263759=CARTESIAN_POINT('Ctrl Pts',(44.5320183562985,-56.6136863880645,
-41.1354834617267));
#263760=CARTESIAN_POINT('Ctrl Pts',(44.5410031705763,-56.6194798267371,
-41.144644186283));
#263761=CARTESIAN_POINT('Ctrl Pts',(44.5674276642847,-56.6374191091633,
-41.1721205907467));
#263762=CARTESIAN_POINT('Ctrl Pts',(44.5843870769067,-56.6501457393646,
-41.1904750382678));
#263763=CARTESIAN_POINT('Ctrl Pts',(44.616987890196,-56.6770839740703,-41.2272237610649));
#263764=CARTESIAN_POINT('Ctrl Pts',(44.640458797708,-56.6984048650555,-41.2548228473058));
#263765=CARTESIAN_POINT('Ctrl Pts',(44.6624514458289,-56.7214114906953,
-41.2824783924342));
#263766=CARTESIAN_POINT('Ctrl Pts',(44.6767798128067,-56.7371294193188,
-41.3009283158679));
#263767=CARTESIAN_POINT('Ctrl Pts',(44.683774397772,-56.7451748501741,-41.3101557240219));
#263768=CARTESIAN_POINT('Ctrl Pts',(44.6940202659092,-56.7575442973705,
-41.324018848177));
#263769=CARTESIAN_POINT('Ctrl Pts',(44.6973914635031,-56.7617145235639,
-41.328639728599));
#263770=CARTESIAN_POINT('Ctrl Pts',(44.7040131878578,-56.770108052971,-41.3378361513053));
#263771=CARTESIAN_POINT('Ctrl Pts',(44.7072703203268,-56.7743392575068,
-41.3424205878605));
#263772=CARTESIAN_POINT('Ctrl Pts',(44.7168707027477,-56.7871217033085,
-41.3561177927451));
#263773=CARTESIAN_POINT('Ctrl Pts',(44.7230524906066,-56.7957731420119,
-41.3651872799216));
#263774=CARTESIAN_POINT('Ctrl Pts',(44.7409373255192,-56.8220955492914,
-41.3921945478314));
#263775=CARTESIAN_POINT('Ctrl Pts',(44.7575187561203,-56.8491712652862,
-41.4188207502394));
#263776=CARTESIAN_POINT('Ctrl Pts',(44.7770214494108,-56.88676384976,-41.453559097464));
#263777=CARTESIAN_POINT('Ctrl Pts',(44.7858965000619,-56.9060633365117,
-41.4706740459328));
#263778=CARTESIAN_POINT('Ctrl Pts',(44.7943266372896,-56.9256180211132,
-41.4876605613939));
#263779=CARTESIAN_POINT('Ctrl Pts',(44.7983169540911,-56.9355169983302,
-41.4960845962979));
#263780=CARTESIAN_POINT('Ctrl Pts',(44.8058516078422,-56.9556000996462,
-41.5128223385875));
#263781=CARTESIAN_POINT('Ctrl Pts',(44.8093727854448,-56.9657242505397,
-41.5210856532432));
#263782=CARTESIAN_POINT('Ctrl Pts',(44.8191505788346,-56.9961959016236,
-41.5454418374945));
#263783=CARTESIAN_POINT('Ctrl Pts',(44.8246597322132,-57.0167187198372,
-41.5611704866007));
#263784=CARTESIAN_POINT('Ctrl Pts',(44.8336688220904,-57.0581479791523,
-41.5916045035181));
#263785=CARTESIAN_POINT('Ctrl Pts',(44.8389236650083,-57.0895139074259,
-41.613669368427));
#263786=CARTESIAN_POINT('Ctrl Pts',(44.8418900765893,-57.1213299669285,
-41.6345866129535));
#263787=CARTESIAN_POINT('Ctrl Pts',(44.8433488372948,-57.142640498193,-41.6482710687869));
#263788=CARTESIAN_POINT('Ctrl Pts',(44.8438191277705,-57.1533552116615,
-41.6549890353504));
#263789=CARTESIAN_POINT('Ctrl Pts',(44.8442270800594,-57.1748537940466,
-41.6681388704993));
#263790=CARTESIAN_POINT('Ctrl Pts',(44.8441639040618,-57.1855561823783,
-41.6745213422017));
#263791=CARTESIAN_POINT('Ctrl Pts',(44.8435122114514,-57.2069000331791,
-41.6869277892926));
#263792=CARTESIAN_POINT('Ctrl Pts',(44.8417458896958,-57.2388084678274,
-41.7049896680882));
#263793=CARTESIAN_POINT('Ctrl Pts',(44.8362687719071,-57.2809279665006,
-41.7269106712316));
#263794=CARTESIAN_POINT('Ctrl Pts',(44.8298088085522,-57.3121969378441,
-41.7417325167562));
#263795=CARTESIAN_POINT('Ctrl Pts',(44.8249713776488,-57.3329705079708,
-41.751249414817));
#263796=CARTESIAN_POINT('Ctrl Pts',(44.8222858794974,-57.3433254378487,
-41.7558274666229));
#263797=CARTESIAN_POINT('Ctrl Pts',(44.8163797073795,-57.3639440769784,
-41.7646063213672));
#263798=CARTESIAN_POINT('Ctrl Pts',(44.8131427147447,-57.3742522416544,
-41.7688238948253));
#263799=CARTESIAN_POINT('Ctrl Pts',(44.8061917406462,-57.3945668799698,
-41.7767918599254));
#263800=CARTESIAN_POINT('Ctrl Pts',(44.7987498536529,-57.4146412549335,
-41.7843210101159));
#263801=CARTESIAN_POINT('Ctrl Pts',(44.7861419817956,-57.4440129710611,
-41.7943060987191));
#263802=CARTESIAN_POINT('Ctrl Pts',(44.7720982599006,-57.4726583092559,
-41.8029984035242));
#263803=CARTESIAN_POINT('Ctrl Pts',(44.7566193423106,-57.5005749992605,
-41.8103989883131));
#263804=CARTESIAN_POINT('Ctrl Pts',(44.7453362941317,-57.518697088903,-41.8144666236875));
#263805=CARTESIAN_POINT('Ctrl Pts',(44.7335642473644,-57.5365709174371,
-41.8180952379985));
#263806=CARTESIAN_POINT('Ctrl Pts',(44.7274378249752,-57.5453780864623,
-41.8196891344695));
#263807=CARTESIAN_POINT('Ctrl Pts',(44.7146685840676,-57.5627610237142,
-41.8224320230444));
#263808=CARTESIAN_POINT('Ctrl Pts',(44.7080700862024,-57.5712755128024,
-41.8235709343319));
#263809=CARTESIAN_POINT('Ctrl Pts',(44.6877341610586,-57.5961705213949,
-41.8262807978491));
#263810=CARTESIAN_POINT('Ctrl Pts',(44.6734117165454,-57.6119810052107,
-41.8271650529119));
#263811=CARTESIAN_POINT('Ctrl Pts',(44.6432859415473,-57.6420285404153,
-41.827118555904));
#263812=CARTESIAN_POINT('Ctrl Pts',(44.6274777219699,-57.6562729242579,
-41.8261892556471));
#263813=CARTESIAN_POINT('Ctrl Pts',(44.6026489360012,-57.6764545436153,
-41.823427013232));
#263814=CARTESIAN_POINT('Ctrl Pts',(44.5941811636919,-57.6829873126311,
-41.8222767907821));
#263815=CARTESIAN_POINT('Ctrl Pts',(44.5812011369499,-57.6924815728277,
-41.820204446988));
#263816=CARTESIAN_POINT('Ctrl Pts',(44.5768239301145,-57.6955981764101,
-41.8194549553751));
#263817=CARTESIAN_POINT('Ctrl Pts',(44.5679795363474,-57.7017261947271,
-41.8178398084084));
#263818=CARTESIAN_POINT('Ctrl Pts',(44.554547495243,-57.7107794649358,-41.8152360293365));
#263819=CARTESIAN_POINT('Ctrl Pts',(44.5408745509057,-57.7192473537464,
-41.812140181677));
#263820=CARTESIAN_POINT('Ctrl Pts',(44.5224181841827,-57.7300417662926,
-41.8075820007456));
#263821=CARTESIAN_POINT('Ctrl Pts',(44.494403164631,-57.7454824222945,-41.8000999642091));
#263822=CARTESIAN_POINT('Ctrl Pts',(44.4557509611988,-57.7631175354143,
-41.7875858630695));
#263823=CARTESIAN_POINT('Ctrl Pts',(44.4257963579031,-57.7741479888816,
-41.7763064650726));
#263824=CARTESIAN_POINT('Ctrl Pts',(44.4056101875344,-57.781009218212,-41.7683613570464));
#263825=CARTESIAN_POINT('Ctrl Pts',(44.3954036594654,-57.7841949818065,
-41.7641737395871));
#263826=CARTESIAN_POINT('Ctrl Pts',(44.3747925009816,-57.7900627169564,
-41.7553761870634));
#263827=CARTESIAN_POINT('Ctrl Pts',(44.3643365899562,-57.7927558542442,
-41.7507422904685));
#263828=CARTESIAN_POINT('Ctrl Pts',(44.3329536886806,-57.7999988857253,
-41.7363257213199));
#263829=CARTESIAN_POINT('Ctrl Pts',(44.3014645871824,-57.8056090798854,
-41.7208580810542));
#263830=CARTESIAN_POINT('Ctrl Pts',(44.2698183189435,-57.8088603667088,
-41.7038603653999));
#263831=CARTESIAN_POINT('Ctrl Pts',(44.2381206623806,-57.8113308880715,
-41.6863549522799));
#263832=CARTESIAN_POINT('Ctrl Pts',(44.2169139506954,-57.8119384373532,
-41.6740048606234));
#263833=CARTESIAN_POINT('Ctrl Pts',(44.1850197107514,-57.811287280344,-41.6544681547659));
#263834=CARTESIAN_POINT('Ctrl Pts',(44.1743613109546,-57.8108078241776,
-41.6477783242763));
#263835=CARTESIAN_POINT('Ctrl Pts',(44.1583626375358,-57.8096935003687,
-41.6374930176863));
#263836=CARTESIAN_POINT('Ctrl Pts',(44.1530230189312,-57.809255510817,-41.6340194660765));
#263837=CARTESIAN_POINT('Ctrl Pts',(44.1423341247923,-57.8082460206643,
-41.6269840076234));
#263838=CARTESIAN_POINT('Ctrl Pts',(44.1369894952372,-57.8076746784434,
-41.6234249849254));
#263839=CARTESIAN_POINT('Ctrl Pts',(44.1103928894951,-57.8045001122898,
-41.6055088472864));
#263840=CARTESIAN_POINT('Ctrl Pts',(44.0684216046586,-57.7973782151022,
-41.5759273380954));
#263841=CARTESIAN_POINT('Ctrl Pts',(44.0275807082801,-57.78632659952,-41.5445717124501));
#263842=CARTESIAN_POINT('Ctrl Pts',(43.9872978152183,-57.7733311875938,
-41.5123297976061));
#263843=CARTESIAN_POINT('Ctrl Pts',(43.9674326520914,-57.7658590768128,
-41.4957625032292));
#263844=CARTESIAN_POINT('Ctrl Pts',(43.942963744406,-57.7552890823142,-41.4744937232973));
#263845=CARTESIAN_POINT('Ctrl Pts',(43.938085174092,-57.7531113051098,-41.4702088025761));
#263846=CARTESIAN_POINT('Ctrl Pts',(43.9283699185172,-57.7486342535987,
-41.4615871928557));
#263847=CARTESIAN_POINT('Ctrl Pts',(43.9235236029976,-57.7463299238453,
-41.4572415669043));
#263848=CARTESIAN_POINT('Ctrl Pts',(43.9090930604083,-57.739254093668,-41.4441663196977));
#263849=CARTESIAN_POINT('Ctrl Pts',(43.8996324205383,-57.7343289686206,
-41.4354132012863));
#263850=CARTESIAN_POINT('Ctrl Pts',(43.8903154257419,-57.7291941381088,
-41.4266127101804));
#263851=CARTESIAN_POINT('',(45.4581751231188,-55.7156010961851,-39.3126317220031));
#263852=CARTESIAN_POINT('',(45.2824537511366,-55.8755132365557,-39.638597553055));
#263853=CARTESIAN_POINT('',(45.4581751231188,-55.7156010961851,-39.3126317220031));
#263854=CARTESIAN_POINT('Origin',(44.4104395346295,-57.5698098586536,-39.4585973766342));
#263855=CARTESIAN_POINT('Ctrl Pts',(45.1065281945089,-55.5671267135029,
-39.2098668976124));
#263856=CARTESIAN_POINT('Ctrl Pts',(44.9196034855776,-55.5452400673183,
-39.2198174688805));
#263857=CARTESIAN_POINT('Ctrl Pts',(44.7296870412447,-55.5423799337785,
-39.2250112643947));
#263858=CARTESIAN_POINT('Ctrl Pts',(44.2390927302324,-55.5906252485044,
-39.2279787011603));
#263859=CARTESIAN_POINT('Ctrl Pts',(44.0090817791515,-55.6680747610649,
-39.2201085375079));
#263860=CARTESIAN_POINT('Ctrl Pts',(43.7382090165708,-55.7808826579177,
-39.2093719638497));
#263861=CARTESIAN_POINT('Ctrl Pts',(43.6231650567784,-55.840997752458,-39.2038428512868));
#263862=CARTESIAN_POINT('Ctrl Pts',(43.5024059980203,-55.917969348109,-39.1959115145055));
#263863=CARTESIAN_POINT('Ctrl Pts',(43.4922077364908,-55.9245826673839,
-39.1952208230375));
#263864=CARTESIAN_POINT('Ctrl Pts',(43.4720389115154,-55.9378870274315,
-39.1938132140166));
#263865=CARTESIAN_POINT('Ctrl Pts',(43.4620602401924,-55.9445806290796,
-39.1930961601356));
#263866=CARTESIAN_POINT('Ctrl Pts',(43.4496915434521,-55.9530170716417,
-39.1921817769743));
#263867=CARTESIAN_POINT('Ctrl Pts',(43.4472466873436,-55.954691516998,-39.1919997813558));
#263868=CARTESIAN_POINT('Ctrl Pts',(43.3583119868597,-56.0158518702413,
-39.1853338681724));
#263869=CARTESIAN_POINT('Ctrl Pts',(43.276069883232,-56.0810726814889,-39.1776023189702));
#263870=CARTESIAN_POINT('Ctrl Pts',(43.0861151222154,-56.2539000103423,
-39.1559361477625));
#263871=CARTESIAN_POINT('Ctrl Pts',(42.9842069097486,-56.3668846933458,
-39.1408381965094));
#263872=CARTESIAN_POINT('Ctrl Pts',(42.7323009654217,-56.7066866053067,
-39.0930140844855));
#263873=CARTESIAN_POINT('Ctrl Pts',(42.6102232298188,-56.9486116620658,
-39.0563926396021));
#263874=CARTESIAN_POINT('Ctrl Pts',(42.5264426781749,-57.2041246092115,
-39.0141963044759));
#263875=CARTESIAN_POINT('Ctrl Pts',(42.5264426236304,-57.2041246472958,
-39.0141972810499));
#263876=CARTESIAN_POINT('Ctrl Pts',(42.5223570304571,-57.2339619119713,
-39.0195734528566));
#263877=CARTESIAN_POINT('Ctrl Pts',(42.5115447559028,-57.3288674986212,
-39.0371239801764));
#263878=CARTESIAN_POINT('Ctrl Pts',(42.506182785202,-57.4564982984358,-39.0625980639181));
#263879=CARTESIAN_POINT('Ctrl Pts',(42.5092432682604,-57.5543877143394,
-39.0835871924589));
#263880=CARTESIAN_POINT('Ctrl Pts',(42.5128918544921,-57.6196827267464,
-39.0979114000806));
#263881=CARTESIAN_POINT('Ctrl Pts',(42.5155178619726,-57.6523290916439,
-39.1052348221532));
#263882=CARTESIAN_POINT('Ctrl Pts',(42.5224092913251,-57.7177332511804,
-39.120233936761));
#263883=CARTESIAN_POINT('Ctrl Pts',(42.5266542176424,-57.7502677264706,
-39.1278590184786));
#263884=CARTESIAN_POINT('Ctrl Pts',(42.5366779815724,-57.8147780230883,
-39.1432995470242));
#263885=CARTESIAN_POINT('Ctrl Pts',(42.5424617625838,-57.8468004016288,
-39.1511256797658));
#263886=CARTESIAN_POINT('Ctrl Pts',(42.5620823726479,-57.9421435490173,
-39.1749053180845));
#263887=CARTESIAN_POINT('Ctrl Pts',(42.5942908295626,-58.0673908049564,
-39.2074251962624));
#263888=CARTESIAN_POINT('Ctrl Pts',(42.6384162470065,-58.1889247195952,
-39.2415287814174));
#263889=CARTESIAN_POINT('Ctrl Pts',(42.676040350531,-58.2786648895678,-39.2677034056768));
#263890=CARTESIAN_POINT('Ctrl Pts',(42.6893426693184,-58.308352422918,-39.2765308704477));
#263891=CARTESIAN_POINT('Ctrl Pts',(42.7174688743488,-58.367210478172,-39.2943764905707));
#263892=CARTESIAN_POINT('Ctrl Pts',(42.7468976399245,-58.4250976736592,
-39.3122747709031));
#263893=CARTESIAN_POINT('Ctrl Pts',(42.7949093409291,-58.5091805688265,
-39.33930500608));
#263894=CARTESIAN_POINT('Ctrl Pts',(42.8639918437047,-58.6176479605168,
-39.3755734228826));
#263895=CARTESIAN_POINT('Ctrl Pts',(42.9458586003439,-58.7277739375476,
-39.4146896477163));
#263896=CARTESIAN_POINT('Ctrl Pts',(43.0153234518519,-58.8072809398543,
-39.4449530869582));
#263897=CARTESIAN_POINT('Ctrl Pts',(43.0434020223321,-58.8374710867404,
-39.4567766041471));
#263898=CARTESIAN_POINT('Ctrl Pts',(43.0434014360654,-58.8374714889306,
-39.456776868572));
#263899=CARTESIAN_POINT('Ctrl Pts',(42.9313536289255,-58.6662175819515,
-39.4482830419655));
#263900=CARTESIAN_POINT('Ctrl Pts',(42.844505428787,-58.4794048505646,-39.4413327045587));
#263901=CARTESIAN_POINT('Ctrl Pts',(42.7299233825216,-58.09580806204,-39.4313779831406));
#263902=CARTESIAN_POINT('Ctrl Pts',(42.7001443335031,-57.9014057226055,
-39.4282539321925));
#263903=CARTESIAN_POINT('Ctrl Pts',(42.6957518169554,-57.5153921394814,
-39.4252456428475));
#263904=CARTESIAN_POINT('Ctrl Pts',(42.7186804830506,-57.2657661474499,
-39.4244208737333));
#263905=CARTESIAN_POINT('Ctrl Pts',(42.881352952887,-56.8215446683501,-39.4348872407336));
#263906=CARTESIAN_POINT('Ctrl Pts',(42.9678495973224,-56.6600017061349,
-39.4410989978245));
#263907=CARTESIAN_POINT('Ctrl Pts',(43.165269885457,-56.3920180420655,-39.4552161772219));
#263908=CARTESIAN_POINT('Ctrl Pts',(43.2687938698745,-56.2817295804231,
-39.4625951676374));
#263909=CARTESIAN_POINT('Ctrl Pts',(43.4087045485911,-56.1645349417216,
-39.4723386928991));
#263910=CARTESIAN_POINT('Ctrl Pts',(43.4337474511219,-56.1446185810003,
-39.4740755133032));
#263911=CARTESIAN_POINT('Ctrl Pts',(43.4624070124288,-56.122993219963,-39.4760548803308));
#263912=CARTESIAN_POINT('Ctrl Pts',(43.4655267799061,-56.1206543087335,
-39.4762702364359));
#263913=CARTESIAN_POINT('Ctrl Pts',(43.4702206900142,-56.117157920804,-39.4765940904724));
#263914=CARTESIAN_POINT('Ctrl Pts',(43.4717893933871,-56.1159932120419,
-39.4767022949794));
#263915=CARTESIAN_POINT('Ctrl Pts',(43.5244120055323,-56.0770493035069,
-39.4803311343257));
#263916=CARTESIAN_POINT('Ctrl Pts',(43.5773300428345,-56.0418702026374,
-39.4839525622719));
#263917=CARTESIAN_POINT('Ctrl Pts',(43.6611219775383,-55.9920607689694,
-39.4896409291132));
#263918=CARTESIAN_POINT('Ctrl Pts',(43.6906998176424,-55.9755391894888,
-39.4916509259111));
#263919=CARTESIAN_POINT('Ctrl Pts',(43.9412200417594,-55.8446488555592,
-39.5091960926514));
#263920=CARTESIAN_POINT('Ctrl Pts',(44.1826052363169,-55.7754693918874,
-39.5285011629926));
#263921=CARTESIAN_POINT('Ctrl Pts',(44.5742546833041,-55.7421335552316,
-39.56393266636));
#263922=CARTESIAN_POINT('Ctrl Pts',(44.7207121507351,-55.7464909499098,
-39.5780619691923));
#263923=CARTESIAN_POINT('Ctrl Pts',(45.008007911895,-55.7878402235656,-39.6076254992843));
#263924=CARTESIAN_POINT('Ctrl Pts',(45.1478398540244,-55.8241870193201,
-39.6229270428342));
#263925=CARTESIAN_POINT('Ctrl Pts',(45.2824630401997,-55.8755167783063,
-39.6385986344006));
#263926=CARTESIAN_POINT('Ctrl Pts',(43.4805770970857,-59.5712767993712,
-39.2399079805728));
#263927=CARTESIAN_POINT('Ctrl Pts',(43.4478249032475,-59.5535604408099,
-39.2311074894668));
#263928=CARTESIAN_POINT('Ctrl Pts',(43.4156055925501,-59.5351039455316,
-39.2222635254953));
#263929=CARTESIAN_POINT('Ctrl Pts',(43.3522169314537,-59.4967329031118,
-39.2044893356988));
#263930=CARTESIAN_POINT('Ctrl Pts',(43.3210476326526,-59.4768182838717,
-39.195559106683));
#263931=CARTESIAN_POINT('Ctrl Pts',(43.22910224469,-59.4149049566893,-39.1686392736337));
#263932=CARTESIAN_POINT('Ctrl Pts',(43.1698853428616,-59.3707413470177,
-39.1505207493783));
#263933=CARTESIAN_POINT('Ctrl Pts',(43.0556331440142,-59.2766098026481,
-39.1139350081145));
#263934=CARTESIAN_POINT('Ctrl Pts',(43.0005921407603,-59.2266373423717,
-39.0954659954893));
#263935=CARTESIAN_POINT('Ctrl Pts',(42.8948534359946,-59.1207134457913,
-39.058173264863));
#263936=CARTESIAN_POINT('Ctrl Pts',(42.8449960335796,-59.065605688259,-39.0396462508422));
#263937=CARTESIAN_POINT('Ctrl Pts',(42.7510810974034,-58.9512122629159,
-39.0028139114377));
#263938=CARTESIAN_POINT('Ctrl Pts',(42.7070287909669,-58.8919306728536,
-38.9845102176061));
#263939=CARTESIAN_POINT('Ctrl Pts',(42.6452866096269,-58.7998959060405,
-38.9572240228595));
#263940=CARTESIAN_POINT('Ctrl Pts',(42.6254297416276,-58.7686980942012,
-38.9481569046653));
#263941=CARTESIAN_POINT('Ctrl Pts',(42.5871755865899,-58.7052547141791,
-38.9300801001639));
#263942=CARTESIAN_POINT('Ctrl Pts',(42.5687782262919,-58.6730091989553,
-38.9210704098267));
#263943=CARTESIAN_POINT('Ctrl Pts',(42.5334651607083,-58.6074544045328,
-38.9031098430389));
#263944=CARTESIAN_POINT('Ctrl Pts',(42.5165536092555,-58.5741539456505,
-38.8941612806853));
#263945=CARTESIAN_POINT('Ctrl Pts',(42.4842288284689,-58.5064298905342,
-38.8763156605622));
#263946=CARTESIAN_POINT('Ctrl Pts',(42.4689425110757,-58.4722695790417,
-38.8674881957913));
#263947=CARTESIAN_POINT('Ctrl Pts',(42.4401223524774,-58.4034275394388,
-38.850038446285));
#263948=CARTESIAN_POINT('Ctrl Pts',(42.4265830216104,-58.3687342215786,
-38.8414131147228));
#263949=CARTESIAN_POINT('Ctrl Pts',(42.4012287621092,-58.2988104506425,
-38.8243608135095));
#263950=CARTESIAN_POINT('Ctrl Pts',(42.3894137311741,-58.2635796417037,
-38.8159337609721));
#263951=CARTESIAN_POINT('Ctrl Pts',(42.3565460901882,-58.1570828792368,
-38.7909502174193));
#263952=CARTESIAN_POINT('Ctrl Pts',(42.3380647593969,-58.08501193977,-38.774690108199));
#263953=CARTESIAN_POINT('Ctrl Pts',(42.3155659483831,-57.9752818676448,
-38.7509104698803));
#263954=CARTESIAN_POINT('Ctrl Pts',(42.3089373897852,-57.9384266392251,
-38.7430843371387));
#263955=CARTESIAN_POINT('Ctrl Pts',(42.2974579811028,-57.8641787720779,
-38.7276438085931));
#263956=CARTESIAN_POINT('Ctrl Pts',(42.2926014835326,-57.8267325462403,
-38.7200187268755));
#263957=CARTESIAN_POINT('Ctrl Pts',(42.2847289598988,-57.7514526438499,
-38.7050196122677));
#263958=CARTESIAN_POINT('Ctrl Pts',(42.2817363203014,-57.7138760098677,
-38.6976961901952));
#263959=CARTESIAN_POINT('Ctrl Pts',(42.2775969609554,-57.6387185090426,
-38.6833719825733));
#263960=CARTESIAN_POINT('Ctrl Pts',(42.2764524982459,-57.601159318647,-38.6763755134769));
#263961=CARTESIAN_POINT('Ctrl Pts',(42.2757725868838,-57.4885396265684,
-38.6558809090593));
#263962=CARTESIAN_POINT('Ctrl Pts',(42.2789845110076,-57.4135368784203,
-38.6428764616153));
#263963=CARTESIAN_POINT('Ctrl Pts',(42.2893332825795,-57.3011476865308,
-38.6243712438732));
#263964=CARTESIAN_POINT('Ctrl Pts',(42.2937061365005,-57.2637038084211,
-38.6183700063105));
#263965=CARTESIAN_POINT('Ctrl Pts',(42.3043246703777,-57.1888547487219,
-38.6067078983536));
#263966=CARTESIAN_POINT('Ctrl Pts',(42.3105742804476,-57.1514345489241,
-38.6010450084679));
#263967=CARTESIAN_POINT('Ctrl Pts',(42.3249703860378,-57.0766935224097,
-38.5900761598925));
#263968=CARTESIAN_POINT('Ctrl Pts',(42.3331591716861,-57.0392159776392,
-38.5847493692274));
#263969=CARTESIAN_POINT('Ctrl Pts',(42.3512949539204,-56.9651221376192,
-38.5745672487527));
#263970=CARTESIAN_POINT('Ctrl Pts',(42.3612585832142,-56.9283882008754,
-38.5696935766092));
#263971=CARTESIAN_POINT('Ctrl Pts',(42.382946766925,-56.8555905629784,-38.5603847482528));
#263972=CARTESIAN_POINT('Ctrl Pts',(42.3946724253985,-56.8195179869541,
-38.5559481805345));
#263973=CARTESIAN_POINT('Ctrl Pts',(42.4198760421967,-56.7480211971863,
-38.5475091590052));
#263974=CARTESIAN_POINT('Ctrl Pts',(42.433354009658,-56.7125969868972,-38.5435067067598));
#263975=CARTESIAN_POINT('Ctrl Pts',(42.4620643367001,-56.6423975987555,
-38.5359374532668));
#263976=CARTESIAN_POINT('Ctrl Pts',(42.4772966787996,-56.6076224144876,
-38.53237064715));
#263977=CARTESIAN_POINT('Ctrl Pts',(42.5095307755788,-56.5387265419139,
-38.5256773524591));
#263978=CARTESIAN_POINT('Ctrl Pts',(42.5265324846308,-56.5046058367601,
-38.5225508521777));
#263979=CARTESIAN_POINT('Ctrl Pts',(42.5623338208904,-56.4370293846275,
-38.5167461114759));
#263980=CARTESIAN_POINT('Ctrl Pts',(42.5811223378823,-56.4035922992139,
-38.51406925145));
#263981=CARTESIAN_POINT('Ctrl Pts',(42.6205844974323,-56.3373241879144,
-38.5091696849532));
#263982=CARTESIAN_POINT('Ctrl Pts',(42.6411082002799,-56.3047465778678,
-38.5069658948843));
#263983=CARTESIAN_POINT('Ctrl Pts',(42.7048067750791,-56.2090283214366,
-38.5011108038064));
#263984=CARTESIAN_POINT('Ctrl Pts',(42.7502234311298,-56.1476408508883,
-38.4981889837996));
#263985=CARTESIAN_POINT('Ctrl Pts',(42.8467942109284,-56.0297655406316,
-38.4942909959747));
#263986=CARTESIAN_POINT('Ctrl Pts',(42.89797152087,-55.9732420296543,-38.493312543871));
#263987=CARTESIAN_POINT('Ctrl Pts',(42.9790570362859,-55.8921695682654,
-38.4933149308443));
#263988=CARTESIAN_POINT('Ctrl Pts',(43.0068373921125,-55.8657400703683,
-38.4935621456146));
#263989=CARTESIAN_POINT('Ctrl Pts',(43.0495800471754,-55.8270637537312,
-38.4943062517503));
#263990=CARTESIAN_POINT('Ctrl Pts',(43.0640221885071,-55.8143203297415,
-38.4946170972135));
#263991=CARTESIAN_POINT('Ctrl Pts',(43.0932714605165,-55.7891564041938,
-38.4953646355488));
#263992=CARTESIAN_POINT('Ctrl Pts',(43.1080901116598,-55.7767277717167,
-38.4958019484811));
#263993=CARTESIAN_POINT('Ctrl Pts',(43.1528523151143,-55.7401326939816,
-38.4972962428884));
#263994=CARTESIAN_POINT('Ctrl Pts',(43.1831712256444,-55.7165901141018,
-38.4985359777345));
#263995=CARTESIAN_POINT('Ctrl Pts',(43.244758341421,-55.671169126854,-38.501493078153));
#263996=CARTESIAN_POINT('Ctrl Pts',(43.2760240772567,-55.6492920651712,
-38.5032102375714));
#263997=CARTESIAN_POINT('Ctrl Pts',(43.3712176334144,-55.58612549871,-38.5090666032762));
#263998=CARTESIAN_POINT('Ctrl Pts',(43.4365388184857,-55.5472953546232,
-38.5139092517118));
#263999=CARTESIAN_POINT('Ctrl Pts',(43.5372923366523,-55.4939420358375,
-38.5225683917069));
#264000=CARTESIAN_POINT('Ctrl Pts',(43.5713395844727,-55.476974296143,-38.5256876830023));
#264001=CARTESIAN_POINT('Ctrl Pts',(43.6403672791554,-55.4446857453381,
-38.5323950948992));
#264002=CARTESIAN_POINT('Ctrl Pts',(43.6753577621025,-55.4293619873053,
-38.5359845082588));
#264003=CARTESIAN_POINT('Ctrl Pts',(43.7462462014538,-55.4003985293068,
-38.5436332514696));
#264004=CARTESIAN_POINT('Ctrl Pts',(43.7822717715004,-55.3867204163754,
-38.5477088311098));
#264005=CARTESIAN_POINT('Ctrl Pts',(43.8543821706563,-55.3613797550828,
-38.5562345876408));
#264006=CARTESIAN_POINT('Ctrl Pts',(43.8906224054099,-55.3496490529759,
-38.5607006893241));
#264007=CARTESIAN_POINT('Ctrl Pts',(43.963378182051,-55.3280633077297,-38.5700203534958));
#264008=CARTESIAN_POINT('Ctrl Pts',(43.9999084017295,-55.3182018771171,
-38.5748754295458));
#264009=CARTESIAN_POINT('Ctrl Pts',(44.0732691659691,-55.3003143634305,
-38.5849691522959));
#264010=CARTESIAN_POINT('Ctrl Pts',(44.1100997173916,-55.2922883228605,
-38.5902078085425));
#264011=CARTESIAN_POINT('Ctrl Pts',(44.1840590840081,-55.278057933328,-38.6010646496354));
#264012=CARTESIAN_POINT('Ctrl Pts',(44.2211879014379,-55.2718535986756,
-38.606682838198));
#264013=CARTESIAN_POINT('Ctrl Pts',(44.2957439119556,-55.261266200021,-38.6182974286047));
#264014=CARTESIAN_POINT('Ctrl Pts',(44.3331711028503,-55.2568831233685,
-38.6242938286285));
#264015=CARTESIAN_POINT('Ctrl Pts',(44.4083261451804,-55.2499510424672,
-38.6366662370891));
#264016=CARTESIAN_POINT('Ctrl Pts',(44.4460560558118,-55.2474028685688,
-38.6430427650303));
#264017=CARTESIAN_POINT('Ctrl Pts',(44.5218128109665,-55.2441636047241,
-38.6561775093914));
#264018=CARTESIAN_POINT('Ctrl Pts',(44.5599089520781,-55.2434808242815,
-38.66294972511));
#264019=CARTESIAN_POINT('Ctrl Pts',(44.6354869653286,-55.2439910765326,
-38.6767129557532));
#264020=CARTESIAN_POINT('Ctrl Pts',(44.6731457008971,-55.245173978475,-38.6837341823244));
#264021=CARTESIAN_POINT('Ctrl Pts',(44.7481014918668,-55.2493619747848,
-38.6980304133054));
#264022=CARTESIAN_POINT('Ctrl Pts',(44.7854165987361,-55.2523661957112,
-38.7053085311543));
#264023=CARTESIAN_POINT('Ctrl Pts',(44.8968808213,-55.2640710443033,-38.7275255991979));
#264024=CARTESIAN_POINT('Ctrl Pts',(44.970549832836,-55.2754583054948,-38.7428464642802));
#264025=CARTESIAN_POINT('Ctrl Pts',(45.0801002188279,-55.2978810234077,
-38.766580365083));
#264026=CARTESIAN_POINT('Ctrl Pts',(45.1164578950735,-55.3062470347631,
-38.7746173156054));
#264027=CARTESIAN_POINT('Ctrl Pts',(45.1888527862828,-55.324776345739,-38.7909433983534));
#264028=CARTESIAN_POINT('Ctrl Pts',(45.2248832273146,-55.3349380647777,
-38.7992310297367));
#264029=CARTESIAN_POINT('Ctrl Pts',(45.2966462910748,-55.3570913037395,
-38.8160671574568));
#264030=CARTESIAN_POINT('Ctrl Pts',(45.3323639181915,-55.3690862993212,
-38.8246135268356));
#264031=CARTESIAN_POINT('Ctrl Pts',(45.4027951684834,-55.3946744168502,
-38.8417981416725));
#264032=CARTESIAN_POINT('Ctrl Pts',(45.4376370576062,-55.4083059928131,
-38.8504662832915));
#264033=CARTESIAN_POINT('Ctrl Pts',(45.5065020448728,-55.4372015304471,
-38.8679331079831));
#264034=CARTESIAN_POINT('Ctrl Pts',(45.5405385294939,-55.4524695704278,
-38.8767349230064));
#264035=CARTESIAN_POINT('Ctrl Pts',(45.6078227830677,-55.4846397608258,
-38.8944741023142));
#264036=CARTESIAN_POINT('Ctrl Pts',(45.6410705511329,-55.5015419127995,
-38.9034114672202));
#264037=CARTESIAN_POINT('Ctrl Pts',(45.7067750180478,-55.5369855589402,
-38.9214215570149));
#264038=CARTESIAN_POINT('Ctrl Pts',(45.7392220186752,-55.5555211850666,
-38.9304915153049));
#264039=CARTESIAN_POINT('Ctrl Pts',(45.8033557152909,-55.5942721902847,
-38.9487787321192));
#264040=CARTESIAN_POINT('Ctrl Pts',(45.8348444017589,-55.6143675059359,
-38.9579394566731));
#264041=CARTESIAN_POINT('Ctrl Pts',(45.9274100185651,-55.676658878309,-38.9854158611437));
#264042=CARTESIAN_POINT('Ctrl Pts',(45.9867611219468,-55.7209352921753,
-39.0037703086594));
#264043=CARTESIAN_POINT('Ctrl Pts',(46.1007338204162,-55.8148102176407,
-39.0405190314579));
#264044=CARTESIAN_POINT('Ctrl Pts',(46.1553754636135,-55.8644173555222,
-39.0589184365119));
#264045=CARTESIAN_POINT('Ctrl Pts',(46.2338037667526,-55.9428521113138,
-39.0865551406703));
#264046=CARTESIAN_POINT('Ctrl Pts',(46.2593566149882,-55.9696687163404,
-39.0957736628265));
#264047=CARTESIAN_POINT('Ctrl Pts',(46.3092668490953,-56.0246630354032,
-39.1142235862602));
#264048=CARTESIAN_POINT('Ctrl Pts',(46.3336138592955,-56.0528283934937,
-39.1234509944141));
#264049=CARTESIAN_POINT('Ctrl Pts',(46.3692509706587,-56.0961546799093,
-39.1373141185695));
#264050=CARTESIAN_POINT('Ctrl Pts',(46.3809719979937,-56.1107655086548,
-39.1419349989914));
#264051=CARTESIAN_POINT('Ctrl Pts',(46.4039851397009,-56.1401806556231,
-39.1511314216979));
#264052=CARTESIAN_POINT('Ctrl Pts',(46.4153002334237,-56.155012646864,-39.1557158582529));
#264053=CARTESIAN_POINT('Ctrl Pts',(46.4486370533476,-56.1998309912202,
-39.1694130631373));
#264054=CARTESIAN_POINT('Ctrl Pts',(46.4700835531906,-56.2301795174735,
-39.1784825503139));
#264055=CARTESIAN_POINT('Ctrl Pts',(46.5320719588418,-56.3225583858835,
-39.2054898182239));
#264056=CARTESIAN_POINT('Ctrl Pts',(46.5703036405633,-56.3859631464818,
-39.2232408011316));
#264057=CARTESIAN_POINT('Ctrl Pts',(46.6230137769529,-56.4837650818566,
-39.2494850822324));
#264058=CARTESIAN_POINT('Ctrl Pts',(46.6398106251204,-56.5168167226216,
-39.2581697490099));
#264059=CARTESIAN_POINT('Ctrl Pts',(46.6718447361749,-56.5838294852714,
-39.2754118634509));
#264060=CARTESIAN_POINT('Ctrl Pts',(46.6870820781819,-56.6177905613574,
-39.2839693163248));
#264061=CARTESIAN_POINT('Ctrl Pts',(46.7159730314734,-56.686636048537,-39.3009558317863));
#264062=CARTESIAN_POINT('Ctrl Pts',(46.7296188510695,-56.7214992835749,
-39.3093798666901));
#264063=CARTESIAN_POINT('Ctrl Pts',(46.7553217489119,-56.7922546342832,
-39.3261176089799));
#264064=CARTESIAN_POINT('Ctrl Pts',(46.767299743662,-56.8279354846841,-39.3343809236343));
#264065=CARTESIAN_POINT('Ctrl Pts',(46.8004531002449,-56.9353633944232,
-39.3587371078895));
#264066=CARTESIAN_POINT('Ctrl Pts',(46.8189796004616,-57.0077635585741,
-39.3744657569928));
#264067=CARTESIAN_POINT('Ctrl Pts',(46.848916262609,-57.1540080970469,-39.4048997739107));
#264068=CARTESIAN_POINT('Ctrl Pts',(46.8603369955464,-57.2278698710425,
-39.4196100030402));
#264069=CARTESIAN_POINT('Ctrl Pts',(46.8720665256814,-57.3397812953029,
-39.4409093089087));
#264070=CARTESIAN_POINT('Ctrl Pts',(46.8750748009162,-57.3772756957559,
-39.4478818833461));
#264071=CARTESIAN_POINT('Ctrl Pts',(46.879254346672,-57.452637038775,-39.4615663391791));
#264072=CARTESIAN_POINT('Ctrl Pts',(46.880425925028,-57.4905390917853,-39.4682843057428));
#264073=CARTESIAN_POINT('Ctrl Pts',(46.8808838257092,-57.5666104472174,
-39.4814341408916));
#264074=CARTESIAN_POINT('Ctrl Pts',(46.8801709150999,-57.6044914055267,
-39.4878166125941));
#264075=CARTESIAN_POINT('Ctrl Pts',(46.8768914392193,-57.6800598105232,
-39.5002230596849));
#264076=CARTESIAN_POINT('Ctrl Pts',(46.8743247149934,-57.7177285118847,
-39.506243785591));
#264077=CARTESIAN_POINT('Ctrl Pts',(46.8638676192418,-57.8303908579074,
-39.5237649045219));
#264078=CARTESIAN_POINT('Ctrl Pts',(46.853226416258,-57.905041503381,-39.5347254344493));
#264079=CARTESIAN_POINT('Ctrl Pts',(46.8317335819185,-58.0163268627736,
-39.550087285924));
#264080=CARTESIAN_POINT('Ctrl Pts',(46.8236460045766,-58.0533066998131,
-39.5550277871486));
#264081=CARTESIAN_POINT('Ctrl Pts',(46.8055990609215,-58.127032513964,-39.5645446852094));
#264082=CARTESIAN_POINT('Ctrl Pts',(46.7956340174415,-58.1637938739027,
-39.5691227370151));
#264083=CARTESIAN_POINT('Ctrl Pts',(46.7738161820537,-58.2370162297126,
-39.5779015917596));
#264084=CARTESIAN_POINT('Ctrl Pts',(46.7619036769789,-58.2736352495457,
-39.582119165218));
#264085=CARTESIAN_POINT('Ctrl Pts',(46.7364060204878,-58.3458256235152,
-39.5900871303177));
#264086=CARTESIAN_POINT('Ctrl Pts',(46.7227944358822,-58.3815079540758,
-39.5938519714545));
#264087=CARTESIAN_POINT('Ctrl Pts',(46.6938811083112,-58.4520118830205,
-39.6009443323402));
#264088=CARTESIAN_POINT('Ctrl Pts',(46.6785776728307,-58.4868414029238,
-39.6042729162555));
#264089=CARTESIAN_POINT('Ctrl Pts',(46.6462897807642,-58.5556617478733,
-39.6104988832622));
#264090=CARTESIAN_POINT('Ctrl Pts',(46.6293053112816,-58.5896525665271,
-39.6133962624303));
#264091=CARTESIAN_POINT('Ctrl Pts',(46.5936553992581,-58.656795488418,-39.6187605166456));
#264092=CARTESIAN_POINT('Ctrl Pts',(46.5749899695051,-58.6899475980592,
-39.621227394548));
#264093=CARTESIAN_POINT('Ctrl Pts',(46.5359657888858,-58.7554069047812,
-39.6257280783136));
#264094=CARTESIAN_POINT('Ctrl Pts',(46.5156070776159,-58.7877141216242,
-39.6277618940797));
#264095=CARTESIAN_POINT('Ctrl Pts',(46.4731711272442,-58.8514710379442,
-39.6313905083909));
#264096=CARTESIAN_POINT('Ctrl Pts',(46.4511086572017,-58.8829006656694,
-39.6329844048618));
#264097=CARTESIAN_POINT('Ctrl Pts',(46.4051673627461,-58.9449633365352,
-39.6357272934367));
#264098=CARTESIAN_POINT('Ctrl Pts',(46.3814480364632,-58.9753776243305,
-39.6368662047246));
#264099=CARTESIAN_POINT('Ctrl Pts',(46.3084069318146,-59.0643493506752,
-39.6395760682405));
#264100=CARTESIAN_POINT('Ctrl Pts',(46.2570408245348,-59.1209150834389,
-39.640460323304));
#264101=CARTESIAN_POINT('Ctrl Pts',(46.1491380135578,-59.2285445031963,
-39.6404138262961));
#264102=CARTESIAN_POINT('Ctrl Pts',(46.0925836924519,-59.2796343454175,
-39.6394845260398));
#264103=CARTESIAN_POINT('Ctrl Pts',(46.0038529790884,-59.3521266547998,
-39.6367222836243));
#264104=CARTESIAN_POINT('Ctrl Pts',(45.9736068426425,-59.3756113980778,
-39.6355720611743));
#264105=CARTESIAN_POINT('Ctrl Pts',(45.9272657300626,-59.4097723979471,
-39.6334997173803));
#264106=CARTESIAN_POINT('Ctrl Pts',(45.9116419552091,-59.4209913255156,
-39.6327502257672));
#264107=CARTESIAN_POINT('Ctrl Pts',(45.8800805125468,-59.4430611241672,
-39.631135078801));
#264108=CARTESIAN_POINT('Ctrl Pts',(45.8641078101822,-59.4539348059586,
-39.6302673429044));
#264109=CARTESIAN_POINT('Ctrl Pts',(45.8159067495927,-59.4858697254365,
-39.627498969587));
#264110=CARTESIAN_POINT('Ctrl Pts',(45.7834097421985,-59.5062439414457,
-39.6254354520693));
#264111=CARTESIAN_POINT('Ctrl Pts',(45.7176331363943,-59.5452482370454,
-39.6208772711381));
#264112=CARTESIAN_POINT('Ctrl Pts',(45.6843658790545,-59.5638704785003,
-39.6183833740186));
#264113=CARTESIAN_POINT('Ctrl Pts',(45.583444956553,-59.6171384596421,-39.6102663728808));
#264114=CARTESIAN_POINT('Ctrl Pts',(45.5146744890979,-59.6491909190302,
-39.6040093397971));
#264115=CARTESIAN_POINT('Ctrl Pts',(45.4093033900763,-59.6921245149476,
-39.5933616765527));
#264116=CARTESIAN_POINT('Ctrl Pts',(45.3738098248103,-59.7055767269039,
-39.589601735465));
#264117=CARTESIAN_POINT('Ctrl Pts',(45.3020779039712,-59.7307512611409,
-39.5816566274386));
#264118=CARTESIAN_POINT('Ctrl Pts',(45.2658207530533,-59.7424780352937,
-39.5774690099792));
#264119=CARTESIAN_POINT('Ctrl Pts',(45.1926264881235,-59.7641596514461,
-39.568671457456));
#264120=CARTESIAN_POINT('Ctrl Pts',(45.1555074107078,-59.7741563012212,
-39.5640375608608));
#264121=CARTESIAN_POINT('Ctrl Pts',(45.0812568665445,-59.7921791067291,
-39.5544265147621));
#264122=CARTESIAN_POINT('Ctrl Pts',(45.0440817477085,-59.8002278395378,
-39.549445784008));
#264123=CARTESIAN_POINT('Ctrl Pts',(44.9696261228349,-59.8144411184057,
-39.5391389954541));
#264124=CARTESIAN_POINT('Ctrl Pts',(44.9323469981084,-59.8206062349248,
-39.5338132734696));
#264125=CARTESIAN_POINT('Ctrl Pts',(44.8576879269541,-59.8310834316045,
-39.5228216022339));
#264126=CARTESIAN_POINT('Ctrl Pts',(44.820307974904,-59.835395411627,-39.517155635792));
#264127=CARTESIAN_POINT('Ctrl Pts',(44.708018468269,-59.8455761125523,-39.4996502226722));
#264128=CARTESIAN_POINT('Ctrl Pts',(44.6329372354107,-59.8486932135334,
-39.487300131016));
#264129=CARTESIAN_POINT('Ctrl Pts',(44.5200834526131,-59.8478515646575,
-39.4677634251584));
#264130=CARTESIAN_POINT('Ctrl Pts',(44.4823810949366,-59.846645023154,-39.4610735946688));
#264131=CARTESIAN_POINT('Ctrl Pts',(44.4258051146807,-59.8434395219468,
-39.4507882880789));
#264132=CARTESIAN_POINT('Ctrl Pts',(44.4069254653865,-59.8421361859431,
-39.4473147364688));
#264133=CARTESIAN_POINT('Ctrl Pts',(44.369137659976,-59.8390582137137,-39.440279278016));
#264134=CARTESIAN_POINT('Ctrl Pts',(44.3502459404613,-59.8372839246163,
-39.4367202553176));
#264135=CARTESIAN_POINT('Ctrl Pts',(44.293847621291,-59.8312837400404,-39.4259705727343));
#264136=CARTESIAN_POINT('Ctrl Pts',(44.2565162798962,-59.8263769106602,
-39.4186892078256));
#264137=CARTESIAN_POINT('Ctrl Pts',(44.1823865447478,-59.8147890715068,
-39.4039021067728));
#264138=CARTESIAN_POINT('Ctrl Pts',(44.1455864865373,-59.8081084264739,
-39.3963961507539));
#264139=CARTESIAN_POINT('Ctrl Pts',(44.035968213109,-59.7854494824361,-39.3735449366146));
#264140=CARTESIAN_POINT('Ctrl Pts',(43.9639303513108,-59.7668593620139,
-39.3578669828429));
#264141=CARTESIAN_POINT('Ctrl Pts',(43.8219158998824,-59.7227862146117,
-39.3256250679982));
#264142=CARTESIAN_POINT('Ctrl Pts',(43.7519290479738,-59.6972943553091,
-39.3090577736246));
#264143=CARTESIAN_POINT('Ctrl Pts',(43.6657831707481,-59.6610676287994,
-39.287788993689));
#264144=CARTESIAN_POINT('Ctrl Pts',(43.6486106593656,-59.6535962458977,
-39.2835040729686));
#264145=CARTESIAN_POINT('Ctrl Pts',(43.6144192936767,-59.6382222836229,
-39.2748824632482));
#264146=CARTESIAN_POINT('Ctrl Pts',(43.5973665746684,-59.6303022827778,
-39.2705368372966));
#264147=CARTESIAN_POINT('Ctrl Pts',(43.5465994091571,-59.6059619503591,
-39.2574615900898));
#264148=CARTESIAN_POINT('Ctrl Pts',(43.513329290924,-59.5889931579325,-39.2487084716788));
#264149=CARTESIAN_POINT('Ctrl Pts',(43.4805770970857,-59.5712767993712,
-39.2399079805728));
#264150=CARTESIAN_POINT('Ctrl Pts',(43.5555688340535,-59.234132410514,-39.6401263014865));
#264151=CARTESIAN_POINT('Ctrl Pts',(43.5271058320223,-59.2187187670665,
-39.6313258103806));
#264152=CARTESIAN_POINT('Ctrl Pts',(43.4991052518144,-59.2026624632065,
-39.6224818464091));
#264153=CARTESIAN_POINT('Ctrl Pts',(43.4440152092532,-59.1692838342202,
-39.6047076566125));
#264154=CARTESIAN_POINT('Ctrl Pts',(43.4169257916853,-59.1519614464883,
-39.5957774275967));
#264155=CARTESIAN_POINT('Ctrl Pts',(43.3370134128483,-59.0981105486717,
-39.5688575945475));
#264156=CARTESIAN_POINT('Ctrl Pts',(43.285543443658,-59.0597022696331,-39.5507390702919));
#264157=CARTESIAN_POINT('Ctrl Pts',(43.1862320317398,-58.9778459096351,
-39.5141533290284));
#264158=CARTESIAN_POINT('Ctrl Pts',(43.1383856292385,-58.9343938929635,
-39.4956843164029));
#264159=CARTESIAN_POINT('Ctrl Pts',(43.0464616123337,-58.8422984996412,
-39.4583915857769));
#264160=CARTESIAN_POINT('Ctrl Pts',(43.0031145131512,-58.7943886576613,
-39.4398645717558));
#264161=CARTESIAN_POINT('Ctrl Pts',(42.9214555277954,-58.694943387258,-39.4030322323516));
#264162=CARTESIAN_POINT('Ctrl Pts',(42.8831481853276,-58.6434115048881,
-39.3847285385198));
#264163=CARTESIAN_POINT('Ctrl Pts',(42.8294517117175,-58.5634128288845,
-39.3574423437733));
#264164=CARTESIAN_POINT('Ctrl Pts',(42.8121813055727,-58.5362957447343,
-39.348375225579));
#264165=CARTESIAN_POINT('Ctrl Pts',(42.7789076210676,-58.4811523680481,
-39.3302984210776));
#264166=CARTESIAN_POINT('Ctrl Pts',(42.7629042791111,-58.453126121455,-39.3212887307404));
#264167=CARTESIAN_POINT('Ctrl Pts',(42.7321838794578,-58.3961505394088,
-39.3033281639527));
#264168=CARTESIAN_POINT('Ctrl Pts',(42.7174704361412,-58.3672088695202,
-39.294379601599));
#264169=CARTESIAN_POINT('Ctrl Pts',(42.689344263748,-58.3083508831849,-39.2765339814759));
#264170=CARTESIAN_POINT('Ctrl Pts',(42.6760419603829,-58.2786633846033,
-39.2677065167051));
#264171=CARTESIAN_POINT('Ctrl Pts',(42.6509592537523,-58.2188366747008,
-39.2502567671988));
#264172=CARTESIAN_POINT('Ctrl Pts',(42.6391740738076,-58.1886873909247,
-39.2416314356366));
#264173=CARTESIAN_POINT('Ctrl Pts',(42.6171012127209,-58.1279234454293,
-39.2245791344233));
#264174=CARTESIAN_POINT('Ctrl Pts',(42.6068134424726,-58.0973084744714,
-39.2161520818859));
#264175=CARTESIAN_POINT('Ctrl Pts',(42.5781884268765,-58.0047666909868,
-39.1911685383331));
#264176=CARTESIAN_POINT('Ctrl Pts',(42.5620841140238,-57.9421424384458,
-39.1749084291127));
#264177=CARTESIAN_POINT('Ctrl Pts',(42.542463526333,-57.8467994028925,-39.151128790794));
#264178=CARTESIAN_POINT('Ctrl Pts',(42.5366797518884,-57.8147770619196,
-39.1433026580524));
#264179=CARTESIAN_POINT('Ctrl Pts',(42.5266559992737,-57.7502668409957,
-39.1278621295069));
#264180=CARTESIAN_POINT('Ctrl Pts',(42.5224110777105,-57.7177324038865,
-39.1202370477892));
#264181=CARTESIAN_POINT('Ctrl Pts',(42.5155196559844,-57.652328321118,-39.1052379331815));
#264182=CARTESIAN_POINT('Ctrl Pts',(42.5128936513538,-57.6196819945454,
-39.0979145111089));
#264183=CARTESIAN_POINT('Ctrl Pts',(42.5092450689372,-57.5543870588034,
-39.0835903034871));
#264184=CARTESIAN_POINT('Ctrl Pts',(42.5082244669781,-57.5217572823762,
-39.0765938343906));
#264185=CARTESIAN_POINT('Ctrl Pts',(42.5075544726465,-57.4239203249817,
-39.0560992299731));
#264186=CARTESIAN_POINT('Ctrl Pts',(42.5102915889976,-57.3587654025749,
-39.043094782529));
#264187=CARTESIAN_POINT('Ctrl Pts',(42.5192017059061,-57.2611370939764,
-39.0245895647869));
#264188=CARTESIAN_POINT('Ctrl Pts',(42.522973744208,-57.2286116980208,-39.0185883272243));
#264189=CARTESIAN_POINT('Ctrl Pts',(42.5321446715301,-57.163595959261,-39.0069262192674));
#264190=CARTESIAN_POINT('Ctrl Pts',(42.5375469638235,-57.1310925726591,
-39.0012633293817));
#264191=CARTESIAN_POINT('Ctrl Pts',(42.5499993493055,-57.0661735854286,
-38.9902944808063));
#264192=CARTESIAN_POINT('Ctrl Pts',(42.5570860671587,-57.033621871048,-38.9849676901412));
#264193=CARTESIAN_POINT('Ctrl Pts',(42.5727873916265,-56.9692679908499,
-38.9747855696665));
#264194=CARTESIAN_POINT('Ctrl Pts',(42.5814163631431,-56.9373636386801,
-38.969911897523));
#264195=CARTESIAN_POINT('Ctrl Pts',(42.6002044275548,-56.8741385448439,
-38.9606030691666));
#264196=CARTESIAN_POINT('Ctrl Pts',(42.6103644732139,-56.8428100941247,
-38.9561665014482));
#264197=CARTESIAN_POINT('Ctrl Pts',(42.6322071886494,-56.7807177933216,
-38.947727479919));
#264198=CARTESIAN_POINT('Ctrl Pts',(42.6438898663583,-56.7499539462467,
-38.9437250276736));
#264199=CARTESIAN_POINT('Ctrl Pts',(42.6687796751254,-56.6889914341204,
-38.9361557741806));
#264200=CARTESIAN_POINT('Ctrl Pts',(42.6819867909859,-56.658792763486,-38.9325889680638));
#264201=CARTESIAN_POINT('Ctrl Pts',(42.7099385396534,-56.5989653584369,
-38.9258956733729));
#264202=CARTESIAN_POINT('Ctrl Pts',(42.7246831328038,-56.5693366093568,
-38.9227691730914));
#264203=CARTESIAN_POINT('Ctrl Pts',(42.7557346180894,-56.510658153127,-38.9169644323897));
#264204=CARTESIAN_POINT('Ctrl Pts',(42.7720318723629,-56.4816246493906,
-38.9142875723637));
#264205=CARTESIAN_POINT('Ctrl Pts',(42.8062644061236,-56.4240855769913,
-38.909388005867));
#264206=CARTESIAN_POINT('Ctrl Pts',(42.8240696175392,-56.3958000441502,
-38.9071842157982));
#264207=CARTESIAN_POINT('Ctrl Pts',(42.8793348313062,-56.3126951718662,
-38.9013291247197));
#264208=CARTESIAN_POINT('Ctrl Pts',(42.9187435313913,-56.259400561899,-38.8984073047134));
#264209=CARTESIAN_POINT('Ctrl Pts',(43.0025486921197,-56.1570720601927,
-38.8945093168885));
#264210=CARTESIAN_POINT('Ctrl Pts',(43.0469652685517,-56.1080071974563,
-38.8935308647847));
#264211=CARTESIAN_POINT('Ctrl Pts',(43.1173453422034,-56.0376384736874,
-38.8935332517581));
#264212=CARTESIAN_POINT('Ctrl Pts',(43.1414589512102,-56.0146993759999,
-38.8937804665284));
#264213=CARTESIAN_POINT('Ctrl Pts',(43.178561457947,-55.981132370469,-38.8945245726641));
#264214=CARTESIAN_POINT('Ctrl Pts',(43.1910981146608,-55.9700726732162,
-38.8948354181272));
#264215=CARTESIAN_POINT('Ctrl Pts',(43.2164887431531,-55.9482340721744,
-38.8955829564625));
#264216=CARTESIAN_POINT('Ctrl Pts',(43.2293527169208,-55.937448113455,-38.8960202693949));
#264217=CARTESIAN_POINT('Ctrl Pts',(43.2682112021707,-55.9056905804555,
-38.8975145638021));
#264218=CARTESIAN_POINT('Ctrl Pts',(43.2945322632909,-55.8852612363732,
-38.8987542986482));
#264219=CARTESIAN_POINT('Ctrl Pts',(43.3480003156045,-55.8458489068529,
-38.9017113990668));
#264220=CARTESIAN_POINT('Ctrl Pts',(43.3751451625608,-55.8268670886173,
-38.9034285584852));
#264221=CARTESIAN_POINT('Ctrl Pts',(43.457794616026,-55.772063647161,-38.90928492419));
#264222=CARTESIAN_POINT('Ctrl Pts',(43.5145115393775,-55.7383794675986,
-38.9141275726255));
#264223=CARTESIAN_POINT('Ctrl Pts',(43.6019985559746,-55.6921046980431,
-38.9227867126206));
#264224=CARTESIAN_POINT('Ctrl Pts',(43.6315635162974,-55.67738956075,-38.925906003916));
#264225=CARTESIAN_POINT('Ctrl Pts',(43.6915053978043,-55.6493906033967,
-38.932613415813));
#264226=CARTESIAN_POINT('Ctrl Pts',(43.7218910354095,-55.6361042305882,
-38.9362028291725));
#264227=CARTESIAN_POINT('Ctrl Pts',(43.7834519549885,-55.6109950253045,
-38.9438515723833));
#264228=CARTESIAN_POINT('Ctrl Pts',(43.8147380697121,-55.5991389154848,
-38.9479271520235));
#264229=CARTESIAN_POINT('Ctrl Pts',(43.8773633283321,-55.577177590229,-38.9564529085545));
#264230=CARTESIAN_POINT('Ctrl Pts',(43.9088374259754,-55.5670132823478,
-38.9609190102379));
#264231=CARTESIAN_POINT('Ctrl Pts',(43.9720262322937,-55.5483141725143,
-38.9702386744095));
#264232=CARTESIAN_POINT('Ctrl Pts',(44.003753687147,-55.5397738324173,-38.9750937504595));
#264233=CARTESIAN_POINT('Ctrl Pts',(44.0674709105135,-55.5242876491131,
-38.9851874732096));
#264234=CARTESIAN_POINT('Ctrl Pts',(44.0994606850175,-55.51734184284,-38.9904261294562));
#264235=CARTESIAN_POINT('Ctrl Pts',(44.1637007452764,-55.5050328545072,
-39.0012829705492));
#264236=CARTESIAN_POINT('Ctrl Pts',(44.1959510329844,-55.4996696848857,
-39.0069011591118));
#264237=CARTESIAN_POINT('Ctrl Pts',(44.2607122139946,-55.4905255962476,
-39.0185157495185));
#264238=CARTESIAN_POINT('Ctrl Pts',(44.2932231053838,-55.4867446662453,
-39.0245121495422));
#264239=CARTESIAN_POINT('Ctrl Pts',(44.358507484825,-55.4807761715604,-39.0368845580029));
#264240=CARTESIAN_POINT('Ctrl Pts',(44.3912827624034,-55.4785893296048,
-39.043261085944));
#264241=CARTESIAN_POINT('Ctrl Pts',(44.4570926895081,-55.4758289910908,
-39.0563958303051));
#264242=CARTESIAN_POINT('Ctrl Pts',(44.4901875455791,-55.475262761327,-39.0631680460238));
#264243=CARTESIAN_POINT('Ctrl Pts',(44.5558450459825,-55.4757592686521,
-39.076931276667));
#264244=CARTESIAN_POINT('Ctrl Pts',(44.5885613296957,-55.476813330479,-39.0839525032381));
#264245=CARTESIAN_POINT('Ctrl Pts',(44.6536810701527,-55.4805040184252,
-39.0982487342192));
#264246=CARTESIAN_POINT('Ctrl Pts',(44.6861002081385,-55.4831398985796,
-39.1055268520681));
#264247=CARTESIAN_POINT('Ctrl Pts',(44.7829416988568,-55.4933857216518,
-39.1277439201117));
#264248=CARTESIAN_POINT('Ctrl Pts',(44.8469489879605,-55.5033290244897,
-39.1430647851939));
#264249=CARTESIAN_POINT('Ctrl Pts',(44.9421358674272,-55.5228833885463,
-39.1667986859967));
#264250=CARTESIAN_POINT('Ctrl Pts',(44.9737272566983,-55.5301760197046,
-39.1748356365191));
#264251=CARTESIAN_POINT('Ctrl Pts',(45.0366329635135,-55.5463222396588,
-39.1911617192672));
#264252=CARTESIAN_POINT('Ctrl Pts',(45.0679413951409,-55.5551744507282,
-39.1994493506505));
#264253=CARTESIAN_POINT('Ctrl Pts',(45.1303008713406,-55.5744680900885,
-39.2162854783706));
#264254=CARTESIAN_POINT('Ctrl Pts',(45.1613388911671,-55.5849125268946,
-39.2248318477494));
#264255=CARTESIAN_POINT('Ctrl Pts',(45.2225438737999,-55.6071888828167,
-39.2420164625862));
#264256=CARTESIAN_POINT('Ctrl Pts',(45.2528222941887,-55.6190542948094,
-39.2506846042053));
#264257=CARTESIAN_POINT('Ctrl Pts',(45.3126689940191,-55.6442024946607,
-39.2681514288968));
#264258=CARTESIAN_POINT('Ctrl Pts',(45.3422489057867,-55.6574888345125,
-39.2769532439202));
#264259=CARTESIAN_POINT('Ctrl Pts',(45.4007247066096,-55.6854804145847,
-39.294692423228));
#264260=CARTESIAN_POINT('Ctrl Pts',(45.4296205949023,-55.7001856561536,
-39.303629788134));
#264261=CARTESIAN_POINT('Ctrl Pts',(45.4867262971545,-55.7310195886299,
-39.3216398779287));
#264262=CARTESIAN_POINT('Ctrl Pts',(45.5149276816543,-55.7471431755038,
-39.3307098362187));
#264263=CARTESIAN_POINT('Ctrl Pts',(45.5706711208682,-55.7808489297168,
-39.3489970530329));
#264264=CARTESIAN_POINT('Ctrl Pts',(45.5980410702153,-55.7983266659973,
-39.3581577775872));
#264265=CARTESIAN_POINT('Ctrl Pts',(45.6785013081512,-55.8525005642884,
-39.3856341820567));
#264266=CARTESIAN_POINT('Ctrl Pts',(45.7300937365428,-55.8910026267882,
-39.4039886295733));
#264267=CARTESIAN_POINT('Ctrl Pts',(45.8291734689818,-55.9726265658168,
-39.4407373523715));
#264268=CARTESIAN_POINT('Ctrl Pts',(45.8766781960947,-56.0157559494116,
-39.4591367574256));
#264269=CARTESIAN_POINT('Ctrl Pts',(45.9448676798055,-56.0839431609313,
-39.486773461584));
#264270=CARTESIAN_POINT('Ctrl Pts',(45.9670854652505,-56.1072552989447,
-39.4959919837403));
#264271=CARTESIAN_POINT('Ctrl Pts',(46.0104833820224,-56.1550611161397,
-39.514441907174));
#264272=CARTESIAN_POINT('Ctrl Pts',(46.0316544908778,-56.1795440550238,
-39.5236693153279));
#264273=CARTESIAN_POINT('Ctrl Pts',(46.0626444084099,-56.2172045128319,
-39.5375324394833));
#264274=CARTESIAN_POINT('Ctrl Pts',(46.0728372208042,-56.2299044661098,
-39.5421533199052));
#264275=CARTESIAN_POINT('Ctrl Pts',(46.0928503481787,-56.2554721633656,
-39.5513497426116));
#264276=CARTESIAN_POINT('Ctrl Pts',(46.1026906457484,-56.268363961677,-39.5559341791666));
#264277=CARTESIAN_POINT('Ctrl Pts',(46.1316831401522,-56.3073189842252,
-39.5696313840511));
#264278=CARTESIAN_POINT('Ctrl Pts',(46.150335839206,-56.3336964338945,-39.5787008712277));
#264279=CARTESIAN_POINT('Ctrl Pts',(46.2042522556268,-56.4139854185625,
-39.6057081391376));
#264280=CARTESIAN_POINT('Ctrl Pts',(46.2375098264188,-56.4690893442278,
-39.6234591220454));
#264281=CARTESIAN_POINT('Ctrl Pts',(46.2833691088139,-56.5540831173889,
-39.6497034031462));
#264282=CARTESIAN_POINT('Ctrl Pts',(46.2979840983916,-56.5828056408614,
-39.6583880699236));
#264283=CARTESIAN_POINT('Ctrl Pts',(46.3258597433761,-56.6410397267288,
-39.6756301843647));
#264284=CARTESIAN_POINT('Ctrl Pts',(46.3391204674906,-56.6705512493805,
-39.6841876372386));
#264285=CARTESIAN_POINT('Ctrl Pts',(46.3642666109142,-56.7303753620795,
-39.7011741527));
#264286=CARTESIAN_POINT('Ctrl Pts',(46.3761452467366,-56.7606695516432,
-39.7095981876039));
#264287=CARTESIAN_POINT('Ctrl Pts',(46.3985229292237,-56.8221506906604,
-39.7263359298937));
#264288=CARTESIAN_POINT('Ctrl Pts',(46.408953127825,-56.8531540648449,-39.7345992445483));
#264289=CARTESIAN_POINT('Ctrl Pts',(46.4378282073617,-56.9464971719099,
-39.7589554288027));
#264290=CARTESIAN_POINT('Ctrl Pts',(46.4539722273909,-57.0094025633998,
-39.7746840779066));
#264291=CARTESIAN_POINT('Ctrl Pts',(46.4800786523228,-57.1364634441695,
-39.8051180948244));
#264292=CARTESIAN_POINT('Ctrl Pts',(46.4900502528004,-57.200634055062,-39.8198283239538));
#264293=CARTESIAN_POINT('Ctrl Pts',(46.500315603497,-57.2978584721872,-39.8411276298225));
#264294=CARTESIAN_POINT('Ctrl Pts',(46.5029542464308,-57.3304316164207,
-39.8481002042598));
#264295=CARTESIAN_POINT('Ctrl Pts',(46.5066358246239,-57.3959003914897,
-39.8617846600929));
#264296=CARTESIAN_POINT('Ctrl Pts',(46.5076790508278,-57.4288265228613,
-39.8685026266565));
#264297=CARTESIAN_POINT('Ctrl Pts',(46.5081278097802,-57.4949097791684,
-39.8816524618054));
#264298=CARTESIAN_POINT('Ctrl Pts',(46.5075338158641,-57.5278164208752,
-39.8880349335079));
#264299=CARTESIAN_POINT('Ctrl Pts',(46.5047352860362,-57.5934604589744,
-39.9004413805986));
#264300=CARTESIAN_POINT('Ctrl Pts',(46.5025305994736,-57.6261815712493,
-39.9064621065048));
#264301=CARTESIAN_POINT('Ctrl Pts',(46.4935211674923,-57.7240445911198,
-39.9239832254356));
#264302=CARTESIAN_POINT('Ctrl Pts',(46.4843263421389,-57.7888868451408,
-39.9349437553631));
#264303=CARTESIAN_POINT('Ctrl Pts',(46.4657284705721,-57.88554690184,-39.9503056068378));
#264304=CARTESIAN_POINT('Ctrl Pts',(46.4587269718586,-57.9176662081948,
-39.9552461080624));
#264305=CARTESIAN_POINT('Ctrl Pts',(46.4430976792663,-57.9817005180905,
-39.9647630061231));
#264306=CARTESIAN_POINT('Ctrl Pts',(46.4344649635437,-58.0136288811654,
-39.9693410579289));
#264307=CARTESIAN_POINT('Ctrl Pts',(46.4155593362243,-58.0772235214093,
-39.9781199126733));
#264308=CARTESIAN_POINT('Ctrl Pts',(46.405234653673,-58.1090270368304,-39.9823374861317));
#264309=CARTESIAN_POINT('Ctrl Pts',(46.3831314756339,-58.1717229328585,
-39.9903054512315));
#264310=CARTESIAN_POINT('Ctrl Pts',(46.3713300900435,-58.2027117021187,
-39.9940702923682));
#264311=CARTESIAN_POINT('Ctrl Pts',(46.346258426029,-58.2639404804981,-40.001162653254));
#264312=CARTESIAN_POINT('Ctrl Pts',(46.3329866824905,-58.2941873699786,
-40.0044912371692));
#264313=CARTESIAN_POINT('Ctrl Pts',(46.3049822647675,-58.3539515341542,
-40.010717204176));
#264314=CARTESIAN_POINT('Ctrl Pts',(46.290249579368,-58.3834688032905,-40.0136145833441));
#264315=CARTESIAN_POINT('Ctrl Pts',(46.259323329411,-58.4417737040611,-40.0189788375594));
#264316=CARTESIAN_POINT('Ctrl Pts',(46.2431297759597,-58.470561341271,-40.0214457154618));
#264317=CARTESIAN_POINT('Ctrl Pts',(46.2092710685098,-58.5274015813425,
-40.0259463992273));
#264318=CARTESIAN_POINT('Ctrl Pts',(46.1916059489149,-58.5554542014027,
-40.0279802149935));
#264319=CARTESIAN_POINT('Ctrl Pts',(46.1547822130534,-58.6108134350802,
-40.0316088293047));
#264320=CARTESIAN_POINT('Ctrl Pts',(46.1356364139942,-58.6381026215683,
-40.0332027257756));
#264321=CARTESIAN_POINT('Ctrl Pts',(46.0957663843932,-58.6919878518662,
-40.0359456143505));
#264322=CARTESIAN_POINT('Ctrl Pts',(46.0751805717983,-58.7183939621751,
-40.0370845256383));
#264323=CARTESIAN_POINT('Ctrl Pts',(46.0117857527956,-58.7956381443108,
-40.0397943891545));
#264324=CARTESIAN_POINT('Ctrl Pts',(45.9671995057833,-58.8447447093681,
-40.0406786442178));
#264325=CARTESIAN_POINT('Ctrl Pts',(45.8735317190067,-58.9381748222192,
-40.0406321472099));
#264326=CARTESIAN_POINT('Ctrl Pts',(45.8244348914145,-58.9825210802309,
-40.0397028469535));
#264327=CARTESIAN_POINT('Ctrl Pts',(45.7473997315196,-59.0454393048068,
-40.036940604538));
#264328=CARTESIAN_POINT('Ctrl Pts',(45.7211395471819,-59.0658214386729,
-40.0357903820881));
#264329=CARTESIAN_POINT('Ctrl Pts',(45.6809042968051,-59.0954678458765,
-40.0337180382941));
#264330=CARTESIAN_POINT('Ctrl Pts',(45.6673389080279,-59.1052038578702,
-40.032968546681));
#264331=CARTESIAN_POINT('Ctrl Pts',(45.6399352188299,-59.1243559363232,
-40.0313533997148));
#264332=CARTESIAN_POINT('Ctrl Pts',(45.6260664980794,-59.1337917962429,
-40.0304856638181));
#264333=CARTESIAN_POINT('Ctrl Pts',(45.584214102782,-59.161503132938,-40.0277172905008));
#264334=CARTESIAN_POINT('Ctrl Pts',(45.5559966208921,-59.1791815977629,
-40.0256537729831));
#264335=CARTESIAN_POINT('Ctrl Pts',(45.4988807301693,-59.2130228222466,
-40.0210955920518));
#264336=CARTESIAN_POINT('Ctrl Pts',(45.469993037139,-59.2291787807534,-40.0186016949324));
#264337=CARTESIAN_POINT('Ctrl Pts',(45.3823561363204,-59.2753882889069,
-40.0104846937946));
#264338=CARTESIAN_POINT('Ctrl Pts',(45.3226351503952,-59.3031882186041,
-40.0042276607109));
#264339=CARTESIAN_POINT('Ctrl Pts',(45.2311259835243,-59.3404168518855,
-39.9935799974664));
#264340=CARTESIAN_POINT('Ctrl Pts',(45.2003010959947,-59.3520799076811,
-39.9898200563787));
#264341=CARTESIAN_POINT('Ctrl Pts',(45.1380032580586,-59.3739026770269,
-39.9818749483524));
#264342=CARTESIAN_POINT('Ctrl Pts',(45.1065139829285,-59.3840662456593,
-39.977687330893));
#264343=CARTESIAN_POINT('Ctrl Pts',(45.0429436614079,-59.4028535501948,
-39.9688897783697));
#264344=CARTESIAN_POINT('Ctrl Pts',(45.0107045696338,-59.4115134856595,
-39.9642558817745));
#264345=CARTESIAN_POINT('Ctrl Pts',(44.9462144135346,-59.4271214577326,
-39.9546448356758));
#264346=CARTESIAN_POINT('Ctrl Pts',(44.9139254426396,-59.4340890792738,
-39.9496641049217));
#264347=CARTESIAN_POINT('Ctrl Pts',(44.849254794685,-59.446387333888,-39.9393573163679));
#264348=CARTESIAN_POINT('Ctrl Pts',(44.8168743179144,-59.451718463481,-39.9340315943834));
#264349=CARTESIAN_POINT('Ctrl Pts',(44.752024642773,-59.4607707923529,-39.9230399231476));
#264350=CARTESIAN_POINT('Ctrl Pts',(44.7195554394538,-59.464491904643,-39.9173739567058));
#264351=CARTESIAN_POINT('Ctrl Pts',(44.622016134105,-59.4732614616325,-39.899868543586));
#264352=CARTESIAN_POINT('Ctrl Pts',(44.5567952038801,-59.4759192557151,
-39.8875184519297));
#264353=CARTESIAN_POINT('Ctrl Pts',(44.4587589187831,-59.4751124713245,
-39.8679817460721));
#264354=CARTESIAN_POINT('Ctrl Pts',(44.4260062405338,-59.4740390035135,
-39.8612919155826));
#264355=CARTESIAN_POINT('Ctrl Pts',(44.3768568603989,-59.4712162368822,
-39.8510066089926));
#264356=CARTESIAN_POINT('Ctrl Pts',(44.3604553547125,-59.470071279602,-39.8475330573825));
#264357=CARTESIAN_POINT('Ctrl Pts',(44.3276272864905,-59.4673718881716,
-39.8404975989298));
#264358=CARTESIAN_POINT('Ctrl Pts',(44.3112150025957,-59.4658177666042,
-39.8369385762314));
#264359=CARTESIAN_POINT('Ctrl Pts',(44.2622182182766,-59.4605671446247,
-39.8261888936481));
#264360=CARTESIAN_POINT('Ctrl Pts',(44.2297855397697,-59.4562791768359,
-39.8189075287393));
#264361=CARTESIAN_POINT('Ctrl Pts',(44.1653820410688,-59.4461622151957,
-39.8041204276866));
#264362=CARTESIAN_POINT('Ctrl Pts',(44.1334097751946,-59.4403335371186,
-39.7966144716676));
#264363=CARTESIAN_POINT('Ctrl Pts',(44.0381705631049,-59.4205744031982,
-39.7737632575285));
#264364=CARTESIAN_POINT('Ctrl Pts',(43.9755798614833,-59.4043753530904,
-39.7580853037566));
#264365=CARTESIAN_POINT('Ctrl Pts',(43.8521846744312,-59.36599016115,-39.725843388912));
#264366=CARTESIAN_POINT('Ctrl Pts',(43.791371268692,-59.343796339026,-39.7092760945378));
#264367=CARTESIAN_POINT('Ctrl Pts',(43.7165137253937,-59.3122653970299,
-39.6880073146029));
#264368=CARTESIAN_POINT('Ctrl Pts',(43.7015912939536,-59.3057628682929,
-39.6837223938823));
#264369=CARTESIAN_POINT('Ctrl Pts',(43.6718796312441,-59.2923832966048,
-39.675100784162));
#264370=CARTESIAN_POINT('Ctrl Pts',(43.6570609707452,-59.2854910954552,
-39.6707551582104));
#264371=CARTESIAN_POINT('Ctrl Pts',(43.6129442606048,-59.2643105724085,
-39.6576799110036));
#264372=CARTESIAN_POINT('Ctrl Pts',(43.5840318360846,-59.2495460539614,
-39.6489267925925));
#264373=CARTESIAN_POINT('Ctrl Pts',(43.5555688340535,-59.234132410514,-39.6401263014865));
#264374=CARTESIAN_POINT('',(45.673922755161,-55.5192637623964,-38.9124165672108));
#264375=CARTESIAN_POINT('',(45.6739227548708,-55.5192637629142,-38.9124165672458));
#264376=CARTESIAN_POINT('',(43.4805771074159,-59.5712767529304,-39.2399080357012));
#264377=CARTESIAN_POINT('Ctrl Pts',(43.4805771074156,-59.5712767529309,
-39.2399080357013));
#264378=CARTESIAN_POINT('Ctrl Pts',(43.2084983655955,-59.4241035716486,
-39.1668006710783));
#264379=CARTESIAN_POINT('Ctrl Pts',(42.9694351505993,-59.2238071870063,
-39.0896600468055));
#264380=CARTESIAN_POINT('Ctrl Pts',(42.5877499895759,-58.7449876099978,
-38.9374284505921));
#264381=CARTESIAN_POINT('Ctrl Pts',(42.4470026012736,-58.4716973584526,
-38.8636131689055));
#264382=CARTESIAN_POINT('Ctrl Pts',(42.2829188141298,-57.8937343216347,
-38.7304874981619));
#264383=CARTESIAN_POINT('Ctrl Pts',(42.2573533055641,-57.5951189999158,
-38.6719031562341));
#264384=CARTESIAN_POINT('Ctrl Pts',(42.3215651079466,-57.0104777473371,
-38.5774816051817));
#264385=CARTESIAN_POINT('Ctrl Pts',(42.4073752536078,-56.7295195546235,
-38.5418707047797));
#264386=CARTESIAN_POINT('Ctrl Pts',(42.6817387181495,-56.2116483083903,
-38.4973862220026));
#264387=CARTESIAN_POINT('Ctrl Pts',(42.8670639833424,-55.9810885822738,
-38.4890931163589));
#264388=CARTESIAN_POINT('Ctrl Pts',(43.3113300107118,-55.6043418037155,
-38.5014475290099));
#264389=CARTESIAN_POINT('Ctrl Pts',(43.563676465166,-55.4612112790788,-38.5214440607413));
#264390=CARTESIAN_POINT('Ctrl Pts',(44.1136708092855,-55.2727963636881,
-38.5873481888105));
#264391=CARTESIAN_POINT('Ctrl Pts',(44.4057389282975,-55.2321785575282,
-38.6330729320601));
#264392=CARTESIAN_POINT('Ctrl Pts',(44.8666382983243,-55.2549155285843,
-38.7204514563686));
#264393=CARTESIAN_POINT('Ctrl Pts',(45.0356772772846,-55.2823862237002,
-38.7558506821669));
#264394=CARTESIAN_POINT('Ctrl Pts',(45.364666265058,-55.3740467165804,-38.8313288315555));
#264395=CARTESIAN_POINT('Ctrl Pts',(45.5236259139144,-55.4381875697362,
-38.8712190690491));
#264396=CARTESIAN_POINT('Ctrl Pts',(45.6739227548708,-55.5192637629143,
-38.9124165672458));
#264397=CARTESIAN_POINT('',(43.4805771074159,-59.5712767529304,-39.2399080357012));
#264398=CARTESIAN_POINT('Origin',(44.615955334411,-57.3789268591943,-39.4599679236673));
#264399=CARTESIAN_POINT('Origin',(48.2118204350714,-55.8145579159494,-52.64995));
#264400=CARTESIAN_POINT('Ctrl Pts',(42.839207175268,-57.4754524783491,-52.64995));
#264401=CARTESIAN_POINT('Ctrl Pts',(42.8226659458708,-57.633184469963,-52.64995));
#264402=CARTESIAN_POINT('Ctrl Pts',(42.8274712764287,-57.792393072249,-52.64995));
#264403=CARTESIAN_POINT('Ctrl Pts',(42.8786574174949,-58.0993235421715,
-52.64995));
#264404=CARTESIAN_POINT('Ctrl Pts',(42.9232286878868,-58.2458922062675,
-52.64995));
#264405=CARTESIAN_POINT('Ctrl Pts',(43.075036817329,-58.5811601802315,-52.64995));
#264406=CARTESIAN_POINT('Ctrl Pts',(43.1992049518545,-58.7594027873514,
-52.64995));
#264407=CARTESIAN_POINT('Ctrl Pts',(43.5542933458002,-59.1104583338343,
-52.64995));
#264408=CARTESIAN_POINT('Ctrl Pts',(43.7742269286883,-59.2312964387871,
-52.64995));
#264409=CARTESIAN_POINT('Ctrl Pts',(44.0795088334533,-59.3596331192527,
-52.64995));
#264410=CARTESIAN_POINT('Ctrl Pts',(44.2169771822695,-59.4004713032236,
-52.64995));
#264411=CARTESIAN_POINT('Ctrl Pts',(44.4991010430761,-59.4516685795711,
-52.64995));
#264412=CARTESIAN_POINT('Ctrl Pts',(44.6429009445505,-59.4617078816742,
-52.64995));
#264413=CARTESIAN_POINT('Ctrl Pts',(44.7865238868913,-59.4559569492311,
-52.64995));
#264414=CARTESIAN_POINT('Ctrl Pts',(46.5079524583205,-57.4754524783491,
-52.64995));
#264415=CARTESIAN_POINT('Ctrl Pts',(46.4950120245218,-57.3275618063643,
-52.64995));
#264416=CARTESIAN_POINT('Ctrl Pts',(46.4647658835114,-57.1817042732835,
-52.64995));
#264417=CARTESIAN_POINT('Ctrl Pts',(46.3748033228779,-56.9120256688023,
-52.64995));
#264418=CARTESIAN_POINT('Ctrl Pts',(46.3180752819212,-56.7881799556783,
-52.64995));
#264419=CARTESIAN_POINT('Ctrl Pts',(46.1241199408223,-56.4626040795241,
-52.64995));
#264420=CARTESIAN_POINT('Ctrl Pts',(45.960561722969,-56.2797546389996,-52.64995));
#264421=CARTESIAN_POINT('Ctrl Pts',(45.6181630929699,-56.0202600517664,
-52.64995));
#264422=CARTESIAN_POINT('Ctrl Pts',(45.4037244819502,-55.8912169339011,
-52.6499500000282));
#264423=CARTESIAN_POINT('Ctrl Pts',(44.9862869603902,-55.7833848066862,
-52.6499500000282));
#264424=CARTESIAN_POINT('Ctrl Pts',(44.8386017522404,-55.7653378340959,
-52.64995));
#264425=CARTESIAN_POINT('Ctrl Pts',(44.5503390053884,-55.7682194115044,
-52.64995));
#264426=CARTESIAN_POINT('Ctrl Pts',(44.4109642294216,-55.7870757183414,
-52.64995));
#264427=CARTESIAN_POINT('Ctrl Pts',(44.2755200796093,-55.8229737314248,
-52.64995));
#264428=CARTESIAN_POINT('Origin',(44.5079524583205,-57.4754524783491,-52.920575));
#264429=CARTESIAN_POINT('Ctrl Pts',(42.839207175268,-57.4754524783491,-52.4912));
#264430=CARTESIAN_POINT('Ctrl Pts',(42.839207175268,-58.4389030167283,-52.4328666666667));
#264431=CARTESIAN_POINT('Ctrl Pts',(43.6735798167943,-58.920628285918,-52.3745333333334));
#264432=CARTESIAN_POINT('Ctrl Pts',(44.5079524583205,-59.4023535551075,
-52.3162000000001));
#264433=CARTESIAN_POINT('Ctrl Pts',(45.3423250998467,-58.920628285918,-52.2578666666667));
#264434=CARTESIAN_POINT('Ctrl Pts',(46.1766977413729,-58.4389030167283,
-52.1995333333334));
#264435=CARTESIAN_POINT('Ctrl Pts',(46.1766977413729,-57.4754524783491,
-52.1412));
#264436=CARTESIAN_POINT('Ctrl Pts',(46.1766977413729,-56.5120019399699,
-52.0828666666667));
#264437=CARTESIAN_POINT('Ctrl Pts',(45.3423250998467,-56.0302766707802,
-52.0245333333333));
#264438=CARTESIAN_POINT('Ctrl Pts',(44.5079524583205,-55.5485514015906,
-51.9662));
#264439=CARTESIAN_POINT('Ctrl Pts',(43.6735798167943,-56.0302766707802,
-51.9078666666667));
#264440=CARTESIAN_POINT('Ctrl Pts',(42.839207175268,-56.5120019399698,-51.8495333333334));
#264441=CARTESIAN_POINT('Ctrl Pts',(42.839207175268,-57.4754524783491,-51.7912));
#264442=CARTESIAN_POINT('Ctrl Pts',(42.839207175268,-57.4754524783491,-52.64995));
#264443=CARTESIAN_POINT('Ctrl Pts',(42.839207175268,-58.4389030167283,-52.5916166666667));
#264444=CARTESIAN_POINT('Ctrl Pts',(43.6735798167943,-58.920628285918,-52.5332833333334));
#264445=CARTESIAN_POINT('Ctrl Pts',(44.5079524583205,-59.4023535551075,
-52.4749500000001));
#264446=CARTESIAN_POINT('Ctrl Pts',(45.3423250998467,-58.920628285918,-52.4166166666667));
#264447=CARTESIAN_POINT('Ctrl Pts',(46.1766977413729,-58.4389030167283,
-52.3582833333334));
#264448=CARTESIAN_POINT('Ctrl Pts',(46.1766977413729,-57.4754524783491,
-52.29995));
#264449=CARTESIAN_POINT('Ctrl Pts',(46.1766977413729,-56.5120019399699,
-52.2416166666667));
#264450=CARTESIAN_POINT('Ctrl Pts',(45.3423250998467,-56.0302766707802,
-52.1832833333333));
#264451=CARTESIAN_POINT('Ctrl Pts',(44.5079524583205,-55.5485514015906,
-52.12495));
#264452=CARTESIAN_POINT('Ctrl Pts',(43.6735798167943,-56.0302766707802,
-52.0666166666667));
#264453=CARTESIAN_POINT('Ctrl Pts',(42.839207175268,-56.5120019399698,-52.0082833333333));
#264454=CARTESIAN_POINT('Ctrl Pts',(42.839207175268,-57.4754524783491,-51.94995));
#264455=CARTESIAN_POINT('Ctrl Pts',(46.5766932247459,-57.4754524783491,
-52.6102625));
#264456=CARTESIAN_POINT('Ctrl Pts',(46.5766932247459,-56.2810644399698,
-52.5519291666666));
#264457=CARTESIAN_POINT('Ctrl Pts',(45.5423228415332,-55.6838704207802,
-52.4935958333333));
#264458=CARTESIAN_POINT('Ctrl Pts',(44.5079524583205,-55.0866764015906,
-52.4352625000001));
#264459=CARTESIAN_POINT('Ctrl Pts',(43.4735820751078,-55.6838704207802,
-52.3769291666667));
#264460=CARTESIAN_POINT('Ctrl Pts',(42.4392116918951,-56.2810644399698,
-52.3185958333334));
#264461=CARTESIAN_POINT('Ctrl Pts',(42.439211691895,-57.4754524783491,-52.2602625));
#264462=CARTESIAN_POINT('Ctrl Pts',(42.4392116918951,-58.6698405167284,
-52.2019291666667));
#264463=CARTESIAN_POINT('Ctrl Pts',(43.4735820751078,-59.267034535918,-52.1435958333333));
#264464=CARTESIAN_POINT('Ctrl Pts',(44.5079524583205,-59.8642285551076,
-52.0852625));
#264465=CARTESIAN_POINT('Ctrl Pts',(45.5423228415332,-59.267034535918,-52.0269291666667));
#264466=CARTESIAN_POINT('Ctrl Pts',(46.5766932247459,-58.6698405167284,
-51.9685958333333));
#264467=CARTESIAN_POINT('Ctrl Pts',(46.5766932247459,-57.4754524783491,
-51.9102625));
#264468=CARTESIAN_POINT('Ctrl Pts',(46.5766932247459,-56.2810644399698,
-51.8519291666667));
#264469=CARTESIAN_POINT('Ctrl Pts',(45.5423228415332,-55.6838704207802,
-51.7935958333333));
#264470=CARTESIAN_POINT('Ctrl Pts',(44.5079524583205,-55.0866764015906,
-51.7352625));
#264471=CARTESIAN_POINT('Ctrl Pts',(43.4735820751078,-55.6838704207802,
-51.6769291666667));
#264472=CARTESIAN_POINT('Ctrl Pts',(42.4392116918951,-56.2810644399698,
-51.6185958333333));
#264473=CARTESIAN_POINT('Ctrl Pts',(42.439211691895,-57.4754524783491,-51.5602625));
#264474=CARTESIAN_POINT('Ctrl Pts',(42.4392116918951,-58.6698405167284,
-51.5019291666666));
#264475=CARTESIAN_POINT('Ctrl Pts',(43.4735820751078,-59.267034535918,-51.4435958333333));
#264476=CARTESIAN_POINT('Ctrl Pts',(44.5079524583205,-59.8642285551076,
-51.3852625));
#264477=CARTESIAN_POINT('Ctrl Pts',(45.5423228415332,-59.267034535918,-51.3269291666667));
#264478=CARTESIAN_POINT('Ctrl Pts',(46.5766932247459,-58.6698405167284,
-51.2685958333333));
#264479=CARTESIAN_POINT('Ctrl Pts',(46.5766932247459,-57.4754524783491,
-51.2102625));
#264480=CARTESIAN_POINT('Ctrl Pts',(46.5766932247459,-56.2810644399698,
-51.1519291666666));
#264481=CARTESIAN_POINT('Ctrl Pts',(45.5423228415332,-55.6838704207802,
-51.0935958333334));
#264482=CARTESIAN_POINT('Ctrl Pts',(44.5079524583205,-55.0866764015906,
-51.0352625));
#264483=CARTESIAN_POINT('Ctrl Pts',(43.4735820751078,-55.6838704207802,
-50.9769291666667));
#264484=CARTESIAN_POINT('Ctrl Pts',(42.4392116918951,-56.2810644399698,
-50.9185958333333));
#264485=CARTESIAN_POINT('Ctrl Pts',(42.439211691895,-57.4754524783491,-50.8602625));
#264486=CARTESIAN_POINT('Ctrl Pts',(42.4392116918951,-58.6698405167284,
-50.8019291666667));
#264487=CARTESIAN_POINT('Ctrl Pts',(43.4735820751078,-59.267034535918,-50.7435958333333));
#264488=CARTESIAN_POINT('Ctrl Pts',(44.5079524583205,-59.8642285551076,
-50.6852625));
#264489=CARTESIAN_POINT('Ctrl Pts',(45.5423228415332,-59.267034535918,-50.6269291666667));
#264490=CARTESIAN_POINT('Ctrl Pts',(46.5766932247459,-58.6698405167284,
-50.5685958333333));
#264491=CARTESIAN_POINT('Ctrl Pts',(46.5766932247459,-57.4754524783491,
-50.5102625));
#264492=CARTESIAN_POINT('Ctrl Pts',(46.5766932247459,-56.2810644399698,
-50.4519291666667));
#264493=CARTESIAN_POINT('Ctrl Pts',(45.5423228415332,-55.6838704207802,
-50.3935958333333));
#264494=CARTESIAN_POINT('Ctrl Pts',(44.5079524583205,-55.0866764015906,
-50.3352625));
#264495=CARTESIAN_POINT('Ctrl Pts',(43.4735820751078,-55.6838704207802,
-50.2769291666667));
#264496=CARTESIAN_POINT('Ctrl Pts',(42.4392116918951,-56.2810644399698,
-50.2185958333333));
#264497=CARTESIAN_POINT('Ctrl Pts',(42.439211691895,-57.4754524783491,-50.1602625));
#264498=CARTESIAN_POINT('Ctrl Pts',(42.4392116918951,-58.6698405167284,
-50.1019291666667));
#264499=CARTESIAN_POINT('Ctrl Pts',(43.4735820751078,-59.267034535918,-50.0435958333333));
#264500=CARTESIAN_POINT('Ctrl Pts',(44.5079524583205,-59.8642285551076,
-49.9852625));
#264501=CARTESIAN_POINT('Ctrl Pts',(45.5423228415332,-59.267034535918,-49.9269291666667));
#264502=CARTESIAN_POINT('Ctrl Pts',(46.5766932247459,-58.6698405167284,
-49.8685958333333));
#264503=CARTESIAN_POINT('Ctrl Pts',(46.5766932247459,-57.4754524783491,
-49.8102625));
#264504=CARTESIAN_POINT('Ctrl Pts',(46.5766932247459,-56.2810644399698,
-49.7519291666667));
#264505=CARTESIAN_POINT('Ctrl Pts',(45.5423228415332,-55.6838704207802,
-49.6935958333334));
#264506=CARTESIAN_POINT('Ctrl Pts',(44.5079524583205,-55.0866764015906,
-49.6352625));
#264507=CARTESIAN_POINT('Ctrl Pts',(43.4735820751078,-55.6838704207802,
-49.5769291666667));
#264508=CARTESIAN_POINT('Ctrl Pts',(42.4392116918951,-56.2810644399698,
-49.5185958333334));
#264509=CARTESIAN_POINT('Ctrl Pts',(42.439211691895,-57.4754524783491,-49.4602625));
#264510=CARTESIAN_POINT('Ctrl Pts',(42.4392116918951,-58.6698405167284,
-49.4019291666667));
#264511=CARTESIAN_POINT('Ctrl Pts',(43.4735820751078,-59.267034535918,-49.3435958333333));
#264512=CARTESIAN_POINT('Ctrl Pts',(44.5079524583205,-59.8642285551076,
-49.2852625));
#264513=CARTESIAN_POINT('Ctrl Pts',(45.5423228415332,-59.267034535918,-49.2269291666667));
#264514=CARTESIAN_POINT('Ctrl Pts',(46.5766932247459,-58.6698405167284,
-49.1685958333334));
#264515=CARTESIAN_POINT('Ctrl Pts',(46.5766932247459,-57.4754524783491,
-49.1102625));
#264516=CARTESIAN_POINT('Ctrl Pts',(46.5766932247459,-56.2810644399698,
-49.0519291666667));
#264517=CARTESIAN_POINT('Ctrl Pts',(45.5423228415332,-55.6838704207802,
-48.9935958333333));
#264518=CARTESIAN_POINT('Ctrl Pts',(44.5079524583205,-55.0866764015906,
-48.9352625));
#264519=CARTESIAN_POINT('Ctrl Pts',(43.4735820751078,-55.6838704207802,
-48.8769291666667));
#264520=CARTESIAN_POINT('Ctrl Pts',(42.4392116918951,-56.2810644399698,
-48.8185958333334));
#264521=CARTESIAN_POINT('Ctrl Pts',(42.439211691895,-57.4754524783491,-48.7602625));
#264522=CARTESIAN_POINT('Ctrl Pts',(42.4392116918951,-58.6698405167284,
-48.7019291666667));
#264523=CARTESIAN_POINT('Ctrl Pts',(43.4735820751078,-59.267034535918,-48.6435958333333));
#264524=CARTESIAN_POINT('Ctrl Pts',(44.5079524583205,-59.8642285551076,
-48.5852625));
#264525=CARTESIAN_POINT('Ctrl Pts',(45.5423228415332,-59.267034535918,-48.5269291666667));
#264526=CARTESIAN_POINT('Ctrl Pts',(46.5766932247459,-58.6698405167284,
-48.4685958333333));
#264527=CARTESIAN_POINT('Ctrl Pts',(46.5766932247459,-57.4754524783491,
-48.4102625));
#264528=CARTESIAN_POINT('Ctrl Pts',(46.5766932247459,-56.2810644399698,
-48.3519291666667));
#264529=CARTESIAN_POINT('Ctrl Pts',(45.5423228415332,-55.6838704207802,
-48.2935958333334));
#264530=CARTESIAN_POINT('Ctrl Pts',(44.5079524583205,-55.0866764015906,
-48.2352625));
#264531=CARTESIAN_POINT('Ctrl Pts',(43.4735820751078,-55.6838704207802,
-48.1769291666667));
#264532=CARTESIAN_POINT('Ctrl Pts',(42.4392116918951,-56.2810644399698,
-48.1185958333334));
#264533=CARTESIAN_POINT('Ctrl Pts',(42.439211691895,-57.4754524783491,-48.0602625));
#264534=CARTESIAN_POINT('Ctrl Pts',(42.4392116918951,-58.6698405167284,
-48.0019291666667));
#264535=CARTESIAN_POINT('Ctrl Pts',(43.4735820751078,-59.267034535918,-47.9435958333334));
#264536=CARTESIAN_POINT('Ctrl Pts',(44.5079524583205,-59.8642285551076,
-47.8852625));
#264537=CARTESIAN_POINT('Ctrl Pts',(45.5423228415332,-59.267034535918,-47.8269291666667));
#264538=CARTESIAN_POINT('Ctrl Pts',(46.5766932247459,-58.6698405167284,
-47.7685958333333));
#264539=CARTESIAN_POINT('Ctrl Pts',(46.5766932247459,-57.4754524783491,
-47.7102625));
#264540=CARTESIAN_POINT('Ctrl Pts',(46.5766932247459,-56.2810644399698,
-47.6519291666667));
#264541=CARTESIAN_POINT('Ctrl Pts',(45.5423228415332,-55.6838704207802,
-47.5935958333333));
#264542=CARTESIAN_POINT('Ctrl Pts',(44.5079524583205,-55.0866764015906,
-47.5352625));
#264543=CARTESIAN_POINT('Ctrl Pts',(43.4735820751078,-55.6838704207802,
-47.4769291666667));
#264544=CARTESIAN_POINT('Ctrl Pts',(42.4392116918951,-56.2810644399698,
-47.4185958333333));
#264545=CARTESIAN_POINT('Ctrl Pts',(42.439211691895,-57.4754524783491,-47.3602625));
#264546=CARTESIAN_POINT('Ctrl Pts',(42.4392116918951,-58.6698405167284,
-47.3019291666666));
#264547=CARTESIAN_POINT('Ctrl Pts',(43.4735820751078,-59.267034535918,-47.2435958333334));
#264548=CARTESIAN_POINT('Ctrl Pts',(44.5079524583205,-59.8642285551076,
-47.1852625));
#264549=CARTESIAN_POINT('Ctrl Pts',(45.5423228415332,-59.267034535918,-47.1269291666667));
#264550=CARTESIAN_POINT('Ctrl Pts',(46.5766932247459,-58.6698405167284,
-47.0685958333333));
#264551=CARTESIAN_POINT('Ctrl Pts',(46.5766932247459,-57.4754524783491,
-47.0102625));
#264552=CARTESIAN_POINT('Ctrl Pts',(46.5766932247459,-56.2810644399698,
-46.9519291666667));
#264553=CARTESIAN_POINT('Ctrl Pts',(45.5423228415332,-55.6838704207802,
-46.8935958333333));
#264554=CARTESIAN_POINT('Ctrl Pts',(44.5079524583205,-55.0866764015906,
-46.8352625));
#264555=CARTESIAN_POINT('Ctrl Pts',(43.4735820751078,-55.6838704207802,
-46.7769291666667));
#264556=CARTESIAN_POINT('Ctrl Pts',(42.4392116918951,-56.2810644399698,
-46.7185958333333));
#264557=CARTESIAN_POINT('Ctrl Pts',(42.439211691895,-57.4754524783491,-46.6602625));
#264558=CARTESIAN_POINT('Ctrl Pts',(42.4392116918951,-58.6698405167284,
-46.6019291666667));
#264559=CARTESIAN_POINT('Ctrl Pts',(43.4735820751078,-59.267034535918,-46.5435958333334));
#264560=CARTESIAN_POINT('Ctrl Pts',(44.5079524583205,-59.8642285551076,
-46.4852625));
#264561=CARTESIAN_POINT('Ctrl Pts',(45.5423228415332,-59.267034535918,-46.4269291666667));
#264562=CARTESIAN_POINT('Ctrl Pts',(46.5766932247459,-58.6698405167284,
-46.3685958333333));
#264563=CARTESIAN_POINT('Ctrl Pts',(46.5766932247459,-57.4754524783491,
-46.3102625));
#264564=CARTESIAN_POINT('Ctrl Pts',(46.5766932247459,-56.2810644399698,
-46.2519291666667));
#264565=CARTESIAN_POINT('Ctrl Pts',(45.5423228415332,-55.6838704207802,
-46.1935958333333));
#264566=CARTESIAN_POINT('Ctrl Pts',(44.5079524583205,-55.0866764015906,
-46.1352625));
#264567=CARTESIAN_POINT('Ctrl Pts',(43.4735820751078,-55.6838704207802,
-46.0769291666667));
#264568=CARTESIAN_POINT('Ctrl Pts',(42.4392116918951,-56.2810644399698,
-46.0185958333334));
#264569=CARTESIAN_POINT('Ctrl Pts',(42.439211691895,-57.4754524783491,-45.9602625));
#264570=CARTESIAN_POINT('Ctrl Pts',(42.4392116918951,-58.6698405167284,
-45.9019291666667));
#264571=CARTESIAN_POINT('Ctrl Pts',(43.4735820751078,-59.267034535918,-45.8435958333333));
#264572=CARTESIAN_POINT('Ctrl Pts',(44.5079524583205,-59.8642285551076,
-45.7852625));
#264573=CARTESIAN_POINT('Ctrl Pts',(45.5423228415332,-59.267034535918,-45.7269291666667));
#264574=CARTESIAN_POINT('Ctrl Pts',(46.5766932247459,-58.6698405167284,
-45.6685958333334));
#264575=CARTESIAN_POINT('Ctrl Pts',(46.5766932247459,-57.4754524783491,
-45.6102625));
#264576=CARTESIAN_POINT('Ctrl Pts',(46.5766932247459,-56.2810644399698,
-45.5519291666667));
#264577=CARTESIAN_POINT('Ctrl Pts',(45.5423228415332,-55.6838704207802,
-45.4935958333333));
#264578=CARTESIAN_POINT('Ctrl Pts',(44.5079524583205,-55.0866764015906,
-45.4352625));
#264579=CARTESIAN_POINT('Ctrl Pts',(43.4735820751078,-55.6838704207802,
-45.3769291666667));
#264580=CARTESIAN_POINT('Ctrl Pts',(42.4392116918951,-56.2810644399698,
-45.3185958333333));
#264581=CARTESIAN_POINT('Ctrl Pts',(42.439211691895,-57.4754524783491,-45.2602625));
#264582=CARTESIAN_POINT('Ctrl Pts',(42.4392116918951,-58.6698405167284,
-45.2019291666667));
#264583=CARTESIAN_POINT('Ctrl Pts',(43.4735820751078,-59.267034535918,-45.1435958333334));
#264584=CARTESIAN_POINT('Ctrl Pts',(44.5079524583205,-59.8642285551076,
-45.0852625));
#264585=CARTESIAN_POINT('Ctrl Pts',(45.5423228415332,-59.267034535918,-45.0269291666667));
#264586=CARTESIAN_POINT('Ctrl Pts',(46.5766932247459,-58.6698405167284,
-44.9685958333334));
#264587=CARTESIAN_POINT('Ctrl Pts',(46.5766932247459,-57.4754524783491,
-44.9102625));
#264588=CARTESIAN_POINT('Ctrl Pts',(46.5766932247459,-56.2810644399698,
-44.8519291666667));
#264589=CARTESIAN_POINT('Ctrl Pts',(45.5423228415332,-55.6838704207802,
-44.7935958333333));
#264590=CARTESIAN_POINT('Ctrl Pts',(44.5079524583205,-55.0866764015906,
-44.7352625));
#264591=CARTESIAN_POINT('Ctrl Pts',(43.4735820751078,-55.6838704207802,
-44.6769291666667));
#264592=CARTESIAN_POINT('Ctrl Pts',(42.4392116918951,-56.2810644399698,
-44.6185958333334));
#264593=CARTESIAN_POINT('Ctrl Pts',(42.439211691895,-57.4754524783491,-44.5602625));
#264594=CARTESIAN_POINT('Ctrl Pts',(42.4392116918951,-58.6698405167284,
-44.5019291666667));
#264595=CARTESIAN_POINT('Ctrl Pts',(43.4735820751078,-59.267034535918,-44.4435958333333));
#264596=CARTESIAN_POINT('Ctrl Pts',(44.5079524583205,-59.8642285551076,
-44.3852625));
#264597=CARTESIAN_POINT('Ctrl Pts',(45.5423228415332,-59.267034535918,-44.3269291666667));
#264598=CARTESIAN_POINT('Ctrl Pts',(46.5766932247459,-58.6698405167284,
-44.2685958333334));
#264599=CARTESIAN_POINT('Ctrl Pts',(46.5766932247459,-57.4754524783491,
-44.2102625));
#264600=CARTESIAN_POINT('Ctrl Pts',(46.5766932247459,-56.2810644399698,
-44.1519291666667));
#264601=CARTESIAN_POINT('Ctrl Pts',(45.5423228415332,-55.6838704207802,
-44.0935958333334));
#264602=CARTESIAN_POINT('Ctrl Pts',(44.5079524583205,-55.0866764015906,
-44.0352625));
#264603=CARTESIAN_POINT('Ctrl Pts',(43.4735820751078,-55.6838704207802,
-43.9769291666667));
#264604=CARTESIAN_POINT('Ctrl Pts',(42.4392116918951,-56.2810644399698,
-43.9185958333334));
#264605=CARTESIAN_POINT('Ctrl Pts',(42.439211691895,-57.4754524783491,-43.8602625));
#264606=CARTESIAN_POINT('Ctrl Pts',(42.4392116918951,-58.6698405167284,
-43.8019291666667));
#264607=CARTESIAN_POINT('Ctrl Pts',(43.4735820751078,-59.267034535918,-43.7435958333334));
#264608=CARTESIAN_POINT('Ctrl Pts',(44.5079524583205,-59.8642285551076,
-43.6852625));
#264609=CARTESIAN_POINT('Ctrl Pts',(45.5423228415332,-59.267034535918,-43.6269291666667));
#264610=CARTESIAN_POINT('Ctrl Pts',(46.5766932247459,-58.6698405167284,
-43.5685958333334));
#264611=CARTESIAN_POINT('Ctrl Pts',(46.5766932247459,-57.4754524783491,
-43.5102625));
#264612=CARTESIAN_POINT('Ctrl Pts',(46.5766932247459,-56.2810644399698,
-43.4519291666667));
#264613=CARTESIAN_POINT('Ctrl Pts',(45.5423228415332,-55.6838704207802,
-43.3935958333334));
#264614=CARTESIAN_POINT('Ctrl Pts',(44.5079524583205,-55.0866764015906,
-43.3352625));
#264615=CARTESIAN_POINT('Ctrl Pts',(43.4735820751078,-55.6838704207802,
-43.2769291666667));
#264616=CARTESIAN_POINT('Ctrl Pts',(42.4392116918951,-56.2810644399698,
-43.2185958333334));
#264617=CARTESIAN_POINT('Ctrl Pts',(42.439211691895,-57.4754524783491,-43.1602625));
#264618=CARTESIAN_POINT('Ctrl Pts',(42.4392116918951,-58.6698405167284,
-43.1019291666667));
#264619=CARTESIAN_POINT('Ctrl Pts',(43.4735820751078,-59.267034535918,-43.0435958333334));
#264620=CARTESIAN_POINT('Ctrl Pts',(44.5079524583205,-59.8642285551076,
-42.9852625));
#264621=CARTESIAN_POINT('Ctrl Pts',(45.5423228415332,-59.267034535918,-42.9269291666667));
#264622=CARTESIAN_POINT('Ctrl Pts',(46.5766932247459,-58.6698405167284,
-42.8685958333333));
#264623=CARTESIAN_POINT('Ctrl Pts',(46.5766932247459,-57.4754524783491,
-42.8102625));
#264624=CARTESIAN_POINT('Ctrl Pts',(46.5766932247459,-56.2810644399698,
-42.7519291666667));
#264625=CARTESIAN_POINT('Ctrl Pts',(45.5423228415332,-55.6838704207802,
-42.6935958333333));
#264626=CARTESIAN_POINT('Ctrl Pts',(44.5079524583205,-55.0866764015906,
-42.6352625));
#264627=CARTESIAN_POINT('Ctrl Pts',(43.4735820751078,-55.6838704207802,
-42.5769291666667));
#264628=CARTESIAN_POINT('Ctrl Pts',(42.4392116918951,-56.2810644399698,
-42.5185958333333));
#264629=CARTESIAN_POINT('Ctrl Pts',(42.439211691895,-57.4754524783491,-42.4602625));
#264630=CARTESIAN_POINT('Ctrl Pts',(42.4392116918951,-58.6698405167284,
-42.4019291666666));
#264631=CARTESIAN_POINT('Ctrl Pts',(43.4735820751078,-59.267034535918,-42.3435958333334));
#264632=CARTESIAN_POINT('Ctrl Pts',(44.5079524583205,-59.8642285551076,
-42.2852625));
#264633=CARTESIAN_POINT('Ctrl Pts',(45.5423228415332,-59.267034535918,-42.2269291666667));
#264634=CARTESIAN_POINT('Ctrl Pts',(46.5766932247459,-58.6698405167284,
-42.1685958333333));
#264635=CARTESIAN_POINT('Ctrl Pts',(46.5766932247459,-57.4754524783491,
-42.1102625));
#264636=CARTESIAN_POINT('Ctrl Pts',(46.5766932247459,-56.2810644399698,
-42.0519291666667));
#264637=CARTESIAN_POINT('Ctrl Pts',(45.5423228415332,-55.6838704207802,
-41.9935958333334));
#264638=CARTESIAN_POINT('Ctrl Pts',(44.5079524583205,-55.0866764015906,
-41.9352625));
#264639=CARTESIAN_POINT('Ctrl Pts',(43.4735820751078,-55.6838704207802,
-41.8769291666667));
#264640=CARTESIAN_POINT('Ctrl Pts',(42.4392116918951,-56.2810644399698,
-41.8185958333333));
#264641=CARTESIAN_POINT('Ctrl Pts',(42.439211691895,-57.4754524783491,-41.7602625));
#264642=CARTESIAN_POINT('Ctrl Pts',(42.4392116918951,-58.6698405167284,
-41.7019291666667));
#264643=CARTESIAN_POINT('Ctrl Pts',(43.4735820751078,-59.267034535918,-41.6435958333334));
#264644=CARTESIAN_POINT('Ctrl Pts',(44.5079524583205,-59.8642285551076,
-41.5852625));
#264645=CARTESIAN_POINT('Ctrl Pts',(45.5423228415332,-59.267034535918,-41.5269291666667));
#264646=CARTESIAN_POINT('Ctrl Pts',(46.5766932247459,-58.6698405167284,
-41.4685958333333));
#264647=CARTESIAN_POINT('Ctrl Pts',(46.5766932247459,-57.4754524783491,
-41.4102625));
#264648=CARTESIAN_POINT('Ctrl Pts',(46.5766932247459,-56.2810644399698,
-41.3519291666666));
#264649=CARTESIAN_POINT('Ctrl Pts',(45.5423228415332,-55.6838704207802,
-41.2935958333334));
#264650=CARTESIAN_POINT('Ctrl Pts',(44.5079524583205,-55.0866764015906,
-41.2352625));
#264651=CARTESIAN_POINT('Ctrl Pts',(43.4735820751078,-55.6838704207802,
-41.1769291666667));
#264652=CARTESIAN_POINT('Ctrl Pts',(42.4392116918951,-56.2810644399698,
-41.1185958333333));
#264653=CARTESIAN_POINT('Ctrl Pts',(42.439211691895,-57.4754524783491,-41.0602625));
#264654=CARTESIAN_POINT('Ctrl Pts',(42.4392116918951,-58.6698405167284,
-41.0019291666666));
#264655=CARTESIAN_POINT('Ctrl Pts',(43.4735820751078,-59.267034535918,-40.9435958333334));
#264656=CARTESIAN_POINT('Ctrl Pts',(44.5079524583205,-59.8642285551076,
-40.8852625));
#264657=CARTESIAN_POINT('Ctrl Pts',(45.5423228415332,-59.267034535918,-40.8269291666667));
#264658=CARTESIAN_POINT('Ctrl Pts',(46.5766932247459,-58.6698405167284,
-40.7685958333333));
#264659=CARTESIAN_POINT('Ctrl Pts',(46.5766932247459,-57.4754524783491,
-40.7102625));
#264660=CARTESIAN_POINT('Ctrl Pts',(46.5766932247459,-56.2810644399698,
-40.6519291666667));
#264661=CARTESIAN_POINT('Ctrl Pts',(45.5423228415332,-55.6838704207802,
-40.5935958333334));
#264662=CARTESIAN_POINT('Ctrl Pts',(44.5079524583205,-55.0866764015906,
-40.5352625));
#264663=CARTESIAN_POINT('Ctrl Pts',(43.4735820751078,-55.6838704207802,
-40.4769291666667));
#264664=CARTESIAN_POINT('Ctrl Pts',(42.4392116918951,-56.2810644399698,
-40.4185958333333));
#264665=CARTESIAN_POINT('Ctrl Pts',(42.439211691895,-57.4754524783491,-40.3602625));
#264666=CARTESIAN_POINT('Ctrl Pts',(42.4392116918951,-58.6698405167284,
-40.3019291666667));
#264667=CARTESIAN_POINT('Ctrl Pts',(43.4735820751078,-59.267034535918,-40.2435958333334));
#264668=CARTESIAN_POINT('Ctrl Pts',(44.5079524583205,-59.8642285551076,
-40.1852625));
#264669=CARTESIAN_POINT('Ctrl Pts',(45.5423228415332,-59.267034535918,-40.1269291666666));
#264670=CARTESIAN_POINT('Ctrl Pts',(46.5766932247459,-58.6698405167284,
-40.0685958333333));
#264671=CARTESIAN_POINT('Ctrl Pts',(46.5766932247459,-57.4754524783491,
-40.0102625));
#264672=CARTESIAN_POINT('Ctrl Pts',(46.5766932247459,-56.2810644399698,
-39.9519291666667));
#264673=CARTESIAN_POINT('Ctrl Pts',(45.5423228415332,-55.6838704207802,
-39.8935958333334));
#264674=CARTESIAN_POINT('Ctrl Pts',(44.5079524583205,-55.0866764015906,
-39.8352625));
#264675=CARTESIAN_POINT('Ctrl Pts',(43.4735820751078,-55.6838704207802,
-39.7769291666667));
#264676=CARTESIAN_POINT('Ctrl Pts',(42.4392116918951,-56.2810644399698,
-39.7185958333334));
#264677=CARTESIAN_POINT('Ctrl Pts',(42.439211691895,-57.4754524783491,-39.6602625));
#264678=CARTESIAN_POINT('Ctrl Pts',(42.4392116918951,-58.6698405167284,
-39.6019291666667));
#264679=CARTESIAN_POINT('Ctrl Pts',(43.4735820751078,-59.267034535918,-39.5435958333333));
#264680=CARTESIAN_POINT('Ctrl Pts',(44.5079524583205,-59.8642285551076,
-39.4852625));
#264681=CARTESIAN_POINT('Ctrl Pts',(45.5423228415332,-59.267034535918,-39.4269291666667));
#264682=CARTESIAN_POINT('Ctrl Pts',(46.5766932247459,-58.6698405167284,
-39.3685958333334));
#264683=CARTESIAN_POINT('Ctrl Pts',(46.5766932247459,-57.4754524783491,
-39.3102625));
#264684=CARTESIAN_POINT('Ctrl Pts',(46.5766932247459,-56.2810644399698,
-39.2519291666667));
#264685=CARTESIAN_POINT('Ctrl Pts',(45.5423228415332,-55.6838704207802,
-39.1935958333334));
#264686=CARTESIAN_POINT('Ctrl Pts',(44.5079524583205,-55.0866764015906,
-39.1352625));
#264687=CARTESIAN_POINT('Ctrl Pts',(43.4735820751078,-55.6838704207802,
-39.0769291666667));
#264688=CARTESIAN_POINT('Ctrl Pts',(42.4392116918951,-56.2810644399698,
-39.0185958333334));
#264689=CARTESIAN_POINT('Ctrl Pts',(42.439211691895,-57.4754524783491,-38.9602625));
#264690=CARTESIAN_POINT('Ctrl Pts',(42.4392116918951,-58.6698405167284,
-38.9019291666667));
#264691=CARTESIAN_POINT('Ctrl Pts',(43.4735820751078,-59.267034535918,-38.8435958333333));
#264692=CARTESIAN_POINT('Ctrl Pts',(44.5079524583205,-59.8642285551076,
-38.7852625));
#264693=CARTESIAN_POINT('Ctrl Pts',(45.5423228415332,-59.267034535918,-38.7269291666667));
#264694=CARTESIAN_POINT('Ctrl Pts',(46.5766932247459,-58.6698405167284,
-38.6685958333334));
#264695=CARTESIAN_POINT('Ctrl Pts',(46.5766932247459,-57.4754524783491,
-38.6102625));
#264696=CARTESIAN_POINT('Ctrl Pts',(46.5766932247459,-56.2810644399698,
-38.5519291666667));
#264697=CARTESIAN_POINT('Ctrl Pts',(45.5423228415332,-55.6838704207802,
-38.4935958333334));
#264698=CARTESIAN_POINT('Ctrl Pts',(44.5079524583205,-55.0866764015906,
-38.4352625));
#264699=CARTESIAN_POINT('Ctrl Pts',(43.4735820751078,-55.6838704207802,
-38.3769291666667));
#264700=CARTESIAN_POINT('Ctrl Pts',(42.4392116918951,-56.2810644399698,
-38.3185958333333));
#264701=CARTESIAN_POINT('Ctrl Pts',(42.439211691895,-57.4754524783491,-38.2602625));
#264702=CARTESIAN_POINT('Ctrl Pts',(42.4392116918951,-58.6698405167284,
-38.2019291666667));
#264703=CARTESIAN_POINT('Ctrl Pts',(43.4735820751078,-59.267034535918,-38.1435958333334));
#264704=CARTESIAN_POINT('Ctrl Pts',(44.5079524583205,-59.8642285551076,
-38.0852625));
#264705=CARTESIAN_POINT('Ctrl Pts',(45.5423228415332,-59.267034535918,-38.0269291666667));
#264706=CARTESIAN_POINT('Ctrl Pts',(46.5766932247459,-58.6698405167284,
-37.9685958333333));
#264707=CARTESIAN_POINT('Ctrl Pts',(46.5766932247459,-57.4754524783491,
-37.9102625));
#264708=CARTESIAN_POINT('Ctrl Pts',(46.5766932247459,-56.2810644399698,
-37.8519291666667));
#264709=CARTESIAN_POINT('Ctrl Pts',(45.5423228415332,-55.6838704207802,
-37.7935958333334));
#264710=CARTESIAN_POINT('Ctrl Pts',(44.5079524583205,-55.0866764015906,
-37.7352625));
#264711=CARTESIAN_POINT('Ctrl Pts',(43.4735820751078,-55.6838704207802,
-37.6769291666667));
#264712=CARTESIAN_POINT('Ctrl Pts',(42.4392116918951,-56.2810644399698,
-37.6185958333333));
#264713=CARTESIAN_POINT('Ctrl Pts',(42.439211691895,-57.4754524783491,-37.5602625));
#264714=CARTESIAN_POINT('Ctrl Pts',(42.4392116918951,-58.6698405167284,
-37.5019291666667));
#264715=CARTESIAN_POINT('Ctrl Pts',(43.4735820751078,-59.267034535918,-37.4435958333333));
#264716=CARTESIAN_POINT('Ctrl Pts',(44.5079524583205,-59.8642285551076,
-37.3852625));
#264717=CARTESIAN_POINT('Ctrl Pts',(45.5423228415332,-59.267034535918,-37.3269291666667));
#264718=CARTESIAN_POINT('Ctrl Pts',(46.5766932247459,-58.6698405167284,
-37.2685958333333));
#264719=CARTESIAN_POINT('Ctrl Pts',(46.5766932247459,-57.4754524783491,
-37.2102625));
#264720=CARTESIAN_POINT('Ctrl Pts',(46.5766932247459,-56.2810644399698,
-37.1519291666667));
#264721=CARTESIAN_POINT('Ctrl Pts',(45.5423228415332,-55.6838704207802,
-37.0935958333333));
#264722=CARTESIAN_POINT('Ctrl Pts',(44.5079524583205,-55.0866764015906,
-37.0352625));
#264723=CARTESIAN_POINT('Ctrl Pts',(43.4735820751078,-55.6838704207802,
-36.9769291666667));
#264724=CARTESIAN_POINT('Ctrl Pts',(42.4392116918951,-56.2810644399698,
-36.9185958333333));
#264725=CARTESIAN_POINT('Ctrl Pts',(42.439211691895,-57.4754524783491,-36.8602625));
#264726=CARTESIAN_POINT('Ctrl Pts',(42.4392116918951,-58.6698405167284,
-36.8019291666666));
#264727=CARTESIAN_POINT('Ctrl Pts',(43.4735820751078,-59.267034535918,-36.7435958333334));
#264728=CARTESIAN_POINT('Ctrl Pts',(44.5079524583205,-59.8642285551076,
-36.6852625));
#264729=CARTESIAN_POINT('Ctrl Pts',(45.5423228415332,-59.267034535918,-36.6269291666667));
#264730=CARTESIAN_POINT('Ctrl Pts',(45.6766051604217,-59.1895066029603,
-36.6193563132714));
#264731=CARTESIAN_POINT('Ctrl Pts',(45.7978303778615,-59.0928279175564,
-36.611216324118));
#264732=CARTESIAN_POINT('Ctrl Pts',(46.1766977413729,-57.4754524783491,
-52.8412));
#264733=CARTESIAN_POINT('Ctrl Pts',(46.1766977413729,-56.5120019399699,
-52.7828666666667));
#264734=CARTESIAN_POINT('Ctrl Pts',(45.3423250998467,-56.0302766707802,
-52.7245333333334));
#264735=CARTESIAN_POINT('Ctrl Pts',(44.5079524583205,-55.5485514015906,
-52.6662));
#264736=CARTESIAN_POINT('Ctrl Pts',(43.6735798167943,-56.0302766707802,
-52.6078666666667));
#264737=CARTESIAN_POINT('Ctrl Pts',(42.839207175268,-56.5120019399698,-52.5495333333333));
#264738=CARTESIAN_POINT('Ctrl Pts',(42.839207175268,-57.4754524783491,-52.4912));
#264739=CARTESIAN_POINT('Ctrl Pts',(42.839207175268,-58.4389030167283,-52.4328666666667));
#264740=CARTESIAN_POINT('Ctrl Pts',(43.6735798167943,-58.920628285918,-52.3745333333334));
#264741=CARTESIAN_POINT('Ctrl Pts',(44.5079524583205,-59.4023535551075,
-52.3162000000001));
#264742=CARTESIAN_POINT('Ctrl Pts',(45.3423250998467,-58.920628285918,-52.2578666666667));
#264743=CARTESIAN_POINT('Ctrl Pts',(46.1766977413729,-58.4389030167283,
-52.1995333333334));
#264744=CARTESIAN_POINT('Ctrl Pts',(46.1766977413729,-57.4754524783491,
-52.1412));
#264745=CARTESIAN_POINT('Ctrl Pts',(46.1766977413729,-56.5120019399699,
-52.0828666666667));
#264746=CARTESIAN_POINT('Ctrl Pts',(45.3423250998467,-56.0302766707802,
-52.0245333333333));
#264747=CARTESIAN_POINT('Ctrl Pts',(44.5079524583205,-55.5485514015906,
-51.9662));
#264748=CARTESIAN_POINT('Ctrl Pts',(43.6735798167943,-56.0302766707802,
-51.9078666666667));
#264749=CARTESIAN_POINT('Ctrl Pts',(42.839207175268,-56.5120019399698,-51.8495333333334));
#264750=CARTESIAN_POINT('Ctrl Pts',(42.839207175268,-57.4754524783491,-51.7912));
#264751=CARTESIAN_POINT('Ctrl Pts',(42.839207175268,-58.4389030167283,-51.7328666666667));
#264752=CARTESIAN_POINT('Ctrl Pts',(43.6735798167943,-58.920628285918,-51.6745333333334));
#264753=CARTESIAN_POINT('Ctrl Pts',(44.5079524583205,-59.4023535551075,
-51.6162));
#264754=CARTESIAN_POINT('Ctrl Pts',(45.3423250998467,-58.920628285918,-51.5578666666667));
#264755=CARTESIAN_POINT('Ctrl Pts',(46.1766977413729,-58.4389030167283,
-51.4995333333334));
#264756=CARTESIAN_POINT('Ctrl Pts',(46.1766977413729,-57.4754524783491,
-51.4412));
#264757=CARTESIAN_POINT('Ctrl Pts',(46.1766977413729,-56.5120019399699,
-51.3828666666667));
#264758=CARTESIAN_POINT('Ctrl Pts',(45.3423250998467,-56.0302766707802,
-51.3245333333334));
#264759=CARTESIAN_POINT('Ctrl Pts',(44.5079524583205,-55.5485514015906,
-51.2662));
#264760=CARTESIAN_POINT('Ctrl Pts',(43.6735798167943,-56.0302766707802,
-51.2078666666667));
#264761=CARTESIAN_POINT('Ctrl Pts',(42.839207175268,-56.5120019399698,-51.1495333333334));
#264762=CARTESIAN_POINT('Ctrl Pts',(42.839207175268,-57.4754524783491,-51.0912));
#264763=CARTESIAN_POINT('Ctrl Pts',(42.839207175268,-58.4389030167283,-51.0328666666667));
#264764=CARTESIAN_POINT('Ctrl Pts',(43.6735798167943,-58.920628285918,-50.9745333333333));
#264765=CARTESIAN_POINT('Ctrl Pts',(44.5079524583205,-59.4023535551075,
-50.9162));
#264766=CARTESIAN_POINT('Ctrl Pts',(45.3423250998467,-58.920628285918,-50.8578666666667));
#264767=CARTESIAN_POINT('Ctrl Pts',(46.1766977413729,-58.4389030167283,
-50.7995333333334));
#264768=CARTESIAN_POINT('Ctrl Pts',(46.1766977413729,-57.4754524783491,
-50.7412));
#264769=CARTESIAN_POINT('Ctrl Pts',(46.1766977413729,-56.5120019399699,
-50.6828666666667));
#264770=CARTESIAN_POINT('Ctrl Pts',(45.3423250998467,-56.0302766707802,
-50.6245333333333));
#264771=CARTESIAN_POINT('Ctrl Pts',(44.5079524583205,-55.5485514015906,
-50.5662));
#264772=CARTESIAN_POINT('Ctrl Pts',(43.6735798167943,-56.0302766707802,
-50.5078666666667));
#264773=CARTESIAN_POINT('Ctrl Pts',(42.839207175268,-56.5120019399698,-50.4495333333333));
#264774=CARTESIAN_POINT('Ctrl Pts',(42.839207175268,-57.4754524783491,-50.3912));
#264775=CARTESIAN_POINT('Ctrl Pts',(42.839207175268,-58.4389030167283,-50.3328666666667));
#264776=CARTESIAN_POINT('Ctrl Pts',(43.6735798167943,-58.920628285918,-50.2745333333334));
#264777=CARTESIAN_POINT('Ctrl Pts',(44.5079524583205,-59.4023535551075,
-50.2162));
#264778=CARTESIAN_POINT('Ctrl Pts',(45.3423250998467,-58.920628285918,-50.1578666666667));
#264779=CARTESIAN_POINT('Ctrl Pts',(46.1766977413729,-58.4389030167283,
-50.0995333333333));
#264780=CARTESIAN_POINT('Ctrl Pts',(46.1766977413729,-57.4754524783491,
-50.0412));
#264781=CARTESIAN_POINT('Ctrl Pts',(46.1766977413729,-56.5120019399699,
-49.9828666666667));
#264782=CARTESIAN_POINT('Ctrl Pts',(45.3423250998467,-56.0302766707802,
-49.9245333333334));
#264783=CARTESIAN_POINT('Ctrl Pts',(44.5079524583205,-55.5485514015906,
-49.8662));
#264784=CARTESIAN_POINT('Ctrl Pts',(43.6735798167943,-56.0302766707802,
-49.8078666666667));
#264785=CARTESIAN_POINT('Ctrl Pts',(42.839207175268,-56.5120019399698,-49.7495333333333));
#264786=CARTESIAN_POINT('Ctrl Pts',(42.839207175268,-57.4754524783491,-49.6912));
#264787=CARTESIAN_POINT('Ctrl Pts',(42.839207175268,-58.4389030167283,-49.6328666666667));
#264788=CARTESIAN_POINT('Ctrl Pts',(43.6735798167943,-58.920628285918,-49.5745333333334));
#264789=CARTESIAN_POINT('Ctrl Pts',(44.5079524583205,-59.4023535551075,
-49.5162));
#264790=CARTESIAN_POINT('Ctrl Pts',(45.3423250998467,-58.920628285918,-49.4578666666667));
#264791=CARTESIAN_POINT('Ctrl Pts',(46.1766977413729,-58.4389030167283,
-49.3995333333333));
#264792=CARTESIAN_POINT('Ctrl Pts',(46.1766977413729,-57.4754524783491,
-49.3412));
#264793=CARTESIAN_POINT('Ctrl Pts',(46.1766977413729,-56.5120019399699,
-49.2828666666666));
#264794=CARTESIAN_POINT('Ctrl Pts',(45.3423250998467,-56.0302766707802,
-49.2245333333334));
#264795=CARTESIAN_POINT('Ctrl Pts',(44.5079524583205,-55.5485514015906,
-49.1662));
#264796=CARTESIAN_POINT('Ctrl Pts',(43.6735798167943,-56.0302766707802,
-49.1078666666667));
#264797=CARTESIAN_POINT('Ctrl Pts',(42.839207175268,-56.5120019399698,-49.0495333333334));
#264798=CARTESIAN_POINT('Ctrl Pts',(42.839207175268,-57.4754524783491,-48.9912));
#264799=CARTESIAN_POINT('Ctrl Pts',(42.839207175268,-58.4389030167283,-48.9328666666667));
#264800=CARTESIAN_POINT('Ctrl Pts',(43.6735798167943,-58.920628285918,-48.8745333333334));
#264801=CARTESIAN_POINT('Ctrl Pts',(44.5079524583205,-59.4023535551075,
-48.8162));
#264802=CARTESIAN_POINT('Ctrl Pts',(45.3423250998467,-58.920628285918,-48.7578666666667));
#264803=CARTESIAN_POINT('Ctrl Pts',(46.1766977413729,-58.4389030167283,
-48.6995333333334));
#264804=CARTESIAN_POINT('Ctrl Pts',(46.1766977413729,-57.4754524783491,
-48.6412));
#264805=CARTESIAN_POINT('Ctrl Pts',(46.1766977413729,-56.5120019399699,
-48.5828666666667));
#264806=CARTESIAN_POINT('Ctrl Pts',(45.3423250998467,-56.0302766707802,
-48.5245333333334));
#264807=CARTESIAN_POINT('Ctrl Pts',(44.5079524583205,-55.5485514015906,
-48.4662));
#264808=CARTESIAN_POINT('Ctrl Pts',(43.6735798167943,-56.0302766707802,
-48.4078666666667));
#264809=CARTESIAN_POINT('Ctrl Pts',(42.839207175268,-56.5120019399698,-48.3495333333333));
#264810=CARTESIAN_POINT('Ctrl Pts',(42.839207175268,-57.4754524783491,-48.2912));
#264811=CARTESIAN_POINT('Ctrl Pts',(42.839207175268,-58.4389030167283,-48.2328666666667));
#264812=CARTESIAN_POINT('Ctrl Pts',(43.6735798167943,-58.920628285918,-48.1745333333334));
#264813=CARTESIAN_POINT('Ctrl Pts',(44.5079524583205,-59.4023535551075,
-48.1162));
#264814=CARTESIAN_POINT('Ctrl Pts',(45.3423250998467,-58.920628285918,-48.0578666666667));
#264815=CARTESIAN_POINT('Ctrl Pts',(46.1766977413729,-58.4389030167283,
-47.9995333333334));
#264816=CARTESIAN_POINT('Ctrl Pts',(46.1766977413729,-57.4754524783491,
-47.9412));
#264817=CARTESIAN_POINT('Ctrl Pts',(46.1766977413729,-56.5120019399699,
-47.8828666666667));
#264818=CARTESIAN_POINT('Ctrl Pts',(45.3423250998467,-56.0302766707802,
-47.8245333333333));
#264819=CARTESIAN_POINT('Ctrl Pts',(44.5079524583205,-55.5485514015906,
-47.7662));
#264820=CARTESIAN_POINT('Ctrl Pts',(43.6735798167943,-56.0302766707802,
-47.7078666666667));
#264821=CARTESIAN_POINT('Ctrl Pts',(42.839207175268,-56.5120019399698,-47.6495333333334));
#264822=CARTESIAN_POINT('Ctrl Pts',(42.839207175268,-57.4754524783491,-47.5912));
#264823=CARTESIAN_POINT('Ctrl Pts',(42.839207175268,-58.4389030167283,-47.5328666666667));
#264824=CARTESIAN_POINT('Ctrl Pts',(43.6735798167943,-58.920628285918,-47.4745333333334));
#264825=CARTESIAN_POINT('Ctrl Pts',(44.5079524583205,-59.4023535551075,
-47.4162));
#264826=CARTESIAN_POINT('Ctrl Pts',(45.3423250998467,-58.920628285918,-47.3578666666667));
#264827=CARTESIAN_POINT('Ctrl Pts',(46.1766977413729,-58.4389030167283,
-47.2995333333334));
#264828=CARTESIAN_POINT('Ctrl Pts',(46.1766977413729,-57.4754524783491,
-47.2412));
#264829=CARTESIAN_POINT('Ctrl Pts',(46.1766977413729,-56.5120019399699,
-47.1828666666667));
#264830=CARTESIAN_POINT('Ctrl Pts',(45.3423250998467,-56.0302766707802,
-47.1245333333333));
#264831=CARTESIAN_POINT('Ctrl Pts',(44.5079524583205,-55.5485514015906,
-47.0662));
#264832=CARTESIAN_POINT('Ctrl Pts',(43.6735798167943,-56.0302766707802,
-47.0078666666667));
#264833=CARTESIAN_POINT('Ctrl Pts',(42.839207175268,-56.5120019399698,-46.9495333333334));
#264834=CARTESIAN_POINT('Ctrl Pts',(42.839207175268,-57.4754524783491,-46.8912));
#264835=CARTESIAN_POINT('Ctrl Pts',(42.839207175268,-58.4389030167283,-46.8328666666667));
#264836=CARTESIAN_POINT('Ctrl Pts',(43.6735798167943,-58.920628285918,-46.7745333333334));
#264837=CARTESIAN_POINT('Ctrl Pts',(44.5079524583205,-59.4023535551075,
-46.7162));
#264838=CARTESIAN_POINT('Ctrl Pts',(45.3423250998467,-58.920628285918,-46.6578666666667));
#264839=CARTESIAN_POINT('Ctrl Pts',(46.1766977413729,-58.4389030167283,
-46.5995333333334));
#264840=CARTESIAN_POINT('Ctrl Pts',(46.1766977413729,-57.4754524783491,
-46.5412));
#264841=CARTESIAN_POINT('Ctrl Pts',(46.1766977413729,-56.5120019399699,
-46.4828666666667));
#264842=CARTESIAN_POINT('Ctrl Pts',(45.3423250998467,-56.0302766707802,
-46.4245333333334));
#264843=CARTESIAN_POINT('Ctrl Pts',(44.5079524583205,-55.5485514015906,
-46.3662));
#264844=CARTESIAN_POINT('Ctrl Pts',(43.6735798167943,-56.0302766707802,
-46.3078666666667));
#264845=CARTESIAN_POINT('Ctrl Pts',(42.839207175268,-56.5120019399698,-46.2495333333334));
#264846=CARTESIAN_POINT('Ctrl Pts',(42.839207175268,-57.4754524783491,-46.1912));
#264847=CARTESIAN_POINT('Ctrl Pts',(42.839207175268,-58.4389030167283,-46.1328666666667));
#264848=CARTESIAN_POINT('Ctrl Pts',(43.6735798167943,-58.920628285918,-46.0745333333334));
#264849=CARTESIAN_POINT('Ctrl Pts',(44.5079524583205,-59.4023535551075,
-46.0162));
#264850=CARTESIAN_POINT('Ctrl Pts',(45.3423250998467,-58.920628285918,-45.9578666666667));
#264851=CARTESIAN_POINT('Ctrl Pts',(46.1766977413729,-58.4389030167283,
-45.8995333333333));
#264852=CARTESIAN_POINT('Ctrl Pts',(46.1766977413729,-57.4754524783491,
-45.8412));
#264853=CARTESIAN_POINT('Ctrl Pts',(46.1766977413729,-56.5120019399699,
-45.7828666666667));
#264854=CARTESIAN_POINT('Ctrl Pts',(45.3423250998467,-56.0302766707802,
-45.7245333333333));
#264855=CARTESIAN_POINT('Ctrl Pts',(44.5079524583205,-55.5485514015906,
-45.6662));
#264856=CARTESIAN_POINT('Ctrl Pts',(43.6735798167943,-56.0302766707802,
-45.6078666666667));
#264857=CARTESIAN_POINT('Ctrl Pts',(42.839207175268,-56.5120019399698,-45.5495333333333));
#264858=CARTESIAN_POINT('Ctrl Pts',(42.839207175268,-57.4754524783491,-45.4912));
#264859=CARTESIAN_POINT('Ctrl Pts',(42.839207175268,-58.4389030167283,-45.4328666666666));
#264860=CARTESIAN_POINT('Ctrl Pts',(43.6735798167943,-58.920628285918,-45.3745333333334));
#264861=CARTESIAN_POINT('Ctrl Pts',(44.5079524583205,-59.4023535551075,
-45.3162));
#264862=CARTESIAN_POINT('Ctrl Pts',(45.3423250998467,-58.920628285918,-45.2578666666667));
#264863=CARTESIAN_POINT('Ctrl Pts',(46.1766977413729,-58.4389030167283,
-45.1995333333333));
#264864=CARTESIAN_POINT('Ctrl Pts',(46.1766977413729,-57.4754524783491,
-45.1412));
#264865=CARTESIAN_POINT('Ctrl Pts',(46.1766977413729,-56.5120019399699,
-45.0828666666667));
#264866=CARTESIAN_POINT('Ctrl Pts',(45.3423250998467,-56.0302766707802,
-45.0245333333334));
#264867=CARTESIAN_POINT('Ctrl Pts',(44.5079524583205,-55.5485514015906,
-44.9662));
#264868=CARTESIAN_POINT('Ctrl Pts',(43.6735798167943,-56.0302766707802,
-44.9078666666667));
#264869=CARTESIAN_POINT('Ctrl Pts',(42.839207175268,-56.5120019399698,-44.8495333333333));
#264870=CARTESIAN_POINT('Ctrl Pts',(42.839207175268,-57.4754524783491,-44.7912));
#264871=CARTESIAN_POINT('Ctrl Pts',(42.839207175268,-58.4389030167283,-44.7328666666667));
#264872=CARTESIAN_POINT('Ctrl Pts',(43.6735798167943,-58.920628285918,-44.6745333333334));
#264873=CARTESIAN_POINT('Ctrl Pts',(44.5079524583205,-59.4023535551075,
-44.6162));
#264874=CARTESIAN_POINT('Ctrl Pts',(45.3423250998467,-58.920628285918,-44.5578666666667));
#264875=CARTESIAN_POINT('Ctrl Pts',(46.1766977413729,-58.4389030167283,
-44.4995333333333));
#264876=CARTESIAN_POINT('Ctrl Pts',(46.1766977413729,-57.4754524783491,
-44.4412));
#264877=CARTESIAN_POINT('Ctrl Pts',(46.1766977413729,-56.5120019399699,
-44.3828666666667));
#264878=CARTESIAN_POINT('Ctrl Pts',(45.3423250998467,-56.0302766707802,
-44.3245333333334));
#264879=CARTESIAN_POINT('Ctrl Pts',(44.5079524583205,-55.5485514015906,
-44.2662));
#264880=CARTESIAN_POINT('Ctrl Pts',(43.6735798167943,-56.0302766707802,
-44.2078666666667));
#264881=CARTESIAN_POINT('Ctrl Pts',(42.839207175268,-56.5120019399698,-44.1495333333334));
#264882=CARTESIAN_POINT('Ctrl Pts',(42.839207175268,-57.4754524783491,-44.0912));
#264883=CARTESIAN_POINT('Ctrl Pts',(42.839207175268,-58.4389030167283,-44.0328666666667));
#264884=CARTESIAN_POINT('Ctrl Pts',(43.6735798167943,-58.920628285918,-43.9745333333333));
#264885=CARTESIAN_POINT('Ctrl Pts',(44.5079524583205,-59.4023535551075,
-43.9162));
#264886=CARTESIAN_POINT('Ctrl Pts',(45.3423250998467,-58.920628285918,-43.8578666666667));
#264887=CARTESIAN_POINT('Ctrl Pts',(46.1766977413729,-58.4389030167283,
-43.7995333333334));
#264888=CARTESIAN_POINT('Ctrl Pts',(46.1766977413729,-57.4754524783491,
-43.7412));
#264889=CARTESIAN_POINT('Ctrl Pts',(46.1766977413729,-56.5120019399699,
-43.6828666666667));
#264890=CARTESIAN_POINT('Ctrl Pts',(45.3423250998467,-56.0302766707802,
-43.6245333333333));
#264891=CARTESIAN_POINT('Ctrl Pts',(44.5079524583205,-55.5485514015906,
-43.5662));
#264892=CARTESIAN_POINT('Ctrl Pts',(43.6735798167943,-56.0302766707802,
-43.5078666666667));
#264893=CARTESIAN_POINT('Ctrl Pts',(42.839207175268,-56.5120019399698,-43.4495333333334));
#264894=CARTESIAN_POINT('Ctrl Pts',(42.839207175268,-57.4754524783491,-43.3912));
#264895=CARTESIAN_POINT('Ctrl Pts',(42.839207175268,-58.4389030167283,-43.3328666666667));
#264896=CARTESIAN_POINT('Ctrl Pts',(43.6735798167943,-58.920628285918,-43.2745333333334));
#264897=CARTESIAN_POINT('Ctrl Pts',(44.5079524583205,-59.4023535551075,
-43.2162));
#264898=CARTESIAN_POINT('Ctrl Pts',(45.3423250998467,-58.920628285918,-43.1578666666667));
#264899=CARTESIAN_POINT('Ctrl Pts',(46.1766977413729,-58.4389030167283,
-43.0995333333334));
#264900=CARTESIAN_POINT('Ctrl Pts',(46.1766977413729,-57.4754524783491,
-43.0412));
#264901=CARTESIAN_POINT('Ctrl Pts',(46.1766977413729,-56.5120019399699,
-42.9828666666667));
#264902=CARTESIAN_POINT('Ctrl Pts',(45.3423250998467,-56.0302766707802,
-42.9245333333334));
#264903=CARTESIAN_POINT('Ctrl Pts',(44.5079524583205,-55.5485514015906,
-42.8662));
#264904=CARTESIAN_POINT('Ctrl Pts',(43.6735798167943,-56.0302766707802,
-42.8078666666667));
#264905=CARTESIAN_POINT('Ctrl Pts',(42.839207175268,-56.5120019399698,-42.7495333333334));
#264906=CARTESIAN_POINT('Ctrl Pts',(42.839207175268,-57.4754524783491,-42.6912));
#264907=CARTESIAN_POINT('Ctrl Pts',(42.839207175268,-58.4389030167283,-42.6328666666667));
#264908=CARTESIAN_POINT('Ctrl Pts',(43.6735798167943,-58.920628285918,-42.5745333333333));
#264909=CARTESIAN_POINT('Ctrl Pts',(44.5079524583205,-59.4023535551075,
-42.5162));
#264910=CARTESIAN_POINT('Ctrl Pts',(45.3423250998467,-58.920628285918,-42.4578666666667));
#264911=CARTESIAN_POINT('Ctrl Pts',(46.1766977413729,-58.4389030167283,
-42.3995333333334));
#264912=CARTESIAN_POINT('Ctrl Pts',(46.1766977413729,-57.4754524783491,
-42.3412));
#264913=CARTESIAN_POINT('Ctrl Pts',(46.1766977413729,-56.5120019399699,
-42.2828666666667));
#264914=CARTESIAN_POINT('Ctrl Pts',(45.3423250998467,-56.0302766707802,
-42.2245333333333));
#264915=CARTESIAN_POINT('Ctrl Pts',(44.5079524583205,-55.5485514015906,
-42.1662));
#264916=CARTESIAN_POINT('Ctrl Pts',(43.6735798167943,-56.0302766707802,
-42.1078666666667));
#264917=CARTESIAN_POINT('Ctrl Pts',(42.839207175268,-56.5120019399698,-42.0495333333334));
#264918=CARTESIAN_POINT('Ctrl Pts',(42.839207175268,-57.4754524783491,-41.9912));
#264919=CARTESIAN_POINT('Ctrl Pts',(42.839207175268,-58.4389030167283,-41.9328666666667));
#264920=CARTESIAN_POINT('Ctrl Pts',(43.6735798167943,-58.920628285918,-41.8745333333334));
#264921=CARTESIAN_POINT('Ctrl Pts',(44.5079524583205,-59.4023535551075,
-41.8162));
#264922=CARTESIAN_POINT('Ctrl Pts',(45.3423250998467,-58.920628285918,-41.7578666666667));
#264923=CARTESIAN_POINT('Ctrl Pts',(46.1766977413729,-58.4389030167283,
-41.6995333333334));
#264924=CARTESIAN_POINT('Ctrl Pts',(46.1766977413729,-57.4754524783491,
-41.6412));
#264925=CARTESIAN_POINT('Ctrl Pts',(46.1766977413729,-56.5120019399699,
-41.5828666666667));
#264926=CARTESIAN_POINT('Ctrl Pts',(45.3423250998467,-56.0302766707802,
-41.5245333333334));
#264927=CARTESIAN_POINT('Ctrl Pts',(44.5079524583205,-55.5485514015906,
-41.4662));
#264928=CARTESIAN_POINT('Ctrl Pts',(43.6735798167943,-56.0302766707802,
-41.4078666666667));
#264929=CARTESIAN_POINT('Ctrl Pts',(42.839207175268,-56.5120019399698,-41.3495333333333));
#264930=CARTESIAN_POINT('Ctrl Pts',(42.839207175268,-57.4754524783491,-41.2912));
#264931=CARTESIAN_POINT('Ctrl Pts',(42.839207175268,-58.4389030167283,-41.2328666666667));
#264932=CARTESIAN_POINT('Ctrl Pts',(43.6735798167943,-58.920628285918,-41.1745333333334));
#264933=CARTESIAN_POINT('Ctrl Pts',(44.5079524583205,-59.4023535551075,
-41.1162));
#264934=CARTESIAN_POINT('Ctrl Pts',(45.3423250998467,-58.920628285918,-41.0578666666667));
#264935=CARTESIAN_POINT('Ctrl Pts',(46.1766977413729,-58.4389030167283,
-40.9995333333333));
#264936=CARTESIAN_POINT('Ctrl Pts',(46.1766977413729,-57.4754524783491,
-40.9412));
#264937=CARTESIAN_POINT('Ctrl Pts',(46.1766977413729,-56.5120019399699,
-40.8828666666667));
#264938=CARTESIAN_POINT('Ctrl Pts',(45.3423250998467,-56.0302766707802,
-40.8245333333333));
#264939=CARTESIAN_POINT('Ctrl Pts',(44.5079524583205,-55.5485514015906,
-40.7662));
#264940=CARTESIAN_POINT('Ctrl Pts',(43.6735798167943,-56.0302766707802,
-40.7078666666667));
#264941=CARTESIAN_POINT('Ctrl Pts',(42.839207175268,-56.5120019399698,-40.6495333333334));
#264942=CARTESIAN_POINT('Ctrl Pts',(42.839207175268,-57.4754524783491,-40.5912));
#264943=CARTESIAN_POINT('Ctrl Pts',(42.839207175268,-58.4389030167283,-40.5328666666667));
#264944=CARTESIAN_POINT('Ctrl Pts',(43.6735798167943,-58.920628285918,-40.4745333333334));
#264945=CARTESIAN_POINT('Ctrl Pts',(44.5079524583205,-59.4023535551075,
-40.4162));
#264946=CARTESIAN_POINT('Ctrl Pts',(45.3423250998467,-58.920628285918,-40.3578666666667));
#264947=CARTESIAN_POINT('Ctrl Pts',(46.1766977413729,-58.4389030167283,
-40.2995333333333));
#264948=CARTESIAN_POINT('Ctrl Pts',(46.1766977413729,-57.4754524783491,
-40.2412));
#264949=CARTESIAN_POINT('Ctrl Pts',(46.1766977413729,-56.5120019399699,
-40.1828666666667));
#264950=CARTESIAN_POINT('Ctrl Pts',(45.3423250998467,-56.0302766707802,
-40.1245333333334));
#264951=CARTESIAN_POINT('Ctrl Pts',(44.5079524583205,-55.5485514015906,
-40.0662));
#264952=CARTESIAN_POINT('Ctrl Pts',(43.6735798167943,-56.0302766707802,
-40.0078666666667));
#264953=CARTESIAN_POINT('Ctrl Pts',(42.839207175268,-56.5120019399698,-39.9495333333333));
#264954=CARTESIAN_POINT('Ctrl Pts',(42.839207175268,-57.4754524783491,-39.8912));
#264955=CARTESIAN_POINT('Ctrl Pts',(42.839207175268,-58.4389030167283,-39.8328666666666));
#264956=CARTESIAN_POINT('Ctrl Pts',(43.6735798167943,-58.920628285918,-39.7745333333334));
#264957=CARTESIAN_POINT('Ctrl Pts',(44.5079524583205,-59.4023535551075,
-39.7162));
#264958=CARTESIAN_POINT('Ctrl Pts',(45.3423250998467,-58.920628285918,-39.6578666666667));
#264959=CARTESIAN_POINT('Ctrl Pts',(46.1766977413729,-58.4389030167283,
-39.5995333333333));
#264960=CARTESIAN_POINT('Ctrl Pts',(46.1766977413729,-57.4754524783491,
-39.5412));
#264961=CARTESIAN_POINT('Ctrl Pts',(46.1766977413729,-56.5120019399699,
-39.4828666666666));
#264962=CARTESIAN_POINT('Ctrl Pts',(45.3423250998467,-56.0302766707802,
-39.4245333333334));
#264963=CARTESIAN_POINT('Ctrl Pts',(44.5079524583205,-55.5485514015906,
-39.3662));
#264964=CARTESIAN_POINT('Ctrl Pts',(43.6735798167943,-56.0302766707802,
-39.3078666666667));
#264965=CARTESIAN_POINT('Ctrl Pts',(42.839207175268,-56.5120019399698,-39.2495333333333));
#264966=CARTESIAN_POINT('Ctrl Pts',(42.839207175268,-57.4754524783491,-39.1912));
#264967=CARTESIAN_POINT('Ctrl Pts',(42.839207175268,-58.4389030167283,-39.1328666666667));
#264968=CARTESIAN_POINT('Ctrl Pts',(43.6735798167943,-58.920628285918,-39.0745333333333));
#264969=CARTESIAN_POINT('Ctrl Pts',(44.5079524583205,-59.4023535551075,
-39.0162));
#264970=CARTESIAN_POINT('Ctrl Pts',(45.3423250998467,-58.920628285918,-38.9578666666667));
#264971=CARTESIAN_POINT('Ctrl Pts',(46.1766977413729,-58.4389030167283,
-38.8995333333334));
#264972=CARTESIAN_POINT('Ctrl Pts',(46.1766977413729,-57.4754524783491,
-38.8412));
#264973=CARTESIAN_POINT('Ctrl Pts',(46.1766977413729,-56.5120019399699,
-38.7828666666667));
#264974=CARTESIAN_POINT('Ctrl Pts',(45.3423250998467,-56.0302766707802,
-38.7245333333334));
#264975=CARTESIAN_POINT('Ctrl Pts',(44.5079524583205,-55.5485514015906,
-38.6662));
#264976=CARTESIAN_POINT('Ctrl Pts',(43.6735798167943,-56.0302766707802,
-38.6078666666667));
#264977=CARTESIAN_POINT('Ctrl Pts',(42.839207175268,-56.5120019399698,-38.5495333333334));
#264978=CARTESIAN_POINT('Ctrl Pts',(42.839207175268,-57.4754524783491,-38.4912));
#264979=CARTESIAN_POINT('Ctrl Pts',(42.839207175268,-58.4389030167283,-38.4328666666667));
#264980=CARTESIAN_POINT('Ctrl Pts',(43.6735798167943,-58.920628285918,-38.3745333333333));
#264981=CARTESIAN_POINT('Ctrl Pts',(44.5079524583205,-59.4023535551075,
-38.3162));
#264982=CARTESIAN_POINT('Ctrl Pts',(45.3423250998467,-58.920628285918,-38.2578666666667));
#264983=CARTESIAN_POINT('Ctrl Pts',(46.1766977413729,-58.4389030167283,
-38.1995333333333));
#264984=CARTESIAN_POINT('Ctrl Pts',(46.1766977413729,-57.4754524783491,
-38.1412));
#264985=CARTESIAN_POINT('Ctrl Pts',(46.1766977413729,-56.5120019399699,
-38.0828666666667));
#264986=CARTESIAN_POINT('Ctrl Pts',(45.3423250998467,-56.0302766707802,
-38.0245333333334));
#264987=CARTESIAN_POINT('Ctrl Pts',(44.5079524583205,-55.5485514015906,
-37.9662));
#264988=CARTESIAN_POINT('Ctrl Pts',(43.6735798167943,-56.0302766707802,
-37.9078666666667));
#264989=CARTESIAN_POINT('Ctrl Pts',(42.839207175268,-56.5120019399698,-37.8495333333334));
#264990=CARTESIAN_POINT('Ctrl Pts',(42.839207175268,-57.4754524783491,-37.7912));
#264991=CARTESIAN_POINT('Ctrl Pts',(42.839207175268,-58.4389030167283,-37.7328666666667));
#264992=CARTESIAN_POINT('Ctrl Pts',(43.6735798167943,-58.920628285918,-37.6745333333334));
#264993=CARTESIAN_POINT('Ctrl Pts',(44.5079524583205,-59.4023535551075,
-37.6162));
#264994=CARTESIAN_POINT('Ctrl Pts',(45.3423250998467,-58.920628285918,-37.5578666666667));
#264995=CARTESIAN_POINT('Ctrl Pts',(46.1766977413729,-58.4389030167283,
-37.4995333333334));
#264996=CARTESIAN_POINT('Ctrl Pts',(46.1766977413729,-57.4754524783491,
-37.4412));
#264997=CARTESIAN_POINT('Ctrl Pts',(46.1766977413729,-56.5120019399699,
-37.3828666666667));
#264998=CARTESIAN_POINT('Ctrl Pts',(45.3423250998467,-56.0302766707802,
-37.3245333333333));
#264999=CARTESIAN_POINT('Ctrl Pts',(44.5079524583205,-55.5485514015906,
-37.2662));
#265000=CARTESIAN_POINT('Ctrl Pts',(43.6735798167943,-56.0302766707802,
-37.2078666666667));
#265001=CARTESIAN_POINT('Ctrl Pts',(42.839207175268,-56.5120019399698,-37.1495333333334));
#265002=CARTESIAN_POINT('Ctrl Pts',(42.839207175268,-57.4754524783491,-37.0912));
#265003=CARTESIAN_POINT('Ctrl Pts',(42.839207175268,-58.4389030167283,-37.0328666666667));
#265004=CARTESIAN_POINT('Ctrl Pts',(43.6735798167943,-58.920628285918,-36.9745333333333));
#265005=CARTESIAN_POINT('Ctrl Pts',(44.5079524583205,-59.4023535551075,
-36.9162));
#265006=CARTESIAN_POINT('Ctrl Pts',(45.3423250998467,-58.920628285918,-36.8578666666667));
#265007=CARTESIAN_POINT('Ctrl Pts',(45.4506436431264,-58.8580905457972,
-36.8502938132714));
#265008=CARTESIAN_POINT('Ctrl Pts',(45.5484297036483,-58.7801048924675,
-36.8421538241181));
#265009=CARTESIAN_POINT('Ctrl Pts',(46.5766932247459,-57.4754524783491,
-52.6102625));
#265010=CARTESIAN_POINT('Ctrl Pts',(46.5766932247459,-56.2810644399698,
-52.5519291666666));
#265011=CARTESIAN_POINT('Ctrl Pts',(45.5423228415332,-55.6838704207802,
-52.4935958333333));
#265012=CARTESIAN_POINT('Ctrl Pts',(44.5079524583205,-55.0866764015906,
-52.4352625000001));
#265013=CARTESIAN_POINT('Ctrl Pts',(43.4735820751078,-55.6838704207802,
-52.3769291666667));
#265014=CARTESIAN_POINT('Ctrl Pts',(42.4392116918951,-56.2810644399698,
-52.3185958333334));
#265015=CARTESIAN_POINT('Ctrl Pts',(42.439211691895,-57.4754524783491,-52.2602625));
#265016=CARTESIAN_POINT('Ctrl Pts',(42.4392116918951,-58.6698405167284,
-52.2019291666667));
#265017=CARTESIAN_POINT('Ctrl Pts',(43.4735820751078,-59.267034535918,-52.1435958333333));
#265018=CARTESIAN_POINT('Ctrl Pts',(44.5079524583205,-59.8642285551076,
-52.0852625));
#265019=CARTESIAN_POINT('Ctrl Pts',(45.5423228415332,-59.267034535918,-52.0269291666667));
#265020=CARTESIAN_POINT('Ctrl Pts',(46.5766932247459,-58.6698405167284,
-51.9685958333333));
#265021=CARTESIAN_POINT('Ctrl Pts',(46.5766932247459,-57.4754524783491,
-51.9102625));
#265022=CARTESIAN_POINT('Ctrl Pts',(46.5766932247459,-56.2810644399698,
-51.8519291666667));
#265023=CARTESIAN_POINT('Ctrl Pts',(45.5423228415332,-55.6838704207802,
-51.7935958333333));
#265024=CARTESIAN_POINT('Ctrl Pts',(44.5079524583205,-55.0866764015906,
-51.7352625));
#265025=CARTESIAN_POINT('Ctrl Pts',(43.4735820751078,-55.6838704207802,
-51.6769291666667));
#265026=CARTESIAN_POINT('Ctrl Pts',(42.4392116918951,-56.2810644399698,
-51.6185958333333));
#265027=CARTESIAN_POINT('Ctrl Pts',(42.439211691895,-57.4754524783491,-51.5602625));
#265028=CARTESIAN_POINT('Ctrl Pts',(42.4392116918951,-58.6698405167284,
-51.5019291666666));
#265029=CARTESIAN_POINT('Ctrl Pts',(43.4735820751078,-59.267034535918,-51.4435958333333));
#265030=CARTESIAN_POINT('Ctrl Pts',(44.5079524583205,-59.8642285551076,
-51.3852625));
#265031=CARTESIAN_POINT('Ctrl Pts',(45.5423228415332,-59.267034535918,-51.3269291666667));
#265032=CARTESIAN_POINT('Ctrl Pts',(46.5766932247459,-58.6698405167284,
-51.2685958333333));
#265033=CARTESIAN_POINT('Ctrl Pts',(46.5766932247459,-57.4754524783491,
-51.2102625));
#265034=CARTESIAN_POINT('Ctrl Pts',(46.5766932247459,-56.2810644399698,
-51.1519291666666));
#265035=CARTESIAN_POINT('Ctrl Pts',(45.5423228415332,-55.6838704207802,
-51.0935958333334));
#265036=CARTESIAN_POINT('Ctrl Pts',(44.5079524583205,-55.0866764015906,
-51.0352625));
#265037=CARTESIAN_POINT('Ctrl Pts',(43.4735820751078,-55.6838704207802,
-50.9769291666667));
#265038=CARTESIAN_POINT('Ctrl Pts',(42.4392116918951,-56.2810644399698,
-50.9185958333333));
#265039=CARTESIAN_POINT('Ctrl Pts',(42.439211691895,-57.4754524783491,-50.8602625));
#265040=CARTESIAN_POINT('Ctrl Pts',(42.4392116918951,-58.6698405167284,
-50.8019291666667));
#265041=CARTESIAN_POINT('Ctrl Pts',(43.4735820751078,-59.267034535918,-50.7435958333333));
#265042=CARTESIAN_POINT('Ctrl Pts',(44.5079524583205,-59.8642285551076,
-50.6852625));
#265043=CARTESIAN_POINT('Ctrl Pts',(45.5423228415332,-59.267034535918,-50.6269291666667));
#265044=CARTESIAN_POINT('Ctrl Pts',(46.5766932247459,-58.6698405167284,
-50.5685958333333));
#265045=CARTESIAN_POINT('Ctrl Pts',(46.5766932247459,-57.4754524783491,
-50.5102625));
#265046=CARTESIAN_POINT('Ctrl Pts',(46.5766932247459,-56.2810644399698,
-50.4519291666667));
#265047=CARTESIAN_POINT('Ctrl Pts',(45.5423228415332,-55.6838704207802,
-50.3935958333333));
#265048=CARTESIAN_POINT('Ctrl Pts',(44.5079524583205,-55.0866764015906,
-50.3352625));
#265049=CARTESIAN_POINT('Ctrl Pts',(43.4735820751078,-55.6838704207802,
-50.2769291666667));
#265050=CARTESIAN_POINT('Ctrl Pts',(42.4392116918951,-56.2810644399698,
-50.2185958333333));
#265051=CARTESIAN_POINT('Ctrl Pts',(42.439211691895,-57.4754524783491,-50.1602625));
#265052=CARTESIAN_POINT('Ctrl Pts',(42.4392116918951,-58.6698405167284,
-50.1019291666667));
#265053=CARTESIAN_POINT('Ctrl Pts',(43.4735820751078,-59.267034535918,-50.0435958333333));
#265054=CARTESIAN_POINT('Ctrl Pts',(44.5079524583205,-59.8642285551076,
-49.9852625));
#265055=CARTESIAN_POINT('Ctrl Pts',(45.5423228415332,-59.267034535918,-49.9269291666667));
#265056=CARTESIAN_POINT('Ctrl Pts',(46.5766932247459,-58.6698405167284,
-49.8685958333333));
#265057=CARTESIAN_POINT('Ctrl Pts',(46.5766932247459,-57.4754524783491,
-49.8102625));
#265058=CARTESIAN_POINT('Ctrl Pts',(46.5766932247459,-56.2810644399698,
-49.7519291666667));
#265059=CARTESIAN_POINT('Ctrl Pts',(45.5423228415332,-55.6838704207802,
-49.6935958333334));
#265060=CARTESIAN_POINT('Ctrl Pts',(44.5079524583205,-55.0866764015906,
-49.6352625));
#265061=CARTESIAN_POINT('Ctrl Pts',(43.4735820751078,-55.6838704207802,
-49.5769291666667));
#265062=CARTESIAN_POINT('Ctrl Pts',(42.4392116918951,-56.2810644399698,
-49.5185958333334));
#265063=CARTESIAN_POINT('Ctrl Pts',(42.439211691895,-57.4754524783491,-49.4602625));
#265064=CARTESIAN_POINT('Ctrl Pts',(42.4392116918951,-58.6698405167284,
-49.4019291666667));
#265065=CARTESIAN_POINT('Ctrl Pts',(43.4735820751078,-59.267034535918,-49.3435958333333));
#265066=CARTESIAN_POINT('Ctrl Pts',(44.5079524583205,-59.8642285551076,
-49.2852625));
#265067=CARTESIAN_POINT('Ctrl Pts',(45.5423228415332,-59.267034535918,-49.2269291666667));
#265068=CARTESIAN_POINT('Ctrl Pts',(46.5766932247459,-58.6698405167284,
-49.1685958333334));
#265069=CARTESIAN_POINT('Ctrl Pts',(46.5766932247459,-57.4754524783491,
-49.1102625));
#265070=CARTESIAN_POINT('Ctrl Pts',(46.5766932247459,-56.2810644399698,
-49.0519291666667));
#265071=CARTESIAN_POINT('Ctrl Pts',(45.5423228415332,-55.6838704207802,
-48.9935958333333));
#265072=CARTESIAN_POINT('Ctrl Pts',(44.5079524583205,-55.0866764015906,
-48.9352625));
#265073=CARTESIAN_POINT('Ctrl Pts',(43.4735820751078,-55.6838704207802,
-48.8769291666667));
#265074=CARTESIAN_POINT('Ctrl Pts',(42.4392116918951,-56.2810644399698,
-48.8185958333334));
#265075=CARTESIAN_POINT('Ctrl Pts',(42.439211691895,-57.4754524783491,-48.7602625));
#265076=CARTESIAN_POINT('Ctrl Pts',(42.4392116918951,-58.6698405167284,
-48.7019291666667));
#265077=CARTESIAN_POINT('Ctrl Pts',(43.4735820751078,-59.267034535918,-48.6435958333333));
#265078=CARTESIAN_POINT('Ctrl Pts',(44.5079524583205,-59.8642285551076,
-48.5852625));
#265079=CARTESIAN_POINT('Ctrl Pts',(45.5423228415332,-59.267034535918,-48.5269291666667));
#265080=CARTESIAN_POINT('Ctrl Pts',(46.5766932247459,-58.6698405167284,
-48.4685958333333));
#265081=CARTESIAN_POINT('Ctrl Pts',(46.5766932247459,-57.4754524783491,
-48.4102625));
#265082=CARTESIAN_POINT('Ctrl Pts',(46.5766932247459,-56.2810644399698,
-48.3519291666667));
#265083=CARTESIAN_POINT('Ctrl Pts',(45.5423228415332,-55.6838704207802,
-48.2935958333334));
#265084=CARTESIAN_POINT('Ctrl Pts',(44.5079524583205,-55.0866764015906,
-48.2352625));
#265085=CARTESIAN_POINT('Ctrl Pts',(43.4735820751078,-55.6838704207802,
-48.1769291666667));
#265086=CARTESIAN_POINT('Ctrl Pts',(42.4392116918951,-56.2810644399698,
-48.1185958333334));
#265087=CARTESIAN_POINT('Ctrl Pts',(42.439211691895,-57.4754524783491,-48.0602625));
#265088=CARTESIAN_POINT('Ctrl Pts',(42.4392116918951,-58.6698405167284,
-48.0019291666667));
#265089=CARTESIAN_POINT('Ctrl Pts',(43.4735820751078,-59.267034535918,-47.9435958333334));
#265090=CARTESIAN_POINT('Ctrl Pts',(44.5079524583205,-59.8642285551076,
-47.8852625));
#265091=CARTESIAN_POINT('Ctrl Pts',(45.5423228415332,-59.267034535918,-47.8269291666667));
#265092=CARTESIAN_POINT('Ctrl Pts',(46.5766932247459,-58.6698405167284,
-47.7685958333333));
#265093=CARTESIAN_POINT('Ctrl Pts',(46.5766932247459,-57.4754524783491,
-47.7102625));
#265094=CARTESIAN_POINT('Ctrl Pts',(46.5766932247459,-56.2810644399698,
-47.6519291666667));
#265095=CARTESIAN_POINT('Ctrl Pts',(45.5423228415332,-55.6838704207802,
-47.5935958333333));
#265096=CARTESIAN_POINT('Ctrl Pts',(44.5079524583205,-55.0866764015906,
-47.5352625));
#265097=CARTESIAN_POINT('Ctrl Pts',(43.4735820751078,-55.6838704207802,
-47.4769291666667));
#265098=CARTESIAN_POINT('Ctrl Pts',(42.4392116918951,-56.2810644399698,
-47.4185958333333));
#265099=CARTESIAN_POINT('Ctrl Pts',(42.439211691895,-57.4754524783491,-47.3602625));
#265100=CARTESIAN_POINT('Ctrl Pts',(42.4392116918951,-58.6698405167284,
-47.3019291666666));
#265101=CARTESIAN_POINT('Ctrl Pts',(43.4735820751078,-59.267034535918,-47.2435958333334));
#265102=CARTESIAN_POINT('Ctrl Pts',(44.5079524583205,-59.8642285551076,
-47.1852625));
#265103=CARTESIAN_POINT('Ctrl Pts',(45.5423228415332,-59.267034535918,-47.1269291666667));
#265104=CARTESIAN_POINT('Ctrl Pts',(46.5766932247459,-58.6698405167284,
-47.0685958333333));
#265105=CARTESIAN_POINT('Ctrl Pts',(46.5766932247459,-57.4754524783491,
-47.0102625));
#265106=CARTESIAN_POINT('Ctrl Pts',(46.5766932247459,-56.2810644399698,
-46.9519291666667));
#265107=CARTESIAN_POINT('Ctrl Pts',(45.5423228415332,-55.6838704207802,
-46.8935958333333));
#265108=CARTESIAN_POINT('Ctrl Pts',(44.5079524583205,-55.0866764015906,
-46.8352625));
#265109=CARTESIAN_POINT('Ctrl Pts',(43.4735820751078,-55.6838704207802,
-46.7769291666667));
#265110=CARTESIAN_POINT('Ctrl Pts',(42.4392116918951,-56.2810644399698,
-46.7185958333333));
#265111=CARTESIAN_POINT('Ctrl Pts',(42.439211691895,-57.4754524783491,-46.6602625));
#265112=CARTESIAN_POINT('Ctrl Pts',(42.4392116918951,-58.6698405167284,
-46.6019291666667));
#265113=CARTESIAN_POINT('Ctrl Pts',(43.4735820751078,-59.267034535918,-46.5435958333334));
#265114=CARTESIAN_POINT('Ctrl Pts',(44.5079524583205,-59.8642285551076,
-46.4852625));
#265115=CARTESIAN_POINT('Ctrl Pts',(45.5423228415332,-59.267034535918,-46.4269291666667));
#265116=CARTESIAN_POINT('Ctrl Pts',(46.5766932247459,-58.6698405167284,
-46.3685958333333));
#265117=CARTESIAN_POINT('Ctrl Pts',(46.5766932247459,-57.4754524783491,
-46.3102625));
#265118=CARTESIAN_POINT('Ctrl Pts',(46.5766932247459,-56.2810644399698,
-46.2519291666667));
#265119=CARTESIAN_POINT('Ctrl Pts',(45.5423228415332,-55.6838704207802,
-46.1935958333333));
#265120=CARTESIAN_POINT('Ctrl Pts',(44.5079524583205,-55.0866764015906,
-46.1352625));
#265121=CARTESIAN_POINT('Ctrl Pts',(43.4735820751078,-55.6838704207802,
-46.0769291666667));
#265122=CARTESIAN_POINT('Ctrl Pts',(42.4392116918951,-56.2810644399698,
-46.0185958333334));
#265123=CARTESIAN_POINT('Ctrl Pts',(42.439211691895,-57.4754524783491,-45.9602625));
#265124=CARTESIAN_POINT('Ctrl Pts',(42.4392116918951,-58.6698405167284,
-45.9019291666667));
#265125=CARTESIAN_POINT('Ctrl Pts',(43.4735820751078,-59.267034535918,-45.8435958333333));
#265126=CARTESIAN_POINT('Ctrl Pts',(44.5079524583205,-59.8642285551076,
-45.7852625));
#265127=CARTESIAN_POINT('Ctrl Pts',(45.5423228415332,-59.267034535918,-45.7269291666667));
#265128=CARTESIAN_POINT('Ctrl Pts',(46.5766932247459,-58.6698405167284,
-45.6685958333334));
#265129=CARTESIAN_POINT('Ctrl Pts',(46.5766932247459,-57.4754524783491,
-45.6102625));
#265130=CARTESIAN_POINT('Ctrl Pts',(46.5766932247459,-56.2810644399698,
-45.5519291666667));
#265131=CARTESIAN_POINT('Ctrl Pts',(45.5423228415332,-55.6838704207802,
-45.4935958333333));
#265132=CARTESIAN_POINT('Ctrl Pts',(44.5079524583205,-55.0866764015906,
-45.4352625));
#265133=CARTESIAN_POINT('Ctrl Pts',(43.4735820751078,-55.6838704207802,
-45.3769291666667));
#265134=CARTESIAN_POINT('Ctrl Pts',(42.4392116918951,-56.2810644399698,
-45.3185958333333));
#265135=CARTESIAN_POINT('Ctrl Pts',(42.439211691895,-57.4754524783491,-45.2602625));
#265136=CARTESIAN_POINT('Ctrl Pts',(42.4392116918951,-58.6698405167284,
-45.2019291666667));
#265137=CARTESIAN_POINT('Ctrl Pts',(43.4735820751078,-59.267034535918,-45.1435958333334));
#265138=CARTESIAN_POINT('Ctrl Pts',(44.5079524583205,-59.8642285551076,
-45.0852625));
#265139=CARTESIAN_POINT('Ctrl Pts',(45.5423228415332,-59.267034535918,-45.0269291666667));
#265140=CARTESIAN_POINT('Ctrl Pts',(46.5766932247459,-58.6698405167284,
-44.9685958333334));
#265141=CARTESIAN_POINT('Ctrl Pts',(46.5766932247459,-57.4754524783491,
-44.9102625));
#265142=CARTESIAN_POINT('Ctrl Pts',(46.5766932247459,-56.2810644399698,
-44.8519291666667));
#265143=CARTESIAN_POINT('Ctrl Pts',(45.5423228415332,-55.6838704207802,
-44.7935958333333));
#265144=CARTESIAN_POINT('Ctrl Pts',(44.5079524583205,-55.0866764015906,
-44.7352625));
#265145=CARTESIAN_POINT('Ctrl Pts',(43.4735820751078,-55.6838704207802,
-44.6769291666667));
#265146=CARTESIAN_POINT('Ctrl Pts',(42.4392116918951,-56.2810644399698,
-44.6185958333334));
#265147=CARTESIAN_POINT('Ctrl Pts',(42.439211691895,-57.4754524783491,-44.5602625));
#265148=CARTESIAN_POINT('Ctrl Pts',(42.4392116918951,-58.6698405167284,
-44.5019291666667));
#265149=CARTESIAN_POINT('Ctrl Pts',(43.4735820751078,-59.267034535918,-44.4435958333333));
#265150=CARTESIAN_POINT('Ctrl Pts',(44.5079524583205,-59.8642285551076,
-44.3852625));
#265151=CARTESIAN_POINT('Ctrl Pts',(45.5423228415332,-59.267034535918,-44.3269291666667));
#265152=CARTESIAN_POINT('Ctrl Pts',(46.5766932247459,-58.6698405167284,
-44.2685958333334));
#265153=CARTESIAN_POINT('Ctrl Pts',(46.5766932247459,-57.4754524783491,
-44.2102625));
#265154=CARTESIAN_POINT('Ctrl Pts',(46.5766932247459,-56.2810644399698,
-44.1519291666667));
#265155=CARTESIAN_POINT('Ctrl Pts',(45.5423228415332,-55.6838704207802,
-44.0935958333334));
#265156=CARTESIAN_POINT('Ctrl Pts',(44.5079524583205,-55.0866764015906,
-44.0352625));
#265157=CARTESIAN_POINT('Ctrl Pts',(43.4735820751078,-55.6838704207802,
-43.9769291666667));
#265158=CARTESIAN_POINT('Ctrl Pts',(42.4392116918951,-56.2810644399698,
-43.9185958333334));
#265159=CARTESIAN_POINT('Ctrl Pts',(42.439211691895,-57.4754524783491,-43.8602625));
#265160=CARTESIAN_POINT('Ctrl Pts',(42.4392116918951,-58.6698405167284,
-43.8019291666667));
#265161=CARTESIAN_POINT('Ctrl Pts',(43.4735820751078,-59.267034535918,-43.7435958333334));
#265162=CARTESIAN_POINT('Ctrl Pts',(44.5079524583205,-59.8642285551076,
-43.6852625));
#265163=CARTESIAN_POINT('Ctrl Pts',(45.5423228415332,-59.267034535918,-43.6269291666667));
#265164=CARTESIAN_POINT('Ctrl Pts',(46.5766932247459,-58.6698405167284,
-43.5685958333334));
#265165=CARTESIAN_POINT('Ctrl Pts',(46.5766932247459,-57.4754524783491,
-43.5102625));
#265166=CARTESIAN_POINT('Ctrl Pts',(46.5766932247459,-56.2810644399698,
-43.4519291666667));
#265167=CARTESIAN_POINT('Ctrl Pts',(45.5423228415332,-55.6838704207802,
-43.3935958333334));
#265168=CARTESIAN_POINT('Ctrl Pts',(44.5079524583205,-55.0866764015906,
-43.3352625));
#265169=CARTESIAN_POINT('Ctrl Pts',(43.4735820751078,-55.6838704207802,
-43.2769291666667));
#265170=CARTESIAN_POINT('Ctrl Pts',(42.4392116918951,-56.2810644399698,
-43.2185958333334));
#265171=CARTESIAN_POINT('Ctrl Pts',(42.439211691895,-57.4754524783491,-43.1602625));
#265172=CARTESIAN_POINT('Ctrl Pts',(42.4392116918951,-58.6698405167284,
-43.1019291666667));
#265173=CARTESIAN_POINT('Ctrl Pts',(43.4735820751078,-59.267034535918,-43.0435958333334));
#265174=CARTESIAN_POINT('Ctrl Pts',(44.5079524583205,-59.8642285551076,
-42.9852625));
#265175=CARTESIAN_POINT('Ctrl Pts',(45.5423228415332,-59.267034535918,-42.9269291666667));
#265176=CARTESIAN_POINT('Ctrl Pts',(46.5766932247459,-58.6698405167284,
-42.8685958333333));
#265177=CARTESIAN_POINT('Ctrl Pts',(46.5766932247459,-57.4754524783491,
-42.8102625));
#265178=CARTESIAN_POINT('Ctrl Pts',(46.5766932247459,-56.2810644399698,
-42.7519291666667));
#265179=CARTESIAN_POINT('Ctrl Pts',(45.5423228415332,-55.6838704207802,
-42.6935958333333));
#265180=CARTESIAN_POINT('Ctrl Pts',(44.5079524583205,-55.0866764015906,
-42.6352625));
#265181=CARTESIAN_POINT('Ctrl Pts',(43.4735820751078,-55.6838704207802,
-42.5769291666667));
#265182=CARTESIAN_POINT('Ctrl Pts',(42.4392116918951,-56.2810644399698,
-42.5185958333333));
#265183=CARTESIAN_POINT('Ctrl Pts',(42.439211691895,-57.4754524783491,-42.4602625));
#265184=CARTESIAN_POINT('Ctrl Pts',(42.4392116918951,-58.6698405167284,
-42.4019291666666));
#265185=CARTESIAN_POINT('Ctrl Pts',(43.4735820751078,-59.267034535918,-42.3435958333334));
#265186=CARTESIAN_POINT('Ctrl Pts',(44.5079524583205,-59.8642285551076,
-42.2852625));
#265187=CARTESIAN_POINT('Ctrl Pts',(45.5423228415332,-59.267034535918,-42.2269291666667));
#265188=CARTESIAN_POINT('Ctrl Pts',(46.5766932247459,-58.6698405167284,
-42.1685958333333));
#265189=CARTESIAN_POINT('Ctrl Pts',(46.5766932247459,-57.4754524783491,
-42.1102625));
#265190=CARTESIAN_POINT('Ctrl Pts',(46.5766932247459,-56.2810644399698,
-42.0519291666667));
#265191=CARTESIAN_POINT('Ctrl Pts',(45.5423228415332,-55.6838704207802,
-41.9935958333334));
#265192=CARTESIAN_POINT('Ctrl Pts',(44.5079524583205,-55.0866764015906,
-41.9352625));
#265193=CARTESIAN_POINT('Ctrl Pts',(43.4735820751078,-55.6838704207802,
-41.8769291666667));
#265194=CARTESIAN_POINT('Ctrl Pts',(42.4392116918951,-56.2810644399698,
-41.8185958333333));
#265195=CARTESIAN_POINT('Ctrl Pts',(42.439211691895,-57.4754524783491,-41.7602625));
#265196=CARTESIAN_POINT('Ctrl Pts',(42.4392116918951,-58.6698405167284,
-41.7019291666667));
#265197=CARTESIAN_POINT('Ctrl Pts',(43.4735820751078,-59.267034535918,-41.6435958333334));
#265198=CARTESIAN_POINT('Ctrl Pts',(44.5079524583205,-59.8642285551076,
-41.5852625));
#265199=CARTESIAN_POINT('Ctrl Pts',(45.5423228415332,-59.267034535918,-41.5269291666667));
#265200=CARTESIAN_POINT('Ctrl Pts',(46.5766932247459,-58.6698405167284,
-41.4685958333333));
#265201=CARTESIAN_POINT('Ctrl Pts',(46.5766932247459,-57.4754524783491,
-41.4102625));
#265202=CARTESIAN_POINT('Ctrl Pts',(46.5766932247459,-56.2810644399698,
-41.3519291666666));
#265203=CARTESIAN_POINT('Ctrl Pts',(45.5423228415332,-55.6838704207802,
-41.2935958333334));
#265204=CARTESIAN_POINT('Ctrl Pts',(44.5079524583205,-55.0866764015906,
-41.2352625));
#265205=CARTESIAN_POINT('Ctrl Pts',(43.4735820751078,-55.6838704207802,
-41.1769291666667));
#265206=CARTESIAN_POINT('Ctrl Pts',(42.4392116918951,-56.2810644399698,
-41.1185958333333));
#265207=CARTESIAN_POINT('Ctrl Pts',(42.439211691895,-57.4754524783491,-41.0602625));
#265208=CARTESIAN_POINT('Ctrl Pts',(42.4392116918951,-58.6698405167284,
-41.0019291666666));
#265209=CARTESIAN_POINT('Ctrl Pts',(43.4735820751078,-59.267034535918,-40.9435958333334));
#265210=CARTESIAN_POINT('Ctrl Pts',(44.5079524583205,-59.8642285551076,
-40.8852625));
#265211=CARTESIAN_POINT('Ctrl Pts',(45.5423228415332,-59.267034535918,-40.8269291666667));
#265212=CARTESIAN_POINT('Ctrl Pts',(46.5766932247459,-58.6698405167284,
-40.7685958333333));
#265213=CARTESIAN_POINT('Ctrl Pts',(46.5766932247459,-57.4754524783491,
-40.7102625));
#265214=CARTESIAN_POINT('Ctrl Pts',(46.5766932247459,-56.2810644399698,
-40.6519291666667));
#265215=CARTESIAN_POINT('Ctrl Pts',(45.5423228415332,-55.6838704207802,
-40.5935958333334));
#265216=CARTESIAN_POINT('Ctrl Pts',(44.5079524583205,-55.0866764015906,
-40.5352625));
#265217=CARTESIAN_POINT('Ctrl Pts',(43.4735820751078,-55.6838704207802,
-40.4769291666667));
#265218=CARTESIAN_POINT('Ctrl Pts',(42.4392116918951,-56.2810644399698,
-40.4185958333333));
#265219=CARTESIAN_POINT('Ctrl Pts',(42.439211691895,-57.4754524783491,-40.3602625));
#265220=CARTESIAN_POINT('Ctrl Pts',(42.4392116918951,-58.6698405167284,
-40.3019291666667));
#265221=CARTESIAN_POINT('Ctrl Pts',(43.4735820751078,-59.267034535918,-40.2435958333334));
#265222=CARTESIAN_POINT('Ctrl Pts',(44.5079524583205,-59.8642285551076,
-40.1852625));
#265223=CARTESIAN_POINT('Ctrl Pts',(45.5423228415332,-59.267034535918,-40.1269291666666));
#265224=CARTESIAN_POINT('Ctrl Pts',(46.5766932247459,-58.6698405167284,
-40.0685958333333));
#265225=CARTESIAN_POINT('Ctrl Pts',(46.5766932247459,-57.4754524783491,
-40.0102625));
#265226=CARTESIAN_POINT('Ctrl Pts',(46.5766932247459,-56.2810644399698,
-39.9519291666667));
#265227=CARTESIAN_POINT('Ctrl Pts',(45.5423228415332,-55.6838704207802,
-39.8935958333334));
#265228=CARTESIAN_POINT('Ctrl Pts',(44.5079524583205,-55.0866764015906,
-39.8352625));
#265229=CARTESIAN_POINT('Ctrl Pts',(43.4735820751078,-55.6838704207802,
-39.7769291666667));
#265230=CARTESIAN_POINT('Ctrl Pts',(42.4392116918951,-56.2810644399698,
-39.7185958333334));
#265231=CARTESIAN_POINT('Ctrl Pts',(42.439211691895,-57.4754524783491,-39.6602625));
#265232=CARTESIAN_POINT('Ctrl Pts',(42.4392116918951,-58.6698405167284,
-39.6019291666667));
#265233=CARTESIAN_POINT('Ctrl Pts',(43.4735820751078,-59.267034535918,-39.5435958333333));
#265234=CARTESIAN_POINT('Ctrl Pts',(44.5079524583205,-59.8642285551076,
-39.4852625));
#265235=CARTESIAN_POINT('Ctrl Pts',(45.5423228415332,-59.267034535918,-39.4269291666667));
#265236=CARTESIAN_POINT('Ctrl Pts',(46.5766932247459,-58.6698405167284,
-39.3685958333334));
#265237=CARTESIAN_POINT('Ctrl Pts',(46.5766932247459,-57.4754524783491,
-39.3102625));
#265238=CARTESIAN_POINT('Ctrl Pts',(46.5766932247459,-56.2810644399698,
-39.2519291666667));
#265239=CARTESIAN_POINT('Ctrl Pts',(45.5423228415332,-55.6838704207802,
-39.1935958333334));
#265240=CARTESIAN_POINT('Ctrl Pts',(44.5079524583205,-55.0866764015906,
-39.1352625));
#265241=CARTESIAN_POINT('Ctrl Pts',(43.4735820751078,-55.6838704207802,
-39.0769291666667));
#265242=CARTESIAN_POINT('Ctrl Pts',(42.4392116918951,-56.2810644399698,
-39.0185958333334));
#265243=CARTESIAN_POINT('Ctrl Pts',(42.439211691895,-57.4754524783491,-38.9602625));
#265244=CARTESIAN_POINT('Ctrl Pts',(42.4392116918951,-58.6698405167284,
-38.9019291666667));
#265245=CARTESIAN_POINT('Ctrl Pts',(43.4735820751078,-59.267034535918,-38.8435958333333));
#265246=CARTESIAN_POINT('Ctrl Pts',(44.5079524583205,-59.8642285551076,
-38.7852625));
#265247=CARTESIAN_POINT('Ctrl Pts',(45.5423228415332,-59.267034535918,-38.7269291666667));
#265248=CARTESIAN_POINT('Ctrl Pts',(46.5766932247459,-58.6698405167284,
-38.6685958333334));
#265249=CARTESIAN_POINT('Ctrl Pts',(46.5766932247459,-57.4754524783491,
-38.6102625));
#265250=CARTESIAN_POINT('Ctrl Pts',(46.5766932247459,-56.2810644399698,
-38.5519291666667));
#265251=CARTESIAN_POINT('Ctrl Pts',(45.5423228415332,-55.6838704207802,
-38.4935958333334));
#265252=CARTESIAN_POINT('Ctrl Pts',(44.5079524583205,-55.0866764015906,
-38.4352625));
#265253=CARTESIAN_POINT('Ctrl Pts',(43.4735820751078,-55.6838704207802,
-38.3769291666667));
#265254=CARTESIAN_POINT('Ctrl Pts',(42.4392116918951,-56.2810644399698,
-38.3185958333333));
#265255=CARTESIAN_POINT('Ctrl Pts',(42.439211691895,-57.4754524783491,-38.2602625));
#265256=CARTESIAN_POINT('Ctrl Pts',(42.4392116918951,-58.6698405167284,
-38.2019291666667));
#265257=CARTESIAN_POINT('Ctrl Pts',(43.4735820751078,-59.267034535918,-38.1435958333334));
#265258=CARTESIAN_POINT('Ctrl Pts',(44.5079524583205,-59.8642285551076,
-38.0852625));
#265259=CARTESIAN_POINT('Ctrl Pts',(45.5423228415332,-59.267034535918,-38.0269291666667));
#265260=CARTESIAN_POINT('Ctrl Pts',(46.5766932247459,-58.6698405167284,
-37.9685958333333));
#265261=CARTESIAN_POINT('Ctrl Pts',(46.5766932247459,-57.4754524783491,
-37.9102625));
#265262=CARTESIAN_POINT('Ctrl Pts',(46.5766932247459,-56.2810644399698,
-37.8519291666667));
#265263=CARTESIAN_POINT('Ctrl Pts',(45.5423228415332,-55.6838704207802,
-37.7935958333334));
#265264=CARTESIAN_POINT('Ctrl Pts',(44.5079524583205,-55.0866764015906,
-37.7352625));
#265265=CARTESIAN_POINT('Ctrl Pts',(43.4735820751078,-55.6838704207802,
-37.6769291666667));
#265266=CARTESIAN_POINT('Ctrl Pts',(42.4392116918951,-56.2810644399698,
-37.6185958333333));
#265267=CARTESIAN_POINT('Ctrl Pts',(42.439211691895,-57.4754524783491,-37.5602625));
#265268=CARTESIAN_POINT('Ctrl Pts',(42.4392116918951,-58.6698405167284,
-37.5019291666667));
#265269=CARTESIAN_POINT('Ctrl Pts',(43.4735820751078,-59.267034535918,-37.4435958333333));
#265270=CARTESIAN_POINT('Ctrl Pts',(44.5079524583205,-59.8642285551076,
-37.3852625));
#265271=CARTESIAN_POINT('Ctrl Pts',(45.5423228415332,-59.267034535918,-37.3269291666667));
#265272=CARTESIAN_POINT('Ctrl Pts',(46.5766932247459,-58.6698405167284,
-37.2685958333333));
#265273=CARTESIAN_POINT('Ctrl Pts',(46.5766932247459,-57.4754524783491,
-37.2102625));
#265274=CARTESIAN_POINT('Ctrl Pts',(46.5766932247459,-56.2810644399698,
-37.1519291666667));
#265275=CARTESIAN_POINT('Ctrl Pts',(45.5423228415332,-55.6838704207802,
-37.0935958333333));
#265276=CARTESIAN_POINT('Ctrl Pts',(44.5079524583205,-55.0866764015906,
-37.0352625));
#265277=CARTESIAN_POINT('Ctrl Pts',(43.4735820751078,-55.6838704207802,
-36.9769291666667));
#265278=CARTESIAN_POINT('Ctrl Pts',(42.4392116918951,-56.2810644399698,
-36.9185958333333));
#265279=CARTESIAN_POINT('Ctrl Pts',(42.439211691895,-57.4754524783491,-36.8602625));
#265280=CARTESIAN_POINT('Ctrl Pts',(42.4392116918951,-58.6698405167284,
-36.8019291666666));
#265281=CARTESIAN_POINT('Ctrl Pts',(43.4735820751078,-59.267034535918,-36.7435958333334));
#265282=CARTESIAN_POINT('Ctrl Pts',(44.5079524583205,-59.8642285551076,
-36.6852625));
#265283=CARTESIAN_POINT('Ctrl Pts',(45.5423228415332,-59.267034535918,-36.6269291666667));
#265284=CARTESIAN_POINT('Ctrl Pts',(45.6766051604217,-59.1895066029603,
-36.6193563132714));
#265285=CARTESIAN_POINT('Ctrl Pts',(45.7978303778615,-59.0928279175564,
-36.611216324118));
#265286=CARTESIAN_POINT('Ctrl Pts',(46.1766975979086,-57.4754524783491,
-52.8412000828291));
#265287=CARTESIAN_POINT('Ctrl Pts',(46.1766975979086,-56.512002022799,-52.7828667494958));
#265288=CARTESIAN_POINT('Ctrl Pts',(45.3423250281146,-56.0302767950239,
-52.7245334161625));
#265289=CARTESIAN_POINT('Ctrl Pts',(44.5079524583205,-55.5485515672488,
-52.6662000828291));
#265290=CARTESIAN_POINT('Ctrl Pts',(43.6735798885264,-56.0302767950239,
-52.6078667494958));
#265291=CARTESIAN_POINT('Ctrl Pts',(42.8392073187323,-56.5120020227989,
-52.5495334161624));
#265292=CARTESIAN_POINT('Ctrl Pts',(42.8392073187323,-57.4754524783491,
-52.4912000828291));
#265293=CARTESIAN_POINT('Ctrl Pts',(42.8392073187323,-58.4389029338992,
-52.4328667494959));
#265294=CARTESIAN_POINT('Ctrl Pts',(43.6735798885264,-58.9206281616743,
-52.3745334161625));
#265295=CARTESIAN_POINT('Ctrl Pts',(44.5079524583205,-59.4023533894493,
-52.3162000828292));
#265296=CARTESIAN_POINT('Ctrl Pts',(45.3423250281146,-58.9206281616743,
-52.2578667494958));
#265297=CARTESIAN_POINT('Ctrl Pts',(46.1766975979086,-58.4389029338992,
-52.1995334161625));
#265298=CARTESIAN_POINT('Ctrl Pts',(46.1766975979086,-57.4754524783491,
-52.1412000828291));
#265299=CARTESIAN_POINT('Ctrl Pts',(46.1766975979086,-56.512002022799,-52.0828667494958));
#265300=CARTESIAN_POINT('Ctrl Pts',(45.3423250281146,-56.0302767950239,
-52.0245334161624));
#265301=CARTESIAN_POINT('Ctrl Pts',(44.5079524583205,-55.5485515672488,
-51.9662000828291));
#265302=CARTESIAN_POINT('Ctrl Pts',(43.6735798885264,-56.0302767950239,
-51.9078667494958));
#265303=CARTESIAN_POINT('Ctrl Pts',(42.8392073187323,-56.5120020227989,
-51.8495334161625));
#265304=CARTESIAN_POINT('Ctrl Pts',(42.8392073187323,-57.4754524783491,
-51.7912000828291));
#265305=CARTESIAN_POINT('Ctrl Pts',(42.8392073187323,-58.4389029338992,
-51.7328667494958));
#265306=CARTESIAN_POINT('Ctrl Pts',(43.6735798885264,-58.9206281616743,
-51.6745334161625));
#265307=CARTESIAN_POINT('Ctrl Pts',(44.5079524583205,-59.4023533894493,
-51.6162000828291));
#265308=CARTESIAN_POINT('Ctrl Pts',(45.3423250281146,-58.9206281616743,
-51.5578667494958));
#265309=CARTESIAN_POINT('Ctrl Pts',(46.1766975979086,-58.4389029338992,
-51.4995334161625));
#265310=CARTESIAN_POINT('Ctrl Pts',(46.1766975979086,-57.4754524783491,
-51.4412000828291));
#265311=CARTESIAN_POINT('Ctrl Pts',(46.1766975979086,-56.512002022799,-51.3828667494958));
#265312=CARTESIAN_POINT('Ctrl Pts',(45.3423250281146,-56.0302767950239,
-51.3245334161625));
#265313=CARTESIAN_POINT('Ctrl Pts',(44.5079524583205,-55.5485515672488,
-51.2662000828291));
#265314=CARTESIAN_POINT('Ctrl Pts',(43.6735798885264,-56.0302767950239,
-51.2078667494958));
#265315=CARTESIAN_POINT('Ctrl Pts',(42.8392073187323,-56.5120020227989,
-51.1495334161625));
#265316=CARTESIAN_POINT('Ctrl Pts',(42.8392073187323,-57.4754524783491,
-51.0912000828291));
#265317=CARTESIAN_POINT('Ctrl Pts',(42.8392073187323,-58.4389029338992,
-51.0328667494958));
#265318=CARTESIAN_POINT('Ctrl Pts',(43.6735798885264,-58.9206281616743,
-50.9745334161624));
#265319=CARTESIAN_POINT('Ctrl Pts',(44.5079524583205,-59.4023533894493,
-50.9162000828291));
#265320=CARTESIAN_POINT('Ctrl Pts',(45.3423250281146,-58.9206281616743,
-50.8578667494958));
#265321=CARTESIAN_POINT('Ctrl Pts',(46.1766975979086,-58.4389029338992,
-50.7995334161625));
#265322=CARTESIAN_POINT('Ctrl Pts',(46.1766975979086,-57.4754524783491,
-50.7412000828291));
#265323=CARTESIAN_POINT('Ctrl Pts',(46.1766975979086,-56.512002022799,-50.6828667494958));
#265324=CARTESIAN_POINT('Ctrl Pts',(45.3423250281146,-56.0302767950239,
-50.6245334161624));
#265325=CARTESIAN_POINT('Ctrl Pts',(44.5079524583205,-55.5485515672488,
-50.5662000828291));
#265326=CARTESIAN_POINT('Ctrl Pts',(43.6735798885264,-56.0302767950239,
-50.5078667494958));
#265327=CARTESIAN_POINT('Ctrl Pts',(42.8392073187323,-56.5120020227989,
-50.4495334161625));
#265328=CARTESIAN_POINT('Ctrl Pts',(42.8392073187323,-57.4754524783491,
-50.3912000828291));
#265329=CARTESIAN_POINT('Ctrl Pts',(42.8392073187323,-58.4389029338992,
-50.3328667494958));
#265330=CARTESIAN_POINT('Ctrl Pts',(43.6735798885264,-58.9206281616743,
-50.2745334161625));
#265331=CARTESIAN_POINT('Ctrl Pts',(44.5079524583205,-59.4023533894493,
-50.2162000828292));
#265332=CARTESIAN_POINT('Ctrl Pts',(45.3423250281146,-58.9206281616743,
-50.1578667494958));
#265333=CARTESIAN_POINT('Ctrl Pts',(46.1766975979086,-58.4389029338992,
-50.0995334161625));
#265334=CARTESIAN_POINT('Ctrl Pts',(46.1766975979086,-57.4754524783491,
-50.0412000828291));
#265335=CARTESIAN_POINT('Ctrl Pts',(46.1766975979086,-56.512002022799,-49.9828667494958));
#265336=CARTESIAN_POINT('Ctrl Pts',(45.3423250281146,-56.0302767950239,
-49.9245334161625));
#265337=CARTESIAN_POINT('Ctrl Pts',(44.5079524583205,-55.5485515672488,
-49.8662000828292));
#265338=CARTESIAN_POINT('Ctrl Pts',(43.6735798885264,-56.0302767950239,
-49.8078667494958));
#265339=CARTESIAN_POINT('Ctrl Pts',(42.8392073187323,-56.5120020227989,
-49.7495334161624));
#265340=CARTESIAN_POINT('Ctrl Pts',(42.8392073187323,-57.4754524783491,
-49.6912000828291));
#265341=CARTESIAN_POINT('Ctrl Pts',(42.8392073187323,-58.4389029338992,
-49.6328667494958));
#265342=CARTESIAN_POINT('Ctrl Pts',(43.6735798885264,-58.9206281616743,
-49.5745334161625));
#265343=CARTESIAN_POINT('Ctrl Pts',(44.5079524583205,-59.4023533894493,
-49.5162000828292));
#265344=CARTESIAN_POINT('Ctrl Pts',(45.3423250281146,-58.9206281616743,
-49.4578667494958));
#265345=CARTESIAN_POINT('Ctrl Pts',(46.1766975979086,-58.4389029338992,
-49.3995334161625));
#265346=CARTESIAN_POINT('Ctrl Pts',(46.1766975979086,-57.4754524783491,
-49.3412000828291));
#265347=CARTESIAN_POINT('Ctrl Pts',(46.1766975979086,-56.512002022799,-49.2828667494958));
#265348=CARTESIAN_POINT('Ctrl Pts',(45.3423250281146,-56.0302767950239,
-49.2245334161625));
#265349=CARTESIAN_POINT('Ctrl Pts',(44.5079524583205,-55.5485515672488,
-49.1662000828291));
#265350=CARTESIAN_POINT('Ctrl Pts',(43.6735798885264,-56.0302767950239,
-49.1078667494958));
#265351=CARTESIAN_POINT('Ctrl Pts',(42.8392073187323,-56.5120020227989,
-49.0495334161625));
#265352=CARTESIAN_POINT('Ctrl Pts',(42.8392073187323,-57.4754524783491,
-48.9912000828291));
#265353=CARTESIAN_POINT('Ctrl Pts',(42.8392073187323,-58.4389029338992,
-48.9328667494958));
#265354=CARTESIAN_POINT('Ctrl Pts',(43.6735798885264,-58.9206281616743,
-48.8745334161625));
#265355=CARTESIAN_POINT('Ctrl Pts',(44.5079524583205,-59.4023533894493,
-48.8162000828292));
#265356=CARTESIAN_POINT('Ctrl Pts',(45.3423250281146,-58.9206281616743,
-48.7578667494958));
#265357=CARTESIAN_POINT('Ctrl Pts',(46.1766975979086,-58.4389029338992,
-48.6995334161625));
#265358=CARTESIAN_POINT('Ctrl Pts',(46.1766975979086,-57.4754524783491,
-48.6412000828291));
#265359=CARTESIAN_POINT('Ctrl Pts',(46.1766975979086,-56.512002022799,-48.5828667494958));
#265360=CARTESIAN_POINT('Ctrl Pts',(45.3423250281146,-56.0302767950239,
-48.5245334161625));
#265361=CARTESIAN_POINT('Ctrl Pts',(44.5079524583205,-55.5485515672488,
-48.4662000828292));
#265362=CARTESIAN_POINT('Ctrl Pts',(43.6735798885264,-56.0302767950239,
-48.4078667494958));
#265363=CARTESIAN_POINT('Ctrl Pts',(42.8392073187323,-56.5120020227989,
-48.3495334161625));
#265364=CARTESIAN_POINT('Ctrl Pts',(42.8392073187323,-57.4754524783491,
-48.2912000828291));
#265365=CARTESIAN_POINT('Ctrl Pts',(42.8392073187323,-58.4389029338992,
-48.2328667494958));
#265366=CARTESIAN_POINT('Ctrl Pts',(43.6735798885264,-58.9206281616743,
-48.1745334161625));
#265367=CARTESIAN_POINT('Ctrl Pts',(44.5079524583205,-59.4023533894493,
-48.1162000828291));
#265368=CARTESIAN_POINT('Ctrl Pts',(45.3423250281146,-58.9206281616743,
-48.0578667494958));
#265369=CARTESIAN_POINT('Ctrl Pts',(46.1766975979086,-58.4389029338992,
-47.9995334161625));
#265370=CARTESIAN_POINT('Ctrl Pts',(46.1766975979086,-57.4754524783491,
-47.9412000828291));
#265371=CARTESIAN_POINT('Ctrl Pts',(46.1766975979086,-56.512002022799,-47.8828667494958));
#265372=CARTESIAN_POINT('Ctrl Pts',(45.3423250281146,-56.0302767950239,
-47.8245334161624));
#265373=CARTESIAN_POINT('Ctrl Pts',(44.5079524583205,-55.5485515672488,
-47.7662000828292));
#265374=CARTESIAN_POINT('Ctrl Pts',(43.6735798885264,-56.0302767950239,
-47.7078667494958));
#265375=CARTESIAN_POINT('Ctrl Pts',(42.8392073187323,-56.5120020227989,
-47.6495334161625));
#265376=CARTESIAN_POINT('Ctrl Pts',(42.8392073187323,-57.4754524783491,
-47.5912000828291));
#265377=CARTESIAN_POINT('Ctrl Pts',(42.8392073187323,-58.4389029338992,
-47.5328667494958));
#265378=CARTESIAN_POINT('Ctrl Pts',(43.6735798885264,-58.9206281616743,
-47.4745334161625));
#265379=CARTESIAN_POINT('Ctrl Pts',(44.5079524583205,-59.4023533894493,
-47.4162000828291));
#265380=CARTESIAN_POINT('Ctrl Pts',(45.3423250281146,-58.9206281616743,
-47.3578667494958));
#265381=CARTESIAN_POINT('Ctrl Pts',(46.1766975979086,-58.4389029338992,
-47.2995334161625));
#265382=CARTESIAN_POINT('Ctrl Pts',(46.1766975979086,-57.4754524783491,
-47.2412000828291));
#265383=CARTESIAN_POINT('Ctrl Pts',(46.1766975979086,-56.512002022799,-47.1828667494958));
#265384=CARTESIAN_POINT('Ctrl Pts',(45.3423250281146,-56.0302767950239,
-47.1245334161624));
#265385=CARTESIAN_POINT('Ctrl Pts',(44.5079524583205,-55.5485515672488,
-47.0662000828291));
#265386=CARTESIAN_POINT('Ctrl Pts',(43.6735798885264,-56.0302767950239,
-47.0078667494958));
#265387=CARTESIAN_POINT('Ctrl Pts',(42.8392073187323,-56.5120020227989,
-46.9495334161625));
#265388=CARTESIAN_POINT('Ctrl Pts',(42.8392073187323,-57.4754524783491,
-46.8912000828291));
#265389=CARTESIAN_POINT('Ctrl Pts',(42.8392073187323,-58.4389029338992,
-46.8328667494958));
#265390=CARTESIAN_POINT('Ctrl Pts',(43.6735798885264,-58.9206281616743,
-46.7745334161625));
#265391=CARTESIAN_POINT('Ctrl Pts',(44.5079524583205,-59.4023533894493,
-46.7162000828291));
#265392=CARTESIAN_POINT('Ctrl Pts',(45.3423250281146,-58.9206281616743,
-46.6578667494958));
#265393=CARTESIAN_POINT('Ctrl Pts',(46.1766975979086,-58.4389029338992,
-46.5995334161625));
#265394=CARTESIAN_POINT('Ctrl Pts',(46.1766975979086,-57.4754524783491,
-46.5412000828291));
#265395=CARTESIAN_POINT('Ctrl Pts',(46.1766975979086,-56.512002022799,-46.4828667494958));
#265396=CARTESIAN_POINT('Ctrl Pts',(45.3423250281146,-56.0302767950239,
-46.4245334161625));
#265397=CARTESIAN_POINT('Ctrl Pts',(44.5079524583205,-55.5485515672488,
-46.3662000828291));
#265398=CARTESIAN_POINT('Ctrl Pts',(43.6735798885264,-56.0302767950239,
-46.3078667494958));
#265399=CARTESIAN_POINT('Ctrl Pts',(42.8392073187323,-56.5120020227989,
-46.2495334161625));
#265400=CARTESIAN_POINT('Ctrl Pts',(42.8392073187323,-57.4754524783491,
-46.1912000828291));
#265401=CARTESIAN_POINT('Ctrl Pts',(42.8392073187323,-58.4389029338992,
-46.1328667494958));
#265402=CARTESIAN_POINT('Ctrl Pts',(43.6735798885264,-58.9206281616743,
-46.0745334161625));
#265403=CARTESIAN_POINT('Ctrl Pts',(44.5079524583205,-59.4023533894493,
-46.0162000828291));
#265404=CARTESIAN_POINT('Ctrl Pts',(45.3423250281146,-58.9206281616743,
-45.9578667494958));
#265405=CARTESIAN_POINT('Ctrl Pts',(46.1766975979086,-58.4389029338992,
-45.8995334161624));
#265406=CARTESIAN_POINT('Ctrl Pts',(46.1766975979086,-57.4754524783491,
-45.8412000828291));
#265407=CARTESIAN_POINT('Ctrl Pts',(46.1766975979086,-56.512002022799,-45.7828667494958));
#265408=CARTESIAN_POINT('Ctrl Pts',(45.3423250281146,-56.0302767950239,
-45.7245334161624));
#265409=CARTESIAN_POINT('Ctrl Pts',(44.5079524583205,-55.5485515672488,
-45.6662000828291));
#265410=CARTESIAN_POINT('Ctrl Pts',(43.6735798885264,-56.0302767950239,
-45.6078667494958));
#265411=CARTESIAN_POINT('Ctrl Pts',(42.8392073187323,-56.5120020227989,
-45.5495334161625));
#265412=CARTESIAN_POINT('Ctrl Pts',(42.8392073187323,-57.4754524783491,
-45.4912000828291));
#265413=CARTESIAN_POINT('Ctrl Pts',(42.8392073187323,-58.4389029338992,
-45.4328667494958));
#265414=CARTESIAN_POINT('Ctrl Pts',(43.6735798885264,-58.9206281616743,
-45.3745334161625));
#265415=CARTESIAN_POINT('Ctrl Pts',(44.5079524583205,-59.4023533894493,
-45.3162000828292));
#265416=CARTESIAN_POINT('Ctrl Pts',(45.3423250281146,-58.9206281616743,
-45.2578667494958));
#265417=CARTESIAN_POINT('Ctrl Pts',(46.1766975979086,-58.4389029338992,
-45.1995334161625));
#265418=CARTESIAN_POINT('Ctrl Pts',(46.1766975979086,-57.4754524783491,
-45.1412000828291));
#265419=CARTESIAN_POINT('Ctrl Pts',(46.1766975979086,-56.512002022799,-45.0828667494958));
#265420=CARTESIAN_POINT('Ctrl Pts',(45.3423250281146,-56.0302767950239,
-45.0245334161625));
#265421=CARTESIAN_POINT('Ctrl Pts',(44.5079524583205,-55.5485515672488,
-44.9662000828292));
#265422=CARTESIAN_POINT('Ctrl Pts',(43.6735798885264,-56.0302767950239,
-44.9078667494958));
#265423=CARTESIAN_POINT('Ctrl Pts',(42.8392073187323,-56.5120020227989,
-44.8495334161625));
#265424=CARTESIAN_POINT('Ctrl Pts',(42.8392073187323,-57.4754524783491,
-44.7912000828291));
#265425=CARTESIAN_POINT('Ctrl Pts',(42.8392073187323,-58.4389029338992,
-44.7328667494958));
#265426=CARTESIAN_POINT('Ctrl Pts',(43.6735798885264,-58.9206281616743,
-44.6745334161625));
#265427=CARTESIAN_POINT('Ctrl Pts',(44.5079524583205,-59.4023533894493,
-44.6162000828292));
#265428=CARTESIAN_POINT('Ctrl Pts',(45.3423250281146,-58.9206281616743,
-44.5578667494959));
#265429=CARTESIAN_POINT('Ctrl Pts',(46.1766975979086,-58.4389029338992,
-44.4995334161625));
#265430=CARTESIAN_POINT('Ctrl Pts',(46.1766975979086,-57.4754524783491,
-44.4412000828291));
#265431=CARTESIAN_POINT('Ctrl Pts',(46.1766975979086,-56.512002022799,-44.3828667494958));
#265432=CARTESIAN_POINT('Ctrl Pts',(45.3423250281146,-56.0302767950239,
-44.3245334161625));
#265433=CARTESIAN_POINT('Ctrl Pts',(44.5079524583205,-55.5485515672488,
-44.2662000828292));
#265434=CARTESIAN_POINT('Ctrl Pts',(43.6735798885264,-56.0302767950239,
-44.2078667494958));
#265435=CARTESIAN_POINT('Ctrl Pts',(42.8392073187323,-56.5120020227989,
-44.1495334161625));
#265436=CARTESIAN_POINT('Ctrl Pts',(42.8392073187323,-57.4754524783491,
-44.0912000828291));
#265437=CARTESIAN_POINT('Ctrl Pts',(42.8392073187323,-58.4389029338992,
-44.0328667494958));
#265438=CARTESIAN_POINT('Ctrl Pts',(43.6735798885264,-58.9206281616743,
-43.9745334161625));
#265439=CARTESIAN_POINT('Ctrl Pts',(44.5079524583205,-59.4023533894493,
-43.9162000828292));
#265440=CARTESIAN_POINT('Ctrl Pts',(45.3423250281146,-58.9206281616743,
-43.8578667494958));
#265441=CARTESIAN_POINT('Ctrl Pts',(46.1766975979086,-58.4389029338992,
-43.7995334161625));
#265442=CARTESIAN_POINT('Ctrl Pts',(46.1766975979086,-57.4754524783491,
-43.7412000828291));
#265443=CARTESIAN_POINT('Ctrl Pts',(46.1766975979086,-56.512002022799,-43.6828667494958));
#265444=CARTESIAN_POINT('Ctrl Pts',(45.3423250281146,-56.0302767950239,
-43.6245334161625));
#265445=CARTESIAN_POINT('Ctrl Pts',(44.5079524583205,-55.5485515672488,
-43.5662000828292));
#265446=CARTESIAN_POINT('Ctrl Pts',(43.6735798885264,-56.0302767950239,
-43.5078667494958));
#265447=CARTESIAN_POINT('Ctrl Pts',(42.8392073187323,-56.5120020227989,
-43.4495334161625));
#265448=CARTESIAN_POINT('Ctrl Pts',(42.8392073187323,-57.4754524783491,
-43.3912000828291));
#265449=CARTESIAN_POINT('Ctrl Pts',(42.8392073187323,-58.4389029338992,
-43.3328667494958));
#265450=CARTESIAN_POINT('Ctrl Pts',(43.6735798885264,-58.9206281616743,
-43.2745334161625));
#265451=CARTESIAN_POINT('Ctrl Pts',(44.5079524583205,-59.4023533894493,
-43.2162000828292));
#265452=CARTESIAN_POINT('Ctrl Pts',(45.3423250281146,-58.9206281616743,
-43.1578667494958));
#265453=CARTESIAN_POINT('Ctrl Pts',(46.1766975979086,-58.4389029338992,
-43.0995334161625));
#265454=CARTESIAN_POINT('Ctrl Pts',(46.1766975979086,-57.4754524783491,
-43.0412000828291));
#265455=CARTESIAN_POINT('Ctrl Pts',(46.1766975979086,-56.512002022799,-42.9828667494958));
#265456=CARTESIAN_POINT('Ctrl Pts',(45.3423250281146,-56.0302767950239,
-42.9245334161625));
#265457=CARTESIAN_POINT('Ctrl Pts',(44.5079524583205,-55.5485515672488,
-42.8662000828291));
#265458=CARTESIAN_POINT('Ctrl Pts',(43.6735798885264,-56.0302767950239,
-42.8078667494958));
#265459=CARTESIAN_POINT('Ctrl Pts',(42.8392073187323,-56.5120020227989,
-42.7495334161625));
#265460=CARTESIAN_POINT('Ctrl Pts',(42.8392073187323,-57.4754524783491,
-42.6912000828291));
#265461=CARTESIAN_POINT('Ctrl Pts',(42.8392073187323,-58.4389029338992,
-42.6328667494958));
#265462=CARTESIAN_POINT('Ctrl Pts',(43.6735798885264,-58.9206281616743,
-42.5745334161625));
#265463=CARTESIAN_POINT('Ctrl Pts',(44.5079524583205,-59.4023533894493,
-42.5162000828291));
#265464=CARTESIAN_POINT('Ctrl Pts',(45.3423250281146,-58.9206281616743,
-42.4578667494958));
#265465=CARTESIAN_POINT('Ctrl Pts',(46.1766975979086,-58.4389029338992,
-42.3995334161625));
#265466=CARTESIAN_POINT('Ctrl Pts',(46.1766975979086,-57.4754524783491,
-42.3412000828291));
#265467=CARTESIAN_POINT('Ctrl Pts',(46.1766975979086,-56.512002022799,-42.2828667494958));
#265468=CARTESIAN_POINT('Ctrl Pts',(45.3423250281146,-56.0302767950239,
-42.2245334161625));
#265469=CARTESIAN_POINT('Ctrl Pts',(44.5079524583205,-55.5485515672488,
-42.1662000828291));
#265470=CARTESIAN_POINT('Ctrl Pts',(43.6735798885264,-56.0302767950239,
-42.1078667494958));
#265471=CARTESIAN_POINT('Ctrl Pts',(42.8392073187323,-56.5120020227989,
-42.0495334161625));
#265472=CARTESIAN_POINT('Ctrl Pts',(42.8392073187323,-57.4754524783491,
-41.9912000828291));
#265473=CARTESIAN_POINT('Ctrl Pts',(42.8392073187323,-58.4389029338992,
-41.9328667494958));
#265474=CARTESIAN_POINT('Ctrl Pts',(43.6735798885264,-58.9206281616743,
-41.8745334161625));
#265475=CARTESIAN_POINT('Ctrl Pts',(44.5079524583205,-59.4023533894493,
-41.8162000828291));
#265476=CARTESIAN_POINT('Ctrl Pts',(45.3423250281146,-58.9206281616743,
-41.7578667494958));
#265477=CARTESIAN_POINT('Ctrl Pts',(46.1766975979086,-58.4389029338992,
-41.6995334161625));
#265478=CARTESIAN_POINT('Ctrl Pts',(46.1766975979086,-57.4754524783491,
-41.6412000828291));
#265479=CARTESIAN_POINT('Ctrl Pts',(46.1766975979086,-56.512002022799,-41.5828667494958));
#265480=CARTESIAN_POINT('Ctrl Pts',(45.3423250281146,-56.0302767950239,
-41.5245334161625));
#265481=CARTESIAN_POINT('Ctrl Pts',(44.5079524583205,-55.5485515672488,
-41.4662000828291));
#265482=CARTESIAN_POINT('Ctrl Pts',(43.6735798885264,-56.0302767950239,
-41.4078667494958));
#265483=CARTESIAN_POINT('Ctrl Pts',(42.8392073187323,-56.5120020227989,
-41.3495334161625));
#265484=CARTESIAN_POINT('Ctrl Pts',(42.8392073187323,-57.4754524783491,
-41.2912000828291));
#265485=CARTESIAN_POINT('Ctrl Pts',(42.8392073187323,-58.4389029338992,
-41.2328667494958));
#265486=CARTESIAN_POINT('Ctrl Pts',(43.6735798885264,-58.9206281616743,
-41.1745334161625));
#265487=CARTESIAN_POINT('Ctrl Pts',(44.5079524583205,-59.4023533894493,
-41.1162000828291));
#265488=CARTESIAN_POINT('Ctrl Pts',(45.3423250281146,-58.9206281616743,
-41.0578667494958));
#265489=CARTESIAN_POINT('Ctrl Pts',(46.1766975979086,-58.4389029338992,
-40.9995334161624));
#265490=CARTESIAN_POINT('Ctrl Pts',(46.1766975979086,-57.4754524783491,
-40.9412000828291));
#265491=CARTESIAN_POINT('Ctrl Pts',(46.1766975979086,-56.512002022799,-40.8828667494959));
#265492=CARTESIAN_POINT('Ctrl Pts',(45.3423250281146,-56.0302767950239,
-40.8245334161625));
#265493=CARTESIAN_POINT('Ctrl Pts',(44.5079524583205,-55.5485515672488,
-40.7662000828291));
#265494=CARTESIAN_POINT('Ctrl Pts',(43.6735798885264,-56.0302767950239,
-40.7078667494958));
#265495=CARTESIAN_POINT('Ctrl Pts',(42.8392073187323,-56.5120020227989,
-40.6495334161625));
#265496=CARTESIAN_POINT('Ctrl Pts',(42.8392073187323,-57.4754524783491,
-40.5912000828291));
#265497=CARTESIAN_POINT('Ctrl Pts',(42.8392073187323,-58.4389029338992,
-40.5328667494958));
#265498=CARTESIAN_POINT('Ctrl Pts',(43.6735798885264,-58.9206281616743,
-40.4745334161625));
#265499=CARTESIAN_POINT('Ctrl Pts',(44.5079524583205,-59.4023533894493,
-40.4162000828291));
#265500=CARTESIAN_POINT('Ctrl Pts',(45.3423250281146,-58.9206281616743,
-40.3578667494958));
#265501=CARTESIAN_POINT('Ctrl Pts',(46.1766975979086,-58.4389029338992,
-40.2995334161625));
#265502=CARTESIAN_POINT('Ctrl Pts',(46.1766975979086,-57.4754524783491,
-40.2412000828291));
#265503=CARTESIAN_POINT('Ctrl Pts',(46.1766975979086,-56.512002022799,-40.1828667494958));
#265504=CARTESIAN_POINT('Ctrl Pts',(45.3423250281146,-56.0302767950239,
-40.1245334161625));
#265505=CARTESIAN_POINT('Ctrl Pts',(44.5079524583205,-55.5485515672488,
-40.0662000828292));
#265506=CARTESIAN_POINT('Ctrl Pts',(43.6735798885264,-56.0302767950239,
-40.0078667494958));
#265507=CARTESIAN_POINT('Ctrl Pts',(42.8392073187323,-56.5120020227989,
-39.9495334161625));
#265508=CARTESIAN_POINT('Ctrl Pts',(42.8392073187323,-57.4754524783491,
-39.8912000828291));
#265509=CARTESIAN_POINT('Ctrl Pts',(42.8392073187323,-58.4389029338992,
-39.8328667494958));
#265510=CARTESIAN_POINT('Ctrl Pts',(43.6735798885264,-58.9206281616743,
-39.7745334161625));
#265511=CARTESIAN_POINT('Ctrl Pts',(44.5079524583205,-59.4023533894493,
-39.7162000828292));
#265512=CARTESIAN_POINT('Ctrl Pts',(45.3423250281146,-58.9206281616743,
-39.6578667494958));
#265513=CARTESIAN_POINT('Ctrl Pts',(46.1766975979086,-58.4389029338992,
-39.5995334161625));
#265514=CARTESIAN_POINT('Ctrl Pts',(46.1766975979086,-57.4754524783491,
-39.5412000828291));
#265515=CARTESIAN_POINT('Ctrl Pts',(46.1766975979086,-56.512002022799,-39.4828667494958));
#265516=CARTESIAN_POINT('Ctrl Pts',(45.3423250281146,-56.0302767950239,
-39.4245334161625));
#265517=CARTESIAN_POINT('Ctrl Pts',(44.5079524583205,-55.5485515672488,
-39.3662000828292));
#265518=CARTESIAN_POINT('Ctrl Pts',(43.6735798885264,-56.0302767950239,
-39.3078667494958));
#265519=CARTESIAN_POINT('Ctrl Pts',(42.8392073187323,-56.5120020227989,
-39.2495334161625));
#265520=CARTESIAN_POINT('Ctrl Pts',(42.8392073187323,-57.4754524783491,
-39.1912000828291));
#265521=CARTESIAN_POINT('Ctrl Pts',(42.8392073187323,-58.4389029338992,
-39.1328667494958));
#265522=CARTESIAN_POINT('Ctrl Pts',(43.6735798885264,-58.9206281616743,
-39.0745334161625));
#265523=CARTESIAN_POINT('Ctrl Pts',(44.5079524583205,-59.4023533894493,
-39.0162000828292));
#265524=CARTESIAN_POINT('Ctrl Pts',(45.3423250281146,-58.9206281616743,
-38.9578667494958));
#265525=CARTESIAN_POINT('Ctrl Pts',(46.1766975979086,-58.4389029338992,
-38.8995334161625));
#265526=CARTESIAN_POINT('Ctrl Pts',(46.1766975979086,-57.4754524783491,
-38.8412000828291));
#265527=CARTESIAN_POINT('Ctrl Pts',(46.1766975979086,-56.512002022799,-38.7828667494958));
#265528=CARTESIAN_POINT('Ctrl Pts',(45.3423250281146,-56.0302767950239,
-38.7245334161625));
#265529=CARTESIAN_POINT('Ctrl Pts',(44.5079524583205,-55.5485515672488,
-38.6662000828292));
#265530=CARTESIAN_POINT('Ctrl Pts',(43.6735798885264,-56.0302767950239,
-38.6078667494958));
#265531=CARTESIAN_POINT('Ctrl Pts',(42.8392073187323,-56.5120020227989,
-38.5495334161625));
#265532=CARTESIAN_POINT('Ctrl Pts',(42.8392073187323,-57.4754524783491,
-38.4912000828291));
#265533=CARTESIAN_POINT('Ctrl Pts',(42.8392073187323,-58.4389029338992,
-38.4328667494958));
#265534=CARTESIAN_POINT('Ctrl Pts',(43.6735798885264,-58.9206281616743,
-38.3745334161625));
#265535=CARTESIAN_POINT('Ctrl Pts',(44.5079524583205,-59.4023533894493,
-38.3162000828291));
#265536=CARTESIAN_POINT('Ctrl Pts',(45.3423250281146,-58.9206281616743,
-38.2578667494958));
#265537=CARTESIAN_POINT('Ctrl Pts',(46.1766975979086,-58.4389029338992,
-38.1995334161625));
#265538=CARTESIAN_POINT('Ctrl Pts',(46.1766975979086,-57.4754524783491,
-38.1412000828291));
#265539=CARTESIAN_POINT('Ctrl Pts',(46.1766975979086,-56.512002022799,-38.0828667494958));
#265540=CARTESIAN_POINT('Ctrl Pts',(45.3423250281146,-56.0302767950239,
-38.0245334161625));
#265541=CARTESIAN_POINT('Ctrl Pts',(44.5079524583205,-55.5485515672488,
-37.9662000828292));
#265542=CARTESIAN_POINT('Ctrl Pts',(43.6735798885264,-56.0302767950239,
-37.9078667494958));
#265543=CARTESIAN_POINT('Ctrl Pts',(42.8392073187323,-56.5120020227989,
-37.8495334161625));
#265544=CARTESIAN_POINT('Ctrl Pts',(42.8392073187323,-57.4754524783491,
-37.7912000828291));
#265545=CARTESIAN_POINT('Ctrl Pts',(42.8392073187323,-58.4389029338992,
-37.7328667494958));
#265546=CARTESIAN_POINT('Ctrl Pts',(43.6735798885264,-58.9206281616743,
-37.6745334161625));
#265547=CARTESIAN_POINT('Ctrl Pts',(44.5079524583205,-59.4023533894493,
-37.6162000828292));
#265548=CARTESIAN_POINT('Ctrl Pts',(45.3423250281146,-58.9206281616743,
-37.5578667494958));
#265549=CARTESIAN_POINT('Ctrl Pts',(46.1766975979086,-58.4389029338992,
-37.4995334161625));
#265550=CARTESIAN_POINT('Ctrl Pts',(46.1766975979086,-57.4754524783491,
-37.4412000828291));
#265551=CARTESIAN_POINT('Ctrl Pts',(46.1766975979086,-56.512002022799,-37.3828667494958));
#265552=CARTESIAN_POINT('Ctrl Pts',(45.3423250281146,-56.0302767950239,
-37.3245334161625));
#265553=CARTESIAN_POINT('Ctrl Pts',(44.5079524583205,-55.5485515672488,
-37.2662000828291));
#265554=CARTESIAN_POINT('Ctrl Pts',(43.6735798885264,-56.0302767950239,
-37.2078667494958));
#265555=CARTESIAN_POINT('Ctrl Pts',(42.8392073187323,-56.5120020227989,
-37.1495334161625));
#265556=CARTESIAN_POINT('Ctrl Pts',(42.8392073187323,-57.4754524783491,
-37.0912000828291));
#265557=CARTESIAN_POINT('Ctrl Pts',(42.8392073187323,-58.4389029338992,
-37.0328667494958));
#265558=CARTESIAN_POINT('Ctrl Pts',(43.6735798885264,-58.9206281616743,
-36.9745334161625));
#265559=CARTESIAN_POINT('Ctrl Pts',(44.5079524583205,-59.4023533894493,
-36.9162000828291));
#265560=CARTESIAN_POINT('Ctrl Pts',(45.3423250281146,-58.9206281616743,
-36.8578667494958));
#265561=CARTESIAN_POINT('Ctrl Pts',(45.450643562082,-58.85809042693,-36.8502938961005));
#265562=CARTESIAN_POINT('Ctrl Pts',(45.5484296141971,-58.7801047803048,
-36.8421539069472));
#265563=CARTESIAN_POINT('Ctrl Pts',(43.0534153750531,-58.2933966653875,
-39.8341885847849));
#265564=CARTESIAN_POINT('Ctrl Pts',(43.0851788151522,-58.4442420125764,
-39.7972051715141));
#265565=CARTESIAN_POINT('Ctrl Pts',(43.1309616784702,-58.5915153842683,
-39.7576523687012));
#265566=CARTESIAN_POINT('Ctrl Pts',(43.247256036382,-58.8749728352147,-39.6755423546175));
#265567=CARTESIAN_POINT('Ctrl Pts',(43.3177680072758,-59.0111108306031,
-39.6330135942989));
#265568=CARTESIAN_POINT('Ctrl Pts',(43.3993758805278,-59.140102067276,-39.5898550959804));
#265569=CARTESIAN_POINT('Ctrl Pts',(46.1766977413729,-57.4754524783491,
-52.99995));
#265570=CARTESIAN_POINT('Ctrl Pts',(46.1766977413729,-56.5120019399699,
-52.9416166666667));
#265571=CARTESIAN_POINT('Ctrl Pts',(45.3423250998467,-56.0302766707802,
-52.8832833333334));
#265572=CARTESIAN_POINT('Ctrl Pts',(44.5079524583205,-55.5485514015906,
-52.82495));
#265573=CARTESIAN_POINT('Ctrl Pts',(43.6735798167943,-56.0302766707802,
-52.7666166666667));
#265574=CARTESIAN_POINT('Ctrl Pts',(42.839207175268,-56.5120019399698,-52.7082833333333));
#265575=CARTESIAN_POINT('Ctrl Pts',(42.839207175268,-57.4754524783491,-52.64995));
#265576=CARTESIAN_POINT('Ctrl Pts',(42.839207175268,-58.4389030167283,-52.5916166666666));
#265577=CARTESIAN_POINT('Ctrl Pts',(43.6735798167943,-58.920628285918,-52.5332833333334));
#265578=CARTESIAN_POINT('Ctrl Pts',(44.5079524583205,-59.4023535551075,
-52.4749500000001));
#265579=CARTESIAN_POINT('Ctrl Pts',(45.3423250998467,-58.920628285918,-52.4166166666667));
#265580=CARTESIAN_POINT('Ctrl Pts',(46.1766977413729,-58.4389030167283,
-52.3582833333334));
#265581=CARTESIAN_POINT('Ctrl Pts',(46.1766977413729,-57.4754524783491,
-52.29995));
#265582=CARTESIAN_POINT('Ctrl Pts',(46.1766977413729,-56.5120019399699,
-52.2416166666667));
#265583=CARTESIAN_POINT('Ctrl Pts',(45.3423250998467,-56.0302766707802,
-52.1832833333333));
#265584=CARTESIAN_POINT('Ctrl Pts',(44.5079524583205,-55.5485514015906,
-52.12495));
#265585=CARTESIAN_POINT('Ctrl Pts',(43.6735798167943,-56.0302766707802,
-52.0666166666667));
#265586=CARTESIAN_POINT('Ctrl Pts',(42.839207175268,-56.5120019399698,-52.0082833333333));
#265587=CARTESIAN_POINT('Ctrl Pts',(42.839207175268,-57.4754524783491,-51.94995));
#265588=CARTESIAN_POINT('Ctrl Pts',(42.839207175268,-58.4389030167283,-51.8916166666667));
#265589=CARTESIAN_POINT('Ctrl Pts',(43.6735798167943,-58.920628285918,-51.8332833333334));
#265590=CARTESIAN_POINT('Ctrl Pts',(44.5079524583205,-59.4023535551075,
-51.77495));
#265591=CARTESIAN_POINT('Ctrl Pts',(45.3423250998467,-58.920628285918,-51.7166166666667));
#265592=CARTESIAN_POINT('Ctrl Pts',(46.1766977413729,-58.4389030167283,
-51.6582833333333));
#265593=CARTESIAN_POINT('Ctrl Pts',(46.1766977413729,-57.4754524783491,
-51.59995));
#265594=CARTESIAN_POINT('Ctrl Pts',(46.1766977413729,-56.5120019399699,
-51.5416166666667));
#265595=CARTESIAN_POINT('Ctrl Pts',(45.3423250998467,-56.0302766707802,
-51.4832833333334));
#265596=CARTESIAN_POINT('Ctrl Pts',(44.5079524583205,-55.5485514015906,
-51.42495));
#265597=CARTESIAN_POINT('Ctrl Pts',(43.6735798167943,-56.0302766707802,
-51.3666166666667));
#265598=CARTESIAN_POINT('Ctrl Pts',(42.839207175268,-56.5120019399698,-51.3082833333333));
#265599=CARTESIAN_POINT('Ctrl Pts',(42.839207175268,-57.4754524783491,-51.24995));
#265600=CARTESIAN_POINT('Ctrl Pts',(42.839207175268,-58.4389030167283,-51.1916166666667));
#265601=CARTESIAN_POINT('Ctrl Pts',(43.6735798167943,-58.920628285918,-51.1332833333334));
#265602=CARTESIAN_POINT('Ctrl Pts',(44.5079524583205,-59.4023535551075,
-51.07495));
#265603=CARTESIAN_POINT('Ctrl Pts',(45.3423250998467,-58.920628285918,-51.0166166666667));
#265604=CARTESIAN_POINT('Ctrl Pts',(46.1766977413729,-58.4389030167283,
-50.9582833333334));
#265605=CARTESIAN_POINT('Ctrl Pts',(46.1766977413729,-57.4754524783491,
-50.89995));
#265606=CARTESIAN_POINT('Ctrl Pts',(46.1766977413729,-56.5120019399699,
-50.8416166666667));
#265607=CARTESIAN_POINT('Ctrl Pts',(45.3423250998467,-56.0302766707802,
-50.7832833333333));
#265608=CARTESIAN_POINT('Ctrl Pts',(44.5079524583205,-55.5485514015906,
-50.72495));
#265609=CARTESIAN_POINT('Ctrl Pts',(43.6735798167943,-56.0302766707802,
-50.6666166666667));
#265610=CARTESIAN_POINT('Ctrl Pts',(42.839207175268,-56.5120019399698,-50.6082833333334));
#265611=CARTESIAN_POINT('Ctrl Pts',(42.839207175268,-57.4754524783491,-50.54995));
#265612=CARTESIAN_POINT('Ctrl Pts',(42.839207175268,-58.4389030167283,-50.4916166666667));
#265613=CARTESIAN_POINT('Ctrl Pts',(43.6735798167943,-58.920628285918,-50.4332833333333));
#265614=CARTESIAN_POINT('Ctrl Pts',(44.5079524583205,-59.4023535551075,
-50.37495));
#265615=CARTESIAN_POINT('Ctrl Pts',(45.3423250998467,-58.920628285918,-50.3166166666667));
#265616=CARTESIAN_POINT('Ctrl Pts',(46.1766977413729,-58.4389030167283,
-50.2582833333334));
#265617=CARTESIAN_POINT('Ctrl Pts',(46.1766977413729,-57.4754524783491,
-50.19995));
#265618=CARTESIAN_POINT('Ctrl Pts',(46.1766977413729,-56.5120019399699,
-50.1416166666667));
#265619=CARTESIAN_POINT('Ctrl Pts',(45.3423250998467,-56.0302766707802,
-50.0832833333334));
#265620=CARTESIAN_POINT('Ctrl Pts',(44.5079524583205,-55.5485514015906,
-50.02495));
#265621=CARTESIAN_POINT('Ctrl Pts',(43.6735798167943,-56.0302766707802,
-49.9666166666667));
#265622=CARTESIAN_POINT('Ctrl Pts',(42.839207175268,-56.5120019399698,-49.9082833333334));
#265623=CARTESIAN_POINT('Ctrl Pts',(42.839207175268,-57.4754524783491,-49.84995));
#265624=CARTESIAN_POINT('Ctrl Pts',(42.839207175268,-58.4389030167283,-49.7916166666667));
#265625=CARTESIAN_POINT('Ctrl Pts',(43.6735798167943,-58.920628285918,-49.7332833333334));
#265626=CARTESIAN_POINT('Ctrl Pts',(44.5079524583205,-59.4023535551075,
-49.67495));
#265627=CARTESIAN_POINT('Ctrl Pts',(45.3423250998467,-58.920628285918,-49.6166166666667));
#265628=CARTESIAN_POINT('Ctrl Pts',(46.1766977413729,-58.4389030167283,
-49.5582833333334));
#265629=CARTESIAN_POINT('Ctrl Pts',(46.1766977413729,-57.4754524783491,
-49.49995));
#265630=CARTESIAN_POINT('Ctrl Pts',(46.1766977413729,-56.5120019399699,
-49.4416166666667));
#265631=CARTESIAN_POINT('Ctrl Pts',(45.3423250998467,-56.0302766707802,
-49.3832833333334));
#265632=CARTESIAN_POINT('Ctrl Pts',(44.5079524583205,-55.5485514015906,
-49.32495));
#265633=CARTESIAN_POINT('Ctrl Pts',(43.6735798167943,-56.0302766707802,
-49.2666166666667));
#265634=CARTESIAN_POINT('Ctrl Pts',(42.839207175268,-56.5120019399698,-49.2082833333334));
#265635=CARTESIAN_POINT('Ctrl Pts',(42.839207175268,-57.4754524783491,-49.14995));
#265636=CARTESIAN_POINT('Ctrl Pts',(42.839207175268,-58.4389030167283,-49.0916166666667));
#265637=CARTESIAN_POINT('Ctrl Pts',(43.6735798167943,-58.920628285918,-49.0332833333333));
#265638=CARTESIAN_POINT('Ctrl Pts',(44.5079524583205,-59.4023535551075,
-48.97495));
#265639=CARTESIAN_POINT('Ctrl Pts',(45.3423250998467,-58.920628285918,-48.9166166666667));
#265640=CARTESIAN_POINT('Ctrl Pts',(46.1766977413729,-58.4389030167283,
-48.8582833333333));
#265641=CARTESIAN_POINT('Ctrl Pts',(46.1766977413729,-57.4754524783491,
-48.79995));
#265642=CARTESIAN_POINT('Ctrl Pts',(46.1766977413729,-56.5120019399699,
-48.7416166666667));
#265643=CARTESIAN_POINT('Ctrl Pts',(45.3423250998467,-56.0302766707802,
-48.6832833333334));
#265644=CARTESIAN_POINT('Ctrl Pts',(44.5079524583205,-55.5485514015906,
-48.62495));
#265645=CARTESIAN_POINT('Ctrl Pts',(43.6735798167943,-56.0302766707802,
-48.5666166666667));
#265646=CARTESIAN_POINT('Ctrl Pts',(42.839207175268,-56.5120019399698,-48.5082833333334));
#265647=CARTESIAN_POINT('Ctrl Pts',(42.839207175268,-57.4754524783491,-48.44995));
#265648=CARTESIAN_POINT('Ctrl Pts',(42.839207175268,-58.4389030167283,-48.3916166666667));
#265649=CARTESIAN_POINT('Ctrl Pts',(43.6735798167943,-58.920628285918,-48.3332833333334));
#265650=CARTESIAN_POINT('Ctrl Pts',(44.5079524583205,-59.4023535551075,
-48.27495));
#265651=CARTESIAN_POINT('Ctrl Pts',(45.3423250998467,-58.920628285918,-48.2166166666667));
#265652=CARTESIAN_POINT('Ctrl Pts',(46.1766977413729,-58.4389030167283,
-48.1582833333334));
#265653=CARTESIAN_POINT('Ctrl Pts',(46.1766977413729,-57.4754524783491,
-48.09995));
#265654=CARTESIAN_POINT('Ctrl Pts',(46.1766977413729,-56.5120019399699,
-48.0416166666667));
#265655=CARTESIAN_POINT('Ctrl Pts',(45.3423250998467,-56.0302766707802,
-47.9832833333334));
#265656=CARTESIAN_POINT('Ctrl Pts',(44.5079524583205,-55.5485514015906,
-47.92495));
#265657=CARTESIAN_POINT('Ctrl Pts',(43.6735798167943,-56.0302766707802,
-47.8666166666667));
#265658=CARTESIAN_POINT('Ctrl Pts',(42.839207175268,-56.5120019399698,-47.8082833333333));
#265659=CARTESIAN_POINT('Ctrl Pts',(42.839207175268,-57.4754524783491,-47.74995));
#265660=CARTESIAN_POINT('Ctrl Pts',(42.839207175268,-58.4389030167283,-47.6916166666667));
#265661=CARTESIAN_POINT('Ctrl Pts',(43.6735798167943,-58.920628285918,-47.6332833333333));
#265662=CARTESIAN_POINT('Ctrl Pts',(44.5079524583205,-59.4023535551075,
-47.57495));
#265663=CARTESIAN_POINT('Ctrl Pts',(45.3423250998467,-58.920628285918,-47.5166166666667));
#265664=CARTESIAN_POINT('Ctrl Pts',(46.1766977413729,-58.4389030167283,
-47.4582833333333));
#265665=CARTESIAN_POINT('Ctrl Pts',(46.1766977413729,-57.4754524783491,
-47.39995));
#265666=CARTESIAN_POINT('Ctrl Pts',(46.1766977413729,-56.5120019399699,
-47.3416166666666));
#265667=CARTESIAN_POINT('Ctrl Pts',(45.3423250998467,-56.0302766707802,
-47.2832833333333));
#265668=CARTESIAN_POINT('Ctrl Pts',(44.5079524583205,-55.5485514015906,
-47.22495));
#265669=CARTESIAN_POINT('Ctrl Pts',(43.6735798167943,-56.0302766707802,
-47.1666166666667));
#265670=CARTESIAN_POINT('Ctrl Pts',(42.839207175268,-56.5120019399698,-47.1082833333333));
#265671=CARTESIAN_POINT('Ctrl Pts',(42.839207175268,-57.4754524783491,-47.04995));
#265672=CARTESIAN_POINT('Ctrl Pts',(42.839207175268,-58.4389030167283,-46.9916166666667));
#265673=CARTESIAN_POINT('Ctrl Pts',(43.6735798167943,-58.920628285918,-46.9332833333334));
#265674=CARTESIAN_POINT('Ctrl Pts',(44.5079524583205,-59.4023535551075,
-46.87495));
#265675=CARTESIAN_POINT('Ctrl Pts',(45.3423250998467,-58.920628285918,-46.8166166666667));
#265676=CARTESIAN_POINT('Ctrl Pts',(46.1766977413729,-58.4389030167283,
-46.7582833333333));
#265677=CARTESIAN_POINT('Ctrl Pts',(46.1766977413729,-57.4754524783491,
-46.69995));
#265678=CARTESIAN_POINT('Ctrl Pts',(46.1766977413729,-56.5120019399699,
-46.6416166666666));
#265679=CARTESIAN_POINT('Ctrl Pts',(45.3423250998467,-56.0302766707802,
-46.5832833333334));
#265680=CARTESIAN_POINT('Ctrl Pts',(44.5079524583205,-55.5485514015906,
-46.52495));
#265681=CARTESIAN_POINT('Ctrl Pts',(43.6735798167943,-56.0302766707802,
-46.4666166666667));
#265682=CARTESIAN_POINT('Ctrl Pts',(42.839207175268,-56.5120019399698,-46.4082833333333));
#265683=CARTESIAN_POINT('Ctrl Pts',(42.839207175268,-57.4754524783491,-46.34995));
#265684=CARTESIAN_POINT('Ctrl Pts',(42.839207175268,-58.4389030167283,-46.2916166666667));
#265685=CARTESIAN_POINT('Ctrl Pts',(43.6735798167943,-58.920628285918,-46.2332833333334));
#265686=CARTESIAN_POINT('Ctrl Pts',(44.5079524583205,-59.4023535551075,
-46.17495));
#265687=CARTESIAN_POINT('Ctrl Pts',(45.3423250998467,-58.920628285918,-46.1166166666667));
#265688=CARTESIAN_POINT('Ctrl Pts',(46.1766977413729,-58.4389030167283,
-46.0582833333333));
#265689=CARTESIAN_POINT('Ctrl Pts',(46.1766977413729,-57.4754524783491,
-45.99995));
#265690=CARTESIAN_POINT('Ctrl Pts',(46.1766977413729,-56.5120019399699,
-45.9416166666667));
#265691=CARTESIAN_POINT('Ctrl Pts',(45.3423250998467,-56.0302766707802,
-45.8832833333333));
#265692=CARTESIAN_POINT('Ctrl Pts',(44.5079524583205,-55.5485514015906,
-45.82495));
#265693=CARTESIAN_POINT('Ctrl Pts',(43.6735798167943,-56.0302766707802,
-45.7666166666667));
#265694=CARTESIAN_POINT('Ctrl Pts',(42.839207175268,-56.5120019399698,-45.7082833333333));
#265695=CARTESIAN_POINT('Ctrl Pts',(42.839207175268,-57.4754524783491,-45.64995));
#265696=CARTESIAN_POINT('Ctrl Pts',(42.839207175268,-58.4389030167283,-45.5916166666667));
#265697=CARTESIAN_POINT('Ctrl Pts',(43.6735798167943,-58.920628285918,-45.5332833333333));
#265698=CARTESIAN_POINT('Ctrl Pts',(44.5079524583205,-59.4023535551075,
-45.47495));
#265699=CARTESIAN_POINT('Ctrl Pts',(45.3423250998467,-58.920628285918,-45.4166166666667));
#265700=CARTESIAN_POINT('Ctrl Pts',(46.1766977413729,-58.4389030167283,
-45.3582833333333));
#265701=CARTESIAN_POINT('Ctrl Pts',(46.1766977413729,-57.4754524783491,
-45.29995));
#265702=CARTESIAN_POINT('Ctrl Pts',(46.1766977413729,-56.5120019399699,
-45.2416166666667));
#265703=CARTESIAN_POINT('Ctrl Pts',(45.3423250998467,-56.0302766707802,
-45.1832833333334));
#265704=CARTESIAN_POINT('Ctrl Pts',(44.5079524583205,-55.5485514015906,
-45.12495));
#265705=CARTESIAN_POINT('Ctrl Pts',(43.6735798167943,-56.0302766707802,
-45.0666166666667));
#265706=CARTESIAN_POINT('Ctrl Pts',(42.839207175268,-56.5120019399698,-45.0082833333334));
#265707=CARTESIAN_POINT('Ctrl Pts',(42.839207175268,-57.4754524783491,-44.94995));
#265708=CARTESIAN_POINT('Ctrl Pts',(42.839207175268,-58.4389030167283,-44.8916166666667));
#265709=CARTESIAN_POINT('Ctrl Pts',(43.6735798167943,-58.920628285918,-44.8332833333334));
#265710=CARTESIAN_POINT('Ctrl Pts',(44.5079524583205,-59.4023535551075,
-44.77495));
#265711=CARTESIAN_POINT('Ctrl Pts',(45.3423250998467,-58.920628285918,-44.7166166666667));
#265712=CARTESIAN_POINT('Ctrl Pts',(46.1766977413729,-58.4389030167283,
-44.6582833333334));
#265713=CARTESIAN_POINT('Ctrl Pts',(46.1766977413729,-57.4754524783491,
-44.59995));
#265714=CARTESIAN_POINT('Ctrl Pts',(46.1766977413729,-56.5120019399699,
-44.5416166666667));
#265715=CARTESIAN_POINT('Ctrl Pts',(45.3423250998467,-56.0302766707802,
-44.4832833333334));
#265716=CARTESIAN_POINT('Ctrl Pts',(44.5079524583205,-55.5485514015906,
-44.42495));
#265717=CARTESIAN_POINT('Ctrl Pts',(43.6735798167943,-56.0302766707802,
-44.3666166666667));
#265718=CARTESIAN_POINT('Ctrl Pts',(42.839207175268,-56.5120019399698,-44.3082833333334));
#265719=CARTESIAN_POINT('Ctrl Pts',(42.839207175268,-57.4754524783491,-44.24995));
#265720=CARTESIAN_POINT('Ctrl Pts',(42.839207175268,-58.4389030167283,-44.1916166666667));
#265721=CARTESIAN_POINT('Ctrl Pts',(43.6735798167943,-58.920628285918,-44.1332833333334));
#265722=CARTESIAN_POINT('Ctrl Pts',(44.5079524583205,-59.4023535551075,
-44.07495));
#265723=CARTESIAN_POINT('Ctrl Pts',(45.3423250998467,-58.920628285918,-44.0166166666667));
#265724=CARTESIAN_POINT('Ctrl Pts',(46.1766977413729,-58.4389030167283,
-43.9582833333334));
#265725=CARTESIAN_POINT('Ctrl Pts',(46.1766977413729,-57.4754524783491,
-43.89995));
#265726=CARTESIAN_POINT('Ctrl Pts',(46.1766977413729,-56.5120019399699,
-43.8416166666667));
#265727=CARTESIAN_POINT('Ctrl Pts',(45.3423250998467,-56.0302766707802,
-43.7832833333334));
#265728=CARTESIAN_POINT('Ctrl Pts',(44.5079524583205,-55.5485514015906,
-43.72495));
#265729=CARTESIAN_POINT('Ctrl Pts',(43.6735798167943,-56.0302766707802,
-43.6666166666667));
#265730=CARTESIAN_POINT('Ctrl Pts',(42.839207175268,-56.5120019399698,-43.6082833333333));
#265731=CARTESIAN_POINT('Ctrl Pts',(42.839207175268,-57.4754524783491,-43.54995));
#265732=CARTESIAN_POINT('Ctrl Pts',(42.839207175268,-58.4389030167283,-43.4916166666667));
#265733=CARTESIAN_POINT('Ctrl Pts',(43.6735798167943,-58.920628285918,-43.4332833333333));
#265734=CARTESIAN_POINT('Ctrl Pts',(44.5079524583205,-59.4023535551075,
-43.37495));
#265735=CARTESIAN_POINT('Ctrl Pts',(45.3423250998467,-58.920628285918,-43.3166166666667));
#265736=CARTESIAN_POINT('Ctrl Pts',(46.1766977413729,-58.4389030167283,
-43.2582833333333));
#265737=CARTESIAN_POINT('Ctrl Pts',(46.1766977413729,-57.4754524783491,
-43.19995));
#265738=CARTESIAN_POINT('Ctrl Pts',(46.1766977413729,-56.5120019399699,
-43.1416166666667));
#265739=CARTESIAN_POINT('Ctrl Pts',(45.3423250998467,-56.0302766707802,
-43.0832833333333));
#265740=CARTESIAN_POINT('Ctrl Pts',(44.5079524583205,-55.5485514015906,
-43.02495));
#265741=CARTESIAN_POINT('Ctrl Pts',(43.6735798167943,-56.0302766707802,
-42.9666166666667));
#265742=CARTESIAN_POINT('Ctrl Pts',(42.839207175268,-56.5120019399698,-42.9082833333333));
#265743=CARTESIAN_POINT('Ctrl Pts',(42.839207175268,-57.4754524783491,-42.84995));
#265744=CARTESIAN_POINT('Ctrl Pts',(42.839207175268,-58.4389030167283,-42.7916166666667));
#265745=CARTESIAN_POINT('Ctrl Pts',(43.6735798167943,-58.920628285918,-42.7332833333334));
#265746=CARTESIAN_POINT('Ctrl Pts',(44.5079524583205,-59.4023535551075,
-42.67495));
#265747=CARTESIAN_POINT('Ctrl Pts',(45.3423250998467,-58.920628285918,-42.6166166666667));
#265748=CARTESIAN_POINT('Ctrl Pts',(46.1766977413729,-58.4389030167283,
-42.5582833333333));
#265749=CARTESIAN_POINT('Ctrl Pts',(46.1766977413729,-57.4754524783491,
-42.49995));
#265750=CARTESIAN_POINT('Ctrl Pts',(46.1766977413729,-56.5120019399699,
-42.4416166666667));
#265751=CARTESIAN_POINT('Ctrl Pts',(45.3423250998467,-56.0302766707802,
-42.3832833333333));
#265752=CARTESIAN_POINT('Ctrl Pts',(44.5079524583205,-55.5485514015906,
-42.32495));
#265753=CARTESIAN_POINT('Ctrl Pts',(43.6735798167943,-56.0302766707802,
-42.2666166666667));
#265754=CARTESIAN_POINT('Ctrl Pts',(42.839207175268,-56.5120019399698,-42.2082833333333));
#265755=CARTESIAN_POINT('Ctrl Pts',(42.839207175268,-57.4754524783491,-42.14995));
#265756=CARTESIAN_POINT('Ctrl Pts',(42.839207175268,-58.4389030167283,-42.0916166666667));
#265757=CARTESIAN_POINT('Ctrl Pts',(43.6735798167943,-58.920628285918,-42.0332833333334));
#265758=CARTESIAN_POINT('Ctrl Pts',(44.5079524583205,-59.4023535551075,
-41.97495));
#265759=CARTESIAN_POINT('Ctrl Pts',(45.3423250998467,-58.920628285918,-41.9166166666667));
#265760=CARTESIAN_POINT('Ctrl Pts',(46.1766977413729,-58.4389030167283,
-41.8582833333333));
#265761=CARTESIAN_POINT('Ctrl Pts',(46.1766977413729,-57.4754524783491,
-41.79995));
#265762=CARTESIAN_POINT('Ctrl Pts',(46.1766977413729,-56.5120019399699,
-41.7416166666667));
#265763=CARTESIAN_POINT('Ctrl Pts',(45.3423250998467,-56.0302766707802,
-41.6832833333333));
#265764=CARTESIAN_POINT('Ctrl Pts',(44.5079524583205,-55.5485514015906,
-41.62495));
#265765=CARTESIAN_POINT('Ctrl Pts',(43.6735798167943,-56.0302766707802,
-41.5666166666667));
#265766=CARTESIAN_POINT('Ctrl Pts',(42.839207175268,-56.5120019399698,-41.5082833333334));
#265767=CARTESIAN_POINT('Ctrl Pts',(42.839207175268,-57.4754524783491,-41.44995));
#265768=CARTESIAN_POINT('Ctrl Pts',(42.839207175268,-58.4389030167283,-41.3916166666667));
#265769=CARTESIAN_POINT('Ctrl Pts',(43.6735798167943,-58.920628285918,-41.3332833333334));
#265770=CARTESIAN_POINT('Ctrl Pts',(44.5079524583205,-59.4023535551075,
-41.27495));
#265771=CARTESIAN_POINT('Ctrl Pts',(45.3423250998467,-58.920628285918,-41.2166166666667));
#265772=CARTESIAN_POINT('Ctrl Pts',(46.1766977413729,-58.4389030167283,
-41.1582833333333));
#265773=CARTESIAN_POINT('Ctrl Pts',(46.1766977413729,-57.4754524783491,
-41.09995));
#265774=CARTESIAN_POINT('Ctrl Pts',(46.1766977413729,-56.5120019399699,
-41.0416166666667));
#265775=CARTESIAN_POINT('Ctrl Pts',(45.3423250998467,-56.0302766707802,
-40.9832833333333));
#265776=CARTESIAN_POINT('Ctrl Pts',(44.5079524583205,-55.5485514015906,
-40.92495));
#265777=CARTESIAN_POINT('Ctrl Pts',(43.6735798167943,-56.0302766707802,
-40.8666166666667));
#265778=CARTESIAN_POINT('Ctrl Pts',(42.839207175268,-56.5120019399698,-40.8082833333334));
#265779=CARTESIAN_POINT('Ctrl Pts',(42.839207175268,-57.4754524783491,-40.74995));
#265780=CARTESIAN_POINT('Ctrl Pts',(42.839207175268,-58.4389030167283,-40.6916166666667));
#265781=CARTESIAN_POINT('Ctrl Pts',(43.6735798167943,-58.920628285918,-40.6332833333334));
#265782=CARTESIAN_POINT('Ctrl Pts',(44.5079524583205,-59.4023535551075,
-40.57495));
#265783=CARTESIAN_POINT('Ctrl Pts',(45.3423250998467,-58.920628285918,-40.5166166666667));
#265784=CARTESIAN_POINT('Ctrl Pts',(46.1766977413729,-58.4389030167283,
-40.4582833333333));
#265785=CARTESIAN_POINT('Ctrl Pts',(46.1766977413729,-57.4754524783491,
-40.39995));
#265786=CARTESIAN_POINT('Ctrl Pts',(46.1766977413729,-56.5120019399699,
-40.3416166666667));
#265787=CARTESIAN_POINT('Ctrl Pts',(45.3423250998467,-56.0302766707802,
-40.2832833333334));
#265788=CARTESIAN_POINT('Ctrl Pts',(44.5079524583205,-55.5485514015906,
-40.22495));
#265789=CARTESIAN_POINT('Ctrl Pts',(43.6735798167943,-56.0302766707802,
-40.1666166666667));
#265790=CARTESIAN_POINT('Ctrl Pts',(42.839207175268,-56.5120019399698,-40.1082833333334));
#265791=CARTESIAN_POINT('Ctrl Pts',(42.839207175268,-57.4754524783491,-40.04995));
#265792=CARTESIAN_POINT('Ctrl Pts',(42.839207175268,-58.4389030167283,-39.9916166666667));
#265793=CARTESIAN_POINT('Ctrl Pts',(43.6735798167943,-58.920628285918,-39.9332833333333));
#265794=CARTESIAN_POINT('Ctrl Pts',(44.5079524583205,-59.4023535551075,
-39.87495));
#265795=CARTESIAN_POINT('Ctrl Pts',(45.3423250998467,-58.920628285918,-39.8166166666667));
#265796=CARTESIAN_POINT('Ctrl Pts',(46.1766977413729,-58.4389030167283,
-39.7582833333334));
#265797=CARTESIAN_POINT('Ctrl Pts',(46.1766977413729,-57.4754524783491,
-39.69995));
#265798=CARTESIAN_POINT('Ctrl Pts',(46.1766977413729,-56.5120019399699,
-39.6416166666667));
#265799=CARTESIAN_POINT('Ctrl Pts',(45.3423250998467,-56.0302766707802,
-39.5832833333333));
#265800=CARTESIAN_POINT('Ctrl Pts',(44.5079524583205,-55.5485514015906,
-39.52495));
#265801=CARTESIAN_POINT('Ctrl Pts',(43.6735798167943,-56.0302766707802,
-39.4666166666667));
#265802=CARTESIAN_POINT('Ctrl Pts',(42.839207175268,-56.5120019399698,-39.4082833333334));
#265803=CARTESIAN_POINT('Ctrl Pts',(42.839207175268,-57.4754524783491,-39.34995));
#265804=CARTESIAN_POINT('Ctrl Pts',(42.839207175268,-58.4389030167283,-39.2916166666667));
#265805=CARTESIAN_POINT('Ctrl Pts',(43.6735798167943,-58.920628285918,-39.2332833333333));
#265806=CARTESIAN_POINT('Ctrl Pts',(44.5079524583205,-59.4023535551075,
-39.17495));
#265807=CARTESIAN_POINT('Ctrl Pts',(45.3423250998467,-58.920628285918,-39.1166166666667));
#265808=CARTESIAN_POINT('Ctrl Pts',(46.1766977413729,-58.4389030167283,
-39.0582833333334));
#265809=CARTESIAN_POINT('Ctrl Pts',(46.1766977413729,-57.4754524783491,
-38.99995));
#265810=CARTESIAN_POINT('Ctrl Pts',(46.1766977413729,-56.5120019399699,
-38.9416166666667));
#265811=CARTESIAN_POINT('Ctrl Pts',(45.3423250998467,-56.0302766707802,
-38.8832833333334));
#265812=CARTESIAN_POINT('Ctrl Pts',(44.5079524583205,-55.5485514015906,
-38.82495));
#265813=CARTESIAN_POINT('Ctrl Pts',(43.6735798167943,-56.0302766707802,
-38.7666166666667));
#265814=CARTESIAN_POINT('Ctrl Pts',(42.839207175268,-56.5120019399698,-38.7082833333334));
#265815=CARTESIAN_POINT('Ctrl Pts',(42.839207175268,-57.4754524783491,-38.64995));
#265816=CARTESIAN_POINT('Ctrl Pts',(42.839207175268,-58.4389030167283,-38.5916166666667));
#265817=CARTESIAN_POINT('Ctrl Pts',(43.6735798167943,-58.920628285918,-38.5332833333334));
#265818=CARTESIAN_POINT('Ctrl Pts',(44.5079524583205,-59.4023535551075,
-38.47495));
#265819=CARTESIAN_POINT('Ctrl Pts',(45.3423250998467,-58.920628285918,-38.4166166666667));
#265820=CARTESIAN_POINT('Ctrl Pts',(46.1766977413729,-58.4389030167283,
-38.3582833333333));
#265821=CARTESIAN_POINT('Ctrl Pts',(46.1766977413729,-57.4754524783491,
-38.29995));
#265822=CARTESIAN_POINT('Ctrl Pts',(46.1766977413729,-56.5120019399699,
-38.2416166666667));
#265823=CARTESIAN_POINT('Ctrl Pts',(45.3423250998467,-56.0302766707802,
-38.1832833333333));
#265824=CARTESIAN_POINT('Ctrl Pts',(44.5079524583205,-55.5485514015906,
-38.12495));
#265825=CARTESIAN_POINT('Ctrl Pts',(43.6735798167943,-56.0302766707802,
-38.0666166666667));
#265826=CARTESIAN_POINT('Ctrl Pts',(42.839207175268,-56.5120019399698,-38.0082833333333));
#265827=CARTESIAN_POINT('Ctrl Pts',(42.839207175268,-57.4754524783491,-37.94995));
#265828=CARTESIAN_POINT('Ctrl Pts',(42.839207175268,-58.4389030167283,-37.8916166666667));
#265829=CARTESIAN_POINT('Ctrl Pts',(43.6735798167943,-58.920628285918,-37.8332833333334));
#265830=CARTESIAN_POINT('Ctrl Pts',(44.5079524583205,-59.4023535551075,
-37.77495));
#265831=CARTESIAN_POINT('Ctrl Pts',(45.3423250998467,-58.920628285918,-37.7166166666667));
#265832=CARTESIAN_POINT('Ctrl Pts',(46.1766977413729,-58.4389030167283,
-37.6582833333333));
#265833=CARTESIAN_POINT('Ctrl Pts',(46.1766977413729,-57.4754524783491,
-37.59995));
#265834=CARTESIAN_POINT('Ctrl Pts',(46.1766977413729,-56.5120019399699,
-37.5416166666667));
#265835=CARTESIAN_POINT('Ctrl Pts',(45.3423250998467,-56.0302766707802,
-37.4832833333334));
#265836=CARTESIAN_POINT('Ctrl Pts',(44.5079524583205,-55.5485514015906,
-37.42495));
#265837=CARTESIAN_POINT('Ctrl Pts',(43.6735798167943,-56.0302766707802,
-37.3666166666667));
#265838=CARTESIAN_POINT('Ctrl Pts',(42.839207175268,-56.5120019399698,-37.3082833333333));
#265839=CARTESIAN_POINT('Ctrl Pts',(42.839207175268,-57.4754524783491,-37.24995));
#265840=CARTESIAN_POINT('Ctrl Pts',(42.839207175268,-58.4389030167283,-37.1916166666667));
#265841=CARTESIAN_POINT('Ctrl Pts',(43.6735798167943,-58.920628285918,-37.1332833333334));
#265842=CARTESIAN_POINT('Ctrl Pts',(44.5079524583205,-59.4023535551075,
-37.07495));
#265843=CARTESIAN_POINT('Ctrl Pts',(45.3423250998467,-58.920628285918,-37.0166166666667));
#265844=CARTESIAN_POINT('Ctrl Pts',(45.4506530446707,-58.8580851178131,
-37.0090431559831));
#265845=CARTESIAN_POINT('Ctrl Pts',(45.5484465834733,-58.7800914304091,
-37.0009024189827));
#265846=CARTESIAN_POINT('Ctrl Pts',(46.5766932247459,-57.4754524783491,
-53.2308875));
#265847=CARTESIAN_POINT('Ctrl Pts',(46.5766932247459,-56.2810644399698,
-53.1725541666667));
#265848=CARTESIAN_POINT('Ctrl Pts',(45.5423228415332,-55.6838704207802,
-53.1142208333334));
#265849=CARTESIAN_POINT('Ctrl Pts',(44.5079524583205,-55.0866764015906,
-53.0558875000001));
#265850=CARTESIAN_POINT('Ctrl Pts',(43.4735820751078,-55.6838704207802,
-52.9975541666667));
#265851=CARTESIAN_POINT('Ctrl Pts',(42.4392116918951,-56.2810644399698,
-52.9392208333334));
#265852=CARTESIAN_POINT('Ctrl Pts',(42.439211691895,-57.4754524783491,-52.8808875));
#265853=CARTESIAN_POINT('Ctrl Pts',(42.4392116918951,-58.6698405167284,
-52.8225541666667));
#265854=CARTESIAN_POINT('Ctrl Pts',(43.4735820751078,-59.267034535918,-52.7642208333334));
#265855=CARTESIAN_POINT('Ctrl Pts',(44.5079524583205,-59.8642285551076,
-52.7058875));
#265856=CARTESIAN_POINT('Ctrl Pts',(45.5423228415332,-59.267034535918,-52.6475541666667));
#265857=CARTESIAN_POINT('Ctrl Pts',(46.5766932247459,-58.6698405167284,
-52.5892208333333));
#265858=CARTESIAN_POINT('Ctrl Pts',(46.5766932247459,-57.4754524783491,
-52.5308875));
#265859=CARTESIAN_POINT('Ctrl Pts',(46.5766932247459,-56.2810644399698,
-52.4725541666667));
#265860=CARTESIAN_POINT('Ctrl Pts',(45.5423228415332,-55.6838704207802,
-52.4142208333334));
#265861=CARTESIAN_POINT('Ctrl Pts',(44.5079524583205,-55.0866764015906,
-52.3558875000001));
#265862=CARTESIAN_POINT('Ctrl Pts',(43.4735820751078,-55.6838704207802,
-52.2975541666667));
#265863=CARTESIAN_POINT('Ctrl Pts',(42.4392116918951,-56.2810644399698,
-52.2392208333334));
#265864=CARTESIAN_POINT('Ctrl Pts',(42.439211691895,-57.4754524783491,-52.1808875));
#265865=CARTESIAN_POINT('Ctrl Pts',(42.4392116918951,-58.6698405167284,
-52.1225541666667));
#265866=CARTESIAN_POINT('Ctrl Pts',(43.4735820751078,-59.267034535918,-52.0642208333334));
#265867=CARTESIAN_POINT('Ctrl Pts',(44.5079524583205,-59.8642285551076,
-52.0058875));
#265868=CARTESIAN_POINT('Ctrl Pts',(45.5423228415332,-59.267034535918,-51.9475541666667));
#265869=CARTESIAN_POINT('Ctrl Pts',(46.5766932247459,-58.6698405167284,
-51.8892208333334));
#265870=CARTESIAN_POINT('Ctrl Pts',(46.5766932247459,-57.4754524783491,
-51.8308875));
#265871=CARTESIAN_POINT('Ctrl Pts',(46.5766932247459,-56.2810644399698,
-51.7725541666667));
#265872=CARTESIAN_POINT('Ctrl Pts',(45.5423228415332,-55.6838704207802,
-51.7142208333334));
#265873=CARTESIAN_POINT('Ctrl Pts',(44.5079524583205,-55.0866764015906,
-51.6558875));
#265874=CARTESIAN_POINT('Ctrl Pts',(43.4735820751078,-55.6838704207802,
-51.5975541666667));
#265875=CARTESIAN_POINT('Ctrl Pts',(42.4392116918951,-56.2810644399698,
-51.5392208333333));
#265876=CARTESIAN_POINT('Ctrl Pts',(42.439211691895,-57.4754524783491,-51.4808875));
#265877=CARTESIAN_POINT('Ctrl Pts',(42.4392116918951,-58.6698405167284,
-51.4225541666667));
#265878=CARTESIAN_POINT('Ctrl Pts',(43.4735820751078,-59.267034535918,-51.3642208333334));
#265879=CARTESIAN_POINT('Ctrl Pts',(44.5079524583205,-59.8642285551076,
-51.3058875));
#265880=CARTESIAN_POINT('Ctrl Pts',(45.5423228415332,-59.267034535918,-51.2475541666667));
#265881=CARTESIAN_POINT('Ctrl Pts',(46.5766932247459,-58.6698405167284,
-51.1892208333334));
#265882=CARTESIAN_POINT('Ctrl Pts',(46.5766932247459,-57.4754524783491,
-51.1308875));
#265883=CARTESIAN_POINT('Ctrl Pts',(46.5766932247459,-56.2810644399698,
-51.0725541666667));
#265884=CARTESIAN_POINT('Ctrl Pts',(45.5423228415332,-55.6838704207802,
-51.0142208333334));
#265885=CARTESIAN_POINT('Ctrl Pts',(44.5079524583205,-55.0866764015906,
-50.9558875));
#265886=CARTESIAN_POINT('Ctrl Pts',(43.4735820751078,-55.6838704207802,
-50.8975541666667));
#265887=CARTESIAN_POINT('Ctrl Pts',(42.4392116918951,-56.2810644399698,
-50.8392208333333));
#265888=CARTESIAN_POINT('Ctrl Pts',(42.439211691895,-57.4754524783491,-50.7808875));
#265889=CARTESIAN_POINT('Ctrl Pts',(42.4392116918951,-58.6698405167284,
-50.7225541666667));
#265890=CARTESIAN_POINT('Ctrl Pts',(43.4735820751078,-59.267034535918,-50.6642208333333));
#265891=CARTESIAN_POINT('Ctrl Pts',(44.5079524583205,-59.8642285551076,
-50.6058875));
#265892=CARTESIAN_POINT('Ctrl Pts',(45.5423228415332,-59.267034535918,-50.5475541666667));
#265893=CARTESIAN_POINT('Ctrl Pts',(46.5766932247459,-58.6698405167284,
-50.4892208333333));
#265894=CARTESIAN_POINT('Ctrl Pts',(46.5766932247459,-57.4754524783491,
-50.4308875));
#265895=CARTESIAN_POINT('Ctrl Pts',(46.5766932247459,-56.2810644399698,
-50.3725541666667));
#265896=CARTESIAN_POINT('Ctrl Pts',(45.5423228415332,-55.6838704207802,
-50.3142208333334));
#265897=CARTESIAN_POINT('Ctrl Pts',(44.5079524583205,-55.0866764015906,
-50.2558875));
#265898=CARTESIAN_POINT('Ctrl Pts',(43.4735820751078,-55.6838704207802,
-50.1975541666667));
#265899=CARTESIAN_POINT('Ctrl Pts',(42.4392116918951,-56.2810644399698,
-50.1392208333333));
#265900=CARTESIAN_POINT('Ctrl Pts',(42.439211691895,-57.4754524783491,-50.0808875));
#265901=CARTESIAN_POINT('Ctrl Pts',(42.4392116918951,-58.6698405167284,
-50.0225541666667));
#265902=CARTESIAN_POINT('Ctrl Pts',(43.4735820751078,-59.267034535918,-49.9642208333334));
#265903=CARTESIAN_POINT('Ctrl Pts',(44.5079524583205,-59.8642285551076,
-49.9058875));
#265904=CARTESIAN_POINT('Ctrl Pts',(45.5423228415332,-59.267034535918,-49.8475541666667));
#265905=CARTESIAN_POINT('Ctrl Pts',(46.5766932247459,-58.6698405167284,
-49.7892208333333));
#265906=CARTESIAN_POINT('Ctrl Pts',(46.5766932247459,-57.4754524783491,
-49.7308875));
#265907=CARTESIAN_POINT('Ctrl Pts',(46.5766932247459,-56.2810644399698,
-49.6725541666667));
#265908=CARTESIAN_POINT('Ctrl Pts',(45.5423228415332,-55.6838704207802,
-49.6142208333334));
#265909=CARTESIAN_POINT('Ctrl Pts',(44.5079524583205,-55.0866764015906,
-49.5558875));
#265910=CARTESIAN_POINT('Ctrl Pts',(43.4735820751078,-55.6838704207802,
-49.4975541666667));
#265911=CARTESIAN_POINT('Ctrl Pts',(42.4392116918951,-56.2810644399698,
-49.4392208333333));
#265912=CARTESIAN_POINT('Ctrl Pts',(42.439211691895,-57.4754524783491,-49.3808875));
#265913=CARTESIAN_POINT('Ctrl Pts',(42.4392116918951,-58.6698405167284,
-49.3225541666667));
#265914=CARTESIAN_POINT('Ctrl Pts',(43.4735820751078,-59.267034535918,-49.2642208333334));
#265915=CARTESIAN_POINT('Ctrl Pts',(44.5079524583205,-59.8642285551076,
-49.2058875));
#265916=CARTESIAN_POINT('Ctrl Pts',(45.5423228415332,-59.267034535918,-49.1475541666667));
#265917=CARTESIAN_POINT('Ctrl Pts',(46.5766932247459,-58.6698405167284,
-49.0892208333333));
#265918=CARTESIAN_POINT('Ctrl Pts',(46.5766932247459,-57.4754524783491,
-49.0308875));
#265919=CARTESIAN_POINT('Ctrl Pts',(46.5766932247459,-56.2810644399698,
-48.9725541666667));
#265920=CARTESIAN_POINT('Ctrl Pts',(45.5423228415332,-55.6838704207802,
-48.9142208333334));
#265921=CARTESIAN_POINT('Ctrl Pts',(44.5079524583205,-55.0866764015906,
-48.8558875));
#265922=CARTESIAN_POINT('Ctrl Pts',(43.4735820751078,-55.6838704207802,
-48.7975541666667));
#265923=CARTESIAN_POINT('Ctrl Pts',(42.4392116918951,-56.2810644399698,
-48.7392208333334));
#265924=CARTESIAN_POINT('Ctrl Pts',(42.439211691895,-57.4754524783491,-48.6808875));
#265925=CARTESIAN_POINT('Ctrl Pts',(42.4392116918951,-58.6698405167284,
-48.6225541666667));
#265926=CARTESIAN_POINT('Ctrl Pts',(43.4735820751078,-59.267034535918,-48.5642208333334));
#265927=CARTESIAN_POINT('Ctrl Pts',(44.5079524583205,-59.8642285551076,
-48.5058875));
#265928=CARTESIAN_POINT('Ctrl Pts',(45.5423228415332,-59.267034535918,-48.4475541666667));
#265929=CARTESIAN_POINT('Ctrl Pts',(46.5766932247459,-58.6698405167284,
-48.3892208333334));
#265930=CARTESIAN_POINT('Ctrl Pts',(46.5766932247459,-57.4754524783491,
-48.3308875));
#265931=CARTESIAN_POINT('Ctrl Pts',(46.5766932247459,-56.2810644399698,
-48.2725541666667));
#265932=CARTESIAN_POINT('Ctrl Pts',(45.5423228415332,-55.6838704207802,
-48.2142208333334));
#265933=CARTESIAN_POINT('Ctrl Pts',(44.5079524583205,-55.0866764015906,
-48.1558875));
#265934=CARTESIAN_POINT('Ctrl Pts',(43.4735820751078,-55.6838704207802,
-48.0975541666667));
#265935=CARTESIAN_POINT('Ctrl Pts',(42.4392116918951,-56.2810644399698,
-48.0392208333334));
#265936=CARTESIAN_POINT('Ctrl Pts',(42.439211691895,-57.4754524783491,-47.9808875));
#265937=CARTESIAN_POINT('Ctrl Pts',(42.4392116918951,-58.6698405167284,
-47.9225541666667));
#265938=CARTESIAN_POINT('Ctrl Pts',(43.4735820751078,-59.267034535918,-47.8642208333334));
#265939=CARTESIAN_POINT('Ctrl Pts',(44.5079524583205,-59.8642285551076,
-47.8058875000001));
#265940=CARTESIAN_POINT('Ctrl Pts',(45.5423228415332,-59.267034535918,-47.7475541666667));
#265941=CARTESIAN_POINT('Ctrl Pts',(46.5766932247459,-58.6698405167284,
-47.6892208333334));
#265942=CARTESIAN_POINT('Ctrl Pts',(46.5766932247459,-57.4754524783491,
-47.6308875));
#265943=CARTESIAN_POINT('Ctrl Pts',(46.5766932247459,-56.2810644399698,
-47.5725541666667));
#265944=CARTESIAN_POINT('Ctrl Pts',(45.5423228415332,-55.6838704207802,
-47.5142208333333));
#265945=CARTESIAN_POINT('Ctrl Pts',(44.5079524583205,-55.0866764015906,
-47.4558875));
#265946=CARTESIAN_POINT('Ctrl Pts',(43.4735820751078,-55.6838704207802,
-47.3975541666667));
#265947=CARTESIAN_POINT('Ctrl Pts',(42.4392116918951,-56.2810644399698,
-47.3392208333334));
#265948=CARTESIAN_POINT('Ctrl Pts',(42.439211691895,-57.4754524783491,-47.2808875));
#265949=CARTESIAN_POINT('Ctrl Pts',(42.4392116918951,-58.6698405167284,
-47.2225541666667));
#265950=CARTESIAN_POINT('Ctrl Pts',(43.4735820751078,-59.267034535918,-47.1642208333334));
#265951=CARTESIAN_POINT('Ctrl Pts',(44.5079524583205,-59.8642285551076,
-47.1058875));
#265952=CARTESIAN_POINT('Ctrl Pts',(45.5423228415332,-59.267034535918,-47.0475541666667));
#265953=CARTESIAN_POINT('Ctrl Pts',(46.5766932247459,-58.6698405167284,
-46.9892208333334));
#265954=CARTESIAN_POINT('Ctrl Pts',(46.5766932247459,-57.4754524783491,
-46.9308875));
#265955=CARTESIAN_POINT('Ctrl Pts',(46.5766932247459,-56.2810644399698,
-46.8725541666667));
#265956=CARTESIAN_POINT('Ctrl Pts',(45.5423228415332,-55.6838704207802,
-46.8142208333334));
#265957=CARTESIAN_POINT('Ctrl Pts',(44.5079524583205,-55.0866764015906,
-46.7558875));
#265958=CARTESIAN_POINT('Ctrl Pts',(43.4735820751078,-55.6838704207802,
-46.6975541666667));
#265959=CARTESIAN_POINT('Ctrl Pts',(42.4392116918951,-56.2810644399698,
-46.6392208333334));
#265960=CARTESIAN_POINT('Ctrl Pts',(42.439211691895,-57.4754524783491,-46.5808875));
#265961=CARTESIAN_POINT('Ctrl Pts',(42.4392116918951,-58.6698405167284,
-46.5225541666667));
#265962=CARTESIAN_POINT('Ctrl Pts',(43.4735820751078,-59.267034535918,-46.4642208333334));
#265963=CARTESIAN_POINT('Ctrl Pts',(44.5079524583205,-59.8642285551076,
-46.4058875));
#265964=CARTESIAN_POINT('Ctrl Pts',(45.5423228415332,-59.267034535918,-46.3475541666667));
#265965=CARTESIAN_POINT('Ctrl Pts',(46.5766932247459,-58.6698405167284,
-46.2892208333334));
#265966=CARTESIAN_POINT('Ctrl Pts',(46.5766932247459,-57.4754524783491,
-46.2308875));
#265967=CARTESIAN_POINT('Ctrl Pts',(46.5766932247459,-56.2810644399698,
-46.1725541666667));
#265968=CARTESIAN_POINT('Ctrl Pts',(45.5423228415332,-55.6838704207802,
-46.1142208333334));
#265969=CARTESIAN_POINT('Ctrl Pts',(44.5079524583205,-55.0866764015906,
-46.0558875));
#265970=CARTESIAN_POINT('Ctrl Pts',(43.4735820751078,-55.6838704207802,
-45.9975541666667));
#265971=CARTESIAN_POINT('Ctrl Pts',(42.4392116918951,-56.2810644399698,
-45.9392208333333));
#265972=CARTESIAN_POINT('Ctrl Pts',(42.439211691895,-57.4754524783491,-45.8808875));
#265973=CARTESIAN_POINT('Ctrl Pts',(42.4392116918951,-58.6698405167284,
-45.8225541666667));
#265974=CARTESIAN_POINT('Ctrl Pts',(43.4735820751078,-59.267034535918,-45.7642208333334));
#265975=CARTESIAN_POINT('Ctrl Pts',(44.5079524583205,-59.8642285551076,
-45.7058875));
#265976=CARTESIAN_POINT('Ctrl Pts',(45.5423228415332,-59.267034535918,-45.6475541666667));
#265977=CARTESIAN_POINT('Ctrl Pts',(46.5766932247459,-58.6698405167284,
-45.5892208333334));
#265978=CARTESIAN_POINT('Ctrl Pts',(46.5766932247459,-57.4754524783491,
-45.5308875));
#265979=CARTESIAN_POINT('Ctrl Pts',(46.5766932247459,-56.2810644399698,
-45.4725541666667));
#265980=CARTESIAN_POINT('Ctrl Pts',(45.5423228415332,-55.6838704207802,
-45.4142208333334));
#265981=CARTESIAN_POINT('Ctrl Pts',(44.5079524583205,-55.0866764015906,
-45.3558875));
#265982=CARTESIAN_POINT('Ctrl Pts',(43.4735820751078,-55.6838704207802,
-45.2975541666667));
#265983=CARTESIAN_POINT('Ctrl Pts',(42.4392116918951,-56.2810644399698,
-45.2392208333333));
#265984=CARTESIAN_POINT('Ctrl Pts',(42.439211691895,-57.4754524783491,-45.1808875));
#265985=CARTESIAN_POINT('Ctrl Pts',(42.4392116918951,-58.6698405167284,
-45.1225541666667));
#265986=CARTESIAN_POINT('Ctrl Pts',(43.4735820751078,-59.267034535918,-45.0642208333334));
#265987=CARTESIAN_POINT('Ctrl Pts',(44.5079524583205,-59.8642285551076,
-45.0058875));
#265988=CARTESIAN_POINT('Ctrl Pts',(45.5423228415332,-59.267034535918,-44.9475541666667));
#265989=CARTESIAN_POINT('Ctrl Pts',(46.5766932247459,-58.6698405167284,
-44.8892208333333));
#265990=CARTESIAN_POINT('Ctrl Pts',(46.5766932247459,-57.4754524783491,
-44.8308875));
#265991=CARTESIAN_POINT('Ctrl Pts',(46.5766932247459,-56.2810644399698,
-44.7725541666667));
#265992=CARTESIAN_POINT('Ctrl Pts',(45.5423228415332,-55.6838704207802,
-44.7142208333334));
#265993=CARTESIAN_POINT('Ctrl Pts',(44.5079524583205,-55.0866764015906,
-44.6558875));
#265994=CARTESIAN_POINT('Ctrl Pts',(43.4735820751078,-55.6838704207802,
-44.5975541666667));
#265995=CARTESIAN_POINT('Ctrl Pts',(42.4392116918951,-56.2810644399698,
-44.5392208333333));
#265996=CARTESIAN_POINT('Ctrl Pts',(42.439211691895,-57.4754524783491,-44.4808875000001));
#265997=CARTESIAN_POINT('Ctrl Pts',(42.4392116918951,-58.6698405167284,
-44.4225541666667));
#265998=CARTESIAN_POINT('Ctrl Pts',(43.4735820751078,-59.267034535918,-44.3642208333333));
#265999=CARTESIAN_POINT('Ctrl Pts',(44.5079524583205,-59.8642285551076,
-44.3058875));
#266000=CARTESIAN_POINT('Ctrl Pts',(45.5423228415332,-59.267034535918,-44.2475541666667));
#266001=CARTESIAN_POINT('Ctrl Pts',(46.5766932247459,-58.6698405167284,
-44.1892208333334));
#266002=CARTESIAN_POINT('Ctrl Pts',(46.5766932247459,-57.4754524783491,
-44.1308875000001));
#266003=CARTESIAN_POINT('Ctrl Pts',(46.5766932247459,-56.2810644399698,
-44.0725541666667));
#266004=CARTESIAN_POINT('Ctrl Pts',(45.5423228415332,-55.6838704207802,
-44.0142208333334));
#266005=CARTESIAN_POINT('Ctrl Pts',(44.5079524583205,-55.0866764015906,
-43.9558875));
#266006=CARTESIAN_POINT('Ctrl Pts',(43.4735820751078,-55.6838704207802,
-43.8975541666667));
#266007=CARTESIAN_POINT('Ctrl Pts',(42.4392116918951,-56.2810644399698,
-43.8392208333333));
#266008=CARTESIAN_POINT('Ctrl Pts',(42.439211691895,-57.4754524783491,-43.7808875));
#266009=CARTESIAN_POINT('Ctrl Pts',(42.4392116918951,-58.6698405167284,
-43.7225541666667));
#266010=CARTESIAN_POINT('Ctrl Pts',(43.4735820751078,-59.267034535918,-43.6642208333334));
#266011=CARTESIAN_POINT('Ctrl Pts',(44.5079524583205,-59.8642285551076,
-43.6058875));
#266012=CARTESIAN_POINT('Ctrl Pts',(45.5423228415332,-59.267034535918,-43.5475541666667));
#266013=CARTESIAN_POINT('Ctrl Pts',(46.5766932247459,-58.6698405167284,
-43.4892208333333));
#266014=CARTESIAN_POINT('Ctrl Pts',(46.5766932247459,-57.4754524783491,
-43.4308875));
#266015=CARTESIAN_POINT('Ctrl Pts',(46.5766932247459,-56.2810644399698,
-43.3725541666667));
#266016=CARTESIAN_POINT('Ctrl Pts',(45.5423228415332,-55.6838704207802,
-43.3142208333334));
#266017=CARTESIAN_POINT('Ctrl Pts',(44.5079524583205,-55.0866764015906,
-43.2558875));
#266018=CARTESIAN_POINT('Ctrl Pts',(43.4735820751078,-55.6838704207802,
-43.1975541666667));
#266019=CARTESIAN_POINT('Ctrl Pts',(42.4392116918951,-56.2810644399698,
-43.1392208333334));
#266020=CARTESIAN_POINT('Ctrl Pts',(42.439211691895,-57.4754524783491,-43.0808875));
#266021=CARTESIAN_POINT('Ctrl Pts',(42.4392116918951,-58.6698405167284,
-43.0225541666667));
#266022=CARTESIAN_POINT('Ctrl Pts',(43.4735820751078,-59.267034535918,-42.9642208333334));
#266023=CARTESIAN_POINT('Ctrl Pts',(44.5079524583205,-59.8642285551076,
-42.9058875));
#266024=CARTESIAN_POINT('Ctrl Pts',(45.5423228415332,-59.267034535918,-42.8475541666667));
#266025=CARTESIAN_POINT('Ctrl Pts',(46.5766932247459,-58.6698405167284,
-42.7892208333334));
#266026=CARTESIAN_POINT('Ctrl Pts',(46.5766932247459,-57.4754524783491,
-42.7308875000001));
#266027=CARTESIAN_POINT('Ctrl Pts',(46.5766932247459,-56.2810644399698,
-42.6725541666667));
#266028=CARTESIAN_POINT('Ctrl Pts',(45.5423228415332,-55.6838704207802,
-42.6142208333334));
#266029=CARTESIAN_POINT('Ctrl Pts',(44.5079524583205,-55.0866764015906,
-42.5558875));
#266030=CARTESIAN_POINT('Ctrl Pts',(43.4735820751078,-55.6838704207802,
-42.4975541666667));
#266031=CARTESIAN_POINT('Ctrl Pts',(42.4392116918951,-56.2810644399698,
-42.4392208333334));
#266032=CARTESIAN_POINT('Ctrl Pts',(42.439211691895,-57.4754524783491,-42.3808875000001));
#266033=CARTESIAN_POINT('Ctrl Pts',(42.4392116918951,-58.6698405167284,
-42.3225541666667));
#266034=CARTESIAN_POINT('Ctrl Pts',(43.4735820751078,-59.267034535918,-42.2642208333334));
#266035=CARTESIAN_POINT('Ctrl Pts',(44.5079524583205,-59.8642285551076,
-42.2058875));
#266036=CARTESIAN_POINT('Ctrl Pts',(45.5423228415332,-59.267034535918,-42.1475541666667));
#266037=CARTESIAN_POINT('Ctrl Pts',(46.5766932247459,-58.6698405167284,
-42.0892208333334));
#266038=CARTESIAN_POINT('Ctrl Pts',(46.5766932247459,-57.4754524783491,
-42.0308875000001));
#266039=CARTESIAN_POINT('Ctrl Pts',(46.5766932247459,-56.2810644399698,
-41.9725541666667));
#266040=CARTESIAN_POINT('Ctrl Pts',(45.5423228415332,-55.6838704207802,
-41.9142208333334));
#266041=CARTESIAN_POINT('Ctrl Pts',(44.5079524583205,-55.0866764015906,
-41.8558875));
#266042=CARTESIAN_POINT('Ctrl Pts',(43.4735820751078,-55.6838704207802,
-41.7975541666667));
#266043=CARTESIAN_POINT('Ctrl Pts',(42.4392116918951,-56.2810644399698,
-41.7392208333334));
#266044=CARTESIAN_POINT('Ctrl Pts',(42.439211691895,-57.4754524783491,-41.6808875000001));
#266045=CARTESIAN_POINT('Ctrl Pts',(42.4392116918951,-58.6698405167284,
-41.6225541666667));
#266046=CARTESIAN_POINT('Ctrl Pts',(43.4735820751078,-59.267034535918,-41.5642208333334));
#266047=CARTESIAN_POINT('Ctrl Pts',(44.5079524583205,-59.8642285551076,
-41.5058875));
#266048=CARTESIAN_POINT('Ctrl Pts',(45.5423228415332,-59.267034535918,-41.4475541666667));
#266049=CARTESIAN_POINT('Ctrl Pts',(46.5766932247459,-58.6698405167284,
-41.3892208333334));
#266050=CARTESIAN_POINT('Ctrl Pts',(46.5766932247459,-57.4754524783491,
-41.3308875000001));
#266051=CARTESIAN_POINT('Ctrl Pts',(46.5766932247459,-56.2810644399698,
-41.2725541666667));
#266052=CARTESIAN_POINT('Ctrl Pts',(45.5423228415332,-55.6838704207802,
-41.2142208333333));
#266053=CARTESIAN_POINT('Ctrl Pts',(44.5079524583205,-55.0866764015906,
-41.1558875));
#266054=CARTESIAN_POINT('Ctrl Pts',(43.4735820751078,-55.6838704207802,
-41.0975541666667));
#266055=CARTESIAN_POINT('Ctrl Pts',(42.4392116918951,-56.2810644399698,
-41.0392208333333));
#266056=CARTESIAN_POINT('Ctrl Pts',(42.439211691895,-57.4754524783491,-40.9808875000001));
#266057=CARTESIAN_POINT('Ctrl Pts',(42.4392116918951,-58.6698405167284,
-40.9225541666667));
#266058=CARTESIAN_POINT('Ctrl Pts',(43.4735820751078,-59.267034535918,-40.8642208333334));
#266059=CARTESIAN_POINT('Ctrl Pts',(44.5079524583205,-59.8642285551076,
-40.8058875));
#266060=CARTESIAN_POINT('Ctrl Pts',(45.5423228415332,-59.267034535918,-40.7475541666667));
#266061=CARTESIAN_POINT('Ctrl Pts',(46.5766932247459,-58.6698405167284,
-40.6892208333333));
#266062=CARTESIAN_POINT('Ctrl Pts',(46.5766932247459,-57.4754524783491,
-40.6308875));
#266063=CARTESIAN_POINT('Ctrl Pts',(46.5766932247459,-56.2810644399698,
-40.5725541666667));
#266064=CARTESIAN_POINT('Ctrl Pts',(45.5423228415332,-55.6838704207802,
-40.5142208333333));
#266065=CARTESIAN_POINT('Ctrl Pts',(44.5079524583205,-55.0866764015906,
-40.4558875));
#266066=CARTESIAN_POINT('Ctrl Pts',(43.4735820751078,-55.6838704207802,
-40.3975541666667));
#266067=CARTESIAN_POINT('Ctrl Pts',(42.4392116918951,-56.2810644399698,
-40.3392208333333));
#266068=CARTESIAN_POINT('Ctrl Pts',(42.439211691895,-57.4754524783491,-40.2808875));
#266069=CARTESIAN_POINT('Ctrl Pts',(42.4392116918951,-58.6698405167284,
-40.2225541666667));
#266070=CARTESIAN_POINT('Ctrl Pts',(43.4735820751078,-59.267034535918,-40.1642208333333));
#266071=CARTESIAN_POINT('Ctrl Pts',(44.5079524583205,-59.8642285551076,
-40.1058875));
#266072=CARTESIAN_POINT('Ctrl Pts',(45.5423228415332,-59.267034535918,-40.0475541666667));
#266073=CARTESIAN_POINT('Ctrl Pts',(46.5766932247459,-58.6698405167284,
-39.9892208333333));
#266074=CARTESIAN_POINT('Ctrl Pts',(46.5766932247459,-57.4754524783491,
-39.9308875));
#266075=CARTESIAN_POINT('Ctrl Pts',(46.5766932247459,-56.2810644399698,
-39.8725541666667));
#266076=CARTESIAN_POINT('Ctrl Pts',(45.5423228415332,-55.6838704207802,
-39.8142208333334));
#266077=CARTESIAN_POINT('Ctrl Pts',(44.5079524583205,-55.0866764015906,
-39.7558875));
#266078=CARTESIAN_POINT('Ctrl Pts',(43.4735820751078,-55.6838704207802,
-39.6975541666667));
#266079=CARTESIAN_POINT('Ctrl Pts',(42.4392116918951,-56.2810644399698,
-39.6392208333334));
#266080=CARTESIAN_POINT('Ctrl Pts',(42.439211691895,-57.4754524783491,-39.5808875000001));
#266081=CARTESIAN_POINT('Ctrl Pts',(42.4392116918951,-58.6698405167284,
-39.5225541666667));
#266082=CARTESIAN_POINT('Ctrl Pts',(43.4735820751078,-59.267034535918,-39.4642208333333));
#266083=CARTESIAN_POINT('Ctrl Pts',(44.5079524583205,-59.8642285551076,
-39.4058875));
#266084=CARTESIAN_POINT('Ctrl Pts',(45.5423228415332,-59.267034535918,-39.3475541666667));
#266085=CARTESIAN_POINT('Ctrl Pts',(46.5766932247459,-58.6698405167284,
-39.2892208333334));
#266086=CARTESIAN_POINT('Ctrl Pts',(46.5766932247459,-57.4754524783491,
-39.2308875));
#266087=CARTESIAN_POINT('Ctrl Pts',(46.5766932247459,-56.2810644399698,
-39.1725541666667));
#266088=CARTESIAN_POINT('Ctrl Pts',(45.5423228415332,-55.6838704207802,
-39.1142208333333));
#266089=CARTESIAN_POINT('Ctrl Pts',(44.5079524583205,-55.0866764015906,
-39.0558875));
#266090=CARTESIAN_POINT('Ctrl Pts',(43.4735820751078,-55.6838704207802,
-38.9975541666667));
#266091=CARTESIAN_POINT('Ctrl Pts',(42.4392116918951,-56.2810644399698,
-38.9392208333334));
#266092=CARTESIAN_POINT('Ctrl Pts',(42.439211691895,-57.4754524783491,-38.8808875));
#266093=CARTESIAN_POINT('Ctrl Pts',(42.4392116918951,-58.6698405167284,
-38.8225541666667));
#266094=CARTESIAN_POINT('Ctrl Pts',(43.4735820751078,-59.267034535918,-38.7642208333333));
#266095=CARTESIAN_POINT('Ctrl Pts',(44.5079524583205,-59.8642285551076,
-38.7058875));
#266096=CARTESIAN_POINT('Ctrl Pts',(45.5423228415332,-59.267034535918,-38.6475541666667));
#266097=CARTESIAN_POINT('Ctrl Pts',(46.5766932247459,-58.6698405167284,
-38.5892208333334));
#266098=CARTESIAN_POINT('Ctrl Pts',(46.5766932247459,-57.4754524783491,
-38.5308875));
#266099=CARTESIAN_POINT('Ctrl Pts',(46.5766932247459,-56.2810644399698,
-38.4725541666667));
#266100=CARTESIAN_POINT('Ctrl Pts',(45.5423228415332,-55.6838704207802,
-38.4142208333334));
#266101=CARTESIAN_POINT('Ctrl Pts',(44.5079524583205,-55.0866764015906,
-38.3558875));
#266102=CARTESIAN_POINT('Ctrl Pts',(43.4735820751078,-55.6838704207802,
-38.2975541666667));
#266103=CARTESIAN_POINT('Ctrl Pts',(42.4392116918951,-56.2810644399698,
-38.2392208333333));
#266104=CARTESIAN_POINT('Ctrl Pts',(42.439211691895,-57.4754524783491,-38.1808875000001));
#266105=CARTESIAN_POINT('Ctrl Pts',(42.4392116918951,-58.6698405167284,
-38.1225541666667));
#266106=CARTESIAN_POINT('Ctrl Pts',(43.4735820751078,-59.267034535918,-38.0642208333334));
#266107=CARTESIAN_POINT('Ctrl Pts',(44.5079524583205,-59.8642285551076,
-38.0058875));
#266108=CARTESIAN_POINT('Ctrl Pts',(45.5423228415332,-59.267034535918,-37.9475541666667));
#266109=CARTESIAN_POINT('Ctrl Pts',(46.5766932247459,-58.6698405167284,
-37.8892208333334));
#266110=CARTESIAN_POINT('Ctrl Pts',(46.5766932247459,-57.4754524783491,
-37.8308875));
#266111=CARTESIAN_POINT('Ctrl Pts',(46.5766932247459,-56.2810644399698,
-37.7725541666667));
#266112=CARTESIAN_POINT('Ctrl Pts',(45.5423228415332,-55.6838704207802,
-37.7142208333333));
#266113=CARTESIAN_POINT('Ctrl Pts',(44.5079524583205,-55.0866764015906,
-37.6558875));
#266114=CARTESIAN_POINT('Ctrl Pts',(43.4735820751078,-55.6838704207802,
-37.5975541666667));
#266115=CARTESIAN_POINT('Ctrl Pts',(42.4392116918951,-56.2810644399698,
-37.5392208333334));
#266116=CARTESIAN_POINT('Ctrl Pts',(42.439211691895,-57.4754524783491,-37.4808875));
#266117=CARTESIAN_POINT('Ctrl Pts',(42.4392116918951,-58.6698405167284,
-37.4225541666667));
#266118=CARTESIAN_POINT('Ctrl Pts',(43.4735820751078,-59.267034535918,-37.3642208333333));
#266119=CARTESIAN_POINT('Ctrl Pts',(44.5079524583205,-59.8642285551076,
-37.3058875));
#266120=CARTESIAN_POINT('Ctrl Pts',(45.5423228415332,-59.267034535918,-37.2475541666667));
#266121=CARTESIAN_POINT('Ctrl Pts',(45.6766168155006,-59.1894998738974,
-37.239980655983));
#266122=CARTESIAN_POINT('Ctrl Pts',(45.7978513037526,-59.0928112286649,
-37.2318399189827));
#266123=CARTESIAN_POINT('Ctrl Pts',(45.2824537511366,-55.8755132365557,
-39.638597553055));
#266124=CARTESIAN_POINT('Ctrl Pts',(45.4486364499857,-55.938875190796,-39.6579429567418));
#266125=CARTESIAN_POINT('Ctrl Pts',(45.6046461036551,-56.0241879535461,
-39.6778552592192));
#266126=CARTESIAN_POINT('Ctrl Pts',(45.9008786079562,-56.2453730623026,
-39.7222494146269));
#266127=CARTESIAN_POINT('Ctrl Pts',(46.0363919947743,-56.3826287328891,
-39.7461336748472));
#266128=CARTESIAN_POINT('Ctrl Pts',(46.2521263249353,-56.6800261237718,
-39.7916412021743));
#266129=CARTESIAN_POINT('Ctrl Pts',(46.3350396458226,-56.8359257464262,
-39.8130825635204));
#266130=CARTESIAN_POINT('Ctrl Pts',(46.4613757977742,-57.1838034186047,
-39.8560922003017));
#266131=CARTESIAN_POINT('Ctrl Pts',(46.4991955457474,-57.3765422463827,
-39.8769823938147));
#266132=CARTESIAN_POINT('Ctrl Pts',(46.5057011933515,-57.57028764973,-39.8960556104567));
#266133=CARTESIAN_POINT('Ctrl Pts',(46.1766977413729,-57.4754524783491,
-52.99995));
#266134=CARTESIAN_POINT('Ctrl Pts',(46.1766977413729,-56.5120019399699,
-52.9416166666667));
#266135=CARTESIAN_POINT('Ctrl Pts',(45.3423250998467,-56.0302766707802,
-52.8832833333334));
#266136=CARTESIAN_POINT('Ctrl Pts',(44.5079524583205,-55.5485514015906,
-52.82495));
#266137=CARTESIAN_POINT('Ctrl Pts',(43.6735798167943,-56.0302766707802,
-52.7666166666667));
#266138=CARTESIAN_POINT('Ctrl Pts',(42.839207175268,-56.5120019399698,-52.7082833333333));
#266139=CARTESIAN_POINT('Ctrl Pts',(42.839207175268,-57.4754524783491,-52.64995));
#266140=CARTESIAN_POINT('Ctrl Pts',(42.839207175268,-58.4389030167283,-52.5916166666666));
#266141=CARTESIAN_POINT('Ctrl Pts',(43.6735798167943,-58.920628285918,-52.5332833333334));
#266142=CARTESIAN_POINT('Ctrl Pts',(44.5079524583205,-59.4023535551075,
-52.4749500000001));
#266143=CARTESIAN_POINT('Ctrl Pts',(45.3423250998467,-58.920628285918,-52.4166166666667));
#266144=CARTESIAN_POINT('Ctrl Pts',(46.1766977413729,-58.4389030167283,
-52.3582833333334));
#266145=CARTESIAN_POINT('Ctrl Pts',(46.1766977413729,-57.4754524783491,
-52.29995));
#266146=CARTESIAN_POINT('Ctrl Pts',(46.1766977413729,-56.5120019399699,
-52.2416166666667));
#266147=CARTESIAN_POINT('Ctrl Pts',(45.3423250998467,-56.0302766707802,
-52.1832833333333));
#266148=CARTESIAN_POINT('Ctrl Pts',(44.5079524583205,-55.5485514015906,
-52.12495));
#266149=CARTESIAN_POINT('Ctrl Pts',(43.6735798167943,-56.0302766707802,
-52.0666166666667));
#266150=CARTESIAN_POINT('Ctrl Pts',(42.839207175268,-56.5120019399698,-52.0082833333333));
#266151=CARTESIAN_POINT('Ctrl Pts',(42.839207175268,-57.4754524783491,-51.94995));
#266152=CARTESIAN_POINT('Ctrl Pts',(42.839207175268,-58.4389030167283,-51.8916166666667));
#266153=CARTESIAN_POINT('Ctrl Pts',(43.6735798167943,-58.920628285918,-51.8332833333334));
#266154=CARTESIAN_POINT('Ctrl Pts',(44.5079524583205,-59.4023535551075,
-51.77495));
#266155=CARTESIAN_POINT('Ctrl Pts',(45.3423250998467,-58.920628285918,-51.7166166666667));
#266156=CARTESIAN_POINT('Ctrl Pts',(46.1766977413729,-58.4389030167283,
-51.6582833333333));
#266157=CARTESIAN_POINT('Ctrl Pts',(46.1766977413729,-57.4754524783491,
-51.59995));
#266158=CARTESIAN_POINT('Ctrl Pts',(46.1766977413729,-56.5120019399699,
-51.5416166666667));
#266159=CARTESIAN_POINT('Ctrl Pts',(45.3423250998467,-56.0302766707802,
-51.4832833333334));
#266160=CARTESIAN_POINT('Ctrl Pts',(44.5079524583205,-55.5485514015906,
-51.42495));
#266161=CARTESIAN_POINT('Ctrl Pts',(43.6735798167943,-56.0302766707802,
-51.3666166666667));
#266162=CARTESIAN_POINT('Ctrl Pts',(42.839207175268,-56.5120019399698,-51.3082833333333));
#266163=CARTESIAN_POINT('Ctrl Pts',(42.839207175268,-57.4754524783491,-51.24995));
#266164=CARTESIAN_POINT('Ctrl Pts',(42.839207175268,-58.4389030167283,-51.1916166666667));
#266165=CARTESIAN_POINT('Ctrl Pts',(43.6735798167943,-58.920628285918,-51.1332833333334));
#266166=CARTESIAN_POINT('Ctrl Pts',(44.5079524583205,-59.4023535551075,
-51.07495));
#266167=CARTESIAN_POINT('Ctrl Pts',(45.3423250998467,-58.920628285918,-51.0166166666667));
#266168=CARTESIAN_POINT('Ctrl Pts',(46.1766977413729,-58.4389030167283,
-50.9582833333334));
#266169=CARTESIAN_POINT('Ctrl Pts',(46.1766977413729,-57.4754524783491,
-50.89995));
#266170=CARTESIAN_POINT('Ctrl Pts',(46.1766977413729,-56.5120019399699,
-50.8416166666667));
#266171=CARTESIAN_POINT('Ctrl Pts',(45.3423250998467,-56.0302766707802,
-50.7832833333333));
#266172=CARTESIAN_POINT('Ctrl Pts',(44.5079524583205,-55.5485514015906,
-50.72495));
#266173=CARTESIAN_POINT('Ctrl Pts',(43.6735798167943,-56.0302766707802,
-50.6666166666667));
#266174=CARTESIAN_POINT('Ctrl Pts',(42.839207175268,-56.5120019399698,-50.6082833333334));
#266175=CARTESIAN_POINT('Ctrl Pts',(42.839207175268,-57.4754524783491,-50.54995));
#266176=CARTESIAN_POINT('Ctrl Pts',(42.839207175268,-58.4389030167283,-50.4916166666667));
#266177=CARTESIAN_POINT('Ctrl Pts',(43.6735798167943,-58.920628285918,-50.4332833333333));
#266178=CARTESIAN_POINT('Ctrl Pts',(44.5079524583205,-59.4023535551075,
-50.37495));
#266179=CARTESIAN_POINT('Ctrl Pts',(45.3423250998467,-58.920628285918,-50.3166166666667));
#266180=CARTESIAN_POINT('Ctrl Pts',(46.1766977413729,-58.4389030167283,
-50.2582833333334));
#266181=CARTESIAN_POINT('Ctrl Pts',(46.1766977413729,-57.4754524783491,
-50.19995));
#266182=CARTESIAN_POINT('Ctrl Pts',(46.1766977413729,-56.5120019399699,
-50.1416166666667));
#266183=CARTESIAN_POINT('Ctrl Pts',(45.3423250998467,-56.0302766707802,
-50.0832833333334));
#266184=CARTESIAN_POINT('Ctrl Pts',(44.5079524583205,-55.5485514015906,
-50.02495));
#266185=CARTESIAN_POINT('Ctrl Pts',(43.6735798167943,-56.0302766707802,
-49.9666166666667));
#266186=CARTESIAN_POINT('Ctrl Pts',(42.839207175268,-56.5120019399698,-49.9082833333334));
#266187=CARTESIAN_POINT('Ctrl Pts',(42.839207175268,-57.4754524783491,-49.84995));
#266188=CARTESIAN_POINT('Ctrl Pts',(42.839207175268,-58.4389030167283,-49.7916166666667));
#266189=CARTESIAN_POINT('Ctrl Pts',(43.6735798167943,-58.920628285918,-49.7332833333334));
#266190=CARTESIAN_POINT('Ctrl Pts',(44.5079524583205,-59.4023535551075,
-49.67495));
#266191=CARTESIAN_POINT('Ctrl Pts',(45.3423250998467,-58.920628285918,-49.6166166666667));
#266192=CARTESIAN_POINT('Ctrl Pts',(46.1766977413729,-58.4389030167283,
-49.5582833333334));
#266193=CARTESIAN_POINT('Ctrl Pts',(46.1766977413729,-57.4754524783491,
-49.49995));
#266194=CARTESIAN_POINT('Ctrl Pts',(46.1766977413729,-56.5120019399699,
-49.4416166666667));
#266195=CARTESIAN_POINT('Ctrl Pts',(45.3423250998467,-56.0302766707802,
-49.3832833333334));
#266196=CARTESIAN_POINT('Ctrl Pts',(44.5079524583205,-55.5485514015906,
-49.32495));
#266197=CARTESIAN_POINT('Ctrl Pts',(43.6735798167943,-56.0302766707802,
-49.2666166666667));
#266198=CARTESIAN_POINT('Ctrl Pts',(42.839207175268,-56.5120019399698,-49.2082833333334));
#266199=CARTESIAN_POINT('Ctrl Pts',(42.839207175268,-57.4754524783491,-49.14995));
#266200=CARTESIAN_POINT('Ctrl Pts',(42.839207175268,-58.4389030167283,-49.0916166666667));
#266201=CARTESIAN_POINT('Ctrl Pts',(43.6735798167943,-58.920628285918,-49.0332833333333));
#266202=CARTESIAN_POINT('Ctrl Pts',(44.5079524583205,-59.4023535551075,
-48.97495));
#266203=CARTESIAN_POINT('Ctrl Pts',(45.3423250998467,-58.920628285918,-48.9166166666667));
#266204=CARTESIAN_POINT('Ctrl Pts',(46.1766977413729,-58.4389030167283,
-48.8582833333333));
#266205=CARTESIAN_POINT('Ctrl Pts',(46.1766977413729,-57.4754524783491,
-48.79995));
#266206=CARTESIAN_POINT('Ctrl Pts',(46.1766977413729,-56.5120019399699,
-48.7416166666667));
#266207=CARTESIAN_POINT('Ctrl Pts',(45.3423250998467,-56.0302766707802,
-48.6832833333334));
#266208=CARTESIAN_POINT('Ctrl Pts',(44.5079524583205,-55.5485514015906,
-48.62495));
#266209=CARTESIAN_POINT('Ctrl Pts',(43.6735798167943,-56.0302766707802,
-48.5666166666667));
#266210=CARTESIAN_POINT('Ctrl Pts',(42.839207175268,-56.5120019399698,-48.5082833333334));
#266211=CARTESIAN_POINT('Ctrl Pts',(42.839207175268,-57.4754524783491,-48.44995));
#266212=CARTESIAN_POINT('Ctrl Pts',(42.839207175268,-58.4389030167283,-48.3916166666667));
#266213=CARTESIAN_POINT('Ctrl Pts',(43.6735798167943,-58.920628285918,-48.3332833333334));
#266214=CARTESIAN_POINT('Ctrl Pts',(44.5079524583205,-59.4023535551075,
-48.27495));
#266215=CARTESIAN_POINT('Ctrl Pts',(45.3423250998467,-58.920628285918,-48.2166166666667));
#266216=CARTESIAN_POINT('Ctrl Pts',(46.1766977413729,-58.4389030167283,
-48.1582833333334));
#266217=CARTESIAN_POINT('Ctrl Pts',(46.1766977413729,-57.4754524783491,
-48.09995));
#266218=CARTESIAN_POINT('Ctrl Pts',(46.1766977413729,-56.5120019399699,
-48.0416166666667));
#266219=CARTESIAN_POINT('Ctrl Pts',(45.3423250998467,-56.0302766707802,
-47.9832833333334));
#266220=CARTESIAN_POINT('Ctrl Pts',(44.5079524583205,-55.5485514015906,
-47.92495));
#266221=CARTESIAN_POINT('Ctrl Pts',(43.6735798167943,-56.0302766707802,
-47.8666166666667));
#266222=CARTESIAN_POINT('Ctrl Pts',(42.839207175268,-56.5120019399698,-47.8082833333333));
#266223=CARTESIAN_POINT('Ctrl Pts',(42.839207175268,-57.4754524783491,-47.74995));
#266224=CARTESIAN_POINT('Ctrl Pts',(42.839207175268,-58.4389030167283,-47.6916166666667));
#266225=CARTESIAN_POINT('Ctrl Pts',(43.6735798167943,-58.920628285918,-47.6332833333333));
#266226=CARTESIAN_POINT('Ctrl Pts',(44.5079524583205,-59.4023535551075,
-47.57495));
#266227=CARTESIAN_POINT('Ctrl Pts',(45.3423250998467,-58.920628285918,-47.5166166666667));
#266228=CARTESIAN_POINT('Ctrl Pts',(46.1766977413729,-58.4389030167283,
-47.4582833333333));
#266229=CARTESIAN_POINT('Ctrl Pts',(46.1766977413729,-57.4754524783491,
-47.39995));
#266230=CARTESIAN_POINT('Ctrl Pts',(46.1766977413729,-56.5120019399699,
-47.3416166666666));
#266231=CARTESIAN_POINT('Ctrl Pts',(45.3423250998467,-56.0302766707802,
-47.2832833333333));
#266232=CARTESIAN_POINT('Ctrl Pts',(44.5079524583205,-55.5485514015906,
-47.22495));
#266233=CARTESIAN_POINT('Ctrl Pts',(43.6735798167943,-56.0302766707802,
-47.1666166666667));
#266234=CARTESIAN_POINT('Ctrl Pts',(42.839207175268,-56.5120019399698,-47.1082833333333));
#266235=CARTESIAN_POINT('Ctrl Pts',(42.839207175268,-57.4754524783491,-47.04995));
#266236=CARTESIAN_POINT('Ctrl Pts',(42.839207175268,-58.4389030167283,-46.9916166666667));
#266237=CARTESIAN_POINT('Ctrl Pts',(43.6735798167943,-58.920628285918,-46.9332833333334));
#266238=CARTESIAN_POINT('Ctrl Pts',(44.5079524583205,-59.4023535551075,
-46.87495));
#266239=CARTESIAN_POINT('Ctrl Pts',(45.3423250998467,-58.920628285918,-46.8166166666667));
#266240=CARTESIAN_POINT('Ctrl Pts',(46.1766977413729,-58.4389030167283,
-46.7582833333333));
#266241=CARTESIAN_POINT('Ctrl Pts',(46.1766977413729,-57.4754524783491,
-46.69995));
#266242=CARTESIAN_POINT('Ctrl Pts',(46.1766977413729,-56.5120019399699,
-46.6416166666666));
#266243=CARTESIAN_POINT('Ctrl Pts',(45.3423250998467,-56.0302766707802,
-46.5832833333334));
#266244=CARTESIAN_POINT('Ctrl Pts',(44.5079524583205,-55.5485514015906,
-46.52495));
#266245=CARTESIAN_POINT('Ctrl Pts',(43.6735798167943,-56.0302766707802,
-46.4666166666667));
#266246=CARTESIAN_POINT('Ctrl Pts',(42.839207175268,-56.5120019399698,-46.4082833333333));
#266247=CARTESIAN_POINT('Ctrl Pts',(42.839207175268,-57.4754524783491,-46.34995));
#266248=CARTESIAN_POINT('Ctrl Pts',(42.839207175268,-58.4389030167283,-46.2916166666667));
#266249=CARTESIAN_POINT('Ctrl Pts',(43.6735798167943,-58.920628285918,-46.2332833333334));
#266250=CARTESIAN_POINT('Ctrl Pts',(44.5079524583205,-59.4023535551075,
-46.17495));
#266251=CARTESIAN_POINT('Ctrl Pts',(45.3423250998467,-58.920628285918,-46.1166166666667));
#266252=CARTESIAN_POINT('Ctrl Pts',(46.1766977413729,-58.4389030167283,
-46.0582833333333));
#266253=CARTESIAN_POINT('Ctrl Pts',(46.1766977413729,-57.4754524783491,
-45.99995));
#266254=CARTESIAN_POINT('Ctrl Pts',(46.1766977413729,-56.5120019399699,
-45.9416166666667));
#266255=CARTESIAN_POINT('Ctrl Pts',(45.3423250998467,-56.0302766707802,
-45.8832833333333));
#266256=CARTESIAN_POINT('Ctrl Pts',(44.5079524583205,-55.5485514015906,
-45.82495));
#266257=CARTESIAN_POINT('Ctrl Pts',(43.6735798167943,-56.0302766707802,
-45.7666166666667));
#266258=CARTESIAN_POINT('Ctrl Pts',(42.839207175268,-56.5120019399698,-45.7082833333333));
#266259=CARTESIAN_POINT('Ctrl Pts',(42.839207175268,-57.4754524783491,-45.64995));
#266260=CARTESIAN_POINT('Ctrl Pts',(42.839207175268,-58.4389030167283,-45.5916166666667));
#266261=CARTESIAN_POINT('Ctrl Pts',(43.6735798167943,-58.920628285918,-45.5332833333333));
#266262=CARTESIAN_POINT('Ctrl Pts',(44.5079524583205,-59.4023535551075,
-45.47495));
#266263=CARTESIAN_POINT('Ctrl Pts',(45.3423250998467,-58.920628285918,-45.4166166666667));
#266264=CARTESIAN_POINT('Ctrl Pts',(46.1766977413729,-58.4389030167283,
-45.3582833333333));
#266265=CARTESIAN_POINT('Ctrl Pts',(46.1766977413729,-57.4754524783491,
-45.29995));
#266266=CARTESIAN_POINT('Ctrl Pts',(46.1766977413729,-56.5120019399699,
-45.2416166666667));
#266267=CARTESIAN_POINT('Ctrl Pts',(45.3423250998467,-56.0302766707802,
-45.1832833333334));
#266268=CARTESIAN_POINT('Ctrl Pts',(44.5079524583205,-55.5485514015906,
-45.12495));
#266269=CARTESIAN_POINT('Ctrl Pts',(43.6735798167943,-56.0302766707802,
-45.0666166666667));
#266270=CARTESIAN_POINT('Ctrl Pts',(42.839207175268,-56.5120019399698,-45.0082833333334));
#266271=CARTESIAN_POINT('Ctrl Pts',(42.839207175268,-57.4754524783491,-44.94995));
#266272=CARTESIAN_POINT('Ctrl Pts',(42.839207175268,-58.4389030167283,-44.8916166666667));
#266273=CARTESIAN_POINT('Ctrl Pts',(43.6735798167943,-58.920628285918,-44.8332833333334));
#266274=CARTESIAN_POINT('Ctrl Pts',(44.5079524583205,-59.4023535551075,
-44.77495));
#266275=CARTESIAN_POINT('Ctrl Pts',(45.3423250998467,-58.920628285918,-44.7166166666667));
#266276=CARTESIAN_POINT('Ctrl Pts',(46.1766977413729,-58.4389030167283,
-44.6582833333334));
#266277=CARTESIAN_POINT('Ctrl Pts',(46.1766977413729,-57.4754524783491,
-44.59995));
#266278=CARTESIAN_POINT('Ctrl Pts',(46.1766977413729,-56.5120019399699,
-44.5416166666667));
#266279=CARTESIAN_POINT('Ctrl Pts',(45.3423250998467,-56.0302766707802,
-44.4832833333334));
#266280=CARTESIAN_POINT('Ctrl Pts',(44.5079524583205,-55.5485514015906,
-44.42495));
#266281=CARTESIAN_POINT('Ctrl Pts',(43.6735798167943,-56.0302766707802,
-44.3666166666667));
#266282=CARTESIAN_POINT('Ctrl Pts',(42.839207175268,-56.5120019399698,-44.3082833333334));
#266283=CARTESIAN_POINT('Ctrl Pts',(42.839207175268,-57.4754524783491,-44.24995));
#266284=CARTESIAN_POINT('Ctrl Pts',(42.839207175268,-58.4389030167283,-44.1916166666667));
#266285=CARTESIAN_POINT('Ctrl Pts',(43.6735798167943,-58.920628285918,-44.1332833333334));
#266286=CARTESIAN_POINT('Ctrl Pts',(44.5079524583205,-59.4023535551075,
-44.07495));
#266287=CARTESIAN_POINT('Ctrl Pts',(45.3423250998467,-58.920628285918,-44.0166166666667));
#266288=CARTESIAN_POINT('Ctrl Pts',(46.1766977413729,-58.4389030167283,
-43.9582833333334));
#266289=CARTESIAN_POINT('Ctrl Pts',(46.1766977413729,-57.4754524783491,
-43.89995));
#266290=CARTESIAN_POINT('Ctrl Pts',(46.1766977413729,-56.5120019399699,
-43.8416166666667));
#266291=CARTESIAN_POINT('Ctrl Pts',(45.3423250998467,-56.0302766707802,
-43.7832833333334));
#266292=CARTESIAN_POINT('Ctrl Pts',(44.5079524583205,-55.5485514015906,
-43.72495));
#266293=CARTESIAN_POINT('Ctrl Pts',(43.6735798167943,-56.0302766707802,
-43.6666166666667));
#266294=CARTESIAN_POINT('Ctrl Pts',(42.839207175268,-56.5120019399698,-43.6082833333333));
#266295=CARTESIAN_POINT('Ctrl Pts',(42.839207175268,-57.4754524783491,-43.54995));
#266296=CARTESIAN_POINT('Ctrl Pts',(42.839207175268,-58.4389030167283,-43.4916166666667));
#266297=CARTESIAN_POINT('Ctrl Pts',(43.6735798167943,-58.920628285918,-43.4332833333333));
#266298=CARTESIAN_POINT('Ctrl Pts',(44.5079524583205,-59.4023535551075,
-43.37495));
#266299=CARTESIAN_POINT('Ctrl Pts',(45.3423250998467,-58.920628285918,-43.3166166666667));
#266300=CARTESIAN_POINT('Ctrl Pts',(46.1766977413729,-58.4389030167283,
-43.2582833333333));
#266301=CARTESIAN_POINT('Ctrl Pts',(46.1766977413729,-57.4754524783491,
-43.19995));
#266302=CARTESIAN_POINT('Ctrl Pts',(46.1766977413729,-56.5120019399699,
-43.1416166666667));
#266303=CARTESIAN_POINT('Ctrl Pts',(45.3423250998467,-56.0302766707802,
-43.0832833333333));
#266304=CARTESIAN_POINT('Ctrl Pts',(44.5079524583205,-55.5485514015906,
-43.02495));
#266305=CARTESIAN_POINT('Ctrl Pts',(43.6735798167943,-56.0302766707802,
-42.9666166666667));
#266306=CARTESIAN_POINT('Ctrl Pts',(42.839207175268,-56.5120019399698,-42.9082833333333));
#266307=CARTESIAN_POINT('Ctrl Pts',(42.839207175268,-57.4754524783491,-42.84995));
#266308=CARTESIAN_POINT('Ctrl Pts',(42.839207175268,-58.4389030167283,-42.7916166666667));
#266309=CARTESIAN_POINT('Ctrl Pts',(43.6735798167943,-58.920628285918,-42.7332833333334));
#266310=CARTESIAN_POINT('Ctrl Pts',(44.5079524583205,-59.4023535551075,
-42.67495));
#266311=CARTESIAN_POINT('Ctrl Pts',(45.3423250998467,-58.920628285918,-42.6166166666667));
#266312=CARTESIAN_POINT('Ctrl Pts',(46.1766977413729,-58.4389030167283,
-42.5582833333333));
#266313=CARTESIAN_POINT('Ctrl Pts',(46.1766977413729,-57.4754524783491,
-42.49995));
#266314=CARTESIAN_POINT('Ctrl Pts',(46.1766977413729,-56.5120019399699,
-42.4416166666667));
#266315=CARTESIAN_POINT('Ctrl Pts',(45.3423250998467,-56.0302766707802,
-42.3832833333333));
#266316=CARTESIAN_POINT('Ctrl Pts',(44.5079524583205,-55.5485514015906,
-42.32495));
#266317=CARTESIAN_POINT('Ctrl Pts',(43.6735798167943,-56.0302766707802,
-42.2666166666667));
#266318=CARTESIAN_POINT('Ctrl Pts',(42.839207175268,-56.5120019399698,-42.2082833333333));
#266319=CARTESIAN_POINT('Ctrl Pts',(42.839207175268,-57.4754524783491,-42.14995));
#266320=CARTESIAN_POINT('Ctrl Pts',(42.839207175268,-58.4389030167283,-42.0916166666667));
#266321=CARTESIAN_POINT('Ctrl Pts',(43.6735798167943,-58.920628285918,-42.0332833333334));
#266322=CARTESIAN_POINT('Ctrl Pts',(44.5079524583205,-59.4023535551075,
-41.97495));
#266323=CARTESIAN_POINT('Ctrl Pts',(45.3423250998467,-58.920628285918,-41.9166166666667));
#266324=CARTESIAN_POINT('Ctrl Pts',(46.1766977413729,-58.4389030167283,
-41.8582833333333));
#266325=CARTESIAN_POINT('Ctrl Pts',(46.1766977413729,-57.4754524783491,
-41.79995));
#266326=CARTESIAN_POINT('Ctrl Pts',(46.1766977413729,-56.5120019399699,
-41.7416166666667));
#266327=CARTESIAN_POINT('Ctrl Pts',(45.3423250998467,-56.0302766707802,
-41.6832833333333));
#266328=CARTESIAN_POINT('Ctrl Pts',(44.5079524583205,-55.5485514015906,
-41.62495));
#266329=CARTESIAN_POINT('Ctrl Pts',(43.6735798167943,-56.0302766707802,
-41.5666166666667));
#266330=CARTESIAN_POINT('Ctrl Pts',(42.839207175268,-56.5120019399698,-41.5082833333334));
#266331=CARTESIAN_POINT('Ctrl Pts',(42.839207175268,-57.4754524783491,-41.44995));
#266332=CARTESIAN_POINT('Ctrl Pts',(42.839207175268,-58.4389030167283,-41.3916166666667));
#266333=CARTESIAN_POINT('Ctrl Pts',(43.6735798167943,-58.920628285918,-41.3332833333334));
#266334=CARTESIAN_POINT('Ctrl Pts',(44.5079524583205,-59.4023535551075,
-41.27495));
#266335=CARTESIAN_POINT('Ctrl Pts',(45.3423250998467,-58.920628285918,-41.2166166666667));
#266336=CARTESIAN_POINT('Ctrl Pts',(46.1766977413729,-58.4389030167283,
-41.1582833333333));
#266337=CARTESIAN_POINT('Ctrl Pts',(46.1766977413729,-57.4754524783491,
-41.09995));
#266338=CARTESIAN_POINT('Ctrl Pts',(46.1766977413729,-56.5120019399699,
-41.0416166666667));
#266339=CARTESIAN_POINT('Ctrl Pts',(45.3423250998467,-56.0302766707802,
-40.9832833333333));
#266340=CARTESIAN_POINT('Ctrl Pts',(44.5079524583205,-55.5485514015906,
-40.92495));
#266341=CARTESIAN_POINT('Ctrl Pts',(43.6735798167943,-56.0302766707802,
-40.8666166666667));
#266342=CARTESIAN_POINT('Ctrl Pts',(42.839207175268,-56.5120019399698,-40.8082833333334));
#266343=CARTESIAN_POINT('Ctrl Pts',(42.839207175268,-57.4754524783491,-40.74995));
#266344=CARTESIAN_POINT('Ctrl Pts',(42.839207175268,-58.4389030167283,-40.6916166666667));
#266345=CARTESIAN_POINT('Ctrl Pts',(43.6735798167943,-58.920628285918,-40.6332833333334));
#266346=CARTESIAN_POINT('Ctrl Pts',(44.5079524583205,-59.4023535551075,
-40.57495));
#266347=CARTESIAN_POINT('Ctrl Pts',(45.3423250998467,-58.920628285918,-40.5166166666667));
#266348=CARTESIAN_POINT('Ctrl Pts',(46.1766977413729,-58.4389030167283,
-40.4582833333333));
#266349=CARTESIAN_POINT('Ctrl Pts',(46.1766977413729,-57.4754524783491,
-40.39995));
#266350=CARTESIAN_POINT('Ctrl Pts',(46.1766977413729,-56.5120019399699,
-40.3416166666667));
#266351=CARTESIAN_POINT('Ctrl Pts',(45.3423250998467,-56.0302766707802,
-40.2832833333334));
#266352=CARTESIAN_POINT('Ctrl Pts',(44.5079524583205,-55.5485514015906,
-40.22495));
#266353=CARTESIAN_POINT('Ctrl Pts',(43.6735798167943,-56.0302766707802,
-40.1666166666667));
#266354=CARTESIAN_POINT('Ctrl Pts',(42.839207175268,-56.5120019399698,-40.1082833333334));
#266355=CARTESIAN_POINT('Ctrl Pts',(42.839207175268,-57.4754524783491,-40.04995));
#266356=CARTESIAN_POINT('Ctrl Pts',(42.839207175268,-58.4389030167283,-39.9916166666667));
#266357=CARTESIAN_POINT('Ctrl Pts',(43.6735798167943,-58.920628285918,-39.9332833333333));
#266358=CARTESIAN_POINT('Ctrl Pts',(44.5079524583205,-59.4023535551075,
-39.87495));
#266359=CARTESIAN_POINT('Ctrl Pts',(45.3423250998467,-58.920628285918,-39.8166166666667));
#266360=CARTESIAN_POINT('Ctrl Pts',(46.1766977413729,-58.4389030167283,
-39.7582833333334));
#266361=CARTESIAN_POINT('Ctrl Pts',(46.1766977413729,-57.4754524783491,
-39.69995));
#266362=CARTESIAN_POINT('Ctrl Pts',(46.1766977413729,-56.5120019399699,
-39.6416166666667));
#266363=CARTESIAN_POINT('Ctrl Pts',(45.3423250998467,-56.0302766707802,
-39.5832833333333));
#266364=CARTESIAN_POINT('Ctrl Pts',(44.5079524583205,-55.5485514015906,
-39.52495));
#266365=CARTESIAN_POINT('Ctrl Pts',(43.6735798167943,-56.0302766707802,
-39.4666166666667));
#266366=CARTESIAN_POINT('Ctrl Pts',(42.839207175268,-56.5120019399698,-39.4082833333334));
#266367=CARTESIAN_POINT('Ctrl Pts',(42.839207175268,-57.4754524783491,-39.34995));
#266368=CARTESIAN_POINT('Ctrl Pts',(42.839207175268,-58.4389030167283,-39.2916166666667));
#266369=CARTESIAN_POINT('Ctrl Pts',(43.6735798167943,-58.920628285918,-39.2332833333333));
#266370=CARTESIAN_POINT('Ctrl Pts',(44.5079524583205,-59.4023535551075,
-39.17495));
#266371=CARTESIAN_POINT('Ctrl Pts',(45.3423250998467,-58.920628285918,-39.1166166666667));
#266372=CARTESIAN_POINT('Ctrl Pts',(46.1766977413729,-58.4389030167283,
-39.0582833333334));
#266373=CARTESIAN_POINT('Ctrl Pts',(46.1766977413729,-57.4754524783491,
-38.99995));
#266374=CARTESIAN_POINT('Ctrl Pts',(46.1766977413729,-56.5120019399699,
-38.9416166666667));
#266375=CARTESIAN_POINT('Ctrl Pts',(45.3423250998467,-56.0302766707802,
-38.8832833333334));
#266376=CARTESIAN_POINT('Ctrl Pts',(44.5079524583205,-55.5485514015906,
-38.82495));
#266377=CARTESIAN_POINT('Ctrl Pts',(43.6735798167943,-56.0302766707802,
-38.7666166666667));
#266378=CARTESIAN_POINT('Ctrl Pts',(42.839207175268,-56.5120019399698,-38.7082833333334));
#266379=CARTESIAN_POINT('Ctrl Pts',(42.839207175268,-57.4754524783491,-38.64995));
#266380=CARTESIAN_POINT('Ctrl Pts',(42.839207175268,-58.4389030167283,-38.5916166666667));
#266381=CARTESIAN_POINT('Ctrl Pts',(43.6735798167943,-58.920628285918,-38.5332833333334));
#266382=CARTESIAN_POINT('Ctrl Pts',(44.5079524583205,-59.4023535551075,
-38.47495));
#266383=CARTESIAN_POINT('Ctrl Pts',(45.3423250998467,-58.920628285918,-38.4166166666667));
#266384=CARTESIAN_POINT('Ctrl Pts',(46.1766977413729,-58.4389030167283,
-38.3582833333333));
#266385=CARTESIAN_POINT('Ctrl Pts',(46.1766977413729,-57.4754524783491,
-38.29995));
#266386=CARTESIAN_POINT('Ctrl Pts',(46.1766977413729,-56.5120019399699,
-38.2416166666667));
#266387=CARTESIAN_POINT('Ctrl Pts',(45.3423250998467,-56.0302766707802,
-38.1832833333333));
#266388=CARTESIAN_POINT('Ctrl Pts',(44.5079524583205,-55.5485514015906,
-38.12495));
#266389=CARTESIAN_POINT('Ctrl Pts',(43.6735798167943,-56.0302766707802,
-38.0666166666667));
#266390=CARTESIAN_POINT('Ctrl Pts',(42.839207175268,-56.5120019399698,-38.0082833333333));
#266391=CARTESIAN_POINT('Ctrl Pts',(42.839207175268,-57.4754524783491,-37.94995));
#266392=CARTESIAN_POINT('Ctrl Pts',(42.839207175268,-58.4389030167283,-37.8916166666667));
#266393=CARTESIAN_POINT('Ctrl Pts',(43.6735798167943,-58.920628285918,-37.8332833333334));
#266394=CARTESIAN_POINT('Ctrl Pts',(44.5079524583205,-59.4023535551075,
-37.77495));
#266395=CARTESIAN_POINT('Ctrl Pts',(45.3423250998467,-58.920628285918,-37.7166166666667));
#266396=CARTESIAN_POINT('Ctrl Pts',(46.1766977413729,-58.4389030167283,
-37.6582833333333));
#266397=CARTESIAN_POINT('Ctrl Pts',(46.1766977413729,-57.4754524783491,
-37.59995));
#266398=CARTESIAN_POINT('Ctrl Pts',(46.1766977413729,-56.5120019399699,
-37.5416166666667));
#266399=CARTESIAN_POINT('Ctrl Pts',(45.3423250998467,-56.0302766707802,
-37.4832833333334));
#266400=CARTESIAN_POINT('Ctrl Pts',(44.5079524583205,-55.5485514015906,
-37.42495));
#266401=CARTESIAN_POINT('Ctrl Pts',(43.6735798167943,-56.0302766707802,
-37.3666166666667));
#266402=CARTESIAN_POINT('Ctrl Pts',(42.839207175268,-56.5120019399698,-37.3082833333333));
#266403=CARTESIAN_POINT('Ctrl Pts',(42.839207175268,-57.4754524783491,-37.24995));
#266404=CARTESIAN_POINT('Ctrl Pts',(42.839207175268,-58.4389030167283,-37.1916166666667));
#266405=CARTESIAN_POINT('Ctrl Pts',(43.6735798167943,-58.920628285918,-37.1332833333334));
#266406=CARTESIAN_POINT('Ctrl Pts',(44.5079524583205,-59.4023535551075,
-37.07495));
#266407=CARTESIAN_POINT('Ctrl Pts',(45.3423250998467,-58.920628285918,-37.0166166666667));
#266408=CARTESIAN_POINT('Ctrl Pts',(45.4506530446707,-58.8580851178131,
-37.0090431559831));
#266409=CARTESIAN_POINT('Ctrl Pts',(45.5484465834733,-58.7800914304091,
-37.0009024189827));
#266410=CARTESIAN_POINT('Ctrl Pts',(46.5766932247459,-57.4754524783491,
-53.2308875));
#266411=CARTESIAN_POINT('Ctrl Pts',(46.5766932247459,-56.2810644399698,
-53.1725541666667));
#266412=CARTESIAN_POINT('Ctrl Pts',(45.5423228415332,-55.6838704207802,
-53.1142208333334));
#266413=CARTESIAN_POINT('Ctrl Pts',(44.5079524583205,-55.0866764015906,
-53.0558875000001));
#266414=CARTESIAN_POINT('Ctrl Pts',(43.4735820751078,-55.6838704207802,
-52.9975541666667));
#266415=CARTESIAN_POINT('Ctrl Pts',(42.4392116918951,-56.2810644399698,
-52.9392208333334));
#266416=CARTESIAN_POINT('Ctrl Pts',(42.439211691895,-57.4754524783491,-52.8808875));
#266417=CARTESIAN_POINT('Ctrl Pts',(42.4392116918951,-58.6698405167284,
-52.8225541666667));
#266418=CARTESIAN_POINT('Ctrl Pts',(43.4735820751078,-59.267034535918,-52.7642208333334));
#266419=CARTESIAN_POINT('Ctrl Pts',(44.5079524583205,-59.8642285551076,
-52.7058875));
#266420=CARTESIAN_POINT('Ctrl Pts',(45.5423228415332,-59.267034535918,-52.6475541666667));
#266421=CARTESIAN_POINT('Ctrl Pts',(46.5766932247459,-58.6698405167284,
-52.5892208333333));
#266422=CARTESIAN_POINT('Ctrl Pts',(46.5766932247459,-57.4754524783491,
-52.5308875));
#266423=CARTESIAN_POINT('Ctrl Pts',(46.5766932247459,-56.2810644399698,
-52.4725541666667));
#266424=CARTESIAN_POINT('Ctrl Pts',(45.5423228415332,-55.6838704207802,
-52.4142208333334));
#266425=CARTESIAN_POINT('Ctrl Pts',(44.5079524583205,-55.0866764015906,
-52.3558875000001));
#266426=CARTESIAN_POINT('Ctrl Pts',(43.4735820751078,-55.6838704207802,
-52.2975541666667));
#266427=CARTESIAN_POINT('Ctrl Pts',(42.4392116918951,-56.2810644399698,
-52.2392208333334));
#266428=CARTESIAN_POINT('Ctrl Pts',(42.439211691895,-57.4754524783491,-52.1808875));
#266429=CARTESIAN_POINT('Ctrl Pts',(42.4392116918951,-58.6698405167284,
-52.1225541666667));
#266430=CARTESIAN_POINT('Ctrl Pts',(43.4735820751078,-59.267034535918,-52.0642208333334));
#266431=CARTESIAN_POINT('Ctrl Pts',(44.5079524583205,-59.8642285551076,
-52.0058875));
#266432=CARTESIAN_POINT('Ctrl Pts',(45.5423228415332,-59.267034535918,-51.9475541666667));
#266433=CARTESIAN_POINT('Ctrl Pts',(46.5766932247459,-58.6698405167284,
-51.8892208333334));
#266434=CARTESIAN_POINT('Ctrl Pts',(46.5766932247459,-57.4754524783491,
-51.8308875));
#266435=CARTESIAN_POINT('Ctrl Pts',(46.5766932247459,-56.2810644399698,
-51.7725541666667));
#266436=CARTESIAN_POINT('Ctrl Pts',(45.5423228415332,-55.6838704207802,
-51.7142208333334));
#266437=CARTESIAN_POINT('Ctrl Pts',(44.5079524583205,-55.0866764015906,
-51.6558875));
#266438=CARTESIAN_POINT('Ctrl Pts',(43.4735820751078,-55.6838704207802,
-51.5975541666667));
#266439=CARTESIAN_POINT('Ctrl Pts',(42.4392116918951,-56.2810644399698,
-51.5392208333333));
#266440=CARTESIAN_POINT('Ctrl Pts',(42.439211691895,-57.4754524783491,-51.4808875));
#266441=CARTESIAN_POINT('Ctrl Pts',(42.4392116918951,-58.6698405167284,
-51.4225541666667));
#266442=CARTESIAN_POINT('Ctrl Pts',(43.4735820751078,-59.267034535918,-51.3642208333334));
#266443=CARTESIAN_POINT('Ctrl Pts',(44.5079524583205,-59.8642285551076,
-51.3058875));
#266444=CARTESIAN_POINT('Ctrl Pts',(45.5423228415332,-59.267034535918,-51.2475541666667));
#266445=CARTESIAN_POINT('Ctrl Pts',(46.5766932247459,-58.6698405167284,
-51.1892208333334));
#266446=CARTESIAN_POINT('Ctrl Pts',(46.5766932247459,-57.4754524783491,
-51.1308875));
#266447=CARTESIAN_POINT('Ctrl Pts',(46.5766932247459,-56.2810644399698,
-51.0725541666667));
#266448=CARTESIAN_POINT('Ctrl Pts',(45.5423228415332,-55.6838704207802,
-51.0142208333334));
#266449=CARTESIAN_POINT('Ctrl Pts',(44.5079524583205,-55.0866764015906,
-50.9558875));
#266450=CARTESIAN_POINT('Ctrl Pts',(43.4735820751078,-55.6838704207802,
-50.8975541666667));
#266451=CARTESIAN_POINT('Ctrl Pts',(42.4392116918951,-56.2810644399698,
-50.8392208333333));
#266452=CARTESIAN_POINT('Ctrl Pts',(42.439211691895,-57.4754524783491,-50.7808875));
#266453=CARTESIAN_POINT('Ctrl Pts',(42.4392116918951,-58.6698405167284,
-50.7225541666667));
#266454=CARTESIAN_POINT('Ctrl Pts',(43.4735820751078,-59.267034535918,-50.6642208333333));
#266455=CARTESIAN_POINT('Ctrl Pts',(44.5079524583205,-59.8642285551076,
-50.6058875));
#266456=CARTESIAN_POINT('Ctrl Pts',(45.5423228415332,-59.267034535918,-50.5475541666667));
#266457=CARTESIAN_POINT('Ctrl Pts',(46.5766932247459,-58.6698405167284,
-50.4892208333333));
#266458=CARTESIAN_POINT('Ctrl Pts',(46.5766932247459,-57.4754524783491,
-50.4308875));
#266459=CARTESIAN_POINT('Ctrl Pts',(46.5766932247459,-56.2810644399698,
-50.3725541666667));
#266460=CARTESIAN_POINT('Ctrl Pts',(45.5423228415332,-55.6838704207802,
-50.3142208333334));
#266461=CARTESIAN_POINT('Ctrl Pts',(44.5079524583205,-55.0866764015906,
-50.2558875));
#266462=CARTESIAN_POINT('Ctrl Pts',(43.4735820751078,-55.6838704207802,
-50.1975541666667));
#266463=CARTESIAN_POINT('Ctrl Pts',(42.4392116918951,-56.2810644399698,
-50.1392208333333));
#266464=CARTESIAN_POINT('Ctrl Pts',(42.439211691895,-57.4754524783491,-50.0808875));
#266465=CARTESIAN_POINT('Ctrl Pts',(42.4392116918951,-58.6698405167284,
-50.0225541666667));
#266466=CARTESIAN_POINT('Ctrl Pts',(43.4735820751078,-59.267034535918,-49.9642208333334));
#266467=CARTESIAN_POINT('Ctrl Pts',(44.5079524583205,-59.8642285551076,
-49.9058875));
#266468=CARTESIAN_POINT('Ctrl Pts',(45.5423228415332,-59.267034535918,-49.8475541666667));
#266469=CARTESIAN_POINT('Ctrl Pts',(46.5766932247459,-58.6698405167284,
-49.7892208333333));
#266470=CARTESIAN_POINT('Ctrl Pts',(46.5766932247459,-57.4754524783491,
-49.7308875));
#266471=CARTESIAN_POINT('Ctrl Pts',(46.5766932247459,-56.2810644399698,
-49.6725541666667));
#266472=CARTESIAN_POINT('Ctrl Pts',(45.5423228415332,-55.6838704207802,
-49.6142208333334));
#266473=CARTESIAN_POINT('Ctrl Pts',(44.5079524583205,-55.0866764015906,
-49.5558875));
#266474=CARTESIAN_POINT('Ctrl Pts',(43.4735820751078,-55.6838704207802,
-49.4975541666667));
#266475=CARTESIAN_POINT('Ctrl Pts',(42.4392116918951,-56.2810644399698,
-49.4392208333333));
#266476=CARTESIAN_POINT('Ctrl Pts',(42.439211691895,-57.4754524783491,-49.3808875));
#266477=CARTESIAN_POINT('Ctrl Pts',(42.4392116918951,-58.6698405167284,
-49.3225541666667));
#266478=CARTESIAN_POINT('Ctrl Pts',(43.4735820751078,-59.267034535918,-49.2642208333334));
#266479=CARTESIAN_POINT('Ctrl Pts',(44.5079524583205,-59.8642285551076,
-49.2058875));
#266480=CARTESIAN_POINT('Ctrl Pts',(45.5423228415332,-59.267034535918,-49.1475541666667));
#266481=CARTESIAN_POINT('Ctrl Pts',(46.5766932247459,-58.6698405167284,
-49.0892208333333));
#266482=CARTESIAN_POINT('Ctrl Pts',(46.5766932247459,-57.4754524783491,
-49.0308875));
#266483=CARTESIAN_POINT('Ctrl Pts',(46.5766932247459,-56.2810644399698,
-48.9725541666667));
#266484=CARTESIAN_POINT('Ctrl Pts',(45.5423228415332,-55.6838704207802,
-48.9142208333334));
#266485=CARTESIAN_POINT('Ctrl Pts',(44.5079524583205,-55.0866764015906,
-48.8558875));
#266486=CARTESIAN_POINT('Ctrl Pts',(43.4735820751078,-55.6838704207802,
-48.7975541666667));
#266487=CARTESIAN_POINT('Ctrl Pts',(42.4392116918951,-56.2810644399698,
-48.7392208333334));
#266488=CARTESIAN_POINT('Ctrl Pts',(42.439211691895,-57.4754524783491,-48.6808875));
#266489=CARTESIAN_POINT('Ctrl Pts',(42.4392116918951,-58.6698405167284,
-48.6225541666667));
#266490=CARTESIAN_POINT('Ctrl Pts',(43.4735820751078,-59.267034535918,-48.5642208333334));
#266491=CARTESIAN_POINT('Ctrl Pts',(44.5079524583205,-59.8642285551076,
-48.5058875));
#266492=CARTESIAN_POINT('Ctrl Pts',(45.5423228415332,-59.267034535918,-48.4475541666667));
#266493=CARTESIAN_POINT('Ctrl Pts',(46.5766932247459,-58.6698405167284,
-48.3892208333334));
#266494=CARTESIAN_POINT('Ctrl Pts',(46.5766932247459,-57.4754524783491,
-48.3308875));
#266495=CARTESIAN_POINT('Ctrl Pts',(46.5766932247459,-56.2810644399698,
-48.2725541666667));
#266496=CARTESIAN_POINT('Ctrl Pts',(45.5423228415332,-55.6838704207802,
-48.2142208333334));
#266497=CARTESIAN_POINT('Ctrl Pts',(44.5079524583205,-55.0866764015906,
-48.1558875));
#266498=CARTESIAN_POINT('Ctrl Pts',(43.4735820751078,-55.6838704207802,
-48.0975541666667));
#266499=CARTESIAN_POINT('Ctrl Pts',(42.4392116918951,-56.2810644399698,
-48.0392208333334));
#266500=CARTESIAN_POINT('Ctrl Pts',(42.439211691895,-57.4754524783491,-47.9808875));
#266501=CARTESIAN_POINT('Ctrl Pts',(42.4392116918951,-58.6698405167284,
-47.9225541666667));
#266502=CARTESIAN_POINT('Ctrl Pts',(43.4735820751078,-59.267034535918,-47.8642208333334));
#266503=CARTESIAN_POINT('Ctrl Pts',(44.5079524583205,-59.8642285551076,
-47.8058875000001));
#266504=CARTESIAN_POINT('Ctrl Pts',(45.5423228415332,-59.267034535918,-47.7475541666667));
#266505=CARTESIAN_POINT('Ctrl Pts',(46.5766932247459,-58.6698405167284,
-47.6892208333334));
#266506=CARTESIAN_POINT('Ctrl Pts',(46.5766932247459,-57.4754524783491,
-47.6308875));
#266507=CARTESIAN_POINT('Ctrl Pts',(46.5766932247459,-56.2810644399698,
-47.5725541666667));
#266508=CARTESIAN_POINT('Ctrl Pts',(45.5423228415332,-55.6838704207802,
-47.5142208333333));
#266509=CARTESIAN_POINT('Ctrl Pts',(44.5079524583205,-55.0866764015906,
-47.4558875));
#266510=CARTESIAN_POINT('Ctrl Pts',(43.4735820751078,-55.6838704207802,
-47.3975541666667));
#266511=CARTESIAN_POINT('Ctrl Pts',(42.4392116918951,-56.2810644399698,
-47.3392208333334));
#266512=CARTESIAN_POINT('Ctrl Pts',(42.439211691895,-57.4754524783491,-47.2808875));
#266513=CARTESIAN_POINT('Ctrl Pts',(42.4392116918951,-58.6698405167284,
-47.2225541666667));
#266514=CARTESIAN_POINT('Ctrl Pts',(43.4735820751078,-59.267034535918,-47.1642208333334));
#266515=CARTESIAN_POINT('Ctrl Pts',(44.5079524583205,-59.8642285551076,
-47.1058875));
#266516=CARTESIAN_POINT('Ctrl Pts',(45.5423228415332,-59.267034535918,-47.0475541666667));
#266517=CARTESIAN_POINT('Ctrl Pts',(46.5766932247459,-58.6698405167284,
-46.9892208333334));
#266518=CARTESIAN_POINT('Ctrl Pts',(46.5766932247459,-57.4754524783491,
-46.9308875));
#266519=CARTESIAN_POINT('Ctrl Pts',(46.5766932247459,-56.2810644399698,
-46.8725541666667));
#266520=CARTESIAN_POINT('Ctrl Pts',(45.5423228415332,-55.6838704207802,
-46.8142208333334));
#266521=CARTESIAN_POINT('Ctrl Pts',(44.5079524583205,-55.0866764015906,
-46.7558875));
#266522=CARTESIAN_POINT('Ctrl Pts',(43.4735820751078,-55.6838704207802,
-46.6975541666667));
#266523=CARTESIAN_POINT('Ctrl Pts',(42.4392116918951,-56.2810644399698,
-46.6392208333334));
#266524=CARTESIAN_POINT('Ctrl Pts',(42.439211691895,-57.4754524783491,-46.5808875));
#266525=CARTESIAN_POINT('Ctrl Pts',(42.4392116918951,-58.6698405167284,
-46.5225541666667));
#266526=CARTESIAN_POINT('Ctrl Pts',(43.4735820751078,-59.267034535918,-46.4642208333334));
#266527=CARTESIAN_POINT('Ctrl Pts',(44.5079524583205,-59.8642285551076,
-46.4058875));
#266528=CARTESIAN_POINT('Ctrl Pts',(45.5423228415332,-59.267034535918,-46.3475541666667));
#266529=CARTESIAN_POINT('Ctrl Pts',(46.5766932247459,-58.6698405167284,
-46.2892208333334));
#266530=CARTESIAN_POINT('Ctrl Pts',(46.5766932247459,-57.4754524783491,
-46.2308875));
#266531=CARTESIAN_POINT('Ctrl Pts',(46.5766932247459,-56.2810644399698,
-46.1725541666667));
#266532=CARTESIAN_POINT('Ctrl Pts',(45.5423228415332,-55.6838704207802,
-46.1142208333334));
#266533=CARTESIAN_POINT('Ctrl Pts',(44.5079524583205,-55.0866764015906,
-46.0558875));
#266534=CARTESIAN_POINT('Ctrl Pts',(43.4735820751078,-55.6838704207802,
-45.9975541666667));
#266535=CARTESIAN_POINT('Ctrl Pts',(42.4392116918951,-56.2810644399698,
-45.9392208333333));
#266536=CARTESIAN_POINT('Ctrl Pts',(42.439211691895,-57.4754524783491,-45.8808875));
#266537=CARTESIAN_POINT('Ctrl Pts',(42.4392116918951,-58.6698405167284,
-45.8225541666667));
#266538=CARTESIAN_POINT('Ctrl Pts',(43.4735820751078,-59.267034535918,-45.7642208333334));
#266539=CARTESIAN_POINT('Ctrl Pts',(44.5079524583205,-59.8642285551076,
-45.7058875));
#266540=CARTESIAN_POINT('Ctrl Pts',(45.5423228415332,-59.267034535918,-45.6475541666667));
#266541=CARTESIAN_POINT('Ctrl Pts',(46.5766932247459,-58.6698405167284,
-45.5892208333334));
#266542=CARTESIAN_POINT('Ctrl Pts',(46.5766932247459,-57.4754524783491,
-45.5308875));
#266543=CARTESIAN_POINT('Ctrl Pts',(46.5766932247459,-56.2810644399698,
-45.4725541666667));
#266544=CARTESIAN_POINT('Ctrl Pts',(45.5423228415332,-55.6838704207802,
-45.4142208333334));
#266545=CARTESIAN_POINT('Ctrl Pts',(44.5079524583205,-55.0866764015906,
-45.3558875));
#266546=CARTESIAN_POINT('Ctrl Pts',(43.4735820751078,-55.6838704207802,
-45.2975541666667));
#266547=CARTESIAN_POINT('Ctrl Pts',(42.4392116918951,-56.2810644399698,
-45.2392208333333));
#266548=CARTESIAN_POINT('Ctrl Pts',(42.439211691895,-57.4754524783491,-45.1808875));
#266549=CARTESIAN_POINT('Ctrl Pts',(42.4392116918951,-58.6698405167284,
-45.1225541666667));
#266550=CARTESIAN_POINT('Ctrl Pts',(43.4735820751078,-59.267034535918,-45.0642208333334));
#266551=CARTESIAN_POINT('Ctrl Pts',(44.5079524583205,-59.8642285551076,
-45.0058875));
#266552=CARTESIAN_POINT('Ctrl Pts',(45.5423228415332,-59.267034535918,-44.9475541666667));
#266553=CARTESIAN_POINT('Ctrl Pts',(46.5766932247459,-58.6698405167284,
-44.8892208333333));
#266554=CARTESIAN_POINT('Ctrl Pts',(46.5766932247459,-57.4754524783491,
-44.8308875));
#266555=CARTESIAN_POINT('Ctrl Pts',(46.5766932247459,-56.2810644399698,
-44.7725541666667));
#266556=CARTESIAN_POINT('Ctrl Pts',(45.5423228415332,-55.6838704207802,
-44.7142208333334));
#266557=CARTESIAN_POINT('Ctrl Pts',(44.5079524583205,-55.0866764015906,
-44.6558875));
#266558=CARTESIAN_POINT('Ctrl Pts',(43.4735820751078,-55.6838704207802,
-44.5975541666667));
#266559=CARTESIAN_POINT('Ctrl Pts',(42.4392116918951,-56.2810644399698,
-44.5392208333333));
#266560=CARTESIAN_POINT('Ctrl Pts',(42.439211691895,-57.4754524783491,-44.4808875000001));
#266561=CARTESIAN_POINT('Ctrl Pts',(42.4392116918951,-58.6698405167284,
-44.4225541666667));
#266562=CARTESIAN_POINT('Ctrl Pts',(43.4735820751078,-59.267034535918,-44.3642208333333));
#266563=CARTESIAN_POINT('Ctrl Pts',(44.5079524583205,-59.8642285551076,
-44.3058875));
#266564=CARTESIAN_POINT('Ctrl Pts',(45.5423228415332,-59.267034535918,-44.2475541666667));
#266565=CARTESIAN_POINT('Ctrl Pts',(46.5766932247459,-58.6698405167284,
-44.1892208333334));
#266566=CARTESIAN_POINT('Ctrl Pts',(46.5766932247459,-57.4754524783491,
-44.1308875000001));
#266567=CARTESIAN_POINT('Ctrl Pts',(46.5766932247459,-56.2810644399698,
-44.0725541666667));
#266568=CARTESIAN_POINT('Ctrl Pts',(45.5423228415332,-55.6838704207802,
-44.0142208333334));
#266569=CARTESIAN_POINT('Ctrl Pts',(44.5079524583205,-55.0866764015906,
-43.9558875));
#266570=CARTESIAN_POINT('Ctrl Pts',(43.4735820751078,-55.6838704207802,
-43.8975541666667));
#266571=CARTESIAN_POINT('Ctrl Pts',(42.4392116918951,-56.2810644399698,
-43.8392208333333));
#266572=CARTESIAN_POINT('Ctrl Pts',(42.439211691895,-57.4754524783491,-43.7808875));
#266573=CARTESIAN_POINT('Ctrl Pts',(42.4392116918951,-58.6698405167284,
-43.7225541666667));
#266574=CARTESIAN_POINT('Ctrl Pts',(43.4735820751078,-59.267034535918,-43.6642208333334));
#266575=CARTESIAN_POINT('Ctrl Pts',(44.5079524583205,-59.8642285551076,
-43.6058875));
#266576=CARTESIAN_POINT('Ctrl Pts',(45.5423228415332,-59.267034535918,-43.5475541666667));
#266577=CARTESIAN_POINT('Ctrl Pts',(46.5766932247459,-58.6698405167284,
-43.4892208333333));
#266578=CARTESIAN_POINT('Ctrl Pts',(46.5766932247459,-57.4754524783491,
-43.4308875));
#266579=CARTESIAN_POINT('Ctrl Pts',(46.5766932247459,-56.2810644399698,
-43.3725541666667));
#266580=CARTESIAN_POINT('Ctrl Pts',(45.5423228415332,-55.6838704207802,
-43.3142208333334));
#266581=CARTESIAN_POINT('Ctrl Pts',(44.5079524583205,-55.0866764015906,
-43.2558875));
#266582=CARTESIAN_POINT('Ctrl Pts',(43.4735820751078,-55.6838704207802,
-43.1975541666667));
#266583=CARTESIAN_POINT('Ctrl Pts',(42.4392116918951,-56.2810644399698,
-43.1392208333334));
#266584=CARTESIAN_POINT('Ctrl Pts',(42.439211691895,-57.4754524783491,-43.0808875));
#266585=CARTESIAN_POINT('Ctrl Pts',(42.4392116918951,-58.6698405167284,
-43.0225541666667));
#266586=CARTESIAN_POINT('Ctrl Pts',(43.4735820751078,-59.267034535918,-42.9642208333334));
#266587=CARTESIAN_POINT('Ctrl Pts',(44.5079524583205,-59.8642285551076,
-42.9058875));
#266588=CARTESIAN_POINT('Ctrl Pts',(45.5423228415332,-59.267034535918,-42.8475541666667));
#266589=CARTESIAN_POINT('Ctrl Pts',(46.5766932247459,-58.6698405167284,
-42.7892208333334));
#266590=CARTESIAN_POINT('Ctrl Pts',(46.5766932247459,-57.4754524783491,
-42.7308875000001));
#266591=CARTESIAN_POINT('Ctrl Pts',(46.5766932247459,-56.2810644399698,
-42.6725541666667));
#266592=CARTESIAN_POINT('Ctrl Pts',(45.5423228415332,-55.6838704207802,
-42.6142208333334));
#266593=CARTESIAN_POINT('Ctrl Pts',(44.5079524583205,-55.0866764015906,
-42.5558875));
#266594=CARTESIAN_POINT('Ctrl Pts',(43.4735820751078,-55.6838704207802,
-42.4975541666667));
#266595=CARTESIAN_POINT('Ctrl Pts',(42.4392116918951,-56.2810644399698,
-42.4392208333334));
#266596=CARTESIAN_POINT('Ctrl Pts',(42.439211691895,-57.4754524783491,-42.3808875000001));
#266597=CARTESIAN_POINT('Ctrl Pts',(42.4392116918951,-58.6698405167284,
-42.3225541666667));
#266598=CARTESIAN_POINT('Ctrl Pts',(43.4735820751078,-59.267034535918,-42.2642208333334));
#266599=CARTESIAN_POINT('Ctrl Pts',(44.5079524583205,-59.8642285551076,
-42.2058875));
#266600=CARTESIAN_POINT('Ctrl Pts',(45.5423228415332,-59.267034535918,-42.1475541666667));
#266601=CARTESIAN_POINT('Ctrl Pts',(46.5766932247459,-58.6698405167284,
-42.0892208333334));
#266602=CARTESIAN_POINT('Ctrl Pts',(46.5766932247459,-57.4754524783491,
-42.0308875000001));
#266603=CARTESIAN_POINT('Ctrl Pts',(46.5766932247459,-56.2810644399698,
-41.9725541666667));
#266604=CARTESIAN_POINT('Ctrl Pts',(45.5423228415332,-55.6838704207802,
-41.9142208333334));
#266605=CARTESIAN_POINT('Ctrl Pts',(44.5079524583205,-55.0866764015906,
-41.8558875));
#266606=CARTESIAN_POINT('Ctrl Pts',(43.4735820751078,-55.6838704207802,
-41.7975541666667));
#266607=CARTESIAN_POINT('Ctrl Pts',(42.4392116918951,-56.2810644399698,
-41.7392208333334));
#266608=CARTESIAN_POINT('Ctrl Pts',(42.439211691895,-57.4754524783491,-41.6808875000001));
#266609=CARTESIAN_POINT('Ctrl Pts',(42.4392116918951,-58.6698405167284,
-41.6225541666667));
#266610=CARTESIAN_POINT('Ctrl Pts',(43.4735820751078,-59.267034535918,-41.5642208333334));
#266611=CARTESIAN_POINT('Ctrl Pts',(44.5079524583205,-59.8642285551076,
-41.5058875));
#266612=CARTESIAN_POINT('Ctrl Pts',(45.5423228415332,-59.267034535918,-41.4475541666667));
#266613=CARTESIAN_POINT('Ctrl Pts',(46.5766932247459,-58.6698405167284,
-41.3892208333334));
#266614=CARTESIAN_POINT('Ctrl Pts',(46.5766932247459,-57.4754524783491,
-41.3308875000001));
#266615=CARTESIAN_POINT('Ctrl Pts',(46.5766932247459,-56.2810644399698,
-41.2725541666667));
#266616=CARTESIAN_POINT('Ctrl Pts',(45.5423228415332,-55.6838704207802,
-41.2142208333333));
#266617=CARTESIAN_POINT('Ctrl Pts',(44.5079524583205,-55.0866764015906,
-41.1558875));
#266618=CARTESIAN_POINT('Ctrl Pts',(43.4735820751078,-55.6838704207802,
-41.0975541666667));
#266619=CARTESIAN_POINT('Ctrl Pts',(42.4392116918951,-56.2810644399698,
-41.0392208333333));
#266620=CARTESIAN_POINT('Ctrl Pts',(42.439211691895,-57.4754524783491,-40.9808875000001));
#266621=CARTESIAN_POINT('Ctrl Pts',(42.4392116918951,-58.6698405167284,
-40.9225541666667));
#266622=CARTESIAN_POINT('Ctrl Pts',(43.4735820751078,-59.267034535918,-40.8642208333334));
#266623=CARTESIAN_POINT('Ctrl Pts',(44.5079524583205,-59.8642285551076,
-40.8058875));
#266624=CARTESIAN_POINT('Ctrl Pts',(45.5423228415332,-59.267034535918,-40.7475541666667));
#266625=CARTESIAN_POINT('Ctrl Pts',(46.5766932247459,-58.6698405167284,
-40.6892208333333));
#266626=CARTESIAN_POINT('Ctrl Pts',(46.5766932247459,-57.4754524783491,
-40.6308875));
#266627=CARTESIAN_POINT('Ctrl Pts',(46.5766932247459,-56.2810644399698,
-40.5725541666667));
#266628=CARTESIAN_POINT('Ctrl Pts',(45.5423228415332,-55.6838704207802,
-40.5142208333333));
#266629=CARTESIAN_POINT('Ctrl Pts',(44.5079524583205,-55.0866764015906,
-40.4558875));
#266630=CARTESIAN_POINT('Ctrl Pts',(43.4735820751078,-55.6838704207802,
-40.3975541666667));
#266631=CARTESIAN_POINT('Ctrl Pts',(42.4392116918951,-56.2810644399698,
-40.3392208333333));
#266632=CARTESIAN_POINT('Ctrl Pts',(42.439211691895,-57.4754524783491,-40.2808875));
#266633=CARTESIAN_POINT('Ctrl Pts',(42.4392116918951,-58.6698405167284,
-40.2225541666667));
#266634=CARTESIAN_POINT('Ctrl Pts',(43.4735820751078,-59.267034535918,-40.1642208333333));
#266635=CARTESIAN_POINT('Ctrl Pts',(44.5079524583205,-59.8642285551076,
-40.1058875));
#266636=CARTESIAN_POINT('Ctrl Pts',(45.5423228415332,-59.267034535918,-40.0475541666667));
#266637=CARTESIAN_POINT('Ctrl Pts',(46.5766932247459,-58.6698405167284,
-39.9892208333333));
#266638=CARTESIAN_POINT('Ctrl Pts',(46.5766932247459,-57.4754524783491,
-39.9308875));
#266639=CARTESIAN_POINT('Ctrl Pts',(46.5766932247459,-56.2810644399698,
-39.8725541666667));
#266640=CARTESIAN_POINT('Ctrl Pts',(45.5423228415332,-55.6838704207802,
-39.8142208333334));
#266641=CARTESIAN_POINT('Ctrl Pts',(44.5079524583205,-55.0866764015906,
-39.7558875));
#266642=CARTESIAN_POINT('Ctrl Pts',(43.4735820751078,-55.6838704207802,
-39.6975541666667));
#266643=CARTESIAN_POINT('Ctrl Pts',(42.4392116918951,-56.2810644399698,
-39.6392208333334));
#266644=CARTESIAN_POINT('Ctrl Pts',(42.439211691895,-57.4754524783491,-39.5808875000001));
#266645=CARTESIAN_POINT('Ctrl Pts',(42.4392116918951,-58.6698405167284,
-39.5225541666667));
#266646=CARTESIAN_POINT('Ctrl Pts',(43.4735820751078,-59.267034535918,-39.4642208333333));
#266647=CARTESIAN_POINT('Ctrl Pts',(44.5079524583205,-59.8642285551076,
-39.4058875));
#266648=CARTESIAN_POINT('Ctrl Pts',(45.5423228415332,-59.267034535918,-39.3475541666667));
#266649=CARTESIAN_POINT('Ctrl Pts',(46.5766932247459,-58.6698405167284,
-39.2892208333334));
#266650=CARTESIAN_POINT('Ctrl Pts',(46.5766932247459,-57.4754524783491,
-39.2308875));
#266651=CARTESIAN_POINT('Ctrl Pts',(46.5766932247459,-56.2810644399698,
-39.1725541666667));
#266652=CARTESIAN_POINT('Ctrl Pts',(45.5423228415332,-55.6838704207802,
-39.1142208333333));
#266653=CARTESIAN_POINT('Ctrl Pts',(44.5079524583205,-55.0866764015906,
-39.0558875));
#266654=CARTESIAN_POINT('Ctrl Pts',(43.4735820751078,-55.6838704207802,
-38.9975541666667));
#266655=CARTESIAN_POINT('Ctrl Pts',(42.4392116918951,-56.2810644399698,
-38.9392208333334));
#266656=CARTESIAN_POINT('Ctrl Pts',(42.439211691895,-57.4754524783491,-38.8808875));
#266657=CARTESIAN_POINT('Ctrl Pts',(42.4392116918951,-58.6698405167284,
-38.8225541666667));
#266658=CARTESIAN_POINT('Ctrl Pts',(43.4735820751078,-59.267034535918,-38.7642208333333));
#266659=CARTESIAN_POINT('Ctrl Pts',(44.5079524583205,-59.8642285551076,
-38.7058875));
#266660=CARTESIAN_POINT('Ctrl Pts',(45.5423228415332,-59.267034535918,-38.6475541666667));
#266661=CARTESIAN_POINT('Ctrl Pts',(46.5766932247459,-58.6698405167284,
-38.5892208333334));
#266662=CARTESIAN_POINT('Ctrl Pts',(46.5766932247459,-57.4754524783491,
-38.5308875));
#266663=CARTESIAN_POINT('Ctrl Pts',(46.5766932247459,-56.2810644399698,
-38.4725541666667));
#266664=CARTESIAN_POINT('Ctrl Pts',(45.5423228415332,-55.6838704207802,
-38.4142208333334));
#266665=CARTESIAN_POINT('Ctrl Pts',(44.5079524583205,-55.0866764015906,
-38.3558875));
#266666=CARTESIAN_POINT('Ctrl Pts',(43.4735820751078,-55.6838704207802,
-38.2975541666667));
#266667=CARTESIAN_POINT('Ctrl Pts',(42.4392116918951,-56.2810644399698,
-38.2392208333333));
#266668=CARTESIAN_POINT('Ctrl Pts',(42.439211691895,-57.4754524783491,-38.1808875000001));
#266669=CARTESIAN_POINT('Ctrl Pts',(42.4392116918951,-58.6698405167284,
-38.1225541666667));
#266670=CARTESIAN_POINT('Ctrl Pts',(43.4735820751078,-59.267034535918,-38.0642208333334));
#266671=CARTESIAN_POINT('Ctrl Pts',(44.5079524583205,-59.8642285551076,
-38.0058875));
#266672=CARTESIAN_POINT('Ctrl Pts',(45.5423228415332,-59.267034535918,-37.9475541666667));
#266673=CARTESIAN_POINT('Ctrl Pts',(46.5766932247459,-58.6698405167284,
-37.8892208333334));
#266674=CARTESIAN_POINT('Ctrl Pts',(46.5766932247459,-57.4754524783491,
-37.8308875));
#266675=CARTESIAN_POINT('Ctrl Pts',(46.5766932247459,-56.2810644399698,
-37.7725541666667));
#266676=CARTESIAN_POINT('Ctrl Pts',(45.5423228415332,-55.6838704207802,
-37.7142208333333));
#266677=CARTESIAN_POINT('Ctrl Pts',(44.5079524583205,-55.0866764015906,
-37.6558875));
#266678=CARTESIAN_POINT('Ctrl Pts',(43.4735820751078,-55.6838704207802,
-37.5975541666667));
#266679=CARTESIAN_POINT('Ctrl Pts',(42.4392116918951,-56.2810644399698,
-37.5392208333334));
#266680=CARTESIAN_POINT('Ctrl Pts',(42.439211691895,-57.4754524783491,-37.4808875));
#266681=CARTESIAN_POINT('Ctrl Pts',(42.4392116918951,-58.6698405167284,
-37.4225541666667));
#266682=CARTESIAN_POINT('Ctrl Pts',(43.4735820751078,-59.267034535918,-37.3642208333333));
#266683=CARTESIAN_POINT('Ctrl Pts',(44.5079524583205,-59.8642285551076,
-37.3058875));
#266684=CARTESIAN_POINT('Ctrl Pts',(45.5423228415332,-59.267034535918,-37.2475541666667));
#266685=CARTESIAN_POINT('Ctrl Pts',(45.6766168155006,-59.1894998738974,
-37.239980655983));
#266686=CARTESIAN_POINT('Ctrl Pts',(45.7978513037526,-59.0928112286649,
-37.2318399189827));
#266687=CARTESIAN_POINT('Ctrl Pts',(43.6172881206077,-58.9566576914661,
-39.9695117808943));
#266688=CARTESIAN_POINT('Ctrl Pts',(43.5704358934015,-58.9167725422626,
-39.9673012254286));
#266689=CARTESIAN_POINT('Ctrl Pts',(43.5257501710543,-58.8744832367377,
-39.9652307185737));
#266690=CARTESIAN_POINT('Ctrl Pts',(43.4408839869852,-58.7852840277194,
-39.9614099505568));
#266691=CARTESIAN_POINT('Ctrl Pts',(43.4008519842798,-58.7385284518944,
-39.9596661889691));
#266692=CARTESIAN_POINT('Ctrl Pts',(43.3633213057583,-58.68975488891,-39.9581073773016));
#266693=CARTESIAN_POINT('Origin',(-44.5079524583208,31.5404524382925,235.35105));
#266694=CARTESIAN_POINT('Origin',(44.5079524583208,31.5404524382925,235.35105));
#266695=CARTESIAN_POINT('Ctrl Pts',(46.2910031021108,32.4463941591995,-40.0133516425908));
#266696=CARTESIAN_POINT('Ctrl Pts',(46.2112828672414,32.6032974266246,-40.0284757239348));
#266697=CARTESIAN_POINT('Ctrl Pts',(46.1110474718835,32.7492894385726,-40.037425339261));
#266698=CARTESIAN_POINT('Ctrl Pts',(45.8745943899832,33.0112912763438,-40.042424287837));
#266699=CARTESIAN_POINT('Ctrl Pts',(45.7398389097727,33.1258434240995,-40.0384792740748));
#266700=CARTESIAN_POINT('Ctrl Pts',(45.443656638496,33.3168393914108,-40.0178747536464));
#266701=CARTESIAN_POINT('Ctrl Pts',(45.2839784166729,33.3920654111451,-40.0013399168391));
#266702=CARTESIAN_POINT('Ctrl Pts',(44.9497236580564,33.498953691193,-39.9566891255367));
#266703=CARTESIAN_POINT('Ctrl Pts',(44.7767592325017,33.5299421883571,-39.9287648350382));
#266704=CARTESIAN_POINT('Ctrl Pts',(44.6028100209088,33.538201682522,-39.8960596555963));
#266705=CARTESIAN_POINT('Origin',(0.,-12.9675000200281,-37.9059960127943));
#266706=CARTESIAN_POINT('Ctrl Pts',(-43.4805771074159,-59.5712767529304,
-39.2399080357012));
#266707=CARTESIAN_POINT('Ctrl Pts',(-43.4478249141681,-59.5535603946867,
-39.2311075445953));
#266708=CARTESIAN_POINT('Ctrl Pts',(-43.4156056040519,-59.5351038997391,
-39.2222635806238));
#266709=CARTESIAN_POINT('Ctrl Pts',(-43.3522169440986,-59.4967328580069,
-39.2044893908274));
#266710=CARTESIAN_POINT('Ctrl Pts',(-43.3210476458595,-59.4768182391239,
-39.1955591618115));
#266711=CARTESIAN_POINT('Ctrl Pts',(-43.2291022595543,-59.4149049130521,
-39.1686393287622));
#266712=CARTESIAN_POINT('Ctrl Pts',(-43.1698853587931,-59.3707413041733,
-39.1505208045068));
#266713=CARTESIAN_POINT('Ctrl Pts',(-43.0556331620037,-59.2766097614945,
-39.113935063243));
#266714=CARTESIAN_POINT('Ctrl Pts',(-43.0005921597408,-59.2266373021163,
-39.0954660506179));
#266715=CARTESIAN_POINT('Ctrl Pts',(-42.8948534568781,-59.1207134074407,
-39.0581733199915));
#266716=CARTESIAN_POINT('Ctrl Pts',(-42.8449960553599,-59.0656056508999,
-39.0396463059707));
#266717=CARTESIAN_POINT('Ctrl Pts',(-42.7510811208719,-58.9512122276158,
-39.0028139665663));
#266718=CARTESIAN_POINT('Ctrl Pts',(-42.7070288152267,-58.891930638621,
-38.9845102727346));
#266719=CARTESIAN_POINT('Ctrl Pts',(-42.6452866349949,-58.7998958734659,
-38.957224077988));
#266720=CARTESIAN_POINT('Ctrl Pts',(-42.625429767352,-58.7686980621887,
-38.9481569597938));
#266721=CARTESIAN_POINT('Ctrl Pts',(-42.5871756130002,-58.7052546833099,
-38.9300801552924));
#266722=CARTESIAN_POINT('Ctrl Pts',(-42.568778253032,-58.6730091686672,
-38.9210704649552));
#266723=CARTESIAN_POINT('Ctrl Pts',(-42.5334651880811,-58.6074543754265,
-38.9031098981675));
#266724=CARTESIAN_POINT('Ctrl Pts',(-42.5165536369311,-58.5741539171446,
-38.8941613358138));
#266725=CARTESIAN_POINT('Ctrl Pts',(-42.4842288567228,-58.5064298632496,
-38.8763157156907));
#266726=CARTESIAN_POINT('Ctrl Pts',(-42.4689425396028,-58.4722695523732,
-38.8674882509199));
#266727=CARTESIAN_POINT('Ctrl Pts',(-42.4401223815193,-58.4034275140121,
-38.8500385014136));
#266728=CARTESIAN_POINT('Ctrl Pts',(-42.426583050894,-58.3687341967778,
-38.8414131698514));
#266729=CARTESIAN_POINT('Ctrl Pts',(-42.4012287918448,-58.2988104271035,
-38.824360868638));
#266730=CARTESIAN_POINT('Ctrl Pts',(-42.3894137611201,-58.2635796188005,
-38.8159338161007));
#266731=CARTESIAN_POINT('Ctrl Pts',(-42.3565461207186,-58.1570828582558,
-38.7909502725479));
#266732=CARTESIAN_POINT('Ctrl Pts',(-42.3380647902547,-58.0850119200903,
-38.7746901633276));
#266733=CARTESIAN_POINT('Ctrl Pts',(-42.3155659796374,-57.9752818499468,
-38.7509105250088));
#266734=CARTESIAN_POINT('Ctrl Pts',(-42.3089374211558,-57.9384266221928,
-38.7430843922672));
#266735=CARTESIAN_POINT('Ctrl Pts',(-42.297458012674,-57.864178756387,-38.7276438637217));
#266736=CARTESIAN_POINT('Ctrl Pts',(-42.292601515188,-57.8267325312259,
-38.720018782004));
#266737=CARTESIAN_POINT('Ctrl Pts',(-42.2847289916893,-57.7514526301959,
-38.7050196673962));
#266738=CARTESIAN_POINT('Ctrl Pts',(-42.2817363521424,-57.7138759968928,
-38.6976962453237));
#266739=CARTESIAN_POINT('Ctrl Pts',(-42.277596992864,-57.6387184974263,
-38.6833720377019));
#266740=CARTESIAN_POINT('Ctrl Pts',(-42.2764525301716,-57.6011593077097,
-38.6763755686054));
#266741=CARTESIAN_POINT('Ctrl Pts',(-42.2757726188108,-57.4885396176673,
-38.6558809641879));
#266742=CARTESIAN_POINT('Ctrl Pts',(-42.2789845428693,-57.4135368708757,
-38.6428765167438));
#266743=CARTESIAN_POINT('Ctrl Pts',(-42.289333314243,-57.3011476810195,
-38.6243712990017));
#266744=CARTESIAN_POINT('Ctrl Pts',(-42.2937061680812,-57.2637038035873,
-38.618370061439));
#266745=CARTESIAN_POINT('Ctrl Pts',(-42.3043247017591,-57.1888547452426,
-38.6067079534822));
#266746=CARTESIAN_POINT('Ctrl Pts',(-42.3105743117123,-57.1514345461221,
-38.6010450635964));
#266747=CARTESIAN_POINT('Ctrl Pts',(-42.3249704170347,-57.0766935209606,
-38.590076215021));
#266748=CARTESIAN_POINT('Ctrl Pts',(-42.3331592025312,-57.0392159768686,
-38.5847494243559));
#266749=CARTESIAN_POINT('Ctrl Pts',(-42.3512949844302,-56.9651221381903,
-38.5745673038812));
#266750=CARTESIAN_POINT('Ctrl Pts',(-42.3612586135401,-56.9283882021117,
-38.5696936317377));
#266751=CARTESIAN_POINT('Ctrl Pts',(-42.3829467968515,-56.8555905655333,
-38.5603848033813));
#266752=CARTESIAN_POINT('Ctrl Pts',(-42.3946724551093,-56.8195179901625,
-38.555948235663));
#266753=CARTESIAN_POINT('Ctrl Pts',(-42.4198760714445,-56.7480212016901,
-38.5475092141337));
#266754=CARTESIAN_POINT('Ctrl Pts',(-42.4333540386586,-56.712596992043,
-38.5435067618884));
#266755=CARTESIAN_POINT('Ctrl Pts',(-42.4620643651744,-56.6423976051736,
-38.5359375083953));
#266756=CARTESIAN_POINT('Ctrl Pts',(-42.4772967069948,-56.6076224215361,
-38.5323707022785));
#266757=CARTESIAN_POINT('Ctrl Pts',(-42.5095308031841,-56.5387265502116,
-38.5256774075877));
#266758=CARTESIAN_POINT('Ctrl Pts',(-42.5265325119253,-56.5046058456765,
-38.5225509073062));
#266759=CARTESIAN_POINT('Ctrl Pts',(-42.5623338475307,-56.4370293947696,
-38.5167461666044));
#266760=CARTESIAN_POINT('Ctrl Pts',(-42.5811223641794,-56.4035923099625,
-38.5140693065785));
#266761=CARTESIAN_POINT('Ctrl Pts',(-42.620584523009,-56.3373241998654,
-38.5091697400817));
#266762=CARTESIAN_POINT('Ctrl Pts',(-42.6411082254821,-56.3047465904101,
-38.5069659500128));
#266763=CARTESIAN_POINT('Ctrl Pts',(-42.7048067991197,-56.2090283357163,
-38.5011108589349));
#266764=CARTESIAN_POINT('Ctrl Pts',(-42.7502234543428,-56.1476408662828,
-38.4981890389281));
#266765=CARTESIAN_POINT('Ctrl Pts',(-42.846794232383,-56.0297655581676,
-38.4942910511032));
#266766=CARTESIAN_POINT('Ctrl Pts',(-42.8979715413934,-55.9732420482177,
-38.4933125989996));
#266767=CARTESIAN_POINT('Ctrl Pts',(-42.9790570553346,-55.8921695883032,
-38.4933149859728));
#266768=CARTESIAN_POINT('Ctrl Pts',(-43.0068374106561,-55.8657400908869,
-38.4935622007431));
#266769=CARTESIAN_POINT('Ctrl Pts',(-43.0495800649421,-55.8270637749536,
-38.4943063068789));
#266770=CARTESIAN_POINT('Ctrl Pts',(-43.0640222060113,-55.8143203511958,
-38.494617152342));
#266771=CARTESIAN_POINT('Ctrl Pts',(-43.0932714774893,-55.7891564261061,
-38.4953646906773));
#266772=CARTESIAN_POINT('Ctrl Pts',(-43.1080901283633,-55.7767277938553,
-38.4958020036096));
#266773=CARTESIAN_POINT('Ctrl Pts',(-43.1528523310046,-55.7401327167866,
-38.4972962980169));
#266774=CARTESIAN_POINT('Ctrl Pts',(-43.183171240984,-55.7165901373356,
-38.498536032863));
#266775=CARTESIAN_POINT('Ctrl Pts',(-43.2447583556422,-55.6711691509155,
-38.5014931332815));
#266776=CARTESIAN_POINT('Ctrl Pts',(-43.2760240909102,-55.6492920896315,
-38.5032102926999));
#266777=CARTESIAN_POINT('Ctrl Pts',(-43.37121764534,-55.5861255243223,-38.5090666584048));
#266778=CARTESIAN_POINT('Ctrl Pts',(-43.4365388292261,-55.5472953809443,
-38.5139093068404));
#266779=CARTESIAN_POINT('Ctrl Pts',(-43.5372923455653,-55.4939420631336,
-38.5225684468354));
#266780=CARTESIAN_POINT('Ctrl Pts',(-43.5713395927683,-55.4769743237494,
-38.5256877381308));
#266781=CARTESIAN_POINT('Ctrl Pts',(-43.6403672861995,-55.4446857735354,
-38.5323951500278));
#266782=CARTESIAN_POINT('Ctrl Pts',(-43.6753577685123,-55.4293620157832,
-38.5359845633874));
#266783=CARTESIAN_POINT('Ctrl Pts',(-43.7462462065787,-55.4003985583156,
-38.5436333065981));
#266784=CARTESIAN_POINT('Ctrl Pts',(-43.7822717759725,-55.3867204456352,
-38.5477088862383));
#266785=CARTESIAN_POINT('Ctrl Pts',(-43.8543821738219,-55.3613797848081,
-38.5562346427693));
#266786=CARTESIAN_POINT('Ctrl Pts',(-43.890622407919,-55.349649082917,-38.5607007444526));
#266787=CARTESIAN_POINT('Ctrl Pts',(-43.9633781832422,-55.3280633380684,
-38.5700204086244));
#266788=CARTESIAN_POINT('Ctrl Pts',(-43.9999084022592,-55.3182019076378,
-38.5748754846743));
#266789=CARTESIAN_POINT('Ctrl Pts',(-44.0732691651704,-55.300314394282,
-38.5849692074244));
#266790=CARTESIAN_POINT('Ctrl Pts',(-44.1100997159262,-55.2922883538608,
-38.590207863671));
#266791=CARTESIAN_POINT('Ctrl Pts',(-44.1840590812038,-55.2780579645929,
-38.6010647047639));
#266792=CARTESIAN_POINT('Ctrl Pts',(-44.2211878979616,-55.2718536300564,
-38.6066828933265));
#266793=CARTESIAN_POINT('Ctrl Pts',(-44.2957439071301,-55.2612662316006,
-38.6182974837333));
#266794=CARTESIAN_POINT('Ctrl Pts',(-44.3331710973477,-55.256883155031,
-38.624293883757));
#266795=CARTESIAN_POINT('Ctrl Pts',(-44.4083261383181,-55.2499510742625,
-38.6366662922177));
#266796=CARTESIAN_POINT('Ctrl Pts',(-44.446056048267,-55.2474029004138,
-38.6430428201589));
#266797=CARTESIAN_POINT('Ctrl Pts',(-44.5218128020516,-55.2441636366351,
-38.6561775645199));
#266798=CARTESIAN_POINT('Ctrl Pts',(-44.5599089424743,-55.2434808562086,
-38.6629497802385));
#266799=CARTESIAN_POINT('Ctrl Pts',(-44.6354869543582,-55.2439911084578,
-38.6767130108817));
#266800=CARTESIAN_POINT('Ctrl Pts',(-44.6731456892459,-55.2451740103824,
-38.6837342374529));
#266801=CARTESIAN_POINT('Ctrl Pts',(-44.7481014788608,-55.2493620066237,
-38.6980304684339));
#266802=CARTESIAN_POINT('Ctrl Pts',(-44.7854165850557,-55.2523662274994,
-38.7053085862828));
#266803=CARTESIAN_POINT('Ctrl Pts',(-44.8968808056053,-55.2640710758905,
-38.7275256543264));
#266804=CARTESIAN_POINT('Ctrl Pts',(-44.9705498158105,-55.2754583368831,
-38.7428465194087));
#266805=CARTESIAN_POINT('Ctrl Pts',(-45.0801001998238,-55.2978810544009,
-38.7665804202115));
#266806=CARTESIAN_POINT('Ctrl Pts',(-45.1164578754129,-55.3062470656085,
-38.7746173707339));
#266807=CARTESIAN_POINT('Ctrl Pts',(-45.1888527653151,-55.3247763762561,
-38.790943453482));
#266808=CARTESIAN_POINT('Ctrl Pts',(-45.2248832056965,-55.3349380951144,
-38.7992310848652));
#266809=CARTESIAN_POINT('Ctrl Pts',(-45.2966462681613,-55.3570913336823,
-38.8160672125853));
#266810=CARTESIAN_POINT('Ctrl Pts',(-45.3323638946335,-55.3690863290504,
-38.8246135819642));
#266811=CARTESIAN_POINT('Ctrl Pts',(-45.4027951436545,-55.3946744461232,
-38.841798196801));
#266812=CARTESIAN_POINT('Ctrl Pts',(-45.4376370321487,-55.4083060218429,
-38.85046633842));
#266813=CARTESIAN_POINT('Ctrl Pts',(-45.506502018173,-55.4372015589607,
-38.8679331631116));
#266814=CARTESIAN_POINT('Ctrl Pts',(-45.5405385021803,-55.4524695986684,
-38.8767349781349));
#266815=CARTESIAN_POINT('Ctrl Pts',(-45.6078227545407,-55.4846397884908,
-38.8944741574428));
#266816=CARTESIAN_POINT('Ctrl Pts',(-45.6410705220065,-55.501541940162,
-38.9034115223487));
#266817=CARTESIAN_POINT('Ctrl Pts',(-45.6739227574752,-55.5192637582493,
-38.9124165669282));
#266818=CARTESIAN_POINT('Ctrl Pts',(45.6739227548717,-55.5192637629147,
-38.9124165672461));
#266819=CARTESIAN_POINT('Ctrl Pts',(45.9463033563028,-55.6661968728795,
-38.9870781453929));
#266820=CARTESIAN_POINT('Ctrl Pts',(46.1858267356293,-55.8663975819995,
-39.0648125841885));
#266821=CARTESIAN_POINT('Ctrl Pts',(46.5670747159648,-56.3440390221876,
-39.2155227881245));
#266822=CARTESIAN_POINT('Ctrl Pts',(46.7077569552424,-56.6157479841383,
-39.2873405177034));
#266823=CARTESIAN_POINT('Ctrl Pts',(46.8732483280237,-57.193117527531,-39.4159630591699));
#266824=CARTESIAN_POINT('Ctrl Pts',(46.8994629299653,-57.491836002201,-39.4718422136366));
#266825=CARTESIAN_POINT('Ctrl Pts',(46.8361488789456,-58.0797309112136,
-39.5617425029226));
#266826=CARTESIAN_POINT('Ctrl Pts',(46.7497210582493,-58.3628620872618,
-39.5952773538707));
#266827=CARTESIAN_POINT('Ctrl Pts',(46.4731716121117,-58.8837138814873,
-39.6368897595136));
#266828=CARTESIAN_POINT('Ctrl Pts',(46.2860677203498,-59.1155468740635,
-39.6444848425935));
#266829=CARTESIAN_POINT('Ctrl Pts',(45.8355505681189,-59.4949344949909,
-39.6323858167165));
#266830=CARTESIAN_POINT('Ctrl Pts',(45.5779522357561,-59.6388002274368,
-39.6130511192697));
#266831=CARTESIAN_POINT('Ctrl Pts',(45.0213200602056,-59.8236634709355,
-39.5495917659915));
#266832=CARTESIAN_POINT('Ctrl Pts',(44.7274799400336,-59.8615367970039,
-39.505809377011));
#266833=CARTESIAN_POINT('Ctrl Pts',(44.2690495794481,-59.8339566709351,
-39.4221844653343));
#266834=CARTESIAN_POINT('Ctrl Pts',(44.1034036286098,-59.805591449331,-39.3887143293807));
#266835=CARTESIAN_POINT('Ctrl Pts',(43.7818822384013,-59.7136905694733,
-39.3171340045734));
#266836=CARTESIAN_POINT('Ctrl Pts',(43.6270995967251,-59.6505338853945,
-39.2792785244787));
#266837=CARTESIAN_POINT('Ctrl Pts',(43.4805771074156,-59.571276752931,-39.2399080357013));
#266838=CARTESIAN_POINT('Ctrl Pts',(42.4577131944625,32.5104083279571,-38.8606823233882));
#266839=CARTESIAN_POINT('Ctrl Pts',(42.5764874766347,32.7913026701199,-38.9320840733657));
#266840=CARTESIAN_POINT('Ctrl Pts',(42.7498620817929,33.045230719566,-39.0079063692694));
#266841=CARTESIAN_POINT('Ctrl Pts',(43.1829971873387,33.4691717941986,-39.1588503042595));
#266842=CARTESIAN_POINT('Ctrl Pts',(43.4403467231087,33.6371317127336,-39.2331900309774));
#266843=CARTESIAN_POINT('Ctrl Pts',(44.0001699490351,33.8600656882486,-39.3691508264002));
#266844=CARTESIAN_POINT('Ctrl Pts',(44.2964171622572,33.9159480336448,-39.4298820593753));
#266845=CARTESIAN_POINT('Ctrl Pts',(44.8897972396321,33.9103079782275,-39.5308335555166));
#266846=CARTESIAN_POINT('Ctrl Pts',(45.1806764898647,33.8516842141669,-39.5705004520691));
#266847=CARTESIAN_POINT('Ctrl Pts',(45.727470817634,33.6260302804986,-39.6252622695383));
#266848=CARTESIAN_POINT('Ctrl Pts',(45.9772544322443,33.4613850473092,-39.6397263367521));
#266849=CARTESIAN_POINT('Ctrl Pts',(46.3987893110107,33.0478618141268,-39.6410888152754));
#266850=CARTESIAN_POINT('Ctrl Pts',(46.5666649958226,32.8049268459807,-39.6283385881241));
#266851=CARTESIAN_POINT('Ctrl Pts',(46.8034309450006,32.2681230437893,-39.5771908821506));
#266852=CARTESIAN_POINT('Ctrl Pts',(46.8689681641379,31.9798098532618,-39.539160660217));
#266853=CARTESIAN_POINT('Ctrl Pts',(46.8852106261357,31.5204813293332,-39.4631024925703));
#266854=CARTESIAN_POINT('Ctrl Pts',(46.8726727347044,31.3524538143514,-39.4320349173607));
#266855=CARTESIAN_POINT('Ctrl Pts',(46.8115489554923,31.0230026598069,-39.3646022158351));
#266856=CARTESIAN_POINT('Ctrl Pts',(46.7632492070739,30.8626951466146,-39.3284790845633));
#266857=CARTESIAN_POINT('Ctrl Pts',(46.6981266849492,30.7091523375488,-39.2904704603133));
#266858=CARTESIAN_POINT('Ctrl Pts',(-46.6981266849484,30.7091523375492,
-39.2904704603132));
#266859=CARTESIAN_POINT('Ctrl Pts',(-46.6835475486277,30.6747783378881,
-39.2819613777041));
#266860=CARTESIAN_POINT('Ctrl Pts',(-46.6681814960651,30.6408774263401,
-39.2733909118473));
#266861=CARTESIAN_POINT('Ctrl Pts',(-46.6359019229579,30.57400615396,-39.2561284882363));
#266862=CARTESIAN_POINT('Ctrl Pts',(-46.618988316466,30.5410358444554,-39.2474365250187));
#266863=CARTESIAN_POINT('Ctrl Pts',(-46.5659489383047,30.443507428437,-39.2211791249421));
#266864=CARTESIAN_POINT('Ctrl Pts',(-46.5275294393937,30.3803289376591,
-39.2034325264408));
#266865=CARTESIAN_POINT('Ctrl Pts',(-46.4653031952286,30.2883271671429,
-39.1764461222039));
#266866=CARTESIAN_POINT('Ctrl Pts',(-46.4437937583117,30.2581216171786,
-39.1673894861782));
#266867=CARTESIAN_POINT('Ctrl Pts',(-46.3992224148768,30.1986447451181,
-39.1491520227249));
#266868=CARTESIAN_POINT('Ctrl Pts',(-46.3761748773305,30.1693908446446,
-39.1399767764946));
#266869=CARTESIAN_POINT('Ctrl Pts',(-46.3284414024809,30.1117648114072,
-39.1214771434543));
#266870=CARTESIAN_POINT('Ctrl Pts',(-46.3038983378397,30.083571828401,-39.112209259666));
#266871=CARTESIAN_POINT('Ctrl Pts',(-46.2537073876081,30.0286632749651,
-39.0937226519629));
#266872=CARTESIAN_POINT('Ctrl Pts',(-46.2280147026909,30.001893564456,-39.0844865568113));
#266873=CARTESIAN_POINT('Ctrl Pts',(-46.1492148010453,29.9236586721517,
-39.0568159196779));
#266874=CARTESIAN_POINT('Ctrl Pts',(-46.0943603797766,29.8742287883655,
-39.0384077341064));
#266875=CARTESIAN_POINT('Ctrl Pts',(-46.0086385356025,29.8041510538917,
-39.0108577119752));
#266876=CARTESIAN_POINT('Ctrl Pts',(-45.979489670606,29.7814700298992,-39.0016845404958));
#266877=CARTESIAN_POINT('Ctrl Pts',(-45.9200349130685,29.737472830651,-38.9833588596733));
#266878=CARTESIAN_POINT('Ctrl Pts',(-45.8897290709698,29.7161565962466,
-38.9742063485759));
#266879=CARTESIAN_POINT('Ctrl Pts',(-45.8279451173857,29.6749068346782,
-38.9559225627414));
#266880=CARTESIAN_POINT('Ctrl Pts',(-45.7964751089327,29.6549785818455,
-38.9467936623891));
#266881=CARTESIAN_POINT('Ctrl Pts',(-45.748348603817,29.6261284949947,-38.9331097524421));
#266882=CARTESIAN_POINT('Ctrl Pts',(-45.7321473284057,29.616684052073,-38.9285487676402));
#266883=CARTESIAN_POINT('Ctrl Pts',(-45.6996106203311,29.5982459977232,
-38.9194791520014));
#266884=CARTESIAN_POINT('Ctrl Pts',(-45.683249044345,29.5892352448745,-38.9149628379355));
#266885=CARTESIAN_POINT('Ctrl Pts',(-45.6010439155842,29.5452684013657,
-38.8924942188443));
#266886=CARTESIAN_POINT('Ctrl Pts',(-45.5339074995994,29.5134615304068,
-38.8748432972593));
#266887=CARTESIAN_POINT('Ctrl Pts',(-45.3969715882024,29.4565064940367,
-38.840197135303));
#266888=CARTESIAN_POINT('Ctrl Pts',(-45.3271662939831,29.4313508132015,
-38.823199542964));
#266889=CARTESIAN_POINT('Ctrl Pts',(-45.2204298442793,29.398652641048,-38.7982016720699));
#266890=CARTESIAN_POINT('Ctrl Pts',(-45.184512437616,29.3885937253944,-38.7899522655792));
#266891=CARTESIAN_POINT('Ctrl Pts',(-45.1119891467798,29.3701842541612,
-38.7736235920333));
#266892=CARTESIAN_POINT('Ctrl Pts',(-45.0754052578815,29.3618381514785,
-38.7655490803555));
#266893=CARTESIAN_POINT('Ctrl Pts',(-45.0014447932704,29.3468760834355,
-38.7495561846596));
#266894=CARTESIAN_POINT('Ctrl Pts',(-44.964301863367,29.3403115562353,-38.7416890516424));
#266895=CARTESIAN_POINT('Ctrl Pts',(-44.8900079594565,29.3290481892184,
-38.726277749838));
#266896=CARTESIAN_POINT('Ctrl Pts',(-44.8527936282157,29.324336495618,-38.7187198739728));
#266897=CARTESIAN_POINT('Ctrl Pts',(-44.7410083373266,29.3129455735289,
-38.6964994820139));
#266898=CARTESIAN_POINT('Ctrl Pts',(-44.6662563757167,29.3089967422249,
-38.6822807693139));
#266899=CARTESIAN_POINT('Ctrl Pts',(-44.516312468428,29.3084067934202,-38.6550493453909));
#266900=CARTESIAN_POINT('Ctrl Pts',(-44.441103189525,29.3117700143417,-38.6420342479066));
#266901=CARTESIAN_POINT('Ctrl Pts',(-44.3468378615956,29.3206690055189,
-38.6265520162729));
#266902=CARTESIAN_POINT('Ctrl Pts',(-44.3279589148655,29.3226883315868,
-38.6234933649988));
#266903=CARTESIAN_POINT('Ctrl Pts',(-44.2901960653061,29.3271995080041,
-38.6174591262491));
#266904=CARTESIAN_POINT('Ctrl Pts',(-44.2712743932921,29.329697893027,-38.614477863833));
#266905=CARTESIAN_POINT('Ctrl Pts',(-44.2146592782018,29.3378915995821,
-38.60568558559));
#266906=CARTESIAN_POINT('Ctrl Pts',(-44.1772069502033,29.344266758826,-38.6000392683017));
#266907=CARTESIAN_POINT('Ctrl Pts',(-44.1027653084072,29.3588321594788,
-38.5891549147378));
#266908=CARTESIAN_POINT('Ctrl Pts',(-44.0657945489017,29.3670194960673,
-38.5839197203675));
#266909=CARTESIAN_POINT('Ctrl Pts',(-43.9923490656542,29.3851892021794,
-38.5738612453122));
#266910=CARTESIAN_POINT('Ctrl Pts',(-43.9558743463703,29.395171587473,-38.5690379674556));
#266911=CARTESIAN_POINT('Ctrl Pts',(-43.8834205276403,29.4169303996784,
-38.5598042480103));
#266912=CARTESIAN_POINT('Ctrl Pts',(-43.8474414251675,29.4287068153425,
-38.5553938031715));
#266913=CARTESIAN_POINT('Ctrl Pts',(-43.7759820586595,29.4540658195324,
-38.5469896320335));
#266914=CARTESIAN_POINT('Ctrl Pts',(-43.7405017838471,29.467648368817,-38.5429958961485));
#266915=CARTESIAN_POINT('Ctrl Pts',(-43.6700470477634,29.4966453401303,
-38.5354320983078));
#266916=CARTESIAN_POINT('Ctrl Pts',(-43.6350719757086,29.512061063653,-38.5318621614261));
#266917=CARTESIAN_POINT('Ctrl Pts',(-43.5656410085295,29.5447591316771,
-38.525155654825));
#266918=CARTESIAN_POINT('Ctrl Pts',(-43.5311320054746,29.5620794464364,
-38.5220163122062));
#266919=CARTESIAN_POINT('Ctrl Pts',(-43.4634866412135,29.5981758355574,
-38.5162526847879));
#266920=CARTESIAN_POINT('Ctrl Pts',(-43.4301834663391,29.6170276546,-38.5136117755133));
#266921=CARTESIAN_POINT('Ctrl Pts',(-43.3647025891651,29.6562685687332,
-38.5088155315793));
#266922=CARTESIAN_POINT('Ctrl Pts',(-43.3325078231767,29.6766655539003,
-38.5066585209069));
#266923=CARTESIAN_POINT('Ctrl Pts',(-43.2375484321327,29.7401688861791,
-38.5009063965958));
#266924=CARTESIAN_POINT('Ctrl Pts',(-43.1764049274077,29.7855824582168,
-38.4980286134812));
#266925=CARTESIAN_POINT('Ctrl Pts',(-43.0584774180437,29.8826126224142,
-38.4942050936184));
#266926=CARTESIAN_POINT('Ctrl Pts',(-43.001681818637,29.9342392650769,-38.4932590761897));
#266927=CARTESIAN_POINT('Ctrl Pts',(-42.8926599718677,30.0438904492243,
-38.4933742455196));
#266928=CARTESIAN_POINT('Ctrl Pts',(-42.8414047150844,30.1009342501745,
-38.4944336470273));
#266929=CARTESIAN_POINT('Ctrl Pts',(-42.7451036203247,30.2193471227021,
-38.498479276642));
#266930=CARTESIAN_POINT('Ctrl Pts',(-42.7000684110598,30.2807072617414,
-38.5014658126213));
#266931=CARTESIAN_POINT('Ctrl Pts',(-42.6161769337401,30.4076992015223,
-38.5093469123445));
#266932=CARTESIAN_POINT('Ctrl Pts',(-42.5773225406026,30.4733365238586,
-38.5142428327574));
#266933=CARTESIAN_POINT('Ctrl Pts',(-42.5326943378214,30.5580963840027,
-38.5215739479982));
#266934=CARTESIAN_POINT('Ctrl Pts',(-42.5239673850246,30.5751883092729,
-38.5231018165939));
#266935=CARTESIAN_POINT('Ctrl Pts',(-42.5069121510755,30.60964376351,-38.5262794637242));
#266936=CARTESIAN_POINT('Ctrl Pts',(-42.4985805781952,30.627019094627,-38.5279307934181));
#266937=CARTESIAN_POINT('Ctrl Pts',(-42.4743295471271,30.6792614198295,
-38.5330409224498));
#266938=CARTESIAN_POINT('Ctrl Pts',(-42.4591078049536,30.7143247172706,
-38.5366620777082));
#266939=CARTESIAN_POINT('Ctrl Pts',(-42.4305062721789,30.7849297925434,
-38.5443248028235));
#266940=CARTESIAN_POINT('Ctrl Pts',(-42.4171273618354,30.8204683264523,
-38.5483659418649));
#266941=CARTESIAN_POINT('Ctrl Pts',(-42.3921837112499,30.89200995013,-38.556860031436));
#266942=CARTESIAN_POINT('Ctrl Pts',(-42.3806190180342,30.9280130518798,
-38.5613129931637));
#266943=CARTESIAN_POINT('Ctrl Pts',(-42.3592881563091,31.0004799414626,
-38.5706260903895));
#266944=CARTESIAN_POINT('Ctrl Pts',(-42.3495220063211,31.0369437339595,
-38.5754862307243));
#266945=CARTESIAN_POINT('Ctrl Pts',(-42.3317857495347,31.1103315158532,
-38.5856119737634));
#266946=CARTESIAN_POINT('Ctrl Pts',(-42.3238156343608,31.1472555030051,
-38.5908775753381));
#266947=CARTESIAN_POINT('Ctrl Pts',(-42.3096820427396,31.2215665449467,
-38.6018154236264));
#266948=CARTESIAN_POINT('Ctrl Pts',(-42.3035171869091,31.2589715314082,
-38.6074906718877));
#266949=CARTESIAN_POINT('Ctrl Pts',(-42.2930235524414,31.3341791410138,
-38.6192399292287));
#266950=CARTESIAN_POINT('Ctrl Pts',(-42.2886818075092,31.3721585359098,
-38.6253436316658));
#266951=CARTESIAN_POINT('Ctrl Pts',(-42.2819306306109,31.4478003630713,
-38.6378362101326));
#266952=CARTESIAN_POINT('Ctrl Pts',(-42.2795025237186,31.4855414978569,
-38.6442360129219));
#266953=CARTESIAN_POINT('Ctrl Pts',(-42.2765060643256,31.5608485897329,
-38.6573322722499));
#266954=CARTESIAN_POINT('Ctrl Pts',(-42.2759365563455,31.5984178297074,
-38.6640291190605));
#266955=CARTESIAN_POINT('Ctrl Pts',(-42.2769710616629,31.710876916496,-38.6845570305479));
#266956=CARTESIAN_POINT('Ctrl Pts',(-42.2813124759152,31.7855186400122,
-38.698824567557));
#266957=CARTESIAN_POINT('Ctrl Pts',(-42.2932531103751,31.8969906134966,
-38.7210841829084));
#266958=CARTESIAN_POINT('Ctrl Pts',(-42.2981395950573,31.934066030451,-38.7286473545921));
#266959=CARTESIAN_POINT('Ctrl Pts',(-42.3097367777483,32.0080522284017,
-38.7440609732535));
#266960=CARTESIAN_POINT('Ctrl Pts',(-42.3164494406915,32.0449687602613,
-38.7519128032936));
#266961=CARTESIAN_POINT('Ctrl Pts',(-42.3317154579634,32.1186122141692,
-38.7679009120377));
#266962=CARTESIAN_POINT('Ctrl Pts',(-42.3402956643805,32.1554227583218,
-38.7760569897633));
#266963=CARTESIAN_POINT('Ctrl Pts',(-42.3591481714288,32.228169160774,-38.7925026060078));
#266964=CARTESIAN_POINT('Ctrl Pts',(-42.3694448348212,32.2642362896146,
-38.8008201507359));
#266965=CARTESIAN_POINT('Ctrl Pts',(-42.391742799968,32.3356900672865,-38.817625053217));
#266966=CARTESIAN_POINT('Ctrl Pts',(-42.4037465150873,32.3710895326604,
-38.8261151521117));
#266967=CARTESIAN_POINT('Ctrl Pts',(-42.4294540540396,32.4412374294073,
-38.8432687881532));
#266968=CARTESIAN_POINT('Ctrl Pts',(-42.443157884724,32.4759858579956,-38.8519323266277));
#266969=CARTESIAN_POINT('Ctrl Pts',(-42.4577131904514,32.5104083297438,
-38.8606823230314));
#266970=CARTESIAN_POINT('Origin',(0.,-12.9675000200281,-55.24995));
#266971=CARTESIAN_POINT('Ctrl Pts',(43.4805771050572,-59.5712767635336,
-39.239908023115));
#266972=CARTESIAN_POINT('Ctrl Pts',(43.4478249116748,-59.553560405217,-39.231107532009));
#266973=CARTESIAN_POINT('Ctrl Pts',(43.415605601426,-59.5351039101939,-39.2222635680375));
#266974=CARTESIAN_POINT('Ctrl Pts',(43.3522169412117,-59.4967328683047,
-39.2044893782411));
#266975=CARTESIAN_POINT('Ctrl Pts',(43.3210476428442,-59.4768182493402,
-39.1955591492252));
#266976=CARTESIAN_POINT('Ctrl Pts',(43.2291022561607,-59.4149049230149,
-39.1686393161759));
#266977=CARTESIAN_POINT('Ctrl Pts',(43.1698853551558,-59.3707413139551,
-39.1505207919205));
#266978=CARTESIAN_POINT('Ctrl Pts',(43.0556331578966,-59.2766097708902,
-39.1139350506567));
#266979=CARTESIAN_POINT('Ctrl Pts',(43.0005921554074,-59.226637311307,-39.0954660380315));
#266980=CARTESIAN_POINT('Ctrl Pts',(42.8948534521102,-59.1207134161965,
-39.0581733074052));
#266981=CARTESIAN_POINT('Ctrl Pts',(42.8449960503872,-59.0656056594293,
-39.0396462933844));
#266982=CARTESIAN_POINT('Ctrl Pts',(42.7510811155138,-58.9512122356751,
-39.00281395398));
#266983=CARTESIAN_POINT('Ctrl Pts',(42.707028809688,-58.8919306464366,-38.9845102601483));
#266984=CARTESIAN_POINT('Ctrl Pts',(42.6452866292032,-58.799895880903,-38.9572240654017));
#266985=CARTESIAN_POINT('Ctrl Pts',(42.6254297614789,-58.7686980694974,
-38.9481569472075));
#266986=CARTESIAN_POINT('Ctrl Pts',(42.5871756069705,-58.7052546903576,
-38.9300801427061));
#266987=CARTESIAN_POINT('Ctrl Pts',(42.568778246927,-58.6730091755822,-38.9210704523689));
#266988=CARTESIAN_POINT('Ctrl Pts',(42.5334651818316,-58.6074543820717,
-38.9031098855812));
#266989=CARTESIAN_POINT('Ctrl Pts',(42.5165536306125,-58.5741539236527,
-38.8941613232275));
#266990=CARTESIAN_POINT('Ctrl Pts',(42.4842288502722,-58.5064298694789,
-38.8763157031044));
#266991=CARTESIAN_POINT('Ctrl Pts',(42.4689425330898,-58.4722695584619,
-38.8674882383336));
#266992=CARTESIAN_POINT('Ctrl Pts',(42.4401223748888,-58.4034275198172,
-38.8500384888273));
#266993=CARTESIAN_POINT('Ctrl Pts',(42.4265830442083,-58.36873420244,-38.841413157265));
#266994=CARTESIAN_POINT('Ctrl Pts',(42.4012287850559,-58.2988104324777,
-38.8243608560517));
#266995=CARTESIAN_POINT('Ctrl Pts',(42.3894137542831,-58.2635796240295,
-38.8159338035143));
#266996=CARTESIAN_POINT('Ctrl Pts',(42.3565461137483,-58.1570828630459,
-38.7909502599615));
#266997=CARTESIAN_POINT('Ctrl Pts',(42.3380647832096,-58.0850119245834,
-38.7746901507413));
#266998=CARTESIAN_POINT('Ctrl Pts',(42.3155659725018,-57.9752818539874,
-38.7509105124225));
#266999=CARTESIAN_POINT('Ctrl Pts',(42.3089374139936,-57.9384266260814,
-38.7430843796809));
#267000=CARTESIAN_POINT('Ctrl Pts',(42.297458005466,-57.8641787599694,-38.7276438511353));
#267001=CARTESIAN_POINT('Ctrl Pts',(42.2926015079608,-57.8267325346538,
-38.7200187694177));
#267002=CARTESIAN_POINT('Ctrl Pts',(42.2847289844313,-57.7514526333132,
-38.7050196548099));
#267003=CARTESIAN_POINT('Ctrl Pts',(42.2817363448728,-57.7138759998551,
-38.6976962327374));
#267004=CARTESIAN_POINT('Ctrl Pts',(42.277596985579,-57.6387185000784,-38.6833720251155));
#267005=CARTESIAN_POINT('Ctrl Pts',(42.2764525228827,-57.6011593102068,
-38.6763755560191));
#267006=CARTESIAN_POINT('Ctrl Pts',(42.2757726115216,-57.4885396196995,
-38.6558809516015));
#267007=CARTESIAN_POINT('Ctrl Pts',(42.278984535595,-57.4135368725982,-38.6428765041575));
#267008=CARTESIAN_POINT('Ctrl Pts',(42.289333307014,-57.3011476822778,-38.6243712864154));
#267009=CARTESIAN_POINT('Ctrl Pts',(42.2937061608711,-57.2637038046909,
-38.6183700488527));
#267010=CARTESIAN_POINT('Ctrl Pts',(42.3043246945944,-57.188854746037,-38.6067079408958));
#267011=CARTESIAN_POINT('Ctrl Pts',(42.3105743045743,-57.1514345467618,
-38.6010450510101));
#267012=CARTESIAN_POINT('Ctrl Pts',(42.3249704099578,-57.0766935212914,
-38.5900762024347));
#267013=CARTESIAN_POINT('Ctrl Pts',(42.333159195489,-57.0392159770445,-38.5847494117696));
#267014=CARTESIAN_POINT('Ctrl Pts',(42.3512949774645,-56.9651221380599,
-38.5745672912949));
#267015=CARTESIAN_POINT('Ctrl Pts',(42.3612586066164,-56.9283882018294,
-38.5696936191514));
#267016=CARTESIAN_POINT('Ctrl Pts',(42.382946790019,-56.85559056495,-38.560384790795));
#267017=CARTESIAN_POINT('Ctrl Pts',(42.394672448326,-56.81951798943,-38.5559482230767));
#267018=CARTESIAN_POINT('Ctrl Pts',(42.419876064767,-56.7480212006618,-38.5475092015474));
#267019=CARTESIAN_POINT('Ctrl Pts',(42.4333540320375,-56.7125969908682,
-38.543506749302));
#267020=CARTESIAN_POINT('Ctrl Pts',(42.4620643586734,-56.6423976037083,
-38.5359374958091));
#267021=CARTESIAN_POINT('Ctrl Pts',(42.4772967005576,-56.6076224199269,
-38.5323706896922));
#267022=CARTESIAN_POINT('Ctrl Pts',(42.5095307968816,-56.5387265483172,
-38.5256773950013));
#267023=CARTESIAN_POINT('Ctrl Pts',(42.5265325056937,-56.5046058436408,
-38.5225508947199));
#267024=CARTESIAN_POINT('Ctrl Pts',(42.5623338414485,-56.4370293924541,
-38.5167461540181));
#267025=CARTESIAN_POINT('Ctrl Pts',(42.5811223581755,-56.4035923075085,
-38.5140692939922));
#267026=CARTESIAN_POINT('Ctrl Pts',(42.6205845171696,-56.3373241971369,
-38.5091697274954));
#267027=CARTESIAN_POINT('Ctrl Pts',(42.6411082197283,-56.3047465875466,
-38.5069659374265));
#267028=CARTESIAN_POINT('Ctrl Pts',(42.704806793631,-56.2090283324561,-38.5011108463486));
#267029=CARTESIAN_POINT('Ctrl Pts',(42.7502234490431,-56.1476408627681,
-38.4981890263418));
#267030=CARTESIAN_POINT('Ctrl Pts',(42.8467942274848,-56.029765554164,-38.4942910385169));
#267031=CARTESIAN_POINT('Ctrl Pts',(42.8979715367077,-55.9732420439795,
-38.4933125864132));
#267032=CARTESIAN_POINT('Ctrl Pts',(42.9790570509856,-55.8921695837284,
-38.4933149733865));
#267033=CARTESIAN_POINT('Ctrl Pts',(43.0068374064224,-55.8657400862024,
-38.4935621881568));
#267034=CARTESIAN_POINT('Ctrl Pts',(43.0495800608858,-55.8270637701084,
-38.4943062942926));
#267035=CARTESIAN_POINT('Ctrl Pts',(43.064022202015,-55.8143203462976,-38.4946171397557));
#267036=CARTESIAN_POINT('Ctrl Pts',(43.0932714736142,-55.7891564211033,
-38.495364678091));
#267037=CARTESIAN_POINT('Ctrl Pts',(43.1080901245497,-55.7767277888009,
-38.4958019910233));
#267038=CARTESIAN_POINT('Ctrl Pts',(43.1528523273767,-55.74013271158,-38.4972962854306));
#267039=CARTESIAN_POINT('Ctrl Pts',(43.1831712374819,-55.7165901320311,
-38.4985360202767));
#267040=CARTESIAN_POINT('Ctrl Pts',(43.2447583523954,-55.6711691454221,
-38.5014931206952));
#267041=CARTESIAN_POINT('Ctrl Pts',(43.276024087793,-55.649292084047,-38.5032102801136));
#267042=CARTESIAN_POINT('Ctrl Pts',(43.3712176426173,-55.5861255184748,
-38.5090666458185));
#267043=CARTESIAN_POINT('Ctrl Pts',(43.436538826774,-55.547295374935,-38.513909294254));
#267044=CARTESIAN_POINT('Ctrl Pts',(43.5372923435304,-55.4939420569017,
-38.5225684342491));
#267045=CARTESIAN_POINT('Ctrl Pts',(43.5713395908744,-55.4769743174466,
-38.5256877255445));
#267046=CARTESIAN_POINT('Ctrl Pts',(43.6403672845913,-55.4446857670977,
-38.5323951374414));
#267047=CARTESIAN_POINT('Ctrl Pts',(43.6753577670489,-55.4293620092815,
-38.535984550801));
#267048=CARTESIAN_POINT('Ctrl Pts',(43.7462462054086,-55.4003985516927,
-38.5436332940118));
#267049=CARTESIAN_POINT('Ctrl Pts',(43.7822717749515,-55.3867204389549,
-38.547708873652));
#267050=CARTESIAN_POINT('Ctrl Pts',(43.8543821730992,-55.3613797780216,
-38.556234630183));
#267051=CARTESIAN_POINT('Ctrl Pts',(43.8906224073461,-55.3496490760812,
-38.5607007318663));
#267052=CARTESIAN_POINT('Ctrl Pts',(43.9633781829702,-55.3280633311418,
-38.570020396038));
#267053=CARTESIAN_POINT('Ctrl Pts',(43.9999084021383,-55.3182019006697,
-38.574875472088));
#267054=CARTESIAN_POINT('Ctrl Pts',(44.0732691653527,-55.3003143872384,
-38.5849691948381));
#267055=CARTESIAN_POINT('Ctrl Pts',(44.1100997162607,-55.2922883467832,
-38.5902078510847));
#267056=CARTESIAN_POINT('Ctrl Pts',(44.1840590818441,-55.2780579574549,
-38.6010646921776));
#267057=CARTESIAN_POINT('Ctrl Pts',(44.2211878987553,-55.2718536228919,
-38.6066828807402));
#267058=CARTESIAN_POINT('Ctrl Pts',(44.2957439082318,-55.2612662243907,
-38.6182974711469));
#267059=CARTESIAN_POINT('Ctrl Pts',(44.333171098604,-55.2568831478022,-38.6242938711707));
#267060=CARTESIAN_POINT('Ctrl Pts',(44.4083261398848,-55.2499510670034,
-38.6366662796313));
#267061=CARTESIAN_POINT('Ctrl Pts',(44.4460560499895,-55.2474028931433,
-38.6430428075725));
#267062=CARTESIAN_POINT('Ctrl Pts',(44.5218128040869,-55.2441636293496,
-38.6561775519336));
#267063=CARTESIAN_POINT('Ctrl Pts',(44.5599089446669,-55.2434808489194,
-38.6629497676522));
#267064=CARTESIAN_POINT('Ctrl Pts',(44.6354869568629,-55.243991101169,-38.6767129982954));
#267065=CARTESIAN_POINT('Ctrl Pts',(44.673145691906,-55.2451740030977,-38.6837342248666));
#267066=CARTESIAN_POINT('Ctrl Pts',(44.7481014818302,-55.2493619993546,
-38.6980304558476));
#267067=CARTESIAN_POINT('Ctrl Pts',(44.785416588179,-55.2523662202419,-38.7053085736965));
#267068=CARTESIAN_POINT('Ctrl Pts',(44.8968808091885,-55.2640710686789,
-38.7275256417401));
#267069=CARTESIAN_POINT('Ctrl Pts',(44.9705498196976,-55.2754583297169,
-38.7428465068224));
#267070=CARTESIAN_POINT('Ctrl Pts',(45.0801002041626,-55.2978810473249,
-38.7665804076252));
#267071=CARTESIAN_POINT('Ctrl Pts',(45.1164578799016,-55.3062470585662,
-38.7746173581476));
#267072=CARTESIAN_POINT('Ctrl Pts',(45.1888527701022,-55.3247763692888,
-38.7909434408956));
#267073=CARTESIAN_POINT('Ctrl Pts',(45.2248832106321,-55.3349380881883,
-38.7992310722789));
#267074=CARTESIAN_POINT('Ctrl Pts',(45.2966462733926,-55.3570913268461,
-38.816067199999));
#267075=CARTESIAN_POINT('Ctrl Pts',(45.332363900012,-55.369086322263,-38.8246135693778));
#267076=CARTESIAN_POINT('Ctrl Pts',(45.4027951493232,-55.3946744394399,
-38.8417981842147));
#267077=CARTESIAN_POINT('Ctrl Pts',(45.4376370379609,-55.4083060152152,
-38.8504663258337));
#267078=CARTESIAN_POINT('Ctrl Pts',(45.5065020242688,-55.4372015524508,
-38.8679331505253));
#267079=CARTESIAN_POINT('Ctrl Pts',(45.5405385084162,-55.4524695922208,
-38.8767349655486));
#267080=CARTESIAN_POINT('Ctrl Pts',(45.6078227610536,-55.4846397821746,
-38.8944741448564));
#267081=CARTESIAN_POINT('Ctrl Pts',(45.6410705286563,-55.5015419339148,
-38.9034115097624));
#267082=CARTESIAN_POINT('Ctrl Pts',(45.7067749946571,-55.5369855795655,
-38.9214215995571));
#267083=CARTESIAN_POINT('Ctrl Pts',(45.7392219948332,-55.5555212054356,
-38.9304915578471));
#267084=CARTESIAN_POINT('Ctrl Pts',(45.8033556905571,-55.5942722101173,
-38.9487787746614));
#267085=CARTESIAN_POINT('Ctrl Pts',(45.8348443765872,-55.6143675254903,
-38.9579394992153));
#267086=CARTESIAN_POINT('Ctrl Pts',(45.9274099921067,-55.6766588970005,
-38.9854159036859));
#267087=CARTESIAN_POINT('Ctrl Pts',(45.9867610946637,-55.720935310253,-39.0037703512016));
#267088=CARTESIAN_POINT('Ctrl Pts',(46.10073379155,-55.8148102344162,-39.0405190740001));
#267089=CARTESIAN_POINT('Ctrl Pts',(46.1553754339886,-55.8644173716091,
-39.0589184790541));
#267090=CARTESIAN_POINT('Ctrl Pts',(46.2338037360394,-55.9428521263115,
-39.0865551832126));
#267091=CARTESIAN_POINT('Ctrl Pts',(46.2593565839205,-55.9696687309655,
-39.0957737053687));
#267092=CARTESIAN_POINT('Ctrl Pts',(46.3092668173353,-56.0246630492642,
-39.1142236288024));
#267093=CARTESIAN_POINT('Ctrl Pts',(46.3336138271979,-56.0528284069633,
-39.1234510369563));
#267094=CARTESIAN_POINT('Ctrl Pts',(46.3692509380672,-56.0961546927766,
-39.1373141611117));
#267095=CARTESIAN_POINT('Ctrl Pts',(46.3809719652397,-56.110765521319,-39.1419350415337));
#267096=CARTESIAN_POINT('Ctrl Pts',(46.4039851066281,-56.1401806678783,
-39.1511314642401));
#267097=CARTESIAN_POINT('Ctrl Pts',(46.415300200194,-56.155012658913,-39.1557159007951));
#267098=CARTESIAN_POINT('Ctrl Pts',(46.4486370196562,-56.1998310026459,
-39.1694131056795));
#267099=CARTESIAN_POINT('Ctrl Pts',(46.4700835192022,-56.2301795284771,
-39.1784825928561));
#267100=CARTESIAN_POINT('Ctrl Pts',(46.5320719239954,-56.322558395602,-39.2054898607661));
#267101=CARTESIAN_POINT('Ctrl Pts',(46.5703036051881,-56.3859631553179,
-39.2232408436738));
#267102=CARTESIAN_POINT('Ctrl Pts',(46.6230137408496,-56.4837650893312,
-39.2494851247746));
#267103=CARTESIAN_POINT('Ctrl Pts',(46.6398105887851,-56.516816729636,-39.2581697915521));
#267104=CARTESIAN_POINT('Ctrl Pts',(46.6718446993975,-56.5838294913527,
-39.2754119059931));
#267105=CARTESIAN_POINT('Ctrl Pts',(46.6870820411944,-56.6177905669658,
-39.283969358867));
#267106=CARTESIAN_POINT('Ctrl Pts',(46.7159729940879,-56.6866360531864,
-39.3009558743285));
#267107=CARTESIAN_POINT('Ctrl Pts',(46.7296188134962,-56.7214992877386,
-39.3093799092323));
#267108=CARTESIAN_POINT('Ctrl Pts',(46.755321710985,-56.7922546374611,-39.3261176515222));
#267109=CARTESIAN_POINT('Ctrl Pts',(46.7672997055706,-56.8279354873648,
-39.3343809661765));
#267110=CARTESIAN_POINT('Ctrl Pts',(46.8004530616987,-56.9353633956067,
-39.3587371504317));
#267111=CARTESIAN_POINT('Ctrl Pts',(46.8189795616622,-57.0077635587484,
-39.374465799535));
#267112=CARTESIAN_POINT('Ctrl Pts',(46.8489162234024,-57.154008095182,-39.4048998164529));
#267113=CARTESIAN_POINT('Ctrl Pts',(46.8603369561858,-57.2278698681474,
-39.4196100455824));
#267114=CARTESIAN_POINT('Ctrl Pts',(46.8720664861652,-57.3397812908466,
-39.4409093514509));
#267115=CARTESIAN_POINT('Ctrl Pts',(46.8750747613607,-57.3772756907765,
-39.4478819258883));
#267116=CARTESIAN_POINT('Ctrl Pts',(46.8792543070635,-57.452637032744,-39.4615663817213));
#267117=CARTESIAN_POINT('Ctrl Pts',(46.8804258854059,-57.4905390852254,
-39.468284348285));
#267118=CARTESIAN_POINT('Ctrl Pts',(46.8808837860862,-57.5666104395958,
-39.4814341834338));
#267119=CARTESIAN_POINT('Ctrl Pts',(46.8801708754895,-57.6044913973763,
-39.4878166551363));
#267120=CARTESIAN_POINT('Ctrl Pts',(46.87689139966,-57.6800598013179,-39.5002231022271));
#267121=CARTESIAN_POINT('Ctrl Pts',(46.8743246754726,-57.7177285021534,
-39.5062438281333));
#267122=CARTESIAN_POINT('Ctrl Pts',(46.8638675798749,-57.8303908466031,
-39.5237649470641));
#267123=CARTESIAN_POINT('Ctrl Pts',(46.8532263770448,-57.905041491034,-39.5347254769916));
#267124=CARTESIAN_POINT('Ctrl Pts',(46.8317335430131,-58.0163268488721,
-39.5500873284662));
#267125=CARTESIAN_POINT('Ctrl Pts',(46.8236459657866,-58.0533066853948,
-39.5550278296908));
#267126=CARTESIAN_POINT('Ctrl Pts',(46.8055990223885,-58.1270324985156,
-39.5645447277516));
#267127=CARTESIAN_POINT('Ctrl Pts',(46.7956339790501,-58.1637938579406,
-39.5691227795573));
#267128=CARTESIAN_POINT('Ctrl Pts',(46.7738161439719,-58.2370162127271,
-39.5779016343018));
#267129=CARTESIAN_POINT('Ctrl Pts',(46.7619036390658,-58.2736352320482,
-39.5821192077603));
#267130=CARTESIAN_POINT('Ctrl Pts',(46.7364059829356,-58.3458256050085,
-39.5900871728599));
#267131=CARTESIAN_POINT('Ctrl Pts',(46.7227943985224,-58.3815079350702,
-39.5938520139967));
#267132=CARTESIAN_POINT('Ctrl Pts',(46.6938810713598,-58.452011863029,-39.6009443748824));
#267133=CARTESIAN_POINT('Ctrl Pts',(46.6785776360953,-58.4868413824451,
-39.6042729587978));
#267134=CARTESIAN_POINT('Ctrl Pts',(46.6462897444841,-58.555661726432,-39.6104989258044));
#267135=CARTESIAN_POINT('Ctrl Pts',(46.6293052752408,-58.5896525446103,
-39.6133963049726));
#267136=CARTESIAN_POINT('Ctrl Pts',(46.5936553637194,-58.6567954655617,
-39.6187605591878));
#267137=CARTESIAN_POINT('Ctrl Pts',(46.5749899342291,-58.689947574739,-39.6212274370902));
#267138=CARTESIAN_POINT('Ctrl Pts',(46.535965754159,-58.7554068805448,-39.6257281208558));
#267139=CARTESIAN_POINT('Ctrl Pts',(46.5156070431754,-58.7877140969356,
-39.627761936622));
#267140=CARTESIAN_POINT('Ctrl Pts',(46.4731710934002,-58.8514710123629,
-39.6313905509331));
#267141=CARTESIAN_POINT('Ctrl Pts',(46.4511086236678,-58.882900639648,-39.6329844474041));
#267142=CARTESIAN_POINT('Ctrl Pts',(46.4051673298575,-58.9449633096445,
-39.6357273359789));
#267143=CARTESIAN_POINT('Ctrl Pts',(46.3814480039077,-58.9753775970138,
-39.6368662472668));
#267144=CARTESIAN_POINT('Ctrl Pts',(46.3084069002845,-59.0643493221119,
-39.6395761107827));
#267145=CARTESIAN_POINT('Ctrl Pts',(46.2570407937254,-59.1209150540827,
-39.6404603658463));
#267146=CARTESIAN_POINT('Ctrl Pts',(46.1491379842615,-59.2285444723307,
-39.6404138688384));
#267147=CARTESIAN_POINT('Ctrl Pts',(46.0925836639483,-59.2796343138351,
-39.639484568582));
#267148=CARTESIAN_POINT('Ctrl Pts',(46.0038529518281,-59.3521266221997,
-39.6367223261665));
#267149=CARTESIAN_POINT('Ctrl Pts',(45.9736068158058,-59.3756113651479,
-39.6355721037165));
#267150=CARTESIAN_POINT('Ctrl Pts',(45.927265703875,-59.4097723645372,-39.6334997599225));
#267151=CARTESIAN_POINT('Ctrl Pts',(45.9116419292403,-59.4209912919482,
-39.6327502683094));
#267152=CARTESIAN_POINT('Ctrl Pts',(45.88008048702,-59.4430610902896,-39.6311351213432));
#267153=CARTESIAN_POINT('Ctrl Pts',(45.864107784879,-59.4539347719282,-39.6302673854466));
#267154=CARTESIAN_POINT('Ctrl Pts',(45.8159067249643,-59.4858696909571,
-39.6274990121292));
#267155=CARTESIAN_POINT('Ctrl Pts',(45.783409718025,-59.5062439066798,-39.6254354946116));
#267156=CARTESIAN_POINT('Ctrl Pts',(45.7176331131415,-59.5452482017306,
-39.6208773136804));
#267157=CARTESIAN_POINT('Ctrl Pts',(45.6843658562672,-59.5638704429234,
-39.6183834165608));
#267158=CARTESIAN_POINT('Ctrl Pts',(45.5834449351778,-59.6171384233149,
-39.610266415423));
#267159=CARTESIAN_POINT('Ctrl Pts',(45.5146744686846,-59.649190882251,-39.6040093823393));
#267160=CARTESIAN_POINT('Ctrl Pts',(45.4093033711364,-59.6921244775619,
-39.5933617190949));
#267161=CARTESIAN_POINT('Ctrl Pts',(45.3738098063667,-59.7055766893281,
-39.5896017780072));
#267162=CARTESIAN_POINT('Ctrl Pts',(45.3020778865304,-59.7307512232088,
-39.5816566699808));
#267163=CARTESIAN_POINT('Ctrl Pts',(45.2658207361194,-59.7424779971954,
-39.5774690525214));
#267164=CARTESIAN_POINT('Ctrl Pts',(45.1926264722126,-59.7641596130402,
-39.5686714999982));
#267165=CARTESIAN_POINT('Ctrl Pts',(45.1555073953157,-59.7741562626731,
-39.564037603403));
#267166=CARTESIAN_POINT('Ctrl Pts',(45.0812568521898,-59.7921790679244,
-39.5544265573043));
#267167=CARTESIAN_POINT('Ctrl Pts',(45.0440817338732,-59.8002278006182,
-39.5494458265502));
#267168=CARTESIAN_POINT('Ctrl Pts',(44.9696261100397,-59.8144410792825,
-39.5391390379963));
#267169=CARTESIAN_POINT('Ctrl Pts',(44.9323469858339,-59.8206061957129,
-39.5338133160118));
#267170=CARTESIAN_POINT('Ctrl Pts',(44.8576879157223,-59.8310833922412,
-39.5228216447761));
#267171=CARTESIAN_POINT('Ctrl Pts',(44.8203079641943,-59.8353953722009,
-39.5171556783342));
#267172=CARTESIAN_POINT('Ctrl Pts',(44.7080184591272,-59.8455760729762,
-39.4996502652144));
#267173=CARTESIAN_POINT('Ctrl Pts',(44.632937227317,-59.8486931739084,-39.4873001735582));
#267174=CARTESIAN_POINT('Ctrl Pts',(44.5200834460945,-59.8478515250362,
-39.4677634677006));
#267175=CARTESIAN_POINT('Ctrl Pts',(44.4823810889441,-59.8466449835469,
-39.461073637211));
#267176=CARTESIAN_POINT('Ctrl Pts',(44.4258051094776,-59.8434394823804,
-39.4507883306211));
#267177=CARTESIAN_POINT('Ctrl Pts',(44.4069254604469,-59.8421361463935,
-39.447314779011));
#267178=CARTESIAN_POINT('Ctrl Pts',(44.3691376555635,-59.8390581742043,
-39.4402793205582));
#267179=CARTESIAN_POINT('Ctrl Pts',(44.3502459363124,-59.8372838851304,
-39.4367202978598));
#267180=CARTESIAN_POINT('Ctrl Pts',(44.2938476179289,-59.8312837006341,
-39.4259706152766));
#267181=CARTESIAN_POINT('Ctrl Pts',(44.2565162770547,-59.8263768713198,
-39.4186892503679));
#267182=CARTESIAN_POINT('Ctrl Pts',(44.1823865429402,-59.8147890323227,
-39.403902149315));
#267183=CARTESIAN_POINT('Ctrl Pts',(44.1455864852429,-59.8081083873803,
-39.3963961932961));
#267184=CARTESIAN_POINT('Ctrl Pts',(44.0359682133432,-59.7854494436508,
-39.3735449791568));
#267185=CARTESIAN_POINT('Ctrl Pts',(43.9639303525491,-59.7668593234827,
-39.3578670253851));
#267186=CARTESIAN_POINT('Ctrl Pts',(43.8219159030999,-59.7227861766851,
-39.3256251105404));
#267187=CARTESIAN_POINT('Ctrl Pts',(43.7519290521664,-59.6972943177331,
-39.3090578161669));
#267188=CARTESIAN_POINT('Ctrl Pts',(43.6657831761406,-59.6610675917225,
-39.2877890362312));
#267189=CARTESIAN_POINT('Ctrl Pts',(43.6486106649973,-59.6535962089239,
-39.2835041155108));
#267190=CARTESIAN_POINT('Ctrl Pts',(43.6144192997846,-59.6382222468611,
-39.2748825057904));
#267191=CARTESIAN_POINT('Ctrl Pts',(43.5973665810138,-59.6303022461252,
-39.2705368798388));
#267192=CARTESIAN_POINT('Ctrl Pts',(43.5465994162094,-59.6059619140424,
-39.257461632632));
#267193=CARTESIAN_POINT('Ctrl Pts',(43.5133292984396,-59.5889931218502,
-39.248708514221));
#267194=CARTESIAN_POINT('Ctrl Pts',(43.4805771050572,-59.5712767635336,
-39.239908023115));
#267195=CARTESIAN_POINT('Ctrl Pts',(43.5555686724225,-59.2341331371673,
-39.6401254388889));
#267196=CARTESIAN_POINT('Ctrl Pts',(43.5271056611467,-59.2187194887567,
-39.631324947783));
#267197=CARTESIAN_POINT('Ctrl Pts',(43.4991050718461,-59.2026631797235,
-39.6224809838115));
#267198=CARTESIAN_POINT('Ctrl Pts',(43.4440150113987,-59.1692845399769,
-39.6047067940149));
#267199=CARTESIAN_POINT('Ctrl Pts',(43.4169255850374,-59.1519621466579,
-39.5957765649991));
#267200=CARTESIAN_POINT('Ctrl Pts',(43.3370131802655,-59.0981112314642,
-39.5688567319499));
#267201=CARTESIAN_POINT('Ctrl Pts',(43.285543194378,-59.0597029400212,-39.5507382076943));
#267202=CARTESIAN_POINT('Ctrl Pts',(43.1862317502577,-58.9778465535662,
-39.5141524664308));
#267203=CARTESIAN_POINT('Ctrl Pts',(43.1383853322497,-58.934394522841,-39.4956834538053));
#267204=CARTESIAN_POINT('Ctrl Pts',(43.04646128557,-58.8422990997139,-39.4583907231793));
#267205=CARTESIAN_POINT('Ctrl Pts',(43.0031141723556,-58.7943892422201,
-39.4398637091582));
#267206=CARTESIAN_POINT('Ctrl Pts',(42.9214551605844,-58.6949439395988,
-39.403031369754));
#267207=CARTESIAN_POINT('Ctrl Pts',(42.8831478057343,-58.6434120405259,
-39.3847276759222));
#267208=CARTESIAN_POINT('Ctrl Pts',(42.8294513147831,-58.5634133385806,
-39.3574414811757));
#267209=CARTESIAN_POINT('Ctrl Pts',(42.8121809030637,-58.5362962456352,
-39.3483743629814));
#267210=CARTESIAN_POINT('Ctrl Pts',(42.7789072078242,-58.4811528510598,
-39.33029755848));
#267211=CARTESIAN_POINT('Ctrl Pts',(42.7629038607078,-58.4531265953729,
-39.3212878681428));
#267212=CARTESIAN_POINT('Ctrl Pts',(42.7321834511559,-58.3961509948357,
-39.3033273013551));
#267213=CARTESIAN_POINT('Ctrl Pts',(42.7174700031016,-58.3672093155525,
-39.2943787390014));
#267214=CARTESIAN_POINT('Ctrl Pts',(42.689343821659,-58.3083513101081,-39.2765331188783));
#267215=CARTESIAN_POINT('Ctrl Pts',(42.6760415140178,-58.2786638018862,
-39.2677056541075));
#267216=CARTESIAN_POINT('Ctrl Pts',(42.6509587993318,-58.2188370725527,
-39.2502559046012));
#267217=CARTESIAN_POINT('Ctrl Pts',(42.6391736156063,-58.1886877789828,
-39.241630573039));
#267218=CARTESIAN_POINT('Ctrl Pts',(42.6171007474472,-58.127923813745,-39.2245782718256));
#267219=CARTESIAN_POINT('Ctrl Pts',(42.6068129739072,-58.0973088328386,
-39.2161512192883));
#267220=CARTESIAN_POINT('Ctrl Pts',(42.5781879491669,-58.0047670192766,
-39.1911676757355));
#267221=CARTESIAN_POINT('Ctrl Pts',(42.5620836311909,-57.942142746375,-39.1749075665151));
#267222=CARTESIAN_POINT('Ctrl Pts',(42.5424630372967,-57.846799679813,-39.1511279281964));
#267223=CARTESIAN_POINT('Ctrl Pts',(42.5366792610313,-57.8147773284237,
-39.1433017954548));
#267224=CARTESIAN_POINT('Ctrl Pts',(42.5266555052792,-57.7502670865121,
-39.1278612669093));
#267225=CARTESIAN_POINT('Ctrl Pts',(42.5224105823978,-57.7177326388165,
-39.1202361851916));
#267226=CARTESIAN_POINT('Ctrl Pts',(42.5155191585571,-57.6523285347624,
-39.1052370705839));
#267227=CARTESIAN_POINT('Ctrl Pts',(42.5128931531363,-57.6196821975634,
-39.0979136485113));
#267228=CARTESIAN_POINT('Ctrl Pts',(42.5092445696619,-57.5543872405645,
-39.0835894408895));
#267229=CARTESIAN_POINT('Ctrl Pts',(42.5082239674359,-57.5217574535128,
-39.076592971793));
#267230=CARTESIAN_POINT('Ctrl Pts',(42.5075539730829,-57.4239204642568,
-39.0560983673755));
#267231=CARTESIAN_POINT('Ctrl Pts',(42.5102910904574,-57.3587655206248,
-39.0430939199314));
#267232=CARTESIAN_POINT('Ctrl Pts',(42.5192012104666,-57.261137180212,-39.0245887021893));
#267233=CARTESIAN_POINT('Ctrl Pts',(42.5229732500635,-57.2286117736555,
-39.0185874646267));
#267234=CARTESIAN_POINT('Ctrl Pts',(42.5321441805056,-57.1635960137018,
-39.0069253566698));
#267235=CARTESIAN_POINT('Ctrl Pts',(42.5375464746252,-57.1310926165026,
-39.0012624667841));
#267236=CARTESIAN_POINT('Ctrl Pts',(42.5499988642966,-57.0661736081024,
-38.9902936182087));
#267237=CARTESIAN_POINT('Ctrl Pts',(42.5570855845251,-57.0336218831051,
-38.9849668275436));
#267238=CARTESIAN_POINT('Ctrl Pts',(42.5727869142399,-56.9692679819142,
-38.9747847070689));
#267239=CARTESIAN_POINT('Ctrl Pts',(42.5814158886332,-56.9373636193352,
-38.9699110349254));
#267240=CARTESIAN_POINT('Ctrl Pts',(42.6002039592955,-56.8741385048671,
-38.960602206569));
#267241=CARTESIAN_POINT('Ctrl Pts',(42.610364008329,-56.8428100439228,-38.9561656388506));
#267242=CARTESIAN_POINT('Ctrl Pts',(42.6322067310083,-56.78071772285,-38.9477266173214));
#267243=CARTESIAN_POINT('Ctrl Pts',(42.6438894125866,-56.7499538657306,
-38.943724165076));
#267244=CARTESIAN_POINT('Ctrl Pts',(42.6687792295882,-56.6889913336959,
-38.936154911583));
#267245=CARTESIAN_POINT('Ctrl Pts',(42.6819863498137,-56.6587926531977,
-38.9325881054662));
#267246=CARTESIAN_POINT('Ctrl Pts',(42.709938107711,-56.5989652286031,-38.9258948107753));
#267247=CARTESIAN_POINT('Ctrl Pts',(42.7246827057262,-56.5693364698414,
-38.9227683104938));
#267248=CARTESIAN_POINT('Ctrl Pts',(42.7557342012492,-56.5106579944336,
-38.9169635697921));
#267249=CARTESIAN_POINT('Ctrl Pts',(42.7720314608922,-56.481624481206,-38.9142867097661));
#267250=CARTESIAN_POINT('Ctrl Pts',(42.8062640059245,-56.424085389993,-38.9093871432694));
#267251=CARTESIAN_POINT('Ctrl Pts',(42.8240692231992,-56.395799847901,-38.9071833532006));
#267252=CARTESIAN_POINT('Ctrl Pts',(42.8793344551428,-56.3126949484312,
-38.9013282621221));
#267253=CARTESIAN_POINT('Ctrl Pts',(42.918743168177,-56.2594003210213,-38.8984064421158));
#267254=CARTESIAN_POINT('Ctrl Pts',(43.0025483564193,-56.1570717858067,
-38.8945084542909));
#267255=CARTESIAN_POINT('Ctrl Pts',(43.0469649474229,-56.1080069069945,
-38.8935300021871));
#267256=CARTESIAN_POINT('Ctrl Pts',(43.1173450441481,-56.0376381601557,
-38.8935323891605));
#267257=CARTESIAN_POINT('Ctrl Pts',(43.141458661058,-56.0146990549453,-38.8937796039308));
#267258=CARTESIAN_POINT('Ctrl Pts',(43.1785611799511,-55.9811320384022,
-38.8945237100665));
#267259=CARTESIAN_POINT('Ctrl Pts',(43.1910978407718,-55.9700723375204,
-38.8948345555296));
#267260=CARTESIAN_POINT('Ctrl Pts',(43.2164884775807,-55.9482337293115,
-38.8955820938649));
#267261=CARTESIAN_POINT('Ctrl Pts',(43.2293524555614,-55.9374477670517,
-38.8960194067973));
#267262=CARTESIAN_POINT('Ctrl Pts',(43.2682109535356,-55.9056902236256,
-38.8975137012045));
#267263=CARTESIAN_POINT('Ctrl Pts',(43.2945320232725,-55.8852608728333,
-38.8987534360506));
#267264=CARTESIAN_POINT('Ctrl Pts',(43.3480000930852,-55.8458485303625,
-38.9017105364692));
#267265=CARTESIAN_POINT('Ctrl Pts',(43.3751449489233,-55.8268667058867,
-38.9034276958876));
#267266=CARTESIAN_POINT('Ctrl Pts',(43.4577944294251,-55.7720632464052,
-38.9092840615924));
#267267=CARTESIAN_POINT('Ctrl Pts',(43.5145113713215,-55.7383790557516,
-38.9141267100279));
#267268=CARTESIAN_POINT('Ctrl Pts',(43.6019984165122,-55.6921042709396,
-38.922785850023));
#267269=CARTESIAN_POINT('Ctrl Pts',(43.6315633864957,-55.6773891287914,
-38.9259051413184));
#267270=CARTESIAN_POINT('Ctrl Pts',(43.6915052875854,-55.6493901621927,
-38.9326125532154));
#267271=CARTESIAN_POINT('Ctrl Pts',(43.7218909351156,-55.636103784993,-38.9362019665749));
#267272=CARTESIAN_POINT('Ctrl Pts',(43.7834518747983,-55.6109945714021,
-38.9438507097857));
#267273=CARTESIAN_POINT('Ctrl Pts',(43.8147379997369,-55.5991384576554,
-38.9479262894259));
#267274=CARTESIAN_POINT('Ctrl Pts',(43.8773632788004,-55.5771771251162,
-38.9564520459569));
#267275=CARTESIAN_POINT('Ctrl Pts',(43.9088373867163,-55.5670128138588,
-38.9609181476403));
#267276=CARTESIAN_POINT('Ctrl Pts',(43.9720262136544,-55.5483136978037,
-38.9702378118119));
#267277=CARTESIAN_POINT('Ctrl Pts',(44.0037536788592,-55.5397733548593,
-38.9750928878619));
#267278=CARTESIAN_POINT('Ctrl Pts',(44.0674709230106,-55.5242871663795,
-38.985186610612));
#267279=CARTESIAN_POINT('Ctrl Pts',(44.099460707948,-55.5173413577782,-38.9904252668586));
#267280=CARTESIAN_POINT('Ctrl Pts',(44.1637007891551,-55.5050323653042,
-39.0012821079516));
#267281=CARTESIAN_POINT('Ctrl Pts',(44.1959510873779,-55.4996691938696,
-39.0069002965142));
#267282=CARTESIAN_POINT('Ctrl Pts',(44.260712289499,-55.4905251021207,-39.0185148869209));
#267283=CARTESIAN_POINT('Ctrl Pts',(44.2932231914844,-55.4867441708206,
-39.0245112869446));
#267284=CARTESIAN_POINT('Ctrl Pts',(44.3585075922001,-55.480775674059,-39.0368836954053));
#267285=CARTESIAN_POINT('Ctrl Pts',(44.3912828804572,-55.4785888313245,
-39.0432602233464));
#267286=CARTESIAN_POINT('Ctrl Pts',(44.4570928290005,-55.4758284917783,
-39.0563949677075));
#267287=CARTESIAN_POINT('Ctrl Pts',(44.4901876958509,-55.4752622617633,
-39.0631671834262));
#267288=CARTESIAN_POINT('Ctrl Pts',(44.5558452176361,-55.475758769118,-39.0769304140694));
#267289=CARTESIAN_POINT('Ctrl Pts',(44.5885615120018,-55.4768128312226,
-39.0839516406405));
#267290=CARTESIAN_POINT('Ctrl Pts',(44.6536812736587,-55.4805035202407,
-39.0982478716216));
#267291=CARTESIAN_POINT('Ctrl Pts',(44.6861004221968,-55.483139401189,-39.1055259894705));
#267292=CARTESIAN_POINT('Ctrl Pts',(44.7829419444318,-55.4933852274058,
-39.1277430575141));
#267293=CARTESIAN_POINT('Ctrl Pts',(44.8469492543596,-55.503328533356,-39.1430639225963));
#267294=CARTESIAN_POINT('Ctrl Pts',(44.9421361647843,-55.5228829035947,
-39.1667978233991));
#267295=CARTESIAN_POINT('Ctrl Pts',(44.9737275643282,-55.5301755370665,
-39.1748347739215));
#267296=CARTESIAN_POINT('Ctrl Pts',(45.0366332915956,-55.546321762157,-39.1911608566696));
#267297=CARTESIAN_POINT('Ctrl Pts',(45.0679417334004,-55.5551739760488,
-39.1994484880529));
#267298=CARTESIAN_POINT('Ctrl Pts',(45.1303012298678,-55.5744676215724,
-39.216284615773));
#267299=CARTESIAN_POINT('Ctrl Pts',(45.1613392597803,-55.5849120617205,
-39.2248309851518));
#267300=CARTESIAN_POINT('Ctrl Pts',(45.2225442622987,-55.6071884247806,
-39.2420155999886));
#267301=CARTESIAN_POINT('Ctrl Pts',(45.2528226925233,-55.6190538405798,
-39.2506837416077));
#267302=CARTESIAN_POINT('Ctrl Pts',(45.3126694117909,-55.6442020485079,
-39.2681505662992));
#267303=CARTESIAN_POINT('Ctrl Pts',(45.3422493331638,-55.6574883926309,
-39.2769523813226));
#267304=CARTESIAN_POINT('Ctrl Pts',(45.4007251529718,-55.6854799817093,
-39.2946915606304));
#267305=CARTESIAN_POINT('Ctrl Pts',(45.4296210506442,-55.7001852280132,
-39.3036289255364));
#267306=CARTESIAN_POINT('Ctrl Pts',(45.4867267714294,-55.7310191704249,
-39.3216390153311));
#267307=CARTESIAN_POINT('Ctrl Pts',(45.5149281650798,-55.7471427624975,
-39.3307089736211));
#267308=CARTESIAN_POINT('Ctrl Pts',(45.5706716223774,-55.7808485275847,
-39.3489961904353));
#267309=CARTESIAN_POINT('Ctrl Pts',(45.5980415806017,-55.7983262695069,
-39.3581569149896));
#267310=CARTESIAN_POINT('Ctrl Pts',(45.6785018446286,-55.8525001852937,
-39.3856333194591));
#267311=CARTESIAN_POINT('Ctrl Pts',(45.7300942897426,-55.891002260239,-39.4039877669757));
#267312=CARTESIAN_POINT('Ctrl Pts',(45.8291740542806,-55.9726262256725,
-39.4407364897739));
#267313=CARTESIAN_POINT('Ctrl Pts',(45.8766787967759,-56.0157556232289,
-39.459135894828));
#267314=CARTESIAN_POINT('Ctrl Pts',(45.9448683025546,-56.0839428568353,
-39.4867725989864));
#267315=CARTESIAN_POINT('Ctrl Pts',(45.9670860951877,-56.1072550024018,
-39.4959911211427));
#267316=CARTESIAN_POINT('Ctrl Pts',(46.0104840259957,-56.1550608350904,
-39.5144410445764));
#267317=CARTESIAN_POINT('Ctrl Pts',(46.0316551416961,-56.1795437819113,
-39.5236684527303));
#267318=CARTESIAN_POINT('Ctrl Pts',(46.0626450692445,-56.217204251931,-39.5375315768857));
#267319=CARTESIAN_POINT('Ctrl Pts',(46.0728378849325,-56.2299042093275,
-39.5421524573076));
#267320=CARTESIAN_POINT('Ctrl Pts',(46.092851018773,-56.2554719148758,-39.551348880014));
#267321=CARTESIAN_POINT('Ctrl Pts',(46.1026913195214,-56.2683637173689,
-39.555933316569));
#267322=CARTESIAN_POINT('Ctrl Pts',(46.1316838232885,-56.3073187525545,
-39.5696305214535));
#267323=CARTESIAN_POINT('Ctrl Pts',(46.1503365283638,-56.3336962107827,
-39.5787000086301));
#267324=CARTESIAN_POINT('Ctrl Pts',(46.2042529621824,-56.4139852215082,
-39.60570727654));
#267325=CARTESIAN_POINT('Ctrl Pts',(46.2375105436952,-56.4690891650644,
-39.6234582594478));
#267326=CARTESIAN_POINT('Ctrl Pts',(46.2833698408561,-56.5540829658312,
-39.6497025405486));
#267327=CARTESIAN_POINT('Ctrl Pts',(46.2979848351363,-56.5828054986343,
-39.658387207326));
#267328=CARTESIAN_POINT('Ctrl Pts',(46.3258604890836,-56.6410396034225,
-39.6756293217671));
#267329=CARTESIAN_POINT('Ctrl Pts',(46.3391212174584,-56.6705511356645,
-39.684186774641));
#267330=CARTESIAN_POINT('Ctrl Pts',(46.3642673689533,-56.7303752678074,
-39.7011732901024));
#267331=CARTESIAN_POINT('Ctrl Pts',(46.3761460085845,-56.7606694672189,
-39.7095973250063));
#267332=CARTESIAN_POINT('Ctrl Pts',(46.3985236982386,-56.8221506262249,
-39.7263350672961));
#267333=CARTESIAN_POINT('Ctrl Pts',(46.4089539001758,-56.8531540104908,
-39.7345983819507));
#267334=CARTESIAN_POINT('Ctrl Pts',(46.4378289889335,-56.9464971479131,
-39.7589545662051));
#267335=CARTESIAN_POINT('Ctrl Pts',(46.4539730140977,-57.0094025598672,
-39.774683215309));
#267336=CARTESIAN_POINT('Ctrl Pts',(46.480079447285,-57.1364634819838,-39.8051172322268));
#267337=CARTESIAN_POINT('Ctrl Pts',(46.490051050886,-57.2006341137638,-39.8198274613562));
#267338=CARTESIAN_POINT('Ctrl Pts',(46.5003164047383,-57.2978585625442,
-39.8411267672249));
#267339=CARTESIAN_POINT('Ctrl Pts',(46.5029550484688,-57.3304317173846,
-39.8480993416622));
#267340=CARTESIAN_POINT('Ctrl Pts',(46.5066366277352,-57.3959005137752,
-39.8617837974953));
#267341=CARTESIAN_POINT('Ctrl Pts',(46.5076798542157,-57.4288266558715,
-39.8685017640589));
#267342=CARTESIAN_POINT('Ctrl Pts',(46.5081286131878,-57.4949099337061,
-39.8816515992078));
#267343=CARTESIAN_POINT('Ctrl Pts',(46.5075346190154,-57.5278165861342,
-39.8880340709103));
#267344=CARTESIAN_POINT('Ctrl Pts',(46.5047360881509,-57.5934606456236,
-39.900440518001));
#267345=CARTESIAN_POINT('Ctrl Pts',(46.502531400808,-57.626181768562,-39.9064612439072));
#267346=CARTESIAN_POINT('Ctrl Pts',(46.4935219657065,-57.7240448203298,
-39.923982362838));
#267347=CARTESIAN_POINT('Ctrl Pts',(46.4843271372358,-57.7888870954909,
-39.9349428927655));
#267348=CARTESIAN_POINT('Ctrl Pts',(46.4657292594294,-57.8855471837123,
-39.9503047442402));
#267349=CARTESIAN_POINT('Ctrl Pts',(46.458727758375,-57.9176665005431,-39.9552452454648));
#267350=CARTESIAN_POINT('Ctrl Pts',(46.4430984605719,-57.9817008313272,
-39.9647621435255));
#267351=CARTESIAN_POINT('Ctrl Pts',(46.4344657419777,-58.0136292048186,
-39.9693401953313));
#267352=CARTESIAN_POINT('Ctrl Pts',(46.4155601083816,-58.0772238658133,
-39.9781190500757));
#267353=CARTESIAN_POINT('Ctrl Pts',(46.405235422408,-58.1090273916134,-39.9823366235341));
#267354=CARTESIAN_POINT('Ctrl Pts',(46.3831322370528,-58.1717233081051,
-39.9903045886339));
#267355=CARTESIAN_POINT('Ctrl Pts',(46.3713308475608,-58.2027120874814,
-39.9940694297706));
#267356=CARTESIAN_POINT('Ctrl Pts',(46.3462591752663,-58.2639408858517,
-40.0011617906564));
#267357=CARTESIAN_POINT('Ctrl Pts',(46.3329874273489,-58.2941877852093,
-40.0044903745716));
#267358=CARTESIAN_POINT('Ctrl Pts',(46.3049830003936,-58.3539519689038,
-40.0107163415784));
#267359=CARTESIAN_POINT('Ctrl Pts',(46.2902503101408,-58.383469247682,-40.0136137207465));
#267360=CARTESIAN_POINT('Ctrl Pts',(46.2593240500028,-58.4417741675014,
-40.0189779749618));
#267361=CARTESIAN_POINT('Ctrl Pts',(46.2431304912238,-58.470561814118,-40.0214448528642));
#267362=CARTESIAN_POINT('Ctrl Pts',(46.2092717726407,-58.5274020727665,
-40.0259455366297));
#267363=CARTESIAN_POINT('Ctrl Pts',(46.1916066472402,-58.5554547019966,
-40.0279793523959));
#267364=CARTESIAN_POINT('Ctrl Pts',(46.1547828992827,-58.6108139537738,
-40.0316079667071));
#267365=CARTESIAN_POINT('Ctrl Pts',(46.1356370939371,-58.6381031491859,
-40.033201863178));
#267366=CARTESIAN_POINT('Ctrl Pts',(46.0957670512506,-58.6919883971087,
-40.0359447517529));
#267367=CARTESIAN_POINT('Ctrl Pts',(46.075181231902,-58.7183945160565,-40.0370836630407));
#267368=CARTESIAN_POINT('Ctrl Pts',(46.0117863921084,-58.7956387234688,
-40.0397935265569));
#267369=CARTESIAN_POINT('Ctrl Pts',(45.9672001304834,-58.844745304603,-40.0406777816202));
#267370=CARTESIAN_POINT('Ctrl Pts',(45.8735323130258,-58.9381754480581,
-40.0406312846123));
#267371=CARTESIAN_POINT('Ctrl Pts',(45.8244354693604,-58.9825217206044,
-40.0397019843559));
#267372=CARTESIAN_POINT('Ctrl Pts',(45.7474002842578,-59.0454399658155,
-40.0369397419404));
#267373=CARTESIAN_POINT('Ctrl Pts',(45.7211400913291,-59.0658221063687,
-40.0357895194905));
#267374=CARTESIAN_POINT('Ctrl Pts',(45.6809048277922,-59.0954685233027,
-40.0337171756965));
#267375=CARTESIAN_POINT('Ctrl Pts',(45.6673394345786,-59.1052045384925,
-40.0329676840834));
#267376=CARTESIAN_POINT('Ctrl Pts',(45.6399357364193,-59.1243566232342,
-40.0313525371172));
#267377=CARTESIAN_POINT('Ctrl Pts',(45.6260670111341,-59.1337924862528,
-40.0304848012205));
#267378=CARTESIAN_POINT('Ctrl Pts',(45.5842146021532,-59.161503832051,-40.0277164279032));
#267379=CARTESIAN_POINT('Ctrl Pts',(45.5559971110396,-59.1791823026862,
-40.0256529103855));
#267380=CARTESIAN_POINT('Ctrl Pts',(45.4988812016502,-59.2130235382979,
-40.0210947294542));
#267381=CARTESIAN_POINT('Ctrl Pts',(45.4699934991806,-59.2291795021203,
-40.0186008323348));
#267382=CARTESIAN_POINT('Ctrl Pts',(45.3823565697306,-59.2753890254871,
-40.010483831197));
#267383=CARTESIAN_POINT('Ctrl Pts',(45.322635564301,-59.3031889643499,-40.0042267981133));
#267384=CARTESIAN_POINT('Ctrl Pts',(45.2311263675532,-59.3404176099272,
-39.9935791348688));
#267385=CARTESIAN_POINT('Ctrl Pts',(45.2003014699612,-59.352080669579,-39.9898191937811));
#267386=CARTESIAN_POINT('Ctrl Pts',(45.1380036116915,-59.373903446149,-39.9818740857548));
#267387=CARTESIAN_POINT('Ctrl Pts',(45.1065143262852,-59.3840670181506,
-39.9776864682954));
#267388=CARTESIAN_POINT('Ctrl Pts',(45.0429439840219,-59.4028543289242,
-39.9688889157721));
#267389=CARTESIAN_POINT('Ctrl Pts',(45.0107048817299,-59.4115142672699,
-39.9642550191769));
#267390=CARTESIAN_POINT('Ctrl Pts',(44.946214704594,-59.4271222445478,-39.9546439730782));
#267391=CARTESIAN_POINT('Ctrl Pts',(44.9139257231678,-59.4340898684192,
-39.9496632423241));
#267392=CARTESIAN_POINT('Ctrl Pts',(44.8492550541234,-59.4463881271609,
-39.9393564537703));
#267393=CARTESIAN_POINT('Ctrl Pts',(44.8168745667947,-59.4517192585513,
-39.9340307317858));
#267394=CARTESIAN_POINT('Ctrl Pts',(44.7520248705109,-59.4607715904943,
-39.92303906055));
#267395=CARTESIAN_POINT('Ctrl Pts',(44.7195556566076,-59.4644927040579,
-39.9173730941082));
#267396=CARTESIAN_POINT('Ctrl Pts',(44.6220163194673,-59.4732622640888,
-39.8998676809884));
#267397=CARTESIAN_POINT('Ctrl Pts',(44.5567953679904,-59.4759200591614,
-39.8875175893321));
#267398=CARTESIAN_POINT('Ctrl Pts',(44.458759050957,-59.4751132746956,-39.8679808834745));
#267399=CARTESIAN_POINT('Ctrl Pts',(44.4260063620395,-59.4740398065978,
-39.861291052985));
#267400=CARTESIAN_POINT('Ctrl Pts',(44.376856965898,-59.4712170391416,-39.851005746395));
#267401=CARTESIAN_POINT('Ctrl Pts',(44.3604554548704,-59.4700720815201,
-39.8475321947849));
#267402=CARTESIAN_POINT('Ctrl Pts',(44.3276273759585,-59.4673726892737,
-39.8404967363322));
#267403=CARTESIAN_POINT('Ctrl Pts',(44.3112150867197,-59.4658185672318,
-39.8369377136338));
#267404=CARTESIAN_POINT('Ctrl Pts',(44.262218286448,-59.4605679436367,-39.8261880310505));
#267405=CARTESIAN_POINT('Ctrl Pts',(44.2297855973829,-59.4562799745141,
-39.8189066661417));
#267406=CARTESIAN_POINT('Ctrl Pts',(44.1653820777189,-59.4461630097037,
-39.804119565089));
#267407=CARTESIAN_POINT('Ctrl Pts',(44.1334098014393,-59.4403343297903,
-39.79661360907));
#267408=CARTESIAN_POINT('Ctrl Pts',(44.0381705583581,-59.4205751896199,
-39.7737623949309));
#267409=CARTESIAN_POINT('Ctrl Pts',(43.9755798363749,-59.4043761343586,
-39.758084441159));
#267410=CARTESIAN_POINT('Ctrl Pts',(43.8521846091923,-59.3659909301588,
-39.7258425263144));
#267411=CARTESIAN_POINT('Ctrl Pts',(43.7913711836815,-59.3437971009265,
-39.7092752319402));
#267412=CARTESIAN_POINT('Ctrl Pts',(43.7165136160533,-59.3122661488096,
-39.6880064520053));
#267413=CARTESIAN_POINT('Ctrl Pts',(43.7015911797635,-59.3057636179843,
-39.6837215312847));
#267414=CARTESIAN_POINT('Ctrl Pts',(43.6718795073988,-59.2923840419977,
-39.6750999215644));
#267415=CARTESIAN_POINT('Ctrl Pts',(43.6570608420848,-59.2854918386329,
-39.6707542956128));
#267416=CARTESIAN_POINT('Ctrl Pts',(43.6129441176106,-59.2643113087757,
-39.657679048406));
#267417=CARTESIAN_POINT('Ctrl Pts',(43.5840316836982,-59.2495467855778,
-39.6489259299949));
#267418=CARTESIAN_POINT('Ctrl Pts',(43.5555686724225,-59.2341331371673,
-39.6401254388889));
#267419=CARTESIAN_POINT('Ctrl Pts',(46.5057031838161,-57.5702877290152,
-39.8960534363005));
#267420=CARTESIAN_POINT('Ctrl Pts',(46.5058563971114,-57.5670514245044,
-39.8954454022393));
#267421=CARTESIAN_POINT('Ctrl Pts',(46.5060007398109,-57.5638457317421,
-39.8948410900405));
#267422=CARTESIAN_POINT('Ctrl Pts',(46.5061374457113,-57.5606390745173,
-39.894235046025));
#267423=CARTESIAN_POINT('Ctrl Pts',(46.5075367124945,-57.527817016895,-39.8880318224796));
#267424=CARTESIAN_POINT('Ctrl Pts',(46.508130707335,-57.4949103365212,-39.8816493507771));
#267425=CARTESIAN_POINT('Ctrl Pts',(46.5079063278233,-57.4618686695473,
-39.8750744332027));
#267426=CARTESIAN_POINT('Ctrl Pts',(46.5076819483115,-57.4288270025733,
-39.8684995156283));
#267427=CARTESIAN_POINT('Ctrl Pts',(46.5066387211099,-57.3959008325223,
-39.8617815490646));
#267428=CARTESIAN_POINT('Ctrl Pts',(46.5047979300779,-57.3631664065387,
-39.854939321148));
#267429=CARTESIAN_POINT('Ctrl Pts',(46.5029571390459,-57.3304319805551,
-39.8480970932315));
#267430=CARTESIAN_POINT('Ctrl Pts',(46.5003186115917,-57.2978599190912,
-39.8411247640299));
#267431=CARTESIAN_POINT('Ctrl Pts',(46.4968968273198,-57.2654506330812,
-39.8340246192596));
#267432=CARTESIAN_POINT('Ctrl Pts',(46.490053258776,-57.2006320610612,-39.819824329719));
#267433=CARTESIAN_POINT('Ctrl Pts',(46.4800815194185,-57.1364635805499,
-39.8051149837962));
#267434=CARTESIAN_POINT('Ctrl Pts',(46.4670282920657,-57.0729330656046,
-39.7898979753373));
#267435=CARTESIAN_POINT('Ctrl Pts',(46.4539750647129,-57.0094025506593,
-39.7746809668783));
#267436=CARTESIAN_POINT('Ctrl Pts',(46.437831026164,-56.9464970853635,-39.7589523177745));
#267437=CARTESIAN_POINT('Ctrl Pts',(46.4185809509685,-56.8842682743296,
-39.7427148616048));
#267438=CARTESIAN_POINT('Ctrl Pts',(46.4089559133708,-56.8531538688126,
-39.73459613352));
#267439=CARTESIAN_POINT('Ctrl Pts',(46.3985257027381,-56.8221504582685,
-39.7263328188654));
#267440=CARTESIAN_POINT('Ctrl Pts',(46.3873368485705,-56.7914098527142,
-39.7179639477205));
#267441=CARTESIAN_POINT('Ctrl Pts',(46.3761479944029,-56.7606692471599,
-39.7095950765756));
#267442=CARTESIAN_POINT('Ctrl Pts',(46.3642693448436,-56.7303750220794,
-39.7011710416717));
#267443=CARTESIAN_POINT('Ctrl Pts',(46.3516962585769,-56.7004629306669,
-39.692677783941));
#267444=CARTESIAN_POINT('Ctrl Pts',(46.3391231723103,-56.6705508392544,
-39.6841845262104));
#267445=CARTESIAN_POINT('Ctrl Pts',(46.3258624209486,-56.6410391769107,
-39.6756270022281));
#267446=CARTESIAN_POINT('Ctrl Pts',(46.3119246240029,-56.6119222266148,
-39.6670060026179));
#267447=CARTESIAN_POINT('Ctrl Pts',(46.2979868270572,-56.5828052763188,
-39.6583850030077));
#267448=CARTESIAN_POINT('Ctrl Pts',(46.2833719995868,-56.5540830376329,
-39.6497004356907));
#267449=CARTESIAN_POINT('Ctrl Pts',(46.2680854169705,-56.5257513241111,
-39.6409521228394));
#267450=CARTESIAN_POINT('Ctrl Pts',(46.2375122517372,-56.4690878970724,
-39.6234554971376));
#267451=CARTESIAN_POINT('Ctrl Pts',(46.2042548038769,-56.4139847078702,
-39.6057050281093));
#267452=CARTESIAN_POINT('Ctrl Pts',(46.1683104844322,-56.3604586554391,
-39.587700182836));
#267453=CARTESIAN_POINT('Ctrl Pts',(46.1503383247098,-56.3336956292236,
-39.5786977601994));
#267454=CARTESIAN_POINT('Ctrl Pts',(46.1316856039389,-56.3073181486858,
-39.5696282730228));
#267455=CARTESIAN_POINT('Ctrl Pts',(46.1123572518232,-56.2813481032686,
-39.5604968030998));
#267456=CARTESIAN_POINT('Ctrl Pts',(46.1026930757653,-56.2683630805599,
-39.5559310681383));
#267457=CARTESIAN_POINT('Ctrl Pts',(46.0928527667315,-56.2554712671669,
-39.5513466315833));
#267458=CARTESIAN_POINT('Ctrl Pts',(46.0828461913842,-56.2426874035852,
-39.5467484202301));
#267459=CARTESIAN_POINT('Ctrl Pts',(46.0728396160369,-56.2299035400036,
-39.5421502088769));
#267460=CARTESIAN_POINT('Ctrl Pts',(46.0626467917633,-56.2172035718718,
-39.537529328455));
#267461=CARTESIAN_POINT('Ctrl Pts',(46.0523168072112,-56.204650071255,-39.5329082870699));
#267462=CARTESIAN_POINT('Ctrl Pts',(46.031656838107,-56.1795430700214,-39.5236662042996));
#267463=CARTESIAN_POINT('Ctrl Pts',(46.0104857045643,-56.1550601025126,
-39.5144387961457));
#267464=CARTESIAN_POINT('Ctrl Pts',(45.9887867208672,-56.1311571659758,
-39.5052138344289));
#267465=CARTESIAN_POINT('Ctrl Pts',(45.96708773717,-56.107254229439,-39.495988872712));
#267466=CARTESIAN_POINT('Ctrl Pts',(45.944869939679,-56.0839420780633,-39.4867703557641));
#267467=CARTESIAN_POINT('Ctrl Pts',(45.9221401573419,-56.0612129236123,
-39.4775579953252));
#267468=CARTESIAN_POINT('Ctrl Pts',(45.8766805926676,-56.0157546147104,
-39.4591332744475));
#267469=CARTESIAN_POINT('Ctrl Pts',(45.8291755799096,-55.9726253390587,
-39.4407342413432));
#267470=CARTESIAN_POINT('Ctrl Pts',(45.7796356558061,-55.9318133219288,
-39.4223598799441));
#267471=CARTESIAN_POINT('Ctrl Pts',(45.7300957317026,-55.891001304799,-39.403985518545));
#267472=CARTESIAN_POINT('Ctrl Pts',(45.6785032430004,-55.8524991974133,
-39.3856310710283));
#267473=CARTESIAN_POINT('Ctrl Pts',(45.6248630216437,-55.8163832231527,
-39.3673134680487));
#267474=CARTESIAN_POINT('Ctrl Pts',(45.5980429109653,-55.7983252360224,
-39.3581546665589));
#267475=CARTESIAN_POINT('Ctrl Pts',(45.5706729296019,-55.7808474793946,
-39.3489939420046));
#267476=CARTESIAN_POINT('Ctrl Pts',(45.5428011773848,-55.7639945826789,
-39.3398503335975));
#267477=CARTESIAN_POINT('Ctrl Pts',(45.5149294251677,-55.7471416859632,
-39.3307067251904));
#267478=CARTESIAN_POINT('Ctrl Pts',(45.4867280076654,-55.7310180803397,
-39.3216367669004));
#267479=CARTESIAN_POINT('Ctrl Pts',(45.4581751231188,-55.7156010961851,
-39.3126317220031));
#267480=CARTESIAN_POINT('Ctrl Pts',(43.4805771074156,-59.5712767529309,
-39.2399080357013));
#267481=CARTESIAN_POINT('Ctrl Pts',(43.4150727209207,-59.5358440364426,
-39.2223070534893));
#267482=CARTESIAN_POINT('Ctrl Pts',(43.2883193276586,-59.4590682572254,
-39.1867578392588));
#267483=CARTESIAN_POINT('Ctrl Pts',(43.1106712693135,-59.32658002426,-39.1324031814995));
#267484=CARTESIAN_POINT('Ctrl Pts',(43.0005921597408,-59.2266373021163,
-39.0954660506179));
#267485=CARTESIAN_POINT('Ctrl Pts',(42.8948534568781,-59.1207134074407,
-39.0581733199915));
#267486=CARTESIAN_POINT('Ctrl Pts',(42.7951360401793,-59.0104958554849,
-39.0211184761739));
#267487=CARTESIAN_POINT('Ctrl Pts',(42.6850011896347,-58.8622904152127,
-38.9753582681256));
#267488=CARTESIAN_POINT('Ctrl Pts',(42.6055727997797,-58.7375004045667,
-38.939089851323));
#267489=CARTESIAN_POINT('Ctrl Pts',(42.5503788594446,-58.6407591922129,
-38.9120596161462));
#267490=CARTESIAN_POINT('Ctrl Pts',(42.5165536369311,-58.5741539171446,
-38.8941613358138));
#267491=CARTESIAN_POINT('Ctrl Pts',(42.4842288567228,-58.5064298632496,
-38.8763157156907));
#267492=CARTESIAN_POINT('Ctrl Pts',(42.4689425396028,-58.4722695523732,
-38.8674882509199));
#267493=CARTESIAN_POINT('Ctrl Pts',(42.4257123024776,-58.3690064948315,
-38.8413136266604));
#267494=CARTESIAN_POINT('Ctrl Pts',(42.3750272156063,-58.229152189777,-38.8072100415055));
#267495=CARTESIAN_POINT('Ctrl Pts',(42.3380647902547,-58.0850119200902,
-38.7746901633276));
#267496=CARTESIAN_POINT('Ctrl Pts',(42.3155659796374,-57.9752818499468,
-38.7509105250088));
#267497=CARTESIAN_POINT('Ctrl Pts',(42.3089374211558,-57.9384266221928,
-38.7430843922672));
#267498=CARTESIAN_POINT('Ctrl Pts',(42.297458012674,-57.864178756387,-38.7276438637217));
#267499=CARTESIAN_POINT('Ctrl Pts',(42.292601515188,-57.8267325312259,-38.720018782004));
#267500=CARTESIAN_POINT('Ctrl Pts',(42.2847289916893,-57.7514526301959,
-38.7050196673963));
#267501=CARTESIAN_POINT('Ctrl Pts',(42.2817363521424,-57.7138759968928,
-38.6976962453237));
#267502=CARTESIAN_POINT('Ctrl Pts',(42.277596992864,-57.6387184974263,-38.6833720377019));
#267503=CARTESIAN_POINT('Ctrl Pts',(42.2741651307842,-57.5260409596698,
-38.6623829091612));
#267504=CARTESIAN_POINT('Ctrl Pts',(42.2805893100654,-57.3760354719141,
-38.6363740800325));
#267505=CARTESIAN_POINT('Ctrl Pts',(42.2937061680812,-57.2637038035873,
-38.618370061439));
#267506=CARTESIAN_POINT('Ctrl Pts',(42.3043247017591,-57.1888547452426,
-38.6067079534822));
#267507=CARTESIAN_POINT('Ctrl Pts',(42.3105743117123,-57.1514345461221,
-38.6010450635964));
#267508=CARTESIAN_POINT('Ctrl Pts',(42.3249704170347,-57.0766935209607,
-38.590076215021));
#267509=CARTESIAN_POINT('Ctrl Pts',(42.3331592025312,-57.0392159768686,
-38.5847494243559));
#267510=CARTESIAN_POINT('Ctrl Pts',(42.3512949844302,-56.9651221381903,
-38.5745673038812));
#267511=CARTESIAN_POINT('Ctrl Pts',(42.3712216906218,-56.8916587034686,
-38.564820665347));
#267512=CARTESIAN_POINT('Ctrl Pts',(42.4063979707918,-56.7834465224234,
-38.5515118436));
#267513=CARTESIAN_POINT('Ctrl Pts',(42.4468320479729,-56.6771725078319,
-38.5395042677724));
#267514=CARTESIAN_POINT('Ctrl Pts',(42.4925290654744,-56.5728473165674,
-38.5288039137004));
#267515=CARTESIAN_POINT('Ctrl Pts',(42.5265325119253,-56.5046058456765,
-38.5225509073062));
#267516=CARTESIAN_POINT('Ctrl Pts',(42.5623338475306,-56.4370293947697,
-38.5167461666044));
#267517=CARTESIAN_POINT('Ctrl Pts',(42.5811223641794,-56.4035923099625,
-38.5140693065785));
#267518=CARTESIAN_POINT('Ctrl Pts',(42.620584523009,-56.3373241998654,-38.5091697400817));
#267519=CARTESIAN_POINT('Ctrl Pts',(42.6411082254821,-56.3047465904101,
-38.5069659500128));
#267520=CARTESIAN_POINT('Ctrl Pts',(42.7048067991197,-56.2090283357163,
-38.501110858935));
#267521=CARTESIAN_POINT('Ctrl Pts',(42.7502234543428,-56.1476408662828,
-38.4981890389281));
#267522=CARTESIAN_POINT('Ctrl Pts',(42.8467942323831,-56.0297655581676,
-38.4942910511033));
#267523=CARTESIAN_POINT('Ctrl Pts',(42.8979715413934,-55.9732420482176,
-38.4933125989996));
#267524=CARTESIAN_POINT('Ctrl Pts',(42.9790570553347,-55.8921695883033,
-38.4933149859729));
#267525=CARTESIAN_POINT('Ctrl Pts',(43.0068374106561,-55.8657400908868,
-38.4935622007431));
#267526=CARTESIAN_POINT('Ctrl Pts',(43.0495800649421,-55.8270637749536,
-38.4943063068789));
#267527=CARTESIAN_POINT('Ctrl Pts',(43.0640222060113,-55.8143203511958,
-38.494617152342));
#267528=CARTESIAN_POINT('Ctrl Pts',(43.0932714774893,-55.7891564261061,
-38.4953646906773));
#267529=CARTESIAN_POINT('Ctrl Pts',(43.1080901283632,-55.7767277938553,
-38.4958020036096));
#267530=CARTESIAN_POINT('Ctrl Pts',(43.1528523310046,-55.7401327167866,
-38.4972962980169));
#267531=CARTESIAN_POINT('Ctrl Pts',(43.2134913856688,-55.6930468850421,
-38.4997758707861));
#267532=CARTESIAN_POINT('Ctrl Pts',(43.3385569247743,-55.6055389451161,
-38.5066450244003));
#267533=CARTESIAN_POINT('Ctrl Pts',(43.4691986576013,-55.5278792007279,
-38.5163302992824));
#267534=CARTESIAN_POINT('Ctrl Pts',(43.5713395927684,-55.4769743237494,
-38.5256877381308));
#267535=CARTESIAN_POINT('Ctrl Pts',(43.6403672861995,-55.4446857735354,
-38.5323951500278));
#267536=CARTESIAN_POINT('Ctrl Pts',(43.6753577685123,-55.4293620157832,
-38.5359845633874));
#267537=CARTESIAN_POINT('Ctrl Pts',(43.7462462065788,-55.4003985583156,
-38.5436333065981));
#267538=CARTESIAN_POINT('Ctrl Pts',(43.7822717759725,-55.3867204456352,
-38.5477088862383));
#267539=CARTESIAN_POINT('Ctrl Pts',(43.8543821738219,-55.3613797848081,
-38.5562346427694));
#267540=CARTESIAN_POINT('Ctrl Pts',(43.890622407919,-55.349649082917,-38.5607007444526));
#267541=CARTESIAN_POINT('Ctrl Pts',(43.9997560709039,-55.3172704656441,
-38.5746802407103));
#267542=CARTESIAN_POINT('Ctrl Pts',(44.1098017310836,-55.290468361793,-38.5898286859852));
#267543=CARTESIAN_POINT('Ctrl Pts',(44.2583166685835,-55.2656490138239,
-38.612301023075));
#267544=CARTESIAN_POINT('Ctrl Pts',(44.3705972700495,-55.2524997368729,
-38.6302900391873));
#267545=CARTESIAN_POINT('Ctrl Pts',(44.446056048267,-55.2474029004138,-38.6430428201589));
#267546=CARTESIAN_POINT('Ctrl Pts',(44.5218128020516,-55.2441636366351,
-38.65617756452));
#267547=CARTESIAN_POINT('Ctrl Pts',(44.5599089424743,-55.2434808562086,
-38.6629497802385));
#267548=CARTESIAN_POINT('Ctrl Pts',(44.6354869543582,-55.2439911084578,
-38.6767130108817));
#267549=CARTESIAN_POINT('Ctrl Pts',(44.6731456892459,-55.2451740103824,
-38.6837342374529));
#267550=CARTESIAN_POINT('Ctrl Pts',(44.7481014788608,-55.2493620066237,
-38.6980304684339));
#267551=CARTESIAN_POINT('Ctrl Pts',(44.860046548974,-55.2583760573225,-38.7198650218829));
#267552=CARTESIAN_POINT('Ctrl Pts',(45.0073845433675,-55.2811507310277,
-38.7505067688753));
#267553=CARTESIAN_POINT('Ctrl Pts',(45.1528189888476,-55.3146135839333,
-38.7826550300594));
#267554=CARTESIAN_POINT('Ctrl Pts',(45.2248832056965,-55.3349380951144,
-38.7992310848652));
#267555=CARTESIAN_POINT('Ctrl Pts',(45.2966462681613,-55.3570913336823,
-38.8160672125853));
#267556=CARTESIAN_POINT('Ctrl Pts',(45.3323638946335,-55.3690863290504,
-38.8246135819642));
#267557=CARTESIAN_POINT('Ctrl Pts',(45.4027951436545,-55.3946744461232,
-38.841798196801));
#267558=CARTESIAN_POINT('Ctrl Pts',(45.4376370321487,-55.4083060218429,
-38.85046633842));
#267559=CARTESIAN_POINT('Ctrl Pts',(45.5409345111852,-55.4516493275196,
-38.8766665754573));
#267560=CARTESIAN_POINT('Ctrl Pts',(45.6082182891413,-55.4838201174091,
-38.8944064774514));
#267561=CARTESIAN_POINT('Ctrl Pts',(45.7067749877369,-55.5369855856676,
-38.9214216121435));
#267562=CARTESIAN_POINT('Ctrl Pts',(45.7392219877795,-55.5555212114618,
-38.9304915704334));
#267563=CARTESIAN_POINT('Ctrl Pts',(45.8033556832395,-55.5942722159849,
-38.9487787872477));
#267564=CARTESIAN_POINT('Ctrl Pts',(45.8348443691401,-55.6143675312756,
-38.9579395118015));
#267565=CARTESIAN_POINT('Ctrl Pts',(45.9274099842789,-55.6766589025306,
-38.9854159162723));
#267566=CARTESIAN_POINT('Ctrl Pts',(45.9867610865919,-55.7209353156014,
-39.0037703637879));
#267567=CARTESIAN_POINT('Ctrl Pts',(46.1007337830098,-55.8148102393793,
-39.0405190865864));
#267568=CARTESIAN_POINT('Ctrl Pts',(46.1826971388658,-55.889219933262,-39.0681181728269));
#267569=CARTESIAN_POINT('Ctrl Pts',(46.259356574729,-55.9696687352924,-39.0957737179551));
#267570=CARTESIAN_POINT('Ctrl Pts',(46.309266807939,-56.024663053365,-39.1142236413887));
#267571=CARTESIAN_POINT('Ctrl Pts',(46.3336138177017,-56.0528284109483,
-39.1234510495426));
#267572=CARTESIAN_POINT('Ctrl Pts',(46.3692509284248,-56.0961546965833,
-39.1373141736981));
#267573=CARTESIAN_POINT('Ctrl Pts',(46.3809719555493,-56.1107655250657,
-39.14193505412));
#267574=CARTESIAN_POINT('Ctrl Pts',(46.4039850968433,-56.1401806715041,
-39.1511314768264));
#267575=CARTESIAN_POINT('Ctrl Pts',(46.4153001903629,-56.1550126624776,
-39.1557159133813));
#267576=CARTESIAN_POINT('Ctrl Pts',(46.4486370096885,-56.1998310060263,
-39.1694131182659));
#267577=CARTESIAN_POINT('Ctrl Pts',(46.4700835091466,-56.2301795317326,
-39.1784826054425));
#267578=CARTESIAN_POINT('Ctrl Pts',(46.532071913686,-56.3225583984772,-39.2054898733524));
#267579=CARTESIAN_POINT('Ctrl Pts',(46.5894197348374,-56.4176636744323,
-39.23211607576));
#267580=CARTESIAN_POINT('Ctrl Pts',(46.6566074362748,-56.5498680842415,
-39.2668544229849));
#267581=CARTESIAN_POINT('Ctrl Pts',(46.6870820302515,-56.617790568625,-39.2839693714534));
#267582=CARTESIAN_POINT('Ctrl Pts',(46.7159729830272,-56.6866360545619,
-39.3009558869148));
#267583=CARTESIAN_POINT('Ctrl Pts',(46.7296188023799,-56.7214992889704,
-39.3093799218186));
#267584=CARTESIAN_POINT('Ctrl Pts',(46.7553216997643,-56.7922546384013,
-39.3261176641085));
#267585=CARTESIAN_POINT('Ctrl Pts',(46.7672996943011,-56.8279354881579,
-39.3343809787628));
#267586=CARTESIAN_POINT('Ctrl Pts',(46.8004530502947,-56.9353633959568,
-39.358737163018));
#267587=CARTESIAN_POINT('Ctrl Pts',(46.8189795501832,-57.0077635587999,
-39.3744658121213));
#267588=CARTESIAN_POINT('Ctrl Pts',(46.848916211803,-57.1540080946302,-39.4048998290393));
#267589=CARTESIAN_POINT('Ctrl Pts',(46.866048617508,-57.2647966217996,-39.4269646939479));
#267590=CARTESIAN_POINT('Ctrl Pts',(46.875074749658,-57.3772756893033,-39.4478819384746));
#267591=CARTESIAN_POINT('Ctrl Pts',(46.8792542953452,-57.4526370309597,
-39.4615663943076));
#267592=CARTESIAN_POINT('Ctrl Pts',(46.8804258736835,-57.4905390832845,
-39.4682843608713));
#267593=CARTESIAN_POINT('Ctrl Pts',(46.8808837743635,-57.566610437341,-39.4814341960201));
#267594=CARTESIAN_POINT('Ctrl Pts',(46.8801708637706,-57.604491394965,-39.4878166677226));
#267595=CARTESIAN_POINT('Ctrl Pts',(46.8768913879562,-57.6800597985945,
-39.5002231148134));
#267596=CARTESIAN_POINT('Ctrl Pts',(46.8691896925243,-57.7930657109158,
-39.5182849936093));
#267597=CARTESIAN_POINT('Ctrl Pts',(46.8479069711518,-57.9423669591112,
-39.540205996752));
#267598=CARTESIAN_POINT('Ctrl Pts',(46.8236459543104,-58.053306681129,-39.5550278422771));
#267599=CARTESIAN_POINT('Ctrl Pts',(46.8055990109883,-58.1270324939452,
-39.5645447403379));
#267600=CARTESIAN_POINT('Ctrl Pts',(46.7956339676918,-58.1637938532181,
-39.5691227921436));
#267601=CARTESIAN_POINT('Ctrl Pts',(46.7738161327052,-58.2370162077019,
-39.5779016468881));
#267602=CARTESIAN_POINT('Ctrl Pts',(46.7619036278491,-58.2736352268715,
-39.5821192203466));
#267603=CARTESIAN_POINT('Ctrl Pts',(46.7364059718256,-58.3458255995332,
-39.5900871854462));
#267604=CARTESIAN_POINT('Ctrl Pts',(46.7091836493705,-58.4171862986019,
-39.5976163356366));
#267605=CARTESIAN_POINT('Ctrl Pts',(46.663274408039,-58.5216699086648,-39.6076014242402));
#267606=CARTESIAN_POINT('Ctrl Pts',(46.6123207377325,-58.6236436013082,
-39.616293729045));
#267607=CARTESIAN_POINT('Ctrl Pts',(46.5563244858032,-58.7230996041114,
-39.6236943138341));
#267608=CARTESIAN_POINT('Ctrl Pts',(46.515607032986,-58.7877140896312,-39.6277619492082));
#267609=CARTESIAN_POINT('Ctrl Pts',(46.4731710833873,-58.8514710047945,
-39.6313905635194));
#267610=CARTESIAN_POINT('Ctrl Pts',(46.4511086137465,-58.8829006319494,
-39.6329844599904));
#267611=CARTESIAN_POINT('Ctrl Pts',(46.4051673201274,-58.9449633016888,
-39.6357273485653));
#267612=CARTESIAN_POINT('Ctrl Pts',(46.381447994276,-58.975377588932,-39.6368662598532));
#267613=CARTESIAN_POINT('Ctrl Pts',(46.3084068909562,-59.0643493136614,
-39.6395761233691));
#267614=CARTESIAN_POINT('Ctrl Pts',(46.2570407846102,-59.1209150453974,
-39.6404603784325));
#267615=CARTESIAN_POINT('Ctrl Pts',(46.1491379755941,-59.228544463199,-39.6404138814247));
#267616=CARTESIAN_POINT('Ctrl Pts',(46.0925836555155,-59.2796343044913,
-39.6394845811684));
#267617=CARTESIAN_POINT('Ctrl Pts',(46.0038529437629,-59.3521266125547,
-39.6367223387528));
#267618=CARTESIAN_POINT('Ctrl Pts',(45.9736068078661,-59.3756113554055,
-39.6355721163029));
#267619=CARTESIAN_POINT('Ctrl Pts',(45.9272656961273,-59.4097723546528,
-39.6334997725088));
#267620=CARTESIAN_POINT('Ctrl Pts',(45.9116419215573,-59.4209912820171,
-39.6327502808957));
#267621=CARTESIAN_POINT('Ctrl Pts',(45.8800804794677,-59.4430610802669,
-39.6311351339295));
#267622=CARTESIAN_POINT('Ctrl Pts',(45.8321587971618,-59.4756823489919,
-39.628531354857));
#267623=CARTESIAN_POINT('Ctrl Pts',(45.7834097108732,-59.5062438963941,
-39.6254355071979));
#267624=CARTESIAN_POINT('Ctrl Pts',(45.717633106262,-59.5452481912826,-39.6208773262667));
#267625=CARTESIAN_POINT('Ctrl Pts',(45.6178307490054,-59.601113548897,-39.6133952897297));
#267626=CARTESIAN_POINT('Ctrl Pts',(45.4802897643185,-59.6652183443042,
-39.6008811885904));
#267627=CARTESIAN_POINT('Ctrl Pts',(45.3738098009101,-59.7055766782111,
-39.5896017905935));
#267628=CARTESIAN_POINT('Ctrl Pts',(45.3020778813705,-59.7307512119865,
-39.5816566825671));
#267629=CARTESIAN_POINT('Ctrl Pts',(45.2658207311094,-59.7424779859237,
-39.5774690651077));
#267630=CARTESIAN_POINT('Ctrl Pts',(45.1926264675053,-59.7641596016776,
-39.5686715125846));
#267631=CARTESIAN_POINT('Ctrl Pts',(45.1555073907618,-59.7741562512684,
-39.5640376159893));
#267632=CARTESIAN_POINT('Ctrl Pts',(45.0441315765335,-59.8011904590316,
-39.5496210468413));
#267633=CARTESIAN_POINT('Ctrl Pts',(44.9324484012679,-59.8224577850013,
-39.5341534065747));
#267634=CARTESIAN_POINT('Ctrl Pts',(44.8203079610257,-59.8353953605365,
-39.5171556909205));
#267635=CARTESIAN_POINT('Ctrl Pts',(44.7080184564226,-59.8455760612675,
-39.4996502778008));
#267636=CARTESIAN_POINT('Ctrl Pts',(44.6329372249224,-59.8486931621852,
-39.4873001861445));
#267637=CARTESIAN_POINT('Ctrl Pts',(44.5200834441659,-59.8478515133141,
-39.4677634802869));
#267638=CARTESIAN_POINT('Ctrl Pts',(44.4823810871712,-59.8466449718289,
-39.4610736497974));
#267639=CARTESIAN_POINT('Ctrl Pts',(44.4258051079382,-59.8434394706745,
-39.4507883432074));
#267640=CARTESIAN_POINT('Ctrl Pts',(44.4069254589855,-59.8421361346926,
-39.4473147915973));
#267641=CARTESIAN_POINT('Ctrl Pts',(44.3691376542581,-59.8390581625153,
-39.4402793331445));
#267642=CARTESIAN_POINT('Ctrl Pts',(44.3502459350849,-59.8372838734483,
-39.4367203104461));
#267643=CARTESIAN_POINT('Ctrl Pts',(44.2562487381671,-59.8272835659938,
-39.4188041728073));
#267644=CARTESIAN_POINT('Ctrl Pts',(44.1080045765469,-59.8040393501646,
-39.3892226636159));
#267645=CARTESIAN_POINT('Ctrl Pts',(43.9639303529155,-59.7668593120831,
-39.3578670379715));
#267646=CARTESIAN_POINT('Ctrl Pts',(43.8219159040518,-59.7227861654643,
-39.3256251231267));
#267647=CARTESIAN_POINT('Ctrl Pts',(43.7519290534068,-59.6972943066161,
-39.3090578287531));
#267648=CARTESIAN_POINT('Ctrl Pts',(43.665783177736,-59.6610675807531,-39.2877890488175));
#267649=CARTESIAN_POINT('Ctrl Pts',(43.6486106666635,-59.653596197985,-39.2835041280971));
#267650=CARTESIAN_POINT('Ctrl Pts',(43.6144193015916,-59.6382222359849,
-39.2748825183767));
#267651=CARTESIAN_POINT('Ctrl Pts',(43.597366582891,-59.6303022352814,-39.2705368924251));
#267652=CARTESIAN_POINT('Ctrl Pts',(43.5465994182959,-59.605961903298,-39.2574616452183));
#267653=CARTESIAN_POINT('Ctrl Pts',(43.513329300663,-59.588993111175,-39.2487085268073));
#267654=CARTESIAN_POINT('Ctrl Pts',(43.4805771074156,-59.5712767529309,
-39.2399080357013));
#267655=CARTESIAN_POINT('Ctrl Pts',(43.8903154257419,-57.7291941381088,
-41.4266127101804));
#267656=CARTESIAN_POINT('Ctrl Pts',(43.8716814361492,-57.7189244770852,
-41.4090117279687));
#267657=CARTESIAN_POINT('Ctrl Pts',(43.8355945080866,-57.6967277837834,
-41.3734625137379));
#267658=CARTESIAN_POINT('Ctrl Pts',(43.7849271573585,-57.6585752750105,
-41.3191078559793));
#267659=CARTESIAN_POINT('Ctrl Pts',(43.753465403225,-57.62988352171,-41.2821707250961));
#267660=CARTESIAN_POINT('Ctrl Pts',(43.7232071092872,-57.5995155202448,
-41.2448779944712));
#267661=CARTESIAN_POINT('Ctrl Pts',(43.694633283399,-57.5679550683129,-41.2078231506529));
#267662=CARTESIAN_POINT('Ctrl Pts',(43.6629744005209,-57.5256074013359,
-41.162062942605));
#267663=CARTESIAN_POINT('Ctrl Pts',(43.6400741040405,-57.4900012877665,
-41.1257945258022));
#267664=CARTESIAN_POINT('Ctrl Pts',(43.624122646482,-57.4624228770549,-41.0987642906252));
#267665=CARTESIAN_POINT('Ctrl Pts',(43.6143188854815,-57.4434516436916,
-41.0808660102928));
#267666=CARTESIAN_POINT('Ctrl Pts',(43.6049343759216,-57.4241698350281,
-41.0630203901697));
#267667=CARTESIAN_POINT('Ctrl Pts',(43.6004882740613,-57.4144479878336,
-41.054192925399));
#267668=CARTESIAN_POINT('Ctrl Pts',(43.5878889573419,-57.3850715912746,
-41.0280183011396));
#267669=CARTESIAN_POINT('Ctrl Pts',(43.5730447416356,-57.3453166524842,
-40.9939147159844));
#267670=CARTESIAN_POINT('Ctrl Pts',(43.5620571572655,-57.3044044614592,
-40.9613948378065));
#267671=CARTESIAN_POINT('Ctrl Pts',(43.5552843243605,-57.2732819874194,
-40.9376151994878));
#267672=CARTESIAN_POINT('Ctrl Pts',(43.5532714802541,-57.2628325912303,
-40.9297890667463));
#267673=CARTESIAN_POINT('Ctrl Pts',(43.5497454556161,-57.2417890776549,
-40.9143485382007));
#267674=CARTESIAN_POINT('Ctrl Pts',(43.5482304746054,-57.2311797832666,
-40.9067234564832));
#267675=CARTESIAN_POINT('Ctrl Pts',(43.5457184756399,-57.2098591834555,
-40.8917243418755));
#267676=CARTESIAN_POINT('Ctrl Pts',(43.5447290487245,-57.199220662917,-40.8844009198028));
#267677=CARTESIAN_POINT('Ctrl Pts',(43.5432711863927,-57.1779500447907,
-40.8700767121812));
#267678=CARTESIAN_POINT('Ctrl Pts',(43.5418684734652,-57.1460721839032,
-40.8490875836402));
#267679=CARTESIAN_POINT('Ctrl Pts',(43.5431039253892,-57.1036793909824,
-40.8230787545116));
#267680=CARTESIAN_POINT('Ctrl Pts',(43.5463738329101,-57.0719682486671,
-40.8050747359183));
#267681=CARTESIAN_POINT('Ctrl Pts',(43.5490829635055,-57.0508462881094,
-40.7934126279614));
#267682=CARTESIAN_POINT('Ctrl Pts',(43.5507030159248,-57.0402904723448,
-40.7877497380755));
#267683=CARTESIAN_POINT('Ctrl Pts',(43.5544790630841,-57.019214904491,-40.7767808895002));
#267684=CARTESIAN_POINT('Ctrl Pts',(43.5566463931059,-57.0086510117152,
-40.7714540988351));
#267685=CARTESIAN_POINT('Ctrl Pts',(43.5614808344627,-56.9877741662596,
-40.7612719783604));
#267686=CARTESIAN_POINT('Ctrl Pts',(43.5668234022498,-56.9670831174431,
-40.7515253398262));
#267687=CARTESIAN_POINT('Ctrl Pts',(43.5763377125496,-56.9366295208774,
-40.7382165180791));
#267688=CARTESIAN_POINT('Ctrl Pts',(43.5873444561754,-56.9067460923864,
-40.7262089422516));
#267689=CARTESIAN_POINT('Ctrl Pts',(43.5998453117462,-56.8774358278222,
-40.7155085881795));
#267690=CARTESIAN_POINT('Ctrl Pts',(43.6091839698139,-56.8582805167828,
-40.7092555817853));
#267691=CARTESIAN_POINT('Ctrl Pts',(43.6190331668358,-56.8393207538612,
-40.7034508410834));
#267692=CARTESIAN_POINT('Ctrl Pts',(43.6242099732076,-56.8299438685379,
-40.7007739810578));
#267693=CARTESIAN_POINT('Ctrl Pts',(43.6350986096338,-56.8113693026126,
-40.6958744145609));
#267694=CARTESIAN_POINT('Ctrl Pts',(43.6407690742328,-56.8022426567881,
-40.6936706244929));
#267695=CARTESIAN_POINT('Ctrl Pts',(43.6583896223854,-56.7754411523649,
-40.6878155334118));
#267696=CARTESIAN_POINT('Ctrl Pts',(43.6709801307092,-56.7582712890167,
-40.6848937134075));
#267697=CARTESIAN_POINT('Ctrl Pts',(43.6978023804218,-56.725340315416,-40.6809957255822));
#267698=CARTESIAN_POINT('Ctrl Pts',(43.7120405319879,-56.7095692151415,
-40.6800172734785));
#267699=CARTESIAN_POINT('Ctrl Pts',(43.7346338722206,-56.6869796178674,
-40.680019660452));
#267700=CARTESIAN_POINT('Ctrl Pts',(43.7423799312797,-56.6796208977126,
-40.6802668752224));
#267701=CARTESIAN_POINT('Ctrl Pts',(43.7543060585229,-56.6688607312791,
-40.681010981358));
#267702=CARTESIAN_POINT('Ctrl Pts',(43.7583370517177,-56.6653168192219,
-40.6813218268212));
#267703=CARTESIAN_POINT('Ctrl Pts',(43.7665035456834,-56.6583217341419,
-40.6820693651562));
#267704=CARTESIAN_POINT('Ctrl Pts',(43.7706422703,-56.6548683091639,-40.6825066780886));
#267705=CARTESIAN_POINT('Ctrl Pts',(43.7831478581881,-56.6447045100584,
-40.6840009724959));
#267706=CARTESIAN_POINT('Ctrl Pts',(43.8000992888712,-56.6316392340345,
-40.6864805452653));
#267707=CARTESIAN_POINT('Ctrl Pts',(43.8351004518507,-56.6074069729907,
-40.6933496988796));
#267708=CARTESIAN_POINT('Ctrl Pts',(43.8717190640765,-56.5859796680779,
-40.7030349737613));
#267709=CARTESIAN_POINT('Ctrl Pts',(43.9003898794618,-56.5719991465823,
-40.7123924126099));
#267710=CARTESIAN_POINT('Ctrl Pts',(43.919774692733,-56.5631479893168,-40.719099824507));
#267711=CARTESIAN_POINT('Ctrl Pts',(43.9296053152689,-56.5589560552736,
-40.722689237866));
#267712=CARTESIAN_POINT('Ctrl Pts',(43.9495302416178,-56.551051384942,-40.7303379810773));
#267713=CARTESIAN_POINT('Ctrl Pts',(43.959660471973,-56.5473282955902,-40.7344135607172));
#267714=CARTESIAN_POINT('Ctrl Pts',(43.9799461530017,-56.5404515818703,
-40.7429393172485));
#267715=CARTESIAN_POINT('Ctrl Pts',(43.9901452646573,-56.5372793127045,
-40.7474054189318));
#267716=CARTESIAN_POINT('Ctrl Pts',(44.0208712025373,-56.5285586047056,
-40.7613849151889));
#267717=CARTESIAN_POINT('Ctrl Pts',(44.0518784813599,-56.521416173947,-40.7765333604643));
#267718=CARTESIAN_POINT('Ctrl Pts',(44.0937728041468,-56.5149820273198,
-40.799005697554));
#267719=CARTESIAN_POINT('Ctrl Pts',(44.1254693703652,-56.5117027703592,
-40.8169947136667));
#267720=CARTESIAN_POINT('Ctrl Pts',(44.1467868482481,-56.5105547568045,
-40.8297474946377));
#267721=CARTESIAN_POINT('Ctrl Pts',(44.1681963264173,-56.50993223545,-40.842882238999));
#267722=CARTESIAN_POINT('Ctrl Pts',(44.1789665479467,-56.509886262238,-40.8496544547178));
#267723=CARTESIAN_POINT('Ctrl Pts',(44.2003410646824,-56.5103214152413,
-40.8634176853611));
#267724=CARTESIAN_POINT('Ctrl Pts',(44.2109953322312,-56.5108003631786,
-40.8704389119319));
#267725=CARTESIAN_POINT('Ctrl Pts',(44.2322091102727,-56.5122711761573,
-40.8847351429132));
#267726=CARTESIAN_POINT('Ctrl Pts',(44.2639028799147,-56.5152466319394,
-40.9065696963621));
#267727=CARTESIAN_POINT('Ctrl Pts',(44.305661850593,-56.5222422564611,-40.9372114433545));
#267728=CARTESIAN_POINT('Ctrl Pts',(44.346925841944,-56.532247127269,-40.9693597045385));
#267729=CARTESIAN_POINT('Ctrl Pts',(44.3673876336497,-56.53826115526,-40.9859357593442));
#267730=CARTESIAN_POINT('Ctrl Pts',(44.3877715667723,-56.5447901720246,
-41.0027718870644));
#267731=CARTESIAN_POINT('Ctrl Pts',(44.3979208506631,-56.5483132560745,
-41.0113182564434));
#267732=CARTESIAN_POINT('Ctrl Pts',(44.4179418071922,-56.5558066378292,
-41.02850287128));
#267733=CARTESIAN_POINT('Ctrl Pts',(44.4278499085732,-56.5597882829787,
-41.0371710128992));
#267734=CARTESIAN_POINT('Ctrl Pts',(44.4572364860018,-56.5724196473794,
-41.0633712499365));
#267735=CARTESIAN_POINT('Ctrl Pts',(44.4763932211824,-56.581758968269,-41.0811111519311));
#267736=CARTESIAN_POINT('Ctrl Pts',(44.5044772880921,-56.5971447477014,
-41.1081262866225));
#267737=CARTESIAN_POINT('Ctrl Pts',(44.5137271775895,-56.6025015227711,
-41.1171962449124));
#267738=CARTESIAN_POINT('Ctrl Pts',(44.5320183562985,-56.6136863880645,
-41.1354834617267));
#267739=CARTESIAN_POINT('Ctrl Pts',(44.5410031705763,-56.6194798267371,
-41.144644186283));
#267740=CARTESIAN_POINT('Ctrl Pts',(44.5674276642847,-56.6374191091633,
-41.1721205907467));
#267741=CARTESIAN_POINT('Ctrl Pts',(44.5843870769067,-56.6501457393646,
-41.1904750382678));
#267742=CARTESIAN_POINT('Ctrl Pts',(44.616987890196,-56.6770839740703,-41.2272237610649));
#267743=CARTESIAN_POINT('Ctrl Pts',(44.640458797708,-56.6984048650555,-41.2548228473058));
#267744=CARTESIAN_POINT('Ctrl Pts',(44.6624514458289,-56.7214114906953,
-41.2824783924342));
#267745=CARTESIAN_POINT('Ctrl Pts',(44.6767798128067,-56.7371294193188,
-41.3009283158679));
#267746=CARTESIAN_POINT('Ctrl Pts',(44.683774397772,-56.7451748501741,-41.3101557240219));
#267747=CARTESIAN_POINT('Ctrl Pts',(44.6940202659092,-56.7575442973705,
-41.324018848177));
#267748=CARTESIAN_POINT('Ctrl Pts',(44.6973914635031,-56.7617145235639,
-41.328639728599));
#267749=CARTESIAN_POINT('Ctrl Pts',(44.7040131878578,-56.770108052971,-41.3378361513053));
#267750=CARTESIAN_POINT('Ctrl Pts',(44.7072703203268,-56.7743392575068,
-41.3424205878605));
#267751=CARTESIAN_POINT('Ctrl Pts',(44.7168707027477,-56.7871217033085,
-41.3561177927451));
#267752=CARTESIAN_POINT('Ctrl Pts',(44.7230524906066,-56.7957731420119,
-41.3651872799216));
#267753=CARTESIAN_POINT('Ctrl Pts',(44.7409373255192,-56.8220955492914,
-41.3921945478314));
#267754=CARTESIAN_POINT('Ctrl Pts',(44.7575187561203,-56.8491712652862,
-41.4188207502394));
#267755=CARTESIAN_POINT('Ctrl Pts',(44.7770214494108,-56.88676384976,-41.453559097464));
#267756=CARTESIAN_POINT('Ctrl Pts',(44.7858965000619,-56.9060633365117,
-41.4706740459328));
#267757=CARTESIAN_POINT('Ctrl Pts',(44.7943266372896,-56.9256180211132,
-41.4876605613939));
#267758=CARTESIAN_POINT('Ctrl Pts',(44.7983169540911,-56.9355169983302,
-41.4960845962979));
#267759=CARTESIAN_POINT('Ctrl Pts',(44.8058516078422,-56.9556000996462,
-41.5128223385875));
#267760=CARTESIAN_POINT('Ctrl Pts',(44.8093727854448,-56.9657242505397,
-41.5210856532432));
#267761=CARTESIAN_POINT('Ctrl Pts',(44.8191505788346,-56.9961959016236,
-41.5454418374945));
#267762=CARTESIAN_POINT('Ctrl Pts',(44.8246597322132,-57.0167187198372,
-41.5611704866007));
#267763=CARTESIAN_POINT('Ctrl Pts',(44.8336688220904,-57.0581479791523,
-41.5916045035181));
#267764=CARTESIAN_POINT('Ctrl Pts',(44.8389236650083,-57.0895139074259,
-41.613669368427));
#267765=CARTESIAN_POINT('Ctrl Pts',(44.8418900765893,-57.1213299669285,
-41.6345866129535));
#267766=CARTESIAN_POINT('Ctrl Pts',(44.8433488372948,-57.142640498193,-41.6482710687869));
#267767=CARTESIAN_POINT('Ctrl Pts',(44.8438191277705,-57.1533552116615,
-41.6549890353504));
#267768=CARTESIAN_POINT('Ctrl Pts',(44.8442270800594,-57.1748537940466,
-41.6681388704993));
#267769=CARTESIAN_POINT('Ctrl Pts',(44.8441639040618,-57.1855561823783,
-41.6745213422017));
#267770=CARTESIAN_POINT('Ctrl Pts',(44.8435122114514,-57.2069000331791,
-41.6869277892926));
#267771=CARTESIAN_POINT('Ctrl Pts',(44.8417458896958,-57.2388084678274,
-41.7049896680882));
#267772=CARTESIAN_POINT('Ctrl Pts',(44.8362687719071,-57.2809279665006,
-41.7269106712316));
#267773=CARTESIAN_POINT('Ctrl Pts',(44.8298088085522,-57.3121969378441,
-41.7417325167562));
#267774=CARTESIAN_POINT('Ctrl Pts',(44.8249713776488,-57.3329705079708,
-41.751249414817));
#267775=CARTESIAN_POINT('Ctrl Pts',(44.8222858794974,-57.3433254378487,
-41.7558274666229));
#267776=CARTESIAN_POINT('Ctrl Pts',(44.8163797073795,-57.3639440769784,
-41.7646063213672));
#267777=CARTESIAN_POINT('Ctrl Pts',(44.8131427147447,-57.3742522416544,
-41.7688238948253));
#267778=CARTESIAN_POINT('Ctrl Pts',(44.8061917406462,-57.3945668799698,
-41.7767918599254));
#267779=CARTESIAN_POINT('Ctrl Pts',(44.7987498536529,-57.4146412549335,
-41.7843210101159));
#267780=CARTESIAN_POINT('Ctrl Pts',(44.7861419817956,-57.4440129710611,
-41.7943060987191));
#267781=CARTESIAN_POINT('Ctrl Pts',(44.7720982599006,-57.4726583092559,
-41.8029984035242));
#267782=CARTESIAN_POINT('Ctrl Pts',(44.7566193423106,-57.5005749992605,
-41.8103989883131));
#267783=CARTESIAN_POINT('Ctrl Pts',(44.7453362941317,-57.518697088903,-41.8144666236875));
#267784=CARTESIAN_POINT('Ctrl Pts',(44.7335642473644,-57.5365709174371,
-41.8180952379985));
#267785=CARTESIAN_POINT('Ctrl Pts',(44.7274378249752,-57.5453780864623,
-41.8196891344695));
#267786=CARTESIAN_POINT('Ctrl Pts',(44.7146685840676,-57.5627610237142,
-41.8224320230444));
#267787=CARTESIAN_POINT('Ctrl Pts',(44.7080700862024,-57.5712755128024,
-41.8235709343319));
#267788=CARTESIAN_POINT('Ctrl Pts',(44.6877341610586,-57.5961705213949,
-41.8262807978491));
#267789=CARTESIAN_POINT('Ctrl Pts',(44.6734117165454,-57.6119810052107,
-41.8271650529119));
#267790=CARTESIAN_POINT('Ctrl Pts',(44.6432859415473,-57.6420285404153,
-41.827118555904));
#267791=CARTESIAN_POINT('Ctrl Pts',(44.6274777219699,-57.6562729242579,
-41.8261892556471));
#267792=CARTESIAN_POINT('Ctrl Pts',(44.6026489360012,-57.6764545436153,
-41.823427013232));
#267793=CARTESIAN_POINT('Ctrl Pts',(44.5941811636919,-57.6829873126311,
-41.8222767907821));
#267794=CARTESIAN_POINT('Ctrl Pts',(44.5812011369499,-57.6924815728277,
-41.820204446988));
#267795=CARTESIAN_POINT('Ctrl Pts',(44.5768239301145,-57.6955981764101,
-41.8194549553751));
#267796=CARTESIAN_POINT('Ctrl Pts',(44.5679795363474,-57.7017261947271,
-41.8178398084084));
#267797=CARTESIAN_POINT('Ctrl Pts',(44.554547495243,-57.7107794649358,-41.8152360293365));
#267798=CARTESIAN_POINT('Ctrl Pts',(44.5408745509057,-57.7192473537464,
-41.812140181677));
#267799=CARTESIAN_POINT('Ctrl Pts',(44.5224181841827,-57.7300417662926,
-41.8075820007456));
#267800=CARTESIAN_POINT('Ctrl Pts',(44.494403164631,-57.7454824222945,-41.8000999642091));
#267801=CARTESIAN_POINT('Ctrl Pts',(44.4557509611988,-57.7631175354143,
-41.7875858630695));
#267802=CARTESIAN_POINT('Ctrl Pts',(44.4257963579031,-57.7741479888816,
-41.7763064650726));
#267803=CARTESIAN_POINT('Ctrl Pts',(44.4056101875344,-57.781009218212,-41.7683613570464));
#267804=CARTESIAN_POINT('Ctrl Pts',(44.3954036594654,-57.7841949818065,
-41.7641737395871));
#267805=CARTESIAN_POINT('Ctrl Pts',(44.3747925009816,-57.7900627169564,
-41.7553761870634));
#267806=CARTESIAN_POINT('Ctrl Pts',(44.3643365899562,-57.7927558542442,
-41.7507422904685));
#267807=CARTESIAN_POINT('Ctrl Pts',(44.3329536886806,-57.7999988857253,
-41.7363257213199));
#267808=CARTESIAN_POINT('Ctrl Pts',(44.3014645871824,-57.8056090798854,
-41.7208580810542));
#267809=CARTESIAN_POINT('Ctrl Pts',(44.2698183189435,-57.8088603667088,
-41.7038603653999));
#267810=CARTESIAN_POINT('Ctrl Pts',(44.2381206623806,-57.8113308880715,
-41.6863549522799));
#267811=CARTESIAN_POINT('Ctrl Pts',(44.2169139506954,-57.8119384373532,
-41.6740048606234));
#267812=CARTESIAN_POINT('Ctrl Pts',(44.1850197107514,-57.811287280344,-41.6544681547659));
#267813=CARTESIAN_POINT('Ctrl Pts',(44.1743613109546,-57.8108078241776,
-41.6477783242763));
#267814=CARTESIAN_POINT('Ctrl Pts',(44.1583626375358,-57.8096935003687,
-41.6374930176863));
#267815=CARTESIAN_POINT('Ctrl Pts',(44.1530230189312,-57.809255510817,-41.6340194660765));
#267816=CARTESIAN_POINT('Ctrl Pts',(44.1423341247923,-57.8082460206643,
-41.6269840076234));
#267817=CARTESIAN_POINT('Ctrl Pts',(44.1369894952372,-57.8076746784434,
-41.6234249849254));
#267818=CARTESIAN_POINT('Ctrl Pts',(44.1103928894951,-57.8045001122898,
-41.6055088472864));
#267819=CARTESIAN_POINT('Ctrl Pts',(44.0684216046586,-57.7973782151022,
-41.5759273380954));
#267820=CARTESIAN_POINT('Ctrl Pts',(44.0275807082801,-57.78632659952,-41.5445717124501));
#267821=CARTESIAN_POINT('Ctrl Pts',(43.9872978152183,-57.7733311875938,
-41.5123297976061));
#267822=CARTESIAN_POINT('Ctrl Pts',(43.9674326520914,-57.7658590768128,
-41.4957625032292));
#267823=CARTESIAN_POINT('Ctrl Pts',(43.942963744406,-57.7552890823142,-41.4744937232973));
#267824=CARTESIAN_POINT('Ctrl Pts',(43.938085174092,-57.7531113051098,-41.4702088025761));
#267825=CARTESIAN_POINT('Ctrl Pts',(43.9283699185172,-57.7486342535987,
-41.4615871928557));
#267826=CARTESIAN_POINT('Ctrl Pts',(43.9235236029976,-57.7463299238453,
-41.4572415669043));
#267827=CARTESIAN_POINT('Ctrl Pts',(43.9090930604083,-57.739254093668,-41.4441663196977));
#267828=CARTESIAN_POINT('Ctrl Pts',(43.8996324205383,-57.7343289686206,
-41.4354132012863));
#267829=CARTESIAN_POINT('Ctrl Pts',(43.8903154257419,-57.7291941381088,
-41.4266127101804));
#267830=CARTESIAN_POINT('Ctrl Pts',(43.4805771074156,-59.5712767529309,
-39.2399080357013));
#267831=CARTESIAN_POINT('Ctrl Pts',(43.4150727209207,-59.5358440364426,
-39.2223070534893));
#267832=CARTESIAN_POINT('Ctrl Pts',(43.2883193276586,-59.4590682572254,
-39.1867578392588));
#267833=CARTESIAN_POINT('Ctrl Pts',(43.1106712693135,-59.32658002426,-39.1324031814995));
#267834=CARTESIAN_POINT('Ctrl Pts',(43.0005921597408,-59.2266373021163,
-39.0954660506179));
#267835=CARTESIAN_POINT('Ctrl Pts',(42.8948534568781,-59.1207134074407,
-39.0581733199915));
#267836=CARTESIAN_POINT('Ctrl Pts',(42.7951360401793,-59.0104958554849,
-39.0211184761739));
#267837=CARTESIAN_POINT('Ctrl Pts',(42.6850011896347,-58.8622904152127,
-38.9753582681256));
#267838=CARTESIAN_POINT('Ctrl Pts',(42.6055727997797,-58.7375004045667,
-38.939089851323));
#267839=CARTESIAN_POINT('Ctrl Pts',(42.5503788594446,-58.6407591922129,
-38.9120596161462));
#267840=CARTESIAN_POINT('Ctrl Pts',(42.5165536369311,-58.5741539171446,
-38.8941613358138));
#267841=CARTESIAN_POINT('Ctrl Pts',(42.4842288567228,-58.5064298632496,
-38.8763157156907));
#267842=CARTESIAN_POINT('Ctrl Pts',(42.4689425396028,-58.4722695523732,
-38.8674882509199));
#267843=CARTESIAN_POINT('Ctrl Pts',(42.4257123024776,-58.3690064948315,
-38.8413136266604));
#267844=CARTESIAN_POINT('Ctrl Pts',(42.3750272156063,-58.229152189777,-38.8072100415055));
#267845=CARTESIAN_POINT('Ctrl Pts',(42.3380647902547,-58.0850119200902,
-38.7746901633276));
#267846=CARTESIAN_POINT('Ctrl Pts',(42.3155659796374,-57.9752818499468,
-38.7509105250088));
#267847=CARTESIAN_POINT('Ctrl Pts',(42.3089374211558,-57.9384266221928,
-38.7430843922672));
#267848=CARTESIAN_POINT('Ctrl Pts',(42.297458012674,-57.864178756387,-38.7276438637217));
#267849=CARTESIAN_POINT('Ctrl Pts',(42.292601515188,-57.8267325312259,-38.720018782004));
#267850=CARTESIAN_POINT('Ctrl Pts',(42.2847289916893,-57.7514526301959,
-38.7050196673963));
#267851=CARTESIAN_POINT('Ctrl Pts',(42.2817363521424,-57.7138759968928,
-38.6976962453237));
#267852=CARTESIAN_POINT('Ctrl Pts',(42.277596992864,-57.6387184974263,-38.6833720377019));
#267853=CARTESIAN_POINT('Ctrl Pts',(42.2741651307842,-57.5260409596698,
-38.6623829091612));
#267854=CARTESIAN_POINT('Ctrl Pts',(42.2805893100654,-57.3760354719141,
-38.6363740800325));
#267855=CARTESIAN_POINT('Ctrl Pts',(42.2937061680812,-57.2637038035873,
-38.618370061439));
#267856=CARTESIAN_POINT('Ctrl Pts',(42.3043247017591,-57.1888547452426,
-38.6067079534822));
#267857=CARTESIAN_POINT('Ctrl Pts',(42.3105743117123,-57.1514345461221,
-38.6010450635964));
#267858=CARTESIAN_POINT('Ctrl Pts',(42.3249704170347,-57.0766935209607,
-38.590076215021));
#267859=CARTESIAN_POINT('Ctrl Pts',(42.3331592025312,-57.0392159768686,
-38.5847494243559));
#267860=CARTESIAN_POINT('Ctrl Pts',(42.3512949844302,-56.9651221381903,
-38.5745673038812));
#267861=CARTESIAN_POINT('Ctrl Pts',(42.3712216906218,-56.8916587034686,
-38.564820665347));
#267862=CARTESIAN_POINT('Ctrl Pts',(42.4063979707918,-56.7834465224234,
-38.5515118436));
#267863=CARTESIAN_POINT('Ctrl Pts',(42.4468320479729,-56.6771725078319,
-38.5395042677724));
#267864=CARTESIAN_POINT('Ctrl Pts',(42.4925290654744,-56.5728473165674,
-38.5288039137004));
#267865=CARTESIAN_POINT('Ctrl Pts',(42.5265325119253,-56.5046058456765,
-38.5225509073062));
#267866=CARTESIAN_POINT('Ctrl Pts',(42.5623338475306,-56.4370293947697,
-38.5167461666044));
#267867=CARTESIAN_POINT('Ctrl Pts',(42.5811223641794,-56.4035923099625,
-38.5140693065785));
#267868=CARTESIAN_POINT('Ctrl Pts',(42.620584523009,-56.3373241998654,-38.5091697400817));
#267869=CARTESIAN_POINT('Ctrl Pts',(42.6411082254821,-56.3047465904101,
-38.5069659500128));
#267870=CARTESIAN_POINT('Ctrl Pts',(42.7048067991197,-56.2090283357163,
-38.501110858935));
#267871=CARTESIAN_POINT('Ctrl Pts',(42.7502234543428,-56.1476408662828,
-38.4981890389281));
#267872=CARTESIAN_POINT('Ctrl Pts',(42.8467942323831,-56.0297655581676,
-38.4942910511033));
#267873=CARTESIAN_POINT('Ctrl Pts',(42.8979715413934,-55.9732420482176,
-38.4933125989996));
#267874=CARTESIAN_POINT('Ctrl Pts',(42.9790570553347,-55.8921695883033,
-38.4933149859729));
#267875=CARTESIAN_POINT('Ctrl Pts',(43.0068374106561,-55.8657400908868,
-38.4935622007431));
#267876=CARTESIAN_POINT('Ctrl Pts',(43.0495800649421,-55.8270637749536,
-38.4943063068789));
#267877=CARTESIAN_POINT('Ctrl Pts',(43.0640222060113,-55.8143203511958,
-38.494617152342));
#267878=CARTESIAN_POINT('Ctrl Pts',(43.0932714774893,-55.7891564261061,
-38.4953646906773));
#267879=CARTESIAN_POINT('Ctrl Pts',(43.1080901283632,-55.7767277938553,
-38.4958020036096));
#267880=CARTESIAN_POINT('Ctrl Pts',(43.1528523310046,-55.7401327167866,
-38.4972962980169));
#267881=CARTESIAN_POINT('Ctrl Pts',(43.2134913856688,-55.6930468850421,
-38.4997758707861));
#267882=CARTESIAN_POINT('Ctrl Pts',(43.3385569247743,-55.6055389451161,
-38.5066450244003));
#267883=CARTESIAN_POINT('Ctrl Pts',(43.4691986576013,-55.5278792007279,
-38.5163302992824));
#267884=CARTESIAN_POINT('Ctrl Pts',(43.5713395927684,-55.4769743237494,
-38.5256877381308));
#267885=CARTESIAN_POINT('Ctrl Pts',(43.6403672861995,-55.4446857735354,
-38.5323951500278));
#267886=CARTESIAN_POINT('Ctrl Pts',(43.6753577685123,-55.4293620157832,
-38.5359845633874));
#267887=CARTESIAN_POINT('Ctrl Pts',(43.7462462065788,-55.4003985583156,
-38.5436333065981));
#267888=CARTESIAN_POINT('Ctrl Pts',(43.7822717759725,-55.3867204456352,
-38.5477088862383));
#267889=CARTESIAN_POINT('Ctrl Pts',(43.8543821738219,-55.3613797848081,
-38.5562346427694));
#267890=CARTESIAN_POINT('Ctrl Pts',(43.890622407919,-55.349649082917,-38.5607007444526));
#267891=CARTESIAN_POINT('Ctrl Pts',(43.9997560709039,-55.3172704656441,
-38.5746802407103));
#267892=CARTESIAN_POINT('Ctrl Pts',(44.1098017310836,-55.290468361793,-38.5898286859852));
#267893=CARTESIAN_POINT('Ctrl Pts',(44.2583166685835,-55.2656490138239,
-38.612301023075));
#267894=CARTESIAN_POINT('Ctrl Pts',(44.3705972700495,-55.2524997368729,
-38.6302900391873));
#267895=CARTESIAN_POINT('Ctrl Pts',(44.446056048267,-55.2474029004138,-38.6430428201589));
#267896=CARTESIAN_POINT('Ctrl Pts',(44.5218128020516,-55.2441636366351,
-38.65617756452));
#267897=CARTESIAN_POINT('Ctrl Pts',(44.5599089424743,-55.2434808562086,
-38.6629497802385));
#267898=CARTESIAN_POINT('Ctrl Pts',(44.6354869543582,-55.2439911084578,
-38.6767130108817));
#267899=CARTESIAN_POINT('Ctrl Pts',(44.6731456892459,-55.2451740103824,
-38.6837342374529));
#267900=CARTESIAN_POINT('Ctrl Pts',(44.7481014788608,-55.2493620066237,
-38.6980304684339));
#267901=CARTESIAN_POINT('Ctrl Pts',(44.860046548974,-55.2583760573225,-38.7198650218829));
#267902=CARTESIAN_POINT('Ctrl Pts',(45.0073845433675,-55.2811507310277,
-38.7505067688753));
#267903=CARTESIAN_POINT('Ctrl Pts',(45.1528189888476,-55.3146135839333,
-38.7826550300594));
#267904=CARTESIAN_POINT('Ctrl Pts',(45.2248832056965,-55.3349380951144,
-38.7992310848652));
#267905=CARTESIAN_POINT('Ctrl Pts',(45.2966462681613,-55.3570913336823,
-38.8160672125853));
#267906=CARTESIAN_POINT('Ctrl Pts',(45.3323638946335,-55.3690863290504,
-38.8246135819642));
#267907=CARTESIAN_POINT('Ctrl Pts',(45.4027951436545,-55.3946744461232,
-38.841798196801));
#267908=CARTESIAN_POINT('Ctrl Pts',(45.4376370321487,-55.4083060218429,
-38.85046633842));
#267909=CARTESIAN_POINT('Ctrl Pts',(45.5409345111852,-55.4516493275196,
-38.8766665754573));
#267910=CARTESIAN_POINT('Ctrl Pts',(45.6082182891413,-55.4838201174091,
-38.8944064774514));
#267911=CARTESIAN_POINT('Ctrl Pts',(45.7067749877369,-55.5369855856676,
-38.9214216121435));
#267912=CARTESIAN_POINT('Ctrl Pts',(45.7392219877795,-55.5555212114618,
-38.9304915704334));
#267913=CARTESIAN_POINT('Ctrl Pts',(45.8033556832395,-55.5942722159849,
-38.9487787872477));
#267914=CARTESIAN_POINT('Ctrl Pts',(45.8348443691401,-55.6143675312756,
-38.9579395118015));
#267915=CARTESIAN_POINT('Ctrl Pts',(45.9274099842789,-55.6766589025306,
-38.9854159162723));
#267916=CARTESIAN_POINT('Ctrl Pts',(45.9867610865919,-55.7209353156014,
-39.0037703637879));
#267917=CARTESIAN_POINT('Ctrl Pts',(46.1007337830098,-55.8148102393793,
-39.0405190865864));
#267918=CARTESIAN_POINT('Ctrl Pts',(46.1826971388658,-55.889219933262,-39.0681181728269));
#267919=CARTESIAN_POINT('Ctrl Pts',(46.259356574729,-55.9696687352924,-39.0957737179551));
#267920=CARTESIAN_POINT('Ctrl Pts',(46.309266807939,-56.024663053365,-39.1142236413887));
#267921=CARTESIAN_POINT('Ctrl Pts',(46.3336138177017,-56.0528284109483,
-39.1234510495426));
#267922=CARTESIAN_POINT('Ctrl Pts',(46.3692509284248,-56.0961546965833,
-39.1373141736981));
#267923=CARTESIAN_POINT('Ctrl Pts',(46.3809719555493,-56.1107655250657,
-39.14193505412));
#267924=CARTESIAN_POINT('Ctrl Pts',(46.4039850968433,-56.1401806715041,
-39.1511314768264));
#267925=CARTESIAN_POINT('Ctrl Pts',(46.4153001903629,-56.1550126624776,
-39.1557159133813));
#267926=CARTESIAN_POINT('Ctrl Pts',(46.4486370096885,-56.1998310060263,
-39.1694131182659));
#267927=CARTESIAN_POINT('Ctrl Pts',(46.4700835091466,-56.2301795317326,
-39.1784826054425));
#267928=CARTESIAN_POINT('Ctrl Pts',(46.532071913686,-56.3225583984772,-39.2054898733524));
#267929=CARTESIAN_POINT('Ctrl Pts',(46.5894197348374,-56.4176636744323,
-39.23211607576));
#267930=CARTESIAN_POINT('Ctrl Pts',(46.6566074362748,-56.5498680842415,
-39.2668544229849));
#267931=CARTESIAN_POINT('Ctrl Pts',(46.6870820302515,-56.617790568625,-39.2839693714534));
#267932=CARTESIAN_POINT('Ctrl Pts',(46.7159729830272,-56.6866360545619,
-39.3009558869148));
#267933=CARTESIAN_POINT('Ctrl Pts',(46.7296188023799,-56.7214992889704,
-39.3093799218186));
#267934=CARTESIAN_POINT('Ctrl Pts',(46.7553216997643,-56.7922546384013,
-39.3261176641085));
#267935=CARTESIAN_POINT('Ctrl Pts',(46.7672996943011,-56.8279354881579,
-39.3343809787628));
#267936=CARTESIAN_POINT('Ctrl Pts',(46.8004530502947,-56.9353633959568,
-39.358737163018));
#267937=CARTESIAN_POINT('Ctrl Pts',(46.8189795501832,-57.0077635587999,
-39.3744658121213));
#267938=CARTESIAN_POINT('Ctrl Pts',(46.848916211803,-57.1540080946302,-39.4048998290393));
#267939=CARTESIAN_POINT('Ctrl Pts',(46.866048617508,-57.2647966217996,-39.4269646939479));
#267940=CARTESIAN_POINT('Ctrl Pts',(46.875074749658,-57.3772756893033,-39.4478819384746));
#267941=CARTESIAN_POINT('Ctrl Pts',(46.8792542953452,-57.4526370309597,
-39.4615663943076));
#267942=CARTESIAN_POINT('Ctrl Pts',(46.8804258736835,-57.4905390832845,
-39.4682843608713));
#267943=CARTESIAN_POINT('Ctrl Pts',(46.8808837743635,-57.566610437341,-39.4814341960201));
#267944=CARTESIAN_POINT('Ctrl Pts',(46.8801708637706,-57.604491394965,-39.4878166677226));
#267945=CARTESIAN_POINT('Ctrl Pts',(46.8768913879562,-57.6800597985945,
-39.5002231148134));
#267946=CARTESIAN_POINT('Ctrl Pts',(46.8691896925243,-57.7930657109158,
-39.5182849936093));
#267947=CARTESIAN_POINT('Ctrl Pts',(46.8479069711518,-57.9423669591112,
-39.540205996752));
#267948=CARTESIAN_POINT('Ctrl Pts',(46.8236459543104,-58.053306681129,-39.5550278422771));
#267949=CARTESIAN_POINT('Ctrl Pts',(46.8055990109883,-58.1270324939452,
-39.5645447403379));
#267950=CARTESIAN_POINT('Ctrl Pts',(46.7956339676918,-58.1637938532181,
-39.5691227921436));
#267951=CARTESIAN_POINT('Ctrl Pts',(46.7738161327052,-58.2370162077019,
-39.5779016468881));
#267952=CARTESIAN_POINT('Ctrl Pts',(46.7619036278491,-58.2736352268715,
-39.5821192203466));
#267953=CARTESIAN_POINT('Ctrl Pts',(46.7364059718256,-58.3458255995332,
-39.5900871854462));
#267954=CARTESIAN_POINT('Ctrl Pts',(46.7091836493705,-58.4171862986019,
-39.5976163356366));
#267955=CARTESIAN_POINT('Ctrl Pts',(46.663274408039,-58.5216699086648,-39.6076014242402));
#267956=CARTESIAN_POINT('Ctrl Pts',(46.6123207377325,-58.6236436013082,
-39.616293729045));
#267957=CARTESIAN_POINT('Ctrl Pts',(46.5563244858032,-58.7230996041114,
-39.6236943138341));
#267958=CARTESIAN_POINT('Ctrl Pts',(46.515607032986,-58.7877140896312,-39.6277619492082));
#267959=CARTESIAN_POINT('Ctrl Pts',(46.4731710833873,-58.8514710047945,
-39.6313905635194));
#267960=CARTESIAN_POINT('Ctrl Pts',(46.4511086137465,-58.8829006319494,
-39.6329844599904));
#267961=CARTESIAN_POINT('Ctrl Pts',(46.4051673201274,-58.9449633016888,
-39.6357273485653));
#267962=CARTESIAN_POINT('Ctrl Pts',(46.381447994276,-58.975377588932,-39.6368662598532));
#267963=CARTESIAN_POINT('Ctrl Pts',(46.3084068909562,-59.0643493136614,
-39.6395761233691));
#267964=CARTESIAN_POINT('Ctrl Pts',(46.2570407846102,-59.1209150453974,
-39.6404603784325));
#267965=CARTESIAN_POINT('Ctrl Pts',(46.1491379755941,-59.228544463199,-39.6404138814247));
#267966=CARTESIAN_POINT('Ctrl Pts',(46.0925836555155,-59.2796343044913,
-39.6394845811684));
#267967=CARTESIAN_POINT('Ctrl Pts',(46.0038529437629,-59.3521266125547,
-39.6367223387528));
#267968=CARTESIAN_POINT('Ctrl Pts',(45.9736068078661,-59.3756113554055,
-39.6355721163029));
#267969=CARTESIAN_POINT('Ctrl Pts',(45.9272656961273,-59.4097723546528,
-39.6334997725088));
#267970=CARTESIAN_POINT('Ctrl Pts',(45.9116419215573,-59.4209912820171,
-39.6327502808957));
#267971=CARTESIAN_POINT('Ctrl Pts',(45.8800804794677,-59.4430610802669,
-39.6311351339295));
#267972=CARTESIAN_POINT('Ctrl Pts',(45.8321587971618,-59.4756823489919,
-39.628531354857));
#267973=CARTESIAN_POINT('Ctrl Pts',(45.7834097108732,-59.5062438963941,
-39.6254355071979));
#267974=CARTESIAN_POINT('Ctrl Pts',(45.717633106262,-59.5452481912826,-39.6208773262667));
#267975=CARTESIAN_POINT('Ctrl Pts',(45.6178307490054,-59.601113548897,-39.6133952897297));
#267976=CARTESIAN_POINT('Ctrl Pts',(45.4802897643185,-59.6652183443042,
-39.6008811885904));
#267977=CARTESIAN_POINT('Ctrl Pts',(45.3738098009101,-59.7055766782111,
-39.5896017905935));
#267978=CARTESIAN_POINT('Ctrl Pts',(45.3020778813705,-59.7307512119865,
-39.5816566825671));
#267979=CARTESIAN_POINT('Ctrl Pts',(45.2658207311094,-59.7424779859237,
-39.5774690651077));
#267980=CARTESIAN_POINT('Ctrl Pts',(45.1926264675053,-59.7641596016776,
-39.5686715125846));
#267981=CARTESIAN_POINT('Ctrl Pts',(45.1555073907618,-59.7741562512684,
-39.5640376159893));
#267982=CARTESIAN_POINT('Ctrl Pts',(45.0441315765335,-59.8011904590316,
-39.5496210468413));
#267983=CARTESIAN_POINT('Ctrl Pts',(44.9324484012679,-59.8224577850013,
-39.5341534065747));
#267984=CARTESIAN_POINT('Ctrl Pts',(44.8203079610257,-59.8353953605365,
-39.5171556909205));
#267985=CARTESIAN_POINT('Ctrl Pts',(44.7080184564226,-59.8455760612675,
-39.4996502778008));
#267986=CARTESIAN_POINT('Ctrl Pts',(44.6329372249224,-59.8486931621852,
-39.4873001861445));
#267987=CARTESIAN_POINT('Ctrl Pts',(44.5200834441659,-59.8478515133141,
-39.4677634802869));
#267988=CARTESIAN_POINT('Ctrl Pts',(44.4823810871712,-59.8466449718289,
-39.4610736497974));
#267989=CARTESIAN_POINT('Ctrl Pts',(44.4258051079382,-59.8434394706745,
-39.4507883432074));
#267990=CARTESIAN_POINT('Ctrl Pts',(44.4069254589855,-59.8421361346926,
-39.4473147915973));
#267991=CARTESIAN_POINT('Ctrl Pts',(44.3691376542581,-59.8390581625153,
-39.4402793331445));
#267992=CARTESIAN_POINT('Ctrl Pts',(44.3502459350849,-59.8372838734483,
-39.4367203104461));
#267993=CARTESIAN_POINT('Ctrl Pts',(44.2562487381671,-59.8272835659938,
-39.4188041728073));
#267994=CARTESIAN_POINT('Ctrl Pts',(44.1080045765469,-59.8040393501646,
-39.3892226636159));
#267995=CARTESIAN_POINT('Ctrl Pts',(43.9639303529155,-59.7668593120831,
-39.3578670379715));
#267996=CARTESIAN_POINT('Ctrl Pts',(43.8219159040518,-59.7227861654643,
-39.3256251231267));
#267997=CARTESIAN_POINT('Ctrl Pts',(43.7519290534068,-59.6972943066161,
-39.3090578287531));
#267998=CARTESIAN_POINT('Ctrl Pts',(43.665783177736,-59.6610675807531,-39.2877890488175));
#267999=CARTESIAN_POINT('Ctrl Pts',(43.6486106666635,-59.653596197985,-39.2835041280971));
#268000=CARTESIAN_POINT('Ctrl Pts',(43.6144193015916,-59.6382222359849,
-39.2748825183767));
#268001=CARTESIAN_POINT('Ctrl Pts',(43.597366582891,-59.6303022352814,-39.2705368924251));
#268002=CARTESIAN_POINT('Ctrl Pts',(43.5465994182959,-59.605961903298,-39.2574616452183));
#268003=CARTESIAN_POINT('Ctrl Pts',(43.513329300663,-59.588993111175,-39.2487085268073));
#268004=CARTESIAN_POINT('Ctrl Pts',(43.4805771074156,-59.5712767529309,
-39.2399080357013));
#268005=CARTESIAN_POINT('Ctrl Pts',(43.8903154257419,-57.7291941381088,
-41.4266127101804));
#268006=CARTESIAN_POINT('Ctrl Pts',(43.8716814361492,-57.7189244770852,
-41.4090117279687));
#268007=CARTESIAN_POINT('Ctrl Pts',(43.8355945080866,-57.6967277837834,
-41.3734625137379));
#268008=CARTESIAN_POINT('Ctrl Pts',(43.7849271573585,-57.6585752750105,
-41.3191078559793));
#268009=CARTESIAN_POINT('Ctrl Pts',(43.753465403225,-57.62988352171,-41.2821707250961));
#268010=CARTESIAN_POINT('Ctrl Pts',(43.7232071092872,-57.5995155202448,
-41.2448779944712));
#268011=CARTESIAN_POINT('Ctrl Pts',(43.694633283399,-57.5679550683129,-41.2078231506529));
#268012=CARTESIAN_POINT('Ctrl Pts',(43.6629744005209,-57.5256074013359,
-41.162062942605));
#268013=CARTESIAN_POINT('Ctrl Pts',(43.6400741040405,-57.4900012877665,
-41.1257945258022));
#268014=CARTESIAN_POINT('Ctrl Pts',(43.624122646482,-57.4624228770549,-41.0987642906252));
#268015=CARTESIAN_POINT('Ctrl Pts',(43.6143188854815,-57.4434516436916,
-41.0808660102928));
#268016=CARTESIAN_POINT('Ctrl Pts',(43.6049343759216,-57.4241698350281,
-41.0630203901697));
#268017=CARTESIAN_POINT('Ctrl Pts',(43.6004882740613,-57.4144479878336,
-41.054192925399));
#268018=CARTESIAN_POINT('Ctrl Pts',(43.5878889573419,-57.3850715912746,
-41.0280183011396));
#268019=CARTESIAN_POINT('Ctrl Pts',(43.5730447416356,-57.3453166524842,
-40.9939147159844));
#268020=CARTESIAN_POINT('Ctrl Pts',(43.5620571572655,-57.3044044614592,
-40.9613948378065));
#268021=CARTESIAN_POINT('Ctrl Pts',(43.5552843243605,-57.2732819874194,
-40.9376151994878));
#268022=CARTESIAN_POINT('Ctrl Pts',(43.5532714802541,-57.2628325912303,
-40.9297890667463));
#268023=CARTESIAN_POINT('Ctrl Pts',(43.5497454556161,-57.2417890776549,
-40.9143485382007));
#268024=CARTESIAN_POINT('Ctrl Pts',(43.5482304746054,-57.2311797832666,
-40.9067234564832));
#268025=CARTESIAN_POINT('Ctrl Pts',(43.5457184756399,-57.2098591834555,
-40.8917243418755));
#268026=CARTESIAN_POINT('Ctrl Pts',(43.5447290487245,-57.199220662917,-40.8844009198028));
#268027=CARTESIAN_POINT('Ctrl Pts',(43.5432711863927,-57.1779500447907,
-40.8700767121812));
#268028=CARTESIAN_POINT('Ctrl Pts',(43.5418684734652,-57.1460721839032,
-40.8490875836402));
#268029=CARTESIAN_POINT('Ctrl Pts',(43.5431039253892,-57.1036793909824,
-40.8230787545116));
#268030=CARTESIAN_POINT('Ctrl Pts',(43.5463738329101,-57.0719682486671,
-40.8050747359183));
#268031=CARTESIAN_POINT('Ctrl Pts',(43.5490829635055,-57.0508462881094,
-40.7934126279614));
#268032=CARTESIAN_POINT('Ctrl Pts',(43.5507030159248,-57.0402904723448,
-40.7877497380755));
#268033=CARTESIAN_POINT('Ctrl Pts',(43.5544790630841,-57.019214904491,-40.7767808895002));
#268034=CARTESIAN_POINT('Ctrl Pts',(43.5566463931059,-57.0086510117152,
-40.7714540988351));
#268035=CARTESIAN_POINT('Ctrl Pts',(43.5614808344627,-56.9877741662596,
-40.7612719783604));
#268036=CARTESIAN_POINT('Ctrl Pts',(43.5668234022498,-56.9670831174431,
-40.7515253398262));
#268037=CARTESIAN_POINT('Ctrl Pts',(43.5763377125496,-56.9366295208774,
-40.7382165180791));
#268038=CARTESIAN_POINT('Ctrl Pts',(43.5873444561754,-56.9067460923864,
-40.7262089422516));
#268039=CARTESIAN_POINT('Ctrl Pts',(43.5998453117462,-56.8774358278222,
-40.7155085881795));
#268040=CARTESIAN_POINT('Ctrl Pts',(43.6091839698139,-56.8582805167828,
-40.7092555817853));
#268041=CARTESIAN_POINT('Ctrl Pts',(43.6190331668358,-56.8393207538612,
-40.7034508410834));
#268042=CARTESIAN_POINT('Ctrl Pts',(43.6242099732076,-56.8299438685379,
-40.7007739810578));
#268043=CARTESIAN_POINT('Ctrl Pts',(43.6350986096338,-56.8113693026126,
-40.6958744145609));
#268044=CARTESIAN_POINT('Ctrl Pts',(43.6407690742328,-56.8022426567881,
-40.6936706244929));
#268045=CARTESIAN_POINT('Ctrl Pts',(43.6583896223854,-56.7754411523649,
-40.6878155334118));
#268046=CARTESIAN_POINT('Ctrl Pts',(43.6709801307092,-56.7582712890167,
-40.6848937134075));
#268047=CARTESIAN_POINT('Ctrl Pts',(43.6978023804218,-56.725340315416,-40.6809957255822));
#268048=CARTESIAN_POINT('Ctrl Pts',(43.7120405319879,-56.7095692151415,
-40.6800172734785));
#268049=CARTESIAN_POINT('Ctrl Pts',(43.7346338722206,-56.6869796178674,
-40.680019660452));
#268050=CARTESIAN_POINT('Ctrl Pts',(43.7423799312797,-56.6796208977126,
-40.6802668752224));
#268051=CARTESIAN_POINT('Ctrl Pts',(43.7543060585229,-56.6688607312791,
-40.681010981358));
#268052=CARTESIAN_POINT('Ctrl Pts',(43.7583370517177,-56.6653168192219,
-40.6813218268212));
#268053=CARTESIAN_POINT('Ctrl Pts',(43.7665035456834,-56.6583217341419,
-40.6820693651562));
#268054=CARTESIAN_POINT('Ctrl Pts',(43.7706422703,-56.6548683091639,-40.6825066780886));
#268055=CARTESIAN_POINT('Ctrl Pts',(43.7831478581881,-56.6447045100584,
-40.6840009724959));
#268056=CARTESIAN_POINT('Ctrl Pts',(43.8000992888712,-56.6316392340345,
-40.6864805452653));
#268057=CARTESIAN_POINT('Ctrl Pts',(43.8351004518507,-56.6074069729907,
-40.6933496988796));
#268058=CARTESIAN_POINT('Ctrl Pts',(43.8717190640765,-56.5859796680779,
-40.7030349737613));
#268059=CARTESIAN_POINT('Ctrl Pts',(43.9003898794618,-56.5719991465823,
-40.7123924126099));
#268060=CARTESIAN_POINT('Ctrl Pts',(43.919774692733,-56.5631479893168,-40.719099824507));
#268061=CARTESIAN_POINT('Ctrl Pts',(43.9296053152689,-56.5589560552736,
-40.722689237866));
#268062=CARTESIAN_POINT('Ctrl Pts',(43.9495302416178,-56.551051384942,-40.7303379810773));
#268063=CARTESIAN_POINT('Ctrl Pts',(43.959660471973,-56.5473282955902,-40.7344135607172));
#268064=CARTESIAN_POINT('Ctrl Pts',(43.9799461530017,-56.5404515818703,
-40.7429393172485));
#268065=CARTESIAN_POINT('Ctrl Pts',(43.9901452646573,-56.5372793127045,
-40.7474054189318));
#268066=CARTESIAN_POINT('Ctrl Pts',(44.0208712025373,-56.5285586047056,
-40.7613849151889));
#268067=CARTESIAN_POINT('Ctrl Pts',(44.0518784813599,-56.521416173947,-40.7765333604643));
#268068=CARTESIAN_POINT('Ctrl Pts',(44.0937728041468,-56.5149820273198,
-40.799005697554));
#268069=CARTESIAN_POINT('Ctrl Pts',(44.1254693703652,-56.5117027703592,
-40.8169947136667));
#268070=CARTESIAN_POINT('Ctrl Pts',(44.1467868482481,-56.5105547568045,
-40.8297474946377));
#268071=CARTESIAN_POINT('Ctrl Pts',(44.1681963264173,-56.50993223545,-40.842882238999));
#268072=CARTESIAN_POINT('Ctrl Pts',(44.1789665479467,-56.509886262238,-40.8496544547178));
#268073=CARTESIAN_POINT('Ctrl Pts',(44.2003410646824,-56.5103214152413,
-40.8634176853611));
#268074=CARTESIAN_POINT('Ctrl Pts',(44.2109953322312,-56.5108003631786,
-40.8704389119319));
#268075=CARTESIAN_POINT('Ctrl Pts',(44.2322091102727,-56.5122711761573,
-40.8847351429132));
#268076=CARTESIAN_POINT('Ctrl Pts',(44.2639028799147,-56.5152466319394,
-40.9065696963621));
#268077=CARTESIAN_POINT('Ctrl Pts',(44.305661850593,-56.5222422564611,-40.9372114433545));
#268078=CARTESIAN_POINT('Ctrl Pts',(44.346925841944,-56.532247127269,-40.9693597045385));
#268079=CARTESIAN_POINT('Ctrl Pts',(44.3673876336497,-56.53826115526,-40.9859357593442));
#268080=CARTESIAN_POINT('Ctrl Pts',(44.3877715667723,-56.5447901720246,
-41.0027718870644));
#268081=CARTESIAN_POINT('Ctrl Pts',(44.3979208506631,-56.5483132560745,
-41.0113182564434));
#268082=CARTESIAN_POINT('Ctrl Pts',(44.4179418071922,-56.5558066378292,
-41.02850287128));
#268083=CARTESIAN_POINT('Ctrl Pts',(44.4278499085732,-56.5597882829787,
-41.0371710128992));
#268084=CARTESIAN_POINT('Ctrl Pts',(44.4572364860018,-56.5724196473794,
-41.0633712499365));
#268085=CARTESIAN_POINT('Ctrl Pts',(44.4763932211824,-56.581758968269,-41.0811111519311));
#268086=CARTESIAN_POINT('Ctrl Pts',(44.5044772880921,-56.5971447477014,
-41.1081262866225));
#268087=CARTESIAN_POINT('Ctrl Pts',(44.5137271775895,-56.6025015227711,
-41.1171962449124));
#268088=CARTESIAN_POINT('Ctrl Pts',(44.5320183562985,-56.6136863880645,
-41.1354834617267));
#268089=CARTESIAN_POINT('Ctrl Pts',(44.5410031705763,-56.6194798267371,
-41.144644186283));
#268090=CARTESIAN_POINT('Ctrl Pts',(44.5674276642847,-56.6374191091633,
-41.1721205907467));
#268091=CARTESIAN_POINT('Ctrl Pts',(44.5843870769067,-56.6501457393646,
-41.1904750382678));
#268092=CARTESIAN_POINT('Ctrl Pts',(44.616987890196,-56.6770839740703,-41.2272237610649));
#268093=CARTESIAN_POINT('Ctrl Pts',(44.640458797708,-56.6984048650555,-41.2548228473058));
#268094=CARTESIAN_POINT('Ctrl Pts',(44.6624514458289,-56.7214114906953,
-41.2824783924342));
#268095=CARTESIAN_POINT('Ctrl Pts',(44.6767798128067,-56.7371294193188,
-41.3009283158679));
#268096=CARTESIAN_POINT('Ctrl Pts',(44.683774397772,-56.7451748501741,-41.3101557240219));
#268097=CARTESIAN_POINT('Ctrl Pts',(44.6940202659092,-56.7575442973705,
-41.324018848177));
#268098=CARTESIAN_POINT('Ctrl Pts',(44.6973914635031,-56.7617145235639,
-41.328639728599));
#268099=CARTESIAN_POINT('Ctrl Pts',(44.7040131878578,-56.770108052971,-41.3378361513053));
#268100=CARTESIAN_POINT('Ctrl Pts',(44.7072703203268,-56.7743392575068,
-41.3424205878605));
#268101=CARTESIAN_POINT('Ctrl Pts',(44.7168707027477,-56.7871217033085,
-41.3561177927451));
#268102=CARTESIAN_POINT('Ctrl Pts',(44.7230524906066,-56.7957731420119,
-41.3651872799216));
#268103=CARTESIAN_POINT('Ctrl Pts',(44.7409373255192,-56.8220955492914,
-41.3921945478314));
#268104=CARTESIAN_POINT('Ctrl Pts',(44.7575187561203,-56.8491712652862,
-41.4188207502394));
#268105=CARTESIAN_POINT('Ctrl Pts',(44.7770214494108,-56.88676384976,-41.453559097464));
#268106=CARTESIAN_POINT('Ctrl Pts',(44.7858965000619,-56.9060633365117,
-41.4706740459328));
#268107=CARTESIAN_POINT('Ctrl Pts',(44.7943266372896,-56.9256180211132,
-41.4876605613939));
#268108=CARTESIAN_POINT('Ctrl Pts',(44.7983169540911,-56.9355169983302,
-41.4960845962979));
#268109=CARTESIAN_POINT('Ctrl Pts',(44.8058516078422,-56.9556000996462,
-41.5128223385875));
#268110=CARTESIAN_POINT('Ctrl Pts',(44.8093727854448,-56.9657242505397,
-41.5210856532432));
#268111=CARTESIAN_POINT('Ctrl Pts',(44.8191505788346,-56.9961959016236,
-41.5454418374945));
#268112=CARTESIAN_POINT('Ctrl Pts',(44.8246597322132,-57.0167187198372,
-41.5611704866007));
#268113=CARTESIAN_POINT('Ctrl Pts',(44.8336688220904,-57.0581479791523,
-41.5916045035181));
#268114=CARTESIAN_POINT('Ctrl Pts',(44.8389236650083,-57.0895139074259,
-41.613669368427));
#268115=CARTESIAN_POINT('Ctrl Pts',(44.8418900765893,-57.1213299669285,
-41.6345866129535));
#268116=CARTESIAN_POINT('Ctrl Pts',(44.8433488372948,-57.142640498193,-41.6482710687869));
#268117=CARTESIAN_POINT('Ctrl Pts',(44.8438191277705,-57.1533552116615,
-41.6549890353504));
#268118=CARTESIAN_POINT('Ctrl Pts',(44.8442270800594,-57.1748537940466,
-41.6681388704993));
#268119=CARTESIAN_POINT('Ctrl Pts',(44.8441639040618,-57.1855561823783,
-41.6745213422017));
#268120=CARTESIAN_POINT('Ctrl Pts',(44.8435122114514,-57.2069000331791,
-41.6869277892926));
#268121=CARTESIAN_POINT('Ctrl Pts',(44.8417458896958,-57.2388084678274,
-41.7049896680882));
#268122=CARTESIAN_POINT('Ctrl Pts',(44.8362687719071,-57.2809279665006,
-41.7269106712316));
#268123=CARTESIAN_POINT('Ctrl Pts',(44.8298088085522,-57.3121969378441,
-41.7417325167562));
#268124=CARTESIAN_POINT('Ctrl Pts',(44.8249713776488,-57.3329705079708,
-41.751249414817));
#268125=CARTESIAN_POINT('Ctrl Pts',(44.8222858794974,-57.3433254378487,
-41.7558274666229));
#268126=CARTESIAN_POINT('Ctrl Pts',(44.8163797073795,-57.3639440769784,
-41.7646063213672));
#268127=CARTESIAN_POINT('Ctrl Pts',(44.8131427147447,-57.3742522416544,
-41.7688238948253));
#268128=CARTESIAN_POINT('Ctrl Pts',(44.8061917406462,-57.3945668799698,
-41.7767918599254));
#268129=CARTESIAN_POINT('Ctrl Pts',(44.7987498536529,-57.4146412549335,
-41.7843210101159));
#268130=CARTESIAN_POINT('Ctrl Pts',(44.7861419817956,-57.4440129710611,
-41.7943060987191));
#268131=CARTESIAN_POINT('Ctrl Pts',(44.7720982599006,-57.4726583092559,
-41.8029984035242));
#268132=CARTESIAN_POINT('Ctrl Pts',(44.7566193423106,-57.5005749992605,
-41.8103989883131));
#268133=CARTESIAN_POINT('Ctrl Pts',(44.7453362941317,-57.518697088903,-41.8144666236875));
#268134=CARTESIAN_POINT('Ctrl Pts',(44.7335642473644,-57.5365709174371,
-41.8180952379985));
#268135=CARTESIAN_POINT('Ctrl Pts',(44.7274378249752,-57.5453780864623,
-41.8196891344695));
#268136=CARTESIAN_POINT('Ctrl Pts',(44.7146685840676,-57.5627610237142,
-41.8224320230444));
#268137=CARTESIAN_POINT('Ctrl Pts',(44.7080700862024,-57.5712755128024,
-41.8235709343319));
#268138=CARTESIAN_POINT('Ctrl Pts',(44.6877341610586,-57.5961705213949,
-41.8262807978491));
#268139=CARTESIAN_POINT('Ctrl Pts',(44.6734117165454,-57.6119810052107,
-41.8271650529119));
#268140=CARTESIAN_POINT('Ctrl Pts',(44.6432859415473,-57.6420285404153,
-41.827118555904));
#268141=CARTESIAN_POINT('Ctrl Pts',(44.6274777219699,-57.6562729242579,
-41.8261892556471));
#268142=CARTESIAN_POINT('Ctrl Pts',(44.6026489360012,-57.6764545436153,
-41.823427013232));
#268143=CARTESIAN_POINT('Ctrl Pts',(44.5941811636919,-57.6829873126311,
-41.8222767907821));
#268144=CARTESIAN_POINT('Ctrl Pts',(44.5812011369499,-57.6924815728277,
-41.820204446988));
#268145=CARTESIAN_POINT('Ctrl Pts',(44.5768239301145,-57.6955981764101,
-41.8194549553751));
#268146=CARTESIAN_POINT('Ctrl Pts',(44.5679795363474,-57.7017261947271,
-41.8178398084084));
#268147=CARTESIAN_POINT('Ctrl Pts',(44.554547495243,-57.7107794649358,-41.8152360293365));
#268148=CARTESIAN_POINT('Ctrl Pts',(44.5408745509057,-57.7192473537464,
-41.812140181677));
#268149=CARTESIAN_POINT('Ctrl Pts',(44.5224181841827,-57.7300417662926,
-41.8075820007456));
#268150=CARTESIAN_POINT('Ctrl Pts',(44.494403164631,-57.7454824222945,-41.8000999642091));
#268151=CARTESIAN_POINT('Ctrl Pts',(44.4557509611988,-57.7631175354143,
-41.7875858630695));
#268152=CARTESIAN_POINT('Ctrl Pts',(44.4257963579031,-57.7741479888816,
-41.7763064650726));
#268153=CARTESIAN_POINT('Ctrl Pts',(44.4056101875344,-57.781009218212,-41.7683613570464));
#268154=CARTESIAN_POINT('Ctrl Pts',(44.3954036594654,-57.7841949818065,
-41.7641737395871));
#268155=CARTESIAN_POINT('Ctrl Pts',(44.3747925009816,-57.7900627169564,
-41.7553761870634));
#268156=CARTESIAN_POINT('Ctrl Pts',(44.3643365899562,-57.7927558542442,
-41.7507422904685));
#268157=CARTESIAN_POINT('Ctrl Pts',(44.3329536886806,-57.7999988857253,
-41.7363257213199));
#268158=CARTESIAN_POINT('Ctrl Pts',(44.3014645871824,-57.8056090798854,
-41.7208580810542));
#268159=CARTESIAN_POINT('Ctrl Pts',(44.2698183189435,-57.8088603667088,
-41.7038603653999));
#268160=CARTESIAN_POINT('Ctrl Pts',(44.2381206623806,-57.8113308880715,
-41.6863549522799));
#268161=CARTESIAN_POINT('Ctrl Pts',(44.2169139506954,-57.8119384373532,
-41.6740048606234));
#268162=CARTESIAN_POINT('Ctrl Pts',(44.1850197107514,-57.811287280344,-41.6544681547659));
#268163=CARTESIAN_POINT('Ctrl Pts',(44.1743613109546,-57.8108078241776,
-41.6477783242763));
#268164=CARTESIAN_POINT('Ctrl Pts',(44.1583626375358,-57.8096935003687,
-41.6374930176863));
#268165=CARTESIAN_POINT('Ctrl Pts',(44.1530230189312,-57.809255510817,-41.6340194660765));
#268166=CARTESIAN_POINT('Ctrl Pts',(44.1423341247923,-57.8082460206643,
-41.6269840076234));
#268167=CARTESIAN_POINT('Ctrl Pts',(44.1369894952372,-57.8076746784434,
-41.6234249849254));
#268168=CARTESIAN_POINT('Ctrl Pts',(44.1103928894951,-57.8045001122898,
-41.6055088472864));
#268169=CARTESIAN_POINT('Ctrl Pts',(44.0684216046586,-57.7973782151022,
-41.5759273380954));
#268170=CARTESIAN_POINT('Ctrl Pts',(44.0275807082801,-57.78632659952,-41.5445717124501));
#268171=CARTESIAN_POINT('Ctrl Pts',(43.9872978152183,-57.7733311875938,
-41.5123297976061));
#268172=CARTESIAN_POINT('Ctrl Pts',(43.9674326520914,-57.7658590768128,
-41.4957625032292));
#268173=CARTESIAN_POINT('Ctrl Pts',(43.942963744406,-57.7552890823142,-41.4744937232973));
#268174=CARTESIAN_POINT('Ctrl Pts',(43.938085174092,-57.7531113051098,-41.4702088025761));
#268175=CARTESIAN_POINT('Ctrl Pts',(43.9283699185172,-57.7486342535987,
-41.4615871928557));
#268176=CARTESIAN_POINT('Ctrl Pts',(43.9235236029976,-57.7463299238453,
-41.4572415669043));
#268177=CARTESIAN_POINT('Ctrl Pts',(43.9090930604083,-57.739254093668,-41.4441663196977));
#268178=CARTESIAN_POINT('Ctrl Pts',(43.8996324205383,-57.7343289686206,
-41.4354132012863));
#268179=CARTESIAN_POINT('Ctrl Pts',(43.8903154257419,-57.7291941381088,
-41.4266127101804));
#268180=CARTESIAN_POINT('Ctrl Pts',(-43.4805771074156,-59.5712767529309,
-39.2399080357013));
#268181=CARTESIAN_POINT('Ctrl Pts',(-43.4478249141681,-59.5535603946867,
-39.2311075445953));
#268182=CARTESIAN_POINT('Ctrl Pts',(-43.4156056040519,-59.5351038997391,
-39.2222635806238));
#268183=CARTESIAN_POINT('Ctrl Pts',(-43.3522169440986,-59.4967328580069,
-39.2044893908274));
#268184=CARTESIAN_POINT('Ctrl Pts',(-43.3210476458595,-59.4768182391239,
-39.1955591618115));
#268185=CARTESIAN_POINT('Ctrl Pts',(-43.2291022595543,-59.4149049130521,
-39.1686393287622));
#268186=CARTESIAN_POINT('Ctrl Pts',(-43.1698853587931,-59.3707413041733,
-39.1505208045068));
#268187=CARTESIAN_POINT('Ctrl Pts',(-43.0556331620037,-59.2766097614945,
-39.113935063243));
#268188=CARTESIAN_POINT('Ctrl Pts',(-43.0005921597408,-59.2266373021163,
-39.0954660506179));
#268189=CARTESIAN_POINT('Ctrl Pts',(-42.8948534568781,-59.1207134074407,
-39.0581733199915));
#268190=CARTESIAN_POINT('Ctrl Pts',(-42.8449960553599,-59.0656056508999,
-39.0396463059707));
#268191=CARTESIAN_POINT('Ctrl Pts',(-42.7510811208719,-58.9512122276158,
-39.0028139665663));
#268192=CARTESIAN_POINT('Ctrl Pts',(-42.7070288152267,-58.891930638621,
-38.9845102727346));
#268193=CARTESIAN_POINT('Ctrl Pts',(-42.6452866349949,-58.7998958734659,
-38.957224077988));
#268194=CARTESIAN_POINT('Ctrl Pts',(-42.625429767352,-58.7686980621887,
-38.9481569597938));
#268195=CARTESIAN_POINT('Ctrl Pts',(-42.5871756130002,-58.7052546833099,
-38.9300801552924));
#268196=CARTESIAN_POINT('Ctrl Pts',(-42.568778253032,-58.6730091686672,
-38.9210704649552));
#268197=CARTESIAN_POINT('Ctrl Pts',(-42.5334651880811,-58.6074543754265,
-38.9031098981675));
#268198=CARTESIAN_POINT('Ctrl Pts',(-42.5165536369311,-58.5741539171446,
-38.8941613358138));
#268199=CARTESIAN_POINT('Ctrl Pts',(-42.4842288567228,-58.5064298632496,
-38.8763157156907));
#268200=CARTESIAN_POINT('Ctrl Pts',(-42.4689425396028,-58.4722695523732,
-38.8674882509199));
#268201=CARTESIAN_POINT('Ctrl Pts',(-42.4401223815193,-58.4034275140121,
-38.8500385014136));
#268202=CARTESIAN_POINT('Ctrl Pts',(-42.426583050894,-58.3687341967778,
-38.8414131698514));
#268203=CARTESIAN_POINT('Ctrl Pts',(-42.4012287918448,-58.2988104271035,
-38.824360868638));
#268204=CARTESIAN_POINT('Ctrl Pts',(-42.3894137611201,-58.2635796188005,
-38.8159338161007));
#268205=CARTESIAN_POINT('Ctrl Pts',(-42.3565461207186,-58.1570828582558,
-38.7909502725479));
#268206=CARTESIAN_POINT('Ctrl Pts',(-42.3380647902547,-58.0850119200903,
-38.7746901633276));
#268207=CARTESIAN_POINT('Ctrl Pts',(-42.3155659796374,-57.9752818499468,
-38.7509105250088));
#268208=CARTESIAN_POINT('Ctrl Pts',(-42.3089374211558,-57.9384266221928,
-38.7430843922672));
#268209=CARTESIAN_POINT('Ctrl Pts',(-42.297458012674,-57.864178756387,-38.7276438637217));
#268210=CARTESIAN_POINT('Ctrl Pts',(-42.292601515188,-57.8267325312259,
-38.720018782004));
#268211=CARTESIAN_POINT('Ctrl Pts',(-42.2847289916893,-57.7514526301959,
-38.7050196673962));
#268212=CARTESIAN_POINT('Ctrl Pts',(-42.2817363521424,-57.7138759968928,
-38.6976962453237));
#268213=CARTESIAN_POINT('Ctrl Pts',(-42.277596992864,-57.6387184974263,
-38.6833720377019));
#268214=CARTESIAN_POINT('Ctrl Pts',(-42.2764525301716,-57.6011593077097,
-38.6763755686054));
#268215=CARTESIAN_POINT('Ctrl Pts',(-42.2757726188108,-57.4885396176673,
-38.6558809641879));
#268216=CARTESIAN_POINT('Ctrl Pts',(-42.2789845428693,-57.4135368708757,
-38.6428765167438));
#268217=CARTESIAN_POINT('Ctrl Pts',(-42.289333314243,-57.3011476810195,
-38.6243712990017));
#268218=CARTESIAN_POINT('Ctrl Pts',(-42.2937061680812,-57.2637038035873,
-38.618370061439));
#268219=CARTESIAN_POINT('Ctrl Pts',(-42.3043247017591,-57.1888547452426,
-38.6067079534822));
#268220=CARTESIAN_POINT('Ctrl Pts',(-42.3105743117123,-57.1514345461221,
-38.6010450635964));
#268221=CARTESIAN_POINT('Ctrl Pts',(-42.3249704170347,-57.0766935209606,
-38.590076215021));
#268222=CARTESIAN_POINT('Ctrl Pts',(-42.3331592025312,-57.0392159768686,
-38.5847494243559));
#268223=CARTESIAN_POINT('Ctrl Pts',(-42.3512949844302,-56.9651221381903,
-38.5745673038812));
#268224=CARTESIAN_POINT('Ctrl Pts',(-42.3612586135401,-56.9283882021117,
-38.5696936317377));
#268225=CARTESIAN_POINT('Ctrl Pts',(-42.3829467968515,-56.8555905655333,
-38.5603848033813));
#268226=CARTESIAN_POINT('Ctrl Pts',(-42.3946724551093,-56.8195179901625,
-38.555948235663));
#268227=CARTESIAN_POINT('Ctrl Pts',(-42.4198760714445,-56.7480212016901,
-38.5475092141337));
#268228=CARTESIAN_POINT('Ctrl Pts',(-42.4333540386586,-56.712596992043,
-38.5435067618884));
#268229=CARTESIAN_POINT('Ctrl Pts',(-42.4620643651744,-56.6423976051736,
-38.5359375083953));
#268230=CARTESIAN_POINT('Ctrl Pts',(-42.4772967069948,-56.6076224215361,
-38.5323707022785));
#268231=CARTESIAN_POINT('Ctrl Pts',(-42.5095308031841,-56.5387265502116,
-38.5256774075877));
#268232=CARTESIAN_POINT('Ctrl Pts',(-42.5265325119253,-56.5046058456765,
-38.5225509073062));
#268233=CARTESIAN_POINT('Ctrl Pts',(-42.5623338475307,-56.4370293947696,
-38.5167461666044));
#268234=CARTESIAN_POINT('Ctrl Pts',(-42.5811223641794,-56.4035923099625,
-38.5140693065785));
#268235=CARTESIAN_POINT('Ctrl Pts',(-42.620584523009,-56.3373241998654,
-38.5091697400817));
#268236=CARTESIAN_POINT('Ctrl Pts',(-42.6411082254821,-56.3047465904101,
-38.5069659500128));
#268237=CARTESIAN_POINT('Ctrl Pts',(-42.7048067991197,-56.2090283357163,
-38.5011108589349));
#268238=CARTESIAN_POINT('Ctrl Pts',(-42.7502234543428,-56.1476408662828,
-38.4981890389281));
#268239=CARTESIAN_POINT('Ctrl Pts',(-42.846794232383,-56.0297655581676,
-38.4942910511032));
#268240=CARTESIAN_POINT('Ctrl Pts',(-42.8979715413934,-55.9732420482177,
-38.4933125989996));
#268241=CARTESIAN_POINT('Ctrl Pts',(-42.9790570553346,-55.8921695883032,
-38.4933149859728));
#268242=CARTESIAN_POINT('Ctrl Pts',(-43.0068374106561,-55.8657400908869,
-38.4935622007431));
#268243=CARTESIAN_POINT('Ctrl Pts',(-43.0495800649421,-55.8270637749536,
-38.4943063068789));
#268244=CARTESIAN_POINT('Ctrl Pts',(-43.0640222060113,-55.8143203511958,
-38.494617152342));
#268245=CARTESIAN_POINT('Ctrl Pts',(-43.0932714774893,-55.7891564261061,
-38.4953646906773));
#268246=CARTESIAN_POINT('Ctrl Pts',(-43.1080901283633,-55.7767277938553,
-38.4958020036096));
#268247=CARTESIAN_POINT('Ctrl Pts',(-43.1528523310046,-55.7401327167866,
-38.4972962980169));
#268248=CARTESIAN_POINT('Ctrl Pts',(-43.183171240984,-55.7165901373356,
-38.498536032863));
#268249=CARTESIAN_POINT('Ctrl Pts',(-43.2447583556422,-55.6711691509155,
-38.5014931332815));
#268250=CARTESIAN_POINT('Ctrl Pts',(-43.2760240909102,-55.6492920896315,
-38.5032102926999));
#268251=CARTESIAN_POINT('Ctrl Pts',(-43.37121764534,-55.5861255243223,-38.5090666584048));
#268252=CARTESIAN_POINT('Ctrl Pts',(-43.4365388292261,-55.5472953809443,
-38.5139093068404));
#268253=CARTESIAN_POINT('Ctrl Pts',(-43.5372923455653,-55.4939420631336,
-38.5225684468354));
#268254=CARTESIAN_POINT('Ctrl Pts',(-43.5713395927683,-55.4769743237494,
-38.5256877381308));
#268255=CARTESIAN_POINT('Ctrl Pts',(-43.6403672861995,-55.4446857735354,
-38.5323951500278));
#268256=CARTESIAN_POINT('Ctrl Pts',(-43.6753577685123,-55.4293620157832,
-38.5359845633874));
#268257=CARTESIAN_POINT('Ctrl Pts',(-43.7462462065787,-55.4003985583156,
-38.5436333065981));
#268258=CARTESIAN_POINT('Ctrl Pts',(-43.7822717759725,-55.3867204456352,
-38.5477088862383));
#268259=CARTESIAN_POINT('Ctrl Pts',(-43.8543821738219,-55.3613797848081,
-38.5562346427693));
#268260=CARTESIAN_POINT('Ctrl Pts',(-43.890622407919,-55.349649082917,-38.5607007444526));
#268261=CARTESIAN_POINT('Ctrl Pts',(-43.9633781832422,-55.3280633380684,
-38.5700204086244));
#268262=CARTESIAN_POINT('Ctrl Pts',(-43.9999084022592,-55.3182019076378,
-38.5748754846743));
#268263=CARTESIAN_POINT('Ctrl Pts',(-44.0732691651704,-55.300314394282,
-38.5849692074244));
#268264=CARTESIAN_POINT('Ctrl Pts',(-44.1100997159262,-55.2922883538608,
-38.590207863671));
#268265=CARTESIAN_POINT('Ctrl Pts',(-44.1840590812038,-55.2780579645929,
-38.6010647047639));
#268266=CARTESIAN_POINT('Ctrl Pts',(-44.2211878979616,-55.2718536300564,
-38.6066828933265));
#268267=CARTESIAN_POINT('Ctrl Pts',(-44.2957439071301,-55.2612662316006,
-38.6182974837333));
#268268=CARTESIAN_POINT('Ctrl Pts',(-44.3331710973477,-55.256883155031,
-38.624293883757));
#268269=CARTESIAN_POINT('Ctrl Pts',(-44.4083261383181,-55.2499510742625,
-38.6366662922177));
#268270=CARTESIAN_POINT('Ctrl Pts',(-44.446056048267,-55.2474029004138,
-38.6430428201589));
#268271=CARTESIAN_POINT('Ctrl Pts',(-44.5218128020516,-55.2441636366351,
-38.6561775645199));
#268272=CARTESIAN_POINT('Ctrl Pts',(-44.5599089424743,-55.2434808562086,
-38.6629497802385));
#268273=CARTESIAN_POINT('Ctrl Pts',(-44.6354869543582,-55.2439911084578,
-38.6767130108817));
#268274=CARTESIAN_POINT('Ctrl Pts',(-44.6731456892459,-55.2451740103824,
-38.6837342374529));
#268275=CARTESIAN_POINT('Ctrl Pts',(-44.7481014788608,-55.2493620066237,
-38.6980304684339));
#268276=CARTESIAN_POINT('Ctrl Pts',(-44.7854165850557,-55.2523662274994,
-38.7053085862828));
#268277=CARTESIAN_POINT('Ctrl Pts',(-44.8968808056053,-55.2640710758905,
-38.7275256543264));
#268278=CARTESIAN_POINT('Ctrl Pts',(-44.9705498158105,-55.2754583368831,
-38.7428465194087));
#268279=CARTESIAN_POINT('Ctrl Pts',(-45.0801001998238,-55.2978810544009,
-38.7665804202115));
#268280=CARTESIAN_POINT('Ctrl Pts',(-45.1164578754129,-55.3062470656085,
-38.7746173707339));
#268281=CARTESIAN_POINT('Ctrl Pts',(-45.1888527653151,-55.3247763762561,
-38.790943453482));
#268282=CARTESIAN_POINT('Ctrl Pts',(-45.2248832056965,-55.3349380951144,
-38.7992310848652));
#268283=CARTESIAN_POINT('Ctrl Pts',(-45.2966462681613,-55.3570913336823,
-38.8160672125853));
#268284=CARTESIAN_POINT('Ctrl Pts',(-45.3323638946335,-55.3690863290504,
-38.8246135819642));
#268285=CARTESIAN_POINT('Ctrl Pts',(-45.4027951436545,-55.3946744461232,
-38.841798196801));
#268286=CARTESIAN_POINT('Ctrl Pts',(-45.4376370321487,-55.4083060218429,
-38.85046633842));
#268287=CARTESIAN_POINT('Ctrl Pts',(-45.506502018173,-55.4372015589607,
-38.8679331631116));
#268288=CARTESIAN_POINT('Ctrl Pts',(-45.5405385021803,-55.4524695986684,
-38.8767349781349));
#268289=CARTESIAN_POINT('Ctrl Pts',(-45.6078227545416,-55.4846397884912,
-38.894474157443));
#268290=CARTESIAN_POINT('Ctrl Pts',(-45.6410705220074,-55.5015419401624,
-38.903411522349));
#268291=CARTESIAN_POINT('Ctrl Pts',(-45.6739227548726,-55.5192637629152,
-38.9124165672463));
#268292=CARTESIAN_POINT('Ctrl Pts',(-43.5555682511181,-59.2341350312479,
-39.6401231904583));
#268293=CARTESIAN_POINT('Ctrl Pts',(-43.5271052157456,-59.2187213699007,
-39.6313226993523));
#268294=CARTESIAN_POINT('Ctrl Pts',(-43.4991046027441,-59.2026650473832,
-39.6224787353808));
#268295=CARTESIAN_POINT('Ctrl Pts',(-43.4440144956751,-59.1692863795892,
-39.6047045455842));
#268296=CARTESIAN_POINT('Ctrl Pts',(-43.416925046393,-59.151963971707,-39.5957743165685));
#268297=CARTESIAN_POINT('Ctrl Pts',(-43.3370125740194,-59.0981130112185,
-39.5688544835192));
#268298=CARTESIAN_POINT('Ctrl Pts',(-43.2855425446096,-59.0597046874419,
-39.5507359592637));
#268299=CARTESIAN_POINT('Ctrl Pts',(-43.1862310165518,-58.9778482320248,
-39.5141502180001));
#268300=CARTESIAN_POINT('Ctrl Pts',(-43.1383845581245,-58.9343961646677,
-39.4956812053746));
#268301=CARTESIAN_POINT('Ctrl Pts',(-43.0464604338337,-58.8423006638519,
-39.4583884747487));
#268302=CARTESIAN_POINT('Ctrl Pts',(-43.0031132840443,-58.7943907659202,
-39.4398614607275));
#268303=CARTESIAN_POINT('Ctrl Pts',(-42.9214542034191,-58.69494537932,-39.4030291213234));
#268304=CARTESIAN_POINT('Ctrl Pts',(-42.8831468162938,-58.6434134367091,
-39.3847254274915));
#268305=CARTESIAN_POINT('Ctrl Pts',(-42.8294502801417,-58.563414667145,
-39.357439232745));
#268306=CARTESIAN_POINT('Ctrl Pts',(-42.8121798538915,-58.536297551274,
-39.3483721145507));
#268307=CARTESIAN_POINT('Ctrl Pts',(-42.7789061306717,-58.4811541100691,
-39.3302953100494));
#268308=CARTESIAN_POINT('Ctrl Pts',(-42.7629027701056,-58.4531278306783,
-39.3212856197121));
#268309=CARTESIAN_POINT('Ctrl Pts',(-42.732182334752,-58.396152181943,-39.3033250529244));
#268310=CARTESIAN_POINT('Ctrl Pts',(-42.7174688743488,-58.3672104781721,
-39.2943764905707));
#268311=CARTESIAN_POINT('Ctrl Pts',(-42.6893426693184,-58.308352422918,
-39.2765308704477));
#268312=CARTESIAN_POINT('Ctrl Pts',(-42.676040350531,-58.2786648895678,
-39.2677034056768));
#268313=CARTESIAN_POINT('Ctrl Pts',(-42.6509576148479,-58.2188381095861,
-39.2502536561705));
#268314=CARTESIAN_POINT('Ctrl Pts',(-42.6391724212676,-58.1886887904878,
-39.2416283246084));
#268315=CARTESIAN_POINT('Ctrl Pts',(-42.6170995346736,-58.12792477379,-39.224576023395));
#268316=CARTESIAN_POINT('Ctrl Pts',(-42.6068117525533,-58.0973097669517,
-39.2161489708576));
#268317=CARTESIAN_POINT('Ctrl Pts',(-42.578186703978,-58.0047678749905,
-39.1911654273048));
#268318=CARTESIAN_POINT('Ctrl Pts',(-42.5620823726479,-57.9421435490173,
-39.1749053180845));
#268319=CARTESIAN_POINT('Ctrl Pts',(-42.5424617625838,-57.8468004016288,
-39.1511256797658));
#268320=CARTESIAN_POINT('Ctrl Pts',(-42.5366779815724,-57.8147780230883,
-39.1432995470242));
#268321=CARTESIAN_POINT('Ctrl Pts',(-42.5266542176424,-57.7502677264705,
-39.1278590184786));
#268322=CARTESIAN_POINT('Ctrl Pts',(-42.5224092913251,-57.7177332511804,
-39.120233936761));
#268323=CARTESIAN_POINT('Ctrl Pts',(-42.5155178619726,-57.6523290916439,
-39.1052348221532));
#268324=CARTESIAN_POINT('Ctrl Pts',(-42.5128918544921,-57.6196827267464,
-39.0979114000806));
#268325=CARTESIAN_POINT('Ctrl Pts',(-42.5092432682604,-57.5543877143394,
-39.0835871924589));
#268326=CARTESIAN_POINT('Ctrl Pts',(-42.5082226653386,-57.5217578995943,
-39.0765907233623));
#268327=CARTESIAN_POINT('Ctrl Pts',(-42.5075526709299,-57.4239208272887,
-39.0560961189448));
#268328=CARTESIAN_POINT('Ctrl Pts',(-42.5102897909719,-57.3587658283315,
-39.0430916715008));
#268329=CARTESIAN_POINT('Ctrl Pts',(-42.5191999190634,-57.2611374049919,
-39.0245864537587));
#268330=CARTESIAN_POINT('Ctrl Pts',(-42.5229719620357,-57.2286119708033,
-39.018585216196));
#268331=CARTESIAN_POINT('Ctrl Pts',(-42.5321429006105,-57.1635961556059,
-39.0069231082391));
#268332=CARTESIAN_POINT('Ctrl Pts',(-42.5375451994904,-57.131092730784,
-39.0012602183534));
#268333=CARTESIAN_POINT('Ctrl Pts',(-42.5499976000816,-57.0661736672035,
-38.990291369778));
#268334=CARTESIAN_POINT('Ctrl Pts',(-42.5570843265014,-57.0336219145328,
-38.9849645791129));
#268335=CARTESIAN_POINT('Ctrl Pts',(-42.5727856698931,-56.9692679586228,
-38.9747824586382));
#268336=CARTESIAN_POINT('Ctrl Pts',(-42.5814146517845,-56.9373635689111,
-38.9699087864947));
#268337=CARTESIAN_POINT('Ctrl Pts',(-42.6002027387397,-56.8741384006643,
-38.9605999581383));
#268338=CARTESIAN_POINT('Ctrl Pts',(-42.6103627965689,-56.8428099130675,
-38.9561633904199));
#268339=CARTESIAN_POINT('Ctrl Pts',(-42.6322055381297,-56.7807175391602,
-38.9477243688907));
#268340=CARTESIAN_POINT('Ctrl Pts',(-42.643888229794,-56.7499536558588,
-38.9437219166454));
#268341=CARTESIAN_POINT('Ctrl Pts',(-42.6687780682593,-56.6889910719312,
-38.9361526631524));
#268342=CARTESIAN_POINT('Ctrl Pts',(-42.6819851998625,-56.6587923657221,
-38.9325858570355));
#268343=CARTESIAN_POINT('Ctrl Pts',(-42.7099369818181,-56.5989648901808,
-38.9258925623447));
#268344=CARTESIAN_POINT('Ctrl Pts',(-42.7246815925139,-56.5693361061833,
-38.9227660620632));
#268345=CARTESIAN_POINT('Ctrl Pts',(-42.7557331147216,-56.5106575807864,
-38.9169613213614));
#268346=CARTESIAN_POINT('Ctrl Pts',(-42.7720303883604,-56.4816240428195,
-38.9142844613354));
#268347=CARTESIAN_POINT('Ctrl Pts',(-42.8062629627728,-56.4240849025666,
-38.9093848948388));
#268348=CARTESIAN_POINT('Ctrl Pts',(-42.8240681953201,-56.3957993363617,
-38.9071811047699));
#268349=CARTESIAN_POINT('Ctrl Pts',(-42.8793334746424,-56.3126943660298,
-38.9013260136915));
#268350=CARTESIAN_POINT('Ctrl Pts',(-42.9187422214293,-56.2593996931541,
-38.8984041936851));
#268351=CARTESIAN_POINT('Ctrl Pts',(-43.0025474813891,-56.1570710705974,
-38.8945062058602));
#268352=CARTESIAN_POINT('Ctrl Pts',(-43.0469641103745,-56.1080061498824,
-38.8935277537565));
#268353=CARTESIAN_POINT('Ctrl Pts',(-43.117344267243,-56.0376373429099,
-38.8935301407298));
#268354=CARTESIAN_POINT('Ctrl Pts',(-43.1414579047527,-56.0146982180904,
-38.8937773555002));
#268355=CARTESIAN_POINT('Ctrl Pts',(-43.1785604553322,-55.9811311728431,
-38.8945214616358));
#268356=CARTESIAN_POINT('Ctrl Pts',(-43.191097126858,-55.9700714625021,
-38.894832307099));
#268357=CARTESIAN_POINT('Ctrl Pts',(-43.2164877853448,-55.9482328356115,
-38.8955798454342));
#268358=CARTESIAN_POINT('Ctrl Pts',(-43.2293517743068,-55.9374468641231,
-38.8960171583666));
#268359=CARTESIAN_POINT('Ctrl Pts',(-43.2682103054482,-55.9056892935197,
-38.8975114527738));
#268360=CARTESIAN_POINT('Ctrl Pts',(-43.2945313976451,-55.8852599252372,
-38.89875118762));
#268361=CARTESIAN_POINT('Ctrl Pts',(-43.3479995130708,-55.8458475490097,
-38.9017082880385));
#268362=CARTESIAN_POINT('Ctrl Pts',(-43.3751443920601,-55.8268657082684,
-38.9034254474569));
#268363=CARTESIAN_POINT('Ctrl Pts',(-43.4577939430348,-55.7720622018028,
-38.9092818131617));
#268364=CARTESIAN_POINT('Ctrl Pts',(-43.51451093327,-55.7383779822391,-38.9141244615973));
#268365=CARTESIAN_POINT('Ctrl Pts',(-43.601998052992,-55.6921031576597,
-38.9227836015924));
#268366=CARTESIAN_POINT('Ctrl Pts',(-43.631563048157,-55.6773880028564,
-38.9259028928878));
#268367=CARTESIAN_POINT('Ctrl Pts',(-43.6915050002909,-55.6493890121587,
-38.9326103047848));
#268368=CARTESIAN_POINT('Ctrl Pts',(-43.7218906736911,-55.6361026235129,
-38.9361997181443));
#268369=CARTESIAN_POINT('Ctrl Pts',(-43.783451665776,-55.6109933882688,
-38.9438484613551));
#268370=CARTESIAN_POINT('Ctrl Pts',(-43.8147378173409,-55.5991372642861,
-38.9479240409953));
#268371=CARTESIAN_POINT('Ctrl Pts',(-43.877363149692,-55.5771759127617,
-38.9564497975263));
#268372=CARTESIAN_POINT('Ctrl Pts',(-43.9088372843841,-55.5670115927043,
-38.9609158992096));
#268373=CARTESIAN_POINT('Ctrl Pts',(-43.9720261650696,-55.5483124604321,
-38.9702355633813));
#268374=CARTESIAN_POINT('Ctrl Pts',(-44.0037536572564,-55.5397721100658,
-38.9750906394313));
#268375=CARTESIAN_POINT('Ctrl Pts',(-44.0674709555852,-55.5242859080953,
-38.9851843621813));
#268376=CARTESIAN_POINT('Ctrl Pts',(-44.0994607677182,-55.5173400934252,
-38.9904230184279));
#268377=CARTESIAN_POINT('Ctrl Pts',(-44.1637009035284,-55.5050310901567,
-39.0012798595209));
#268378=CARTESIAN_POINT('Ctrl Pts',(-44.1959512291589,-55.4996679139965,
-39.0068980480835));
#268379=CARTESIAN_POINT('Ctrl Pts',(-44.2607124863074,-55.4905238141391,
-39.0185126384903));
#268380=CARTESIAN_POINT('Ctrl Pts',(-44.2932234159127,-55.4867428794561,
-39.0245090385139));
#268381=CARTESIAN_POINT('Ctrl Pts',(-44.3585078720818,-55.480774377281,
-39.0368814469747));
#268382=CARTESIAN_POINT('Ctrl Pts',(-44.3912831881742,-55.4785875325166,
-39.0432579749157));
#268383=CARTESIAN_POINT('Ctrl Pts',(-44.4570931925988,-55.4758271902798,
-39.0563927192769));
#268384=CARTESIAN_POINT('Ctrl Pts',(-44.4901880875464,-55.47526095961,-39.0631649349955));
#268385=CARTESIAN_POINT('Ctrl Pts',(-44.5558456650652,-55.4757574670419,
-39.0769281656387));
#268386=CARTESIAN_POINT('Ctrl Pts',(-44.5885619871977,-55.4768115298703,
-39.0839493922098));
#268387=CARTESIAN_POINT('Ctrl Pts',(-44.6536818041136,-55.4805022216823,
-39.0982456231909));
#268388=CARTESIAN_POINT('Ctrl Pts',(-44.6861009801573,-55.4831381046999,
-39.1055237410398));
#268389=CARTESIAN_POINT('Ctrl Pts',(-44.782942584543,-55.4933839391136,
-39.1277408090834));
#268390=CARTESIAN_POINT('Ctrl Pts',(-44.8469499487504,-55.5033272531759,
-39.1430616741657));
#268391=CARTESIAN_POINT('Ctrl Pts',(-44.9421369398694,-55.5228816395291,
-39.1667955749684));
#268392=CARTESIAN_POINT('Ctrl Pts',(-44.9737283661904,-55.5301742790311,
-39.1748325254908));
#268393=CARTESIAN_POINT('Ctrl Pts',(-45.0366341467681,-55.5463205175099,
-39.1911586082389));
#268394=CARTESIAN_POINT('Ctrl Pts',(-45.0679426151012,-55.5551727387585,
-39.1994462396222));
#268395=CARTESIAN_POINT('Ctrl Pts',(-45.1303021643981,-55.5744664003474,
-39.2162823673423));
#268396=CARTESIAN_POINT('Ctrl Pts',(-45.1613402206007,-55.5849108492065,
-39.2248287367212));
#268397=CARTESIAN_POINT('Ctrl Pts',(-45.2225452749523,-55.6071872308721,
-39.242013351558));
#268398=CARTESIAN_POINT('Ctrl Pts',(-45.2528237308145,-55.6190526565937,
-39.250681493177));
#268399=CARTESIAN_POINT('Ctrl Pts',(-45.312670500747,-55.6442008855743,
-39.2681483178686));
#268400=CARTESIAN_POINT('Ctrl Pts',(-45.342250447157,-55.6574872408305,
-39.276950132892));
#268401=CARTESIAN_POINT('Ctrl Pts',(-45.4007263164517,-55.6854788533848,
-39.2946893121999));
#268402=CARTESIAN_POINT('Ctrl Pts',(-45.429622238573,-55.700184112031,-39.303626677106));
#268403=CARTESIAN_POINT('Ctrl Pts',(-45.4581751231196,-55.7156010961856,
-39.3126317220034));
#268404=CARTESIAN_POINT('Ctrl Pts',(-44.2366247954661,-55.49394262042,-39.0141963249616));
#268405=CARTESIAN_POINT('Ctrl Pts',(-44.2662621726756,-55.4898840014969,
-39.0195373795186));
#268406=CARTESIAN_POINT('Ctrl Pts',(-44.3285305334225,-55.4827749995086,
-39.031049367808));
#268407=CARTESIAN_POINT('Ctrl Pts',(-44.3912831881742,-55.4785875325166,
-39.0432579749157));
#268408=CARTESIAN_POINT('Ctrl Pts',(-44.4570931925989,-55.4758271902798,
-39.0563927192769));
#268409=CARTESIAN_POINT('Ctrl Pts',(-44.4901880875464,-55.47526095961,-39.0631649349955));
#268410=CARTESIAN_POINT('Ctrl Pts',(-44.5558456650653,-55.4757574670419,
-39.0769281656387));
#268411=CARTESIAN_POINT('Ctrl Pts',(-44.5885619871977,-55.4768115298702,
-39.0839493922098));
#268412=CARTESIAN_POINT('Ctrl Pts',(-44.6536818041136,-55.4805022216824,
-39.0982456231909));
#268413=CARTESIAN_POINT('Ctrl Pts',(-44.750939117342,-55.4884110764087,
-39.1200801766399));
#268414=CARTESIAN_POINT('Ctrl Pts',(-44.8789538232237,-55.5082978363117,
-39.1507219236323));
#268415=CARTESIAN_POINT('Ctrl Pts',(-45.0053227794738,-55.5374673614327,
-39.1828701848163));
#268416=CARTESIAN_POINT('Ctrl Pts',(-45.0679426151012,-55.5551727387585,
-39.1994462396222));
#268417=CARTESIAN_POINT('Ctrl Pts',(-45.1303021643981,-55.5744664003474,
-39.2162823673423));
#268418=CARTESIAN_POINT('Ctrl Pts',(-45.1613402206007,-55.5849108492065,
-39.2248287367212));
#268419=CARTESIAN_POINT('Ctrl Pts',(-45.2225452749523,-55.6071872308721,
-39.2420133515579));
#268420=CARTESIAN_POINT('Ctrl Pts',(-45.2528237308145,-55.6190526565937,
-39.250681493177));
#268421=CARTESIAN_POINT('Ctrl Pts',(-45.3425938857133,-55.6567750000645,
-39.2768817302143));
#268422=CARTESIAN_POINT('Ctrl Pts',(-45.4010693540256,-55.684767127876,
-39.2946216322085));
#268423=CARTESIAN_POINT('Ctrl Pts',(-45.4581751231188,-55.7156010961851,
-39.3126317220031));
#268424=CARTESIAN_POINT('Ctrl Pts',(-43.5555682511181,-59.2341350312479,
-39.6401231904583));
#268425=CARTESIAN_POINT('Ctrl Pts',(-43.4986421803732,-59.2033077085535,
-39.6225222082463));
#268426=CARTESIAN_POINT('Ctrl Pts',(-43.3884827487122,-59.1365211050906,
-39.5869729940158));
#268427=CARTESIAN_POINT('Ctrl Pts',(-43.2340749587687,-59.0212983889997,
-39.5326183362566));
#268428=CARTESIAN_POINT('Ctrl Pts',(-43.1383845581245,-58.9343961646677,
-39.4956812053746));
#268429=CARTESIAN_POINT('Ctrl Pts',(-43.0464604338337,-58.8423006638519,
-39.4583884747486));
#268430=CARTESIAN_POINT('Ctrl Pts',(-42.9597638623997,-58.7464790949597,
-39.4213336309308));
#268431=CARTESIAN_POINT('Ctrl Pts',(-42.8639918437047,-58.6176479605167,
-39.3755734228827));
#268432=CARTESIAN_POINT('Ctrl Pts',(-42.7949093409291,-58.5091805688265,
-39.33930500608));
#268433=CARTESIAN_POINT('Ctrl Pts',(-42.7468976399245,-58.4250976736591,
-39.3122747709031));
#268434=CARTESIAN_POINT('Ctrl Pts',(-42.7174688743488,-58.3672104781721,
-39.2943764905707));
#268435=CARTESIAN_POINT('Ctrl Pts',(-42.6893426693184,-58.308352422918,
-39.2765308704476));
#268436=CARTESIAN_POINT('Ctrl Pts',(-42.676040350531,-58.2786648895678,
-39.2677034056768));
#268437=CARTESIAN_POINT('Ctrl Pts',(-42.6394421976857,-58.1913717942018,
-39.242242522637));
#268438=CARTESIAN_POINT('Ctrl Pts',(-42.6181634379433,-58.1331272500595,
-39.225872582076));
#268439=CARTESIAN_POINT('Ctrl Pts',(-42.5996267543263,-58.074028296276,
-39.2098669458287));
#268440=CARTESIAN_POINT('Ctrl Pts',(-43.4805771074156,-59.5712767529309,
-39.2399080357013));
#268441=CARTESIAN_POINT('Ctrl Pts',(-43.4150727209207,-59.5358440364426,
-39.2223070534893));
#268442=CARTESIAN_POINT('Ctrl Pts',(-43.2883193276586,-59.4590682572254,
-39.1867578392588));
#268443=CARTESIAN_POINT('Ctrl Pts',(-43.1106712693135,-59.32658002426,-39.1324031814995));
#268444=CARTESIAN_POINT('Ctrl Pts',(-43.0005921597408,-59.2266373021163,
-39.0954660506179));
#268445=CARTESIAN_POINT('Ctrl Pts',(-42.8948534568781,-59.1207134074407,
-39.0581733199915));
#268446=CARTESIAN_POINT('Ctrl Pts',(-42.7951360401793,-59.0104958554849,
-39.0211184761739));
#268447=CARTESIAN_POINT('Ctrl Pts',(-42.6850011896347,-58.8622904152127,
-38.9753582681256));
#268448=CARTESIAN_POINT('Ctrl Pts',(-42.6055727997797,-58.7375004045667,
-38.939089851323));
#268449=CARTESIAN_POINT('Ctrl Pts',(-42.5503788594446,-58.6407591922129,
-38.9120596161462));
#268450=CARTESIAN_POINT('Ctrl Pts',(-42.5165536369311,-58.5741539171446,
-38.8941613358138));
#268451=CARTESIAN_POINT('Ctrl Pts',(-42.4842288567228,-58.5064298632496,
-38.8763157156907));
#268452=CARTESIAN_POINT('Ctrl Pts',(-42.4689425396028,-58.4722695523732,
-38.8674882509199));
#268453=CARTESIAN_POINT('Ctrl Pts',(-42.4257123024776,-58.3690064948315,
-38.8413136266604));
#268454=CARTESIAN_POINT('Ctrl Pts',(-42.3750272156063,-58.229152189777,
-38.8072100415055));
#268455=CARTESIAN_POINT('Ctrl Pts',(-42.3380647902547,-58.0850119200902,
-38.7746901633276));
#268456=CARTESIAN_POINT('Ctrl Pts',(-42.3155659796374,-57.9752818499468,
-38.7509105250088));
#268457=CARTESIAN_POINT('Ctrl Pts',(-42.3089374211558,-57.9384266221928,
-38.7430843922672));
#268458=CARTESIAN_POINT('Ctrl Pts',(-42.297458012674,-57.864178756387,-38.7276438637217));
#268459=CARTESIAN_POINT('Ctrl Pts',(-42.292601515188,-57.8267325312259,
-38.720018782004));
#268460=CARTESIAN_POINT('Ctrl Pts',(-42.2847289916893,-57.7514526301959,
-38.7050196673963));
#268461=CARTESIAN_POINT('Ctrl Pts',(-42.2817363521424,-57.7138759968928,
-38.6976962453237));
#268462=CARTESIAN_POINT('Ctrl Pts',(-42.277596992864,-57.6387184974263,
-38.6833720377019));
#268463=CARTESIAN_POINT('Ctrl Pts',(-42.2741651307842,-57.5260409596698,
-38.6623829091612));
#268464=CARTESIAN_POINT('Ctrl Pts',(-42.2805893100654,-57.3760354719141,
-38.6363740800325));
#268465=CARTESIAN_POINT('Ctrl Pts',(-42.2937061680812,-57.2637038035873,
-38.618370061439));
#268466=CARTESIAN_POINT('Ctrl Pts',(-42.3043247017591,-57.1888547452426,
-38.6067079534822));
#268467=CARTESIAN_POINT('Ctrl Pts',(-42.3105743117123,-57.1514345461221,
-38.6010450635964));
#268468=CARTESIAN_POINT('Ctrl Pts',(-42.3249704170347,-57.0766935209607,
-38.590076215021));
#268469=CARTESIAN_POINT('Ctrl Pts',(-42.3331592025312,-57.0392159768686,
-38.5847494243559));
#268470=CARTESIAN_POINT('Ctrl Pts',(-42.3512949844302,-56.9651221381903,
-38.5745673038812));
#268471=CARTESIAN_POINT('Ctrl Pts',(-42.3712216906218,-56.8916587034686,
-38.564820665347));
#268472=CARTESIAN_POINT('Ctrl Pts',(-42.4063979707918,-56.7834465224234,
-38.5515118436));
#268473=CARTESIAN_POINT('Ctrl Pts',(-42.4468320479729,-56.6771725078319,
-38.5395042677724));
#268474=CARTESIAN_POINT('Ctrl Pts',(-42.4925290654744,-56.5728473165674,
-38.5288039137004));
#268475=CARTESIAN_POINT('Ctrl Pts',(-42.5265325119253,-56.5046058456765,
-38.5225509073062));
#268476=CARTESIAN_POINT('Ctrl Pts',(-42.5623338475306,-56.4370293947697,
-38.5167461666044));
#268477=CARTESIAN_POINT('Ctrl Pts',(-42.5811223641794,-56.4035923099625,
-38.5140693065785));
#268478=CARTESIAN_POINT('Ctrl Pts',(-42.620584523009,-56.3373241998654,
-38.5091697400817));
#268479=CARTESIAN_POINT('Ctrl Pts',(-42.6411082254821,-56.3047465904101,
-38.5069659500128));
#268480=CARTESIAN_POINT('Ctrl Pts',(-42.7048067991197,-56.2090283357163,
-38.501110858935));
#268481=CARTESIAN_POINT('Ctrl Pts',(-42.7502234543428,-56.1476408662828,
-38.4981890389281));
#268482=CARTESIAN_POINT('Ctrl Pts',(-42.8467942323831,-56.0297655581676,
-38.4942910511033));
#268483=CARTESIAN_POINT('Ctrl Pts',(-42.8979715413934,-55.9732420482176,
-38.4933125989996));
#268484=CARTESIAN_POINT('Ctrl Pts',(-42.9790570553347,-55.8921695883033,
-38.4933149859729));
#268485=CARTESIAN_POINT('Ctrl Pts',(-43.0068374106561,-55.8657400908868,
-38.4935622007431));
#268486=CARTESIAN_POINT('Ctrl Pts',(-43.0495800649421,-55.8270637749536,
-38.4943063068789));
#268487=CARTESIAN_POINT('Ctrl Pts',(-43.0640222060113,-55.8143203511958,
-38.494617152342));
#268488=CARTESIAN_POINT('Ctrl Pts',(-43.0932714774893,-55.7891564261061,
-38.4953646906773));
#268489=CARTESIAN_POINT('Ctrl Pts',(-43.1080901283632,-55.7767277938553,
-38.4958020036096));
#268490=CARTESIAN_POINT('Ctrl Pts',(-43.1528523310046,-55.7401327167866,
-38.4972962980169));
#268491=CARTESIAN_POINT('Ctrl Pts',(-43.2134913856688,-55.6930468850421,
-38.4997758707861));
#268492=CARTESIAN_POINT('Ctrl Pts',(-43.3385569247743,-55.6055389451161,
-38.5066450244003));
#268493=CARTESIAN_POINT('Ctrl Pts',(-43.4691986576013,-55.5278792007279,
-38.5163302992824));
#268494=CARTESIAN_POINT('Ctrl Pts',(-43.5713395927684,-55.4769743237494,
-38.5256877381308));
#268495=CARTESIAN_POINT('Ctrl Pts',(-43.6403672861995,-55.4446857735354,
-38.5323951500278));
#268496=CARTESIAN_POINT('Ctrl Pts',(-43.6753577685123,-55.4293620157832,
-38.5359845633874));
#268497=CARTESIAN_POINT('Ctrl Pts',(-43.7462462065788,-55.4003985583156,
-38.5436333065981));
#268498=CARTESIAN_POINT('Ctrl Pts',(-43.7822717759725,-55.3867204456352,
-38.5477088862383));
#268499=CARTESIAN_POINT('Ctrl Pts',(-43.8543821738219,-55.3613797848081,
-38.5562346427694));
#268500=CARTESIAN_POINT('Ctrl Pts',(-43.890622407919,-55.349649082917,-38.5607007444526));
#268501=CARTESIAN_POINT('Ctrl Pts',(-43.9997560709039,-55.3172704656441,
-38.5746802407103));
#268502=CARTESIAN_POINT('Ctrl Pts',(-44.1098017310836,-55.290468361793,
-38.5898286859852));
#268503=CARTESIAN_POINT('Ctrl Pts',(-44.2583166685835,-55.2656490138239,
-38.612301023075));
#268504=CARTESIAN_POINT('Ctrl Pts',(-44.3705972700495,-55.2524997368729,
-38.6302900391873));
#268505=CARTESIAN_POINT('Ctrl Pts',(-44.446056048267,-55.2474029004138,
-38.6430428201589));
#268506=CARTESIAN_POINT('Ctrl Pts',(-44.5218128020516,-55.2441636366351,
-38.65617756452));
#268507=CARTESIAN_POINT('Ctrl Pts',(-44.5599089424743,-55.2434808562086,
-38.6629497802385));
#268508=CARTESIAN_POINT('Ctrl Pts',(-44.6354869543582,-55.2439911084578,
-38.6767130108817));
#268509=CARTESIAN_POINT('Ctrl Pts',(-44.6731456892459,-55.2451740103824,
-38.6837342374529));
#268510=CARTESIAN_POINT('Ctrl Pts',(-44.7481014788608,-55.2493620066237,
-38.6980304684339));
#268511=CARTESIAN_POINT('Ctrl Pts',(-44.860046548974,-55.2583760573225,
-38.7198650218829));
#268512=CARTESIAN_POINT('Ctrl Pts',(-45.0073845433675,-55.2811507310277,
-38.7505067688753));
#268513=CARTESIAN_POINT('Ctrl Pts',(-45.1528189888476,-55.3146135839333,
-38.7826550300594));
#268514=CARTESIAN_POINT('Ctrl Pts',(-45.2248832056965,-55.3349380951144,
-38.7992310848652));
#268515=CARTESIAN_POINT('Ctrl Pts',(-45.2966462681613,-55.3570913336823,
-38.8160672125853));
#268516=CARTESIAN_POINT('Ctrl Pts',(-45.3323638946335,-55.3690863290504,
-38.8246135819642));
#268517=CARTESIAN_POINT('Ctrl Pts',(-45.4027951436545,-55.3946744461232,
-38.841798196801));
#268518=CARTESIAN_POINT('Ctrl Pts',(-45.4376370321487,-55.4083060218429,
-38.85046633842));
#268519=CARTESIAN_POINT('Ctrl Pts',(-45.5409345111852,-55.4516493275196,
-38.8766665754573));
#268520=CARTESIAN_POINT('Ctrl Pts',(-45.6082182891413,-55.4838201174091,
-38.8944064774514));
#268521=CARTESIAN_POINT('Ctrl Pts',(-45.7067749877369,-55.5369855856676,
-38.9214216121435));
#268522=CARTESIAN_POINT('Ctrl Pts',(-45.7392219877795,-55.5555212114618,
-38.9304915704334));
#268523=CARTESIAN_POINT('Ctrl Pts',(-45.8033556832395,-55.5942722159849,
-38.9487787872477));
#268524=CARTESIAN_POINT('Ctrl Pts',(-45.8348443691401,-55.6143675312756,
-38.9579395118015));
#268525=CARTESIAN_POINT('Ctrl Pts',(-45.9274099842789,-55.6766589025306,
-38.9854159162723));
#268526=CARTESIAN_POINT('Ctrl Pts',(-45.9867610865919,-55.7209353156014,
-39.0037703637879));
#268527=CARTESIAN_POINT('Ctrl Pts',(-46.1007337830098,-55.8148102393793,
-39.0405190865864));
#268528=CARTESIAN_POINT('Ctrl Pts',(-46.1826971388658,-55.889219933262,
-39.0681181728269));
#268529=CARTESIAN_POINT('Ctrl Pts',(-46.259356574729,-55.9696687352924,
-39.0957737179551));
#268530=CARTESIAN_POINT('Ctrl Pts',(-46.309266807939,-56.024663053365,-39.1142236413887));
#268531=CARTESIAN_POINT('Ctrl Pts',(-46.3336138177017,-56.0528284109483,
-39.1234510495426));
#268532=CARTESIAN_POINT('Ctrl Pts',(-46.3692509284248,-56.0961546965833,
-39.1373141736981));
#268533=CARTESIAN_POINT('Ctrl Pts',(-46.3809719555493,-56.1107655250657,
-39.14193505412));
#268534=CARTESIAN_POINT('Ctrl Pts',(-46.4039850968433,-56.1401806715041,
-39.1511314768264));
#268535=CARTESIAN_POINT('Ctrl Pts',(-46.4153001903629,-56.1550126624776,
-39.1557159133813));
#268536=CARTESIAN_POINT('Ctrl Pts',(-46.4486370096885,-56.1998310060263,
-39.1694131182659));
#268537=CARTESIAN_POINT('Ctrl Pts',(-46.4700835091466,-56.2301795317326,
-39.1784826054425));
#268538=CARTESIAN_POINT('Ctrl Pts',(-46.532071913686,-56.3225583984772,
-39.2054898733524));
#268539=CARTESIAN_POINT('Ctrl Pts',(-46.5894197348374,-56.4176636744323,
-39.23211607576));
#268540=CARTESIAN_POINT('Ctrl Pts',(-46.6566074362748,-56.5498680842415,
-39.2668544229849));
#268541=CARTESIAN_POINT('Ctrl Pts',(-46.6870820302515,-56.617790568625,
-39.2839693714534));
#268542=CARTESIAN_POINT('Ctrl Pts',(-46.7159729830272,-56.6866360545619,
-39.3009558869148));
#268543=CARTESIAN_POINT('Ctrl Pts',(-46.7296188023799,-56.7214992889704,
-39.3093799218186));
#268544=CARTESIAN_POINT('Ctrl Pts',(-46.7553216997643,-56.7922546384013,
-39.3261176641085));
#268545=CARTESIAN_POINT('Ctrl Pts',(-46.7672996943011,-56.8279354881579,
-39.3343809787628));
#268546=CARTESIAN_POINT('Ctrl Pts',(-46.8004530502947,-56.9353633959568,
-39.358737163018));
#268547=CARTESIAN_POINT('Ctrl Pts',(-46.8189795501832,-57.0077635587999,
-39.3744658121213));
#268548=CARTESIAN_POINT('Ctrl Pts',(-46.848916211803,-57.1540080946302,
-39.4048998290393));
#268549=CARTESIAN_POINT('Ctrl Pts',(-46.866048617508,-57.2647966217996,
-39.4269646939479));
#268550=CARTESIAN_POINT('Ctrl Pts',(-46.875074749658,-57.3772756893033,
-39.4478819384746));
#268551=CARTESIAN_POINT('Ctrl Pts',(-46.8792542953452,-57.4526370309597,
-39.4615663943076));
#268552=CARTESIAN_POINT('Ctrl Pts',(-46.8804258736835,-57.4905390832845,
-39.4682843608713));
#268553=CARTESIAN_POINT('Ctrl Pts',(-46.8808837743635,-57.566610437341,
-39.4814341960201));
#268554=CARTESIAN_POINT('Ctrl Pts',(-46.8801708637706,-57.604491394965,
-39.4878166677226));
#268555=CARTESIAN_POINT('Ctrl Pts',(-46.8768913879562,-57.6800597985945,
-39.5002231148134));
#268556=CARTESIAN_POINT('Ctrl Pts',(-46.8691896925243,-57.7930657109158,
-39.5182849936093));
#268557=CARTESIAN_POINT('Ctrl Pts',(-46.8479069711518,-57.9423669591112,
-39.540205996752));
#268558=CARTESIAN_POINT('Ctrl Pts',(-46.8236459543104,-58.053306681129,
-39.5550278422771));
#268559=CARTESIAN_POINT('Ctrl Pts',(-46.8055990109883,-58.1270324939452,
-39.5645447403379));
#268560=CARTESIAN_POINT('Ctrl Pts',(-46.7956339676918,-58.1637938532181,
-39.5691227921436));
#268561=CARTESIAN_POINT('Ctrl Pts',(-46.7738161327052,-58.2370162077019,
-39.5779016468881));
#268562=CARTESIAN_POINT('Ctrl Pts',(-46.7619036278491,-58.2736352268715,
-39.5821192203466));
#268563=CARTESIAN_POINT('Ctrl Pts',(-46.7364059718256,-58.3458255995332,
-39.5900871854462));
#268564=CARTESIAN_POINT('Ctrl Pts',(-46.7091836493705,-58.4171862986019,
-39.5976163356366));
#268565=CARTESIAN_POINT('Ctrl Pts',(-46.663274408039,-58.5216699086648,
-39.6076014242402));
#268566=CARTESIAN_POINT('Ctrl Pts',(-46.6123207377325,-58.6236436013082,
-39.616293729045));
#268567=CARTESIAN_POINT('Ctrl Pts',(-46.5563244858032,-58.7230996041114,
-39.6236943138341));
#268568=CARTESIAN_POINT('Ctrl Pts',(-46.515607032986,-58.7877140896312,
-39.6277619492082));
#268569=CARTESIAN_POINT('Ctrl Pts',(-46.4731710833873,-58.8514710047945,
-39.6313905635194));
#268570=CARTESIAN_POINT('Ctrl Pts',(-46.4511086137465,-58.8829006319494,
-39.6329844599904));
#268571=CARTESIAN_POINT('Ctrl Pts',(-46.4051673201274,-58.9449633016888,
-39.6357273485653));
#268572=CARTESIAN_POINT('Ctrl Pts',(-46.381447994276,-58.975377588932,-39.6368662598532));
#268573=CARTESIAN_POINT('Ctrl Pts',(-46.3084068909562,-59.0643493136614,
-39.6395761233691));
#268574=CARTESIAN_POINT('Ctrl Pts',(-46.2570407846102,-59.1209150453974,
-39.6404603784325));
#268575=CARTESIAN_POINT('Ctrl Pts',(-46.1491379755941,-59.228544463199,
-39.6404138814247));
#268576=CARTESIAN_POINT('Ctrl Pts',(-46.0925836555155,-59.2796343044913,
-39.6394845811684));
#268577=CARTESIAN_POINT('Ctrl Pts',(-46.0038529437629,-59.3521266125547,
-39.6367223387528));
#268578=CARTESIAN_POINT('Ctrl Pts',(-45.9736068078661,-59.3756113554055,
-39.6355721163029));
#268579=CARTESIAN_POINT('Ctrl Pts',(-45.9272656961273,-59.4097723546528,
-39.6334997725088));
#268580=CARTESIAN_POINT('Ctrl Pts',(-45.9116419215573,-59.4209912820171,
-39.6327502808957));
#268581=CARTESIAN_POINT('Ctrl Pts',(-45.8800804794677,-59.4430610802669,
-39.6311351339295));
#268582=CARTESIAN_POINT('Ctrl Pts',(-45.8321587971618,-59.4756823489919,
-39.628531354857));
#268583=CARTESIAN_POINT('Ctrl Pts',(-45.7834097108732,-59.5062438963941,
-39.6254355071979));
#268584=CARTESIAN_POINT('Ctrl Pts',(-45.717633106262,-59.5452481912826,
-39.6208773262667));
#268585=CARTESIAN_POINT('Ctrl Pts',(-45.6178307490054,-59.601113548897,
-39.6133952897297));
#268586=CARTESIAN_POINT('Ctrl Pts',(-45.4802897643185,-59.6652183443042,
-39.6008811885904));
#268587=CARTESIAN_POINT('Ctrl Pts',(-45.3738098009101,-59.7055766782111,
-39.5896017905935));
#268588=CARTESIAN_POINT('Ctrl Pts',(-45.3020778813705,-59.7307512119865,
-39.5816566825671));
#268589=CARTESIAN_POINT('Ctrl Pts',(-45.2658207311094,-59.7424779859237,
-39.5774690651077));
#268590=CARTESIAN_POINT('Ctrl Pts',(-45.1926264675053,-59.7641596016776,
-39.5686715125846));
#268591=CARTESIAN_POINT('Ctrl Pts',(-45.1555073907618,-59.7741562512684,
-39.5640376159893));
#268592=CARTESIAN_POINT('Ctrl Pts',(-45.0441315765335,-59.8011904590316,
-39.5496210468413));
#268593=CARTESIAN_POINT('Ctrl Pts',(-44.9324484012679,-59.8224577850013,
-39.5341534065747));
#268594=CARTESIAN_POINT('Ctrl Pts',(-44.8203079610257,-59.8353953605365,
-39.5171556909205));
#268595=CARTESIAN_POINT('Ctrl Pts',(-44.7080184564226,-59.8455760612675,
-39.4996502778008));
#268596=CARTESIAN_POINT('Ctrl Pts',(-44.6329372249224,-59.8486931621852,
-39.4873001861445));
#268597=CARTESIAN_POINT('Ctrl Pts',(-44.5200834441659,-59.8478515133141,
-39.4677634802869));
#268598=CARTESIAN_POINT('Ctrl Pts',(-44.4823810871712,-59.8466449718289,
-39.4610736497974));
#268599=CARTESIAN_POINT('Ctrl Pts',(-44.4258051079382,-59.8434394706745,
-39.4507883432074));
#268600=CARTESIAN_POINT('Ctrl Pts',(-44.4069254589855,-59.8421361346926,
-39.4473147915973));
#268601=CARTESIAN_POINT('Ctrl Pts',(-44.3691376542581,-59.8390581625153,
-39.4402793331445));
#268602=CARTESIAN_POINT('Ctrl Pts',(-44.3502459350849,-59.8372838734483,
-39.4367203104461));
#268603=CARTESIAN_POINT('Ctrl Pts',(-44.2562487381671,-59.8272835659938,
-39.4188041728073));
#268604=CARTESIAN_POINT('Ctrl Pts',(-44.1080045765469,-59.8040393501646,
-39.3892226636159));
#268605=CARTESIAN_POINT('Ctrl Pts',(-43.9639303529155,-59.7668593120831,
-39.3578670379715));
#268606=CARTESIAN_POINT('Ctrl Pts',(-43.8219159040518,-59.7227861654643,
-39.3256251231267));
#268607=CARTESIAN_POINT('Ctrl Pts',(-43.7519290534068,-59.6972943066161,
-39.3090578287531));
#268608=CARTESIAN_POINT('Ctrl Pts',(-43.665783177736,-59.6610675807531,
-39.2877890488175));
#268609=CARTESIAN_POINT('Ctrl Pts',(-43.6486106666635,-59.653596197985,
-39.2835041280971));
#268610=CARTESIAN_POINT('Ctrl Pts',(-43.6144193015916,-59.6382222359849,
-39.2748825183767));
#268611=CARTESIAN_POINT('Ctrl Pts',(-43.597366582891,-59.6303022352814,
-39.2705368924251));
#268612=CARTESIAN_POINT('Ctrl Pts',(-43.5465994182959,-59.605961903298,
-39.2574616452183));
#268613=CARTESIAN_POINT('Ctrl Pts',(-43.513329300663,-59.588993111175,-39.2487085268073));
#268614=CARTESIAN_POINT('Ctrl Pts',(-43.4805771074156,-59.5712767529309,
-39.2399080357013));
#268615=CARTESIAN_POINT('Ctrl Pts',(-43.8341420587998,-57.9817357678076,
-41.1268248734572));
#268616=CARTESIAN_POINT('Ctrl Pts',(-43.8090823387197,-57.9680163597508,
-41.1092238912453));
#268617=CARTESIAN_POINT('Ctrl Pts',(-43.7605654269547,-57.9383371077444,
-41.0736746770147));
#268618=CARTESIAN_POINT('Ctrl Pts',(-43.6924895655639,-57.8872515755908,
-41.019320019256));
#268619=CARTESIAN_POINT('Ctrl Pts',(-43.6502497090231,-57.8487916199066,
-40.9823828883729));
#268620=CARTESIAN_POINT('Ctrl Pts',(-43.6096433745973,-57.8080652293815,
-40.945090157748));
#268621=CARTESIAN_POINT('Ctrl Pts',(-43.5713160673933,-57.7657212262301,
-40.9080353139296));
#268622=CARTESIAN_POINT('Ctrl Pts',(-43.5288984657655,-57.7088609123343,
-40.8622751058818));
#268623=CARTESIAN_POINT('Ctrl Pts',(-43.4982484100127,-57.6610280687967,
-40.826006689079));
#268624=CARTESIAN_POINT('Ctrl Pts',(-43.4769169762936,-57.6239677344727,
-40.798976453902));
#268625=CARTESIAN_POINT('Ctrl Pts',(-43.4638199758968,-57.5984660781933,
-40.7810781735695));
#268626=CARTESIAN_POINT('Ctrl Pts',(-43.4512904535732,-57.5725430453748,
-40.7632325534464));
#268627=CARTESIAN_POINT('Ctrl Pts',(-43.4453582046716,-57.5594707895743,
-40.7544050886758));
#268628=CARTESIAN_POINT('Ctrl Pts',(-43.4285595200757,-57.5199648485381,
-40.7282304644163));
#268629=CARTESIAN_POINT('Ctrl Pts',(-43.4088016745783,-57.4664867157472,
-40.6941268792613));
#268630=CARTESIAN_POINT('Ctrl Pts',(-43.3942530508608,-57.4114223976644,
-40.6616070010832));
#268631=CARTESIAN_POINT('Ctrl Pts',(-43.3853242538269,-57.3695231591805,
-40.6378273627645));
#268632=CARTESIAN_POINT('Ctrl Pts',(-43.3826786150667,-57.3554536366825,
-40.630001230023));
#268633=CARTESIAN_POINT('Ctrl Pts',(-43.378062215599,-57.3271160344971,
-40.6145607014775));
#268634=CARTESIAN_POINT('Ctrl Pts',(-43.3760891270041,-57.3128275119467,
-40.60693561976));
#268635=CARTESIAN_POINT('Ctrl Pts',(-43.3728422231051,-57.2841093232557,
-40.5919365051523));
#268636=CARTESIAN_POINT('Ctrl Pts',(-43.3715781643254,-57.2697777029377,
-40.5846130830795));
#268637=CARTESIAN_POINT('Ctrl Pts',(-43.3697526802575,-57.2411194243864,
-40.5702888754578));
#268638=CARTESIAN_POINT('Ctrl Pts',(-43.3680717796799,-57.1981642741791,
-40.5492997469169));
#268639=CARTESIAN_POINT('Ctrl Pts',(-43.3700185838812,-57.1410182421193,
-40.5232909177883));
#268640=CARTESIAN_POINT('Ctrl Pts',(-43.3746384661022,-57.0982543712987,
-40.505286899195));
#268641=CARTESIAN_POINT('Ctrl Pts',(-43.3784319419536,-57.0697666559562,
-40.4936247912381));
#268642=CARTESIAN_POINT('Ctrl Pts',(-43.3806866868643,-57.0555278483981,
-40.4879619013523));
#268643=CARTESIAN_POINT('Ctrl Pts',(-43.3859186984709,-57.0270949764048,
-40.476993052777));
#268644=CARTESIAN_POINT('Ctrl Pts',(-43.3889115442249,-57.0128413374093,
-40.4716662621118));
#268645=CARTESIAN_POINT('Ctrl Pts',(-43.3955695423488,-56.984668670318,
-40.4614841416371));
#268646=CARTESIAN_POINT('Ctrl Pts',(-43.4029115329907,-56.9567427536229,
-40.4517375031029));
#268647=CARTESIAN_POINT('Ctrl Pts',(-43.4159439893498,-56.915628788467,
-40.4384286813559));
#268648=CARTESIAN_POINT('Ctrl Pts',(-43.4309850942545,-56.8752725380991,
-40.4264211055283));
#268649=CARTESIAN_POINT('Ctrl Pts',(-43.4480370013178,-56.8356780486645,
-40.4157207514563));
#268650=CARTESIAN_POINT('Ctrl Pts',(-43.4607570961379,-56.8097932355363,
-40.409467745062));
#268651=CARTESIAN_POINT('Ctrl Pts',(-43.4741642201056,-56.7841683331057,
-40.4036630043601));
#268652=CARTESIAN_POINT('Ctrl Pts',(-43.4812071336048,-56.7714928975767,
-40.4009861443346));
#268653=CARTESIAN_POINT('Ctrl Pts',(-43.4960130774609,-56.7463797512019,
-40.3960865778375));
#268654=CARTESIAN_POINT('Ctrl Pts',(-43.5037198572985,-56.7340380787953,
-40.3938827877695));
#268655=CARTESIAN_POINT('Ctrl Pts',(-43.527657505214,-56.6977883833479,
-40.3880276966888));
#268656=CARTESIAN_POINT('Ctrl Pts',(-43.5447483375558,-56.6745564757614,
-40.3851058766842));
#268657=CARTESIAN_POINT('Ctrl Pts',(-43.5811328114983,-56.629979998045,
-40.3812078888591));
#268658=CARTESIAN_POINT('Ctrl Pts',(-43.6004351631962,-56.6086219171049,
-40.3802294367552));
#268659=CARTESIAN_POINT('Ctrl Pts',(-43.6310475296952,-56.578014570072,
-40.3802318237287));
#268660=CARTESIAN_POINT('Ctrl Pts',(-43.6415402048873,-56.5680413281089,
-40.3804790384992));
#268661=CARTESIAN_POINT('Ctrl Pts',(-43.6576911458811,-56.5534539772523,
-40.3812231446347));
#268662=CARTESIAN_POINT('Ctrl Pts',(-43.6631494628181,-56.5486488515781,
-40.3815339900979));
#268663=CARTESIAN_POINT('Ctrl Pts',(-43.6742063152013,-56.5391628964206,
-40.3822815284329));
#268664=CARTESIAN_POINT('Ctrl Pts',(-43.6798092119243,-56.534479009001,
-40.3827188413654));
#268665=CARTESIAN_POINT('Ctrl Pts',(-43.6967370434146,-56.5206915949946,
-40.3842131357726));
#268666=CARTESIAN_POINT('Ctrl Pts',(-43.7196778600618,-56.5029622466235,
-40.386692708542));
#268667=CARTESIAN_POINT('Ctrl Pts',(-43.7670264629127,-56.4700551612604,
-40.3935618621563));
#268668=CARTESIAN_POINT('Ctrl Pts',(-43.8165352419067,-56.4409186299576,
-40.4032471370382));
#268669=CARTESIAN_POINT('Ctrl Pts',(-43.8552784957563,-56.4218759376155,
-40.4126045758866));
#268670=CARTESIAN_POINT('Ctrl Pts',(-43.8814691350842,-56.4098116142502,
-40.4193119877837));
#268671=CARTESIAN_POINT('Ctrl Pts',(-43.8947490665381,-56.4040935548973,
-40.4229014011429));
#268672=CARTESIAN_POINT('Ctrl Pts',(-43.9216608718689,-56.3933018151258,
-40.430550144354));
#268673=CARTESIAN_POINT('Ctrl Pts',(-43.9353412421961,-56.3882139347518,
-40.434625723994));
#268674=CARTESIAN_POINT('Ctrl Pts',(-43.9627318697344,-56.3788058930362,
-40.4431514805252));
#268675=CARTESIAN_POINT('Ctrl Pts',(-43.9765011076412,-56.3744602994329,
-40.4476175822086));
#268676=CARTESIAN_POINT('Ctrl Pts',(-44.0179764085085,-56.3624961934912,
-40.4615970784657));
#268677=CARTESIAN_POINT('Ctrl Pts',(-44.0598195105868,-56.3526585058303,
-40.4767455237411));
#268678=CARTESIAN_POINT('Ctrl Pts',(-44.1163310625808,-56.3437038269143,
-40.4992178608308));
#268679=CARTESIAN_POINT('Ctrl Pts',(-44.1590753545772,-56.3390714325247,
-40.5172068769433));
#268680=CARTESIAN_POINT('Ctrl Pts',(-44.1878153726385,-56.337382052278,
-40.5299596579145));
#268681=CARTESIAN_POINT('Ctrl Pts',(-44.2166756293141,-56.3364007867548,
-40.5430944022758));
#268682=CARTESIAN_POINT('Ctrl Pts',(-44.2311921171808,-56.3362675100036,
-40.5498666179945));
#268683=CARTESIAN_POINT('Ctrl Pts',(-44.2599977007373,-56.3367129587916,
-40.5636298486377));
#268684=CARTESIAN_POINT('Ctrl Pts',(-44.2743541649932,-56.3372884158027,
-40.5706510752088));
#268685=CARTESIAN_POINT('Ctrl Pts',(-44.3029357424357,-56.3391317429585,
-40.5849473061899));
#268686=CARTESIAN_POINT('Ctrl Pts',(-44.3456316213443,-56.3429350642169,
-40.6067818596389));
#268687=CARTESIAN_POINT('Ctrl Pts',(-44.4018650235691,-56.3520939287388,
-40.6374236066311));
#268688=CARTESIAN_POINT('Ctrl Pts',(-44.4574103376146,-56.3653147883305,
-40.6695718678152));
#268689=CARTESIAN_POINT('Ctrl Pts',(-44.4849466005937,-56.3732907222196,
-40.686147922621));
#268690=CARTESIAN_POINT('Ctrl Pts',(-44.512374392093,-56.3819617528141,
-40.7029840503412));
#268691=CARTESIAN_POINT('Ctrl Pts',(-44.5260289861432,-56.3866462995878,
-40.7115304197201));
#268692=CARTESIAN_POINT('Ctrl Pts',(-44.5529609776699,-56.3966203919845,
-40.7287150345567));
#268693=CARTESIAN_POINT('Ctrl Pts',(-44.5662873943758,-56.4019250012471,
-40.737383176176));
#268694=CARTESIAN_POINT('Ctrl Pts',(-44.6058068395674,-56.4187668411382,
-40.7635834132132));
#268695=CARTESIAN_POINT('Ctrl Pts',(-44.6315615859976,-56.4312362585519,
-40.7813233152079));
#268696=CARTESIAN_POINT('Ctrl Pts',(-44.6693071486035,-56.4518014713652,
-40.8083384498991));
#268697=CARTESIAN_POINT('Ctrl Pts',(-44.6817372625133,-56.458965010373,
-40.8174084081892));
#268698=CARTESIAN_POINT('Ctrl Pts',(-44.7063132537473,-56.473929075182,
-40.8356956250034));
#268699=CARTESIAN_POINT('Ctrl Pts',(-44.7183832523531,-56.4816832398284,
-40.8448563495594));
#268700=CARTESIAN_POINT('Ctrl Pts',(-44.7538754102704,-56.505703003501,
-40.8723327540241));
#268701=CARTESIAN_POINT('Ctrl Pts',(-44.7766465418209,-56.5227549736834,
-40.8906872015444));
#268702=CARTESIAN_POINT('Ctrl Pts',(-44.8204030914552,-56.5588699415109,
-40.9274359243417));
#268703=CARTESIAN_POINT('Ctrl Pts',(-44.851893062885,-56.5874690797881,
-40.9550350105826));
#268704=CARTESIAN_POINT('Ctrl Pts',(-44.8813802932551,-56.6183507815631,
-40.982690555711));
#268705=CARTESIAN_POINT('Ctrl Pts',(-44.9005867815582,-56.6394533348067,
-41.0011404791447));
#268706=CARTESIAN_POINT('Ctrl Pts',(-44.9099603095753,-56.6502571213647,
-41.0103678872986));
#268707=CARTESIAN_POINT('Ctrl Pts',(-44.9236872082217,-56.6668706184025,
-41.0242310114538));
#268708=CARTESIAN_POINT('Ctrl Pts',(-44.9282031316495,-56.6724722064122,
-41.0288518918758));
#268709=CARTESIAN_POINT('Ctrl Pts',(-44.9370720489983,-56.6837477093971,
-41.038048314582));
#268710=CARTESIAN_POINT('Ctrl Pts',(-44.9414338933841,-56.6894322363092,
-41.0426327511372));
#268711=CARTESIAN_POINT('Ctrl Pts',(-44.9542884395491,-56.7066066663578,
-41.0563299560217));
#268712=CARTESIAN_POINT('Ctrl Pts',(-44.9625629539304,-56.7182326826763,
-41.0653994431984));
#268713=CARTESIAN_POINT('Ctrl Pts',(-44.9864941991718,-56.7536111473724,
-41.0924067111081));
#268714=CARTESIAN_POINT('Ctrl Pts',(-45.0086645271567,-56.7900134244028,
-41.1190329135161));
#268715=CARTESIAN_POINT('Ctrl Pts',(-45.034704630644,-56.8405768845403,
-41.1537712607408));
#268716=CARTESIAN_POINT('Ctrl Pts',(-45.0465408860903,-56.8665423758261,
-41.1708862092094));
#268717=CARTESIAN_POINT('Ctrl Pts',(-45.0577761134165,-56.8928546179869,
-41.1878727246706));
#268718=CARTESIAN_POINT('Ctrl Pts',(-45.0630901582258,-56.906176087846,
-41.1962967595746));
#268719=CARTESIAN_POINT('Ctrl Pts',(-45.0731156002939,-56.9332061371524,
-41.2130345018643));
#268720=CARTESIAN_POINT('Ctrl Pts',(-45.0777961712447,-56.9468340019015,
-41.2212978165198));
#268721=CARTESIAN_POINT('Ctrl Pts',(-45.0907786540592,-56.9878560258786,
-41.2456540007716));
#268722=CARTESIAN_POINT('Ctrl Pts',(-45.0980724298404,-57.0154910056487,
-41.2613826498774));
#268723=CARTESIAN_POINT('Ctrl Pts',(-45.1099506000897,-57.0712899900431,
-41.2918166667949));
#268724=CARTESIAN_POINT('Ctrl Pts',(-45.1168338059478,-57.11354441615,-41.3138815317038));
#268725=CARTESIAN_POINT('Ctrl Pts',(-45.1206309792415,-57.1564190282566,
-41.3347987762303));
#268726=CARTESIAN_POINT('Ctrl Pts',(-45.1224627479043,-57.1851396939165,
-41.3484832320635));
#268727=CARTESIAN_POINT('Ctrl Pts',(-45.1230291819396,-57.199581674993,
-41.3552011986272));
#268728=CARTESIAN_POINT('Ctrl Pts',(-45.1234439819388,-57.2285619504273,
-41.3683510337761));
#268729=CARTESIAN_POINT('Ctrl Pts',(-45.1232917301137,-57.2429904040975,
-41.3747335054784));
#268730=CARTESIAN_POINT('Ctrl Pts',(-45.122279779691,-57.2717682086368,
-41.3871399525693));
#268731=CARTESIAN_POINT('Ctrl Pts',(-45.1196997436484,-57.3147947598186,
-41.4052018313649));
#268732=CARTESIAN_POINT('Ctrl Pts',(-45.1120557453653,-57.3716084168758,
-41.4271228345082));
#268733=CARTESIAN_POINT('Ctrl Pts',(-45.1031553338884,-57.4137999065974,
-41.4419446800329));
#268734=CARTESIAN_POINT('Ctrl Pts',(-45.09650693546,-57.4418330021969,-41.4514615780937));
#268735=CARTESIAN_POINT('Ctrl Pts',(-45.092823442876,-57.4558081403435,
-41.4560396298995));
#268736=CARTESIAN_POINT('Ctrl Pts',(-45.08473584999,-57.4836385233421,-41.464818484644));
#268737=CARTESIAN_POINT('Ctrl Pts',(-45.0803094818206,-57.4975537933777,
-41.4690360581021));
#268738=CARTESIAN_POINT('Ctrl Pts',(-45.0708158371377,-57.5249803724867,
-41.4770040232021));
#268739=CARTESIAN_POINT('Ctrl Pts',(-45.060662137239,-57.5520858826269,
-41.4845331733926));
#268740=CARTESIAN_POINT('Ctrl Pts',(-45.0434887903859,-57.591755117417,
-41.4945182619959));
#268741=CARTESIAN_POINT('Ctrl Pts',(-45.0243848727922,-57.6304534586566,
-41.5032105668009));
#268742=CARTESIAN_POINT('Ctrl Pts',(-45.0033512023575,-57.6681778817651,
-41.51061115159));
#268743=CARTESIAN_POINT('Ctrl Pts',(-44.9880328234845,-57.692673879575,
-41.5146787869643));
#268744=CARTESIAN_POINT('Ctrl Pts',(-44.9720568870916,-57.7168380825906,
-41.5183074012753));
#268745=CARTESIAN_POINT('Ctrl Pts',(-44.9637457009402,-57.7287466936453,
-41.5199012977462));
#268746=CARTESIAN_POINT('Ctrl Pts',(-44.9464287138105,-57.7522550306847,
-41.5226441863212));
#268747=CARTESIAN_POINT('Ctrl Pts',(-44.9374830238235,-57.7637718882179,
-41.5237830976086));
#268748=CARTESIAN_POINT('Ctrl Pts',(-44.9099214446927,-57.7974515399035,
-41.5264929611258));
#268749=CARTESIAN_POINT('Ctrl Pts',(-44.8905204729439,-57.8188493934961,
-41.5273772161885));
#268750=CARTESIAN_POINT('Ctrl Pts',(-44.8497318000032,-57.8595330722204,
-41.5273307191807));
#268751=CARTESIAN_POINT('Ctrl Pts',(-44.8283374647208,-57.878828810327,
-41.5264014189239));
#268752=CARTESIAN_POINT('Ctrl Pts',(-44.7947479986672,-57.9061820008563,
-41.5236391765087));
#268753=CARTESIAN_POINT('Ctrl Pts',(-44.7832945060713,-57.9150388128137,
-41.5224889540588));
#268754=CARTESIAN_POINT('Ctrl Pts',(-44.7657408175914,-57.9279147771907,
-41.5204166102647));
#268755=CARTESIAN_POINT('Ctrl Pts',(-44.7598217545323,-57.9321421746299,
-41.5196671186517));
#268756=CARTESIAN_POINT('Ctrl Pts',(-44.7478629508254,-57.9404557426351,
-41.5180519716851));
#268757=CARTESIAN_POINT('Ctrl Pts',(-44.7297025277655,-57.9527400844071,
-41.5154481926132));
#268758=CARTESIAN_POINT('Ctrl Pts',(-44.711220794734,-57.9642369190977,
-41.5123523449538));
#268759=CARTESIAN_POINT('Ctrl Pts',(-44.6862770262529,-57.9788987855805,
-41.5077941640223));
#268760=CARTESIAN_POINT('Ctrl Pts',(-44.6484202704456,-57.9998814948776,
-41.5003121274858));
#268761=CARTESIAN_POINT('Ctrl Pts',(-44.5962108390282,-58.0238874022289,
-41.4877980263462));
#268762=CARTESIAN_POINT('Ctrl Pts',(-44.5557649369164,-58.0389385823793,
-41.4765186283493));
#268763=CARTESIAN_POINT('Ctrl Pts',(-44.5285120653069,-58.048310487242,
-41.4685735203231));
#268764=CARTESIAN_POINT('Ctrl Pts',(-44.5147341086114,-58.0526671867402,
-41.4643859028639));
#268765=CARTESIAN_POINT('Ctrl Pts',(-44.4869140318333,-58.0607029371288,
-41.4555883503401));
#268766=CARTESIAN_POINT('Ctrl Pts',(-44.4728027150897,-58.0643973546439,
-41.4509544537452));
#268767=CARTESIAN_POINT('Ctrl Pts',(-44.4304531283686,-58.0743536715507,
-41.4365378845966));
#268768=CARTESIAN_POINT('Ctrl Pts',(-44.3879697631396,-58.0821103913619,
-41.4210702443308));
#268769=CARTESIAN_POINT('Ctrl Pts',(-44.3452880889881,-58.0866896268435,
-41.4040725286766));
#268770=CARTESIAN_POINT('Ctrl Pts',(-44.3025416355467,-58.090217180745,
-41.3865671155567));
#268771=CARTESIAN_POINT('Ctrl Pts',(-44.2739489581488,-58.0911687787978,
-41.3742170239002));
#268772=CARTESIAN_POINT('Ctrl Pts',(-44.2309555122234,-58.090491506171,
-41.3546803180427));
#268773=CARTESIAN_POINT('Ctrl Pts',(-44.2165895018292,-58.0899123697243,
-41.347990487553));
#268774=CARTESIAN_POINT('Ctrl Pts',(-44.1950278537333,-58.0885113544661,
-41.337705180963));
#268775=CARTESIAN_POINT('Ctrl Pts',(-44.1878319550126,-58.0879547296283,
-41.3342316293533));
#268776=CARTESIAN_POINT('Ctrl Pts',(-44.1734279164018,-58.0866616594573,
-41.3271961709002));
#268777=CARTESIAN_POINT('Ctrl Pts',(-44.1662260389348,-58.0859253983809,
-41.3236371482021));
#268778=CARTESIAN_POINT('Ctrl Pts',(-44.130389101081,-58.0818150523559,
-41.3057210105631));
#268779=CARTESIAN_POINT('Ctrl Pts',(-44.073848260417,-58.0724828543971,
-41.2761395013722));
#268780=CARTESIAN_POINT('Ctrl Pts',(-44.0188545174212,-58.0578491440998,
-41.2447838757269));
#268781=CARTESIAN_POINT('Ctrl Pts',(-43.9646246641704,-58.0405931079736,
-41.2125419608827));
#268782=CARTESIAN_POINT('Ctrl Pts',(-43.9378880325505,-58.0306505669816,
-41.1959746665064));
#268783=CARTESIAN_POINT('Ctrl Pts',(-43.9049634769563,-58.0165631445999,
-41.174705886574));
#268784=CARTESIAN_POINT('Ctrl Pts',(-43.898399460067,-58.0136596367661,
-41.1704209658528));
#268785=CARTESIAN_POINT('Ctrl Pts',(-43.8853286348063,-58.0076886655405,
-41.1617993561325));
#268786=CARTESIAN_POINT('Ctrl Pts',(-43.8788088737381,-58.0046144513738,
-41.157453730181));
#268787=CARTESIAN_POINT('Ctrl Pts',(-43.8593967360427,-57.9951717320096,
-41.1443784829743));
#268788=CARTESIAN_POINT('Ctrl Pts',(-43.8466719188398,-57.9885954718361,
-41.1356253645631));
#268789=CARTESIAN_POINT('Ctrl Pts',(-43.8341420587998,-57.9817357678076,
-41.1268248734572));
#268790=CARTESIAN_POINT('',(-43.5555682511181,-59.2341350312479,-39.6401231904583));
#268791=CARTESIAN_POINT('Ctrl Pts',(-43.4805771074156,-59.5712767529309,
-39.2399080357013));
#268792=CARTESIAN_POINT('Ctrl Pts',(-43.4150727209207,-59.5358440364426,
-39.2223070534893));
#268793=CARTESIAN_POINT('Ctrl Pts',(-43.2883193276586,-59.4590682572254,
-39.1867578392588));
#268794=CARTESIAN_POINT('Ctrl Pts',(-43.1106712693135,-59.32658002426,-39.1324031814995));
#268795=CARTESIAN_POINT('Ctrl Pts',(-43.0005921597408,-59.2266373021163,
-39.0954660506179));
#268796=CARTESIAN_POINT('Ctrl Pts',(-42.8948534568781,-59.1207134074407,
-39.0581733199915));
#268797=CARTESIAN_POINT('Ctrl Pts',(-42.7951360401793,-59.0104958554849,
-39.0211184761739));
#268798=CARTESIAN_POINT('Ctrl Pts',(-42.6850011896347,-58.8622904152127,
-38.9753582681256));
#268799=CARTESIAN_POINT('Ctrl Pts',(-42.6055727997797,-58.7375004045667,
-38.939089851323));
#268800=CARTESIAN_POINT('Ctrl Pts',(-42.5503788594446,-58.6407591922129,
-38.9120596161462));
#268801=CARTESIAN_POINT('Ctrl Pts',(-42.5165536369311,-58.5741539171446,
-38.8941613358138));
#268802=CARTESIAN_POINT('Ctrl Pts',(-42.4842288567228,-58.5064298632496,
-38.8763157156907));
#268803=CARTESIAN_POINT('Ctrl Pts',(-42.4689425396028,-58.4722695523732,
-38.8674882509199));
#268804=CARTESIAN_POINT('Ctrl Pts',(-42.4257123024776,-58.3690064948315,
-38.8413136266604));
#268805=CARTESIAN_POINT('Ctrl Pts',(-42.3750272156063,-58.229152189777,
-38.8072100415055));
#268806=CARTESIAN_POINT('Ctrl Pts',(-42.3380647902547,-58.0850119200902,
-38.7746901633276));
#268807=CARTESIAN_POINT('Ctrl Pts',(-42.3155659796374,-57.9752818499468,
-38.7509105250088));
#268808=CARTESIAN_POINT('Ctrl Pts',(-42.3089374211558,-57.9384266221928,
-38.7430843922672));
#268809=CARTESIAN_POINT('Ctrl Pts',(-42.297458012674,-57.864178756387,-38.7276438637217));
#268810=CARTESIAN_POINT('Ctrl Pts',(-42.292601515188,-57.8267325312259,
-38.720018782004));
#268811=CARTESIAN_POINT('Ctrl Pts',(-42.2847289916893,-57.7514526301959,
-38.7050196673963));
#268812=CARTESIAN_POINT('Ctrl Pts',(-42.2817363521424,-57.7138759968928,
-38.6976962453237));
#268813=CARTESIAN_POINT('Ctrl Pts',(-42.277596992864,-57.6387184974263,
-38.6833720377019));
#268814=CARTESIAN_POINT('Ctrl Pts',(-42.2741651307842,-57.5260409596698,
-38.6623829091612));
#268815=CARTESIAN_POINT('Ctrl Pts',(-42.2805893100654,-57.3760354719141,
-38.6363740800325));
#268816=CARTESIAN_POINT('Ctrl Pts',(-42.2937061680812,-57.2637038035873,
-38.618370061439));
#268817=CARTESIAN_POINT('Ctrl Pts',(-42.3043247017591,-57.1888547452426,
-38.6067079534822));
#268818=CARTESIAN_POINT('Ctrl Pts',(-42.3105743117123,-57.1514345461221,
-38.6010450635964));
#268819=CARTESIAN_POINT('Ctrl Pts',(-42.3249704170347,-57.0766935209607,
-38.590076215021));
#268820=CARTESIAN_POINT('Ctrl Pts',(-42.3331592025312,-57.0392159768686,
-38.5847494243559));
#268821=CARTESIAN_POINT('Ctrl Pts',(-42.3512949844302,-56.9651221381903,
-38.5745673038812));
#268822=CARTESIAN_POINT('Ctrl Pts',(-42.3712216906218,-56.8916587034686,
-38.564820665347));
#268823=CARTESIAN_POINT('Ctrl Pts',(-42.4063979707918,-56.7834465224234,
-38.5515118436));
#268824=CARTESIAN_POINT('Ctrl Pts',(-42.4468320479729,-56.6771725078319,
-38.5395042677724));
#268825=CARTESIAN_POINT('Ctrl Pts',(-42.4925290654744,-56.5728473165674,
-38.5288039137004));
#268826=CARTESIAN_POINT('Ctrl Pts',(-42.5265325119253,-56.5046058456765,
-38.5225509073062));
#268827=CARTESIAN_POINT('Ctrl Pts',(-42.5623338475306,-56.4370293947697,
-38.5167461666044));
#268828=CARTESIAN_POINT('Ctrl Pts',(-42.5811223641794,-56.4035923099625,
-38.5140693065785));
#268829=CARTESIAN_POINT('Ctrl Pts',(-42.620584523009,-56.3373241998654,
-38.5091697400817));
#268830=CARTESIAN_POINT('Ctrl Pts',(-42.6411082254821,-56.3047465904101,
-38.5069659500128));
#268831=CARTESIAN_POINT('Ctrl Pts',(-42.7048067991197,-56.2090283357163,
-38.501110858935));
#268832=CARTESIAN_POINT('Ctrl Pts',(-42.7502234543428,-56.1476408662828,
-38.4981890389281));
#268833=CARTESIAN_POINT('Ctrl Pts',(-42.8467942323831,-56.0297655581676,
-38.4942910511033));
#268834=CARTESIAN_POINT('Ctrl Pts',(-42.8979715413934,-55.9732420482176,
-38.4933125989996));
#268835=CARTESIAN_POINT('Ctrl Pts',(-42.9790570553347,-55.8921695883033,
-38.4933149859729));
#268836=CARTESIAN_POINT('Ctrl Pts',(-43.0068374106561,-55.8657400908868,
-38.4935622007431));
#268837=CARTESIAN_POINT('Ctrl Pts',(-43.0495800649421,-55.8270637749536,
-38.4943063068789));
#268838=CARTESIAN_POINT('Ctrl Pts',(-43.0640222060113,-55.8143203511958,
-38.494617152342));
#268839=CARTESIAN_POINT('Ctrl Pts',(-43.0932714774893,-55.7891564261061,
-38.4953646906773));
#268840=CARTESIAN_POINT('Ctrl Pts',(-43.1080901283632,-55.7767277938553,
-38.4958020036096));
#268841=CARTESIAN_POINT('Ctrl Pts',(-43.1528523310046,-55.7401327167866,
-38.4972962980169));
#268842=CARTESIAN_POINT('Ctrl Pts',(-43.2134913856688,-55.6930468850421,
-38.4997758707861));
#268843=CARTESIAN_POINT('Ctrl Pts',(-43.3385569247743,-55.6055389451161,
-38.5066450244003));
#268844=CARTESIAN_POINT('Ctrl Pts',(-43.4691986576013,-55.5278792007279,
-38.5163302992824));
#268845=CARTESIAN_POINT('Ctrl Pts',(-43.5713395927684,-55.4769743237494,
-38.5256877381308));
#268846=CARTESIAN_POINT('Ctrl Pts',(-43.6403672861995,-55.4446857735354,
-38.5323951500278));
#268847=CARTESIAN_POINT('Ctrl Pts',(-43.6753577685123,-55.4293620157832,
-38.5359845633874));
#268848=CARTESIAN_POINT('Ctrl Pts',(-43.7462462065788,-55.4003985583156,
-38.5436333065981));
#268849=CARTESIAN_POINT('Ctrl Pts',(-43.7822717759725,-55.3867204456352,
-38.5477088862383));
#268850=CARTESIAN_POINT('Ctrl Pts',(-43.8543821738219,-55.3613797848081,
-38.5562346427694));
#268851=CARTESIAN_POINT('Ctrl Pts',(-43.890622407919,-55.349649082917,-38.5607007444526));
#268852=CARTESIAN_POINT('Ctrl Pts',(-43.9997560709039,-55.3172704656441,
-38.5746802407103));
#268853=CARTESIAN_POINT('Ctrl Pts',(-44.1098017310836,-55.290468361793,
-38.5898286859852));
#268854=CARTESIAN_POINT('Ctrl Pts',(-44.2583166685835,-55.2656490138239,
-38.612301023075));
#268855=CARTESIAN_POINT('Ctrl Pts',(-44.3705972700495,-55.2524997368729,
-38.6302900391873));
#268856=CARTESIAN_POINT('Ctrl Pts',(-44.446056048267,-55.2474029004138,
-38.6430428201589));
#268857=CARTESIAN_POINT('Ctrl Pts',(-44.5218128020516,-55.2441636366351,
-38.65617756452));
#268858=CARTESIAN_POINT('Ctrl Pts',(-44.5599089424743,-55.2434808562086,
-38.6629497802385));
#268859=CARTESIAN_POINT('Ctrl Pts',(-44.6354869543582,-55.2439911084578,
-38.6767130108817));
#268860=CARTESIAN_POINT('Ctrl Pts',(-44.6731456892459,-55.2451740103824,
-38.6837342374529));
#268861=CARTESIAN_POINT('Ctrl Pts',(-44.7481014788608,-55.2493620066237,
-38.6980304684339));
#268862=CARTESIAN_POINT('Ctrl Pts',(-44.860046548974,-55.2583760573225,
-38.7198650218829));
#268863=CARTESIAN_POINT('Ctrl Pts',(-45.0073845433675,-55.2811507310277,
-38.7505067688753));
#268864=CARTESIAN_POINT('Ctrl Pts',(-45.1528189888476,-55.3146135839333,
-38.7826550300594));
#268865=CARTESIAN_POINT('Ctrl Pts',(-45.2248832056965,-55.3349380951144,
-38.7992310848652));
#268866=CARTESIAN_POINT('Ctrl Pts',(-45.2966462681613,-55.3570913336823,
-38.8160672125853));
#268867=CARTESIAN_POINT('Ctrl Pts',(-45.3323638946335,-55.3690863290504,
-38.8246135819642));
#268868=CARTESIAN_POINT('Ctrl Pts',(-45.4027951436545,-55.3946744461232,
-38.841798196801));
#268869=CARTESIAN_POINT('Ctrl Pts',(-45.4376370321487,-55.4083060218429,
-38.85046633842));
#268870=CARTESIAN_POINT('Ctrl Pts',(-45.5409345111852,-55.4516493275196,
-38.8766665754573));
#268871=CARTESIAN_POINT('Ctrl Pts',(-45.6082182891413,-55.4838201174091,
-38.8944064774514));
#268872=CARTESIAN_POINT('Ctrl Pts',(-45.7067749877369,-55.5369855856676,
-38.9214216121435));
#268873=CARTESIAN_POINT('Ctrl Pts',(-45.7392219877795,-55.5555212114618,
-38.9304915704334));
#268874=CARTESIAN_POINT('Ctrl Pts',(-45.8033556832395,-55.5942722159849,
-38.9487787872477));
#268875=CARTESIAN_POINT('Ctrl Pts',(-45.8348443691401,-55.6143675312756,
-38.9579395118015));
#268876=CARTESIAN_POINT('Ctrl Pts',(-45.9274099842789,-55.6766589025306,
-38.9854159162723));
#268877=CARTESIAN_POINT('Ctrl Pts',(-45.9867610865919,-55.7209353156014,
-39.0037703637879));
#268878=CARTESIAN_POINT('Ctrl Pts',(-46.1007337830098,-55.8148102393793,
-39.0405190865864));
#268879=CARTESIAN_POINT('Ctrl Pts',(-46.1826971388658,-55.889219933262,
-39.0681181728269));
#268880=CARTESIAN_POINT('Ctrl Pts',(-46.259356574729,-55.9696687352924,
-39.0957737179551));
#268881=CARTESIAN_POINT('Ctrl Pts',(-46.309266807939,-56.024663053365,-39.1142236413887));
#268882=CARTESIAN_POINT('Ctrl Pts',(-46.3336138177017,-56.0528284109483,
-39.1234510495426));
#268883=CARTESIAN_POINT('Ctrl Pts',(-46.3692509284248,-56.0961546965833,
-39.1373141736981));
#268884=CARTESIAN_POINT('Ctrl Pts',(-46.3809719555493,-56.1107655250657,
-39.14193505412));
#268885=CARTESIAN_POINT('Ctrl Pts',(-46.4039850968433,-56.1401806715041,
-39.1511314768264));
#268886=CARTESIAN_POINT('Ctrl Pts',(-46.4153001903629,-56.1550126624776,
-39.1557159133813));
#268887=CARTESIAN_POINT('Ctrl Pts',(-46.4486370096885,-56.1998310060263,
-39.1694131182659));
#268888=CARTESIAN_POINT('Ctrl Pts',(-46.4700835091466,-56.2301795317326,
-39.1784826054425));
#268889=CARTESIAN_POINT('Ctrl Pts',(-46.532071913686,-56.3225583984772,
-39.2054898733524));
#268890=CARTESIAN_POINT('Ctrl Pts',(-46.5894197348374,-56.4176636744323,
-39.23211607576));
#268891=CARTESIAN_POINT('Ctrl Pts',(-46.6566074362748,-56.5498680842415,
-39.2668544229849));
#268892=CARTESIAN_POINT('Ctrl Pts',(-46.6870820302515,-56.617790568625,
-39.2839693714534));
#268893=CARTESIAN_POINT('Ctrl Pts',(-46.7159729830272,-56.6866360545619,
-39.3009558869148));
#268894=CARTESIAN_POINT('Ctrl Pts',(-46.7296188023799,-56.7214992889704,
-39.3093799218186));
#268895=CARTESIAN_POINT('Ctrl Pts',(-46.7553216997643,-56.7922546384013,
-39.3261176641085));
#268896=CARTESIAN_POINT('Ctrl Pts',(-46.7672996943011,-56.8279354881579,
-39.3343809787628));
#268897=CARTESIAN_POINT('Ctrl Pts',(-46.8004530502947,-56.9353633959568,
-39.358737163018));
#268898=CARTESIAN_POINT('Ctrl Pts',(-46.8189795501832,-57.0077635587999,
-39.3744658121213));
#268899=CARTESIAN_POINT('Ctrl Pts',(-46.848916211803,-57.1540080946302,
-39.4048998290393));
#268900=CARTESIAN_POINT('Ctrl Pts',(-46.866048617508,-57.2647966217996,
-39.4269646939479));
#268901=CARTESIAN_POINT('Ctrl Pts',(-46.875074749658,-57.3772756893033,
-39.4478819384746));
#268902=CARTESIAN_POINT('Ctrl Pts',(-46.8792542953452,-57.4526370309597,
-39.4615663943076));
#268903=CARTESIAN_POINT('Ctrl Pts',(-46.8804258736835,-57.4905390832845,
-39.4682843608713));
#268904=CARTESIAN_POINT('Ctrl Pts',(-46.8808837743635,-57.566610437341,
-39.4814341960201));
#268905=CARTESIAN_POINT('Ctrl Pts',(-46.8801708637706,-57.604491394965,
-39.4878166677226));
#268906=CARTESIAN_POINT('Ctrl Pts',(-46.8768913879562,-57.6800597985945,
-39.5002231148134));
#268907=CARTESIAN_POINT('Ctrl Pts',(-46.8691896925243,-57.7930657109158,
-39.5182849936093));
#268908=CARTESIAN_POINT('Ctrl Pts',(-46.8479069711518,-57.9423669591112,
-39.540205996752));
#268909=CARTESIAN_POINT('Ctrl Pts',(-46.8236459543104,-58.053306681129,
-39.5550278422771));
#268910=CARTESIAN_POINT('Ctrl Pts',(-46.8055990109883,-58.1270324939452,
-39.5645447403379));
#268911=CARTESIAN_POINT('Ctrl Pts',(-46.7956339676918,-58.1637938532181,
-39.5691227921436));
#268912=CARTESIAN_POINT('Ctrl Pts',(-46.7738161327052,-58.2370162077019,
-39.5779016468881));
#268913=CARTESIAN_POINT('Ctrl Pts',(-46.7619036278491,-58.2736352268715,
-39.5821192203466));
#268914=CARTESIAN_POINT('Ctrl Pts',(-46.7364059718256,-58.3458255995332,
-39.5900871854462));
#268915=CARTESIAN_POINT('Ctrl Pts',(-46.7091836493705,-58.4171862986019,
-39.5976163356366));
#268916=CARTESIAN_POINT('Ctrl Pts',(-46.663274408039,-58.5216699086648,
-39.6076014242402));
#268917=CARTESIAN_POINT('Ctrl Pts',(-46.6123207377325,-58.6236436013082,
-39.616293729045));
#268918=CARTESIAN_POINT('Ctrl Pts',(-46.5563244858032,-58.7230996041114,
-39.6236943138341));
#268919=CARTESIAN_POINT('Ctrl Pts',(-46.515607032986,-58.7877140896312,
-39.6277619492082));
#268920=CARTESIAN_POINT('Ctrl Pts',(-46.4731710833873,-58.8514710047945,
-39.6313905635194));
#268921=CARTESIAN_POINT('Ctrl Pts',(-46.4511086137465,-58.8829006319494,
-39.6329844599904));
#268922=CARTESIAN_POINT('Ctrl Pts',(-46.4051673201274,-58.9449633016888,
-39.6357273485653));
#268923=CARTESIAN_POINT('Ctrl Pts',(-46.381447994276,-58.975377588932,-39.6368662598532));
#268924=CARTESIAN_POINT('Ctrl Pts',(-46.3084068909562,-59.0643493136614,
-39.6395761233691));
#268925=CARTESIAN_POINT('Ctrl Pts',(-46.2570407846102,-59.1209150453974,
-39.6404603784325));
#268926=CARTESIAN_POINT('Ctrl Pts',(-46.1491379755941,-59.228544463199,
-39.6404138814247));
#268927=CARTESIAN_POINT('Ctrl Pts',(-46.0925836555155,-59.2796343044913,
-39.6394845811684));
#268928=CARTESIAN_POINT('Ctrl Pts',(-46.0038529437629,-59.3521266125547,
-39.6367223387528));
#268929=CARTESIAN_POINT('Ctrl Pts',(-45.9736068078661,-59.3756113554055,
-39.6355721163029));
#268930=CARTESIAN_POINT('Ctrl Pts',(-45.9272656961273,-59.4097723546528,
-39.6334997725088));
#268931=CARTESIAN_POINT('Ctrl Pts',(-45.9116419215573,-59.4209912820171,
-39.6327502808957));
#268932=CARTESIAN_POINT('Ctrl Pts',(-45.8800804794677,-59.4430610802669,
-39.6311351339295));
#268933=CARTESIAN_POINT('Ctrl Pts',(-45.8321587971618,-59.4756823489919,
-39.628531354857));
#268934=CARTESIAN_POINT('Ctrl Pts',(-45.7834097108732,-59.5062438963941,
-39.6254355071979));
#268935=CARTESIAN_POINT('Ctrl Pts',(-45.717633106262,-59.5452481912826,
-39.6208773262667));
#268936=CARTESIAN_POINT('Ctrl Pts',(-45.6178307490054,-59.601113548897,
-39.6133952897297));
#268937=CARTESIAN_POINT('Ctrl Pts',(-45.4802897643185,-59.6652183443042,
-39.6008811885904));
#268938=CARTESIAN_POINT('Ctrl Pts',(-45.3738098009101,-59.7055766782111,
-39.5896017905935));
#268939=CARTESIAN_POINT('Ctrl Pts',(-45.3020778813705,-59.7307512119865,
-39.5816566825671));
#268940=CARTESIAN_POINT('Ctrl Pts',(-45.2658207311094,-59.7424779859237,
-39.5774690651077));
#268941=CARTESIAN_POINT('Ctrl Pts',(-45.1926264675053,-59.7641596016776,
-39.5686715125846));
#268942=CARTESIAN_POINT('Ctrl Pts',(-45.1555073907618,-59.7741562512684,
-39.5640376159893));
#268943=CARTESIAN_POINT('Ctrl Pts',(-45.0441315765335,-59.8011904590316,
-39.5496210468413));
#268944=CARTESIAN_POINT('Ctrl Pts',(-44.9324484012679,-59.8224577850013,
-39.5341534065747));
#268945=CARTESIAN_POINT('Ctrl Pts',(-44.8203079610257,-59.8353953605365,
-39.5171556909205));
#268946=CARTESIAN_POINT('Ctrl Pts',(-44.7080184564226,-59.8455760612675,
-39.4996502778008));
#268947=CARTESIAN_POINT('Ctrl Pts',(-44.6329372249224,-59.8486931621852,
-39.4873001861445));
#268948=CARTESIAN_POINT('Ctrl Pts',(-44.5200834441659,-59.8478515133141,
-39.4677634802869));
#268949=CARTESIAN_POINT('Ctrl Pts',(-44.4823810871712,-59.8466449718289,
-39.4610736497974));
#268950=CARTESIAN_POINT('Ctrl Pts',(-44.4258051079382,-59.8434394706745,
-39.4507883432074));
#268951=CARTESIAN_POINT('Ctrl Pts',(-44.4069254589855,-59.8421361346926,
-39.4473147915973));
#268952=CARTESIAN_POINT('Ctrl Pts',(-44.3691376542581,-59.8390581625153,
-39.4402793331445));
#268953=CARTESIAN_POINT('Ctrl Pts',(-44.3502459350849,-59.8372838734483,
-39.4367203104461));
#268954=CARTESIAN_POINT('Ctrl Pts',(-44.2562487381671,-59.8272835659938,
-39.4188041728073));
#268955=CARTESIAN_POINT('Ctrl Pts',(-44.1080045765469,-59.8040393501646,
-39.3892226636159));
#268956=CARTESIAN_POINT('Ctrl Pts',(-43.9639303529155,-59.7668593120831,
-39.3578670379715));
#268957=CARTESIAN_POINT('Ctrl Pts',(-43.8219159040518,-59.7227861654643,
-39.3256251231267));
#268958=CARTESIAN_POINT('Ctrl Pts',(-43.7519290534068,-59.6972943066161,
-39.3090578287531));
#268959=CARTESIAN_POINT('Ctrl Pts',(-43.665783177736,-59.6610675807531,
-39.2877890488175));
#268960=CARTESIAN_POINT('Ctrl Pts',(-43.6486106666635,-59.653596197985,
-39.2835041280971));
#268961=CARTESIAN_POINT('Ctrl Pts',(-43.6144193015916,-59.6382222359849,
-39.2748825183767));
#268962=CARTESIAN_POINT('Ctrl Pts',(-43.597366582891,-59.6303022352814,
-39.2705368924251));
#268963=CARTESIAN_POINT('Ctrl Pts',(-43.5465994182959,-59.605961903298,
-39.2574616452183));
#268964=CARTESIAN_POINT('Ctrl Pts',(-43.513329300663,-59.588993111175,-39.2487085268073));
#268965=CARTESIAN_POINT('Ctrl Pts',(-43.4805771074156,-59.5712767529309,
-39.2399080357013));
#268966=CARTESIAN_POINT('Ctrl Pts',(-43.8341420587998,-57.9817357678076,
-41.1268248734572));
#268967=CARTESIAN_POINT('Ctrl Pts',(-43.8090823387197,-57.9680163597508,
-41.1092238912453));
#268968=CARTESIAN_POINT('Ctrl Pts',(-43.7605654269547,-57.9383371077444,
-41.0736746770147));
#268969=CARTESIAN_POINT('Ctrl Pts',(-43.6924895655639,-57.8872515755908,
-41.019320019256));
#268970=CARTESIAN_POINT('Ctrl Pts',(-43.6502497090231,-57.8487916199066,
-40.9823828883729));
#268971=CARTESIAN_POINT('Ctrl Pts',(-43.6096433745973,-57.8080652293815,
-40.945090157748));
#268972=CARTESIAN_POINT('Ctrl Pts',(-43.5713160673933,-57.7657212262301,
-40.9080353139296));
#268973=CARTESIAN_POINT('Ctrl Pts',(-43.5288984657655,-57.7088609123343,
-40.8622751058818));
#268974=CARTESIAN_POINT('Ctrl Pts',(-43.4982484100127,-57.6610280687967,
-40.826006689079));
#268975=CARTESIAN_POINT('Ctrl Pts',(-43.4769169762936,-57.6239677344727,
-40.798976453902));
#268976=CARTESIAN_POINT('Ctrl Pts',(-43.4638199758968,-57.5984660781933,
-40.7810781735695));
#268977=CARTESIAN_POINT('Ctrl Pts',(-43.4512904535732,-57.5725430453748,
-40.7632325534464));
#268978=CARTESIAN_POINT('Ctrl Pts',(-43.4453582046716,-57.5594707895743,
-40.7544050886758));
#268979=CARTESIAN_POINT('Ctrl Pts',(-43.4285595200757,-57.5199648485381,
-40.7282304644163));
#268980=CARTESIAN_POINT('Ctrl Pts',(-43.4088016745783,-57.4664867157472,
-40.6941268792613));
#268981=CARTESIAN_POINT('Ctrl Pts',(-43.3942530508608,-57.4114223976644,
-40.6616070010832));
#268982=CARTESIAN_POINT('Ctrl Pts',(-43.3853242538269,-57.3695231591805,
-40.6378273627645));
#268983=CARTESIAN_POINT('Ctrl Pts',(-43.3826786150667,-57.3554536366825,
-40.630001230023));
#268984=CARTESIAN_POINT('Ctrl Pts',(-43.378062215599,-57.3271160344971,
-40.6145607014775));
#268985=CARTESIAN_POINT('Ctrl Pts',(-43.3760891270041,-57.3128275119467,
-40.60693561976));
#268986=CARTESIAN_POINT('Ctrl Pts',(-43.3728422231051,-57.2841093232557,
-40.5919365051523));
#268987=CARTESIAN_POINT('Ctrl Pts',(-43.3715781643254,-57.2697777029377,
-40.5846130830795));
#268988=CARTESIAN_POINT('Ctrl Pts',(-43.3697526802575,-57.2411194243864,
-40.5702888754578));
#268989=CARTESIAN_POINT('Ctrl Pts',(-43.3680717796799,-57.1981642741791,
-40.5492997469169));
#268990=CARTESIAN_POINT('Ctrl Pts',(-43.3700185838812,-57.1410182421193,
-40.5232909177883));
#268991=CARTESIAN_POINT('Ctrl Pts',(-43.3746384661022,-57.0982543712987,
-40.505286899195));
#268992=CARTESIAN_POINT('Ctrl Pts',(-43.3784319419536,-57.0697666559562,
-40.4936247912381));
#268993=CARTESIAN_POINT('Ctrl Pts',(-43.3806866868643,-57.0555278483981,
-40.4879619013523));
#268994=CARTESIAN_POINT('Ctrl Pts',(-43.3859186984709,-57.0270949764048,
-40.476993052777));
#268995=CARTESIAN_POINT('Ctrl Pts',(-43.3889115442249,-57.0128413374093,
-40.4716662621118));
#268996=CARTESIAN_POINT('Ctrl Pts',(-43.3955695423488,-56.984668670318,
-40.4614841416371));
#268997=CARTESIAN_POINT('Ctrl Pts',(-43.4029115329907,-56.9567427536229,
-40.4517375031029));
#268998=CARTESIAN_POINT('Ctrl Pts',(-43.4159439893498,-56.915628788467,
-40.4384286813559));
#268999=CARTESIAN_POINT('Ctrl Pts',(-43.4309850942545,-56.8752725380991,
-40.4264211055283));
#269000=CARTESIAN_POINT('Ctrl Pts',(-43.4480370013178,-56.8356780486645,
-40.4157207514563));
#269001=CARTESIAN_POINT('Ctrl Pts',(-43.4607570961379,-56.8097932355363,
-40.409467745062));
#269002=CARTESIAN_POINT('Ctrl Pts',(-43.4741642201056,-56.7841683331057,
-40.4036630043601));
#269003=CARTESIAN_POINT('Ctrl Pts',(-43.4812071336048,-56.7714928975767,
-40.4009861443346));
#269004=CARTESIAN_POINT('Ctrl Pts',(-43.4960130774609,-56.7463797512019,
-40.3960865778375));
#269005=CARTESIAN_POINT('Ctrl Pts',(-43.5037198572985,-56.7340380787953,
-40.3938827877695));
#269006=CARTESIAN_POINT('Ctrl Pts',(-43.527657505214,-56.6977883833479,
-40.3880276966888));
#269007=CARTESIAN_POINT('Ctrl Pts',(-43.5447483375558,-56.6745564757614,
-40.3851058766842));
#269008=CARTESIAN_POINT('Ctrl Pts',(-43.5811328114983,-56.629979998045,
-40.3812078888591));
#269009=CARTESIAN_POINT('Ctrl Pts',(-43.6004351631962,-56.6086219171049,
-40.3802294367552));
#269010=CARTESIAN_POINT('Ctrl Pts',(-43.6310475296952,-56.578014570072,
-40.3802318237287));
#269011=CARTESIAN_POINT('Ctrl Pts',(-43.6415402048873,-56.5680413281089,
-40.3804790384992));
#269012=CARTESIAN_POINT('Ctrl Pts',(-43.6576911458811,-56.5534539772523,
-40.3812231446347));
#269013=CARTESIAN_POINT('Ctrl Pts',(-43.6631494628181,-56.5486488515781,
-40.3815339900979));
#269014=CARTESIAN_POINT('Ctrl Pts',(-43.6742063152013,-56.5391628964206,
-40.3822815284329));
#269015=CARTESIAN_POINT('Ctrl Pts',(-43.6798092119243,-56.534479009001,
-40.3827188413654));
#269016=CARTESIAN_POINT('Ctrl Pts',(-43.6967370434146,-56.5206915949946,
-40.3842131357726));
#269017=CARTESIAN_POINT('Ctrl Pts',(-43.7196778600618,-56.5029622466235,
-40.386692708542));
#269018=CARTESIAN_POINT('Ctrl Pts',(-43.7670264629127,-56.4700551612604,
-40.3935618621563));
#269019=CARTESIAN_POINT('Ctrl Pts',(-43.8165352419067,-56.4409186299576,
-40.4032471370382));
#269020=CARTESIAN_POINT('Ctrl Pts',(-43.8552784957563,-56.4218759376155,
-40.4126045758866));
#269021=CARTESIAN_POINT('Ctrl Pts',(-43.8814691350842,-56.4098116142502,
-40.4193119877837));
#269022=CARTESIAN_POINT('Ctrl Pts',(-43.8947490665381,-56.4040935548973,
-40.4229014011429));
#269023=CARTESIAN_POINT('Ctrl Pts',(-43.9216608718689,-56.3933018151258,
-40.430550144354));
#269024=CARTESIAN_POINT('Ctrl Pts',(-43.9353412421961,-56.3882139347518,
-40.434625723994));
#269025=CARTESIAN_POINT('Ctrl Pts',(-43.9627318697344,-56.3788058930362,
-40.4431514805252));
#269026=CARTESIAN_POINT('Ctrl Pts',(-43.9765011076412,-56.3744602994329,
-40.4476175822086));
#269027=CARTESIAN_POINT('Ctrl Pts',(-44.0179764085085,-56.3624961934912,
-40.4615970784657));
#269028=CARTESIAN_POINT('Ctrl Pts',(-44.0598195105868,-56.3526585058303,
-40.4767455237411));
#269029=CARTESIAN_POINT('Ctrl Pts',(-44.1163310625808,-56.3437038269143,
-40.4992178608308));
#269030=CARTESIAN_POINT('Ctrl Pts',(-44.1590753545772,-56.3390714325247,
-40.5172068769433));
#269031=CARTESIAN_POINT('Ctrl Pts',(-44.1878153726385,-56.337382052278,
-40.5299596579145));
#269032=CARTESIAN_POINT('Ctrl Pts',(-44.2166756293141,-56.3364007867548,
-40.5430944022758));
#269033=CARTESIAN_POINT('Ctrl Pts',(-44.2311921171808,-56.3362675100036,
-40.5498666179945));
#269034=CARTESIAN_POINT('Ctrl Pts',(-44.2599977007373,-56.3367129587916,
-40.5636298486377));
#269035=CARTESIAN_POINT('Ctrl Pts',(-44.2743541649932,-56.3372884158027,
-40.5706510752088));
#269036=CARTESIAN_POINT('Ctrl Pts',(-44.3029357424357,-56.3391317429585,
-40.5849473061899));
#269037=CARTESIAN_POINT('Ctrl Pts',(-44.3456316213443,-56.3429350642169,
-40.6067818596389));
#269038=CARTESIAN_POINT('Ctrl Pts',(-44.4018650235691,-56.3520939287388,
-40.6374236066311));
#269039=CARTESIAN_POINT('Ctrl Pts',(-44.4574103376146,-56.3653147883305,
-40.6695718678152));
#269040=CARTESIAN_POINT('Ctrl Pts',(-44.4849466005937,-56.3732907222196,
-40.686147922621));
#269041=CARTESIAN_POINT('Ctrl Pts',(-44.512374392093,-56.3819617528141,
-40.7029840503412));
#269042=CARTESIAN_POINT('Ctrl Pts',(-44.5260289861432,-56.3866462995878,
-40.7115304197201));
#269043=CARTESIAN_POINT('Ctrl Pts',(-44.5529609776699,-56.3966203919845,
-40.7287150345567));
#269044=CARTESIAN_POINT('Ctrl Pts',(-44.5662873943758,-56.4019250012471,
-40.737383176176));
#269045=CARTESIAN_POINT('Ctrl Pts',(-44.6058068395674,-56.4187668411382,
-40.7635834132132));
#269046=CARTESIAN_POINT('Ctrl Pts',(-44.6315615859976,-56.4312362585519,
-40.7813233152079));
#269047=CARTESIAN_POINT('Ctrl Pts',(-44.6693071486035,-56.4518014713652,
-40.8083384498991));
#269048=CARTESIAN_POINT('Ctrl Pts',(-44.6817372625133,-56.458965010373,
-40.8174084081892));
#269049=CARTESIAN_POINT('Ctrl Pts',(-44.7063132537473,-56.473929075182,
-40.8356956250034));
#269050=CARTESIAN_POINT('Ctrl Pts',(-44.7183832523531,-56.4816832398284,
-40.8448563495594));
#269051=CARTESIAN_POINT('Ctrl Pts',(-44.7538754102704,-56.505703003501,
-40.8723327540241));
#269052=CARTESIAN_POINT('Ctrl Pts',(-44.7766465418209,-56.5227549736834,
-40.8906872015444));
#269053=CARTESIAN_POINT('Ctrl Pts',(-44.8204030914552,-56.5588699415109,
-40.9274359243417));
#269054=CARTESIAN_POINT('Ctrl Pts',(-44.851893062885,-56.5874690797881,
-40.9550350105826));
#269055=CARTESIAN_POINT('Ctrl Pts',(-44.8813802932551,-56.6183507815631,
-40.982690555711));
#269056=CARTESIAN_POINT('Ctrl Pts',(-44.9005867815582,-56.6394533348067,
-41.0011404791447));
#269057=CARTESIAN_POINT('Ctrl Pts',(-44.9099603095753,-56.6502571213647,
-41.0103678872986));
#269058=CARTESIAN_POINT('Ctrl Pts',(-44.9236872082217,-56.6668706184025,
-41.0242310114538));
#269059=CARTESIAN_POINT('Ctrl Pts',(-44.9282031316495,-56.6724722064122,
-41.0288518918758));
#269060=CARTESIAN_POINT('Ctrl Pts',(-44.9370720489983,-56.6837477093971,
-41.038048314582));
#269061=CARTESIAN_POINT('Ctrl Pts',(-44.9414338933841,-56.6894322363092,
-41.0426327511372));
#269062=CARTESIAN_POINT('Ctrl Pts',(-44.9542884395491,-56.7066066663578,
-41.0563299560217));
#269063=CARTESIAN_POINT('Ctrl Pts',(-44.9625629539304,-56.7182326826763,
-41.0653994431984));
#269064=CARTESIAN_POINT('Ctrl Pts',(-44.9864941991718,-56.7536111473724,
-41.0924067111081));
#269065=CARTESIAN_POINT('Ctrl Pts',(-45.0086645271567,-56.7900134244028,
-41.1190329135161));
#269066=CARTESIAN_POINT('Ctrl Pts',(-45.034704630644,-56.8405768845403,
-41.1537712607408));
#269067=CARTESIAN_POINT('Ctrl Pts',(-45.0465408860903,-56.8665423758261,
-41.1708862092094));
#269068=CARTESIAN_POINT('Ctrl Pts',(-45.0577761134165,-56.8928546179869,
-41.1878727246706));
#269069=CARTESIAN_POINT('Ctrl Pts',(-45.0630901582258,-56.906176087846,
-41.1962967595746));
#269070=CARTESIAN_POINT('Ctrl Pts',(-45.0731156002939,-56.9332061371524,
-41.2130345018643));
#269071=CARTESIAN_POINT('Ctrl Pts',(-45.0777961712447,-56.9468340019015,
-41.2212978165198));
#269072=CARTESIAN_POINT('Ctrl Pts',(-45.0907786540592,-56.9878560258786,
-41.2456540007716));
#269073=CARTESIAN_POINT('Ctrl Pts',(-45.0980724298404,-57.0154910056487,
-41.2613826498774));
#269074=CARTESIAN_POINT('Ctrl Pts',(-45.1099506000897,-57.0712899900431,
-41.2918166667949));
#269075=CARTESIAN_POINT('Ctrl Pts',(-45.1168338059478,-57.11354441615,-41.3138815317038));
#269076=CARTESIAN_POINT('Ctrl Pts',(-45.1206309792415,-57.1564190282566,
-41.3347987762303));
#269077=CARTESIAN_POINT('Ctrl Pts',(-45.1224627479043,-57.1851396939165,
-41.3484832320635));
#269078=CARTESIAN_POINT('Ctrl Pts',(-45.1230291819396,-57.199581674993,
-41.3552011986272));
#269079=CARTESIAN_POINT('Ctrl Pts',(-45.1234439819388,-57.2285619504273,
-41.3683510337761));
#269080=CARTESIAN_POINT('Ctrl Pts',(-45.1232917301137,-57.2429904040975,
-41.3747335054784));
#269081=CARTESIAN_POINT('Ctrl Pts',(-45.122279779691,-57.2717682086368,
-41.3871399525693));
#269082=CARTESIAN_POINT('Ctrl Pts',(-45.1196997436484,-57.3147947598186,
-41.4052018313649));
#269083=CARTESIAN_POINT('Ctrl Pts',(-45.1120557453653,-57.3716084168758,
-41.4271228345082));
#269084=CARTESIAN_POINT('Ctrl Pts',(-45.1031553338884,-57.4137999065974,
-41.4419446800329));
#269085=CARTESIAN_POINT('Ctrl Pts',(-45.09650693546,-57.4418330021969,-41.4514615780937));
#269086=CARTESIAN_POINT('Ctrl Pts',(-45.092823442876,-57.4558081403435,
-41.4560396298995));
#269087=CARTESIAN_POINT('Ctrl Pts',(-45.08473584999,-57.4836385233421,-41.464818484644));
#269088=CARTESIAN_POINT('Ctrl Pts',(-45.0803094818206,-57.4975537933777,
-41.4690360581021));
#269089=CARTESIAN_POINT('Ctrl Pts',(-45.0708158371377,-57.5249803724867,
-41.4770040232021));
#269090=CARTESIAN_POINT('Ctrl Pts',(-45.060662137239,-57.5520858826269,
-41.4845331733926));
#269091=CARTESIAN_POINT('Ctrl Pts',(-45.0434887903859,-57.591755117417,
-41.4945182619959));
#269092=CARTESIAN_POINT('Ctrl Pts',(-45.0243848727922,-57.6304534586566,
-41.5032105668009));
#269093=CARTESIAN_POINT('Ctrl Pts',(-45.0033512023575,-57.6681778817651,
-41.51061115159));
#269094=CARTESIAN_POINT('Ctrl Pts',(-44.9880328234845,-57.692673879575,
-41.5146787869643));
#269095=CARTESIAN_POINT('Ctrl Pts',(-44.9720568870916,-57.7168380825906,
-41.5183074012753));
#269096=CARTESIAN_POINT('Ctrl Pts',(-44.9637457009402,-57.7287466936453,
-41.5199012977462));
#269097=CARTESIAN_POINT('Ctrl Pts',(-44.9464287138105,-57.7522550306847,
-41.5226441863212));
#269098=CARTESIAN_POINT('Ctrl Pts',(-44.9374830238235,-57.7637718882179,
-41.5237830976086));
#269099=CARTESIAN_POINT('Ctrl Pts',(-44.9099214446927,-57.7974515399035,
-41.5264929611258));
#269100=CARTESIAN_POINT('Ctrl Pts',(-44.8905204729439,-57.8188493934961,
-41.5273772161885));
#269101=CARTESIAN_POINT('Ctrl Pts',(-44.8497318000032,-57.8595330722204,
-41.5273307191807));
#269102=CARTESIAN_POINT('Ctrl Pts',(-44.8283374647208,-57.878828810327,
-41.5264014189239));
#269103=CARTESIAN_POINT('Ctrl Pts',(-44.7947479986672,-57.9061820008563,
-41.5236391765087));
#269104=CARTESIAN_POINT('Ctrl Pts',(-44.7832945060713,-57.9150388128137,
-41.5224889540588));
#269105=CARTESIAN_POINT('Ctrl Pts',(-44.7657408175914,-57.9279147771907,
-41.5204166102647));
#269106=CARTESIAN_POINT('Ctrl Pts',(-44.7598217545323,-57.9321421746299,
-41.5196671186517));
#269107=CARTESIAN_POINT('Ctrl Pts',(-44.7478629508254,-57.9404557426351,
-41.5180519716851));
#269108=CARTESIAN_POINT('Ctrl Pts',(-44.7297025277655,-57.9527400844071,
-41.5154481926132));
#269109=CARTESIAN_POINT('Ctrl Pts',(-44.711220794734,-57.9642369190977,
-41.5123523449538));
#269110=CARTESIAN_POINT('Ctrl Pts',(-44.6862770262529,-57.9788987855805,
-41.5077941640223));
#269111=CARTESIAN_POINT('Ctrl Pts',(-44.6484202704456,-57.9998814948776,
-41.5003121274858));
#269112=CARTESIAN_POINT('Ctrl Pts',(-44.5962108390282,-58.0238874022289,
-41.4877980263462));
#269113=CARTESIAN_POINT('Ctrl Pts',(-44.5557649369164,-58.0389385823793,
-41.4765186283493));
#269114=CARTESIAN_POINT('Ctrl Pts',(-44.5285120653069,-58.048310487242,
-41.4685735203231));
#269115=CARTESIAN_POINT('Ctrl Pts',(-44.5147341086114,-58.0526671867402,
-41.4643859028639));
#269116=CARTESIAN_POINT('Ctrl Pts',(-44.4869140318333,-58.0607029371288,
-41.4555883503401));
#269117=CARTESIAN_POINT('Ctrl Pts',(-44.4728027150897,-58.0643973546439,
-41.4509544537452));
#269118=CARTESIAN_POINT('Ctrl Pts',(-44.4304531283686,-58.0743536715507,
-41.4365378845966));
#269119=CARTESIAN_POINT('Ctrl Pts',(-44.3879697631396,-58.0821103913619,
-41.4210702443308));
#269120=CARTESIAN_POINT('Ctrl Pts',(-44.3452880889881,-58.0866896268435,
-41.4040725286766));
#269121=CARTESIAN_POINT('Ctrl Pts',(-44.3025416355467,-58.090217180745,
-41.3865671155567));
#269122=CARTESIAN_POINT('Ctrl Pts',(-44.2739489581488,-58.0911687787978,
-41.3742170239002));
#269123=CARTESIAN_POINT('Ctrl Pts',(-44.2309555122234,-58.090491506171,
-41.3546803180427));
#269124=CARTESIAN_POINT('Ctrl Pts',(-44.2165895018292,-58.0899123697243,
-41.347990487553));
#269125=CARTESIAN_POINT('Ctrl Pts',(-44.1950278537333,-58.0885113544661,
-41.337705180963));
#269126=CARTESIAN_POINT('Ctrl Pts',(-44.1878319550126,-58.0879547296283,
-41.3342316293533));
#269127=CARTESIAN_POINT('Ctrl Pts',(-44.1734279164018,-58.0866616594573,
-41.3271961709002));
#269128=CARTESIAN_POINT('Ctrl Pts',(-44.1662260389348,-58.0859253983809,
-41.3236371482021));
#269129=CARTESIAN_POINT('Ctrl Pts',(-44.130389101081,-58.0818150523559,
-41.3057210105631));
#269130=CARTESIAN_POINT('Ctrl Pts',(-44.073848260417,-58.0724828543971,
-41.2761395013722));
#269131=CARTESIAN_POINT('Ctrl Pts',(-44.0188545174212,-58.0578491440998,
-41.2447838757269));
#269132=CARTESIAN_POINT('Ctrl Pts',(-43.9646246641704,-58.0405931079736,
-41.2125419608827));
#269133=CARTESIAN_POINT('Ctrl Pts',(-43.9378880325505,-58.0306505669816,
-41.1959746665064));
#269134=CARTESIAN_POINT('Ctrl Pts',(-43.9049634769563,-58.0165631445999,
-41.174705886574));
#269135=CARTESIAN_POINT('Ctrl Pts',(-43.898399460067,-58.0136596367661,
-41.1704209658528));
#269136=CARTESIAN_POINT('Ctrl Pts',(-43.8853286348063,-58.0076886655405,
-41.1617993561325));
#269137=CARTESIAN_POINT('Ctrl Pts',(-43.8788088737381,-58.0046144513738,
-41.157453730181));
#269138=CARTESIAN_POINT('Ctrl Pts',(-43.8593967360427,-57.9951717320096,
-41.1443784829743));
#269139=CARTESIAN_POINT('Ctrl Pts',(-43.8466719188398,-57.9885954718361,
-41.1356253645631));
#269140=CARTESIAN_POINT('Ctrl Pts',(-43.8341420587998,-57.9817357678076,
-41.1268248734572));
#269141=CARTESIAN_POINT('Ctrl Pts',(-46.6981266849492,30.7091523375488,
-39.2904704603133));
#269142=CARTESIAN_POINT('Ctrl Pts',(-46.6835475486277,30.6747783378881,
-39.2819613777041));
#269143=CARTESIAN_POINT('Ctrl Pts',(-46.6681814960651,30.6408774263401,
-39.2733909118473));
#269144=CARTESIAN_POINT('Ctrl Pts',(-46.6359019229579,30.57400615396,-39.2561284882363));
#269145=CARTESIAN_POINT('Ctrl Pts',(-46.618988316466,30.5410358444554,-39.2474365250187));
#269146=CARTESIAN_POINT('Ctrl Pts',(-46.5659489383047,30.443507428437,-39.2211791249421));
#269147=CARTESIAN_POINT('Ctrl Pts',(-46.5275294393937,30.3803289376591,
-39.2034325264408));
#269148=CARTESIAN_POINT('Ctrl Pts',(-46.4653031952286,30.2883271671429,
-39.1764461222039));
#269149=CARTESIAN_POINT('Ctrl Pts',(-46.4437937583117,30.2581216171786,
-39.1673894861782));
#269150=CARTESIAN_POINT('Ctrl Pts',(-46.3992224148768,30.1986447451181,
-39.1491520227249));
#269151=CARTESIAN_POINT('Ctrl Pts',(-46.3761748773305,30.1693908446446,
-39.1399767764946));
#269152=CARTESIAN_POINT('Ctrl Pts',(-46.3284414024809,30.1117648114072,
-39.1214771434543));
#269153=CARTESIAN_POINT('Ctrl Pts',(-46.3038983378397,30.083571828401,-39.112209259666));
#269154=CARTESIAN_POINT('Ctrl Pts',(-46.2537073876081,30.0286632749651,
-39.0937226519629));
#269155=CARTESIAN_POINT('Ctrl Pts',(-46.2280147026909,30.001893564456,-39.0844865568113));
#269156=CARTESIAN_POINT('Ctrl Pts',(-46.1492148010453,29.9236586721517,
-39.0568159196779));
#269157=CARTESIAN_POINT('Ctrl Pts',(-46.0943603797766,29.8742287883655,
-39.0384077341064));
#269158=CARTESIAN_POINT('Ctrl Pts',(-46.0086385356025,29.8041510538917,
-39.0108577119752));
#269159=CARTESIAN_POINT('Ctrl Pts',(-45.979489670606,29.7814700298992,-39.0016845404958));
#269160=CARTESIAN_POINT('Ctrl Pts',(-45.9200349130685,29.737472830651,-38.9833588596733));
#269161=CARTESIAN_POINT('Ctrl Pts',(-45.8897290709698,29.7161565962466,
-38.9742063485759));
#269162=CARTESIAN_POINT('Ctrl Pts',(-45.8279451173857,29.6749068346782,
-38.9559225627414));
#269163=CARTESIAN_POINT('Ctrl Pts',(-45.7964751089327,29.6549785818455,
-38.9467936623891));
#269164=CARTESIAN_POINT('Ctrl Pts',(-45.748348603817,29.6261284949947,-38.9331097524421));
#269165=CARTESIAN_POINT('Ctrl Pts',(-45.7321473284057,29.616684052073,-38.9285487676402));
#269166=CARTESIAN_POINT('Ctrl Pts',(-45.6996106203311,29.5982459977232,
-38.9194791520014));
#269167=CARTESIAN_POINT('Ctrl Pts',(-45.683249044345,29.5892352448745,-38.9149628379355));
#269168=CARTESIAN_POINT('Ctrl Pts',(-45.6010439155842,29.5452684013657,
-38.8924942188443));
#269169=CARTESIAN_POINT('Ctrl Pts',(-45.5339074995994,29.5134615304068,
-38.8748432972593));
#269170=CARTESIAN_POINT('Ctrl Pts',(-45.3969715882024,29.4565064940367,
-38.840197135303));
#269171=CARTESIAN_POINT('Ctrl Pts',(-45.3271662939831,29.4313508132015,
-38.823199542964));
#269172=CARTESIAN_POINT('Ctrl Pts',(-45.2204298442793,29.398652641048,-38.7982016720699));
#269173=CARTESIAN_POINT('Ctrl Pts',(-45.184512437616,29.3885937253944,-38.7899522655792));
#269174=CARTESIAN_POINT('Ctrl Pts',(-45.1119891467798,29.3701842541612,
-38.7736235920333));
#269175=CARTESIAN_POINT('Ctrl Pts',(-45.0754052578815,29.3618381514785,
-38.7655490803555));
#269176=CARTESIAN_POINT('Ctrl Pts',(-45.0014447932704,29.3468760834355,
-38.7495561846596));
#269177=CARTESIAN_POINT('Ctrl Pts',(-44.964301863367,29.3403115562353,-38.7416890516424));
#269178=CARTESIAN_POINT('Ctrl Pts',(-44.8900079594565,29.3290481892184,
-38.726277749838));
#269179=CARTESIAN_POINT('Ctrl Pts',(-44.8527936282157,29.324336495618,-38.7187198739728));
#269180=CARTESIAN_POINT('Ctrl Pts',(-44.7410083373266,29.3129455735289,
-38.6964994820139));
#269181=CARTESIAN_POINT('Ctrl Pts',(-44.6662563757167,29.3089967422249,
-38.6822807693139));
#269182=CARTESIAN_POINT('Ctrl Pts',(-44.516312468428,29.3084067934202,-38.6550493453909));
#269183=CARTESIAN_POINT('Ctrl Pts',(-44.441103189525,29.3117700143417,-38.6420342479066));
#269184=CARTESIAN_POINT('Ctrl Pts',(-44.3468378615956,29.3206690055189,
-38.6265520162729));
#269185=CARTESIAN_POINT('Ctrl Pts',(-44.3279589148655,29.3226883315868,
-38.6234933649988));
#269186=CARTESIAN_POINT('Ctrl Pts',(-44.2901960653061,29.3271995080041,
-38.6174591262491));
#269187=CARTESIAN_POINT('Ctrl Pts',(-44.2712743932921,29.329697893027,-38.614477863833));
#269188=CARTESIAN_POINT('Ctrl Pts',(-44.2146592782018,29.3378915995821,
-38.60568558559));
#269189=CARTESIAN_POINT('Ctrl Pts',(-44.1772069502033,29.344266758826,-38.6000392683017));
#269190=CARTESIAN_POINT('Ctrl Pts',(-44.1027653084072,29.3588321594788,
-38.5891549147378));
#269191=CARTESIAN_POINT('Ctrl Pts',(-44.0657945489017,29.3670194960673,
-38.5839197203675));
#269192=CARTESIAN_POINT('Ctrl Pts',(-43.9923490656542,29.3851892021794,
-38.5738612453122));
#269193=CARTESIAN_POINT('Ctrl Pts',(-43.9558743463703,29.395171587473,-38.5690379674556));
#269194=CARTESIAN_POINT('Ctrl Pts',(-43.8834205276403,29.4169303996784,
-38.5598042480103));
#269195=CARTESIAN_POINT('Ctrl Pts',(-43.8474414251675,29.4287068153425,
-38.5553938031715));
#269196=CARTESIAN_POINT('Ctrl Pts',(-43.7759820586595,29.4540658195324,
-38.5469896320335));
#269197=CARTESIAN_POINT('Ctrl Pts',(-43.7405017838471,29.467648368817,-38.5429958961485));
#269198=CARTESIAN_POINT('Ctrl Pts',(-43.6700470477634,29.4966453401303,
-38.5354320983078));
#269199=CARTESIAN_POINT('Ctrl Pts',(-43.6350719757086,29.512061063653,-38.5318621614261));
#269200=CARTESIAN_POINT('Ctrl Pts',(-43.5656410085295,29.5447591316771,
-38.525155654825));
#269201=CARTESIAN_POINT('Ctrl Pts',(-43.5311320054746,29.5620794464364,
-38.5220163122062));
#269202=CARTESIAN_POINT('Ctrl Pts',(-43.4634866412135,29.5981758355574,
-38.5162526847879));
#269203=CARTESIAN_POINT('Ctrl Pts',(-43.4301834663391,29.6170276546,-38.5136117755133));
#269204=CARTESIAN_POINT('Ctrl Pts',(-43.3647025891651,29.6562685687332,
-38.5088155315793));
#269205=CARTESIAN_POINT('Ctrl Pts',(-43.3325078231767,29.6766655539003,
-38.5066585209069));
#269206=CARTESIAN_POINT('Ctrl Pts',(-43.2375484321327,29.7401688861791,
-38.5009063965958));
#269207=CARTESIAN_POINT('Ctrl Pts',(-43.1764049274077,29.7855824582168,
-38.4980286134812));
#269208=CARTESIAN_POINT('Ctrl Pts',(-43.0584774180437,29.8826126224142,
-38.4942050936184));
#269209=CARTESIAN_POINT('Ctrl Pts',(-43.001681818637,29.9342392650769,-38.4932590761897));
#269210=CARTESIAN_POINT('Ctrl Pts',(-42.8926599718677,30.0438904492243,
-38.4933742455196));
#269211=CARTESIAN_POINT('Ctrl Pts',(-42.8414047150844,30.1009342501745,
-38.4944336470273));
#269212=CARTESIAN_POINT('Ctrl Pts',(-42.7451036203247,30.2193471227021,
-38.498479276642));
#269213=CARTESIAN_POINT('Ctrl Pts',(-42.7000684110598,30.2807072617414,
-38.5014658126213));
#269214=CARTESIAN_POINT('Ctrl Pts',(-42.6161769337401,30.4076992015223,
-38.5093469123445));
#269215=CARTESIAN_POINT('Ctrl Pts',(-42.5773225406026,30.4733365238586,
-38.5142428327574));
#269216=CARTESIAN_POINT('Ctrl Pts',(-42.5326943378214,30.5580963840027,
-38.5215739479982));
#269217=CARTESIAN_POINT('Ctrl Pts',(-42.5239673850246,30.5751883092729,
-38.5231018165939));
#269218=CARTESIAN_POINT('Ctrl Pts',(-42.5069121510755,30.60964376351,-38.5262794637242));
#269219=CARTESIAN_POINT('Ctrl Pts',(-42.4985805781952,30.627019094627,-38.5279307934181));
#269220=CARTESIAN_POINT('Ctrl Pts',(-42.4743295471271,30.6792614198295,
-38.5330409224498));
#269221=CARTESIAN_POINT('Ctrl Pts',(-42.4591078049536,30.7143247172706,
-38.5366620777082));
#269222=CARTESIAN_POINT('Ctrl Pts',(-42.4305062721789,30.7849297925434,
-38.5443248028235));
#269223=CARTESIAN_POINT('Ctrl Pts',(-42.4171273618354,30.8204683264523,
-38.5483659418649));
#269224=CARTESIAN_POINT('Ctrl Pts',(-42.3921837112499,30.89200995013,-38.556860031436));
#269225=CARTESIAN_POINT('Ctrl Pts',(-42.3806190180342,30.9280130518798,
-38.5613129931637));
#269226=CARTESIAN_POINT('Ctrl Pts',(-42.3592881563091,31.0004799414626,
-38.5706260903895));
#269227=CARTESIAN_POINT('Ctrl Pts',(-42.3495220063211,31.0369437339595,
-38.5754862307243));
#269228=CARTESIAN_POINT('Ctrl Pts',(-42.3317857495347,31.1103315158532,
-38.5856119737634));
#269229=CARTESIAN_POINT('Ctrl Pts',(-42.3238156343608,31.1472555030051,
-38.5908775753381));
#269230=CARTESIAN_POINT('Ctrl Pts',(-42.3096820427396,31.2215665449467,
-38.6018154236264));
#269231=CARTESIAN_POINT('Ctrl Pts',(-42.3035171869091,31.2589715314082,
-38.6074906718877));
#269232=CARTESIAN_POINT('Ctrl Pts',(-42.2930235524414,31.3341791410138,
-38.6192399292287));
#269233=CARTESIAN_POINT('Ctrl Pts',(-42.2886818075092,31.3721585359098,
-38.6253436316658));
#269234=CARTESIAN_POINT('Ctrl Pts',(-42.2819306306109,31.4478003630713,
-38.6378362101326));
#269235=CARTESIAN_POINT('Ctrl Pts',(-42.2795025237186,31.4855414978569,
-38.6442360129219));
#269236=CARTESIAN_POINT('Ctrl Pts',(-42.2765060643256,31.5608485897329,
-38.6573322722499));
#269237=CARTESIAN_POINT('Ctrl Pts',(-42.2759365563455,31.5984178297074,
-38.6640291190605));
#269238=CARTESIAN_POINT('Ctrl Pts',(-42.2769710616629,31.710876916496,-38.6845570305479));
#269239=CARTESIAN_POINT('Ctrl Pts',(-42.2813124759152,31.7855186400122,
-38.698824567557));
#269240=CARTESIAN_POINT('Ctrl Pts',(-42.2932531103751,31.8969906134966,
-38.7210841829084));
#269241=CARTESIAN_POINT('Ctrl Pts',(-42.2981395950573,31.934066030451,-38.7286473545921));
#269242=CARTESIAN_POINT('Ctrl Pts',(-42.3097367777483,32.0080522284017,
-38.7440609732535));
#269243=CARTESIAN_POINT('Ctrl Pts',(-42.3164494406915,32.0449687602613,
-38.7519128032936));
#269244=CARTESIAN_POINT('Ctrl Pts',(-42.3317154579634,32.1186122141692,
-38.7679009120377));
#269245=CARTESIAN_POINT('Ctrl Pts',(-42.3402956643805,32.1554227583218,
-38.7760569897633));
#269246=CARTESIAN_POINT('Ctrl Pts',(-42.3591481714288,32.228169160774,-38.7925026060078));
#269247=CARTESIAN_POINT('Ctrl Pts',(-42.3694448348212,32.2642362896146,
-38.8008201507359));
#269248=CARTESIAN_POINT('Ctrl Pts',(-42.391742799968,32.3356900672865,-38.817625053217));
#269249=CARTESIAN_POINT('Ctrl Pts',(-42.4037465150873,32.3710895326604,
-38.8261151521117));
#269250=CARTESIAN_POINT('Ctrl Pts',(-42.4294540540394,32.4412374294065,
-38.843268788153));
#269251=CARTESIAN_POINT('Ctrl Pts',(-42.4431578847231,32.4759858579934,
-38.8519323266271));
#269252=CARTESIAN_POINT('Ctrl Pts',(-42.4577131944628,32.5104083279579,
-38.8606823233885));
#269253=CARTESIAN_POINT('Ctrl Pts',(-46.348736272544,30.7584582252104,-39.6906856150703));
#269254=CARTESIAN_POINT('Ctrl Pts',(-46.3360470969151,30.7285883901681,
-39.6821765324611));
#269255=CARTESIAN_POINT('Ctrl Pts',(-46.3226745755283,30.699129013129,-39.6736060666043));
#269256=CARTESIAN_POINT('Ctrl Pts',(-46.2945857386662,30.6410176089828,
-39.6563436429933));
#269257=CARTESIAN_POINT('Ctrl Pts',(-46.2798693485556,30.6123656264171,
-39.6476516797756));
#269258=CARTESIAN_POINT('Ctrl Pts',(-46.2337241557402,30.5276091385302,
-39.6213942796991));
#269259=CARTESIAN_POINT('Ctrl Pts',(-46.2003035256421,30.4727015800282,
-39.6036476811977));
#269260=CARTESIAN_POINT('Ctrl Pts',(-46.1461806704985,30.3927399191851,
-39.5766612769609));
#269261=CARTESIAN_POINT('Ctrl Pts',(-46.1274733675407,30.3664865966257,
-39.5676046409352));
#269262=CARTESIAN_POINT('Ctrl Pts',(-46.0887106443918,30.3147904520985,
-39.549367177482));
#269263=CARTESIAN_POINT('Ctrl Pts',(-46.0686677193846,30.2893627735597,
-39.5401919312515));
#269264=CARTESIAN_POINT('Ctrl Pts',(-46.0271590696364,30.2392722779402,
-39.5216922982112));
#269265=CARTESIAN_POINT('Ctrl Pts',(-46.0058175903831,30.2147651800999,
-39.512424414423));
#269266=CARTESIAN_POINT('Ctrl Pts',(-45.9621758028444,30.1670336173528,
-39.4939378067199));
#269267=CARTESIAN_POINT('Ctrl Pts',(-45.93983653738,30.1437620920995,-39.4847017115683));
#269268=CARTESIAN_POINT('Ctrl Pts',(-45.8713242771536,30.0757481602649,
-39.4570310744349));
#269269=CARTESIAN_POINT('Ctrl Pts',(-45.8236347617589,30.0327725532112,
-39.4386228888633));
#269270=CARTESIAN_POINT('Ctrl Pts',(-45.7491145832093,29.9718396783148,
-39.4110728667323));
#269271=CARTESIAN_POINT('Ctrl Pts',(-45.7237755280245,29.952117465038,-39.4018996952527));
#269272=CARTESIAN_POINT('Ctrl Pts',(-45.6720931922673,29.9138578177121,
-39.3835740144303));
#269273=CARTESIAN_POINT('Ctrl Pts',(-45.6457499554623,29.8953203323242,
-39.3744215033328));
#269274=CARTESIAN_POINT('Ctrl Pts',(-45.5920460375509,29.8594456348434,
-39.3561377174984));
#269275=CARTESIAN_POINT('Ctrl Pts',(-45.5646923996724,29.8421130099496,
-39.347008817146));
#269276=CARTESIAN_POINT('Ctrl Pts',(-45.5228621313133,29.817018813152,-39.333324907199));
#269277=CARTESIAN_POINT('Ctrl Pts',(-45.5087806057656,29.8088035965387,
-39.3287639223973));
#269278=CARTESIAN_POINT('Ctrl Pts',(-45.4805013249128,29.7927646822922,
-39.3196943067583));
#269279=CARTESIAN_POINT('Ctrl Pts',(-45.4662808454981,29.7849260765311,
-39.3151779926924));
#269280=CARTESIAN_POINT('Ctrl Pts',(-45.394834111845,29.7466769167217,-39.2927093736018));
#269281=CARTESIAN_POINT('Ctrl Pts',(-45.3364869241018,29.7190010072829,
-39.2750584520161));
#269282=CARTESIAN_POINT('Ctrl Pts',(-45.2174838212522,29.6694313228168,
-39.24041229006));
#269283=CARTESIAN_POINT('Ctrl Pts',(-45.1568228629401,29.6475310155415,
-39.223414697721));
#269284=CARTESIAN_POINT('Ctrl Pts',(-45.0640728677801,29.6190530040921,
-39.1984168268269));
#269285=CARTESIAN_POINT('Ctrl Pts',(-45.0328626716162,29.6102901609231,
-39.1901674203362));
#269286=CARTESIAN_POINT('Ctrl Pts',(-44.9698454327154,29.5942479284802,
-39.1738387467903));
#269287=CARTESIAN_POINT('Ctrl Pts',(-44.9380575013641,29.5869724226462,
-39.1657642351124));
#269288=CARTESIAN_POINT('Ctrl Pts',(-44.873794287365,29.5739237069059,-39.1497713394166));
#269289=CARTESIAN_POINT('Ctrl Pts',(-44.8415220194395,29.5681953426883,
-39.1419042063994));
#269290=CARTESIAN_POINT('Ctrl Pts',(-44.7769718892781,29.5583592071516,
-39.126492904595));
#269291=CARTESIAN_POINT('Ctrl Pts',(-44.7446389767916,29.5542402259256,
-39.1189350287298));
#269292=CARTESIAN_POINT('Ctrl Pts',(-44.64751868345,29.5442668522271,-39.0967146367708));
#269293=CARTESIAN_POINT('Ctrl Pts',(-44.5825761125008,29.5407840481455,
-39.0824959240709));
#269294=CARTESIAN_POINT('Ctrl Pts',(-44.4523142911657,29.540165884783,-39.055264500148));
#269295=CARTESIAN_POINT('Ctrl Pts',(-44.386979986101,29.5430342817064,-39.0422494026637));
#269296=CARTESIAN_POINT('Ctrl Pts',(-44.3050952734897,29.5506978499007,
-39.0267671710297));
#269297=CARTESIAN_POINT('Ctrl Pts',(-44.288696030367,29.5524386096434,-39.0237085197559));
#269298=CARTESIAN_POINT('Ctrl Pts',(-44.2558936005359,29.556330581768,-39.017674281006));
#269299=CARTESIAN_POINT('Ctrl Pts',(-44.2394576074491,29.5584874438222,
-39.01469301859));
#269300=CARTESIAN_POINT('Ctrl Pts',(-44.1902803880436,29.5655649308415,
-39.0059007403469));
#269301=CARTESIAN_POINT('Ctrl Pts',(-44.1577491481311,29.5710762653616,
-39.0002544230587));
#269302=CARTESIAN_POINT('Ctrl Pts',(-44.0930902993264,29.5836759361658,
-38.9893700694948));
#269303=CARTESIAN_POINT('Ctrl Pts',(-44.0609788069576,29.5907617622781,
-38.9841348751245));
#269304=CARTESIAN_POINT('Ctrl Pts',(-43.9971881260961,29.6064930329024,
-38.9740764000692));
#269305=CARTESIAN_POINT('Ctrl Pts',(-43.9655089414875,29.6151384911107,
-38.9692531222126));
#269306=CARTESIAN_POINT('Ctrl Pts',(-43.9025825141023,29.6339881744307,
-38.9600194027673));
#269307=CARTESIAN_POINT('Ctrl Pts',(-43.8713352686894,29.644192389763,-38.9556089579285));
#269308=CARTESIAN_POINT('Ctrl Pts',(-43.8092755239302,29.666170138253,-38.9472047867905));
#269309=CARTESIAN_POINT('Ctrl Pts',(-43.7784630151957,29.6779436373071,
-38.9432110509055));
#269310=CARTESIAN_POINT('Ctrl Pts',(-43.7172788205642,29.7030822942954,
-38.9356472530647));
#269311=CARTESIAN_POINT('Ctrl Pts',(-43.68690660506,29.7164485823689,-38.9320773161832));
#269312=CARTESIAN_POINT('Ctrl Pts',(-43.6266146289649,29.7448030239206,
-38.9253708095819));
#269313=CARTESIAN_POINT('Ctrl Pts',(-43.5966487607817,29.7598241234161,
-38.9222314669632));
#269314=CARTESIAN_POINT('Ctrl Pts',(-43.5379105932515,29.7911319045234,
-38.9164678395448));
#269315=CARTESIAN_POINT('Ctrl Pts',(-43.5089934352673,29.8074842645775,
-38.9138269302702));
#269316=CARTESIAN_POINT('Ctrl Pts',(-43.4521380201768,29.8415252139572,
-38.9090306863362));
#269317=CARTESIAN_POINT('Ctrl Pts',(-43.4241849453146,29.8592206450036,
-38.9068736756639));
#269318=CARTESIAN_POINT('Ctrl Pts',(-43.3417390736822,29.9143168693475,
-38.9011215513527));
#269319=CARTESIAN_POINT('Ctrl Pts',(-43.2886563370204,29.9537231156165,
-38.8982437682382));
#269320=CARTESIAN_POINT('Ctrl Pts',(-43.1862827102732,30.0379274090563,
-38.8944202483754));
#269321=CARTESIAN_POINT('Ctrl Pts',(-43.1369817552336,30.0827341785328,
-38.8934742309467));
#269322=CARTESIAN_POINT('Ctrl Pts',(-43.0423540539346,30.1779090615142,
-38.8935894002766));
#269323=CARTESIAN_POINT('Ctrl Pts',(-42.9978700944569,30.2274259110637,
-38.8946488017843));
#269324=CARTESIAN_POINT('Ctrl Pts',(-42.9142995039568,30.330221730441,-38.898694431399));
#269325=CARTESIAN_POINT('Ctrl Pts',(-42.8752220997707,30.3834929481532,
-38.9016809673782));
#269326=CARTESIAN_POINT('Ctrl Pts',(-42.802438005755,30.4937509787714,-38.9095620671015));
#269327=CARTESIAN_POINT('Ctrl Pts',(-42.7687329487861,30.5507425897786,
-38.9144579875143));
#269328=CARTESIAN_POINT('Ctrl Pts',(-42.7300260074317,30.6243421619354,
-38.9217891027552));
#269329=CARTESIAN_POINT('Ctrl Pts',(-42.7224573165159,30.6391838099202,
-38.9233169713508));
#269330=CARTESIAN_POINT('Ctrl Pts',(-42.7076664478388,30.6691033617142,
-38.9264946184813));
#269331=CARTESIAN_POINT('Ctrl Pts',(-42.7004414190611,30.6841915159301,
-38.9281459481751));
#269332=CARTESIAN_POINT('Ctrl Pts',(-42.6794124410656,30.7295576092503,
-38.9332560772068));
#269333=CARTESIAN_POINT('Ctrl Pts',(-42.6662147228328,30.7600066178112,
-38.9368772324651));
#269334=CARTESIAN_POINT('Ctrl Pts',(-42.6414196796479,30.8213217206122,
-38.9445399575806));
#269335=CARTESIAN_POINT('Ctrl Pts',(-42.6298231170419,30.8521849974158,
-38.9485810966219));
#269336=CARTESIAN_POINT('Ctrl Pts',(-42.6082062309801,30.9143165209769,
-38.9570751861931));
#269337=CARTESIAN_POINT('Ctrl Pts',(-42.5981859483915,30.9455847781742,
-38.9615281479207));
#269338=CARTESIAN_POINT('Ctrl Pts',(-42.5797080184842,31.0085228897363,
-38.9708412451465));
#269339=CARTESIAN_POINT('Ctrl Pts',(-42.5712503872647,31.040192748165,-38.9757013854813));
#269340=CARTESIAN_POINT('Ctrl Pts',(-42.555895594383,31.1039336351222,-38.9858271285205));
#269341=CARTESIAN_POINT('Ctrl Pts',(-42.5489984254493,31.1360046616943,
-38.9910927300951));
#269342=CARTESIAN_POINT('Ctrl Pts',(-42.5367737540442,31.2005503855788,
-39.0020305783833));
#269343=CARTESIAN_POINT('Ctrl Pts',(-42.5314450660311,31.2330406596962,
-39.0077058266447));
#269344=CARTESIAN_POINT('Ctrl Pts',(-42.5223828738566,31.2983680565044,
-39.0194550839858));
#269345=CARTESIAN_POINT('Ctrl Pts',(-42.5186382312793,31.3313587369558,
-39.0255587864228));
#269346=CARTESIAN_POINT('Ctrl Pts',(-42.5128272133948,31.3970662193109,
-39.0380513648896));
#269347=CARTESIAN_POINT('Ctrl Pts',(-42.5107446717144,31.4298513784848,
-39.0444511676788));
#269348=CARTESIAN_POINT('Ctrl Pts',(-42.5081949220986,31.4952709313388,
-39.0575474270069));
#269349=CARTESIAN_POINT('Ctrl Pts',(-42.5077267127911,31.5279081760849,
-39.0642442738175));
#269350=CARTESIAN_POINT('Ctrl Pts',(-42.5087046075987,31.6256059960414,
-39.0847721853048));
#269351=CARTESIAN_POINT('Ctrl Pts',(-42.5125283453785,31.6904530960276,
-39.099039722314));
#269352=CARTESIAN_POINT('Ctrl Pts',(-42.5229789971415,31.7873016127624,
-39.1212993376654));
#269353=CARTESIAN_POINT('Ctrl Pts',(-42.5272497098319,31.8195139765299,
-39.128862509349));
#269354=CARTESIAN_POINT('Ctrl Pts',(-42.5373755918422,31.8837970410461,
-39.1442761280104));
#269355=CARTESIAN_POINT('Ctrl Pts',(-42.5432324720224,31.9158727392425,
-39.1521279580505));
#269356=CARTESIAN_POINT('Ctrl Pts',(-42.5565449846397,31.9798607801841,
-39.1681160667947));
#269357=CARTESIAN_POINT('Ctrl Pts',(-42.5640240006773,32.0118457883453,
-39.1762721445204));
#269358=CARTESIAN_POINT('Ctrl Pts',(-42.5804512263956,32.0750571790556,
-39.1927177607647));
#269359=CARTESIAN_POINT('Ctrl Pts',(-42.5894206909713,32.1063976191197,
-39.2010353054929));
#269360=CARTESIAN_POINT('Ctrl Pts',(-42.6088398491466,32.1684885866316,
-39.2178402079739));
#269361=CARTESIAN_POINT('Ctrl Pts',(-42.6192916481159,32.1992502500668,
-39.2263303068687));
#269362=CARTESIAN_POINT('Ctrl Pts',(-42.6416715644566,32.2602092315461,
-39.2434839429101));
#269363=CARTESIAN_POINT('Ctrl Pts',(-42.6535996877758,32.290406547182,-39.252147481384));
#269364=CARTESIAN_POINT('Ctrl Pts',(-42.6662672096695,32.3203213022051,
-39.2608974781455));
#269365=CARTESIAN_POINT('Ctrl Pts',(-42.5264432849996,31.269119253141,-39.0141952505087));
#269366=CARTESIAN_POINT('Ctrl Pts',(-42.5221224658057,31.3006702972118,
-39.0198812138034));
#269367=CARTESIAN_POINT('Ctrl Pts',(-42.5185368438515,31.3325051647859,
-39.0257767500263));
#269368=CARTESIAN_POINT('Ctrl Pts',(-42.515732722337,31.3642124781334,-39.0318050756562));
#269369=CARTESIAN_POINT('Ctrl Pts',(-42.5128272155788,31.3970661946154,
-39.0380513601944));
#269370=CARTESIAN_POINT('Ctrl Pts',(-42.5107447016068,31.4298506115284,
-39.0444510141427));
#269371=CARTESIAN_POINT('Ctrl Pts',(-42.5094697969065,31.4625611549118,
-39.0509992973428));
#269372=CARTESIAN_POINT('Ctrl Pts',(-42.508194891176,31.495271724727,-39.0575475858343));
#269373=CARTESIAN_POINT('Ctrl Pts',(-42.5077267152746,31.5279084227224,
-39.0642443261397));
#269374=CARTESIAN_POINT('Ctrl Pts',(-42.5080525657557,31.5604741525115,
-39.0710867176316));
#269375=CARTESIAN_POINT('Ctrl Pts',(-42.5087042669078,31.6256056310615,
-39.0847715046015));
#269376=CARTESIAN_POINT('Ctrl Pts',(-42.5125279911245,31.6904531051536,
-39.0990390579777));
#269377=CARTESIAN_POINT('Ctrl Pts',(-42.5194952327192,31.7550179760245,
-39.1138790580997));
#269378=CARTESIAN_POINT('Ctrl Pts',(-42.5229788523054,31.7873004002368,
-39.1212990555811));
#269379=CARTESIAN_POINT('Ctrl Pts',(-42.5272493642385,31.8195120978489,
-39.1288619647275));
#269380=CARTESIAN_POINT('Ctrl Pts',(-42.5323125754593,31.8516552046985,
-39.1365691980944));
#269381=CARTESIAN_POINT('Ctrl Pts',(-42.5373757866802,31.8837983115481,
-39.1442764314613));
#269382=CARTESIAN_POINT('Ctrl Pts',(-42.5432324720224,31.9158727392424,
-39.1521279580505));
#269383=CARTESIAN_POINT('Ctrl Pts',(-42.5498887283311,31.9478667597133,
-39.1601220124226));
#269384=CARTESIAN_POINT('Ctrl Pts',(-42.5565449846397,31.9798607801841,
-39.1681160667947));
#269385=CARTESIAN_POINT('Ctrl Pts',(-42.5640240006772,32.0118457883453,
-39.1762721445203));
#269386=CARTESIAN_POINT('Ctrl Pts',(-42.5722376135364,32.0434514837005,
-39.1844949526425));
#269387=CARTESIAN_POINT('Ctrl Pts',(-42.5804512263956,32.0750571790557,
-39.1927177607647));
#269388=CARTESIAN_POINT('Ctrl Pts',(-42.5894206909713,32.1063976191197,
-39.2010353054928));
#269389=CARTESIAN_POINT('Ctrl Pts',(-42.599130270059,32.1374431028757,-39.2094377567334));
#269390=CARTESIAN_POINT('Ctrl Pts',(-42.6088398491467,32.1684885866317,
-39.217840207974));
#269391=CARTESIAN_POINT('Ctrl Pts',(-42.619291648116,32.1992502500668,-39.2263303068687));
#269392=CARTESIAN_POINT('Ctrl Pts',(-42.6304816062863,32.2297297408064,
-39.2349071248894));
#269393=CARTESIAN_POINT('Ctrl Pts',(-42.6416715644565,32.2602092315458,
-39.24348394291));
#269394=CARTESIAN_POINT('Ctrl Pts',(-42.6535996877756,32.2904065471814,
-39.2521474813839));
#269395=CARTESIAN_POINT('Ctrl Pts',(-42.6662672096693,32.3203213022045,
-39.2608974781453));
#269396=CARTESIAN_POINT('Ctrl Pts',(-46.348736272544,30.7584582252104,-39.6906856150703));
#269397=CARTESIAN_POINT('Ctrl Pts',(-46.3360470973409,30.7285883911703,
-39.6821765327467));
#269398=CARTESIAN_POINT('Ctrl Pts',(-46.3226745905749,30.6991290109582,
-39.6736060493954));
#269399=CARTESIAN_POINT('Ctrl Pts',(-46.3086301900114,30.670073305053,-39.6649748164403));
#269400=CARTESIAN_POINT('Ctrl Pts',(-46.2945857887134,30.6410175976279,
-39.6563435830337));
#269401=CARTESIAN_POINT('Ctrl Pts',(-46.2798694188995,30.6123656091012,
-39.6476515945533));
#269402=CARTESIAN_POINT('Ctrl Pts',(-46.2644877017587,30.5841134449057,
-39.6388991131053));
#269403=CARTESIAN_POINT('Ctrl Pts',(-46.2337242678266,30.5276091171564,
-39.6213941504079));
#269404=CARTESIAN_POINT('Ctrl Pts',(-46.2003039001332,30.4727015444266,
-39.6036472934442));
#269405=CARTESIAN_POINT('Ctrl Pts',(-46.1642217344127,30.4193937755162,
-39.5856566097807));
#269406=CARTESIAN_POINT('Ctrl Pts',(-46.146180651686,30.3927398912582,-39.5766612680155));
#269407=CARTESIAN_POINT('Ctrl Pts',(-46.1274733675408,30.3664865966258,
-39.5676046409352));
#269408=CARTESIAN_POINT('Ctrl Pts',(-46.1080920059663,30.3406385243622,
-39.5584859092086));
#269409=CARTESIAN_POINT('Ctrl Pts',(-46.0887106443919,30.3147904520986,
-39.5493671774819));
#269410=CARTESIAN_POINT('Ctrl Pts',(-46.0686677193846,30.2893627735597,
-39.5401919312515));
#269411=CARTESIAN_POINT('Ctrl Pts',(-46.0479133945105,30.2643175257499,
-39.5309421147314));
#269412=CARTESIAN_POINT('Ctrl Pts',(-46.0271590696364,30.2392722779402,
-39.5216922982112));
#269413=CARTESIAN_POINT('Ctrl Pts',(-46.0058175903831,30.2147651800999,
-39.512424414423));
#269414=CARTESIAN_POINT('Ctrl Pts',(-45.9839966966138,30.1908993987264,
-39.5031811105714));
#269415=CARTESIAN_POINT('Ctrl Pts',(-45.9621758028444,30.1670336173528,
-39.4939378067199));
#269416=CARTESIAN_POINT('Ctrl Pts',(-45.93983653738,30.1437620920996,-39.4847017115683));
#269417=CARTESIAN_POINT('Ctrl Pts',(-45.9169991173045,30.121090781488,-39.4754781658572));
#269418=CARTESIAN_POINT('Ctrl Pts',(-45.8713242883866,30.0757481714161,
-39.4570310789716));
#269419=CARTESIAN_POINT('Ctrl Pts',(-45.8236354571138,30.0327727895174,
-39.4386227099774));
#269420=CARTESIAN_POINT('Ctrl Pts',(-45.773954719475,29.992150588615,-39.4202560907654));
#269421=CARTESIAN_POINT('Ctrl Pts',(-45.7491145157246,29.971839623135,-39.4110728421843));
#269422=CARTESIAN_POINT('Ctrl Pts',(-45.7237758311101,29.9521176894074,
-39.4018998026794));
#269423=CARTESIAN_POINT('Ctrl Pts',(-45.6979343678929,29.9329876360372,
-39.3927368425297));
#269424=CARTESIAN_POINT('Ctrl Pts',(-45.6720926283413,29.9138573781007,
-39.3835737843965));
#269425=CARTESIAN_POINT('Ctrl Pts',(-45.6457480380852,29.8953190514989,
-39.3744208505476));
#269426=CARTESIAN_POINT('Ctrl Pts',(-45.6188979971575,29.8773829830905,
-39.36527960933));
#269427=CARTESIAN_POINT('Ctrl Pts',(-45.5920479621773,29.859446918655,-39.3561383701372));
#269428=CARTESIAN_POINT('Ctrl Pts',(-45.5646924995279,29.8421130698535,
-39.3470088498117));
#269429=CARTESIAN_POINT('Ctrl Pts',(-45.5368055540997,29.8253835454179,
-39.3378862105147));
#269430=CARTESIAN_POINT('Ctrl Pts',(-45.5228621313133,29.817018813152,-39.3333249071991));
#269431=CARTESIAN_POINT('Ctrl Pts',(-45.5087806057656,29.8088035965387,
-39.3287639223973));
#269432=CARTESIAN_POINT('Ctrl Pts',(-45.4946409653392,29.8007841394154,
-39.3242291145778));
#269433=CARTESIAN_POINT('Ctrl Pts',(-45.4805013249128,29.7927646822922,
-39.3196943067583));
#269434=CARTESIAN_POINT('Ctrl Pts',(-45.4662808454981,29.7849260765311,
-39.3151779926924));
#269435=CARTESIAN_POINT('Ctrl Pts',(-45.4519914987675,29.7772762445693,
-39.3106842688742));
#269436=CARTESIAN_POINT('Ctrl Pts',(-45.3948341399523,29.746676931769,-39.292709382441));
#269437=CARTESIAN_POINT('Ctrl Pts',(-45.3364886465416,29.7190017247075,
-39.2750589508555));
#269438=CARTESIAN_POINT('Ctrl Pts',(-45.276985562247,29.6942159545788,-39.2577349684532));
#269439=CARTESIAN_POINT('Ctrl Pts',(-45.2211882780065,29.6709738205385,
-39.241489908525));
#269440=CARTESIAN_POINT('Ctrl Pts',(-45.1643742277393,29.6502692579128,
-39.2255326383472));
#269441=CARTESIAN_POINT('Ctrl Pts',(-45.1065114146008,29.6321213447558,
-39.209862333485));
#269442=CARTESIAN_POINT('Ctrl Pts',(-46.8777108695604,31.7246583249715,
-39.4968621491069));
#269443=CARTESIAN_POINT('Ctrl Pts',(-46.8781729355344,31.7155928097276,
-39.4953858594052));
#269444=CARTESIAN_POINT('Ctrl Pts',(-46.8785816536823,31.7065201757618,
-39.4938989911198));
#269445=CARTESIAN_POINT('Ctrl Pts',(-46.8796767940079,31.6785286095959,
-39.4892824810203));
#269446=CARTESIAN_POINT('Ctrl Pts',(-46.8801843407089,31.6595724593507,
-39.4861150486293));
#269447=CARTESIAN_POINT('Ctrl Pts',(-46.8807312344332,31.6216180949417,
-39.479690628598));
#269448=CARTESIAN_POINT('Ctrl Pts',(-46.8807699646674,31.6025797052015,
-39.4764266299692));
#269449=CARTESIAN_POINT('Ctrl Pts',(-46.8801790388754,31.5455906639181,
-39.4665317368708));
#269450=CARTESIAN_POINT('Ctrl Pts',(-46.8788490796135,31.5078273383739,
-39.4598096545541));
#269451=CARTESIAN_POINT('Ctrl Pts',(-46.874360617844,31.4326451774338,-39.4461013696832));
#269452=CARTESIAN_POINT('Ctrl Pts',(-46.864884835636,31.320441459725,-39.4251517854185));
#269453=CARTESIAN_POINT('Ctrl Pts',(-46.8414902947658,31.1730719473388,
-39.3956936109857));
#269454=CARTESIAN_POINT('Ctrl Pts',(-46.8074810934279,31.0279105813681,
-39.364717848004));
#269455=CARTESIAN_POINT('Ctrl Pts',(-46.7869180083019,30.9560697433081,
-39.3487190247537));
#269456=CARTESIAN_POINT('Ctrl Pts',(-46.7645577771926,30.884604709384,-39.332461491893));
#269457=CARTESIAN_POINT('Ctrl Pts',(-46.7524740339114,30.8490466969583,
-39.3242001683612));
#269458=CARTESIAN_POINT('Ctrl Pts',(-46.7264943673172,30.7783632715819,
-39.3074248425479));
#269459=CARTESIAN_POINT('Ctrl Pts',(-46.7127058212706,30.7435263372096,
-39.2989795429224));
#269460=CARTESIAN_POINT('Ctrl Pts',(-46.6981266849492,30.7091523375488,
-39.2904704603133));
#269461=CARTESIAN_POINT('Ctrl Pts',(-45.1104359790682,31.3262729516313,
-41.3967784080596));
#269462=CARTESIAN_POINT('Ctrl Pts',(-45.1105813863711,31.3228595121998,
-41.3953021183579));
#269463=CARTESIAN_POINT('Ctrl Pts',(-45.1107066559544,31.3194432352723,
-41.3938152500725));
#269464=CARTESIAN_POINT('Ctrl Pts',(-45.1110306052012,31.30890259785,-41.3891987399731));
#269465=CARTESIAN_POINT('Ctrl Pts',(-45.1111617199316,31.3017636946428,
-41.3860313075819));
#269466=CARTESIAN_POINT('Ctrl Pts',(-45.1112472734604,31.2874686716035,
-41.3796068875509));
#269467=CARTESIAN_POINT('Ctrl Pts',(-45.111201351958,31.2802974166487,-41.3763428889219));
#269468=CARTESIAN_POINT('Ctrl Pts',(-45.1107973541963,31.25882908612,-41.3664479958234));
#269469=CARTESIAN_POINT('Ctrl Pts',(-45.11017580813,31.2446005169708,-41.3597259135069));
#269470=CARTESIAN_POINT('Ctrl Pts',(-45.1082442962718,31.2162677536902,
-41.3460176286356));
#269471=CARTESIAN_POINT('Ctrl Pts',(-45.104314463686,31.1739750543259,-41.3250680443717));
#269472=CARTESIAN_POINT('Ctrl Pts',(-45.0950241996196,31.1183949914011,
-41.295609869938));
#269473=CARTESIAN_POINT('Ctrl Pts',(-45.0817381040079,31.0636149263882,
-41.264634106957));
#269474=CARTESIAN_POINT('Ctrl Pts',(-45.0737554763462,31.0364928582332,
-41.2486352837062));
#269475=CARTESIAN_POINT('Ctrl Pts',(-45.0650963255467,31.0095068957897,
-41.2323777508457));
#269476=CARTESIAN_POINT('Ctrl Pts',(-45.0604265398991,30.996076905732,-41.224116427314));
#269477=CARTESIAN_POINT('Ctrl Pts',(-45.0504049610752,30.9693743366894,
-41.2073411015006));
#269478=CARTESIAN_POINT('Ctrl Pts',(-45.0450945767524,30.9562107421528,
-41.1988958018751));
#269479=CARTESIAN_POINT('Ctrl Pts',(-45.0394875320819,30.9432190801919,
-41.190386719266));
#269480=CARTESIAN_POINT('',(-46.348736272544,30.7584582252104,-39.6906856150703));
#269481=CARTESIAN_POINT('Ctrl Pts',(-46.6981266849492,30.7091523375488,
-39.2904704603133));
#269482=CARTESIAN_POINT('Ctrl Pts',(-46.6689684123063,30.6404043382273,
-39.273452295095));
#269483=CARTESIAN_POINT('Ctrl Pts',(-46.6043681216411,30.5066861069553,
-39.238925705885));
#269484=CARTESIAN_POINT('Ctrl Pts',(-46.5083209189471,30.3487389562033,
-39.1945593129175));
#269485=CARTESIAN_POINT('Ctrl Pts',(-46.4437937583117,30.2581216171786,
-39.1673894861782));
#269486=CARTESIAN_POINT('Ctrl Pts',(-46.3992224148768,30.1986447451181,
-39.1491520227249));
#269487=CARTESIAN_POINT('Ctrl Pts',(-46.3761748773305,30.1693908446446,
-39.1399767764946));
#269488=CARTESIAN_POINT('Ctrl Pts',(-46.3284414024809,30.1117648114071,
-39.1214771434543));
#269489=CARTESIAN_POINT('Ctrl Pts',(-46.3038983378397,30.083571828401,-39.112209259666));
#269490=CARTESIAN_POINT('Ctrl Pts',(-46.253707387608,30.0286632749651,-39.0937226519629));
#269491=CARTESIAN_POINT('Ctrl Pts',(-46.2280147026909,30.001893564456,-39.0844865568113));
#269492=CARTESIAN_POINT('Ctrl Pts',(-46.1492148010453,29.9236586721517,
-39.0568159196779));
#269493=CARTESIAN_POINT('Ctrl Pts',(-46.0669347173688,29.8495134741745,
-39.0292038481275));
#269494=CARTESIAN_POINT('Ctrl Pts',(-45.9503410384262,29.7587889734315,
-38.9925114043613));
#269495=CARTESIAN_POINT('Ctrl Pts',(-45.8594191065401,29.6948377475824,
-38.9650526418885));
#269496=CARTESIAN_POINT('Ctrl Pts',(-45.7964751089327,29.6549785818455,
-38.9467936623891));
#269497=CARTESIAN_POINT('Ctrl Pts',(-45.748348603817,29.6261284949947,-38.9331097524421));
#269498=CARTESIAN_POINT('Ctrl Pts',(-45.7321473284057,29.616684052073,-38.9285487676403));
#269499=CARTESIAN_POINT('Ctrl Pts',(-45.6996106203311,29.5982459977232,
-38.9194791520014));
#269500=CARTESIAN_POINT('Ctrl Pts',(-45.683249044345,29.5892352448745,-38.9149628379356));
#269501=CARTESIAN_POINT('Ctrl Pts',(-45.6010439155842,29.5452684013657,
-38.8924942188443));
#269502=CARTESIAN_POINT('Ctrl Pts',(-45.4667739830181,29.4816584171599,
-38.8571935516581));
#269503=CARTESIAN_POINT('Ctrl Pts',(-45.2922645146651,29.4187721922835,
-38.8147007629208));
#269504=CARTESIAN_POINT('Ctrl Pts',(-45.184512437616,29.3885937253944,-38.7899522655792));
#269505=CARTESIAN_POINT('Ctrl Pts',(-45.1119891467798,29.3701842541612,
-38.7736235920333));
#269506=CARTESIAN_POINT('Ctrl Pts',(-45.0754052578815,29.3618381514785,
-38.7655490803555));
#269507=CARTESIAN_POINT('Ctrl Pts',(-45.0014447932705,29.3468760834356,
-38.7495561846596));
#269508=CARTESIAN_POINT('Ctrl Pts',(-44.964301863367,29.3403115562353,-38.7416890516424));
#269509=CARTESIAN_POINT('Ctrl Pts',(-44.8900079594565,29.3290481892184,
-38.726277749838));
#269510=CARTESIAN_POINT('Ctrl Pts',(-44.8527936282157,29.324336495618,-38.7187198739728));
#269511=CARTESIAN_POINT('Ctrl Pts',(-44.7410083373266,29.3129455735289,
-38.6964994820139));
#269512=CARTESIAN_POINT('Ctrl Pts',(-44.6662563757167,29.3089967422249,
-38.6822807693139));
#269513=CARTESIAN_POINT('Ctrl Pts',(-44.516312468428,29.3084067934202,-38.6550493453909));
#269514=CARTESIAN_POINT('Ctrl Pts',(-44.441103189525,29.3117700143417,-38.6420342479066));
#269515=CARTESIAN_POINT('Ctrl Pts',(-44.3468378615956,29.3206690055189,
-38.6265520162729));
#269516=CARTESIAN_POINT('Ctrl Pts',(-44.3279589148655,29.3226883315868,
-38.6234933649988));
#269517=CARTESIAN_POINT('Ctrl Pts',(-44.2901960653062,29.3271995080042,
-38.6174591262491));
#269518=CARTESIAN_POINT('Ctrl Pts',(-44.271274393292,29.329697893027,-38.614477863833));
#269519=CARTESIAN_POINT('Ctrl Pts',(-44.2146592782019,29.3378915995821,
-38.60568558559));
#269520=CARTESIAN_POINT('Ctrl Pts',(-44.1772069502033,29.344266758826,-38.6000392683017));
#269521=CARTESIAN_POINT('Ctrl Pts',(-44.0655444875092,29.3661148598052,
-38.5837127379559));
#269522=CARTESIAN_POINT('Ctrl Pts',(-43.9553791862171,29.3933792052515,
-38.5686255047386));
#269523=CARTESIAN_POINT('Ctrl Pts',(-43.8114622524781,29.4404829778103,
-38.5509833019505));
#269524=CARTESIAN_POINT('Ctrl Pts',(-43.705021834675,29.481230340464,-38.5390021142185));
#269525=CARTESIAN_POINT('Ctrl Pts',(-43.6350719757086,29.512061063653,-38.5318621614261));
#269526=CARTESIAN_POINT('Ctrl Pts',(-43.5656410085295,29.5447591316771,
-38.525155654825));
#269527=CARTESIAN_POINT('Ctrl Pts',(-43.5311320054746,29.5620794464364,
-38.5220163122062));
#269528=CARTESIAN_POINT('Ctrl Pts',(-43.4634866412134,29.5981758355574,
-38.5162526847879));
#269529=CARTESIAN_POINT('Ctrl Pts',(-43.4301834663392,29.6170276546,-38.5136117755133));
#269530=CARTESIAN_POINT('Ctrl Pts',(-43.3647025891651,29.6562685687332,
-38.5088155315793));
#269531=CARTESIAN_POINT('Ctrl Pts',(-43.2681192378476,29.7174608121974,
-38.5023448938576));
#269532=CARTESIAN_POINT('Ctrl Pts',(-43.1764049274077,29.7855824582168,
-38.4980286134812));
#269533=CARTESIAN_POINT('Ctrl Pts',(-43.0584774180437,29.8826126224142,
-38.4942050936184));
#269534=CARTESIAN_POINT('Ctrl Pts',(-43.001681818637,29.9342392650769,-38.4932590761897));
#269535=CARTESIAN_POINT('Ctrl Pts',(-42.8926599718677,30.0438904492243,
-38.4933742455196));
#269536=CARTESIAN_POINT('Ctrl Pts',(-42.8414047150844,30.1009342501745,
-38.4944336470273));
#269537=CARTESIAN_POINT('Ctrl Pts',(-42.7451036203247,30.2193471227021,
-38.498479276642));
#269538=CARTESIAN_POINT('Ctrl Pts',(-42.6550322643363,30.3420646399833,
-38.5044516702661));
#269539=CARTESIAN_POINT('Ctrl Pts',(-42.5773225406025,30.4733365238586,
-38.5142428327574));
#269540=CARTESIAN_POINT('Ctrl Pts',(-42.5326943378214,30.5580963840027,
-38.5215739479982));
#269541=CARTESIAN_POINT('Ctrl Pts',(-42.5239673850246,30.5751883092729,
-38.5231018165939));
#269542=CARTESIAN_POINT('Ctrl Pts',(-42.5069121510755,30.60964376351,-38.5262794637242));
#269543=CARTESIAN_POINT('Ctrl Pts',(-42.4985805781952,30.627019094627,-38.5279307934181));
#269544=CARTESIAN_POINT('Ctrl Pts',(-42.4743295471271,30.6792614198295,
-38.5330409224498));
#269545=CARTESIAN_POINT('Ctrl Pts',(-42.4438856226513,30.7493896366731,
-38.5402834483744));
#269546=CARTESIAN_POINT('Ctrl Pts',(-42.4037483179465,30.8560072598611,
-38.5524071291592));
#269547=CARTESIAN_POINT('Ctrl Pts',(-42.3690543371876,30.9640160484273,
-38.5657659376104));
#269548=CARTESIAN_POINT('Ctrl Pts',(-42.3397558527982,31.0734075527136,
-38.5803463747351));
#269549=CARTESIAN_POINT('Ctrl Pts',(-42.3238156343608,31.1472555030051,
-38.5908775753381));
#269550=CARTESIAN_POINT('Ctrl Pts',(-42.3096820427396,31.2215665449467,
-38.6018154236264));
#269551=CARTESIAN_POINT('Ctrl Pts',(-42.3035171869091,31.2589715314082,
-38.6074906718877));
#269552=CARTESIAN_POINT('Ctrl Pts',(-42.2930235524414,31.3341791410138,
-38.6192399292287));
#269553=CARTESIAN_POINT('Ctrl Pts',(-42.2886818075092,31.3721585359098,
-38.6253436316658));
#269554=CARTESIAN_POINT('Ctrl Pts',(-42.281930630611,31.4478003630713,-38.6378362101326));
#269555=CARTESIAN_POINT('Ctrl Pts',(-42.277074994566,31.5232809912004,-38.6506356205751));
#269556=CARTESIAN_POINT('Ctrl Pts',(-42.2747992363309,31.6735553614761,
-38.6774229397946));
#269557=CARTESIAN_POINT('Ctrl Pts',(-42.2834818483937,31.8228397562226,
-38.7059581415094));
#269558=CARTESIAN_POINT('Ctrl Pts',(-42.3030248127084,31.9711385758679,
-38.7362097844166));
#269559=CARTESIAN_POINT('Ctrl Pts',(-42.3164494406915,32.0449687602614,
-38.7519128032936));
#269560=CARTESIAN_POINT('Ctrl Pts',(-42.3317154579634,32.1186122141692,
-38.7679009120377));
#269561=CARTESIAN_POINT('Ctrl Pts',(-42.3402956643805,32.1554227583218,
-38.7760569897633));
#269562=CARTESIAN_POINT('Ctrl Pts',(-42.3591481714288,32.228169160774,-38.7925026060078));
#269563=CARTESIAN_POINT('Ctrl Pts',(-42.3694448348212,32.2642362896146,
-38.8008201507359));
#269564=CARTESIAN_POINT('Ctrl Pts',(-42.4028917825415,32.3714169561226,
-38.8260275044574));
#269565=CARTESIAN_POINT('Ctrl Pts',(-42.428602574983,32.4415633880281,-38.8431823298655));
#269566=CARTESIAN_POINT('Ctrl Pts',(-42.4722685042023,32.5448307979217,
-38.8694323201497));
#269567=CARTESIAN_POINT('Ctrl Pts',(-42.4876674804306,32.5789105800712,
-38.8782643966373));
#269568=CARTESIAN_POINT('Ctrl Pts',(-42.5202146590728,32.6464795812123,
-38.8961197808447));
#269569=CARTESIAN_POINT('Ctrl Pts',(-42.5373018269229,32.6798350022668,
-38.9051083126545));
#269570=CARTESIAN_POINT('Ctrl Pts',(-42.5906929412925,32.7780783962456,
-38.9321048428364));
#269571=CARTESIAN_POINT('Ctrl Pts',(-42.629225789877,32.8414173722334,-38.9502105255135));
#269572=CARTESIAN_POINT('Ctrl Pts',(-42.7120000069194,32.9638220552461,
-38.9866125955294));
#269573=CARTESIAN_POINT('Ctrl Pts',(-42.7783647966162,33.0524402968179,
-39.0140612314234));
#269574=CARTESIAN_POINT('Ctrl Pts',(-42.8754380724448,33.1642175243331,
-39.0509520337677));
#269575=CARTESIAN_POINT('Ctrl Pts',(-42.9268673384212,33.2179450225078,
-39.0694937486382));
#269576=CARTESIAN_POINT('Ctrl Pts',(-42.9797817061918,33.2705900457306,
-39.088089881442));
#269577=CARTESIAN_POINT('Ctrl Pts',(-43.0069972096607,33.2963736994336,
-39.097418269769));
#269578=CARTESIAN_POINT('Ctrl Pts',(-43.0622936398443,33.3462615369726,
-39.1159154063528));
#269579=CARTESIAN_POINT('Ctrl Pts',(-43.0904949946047,33.3704876748183,
-39.1251268688783));
#269580=CARTESIAN_POINT('Ctrl Pts',(-43.176562606447,33.4408730143712,-39.1525915568785));
#269581=CARTESIAN_POINT('Ctrl Pts',(-43.2360245534179,33.4848790444095,
-39.1707230137558));
#269582=CARTESIAN_POINT('Ctrl Pts',(-43.358992255749,33.5670176609587,-39.2066046432507));
#269583=CARTESIAN_POINT('Ctrl Pts',(-43.4542745623933,33.6242424638975,
-39.233238623837));
#269584=CARTESIAN_POINT('Ctrl Pts',(-43.5542222374601,33.6747516510336,
-39.2594493821381));
#269585=CARTESIAN_POINT('Ctrl Pts',(-43.6219256430316,33.7069073870393,
-39.2768314299875));
#269586=CARTESIAN_POINT('Ctrl Pts',(-43.6563381479934,33.7222286468184,
-39.2854811722856));
#269587=CARTESIAN_POINT('Ctrl Pts',(-43.7254519170511,33.7509934760635,
-39.3024907499371));
#269588=CARTESIAN_POINT('Ctrl Pts',(-43.7602995448845,33.7645084608315,
-39.3108885064059));
#269589=CARTESIAN_POINT('Ctrl Pts',(-43.8304781084082,33.789780836939,-39.3274499785309));
#269590=CARTESIAN_POINT('Ctrl Pts',(-43.9365171946568,33.8250735562425,
-39.3519527568515));
#269591=CARTESIAN_POINT('Ctrl Pts',(-44.0809642638621,33.8617420360433,
-39.3832806139221));
#269592=CARTESIAN_POINT('Ctrl Pts',(-44.1916183723467,33.8813683146414,
-39.4057679385072));
#269593=CARTESIAN_POINT('Ctrl Pts',(-44.2659122959159,33.8926702964892,
-39.4205323411483));
#269594=CARTESIAN_POINT('Ctrl Pts',(-44.3033049221432,33.8974288658374,
-39.4277978831022));
#269595=CARTESIAN_POINT('Ctrl Pts',(-44.3598453576919,33.9032050944765,
-39.4385322478049));
#269596=CARTESIAN_POINT('Ctrl Pts',(-44.3787527158677,33.9049006163346,
-39.4420799976889));
#269597=CARTESIAN_POINT('Ctrl Pts',(-44.4164967874688,33.9078161173588,
-39.4490791780208));
#269598=CARTESIAN_POINT('Ctrl Pts',(-44.4353708468856,33.9090400957878,
-39.4525377314439));
#269599=CARTESIAN_POINT('Ctrl Pts',(-44.4919347179527,33.9120095261765,
-39.462779235967));
#269600=CARTESIAN_POINT('Ctrl Pts',(-44.52962054914,33.9130584408517,-39.4694384189012));
#269601=CARTESIAN_POINT('Ctrl Pts',(-44.6425299001817,33.9134342925821,
-39.4889026473125));
#269602=CARTESIAN_POINT('Ctrl Pts',(-44.7176656228988,33.9100023852834,
-39.5012068570978));
#269603=CARTESIAN_POINT('Ctrl Pts',(-44.867623327666,33.8957625538083,-39.524471978366));
#269604=CARTESIAN_POINT('Ctrl Pts',(-44.9424659600731,33.8849485744664,
-39.5354353652432));
#269605=CARTESIAN_POINT('Ctrl Pts',(-45.0357885152669,33.8666999843662,
-39.5482785606344));
#269606=CARTESIAN_POINT('Ctrl Pts',(-45.0544546343785,33.8628074782943,
-39.5508053225112));
#269607=CARTESIAN_POINT('Ctrl Pts',(-45.091743102575,33.8545484160302,-39.5557691634051));
#269608=CARTESIAN_POINT('Ctrl Pts',(-45.1104022544846,33.850171655015,-39.5582107864407));
#269609=CARTESIAN_POINT('Ctrl Pts',(-45.1661672125598,33.8363538303533,
-39.5653802281989));
#269610=CARTESIAN_POINT('Ctrl Pts',(-45.2029511118778,33.8262578362557,
-39.5699395109212));
#269611=CARTESIAN_POINT('Ctrl Pts',(-45.312316831343,33.7933159380614,-39.582990524906));
#269612=CARTESIAN_POINT('Ctrl Pts',(-45.4195983160475,33.7551076509549,
-39.5947758536238));
#269613=CARTESIAN_POINT('Ctrl Pts',(-45.5585113890164,33.6937328563153,
-39.6079933748399));
#269614=CARTESIAN_POINT('Ctrl Pts',(-45.6606150024606,33.6424505696195,
-39.6166516297843));
#269615=CARTESIAN_POINT('Ctrl Pts',(-45.7272860947277,33.6047101271221,
-39.6215780075552));
#269616=CARTESIAN_POINT('Ctrl Pts',(-45.7932287365117,33.5651705839516,
-39.6260731428005));
#269617=CARTESIAN_POINT('Ctrl Pts',(-45.8259059249178,33.5444453395394,
-39.6281074988013));
#269618=CARTESIAN_POINT('Ctrl Pts',(-45.8897275017006,33.5016881508368,
-39.6316923737189));
#269619=CARTESIAN_POINT('Ctrl Pts',(-45.9210297733036,33.4795651380848,
-39.6332542688506));
#269620=CARTESIAN_POINT('Ctrl Pts',(-45.9823424846244,33.4339088874735,
-39.6359180193303));
#269621=CARTESIAN_POINT('Ctrl Pts',(-46.0724202597563,33.3632801300718,
-39.6392265347984));
#269622=CARTESIAN_POINT('Ctrl Pts',(-46.1850394564173,33.2606222983665,
-39.6409205727319));
#269623=CARTESIAN_POINT('Ctrl Pts',(-46.2638636333332,33.1772336958075,
-39.6401443034625));
#269624=CARTESIAN_POINT('Ctrl Pts',(-46.3151397511292,33.1201974856456,
-39.6391646017005));
#269625=CARTESIAN_POINT('Ctrl Pts',(-46.3401349353408,33.0909661742941,
-39.6384440851485));
#269626=CARTESIAN_POINT('Ctrl Pts',(-46.3888523044997,33.0309971480077,
-39.6365301000439));
#269627=CARTESIAN_POINT('Ctrl Pts',(-46.4123735341802,33.0005036828642,
-39.6353439924849));
#269628=CARTESIAN_POINT('Ctrl Pts',(-46.4576879006691,32.9386388625828,
-39.6325280276393));
#269629=CARTESIAN_POINT('Ctrl Pts',(-46.52311576659,32.8444620833496,-39.6276360146217));
#269630=CARTESIAN_POINT('Ctrl Pts',(-46.5810426872604,32.7462345994881,
-39.6207752343847));
#269631=CARTESIAN_POINT('Ctrl Pts',(-46.6516918187307,32.6117039458857,
-39.6098936921283));
#269632=CARTESIAN_POINT('Ctrl Pts',(-46.683723185051,32.5426422373878,-39.6035832967262));
#269633=CARTESIAN_POINT('Ctrl Pts',(-46.7195635412788,32.4540883209461,
-39.5945936116187));
#269634=CARTESIAN_POINT('Ctrl Pts',(-46.7265235775841,32.4362514419463,
-39.5927383889278));
#269635=CARTESIAN_POINT('Ctrl Pts',(-46.7400123459627,32.4003742100513,
-39.5889189813535));
#269636=CARTESIAN_POINT('Ctrl Pts',(-46.7465535157541,32.3822946053341,
-39.5869502184844));
#269637=CARTESIAN_POINT('Ctrl Pts',(-46.7654644360989,32.3279072933142,
-39.5808958427402));
#269638=CARTESIAN_POINT('Ctrl Pts',(-46.7770937339888,32.2915493874551,
-39.5766741707955));
#269639=CARTESIAN_POINT('Ctrl Pts',(-46.8091770518909,32.182013131159,-39.5634457571489));
#269640=CARTESIAN_POINT('Ctrl Pts',(-46.8444383818759,32.034891308334,-39.5443264312115));
#269641=CARTESIAN_POINT('Ctrl Pts',(-46.8650708643864,31.8856621776612,
-39.5223044891954));
#269642=CARTESIAN_POINT('Ctrl Pts',(-46.8750487417844,31.7729724844591,
-39.50469487268));
#269643=CARTESIAN_POINT('Ctrl Pts',(-46.8774570362353,31.7352651712118,
-39.4986397605723));
#269644=CARTESIAN_POINT('Ctrl Pts',(-46.8796767940079,31.6785286095959,
-39.4892824810203));
#269645=CARTESIAN_POINT('Ctrl Pts',(-46.8801843407089,31.6595724593507,
-39.4861150486293));
#269646=CARTESIAN_POINT('Ctrl Pts',(-46.8807312344332,31.6216180949417,
-39.479690628598));
#269647=CARTESIAN_POINT('Ctrl Pts',(-46.8807699646674,31.6025797052015,
-39.4764266299692));
#269648=CARTESIAN_POINT('Ctrl Pts',(-46.8801790388754,31.5455906639181,
-39.4665317368708));
#269649=CARTESIAN_POINT('Ctrl Pts',(-46.8788490796135,31.5078273383739,
-39.4598096545541));
#269650=CARTESIAN_POINT('Ctrl Pts',(-46.874360617844,31.4326451774338,-39.4461013696832));
#269651=CARTESIAN_POINT('Ctrl Pts',(-46.864884835636,31.320441459725,-39.4251517854185));
#269652=CARTESIAN_POINT('Ctrl Pts',(-46.8414902947658,31.1730719473388,
-39.3956936109857));
#269653=CARTESIAN_POINT('Ctrl Pts',(-46.8074810934279,31.0279105813681,
-39.364717848004));
#269654=CARTESIAN_POINT('Ctrl Pts',(-46.7869180083019,30.9560697433081,
-39.3487190247537));
#269655=CARTESIAN_POINT('Ctrl Pts',(-46.7645577771926,30.884604709384,-39.332461491893));
#269656=CARTESIAN_POINT('Ctrl Pts',(-46.7524740339114,30.8490466969583,
-39.3242001683612));
#269657=CARTESIAN_POINT('Ctrl Pts',(-46.7264943673172,30.7783632715819,
-39.3074248425479));
#269658=CARTESIAN_POINT('Ctrl Pts',(-46.7127058212706,30.7435263372096,
-39.2989795429224));
#269659=CARTESIAN_POINT('Ctrl Pts',(-46.6981266849492,30.7091523375488,
-39.2904704603133));
#269660=CARTESIAN_POINT('Ctrl Pts',(-45.0394875320819,30.9432190801919,
-41.190386719266));
#269661=CARTESIAN_POINT('Ctrl Pts',(-45.0282734427409,30.91723575627,-41.1733685540478));
#269662=CARTESIAN_POINT('Ctrl Pts',(-45.0034876660128,30.8666726764904,
-41.1388419648381));
#269663=CARTESIAN_POINT('Ctrl Pts',(-44.9667665375866,30.8068862988478,
-41.09447557187));
#269664=CARTESIAN_POINT('Ctrl Pts',(-44.9421458413835,30.7725558756156,
-41.0673057451311));
#269665=CARTESIAN_POINT('Ctrl Pts',(-44.9251493960809,30.7500159625169,
-41.0490682816776));
#269666=CARTESIAN_POINT('Ctrl Pts',(-44.9163654668634,30.7389260450349,
-41.0398930354472));
#269667=CARTESIAN_POINT('Ctrl Pts',(-44.8981827131164,30.7170729960788,
-41.0213934024069));
#269668=CARTESIAN_POINT('Ctrl Pts',(-44.888838333634,30.7063777841388,-41.0121255186188));
#269669=CARTESIAN_POINT('Ctrl Pts',(-44.8697378119757,30.6855401076749,
-40.9936389109155));
#269670=CARTESIAN_POINT('Ctrl Pts',(-44.8599646045333,30.6753771122426,
-40.984402815764));
#269671=CARTESIAN_POINT('Ctrl Pts',(-44.8300025766326,30.6456635434001,
-40.9567321786306));
#269672=CARTESIAN_POINT('Ctrl Pts',(-44.7987417882795,30.6174785558847,
-40.9291201070801));
#269673=CARTESIAN_POINT('Ctrl Pts',(-44.7544912812914,30.5829390177582,
-40.8924276633141));
#269674=CARTESIAN_POINT('Ctrl Pts',(-44.7200063674423,30.5585634922437,
-40.8649689008411));
#269675=CARTESIAN_POINT('Ctrl Pts',(-44.6961476159991,30.5433500948652,
-40.8467099213417));
#269676=CARTESIAN_POINT('Ctrl Pts',(-44.6779108400504,30.5323301088838,
-40.8330260113948));
#269677=CARTESIAN_POINT('Ctrl Pts',(-44.6717725199842,30.5287210947847,
-40.8284650265932));
#269678=CARTESIAN_POINT('Ctrl Pts',(-44.6594468286685,30.521672327511,-40.8193954109541));
#269679=CARTESIAN_POINT('Ctrl Pts',(-44.6532495459125,30.5182260348866,
-40.8148790968875));
#269680=CARTESIAN_POINT('Ctrl Pts',(-44.6221170703041,30.5014023919654,
-40.7924104777995));
#269681=CARTESIAN_POINT('Ctrl Pts',(-44.5712944462502,30.4770113822335,
-40.7571098106096));
#269682=CARTESIAN_POINT('Ctrl Pts',(-44.5053084694641,30.4527583886953,
-40.7146170218743));
#269683=CARTESIAN_POINT('Ctrl Pts',(-44.4645950315289,30.4410392847555,
-40.6898685245315));
#269684=CARTESIAN_POINT('Ctrl Pts',(-44.4371992237873,30.4338676574989,
-40.6735398509862));
#269685=CARTESIAN_POINT('Ctrl Pts',(-44.4233828828253,30.4306039319716,
-40.6654653393082));
#269686=CARTESIAN_POINT('Ctrl Pts',(-44.395457566773,30.4247250011004,-40.6494724436125));
#269687=CARTESIAN_POINT('Ctrl Pts',(-44.3814368244576,30.4221299378924,
-40.6416053105951));
#269688=CARTESIAN_POINT('Ctrl Pts',(-44.353398925472,30.4176419772095,-40.6261940087904));
#269689=CARTESIAN_POINT('Ctrl Pts',(-44.3393578467875,30.4157440298243,
-40.6186361329255));
#269690=CARTESIAN_POINT('Ctrl Pts',(-44.2971907773647,30.4110825461462,
-40.5964157409664));
#269691=CARTESIAN_POINT('Ctrl Pts',(-44.2690063197214,30.4093460565949,
-40.5821970282665));
#269692=CARTESIAN_POINT('Ctrl Pts',(-44.212497942469,30.4086221665927,-40.5549656043439));
#269693=CARTESIAN_POINT('Ctrl Pts',(-44.1841675064314,30.4096363406377,
-40.5419505068598));
#269694=CARTESIAN_POINT('Ctrl Pts',(-44.1486758957365,30.4126704859088,
-40.5264682752254));
#269695=CARTESIAN_POINT('Ctrl Pts',(-44.141568690144,30.4133673915631,-40.5234096239519));
#269696=CARTESIAN_POINT('Ctrl Pts',(-44.1273541295014,30.414939058346,-40.5173753852017));
#269697=CARTESIAN_POINT('Ctrl Pts',(-44.1202325648852,30.4158161528369,
-40.5143941227858));
#269698=CARTESIAN_POINT('Ctrl Pts',(-44.0989269046614,30.418710900521,-40.5056018445424));
#269699=CARTESIAN_POINT('Ctrl Pts',(-44.0848361489451,30.4209852789275,
-40.4999555272545));
#269700=CARTESIAN_POINT('Ctrl Pts',(-44.0428355440345,30.4288357011986,
-40.4836289969086));
#269701=CARTESIAN_POINT('Ctrl Pts',(-44.001418907738,30.4387301387603,-40.4685417636913));
#269702=CARTESIAN_POINT('Ctrl Pts',(-43.9473552852602,30.4559806561897,
-40.4508995609031));
#269703=CARTESIAN_POINT('Ctrl Pts',(-43.9073915907435,30.4709642266074,
-40.4389183731711));
#269704=CARTESIAN_POINT('Ctrl Pts',(-43.8811432548962,30.4823370897352,
-40.4317784203789));
#269705=CARTESIAN_POINT('Ctrl Pts',(-43.8550972458946,30.4944149327137,
-40.4250719137776));
#269706=CARTESIAN_POINT('Ctrl Pts',(-43.8421555815742,30.5008203273088,
-40.4219325711588));
#269707=CARTESIAN_POINT('Ctrl Pts',(-43.8167947927211,30.5141840584711,
-40.4161689437405));
#269708=CARTESIAN_POINT('Ctrl Pts',(-43.8043130802594,30.5211703528968,
-40.413528034466));
#269709=CARTESIAN_POINT('Ctrl Pts',(-43.7797793173031,30.5357258010655,
-40.4087317905317));
#269710=CARTESIAN_POINT('Ctrl Pts',(-43.7436043213473,30.5584424906522,
-40.4022611528103));
#269711=CARTESIAN_POINT('Ctrl Pts',(-43.7092889915882,30.583786036936,-40.397944872434));
#269712=CARTESIAN_POINT('Ctrl Pts',(-43.6651994519323,30.6199287507259,
-40.394121352571));
#269713=CARTESIAN_POINT('Ctrl Pts',(-43.6439827068456,30.6391798378995,
-40.3931753351425));
#269714=CARTESIAN_POINT('Ctrl Pts',(-43.6032932824946,30.680108587057,-40.3932905044721));
#269715=CARTESIAN_POINT('Ctrl Pts',(-43.5841829799745,30.7014201645355,
-40.3943499059801));
#269716=CARTESIAN_POINT('Ctrl Pts',(-43.5483166082379,30.7456951818503,
-40.3983955355947));
#269717=CARTESIAN_POINT('Ctrl Pts',(-43.5148120542517,30.7916143604394,
-40.4043679292189));
#269718=CARTESIAN_POINT('Ctrl Pts',(-43.4859931451963,30.8408014772341,
-40.4141590917094));
#269719=CARTESIAN_POINT('Ctrl Pts',(-43.469474574758,30.8725808034089,-40.4214902069511));
#269720=CARTESIAN_POINT('Ctrl Pts',(-43.4662461658165,30.8789901287051,
-40.4230180755467));
#269721=CARTESIAN_POINT('Ctrl Pts',(-43.4599404108544,30.8919125782622,
-40.4261957226772));
#269722=CARTESIAN_POINT('Ctrl Pts',(-43.4568618652692,30.8984301381776,
-40.4278470523708));
#269723=CARTESIAN_POINT('Ctrl Pts',(-43.4479066843131,30.9180293597941,
-40.4329571814025));
#269724=CARTESIAN_POINT('Ctrl Pts',(-43.4366800830858,30.9443463169446,
-40.440199707327));
#269725=CARTESIAN_POINT('Ctrl Pts',(-43.4219268251392,30.9843790154574,
-40.4523233881121));
#269726=CARTESIAN_POINT('Ctrl Pts',(-43.4092278315493,31.0249558361973,
-40.4656821965631));
#269727=CARTESIAN_POINT('Ctrl Pts',(-43.3985649158327,31.0660734353404,
-40.4802626336878));
#269728=CARTESIAN_POINT('Ctrl Pts',(-43.3928117504253,31.0938450909326,
-40.4907938342908));
#269729=CARTESIAN_POINT('Ctrl Pts',(-43.3877402558097,31.1217978520093,
-40.5017316825792));
#269730=CARTESIAN_POINT('Ctrl Pts',(-43.3855448869231,31.1358715333473,
-40.5074069308404));
#269731=CARTESIAN_POINT('Ctrl Pts',(-43.3818466485176,31.1641754295066,
-40.5191561881817));
#269732=CARTESIAN_POINT('Ctrl Pts',(-43.3803394900793,31.1784722137567,
-40.5252598906186));
#269733=CARTESIAN_POINT('Ctrl Pts',(-43.3780514709974,31.2069533499868,
-40.5377524690855));
#269734=CARTESIAN_POINT('Ctrl Pts',(-43.3764764291988,31.2353806198054,
-40.5505518795279));
#269735=CARTESIAN_POINT('Ctrl Pts',(-43.3761228002374,31.292003207243,-40.577339198747));
#269736=CARTESIAN_POINT('Ctrl Pts',(-43.3798904844517,31.3482922086547,
-40.6058744004623));
#269737=CARTESIAN_POINT('Ctrl Pts',(-43.3877424304871,31.4042485256067,
-40.6361260433691));
#269738=CARTESIAN_POINT('Ctrl Pts',(-43.393042276717,31.4321193306868,-40.6518290622461));
#269739=CARTESIAN_POINT('Ctrl Pts',(-43.3990345440792,31.4599262492628,
-40.6678171709904));
#269740=CARTESIAN_POINT('Ctrl Pts',(-43.4023871385948,31.4738288295879,
-40.6759732487162));
#269741=CARTESIAN_POINT('Ctrl Pts',(-43.4097262599636,31.5013102698765,
-40.6924188649606));
#269742=CARTESIAN_POINT('Ctrl Pts',(-43.4137223958007,31.5149386860624,
-40.7007364096885));
#269743=CARTESIAN_POINT('Ctrl Pts',(-43.4266697743275,31.5554481319482,
-40.7259437634106));
#269744=CARTESIAN_POINT('Ctrl Pts',(-43.4365815013438,31.5819735775504,
-40.743098588818));
#269745=CARTESIAN_POINT('Ctrl Pts',(-43.453362100664,31.6210434116697,-40.7693485791028));
#269746=CARTESIAN_POINT('Ctrl Pts',(-43.4592720436944,31.6339404199602,
-40.77818065559));
#269747=CARTESIAN_POINT('Ctrl Pts',(-43.471748387858,31.6595177912398,-40.7960360397975));
#269748=CARTESIAN_POINT('Ctrl Pts',(-43.4782913690647,31.6721475181291,
-40.8050245716083));
#269749=CARTESIAN_POINT('Ctrl Pts',(-43.4987158872668,31.7093568101663,
-40.832021101787));
#269750=CARTESIAN_POINT('Ctrl Pts',(-43.5134312848982,31.7333600460206,
-40.8501267844669));
#269751=CARTESIAN_POINT('Ctrl Pts',(-43.5449969636312,31.7797747067972,
-40.8865288544817));
#269752=CARTESIAN_POINT('Ctrl Pts',(-43.570273480101,31.8133992725601,-40.9139774903764));
#269753=CARTESIAN_POINT('Ctrl Pts',(-43.6071874842548,31.8558549470217,
-40.9508682927202));
#269754=CARTESIAN_POINT('Ctrl Pts',(-43.6267265436653,31.8762775041081,
-40.9694100075909));
#269755=CARTESIAN_POINT('Ctrl Pts',(-43.6468212761471,31.8962967826001,
-40.9880061403947));
#269756=CARTESIAN_POINT('Ctrl Pts',(-43.6571524242715,31.9061057307006,
-40.997334528722));
#269757=CARTESIAN_POINT('Ctrl Pts',(-43.6781351765956,31.9250932263188,
-41.0158316653051));
#269758=CARTESIAN_POINT('Ctrl Pts',(-43.6888325213991,31.9343181422645,
-41.0250431278314));
#269759=CARTESIAN_POINT('Ctrl Pts',(-43.7214683281725,31.961133026229,-41.0525078158304));
#269760=CARTESIAN_POINT('Ctrl Pts',(-43.744000771517,31.977916302359,-41.070639272709));
#269761=CARTESIAN_POINT('Ctrl Pts',(-43.7905699795511,32.0092811177654,
-41.106520902203));
#269762=CARTESIAN_POINT('Ctrl Pts',(-43.8266341229871,32.0311632771839,
-41.1331548827895));
#269763=CARTESIAN_POINT('Ctrl Pts',(-43.8644344365312,32.050527928199,-41.1593656410909));
#269764=CARTESIAN_POINT('Ctrl Pts',(-43.8900335656271,32.0628690313763,
-41.1767476889401));
#269765=CARTESIAN_POINT('Ctrl Pts',(-43.903042008964,32.0687560539784,-41.1853974312384));
#269766=CARTESIAN_POINT('Ctrl Pts',(-43.9291618902095,32.0798229381751,
-41.2024070088898));
#269767=CARTESIAN_POINT('Ctrl Pts',(-43.9423286751247,32.0850301956599,
-41.2108047653586));
#269768=CARTESIAN_POINT('Ctrl Pts',(-43.9688389276373,32.0947834481969,
-41.2273662374836));
#269769=CARTESIAN_POINT('Ctrl Pts',(-44.0088868242005,32.1084293286422,
-41.2518690158044));
#269770=CARTESIAN_POINT('Ctrl Pts',(-44.0634057706764,32.1227159830699,
-41.2831968728749));
#269771=CARTESIAN_POINT('Ctrl Pts',(-44.1051448739617,32.1304686073096,
-41.30568419746));
#269772=CARTESIAN_POINT('Ctrl Pts',(-44.1331632182567,32.1349666221674,
-41.3204486001008));
#269773=CARTESIAN_POINT('Ctrl Pts',(-44.1472622735965,32.1368798783668,
-41.3277141420552));
#269774=CARTESIAN_POINT('Ctrl Pts',(-44.1685768983456,32.1392377391899,
-41.3384485067576));
#269775=CARTESIAN_POINT('Ctrl Pts',(-44.1757038998442,32.1399371964,-41.3419962566417));
#269776=CARTESIAN_POINT('Ctrl Pts',(-44.1899298892594,32.1411565650423,
-41.3489954369734));
#269777=CARTESIAN_POINT('Ctrl Pts',(-44.1970429564213,32.1416781032566,
-41.3524539903966));
#269778=CARTESIAN_POINT('Ctrl Pts',(-44.2183581262916,32.1429776302475,
-41.3626954949199));
#269779=CARTESIAN_POINT('Ctrl Pts',(-44.232556678806,32.1434929542666,-41.3693546778539));
#269780=CARTESIAN_POINT('Ctrl Pts',(-44.2750884056492,32.1439936324359,
-41.3888189062651));
#269781=CARTESIAN_POINT('Ctrl Pts',(-44.3033804172497,32.1429384256622,
-41.4011231160504));
#269782=CARTESIAN_POINT('Ctrl Pts',(-44.3598247343314,32.13804594572,-41.4243882373187));
#269783=CARTESIAN_POINT('Ctrl Pts',(-44.3879848006206,32.1342064546963,
-41.4353516241949));
#269784=CARTESIAN_POINT('Ctrl Pts',(-44.4230841862873,32.1276226980045,
-41.4481948195873));
#269785=CARTESIAN_POINT('Ctrl Pts',(-44.4301039616143,32.126214419323,-41.4507215814638));
#269786=CARTESIAN_POINT('Ctrl Pts',(-44.4441256434231,32.1232190082407,
-41.455685422358));
#269787=CARTESIAN_POINT('Ctrl Pts',(-44.4511413829898,32.1216281453652,
-41.4581270453932));
#269788=CARTESIAN_POINT('Ctrl Pts',(-44.472106554004,32.1165956901708,-41.4652964871519));
#269789=CARTESIAN_POINT('Ctrl Pts',(-44.4859328208737,32.1129061786889,
-41.4698557698741));
#269790=CARTESIAN_POINT('Ctrl Pts',(-44.5270324780087,32.1008340938932,
-41.4829067838587));
#269791=CARTESIAN_POINT('Ctrl Pts',(-44.5673316800757,32.08677017453,-41.4946921125766));
#269792=CARTESIAN_POINT('Ctrl Pts',(-44.6194780799712,32.0640738471498,
-41.5079096337926));
#269793=CARTESIAN_POINT('Ctrl Pts',(-44.6577884739158,32.045065905176,-41.5165678887371));
#269794=CARTESIAN_POINT('Ctrl Pts',(-44.6827916371924,32.031050813041,-41.5214942665077));
#269795=CARTESIAN_POINT('Ctrl Pts',(-44.7075150580676,32.0163554529027,
-41.5259894017533));
#269796=CARTESIAN_POINT('Ctrl Pts',(-44.7197631353705,32.0086467826241,
-41.5280237577537));
#269797=CARTESIAN_POINT('Ctrl Pts',(-44.7436779765282,31.9927322821733,
-41.5316086326721));
#269798=CARTESIAN_POINT('Ctrl Pts',(-44.7554039451266,31.9844926239501,
-41.5331705278033));
#269799=CARTESIAN_POINT('Ctrl Pts',(-44.7783650010144,31.9674779303508,
-41.5358342782831));
#269800=CARTESIAN_POINT('Ctrl Pts',(-44.8120876763637,31.941142023486,-41.5391427937509));
#269801=CARTESIAN_POINT('Ctrl Pts',(-44.8542060542843,31.9028069711657,
-41.5408368316843));
#269802=CARTESIAN_POINT('Ctrl Pts',(-44.883650374082,31.8716290815775,-41.5400605624154));
#269803=CARTESIAN_POINT('Ctrl Pts',(-44.9027957424029,31.8502960261458,
-41.5390808606534));
#269804=CARTESIAN_POINT('Ctrl Pts',(-44.912124025092,31.8393588588263,-41.5383603441012));
#269805=CARTESIAN_POINT('Ctrl Pts',(-44.9302963003321,31.816913187918,-41.5364463589967));
#269806=CARTESIAN_POINT('Ctrl Pts',(-44.9390653236876,31.8054960967264,
-41.5352602514373));
#269807=CARTESIAN_POINT('Ctrl Pts',(-44.9559494861592,31.7823260274566,
-41.532444286592));
#269808=CARTESIAN_POINT('Ctrl Pts',(-44.9803129684955,31.7470436123751,
-41.5275522735743));
#269809=CARTESIAN_POINT('Ctrl Pts',(-45.00183725318,31.7102129370948,-41.5206914933375));
#269810=CARTESIAN_POINT('Ctrl Pts',(-45.0280427451288,31.6597446570548,
-41.5098099510806));
#269811=CARTESIAN_POINT('Ctrl Pts',(-45.0398987329805,31.6338241168053,
-41.5034995556801));
#269812=CARTESIAN_POINT('Ctrl Pts',(-45.0531290598229,31.6005723463994,
-41.4945098705711));
#269813=CARTESIAN_POINT('Ctrl Pts',(-45.0556963147994,31.5938738844661,
-41.4926546478805));
#269814=CARTESIAN_POINT('Ctrl Pts',(-45.0606676096559,31.5803990532317,
-41.4888352403062));
#269815=CARTESIAN_POINT('Ctrl Pts',(-45.0630762139805,31.5736079348959,
-41.4868664774371));
#269816=CARTESIAN_POINT('Ctrl Pts',(-45.0700329505347,31.5531765604049,
-41.4808121016924));
#269817=CARTESIAN_POINT('Ctrl Pts',(-45.0743018132827,31.5395152309552,
-41.4765904297482));
#269818=CARTESIAN_POINT('Ctrl Pts',(-45.0860497029301,31.4983488303989,
-41.4633620161014));
#269819=CARTESIAN_POINT('Ctrl Pts',(-45.0988767040151,31.4430340104486,
-41.4442426901641));
#269820=CARTESIAN_POINT('Ctrl Pts',(-45.1061818129997,31.386882792419,-41.4222207481485));
#269821=CARTESIAN_POINT('Ctrl Pts',(-45.1095857869151,31.3444641027996,
-41.4046111316328));
#269822=CARTESIAN_POINT('Ctrl Pts',(-45.1103739871937,31.3302675876129,
-41.3985560195248));
#269823=CARTESIAN_POINT('Ctrl Pts',(-45.1110306052012,31.30890259785,-41.3891987399731));
#269824=CARTESIAN_POINT('Ctrl Pts',(-45.1111617199316,31.3017636946428,
-41.3860313075819));
#269825=CARTESIAN_POINT('Ctrl Pts',(-45.1112472734604,31.2874686716035,
-41.3796068875509));
#269826=CARTESIAN_POINT('Ctrl Pts',(-45.111201351958,31.2802974166487,-41.3763428889219));
#269827=CARTESIAN_POINT('Ctrl Pts',(-45.1107973541963,31.25882908612,-41.3664479958234));
#269828=CARTESIAN_POINT('Ctrl Pts',(-45.11017580813,31.2446005169708,-41.3597259135069));
#269829=CARTESIAN_POINT('Ctrl Pts',(-45.1082442962718,31.2162677536902,
-41.3460176286356));
#269830=CARTESIAN_POINT('Ctrl Pts',(-45.104314463686,31.1739750543259,-41.3250680443717));
#269831=CARTESIAN_POINT('Ctrl Pts',(-45.0950241996196,31.1183949914011,
-41.295609869938));
#269832=CARTESIAN_POINT('Ctrl Pts',(-45.0817381040079,31.0636149263882,
-41.264634106957));
#269833=CARTESIAN_POINT('Ctrl Pts',(-45.0737554763462,31.0364928582332,
-41.2486352837062));
#269834=CARTESIAN_POINT('Ctrl Pts',(-45.0650963255467,31.0095068957897,
-41.2323777508457));
#269835=CARTESIAN_POINT('Ctrl Pts',(-45.0604265398991,30.996076905732,-41.224116427314));
#269836=CARTESIAN_POINT('Ctrl Pts',(-45.0504049610752,30.9693743366894,
-41.2073411015006));
#269837=CARTESIAN_POINT('Ctrl Pts',(-45.0450945767524,30.9562107421528,
-41.1988958018751));
#269838=CARTESIAN_POINT('Ctrl Pts',(-45.0394875320819,30.9432190801919,
-41.190386719266));
#269839=CARTESIAN_POINT('Ctrl Pts',(46.6981266907859,30.7091523367251,-39.2904704536276));
#269840=CARTESIAN_POINT('Ctrl Pts',(46.6835475544328,30.6747783369892,-39.2819613710184));
#269841=CARTESIAN_POINT('Ctrl Pts',(46.6681815018369,30.6408774253669,-39.2733909051616));
#269842=CARTESIAN_POINT('Ctrl Pts',(46.6359019286597,30.5740061528406,-39.2561284815506));
#269843=CARTESIAN_POINT('Ctrl Pts',(46.6189883221311,30.5410358432638,-39.2474365183329));
#269844=CARTESIAN_POINT('Ctrl Pts',(46.5659489438546,30.4435074270321,-39.2211791182564));
#269845=CARTESIAN_POINT('Ctrl Pts',(46.5275294448601,30.380328936116,-39.2034325197551));
#269846=CARTESIAN_POINT('Ctrl Pts',(46.4653032005596,30.2883271653987,-39.1764461155182));
#269847=CARTESIAN_POINT('Ctrl Pts',(46.4437937635959,30.2581216153683,-39.1673894794925));
#269848=CARTESIAN_POINT('Ctrl Pts',(46.399222420064,30.1986447431778,-39.1491520160392));
#269849=CARTESIAN_POINT('Ctrl Pts',(46.3761748824675,30.1693908426405,-39.1399767698089));
#269850=CARTESIAN_POINT('Ctrl Pts',(46.3284414075139,30.1117648092771,-39.1214771367686));
#269851=CARTESIAN_POINT('Ctrl Pts',(46.3038983428192,30.0835718262094,-39.1122092529802));
#269852=CARTESIAN_POINT('Ctrl Pts',(46.2537073924782,30.0286632726536,-39.0937226452772));
#269853=CARTESIAN_POINT('Ctrl Pts',(46.228014707505,30.001893562086,-39.0844865501256));
#269854=CARTESIAN_POINT('Ctrl Pts',(46.1492148056875,29.923658669611,-39.0568159129922));
#269855=CARTESIAN_POINT('Ctrl Pts',(46.0943603842992,29.874228785717,-39.0384077274207));
#269856=CARTESIAN_POINT('Ctrl Pts',(46.0086385399379,29.8041510510904,-39.0108577052895));
#269857=CARTESIAN_POINT('Ctrl Pts',(45.9794896748778,29.7814700270485,-39.00168453381));
#269858=CARTESIAN_POINT('Ctrl Pts',(45.9200349172104,29.7374728277044,-38.9833588529876));
#269859=CARTESIAN_POINT('Ctrl Pts',(45.8897290750455,29.7161565932536,-38.9742063418902));
#269860=CARTESIAN_POINT('Ctrl Pts',(45.8279451213265,29.6749068315954,-38.9559225560557));
#269861=CARTESIAN_POINT('Ctrl Pts',(45.7964751128047,29.6549785787194,-38.9467936557034));
#269862=CARTESIAN_POINT('Ctrl Pts',(45.7483486075838,29.6261284918058,-38.9331097457563));
#269863=CARTESIAN_POINT('Ctrl Pts',(45.7321473321371,29.6166840488636,-38.9285487609545));
#269864=CARTESIAN_POINT('Ctrl Pts',(45.6996106239914,29.5982459944737,-38.9194791453156));
#269865=CARTESIAN_POINT('Ctrl Pts',(45.6832490479695,29.5892352416054,-38.9149628312498));
#269866=CARTESIAN_POINT('Ctrl Pts',(45.601043919029,29.5452683980011,-38.8924942121586));
#269867=CARTESIAN_POINT('Ctrl Pts',(45.5339075028974,29.5134615269732,-38.8748432905736));
#269868=CARTESIAN_POINT('Ctrl Pts',(45.3969715912008,29.4565064904797,-38.8401971286172));
#269869=CARTESIAN_POINT('Ctrl Pts',(45.3271662968287,29.4313508095901,-38.8231995362783));
#269870=CARTESIAN_POINT('Ctrl Pts',(45.2204298468913,29.3986526373661,-38.7982016653842));
#269871=CARTESIAN_POINT('Ctrl Pts',(45.1845124401493,29.3885937216909,-38.7899522588935));
#269872=CARTESIAN_POINT('Ctrl Pts',(45.1119891491544,29.3701842504182,-38.7736235853476));
#269873=CARTESIAN_POINT('Ctrl Pts',(45.0754052601759,29.3618381477176,-38.7655490736698));
#269874=CARTESIAN_POINT('Ctrl Pts',(45.0014447954028,29.3468760796426,-38.7495561779739));
#269875=CARTESIAN_POINT('Ctrl Pts',(44.964301865418,29.3403115524284,-38.7416890449567));
#269876=CARTESIAN_POINT('Ctrl Pts',(44.8900079613448,29.3290481853876,-38.7262777431523));
#269877=CARTESIAN_POINT('Ctrl Pts',(44.8527936300225,29.3243364917773,-38.7187198672871));
#269878=CARTESIAN_POINT('Ctrl Pts',(44.7410083388884,29.3129455696646,-38.6964994753282));
#269879=CARTESIAN_POINT('Ctrl Pts',(44.6662563771146,29.3089967383529,-38.6822807626282));
#269880=CARTESIAN_POINT('Ctrl Pts',(44.5163124694972,29.3084067895486,-38.6550493387052));
#269881=CARTESIAN_POINT('Ctrl Pts',(44.4411031904291,29.3117700104783,-38.6420342412209));
#269882=CARTESIAN_POINT('Ctrl Pts',(44.3468378622929,29.3206690016762,-38.6265520095871));
#269883=CARTESIAN_POINT('Ctrl Pts',(44.3279589155214,29.3226883277488,-38.6234933583131));
#269884=CARTESIAN_POINT('Ctrl Pts',(44.2901960658791,29.3271995041764,-38.6174591195633));
#269885=CARTESIAN_POINT('Ctrl Pts',(44.2712743938236,29.3296978892051,-38.6144778571473));
#269886=CARTESIAN_POINT('Ctrl Pts',(44.2146592786091,29.3378915957788,-38.6056855789043));
#269887=CARTESIAN_POINT('Ctrl Pts',(44.1772069505284,29.344266755037,-38.600039261616));
#269888=CARTESIAN_POINT('Ctrl Pts',(44.1027653085689,29.3588321557227,-38.5891549080521));
#269889=CARTESIAN_POINT('Ctrl Pts',(44.0657945489821,29.3670194923296,-38.5839197136818));
#269890=CARTESIAN_POINT('Ctrl Pts',(43.9923490655734,29.3851891984824,-38.5738612386265));
#269891=CARTESIAN_POINT('Ctrl Pts',(43.9558743462093,29.3951715837984,-38.5690379607699));
#269892=CARTESIAN_POINT('Ctrl Pts',(43.8834205273202,29.4169303960524,-38.5598042413246));
#269893=CARTESIAN_POINT('Ctrl Pts',(43.8474414247684,29.4287068117428,-38.5553937964858));
#269894=CARTESIAN_POINT('Ctrl Pts',(43.7759820581033,29.4540658159891,-38.5469896253478));
#269895=CARTESIAN_POINT('Ctrl Pts',(43.7405017832129,29.467648365304,-38.5429958894628));
#269896=CARTESIAN_POINT('Ctrl Pts',(43.6700470469744,29.4966453366817,-38.5354320916221));
#269897=CARTESIAN_POINT('Ctrl Pts',(43.6350719748427,29.5120610602386,-38.5318621547404));
#269898=CARTESIAN_POINT('Ctrl Pts',(43.5656410075109,29.5447591283353,-38.5251556481393));
#269899=CARTESIAN_POINT('Ctrl Pts',(43.5311320043801,29.562079443133,-38.5220163055204));
#269900=CARTESIAN_POINT('Ctrl Pts',(43.4634866399702,29.598175832334,-38.5162526781022));
#269901=CARTESIAN_POINT('Ctrl Pts',(43.4301834650226,29.6170276514184,-38.5136117688276));
#269902=CARTESIAN_POINT('Ctrl Pts',(43.3647025877044,29.6562685656384,-38.5088155248935));
#269903=CARTESIAN_POINT('Ctrl Pts',(43.3325078216452,29.6766655508507,-38.5066585142211));
#269904=CARTESIAN_POINT('Ctrl Pts',(43.2375484303922,29.7401688832699,-38.5009063899101));
#269905=CARTESIAN_POINT('Ctrl Pts',(43.1764049255325,29.7855824554079,-38.4980286067954));
#269906=CARTESIAN_POINT('Ctrl Pts',(43.0584774159086,29.8826126198196,-38.4942050869327));
#269907=CARTESIAN_POINT('Ctrl Pts',(43.0016818163768,29.9342392625963,-38.4932590695039));
#269908=CARTESIAN_POINT('Ctrl Pts',(42.892659969367,30.0438904469854,-38.4933742388339));
#269909=CARTESIAN_POINT('Ctrl Pts',(42.8414047124706,30.1009342480614,-38.4944336403416));
#269910=CARTESIAN_POINT('Ctrl Pts',(42.7451036174982,30.21934712085,-38.4984792699563));
#269911=CARTESIAN_POINT('Ctrl Pts',(42.7000684081338,30.2807072600243,-38.5014658059356));
#269912=CARTESIAN_POINT('Ctrl Pts',(42.6161769306285,30.4076992000848,-38.5093469056588));
#269913=CARTESIAN_POINT('Ctrl Pts',(42.577322537405,30.4733365225655,-38.5142428260717));
#269914=CARTESIAN_POINT('Ctrl Pts',(42.5326943345249,30.558096382896,-38.5215739413125));
#269915=CARTESIAN_POINT('Ctrl Pts',(42.5239673817088,30.5751883082038,-38.5231018099081));
#269916=CARTESIAN_POINT('Ctrl Pts',(42.5069121477218,30.6096437625167,-38.5262794570385));
#269917=CARTESIAN_POINT('Ctrl Pts',(42.498580574823,30.627019093672,-38.5279307867324));
#269918=CARTESIAN_POINT('Ctrl Pts',(42.4743295437012,30.6792614189893,-38.5330409157641));
#269919=CARTESIAN_POINT('Ctrl Pts',(42.4591078014939,30.7143247165074,-38.5366620710225));
#269920=CARTESIAN_POINT('Ctrl Pts',(42.4305062686555,30.7849297919355,-38.5443247961378));
#269921=CARTESIAN_POINT('Ctrl Pts',(42.4171273582822,30.8204683259224,-38.5483659351791));
#269922=CARTESIAN_POINT('Ctrl Pts',(42.3921837076412,30.8920099497574,-38.5568600247503));
#269923=CARTESIAN_POINT('Ctrl Pts',(42.3806190143997,30.9280130515862,-38.561312986478));
#269924=CARTESIAN_POINT('Ctrl Pts',(42.3592881526269,31.0004799413282,-38.5706260837038));
#269925=CARTESIAN_POINT('Ctrl Pts',(42.3495220026171,31.0369437339053,-38.5754862240386));
#269926=CARTESIAN_POINT('Ctrl Pts',(42.3317857457909,31.1103315159601,-38.5856119670777));
#269927=CARTESIAN_POINT('Ctrl Pts',(42.3238156305991,31.147255503193,-38.5908775686523));
#269928=CARTESIAN_POINT('Ctrl Pts',(42.309682038946,31.2215665452978,-38.6018154169406));
#269929=CARTESIAN_POINT('Ctrl Pts',(42.3035171831015,31.2589715318414,-38.607490665202));
#269930=CARTESIAN_POINT('Ctrl Pts',(42.2930235486099,31.334179141612,-38.619239922543));
#269931=CARTESIAN_POINT('Ctrl Pts',(42.2886818036678,31.3721585365914,-38.6253436249801));
#269932=CARTESIAN_POINT('Ctrl Pts',(42.2819306267537,31.4478003639188,-38.6378362034469));
#269933=CARTESIAN_POINT('Ctrl Pts',(42.2795025198556,31.4855414987872,-38.6442360062361));
#269934=CARTESIAN_POINT('Ctrl Pts',(42.2765060604552,31.5608485908284,-38.6573322655641));
#269935=CARTESIAN_POINT('Ctrl Pts',(42.2759365524734,31.5984178308852,-38.6640291123748));
#269936=CARTESIAN_POINT('Ctrl Pts',(42.2769710577917,31.7108769179205,-38.6845570238621));
#269937=CARTESIAN_POINT('Ctrl Pts',(42.2813124720526,31.7855186416003,-38.6988245608712));
#269938=CARTESIAN_POINT('Ctrl Pts',(42.2932531065375,31.896990615329,-38.7210841762227));
#269939=CARTESIAN_POINT('Ctrl Pts',(42.2981395912299,31.9340660323646,-38.7286473479064));
#269940=CARTESIAN_POINT('Ctrl Pts',(42.3097367739455,32.0080522304774,-38.7440609665678));
#269941=CARTESIAN_POINT('Ctrl Pts',(42.3164494369031,32.0449687624179,-38.7519127966078));
#269942=CARTESIAN_POINT('Ctrl Pts',(42.3317154542076,32.1186122164871,-38.767900905352));
#269943=CARTESIAN_POINT('Ctrl Pts',(42.340295660643,32.1554227607203,-38.7760569830776));
#269944=CARTESIAN_POINT('Ctrl Pts',(42.3591481677318,32.2281691633317,-38.792502599322));
#269945=CARTESIAN_POINT('Ctrl Pts',(42.3694448311464,32.2642362922514,-38.8008201440502));
#269946=CARTESIAN_POINT('Ctrl Pts',(42.3917427963414,32.3356900700797,-38.8176250465312));
#269947=CARTESIAN_POINT('Ctrl Pts',(42.4037465114866,32.3710895355311,-38.826115145426));
#269948=CARTESIAN_POINT('Ctrl Pts',(42.4294540504939,32.4412374324299,-38.8432687814672));
#269949=CARTESIAN_POINT('Ctrl Pts',(42.4431578812073,32.4759858610929,-38.8519323199412));
#269950=CARTESIAN_POINT('Ctrl Pts',(42.4722685007499,32.5448308011725,-38.869432313464));
#269951=CARTESIAN_POINT('Ctrl Pts',(42.4876674770116,32.5789105833965,-38.8782643899516));
#269952=CARTESIAN_POINT('Ctrl Pts',(42.5202146557244,32.6464795846854,-38.896119774159));
#269953=CARTESIAN_POINT('Ctrl Pts',(42.5373018236116,32.6798350058129,-38.9051083059688));
#269954=CARTESIAN_POINT('Ctrl Pts',(42.5906929380972,32.7780784000063,-38.9321048361507));
#269955=CARTESIAN_POINT('Ctrl Pts',(42.6292257867655,32.8414173761326,-38.9502105188277));
#269956=CARTESIAN_POINT('Ctrl Pts',(42.7120000039881,32.9638220594128,-38.9866125888437));
#269957=CARTESIAN_POINT('Ctrl Pts',(42.75624392991,33.0229003398858,-39.0049117127868));
#269958=CARTESIAN_POINT('Ctrl Pts',(42.8269002174294,33.1083282810888,-39.0325062982755));
#269959=CARTESIAN_POINT('Ctrl Pts',(42.85116847875,33.1362718605164,-39.0417288600547));
#269960=CARTESIAN_POINT('Ctrl Pts',(42.9011535509872,33.1910821857371,-39.060223195478));
#269961=CARTESIAN_POINT('Ctrl Pts',(42.9268673359585,33.2179450272291,-39.0694937419525));
#269962=CARTESIAN_POINT('Ctrl Pts',(42.9797817038445,33.2705900505667,-39.0880898747562));
#269963=CARTESIAN_POINT('Ctrl Pts',(43.0069972073728,33.296373704326,-39.0974182630833));
#269964=CARTESIAN_POINT('Ctrl Pts',(43.0622936376772,33.3462615419736,-39.1159153996671));
#269965=CARTESIAN_POINT('Ctrl Pts',(43.0904949924992,33.3704876798722,-39.1251268621925));
#269966=CARTESIAN_POINT('Ctrl Pts',(43.1765626045295,33.4408730195783,-39.1525915501928));
#269967=CARTESIAN_POINT('Ctrl Pts',(43.2360245516304,33.4848790497124,-39.1707230070701));
#269968=CARTESIAN_POINT('Ctrl Pts',(43.3282503285803,33.5464830122584,-39.1976342291912));
#269969=CARTESIAN_POINT('Ctrl Pts',(43.3595022250126,33.5662859422569,-39.2065581988407));
#269970=CARTESIAN_POINT('Ctrl Pts',(43.4230323983204,33.6044188752118,-39.224313204774));
#269971=CARTESIAN_POINT('Ctrl Pts',(43.4553106306814,33.6227489424813,-39.2331442440926));
#269972=CARTESIAN_POINT('Ctrl Pts',(43.5209070235488,33.6579164289522,-39.2507127796806));
#269973=CARTESIAN_POINT('Ctrl Pts',(43.5542222363685,33.6747516567492,-39.2594493754524));
#269974=CARTESIAN_POINT('Ctrl Pts',(43.6219256420881,33.7069073928245,-39.2768314233018));
#269975=CARTESIAN_POINT('Ctrl Pts',(43.6563381471253,33.7222286526369,-39.2854811655998));
#269976=CARTESIAN_POINT('Ctrl Pts',(43.7254519163343,33.7509934819442,-39.3024907432514));
#269977=CARTESIAN_POINT('Ctrl Pts',(43.760299544244,33.7645084667414,-39.3108884997202));
#269978=CARTESIAN_POINT('Ctrl Pts',(43.8304781079213,33.7897808429036,-39.3274499718452));
#269979=CARTESIAN_POINT('Ctrl Pts',(43.8658243281891,33.8015455663885,-39.3356176240585));
#269980=CARTESIAN_POINT('Ctrl Pts',(43.9726293605948,33.8342393235301,-39.3597845464139));
#269981=CARTESIAN_POINT('Ctrl Pts',(44.0448528416252,33.8525737481731,-39.3754484955492));
#269982=CARTESIAN_POINT('Ctrl Pts',(44.1547335163723,33.8748267497094,-39.3982722224796));
#269983=CARTESIAN_POINT('Ctrl Pts',(44.191618372651,33.8813683208027,-39.4057679318215));
#269984=CARTESIAN_POINT('Ctrl Pts',(44.2659122963829,33.8926703026745,-39.4205323344626));
#269985=CARTESIAN_POINT('Ctrl Pts',(44.3033049226923,33.8974288720327,-39.4277978764165));
#269986=CARTESIAN_POINT('Ctrl Pts',(44.359845358365,33.9032051006838,-39.4385322411192));
#269987=CARTESIAN_POINT('Ctrl Pts',(44.3787527165822,33.9049006225454,-39.4420799910032));
#269988=CARTESIAN_POINT('Ctrl Pts',(44.4164967882661,33.9078161235755,-39.449079171335));
#269989=CARTESIAN_POINT('Ctrl Pts',(44.4353708477243,33.9090401020071,-39.4525377247581));
#269990=CARTESIAN_POINT('Ctrl Pts',(44.4919347189154,33.9120095324017,-39.4627792292813));
#269991=CARTESIAN_POINT('Ctrl Pts',(44.5296205501853,33.9130584470787,-39.4694384122155));
#269992=CARTESIAN_POINT('Ctrl Pts',(44.6425299014747,33.9134342988086,-39.4889026406268));
#269993=CARTESIAN_POINT('Ctrl Pts',(44.7176656243566,33.9100023915017,-39.501206850412));
#269994=CARTESIAN_POINT('Ctrl Pts',(44.8676233294529,33.8957625599936,-39.5244719716803));
#269995=CARTESIAN_POINT('Ctrl Pts',(44.9424659620243,33.8849485806272,-39.5354353585575));
#269996=CARTESIAN_POINT('Ctrl Pts',(45.035788517423,33.8666999904859,-39.5482785539486));
#269997=CARTESIAN_POINT('Ctrl Pts',(45.0544546365756,33.8628074844052,-39.5508053158255));
#269998=CARTESIAN_POINT('Ctrl Pts',(45.091743104854,33.8545484221227,-39.5557691567194));
#269999=CARTESIAN_POINT('Ctrl Pts',(45.1104022568045,33.8501716610976,-39.5582107797549));
#270000=CARTESIAN_POINT('Ctrl Pts',(45.1661672150022,33.836353836405,-39.5653802215133));
#270001=CARTESIAN_POINT('Ctrl Pts',(45.202951114401,33.8262578422849,-39.5699395042355));
#270002=CARTESIAN_POINT('Ctrl Pts',(45.2758615942045,33.804296576773,-39.5786401802253));
#270003=CARTESIAN_POINT('Ctrl Pts',(45.3119687162999,33.7924363258948,-39.5827791057116));
#270004=CARTESIAN_POINT('Ctrl Pts',(45.3834929107785,33.76697243113,-39.5906388608178));
#270005=CARTESIAN_POINT('Ctrl Pts',(45.4189099756201,33.7533687680179,-39.5943596850842));
#270006=CARTESIAN_POINT('Ctrl Pts',(45.4890551228987,33.7244209358064,-39.6013847741846));
#270007=CARTESIAN_POINT('Ctrl Pts',(45.5237832082604,33.7090767739723,-39.6046890401843));
#270008=CARTESIAN_POINT('Ctrl Pts',(45.5925464222574,33.6766380727023,-39.6108794174069));
#270009=CARTESIAN_POINT('Ctrl Pts',(45.6265815645382,33.6595435676593,-39.6137655364386));
#270010=CARTESIAN_POINT('Ctrl Pts',(45.6939497298677,33.6235811813386,-39.6191148132429));
#270011=CARTESIAN_POINT('Ctrl Pts',(45.7272860984032,33.6047101326598,-39.6215780008695));
#270012=CARTESIAN_POINT('Ctrl Pts',(45.7932287403323,33.5651705894019,-39.6260731361148));
#270013=CARTESIAN_POINT('Ctrl Pts',(45.8259059288103,33.5444453449438,-39.6281074921155));
#270014=CARTESIAN_POINT('Ctrl Pts',(45.8897275057335,33.5016881561468,-39.6316923670332));
#270015=CARTESIAN_POINT('Ctrl Pts',(45.9210297774054,33.4795651433458,-39.6332542621649));
#270016=CARTESIAN_POINT('Ctrl Pts',(45.9823424888611,33.4339088926338,-39.6359180126446));
#270017=CARTESIAN_POINT('Ctrl Pts',(46.0123687663031,33.4103663730771,-39.6370209832341));
#270018=CARTESIAN_POINT('Ctrl Pts',(46.1005740614019,33.3376145406148,-39.6396496617403));
#270019=CARTESIAN_POINT('Ctrl Pts',(46.1568837698145,33.2862857494669,-39.6404967215965));
#270020=CARTESIAN_POINT('Ctrl Pts',(46.2375893089641,33.2050303509431,-39.6404032020738));
#270021=CARTESIAN_POINT('Ctrl Pts',(46.2638636381901,33.1772337004019,-39.6401442967768));
#270022=CARTESIAN_POINT('Ctrl Pts',(46.3151397560992,33.1201974901143,-39.6391645950147));
#270023=CARTESIAN_POINT('Ctrl Pts',(46.3401349403659,33.0909661786984,-39.6384440784628));
#270024=CARTESIAN_POINT('Ctrl Pts',(46.3888523096323,33.03099715228,-39.6365300933582));
#270025=CARTESIAN_POINT('Ctrl Pts',(46.4123735393647,33.0005036870694,-39.6353439857992));
#270026=CARTESIAN_POINT('Ctrl Pts',(46.4576879059536,32.9386388666518,-39.6325280209535));
#270027=CARTESIAN_POINT('Ctrl Pts',(46.4794979921318,32.9072463868165,-39.6308974524097));
#270028=CARTESIAN_POINT('Ctrl Pts',(46.5424231506391,32.8117200325625,-39.6253488762663));
#270029=CARTESIAN_POINT('Ctrl Pts',(46.5810426928175,32.7462346031338,-39.620775227699));
#270030=CARTESIAN_POINT('Ctrl Pts',(46.6516918244441,32.6117039492356,-39.6098936854426));
#270031=CARTESIAN_POINT('Ctrl Pts',(46.6837231908355,32.5426422405858,-39.6035832900405));
#270032=CARTESIAN_POINT('Ctrl Pts',(46.7195635471429,32.4540883239497,-39.594593604933));
#270033=CARTESIAN_POINT('Ctrl Pts',(46.7265235834636,32.4362514449106,-39.592738382242));
#270034=CARTESIAN_POINT('Ctrl Pts',(46.7400123518722,32.4003742129367,-39.5889189746678));
#270035=CARTESIAN_POINT('Ctrl Pts',(46.7465535216782,32.3822946081798,-39.5869502117987));
#270036=CARTESIAN_POINT('Ctrl Pts',(46.765464442065,32.3279072960404,-39.5808958360545));
#270037=CARTESIAN_POINT('Ctrl Pts',(46.7770937399808,32.2915493901016,-39.5766741641098));
#270038=CARTESIAN_POINT('Ctrl Pts',(46.7984826186299,32.218525219077,-39.5678552216787));
#270039=CARTESIAN_POINT('Ctrl Pts',(46.8082357029931,32.1818782650522,-39.5632601386704));
#270040=CARTESIAN_POINT('Ctrl Pts',(46.8258916183201,32.1083194058768,-39.5537041697811));
#270041=CARTESIAN_POINT('Ctrl Pts',(46.8337943402473,32.0714074849882,-39.5487432633557));
#270042=CARTESIAN_POINT('Ctrl Pts',(46.8547548479309,31.9602784803845,-39.5333157848068));
#270043=CARTESIAN_POINT('Ctrl Pts',(46.8650708705757,31.8856621794164,-39.5223044825097));
#270044=CARTESIAN_POINT('Ctrl Pts',(46.875048747997,31.772972485967,-39.5046948659943));
#270045=CARTESIAN_POINT('Ctrl Pts',(46.8774570424536,31.7352651726369,-39.4986397538865));
#270046=CARTESIAN_POINT('Ctrl Pts',(46.8796768002317,31.6785286108966,-39.4892824743346));
#270047=CARTESIAN_POINT('Ctrl Pts',(46.880184346934,31.6595724606098,-39.4861150419436));
#270048=CARTESIAN_POINT('Ctrl Pts',(46.88073124066,31.6216180961176,-39.4796906219123));
#270049=CARTESIAN_POINT('Ctrl Pts',(46.8807699708944,31.6025797063356,-39.4764266232835));
#270050=CARTESIAN_POINT('Ctrl Pts',(46.8801790451018,31.5455906649272,-39.4665317301851));
#270051=CARTESIAN_POINT('Ctrl Pts',(46.8788490858374,31.5078273393001,-39.4598096478684));
#270052=CARTESIAN_POINT('Ctrl Pts',(46.8743606240589,31.4326451781951,-39.4461013629975));
#270053=CARTESIAN_POINT('Ctrl Pts',(46.8712024781441,31.395243845809,-39.4391182314914));
#270054=CARTESIAN_POINT('Ctrl Pts',(46.859034876608,31.2835993580034,-39.4177870486965));
#270055=CARTESIAN_POINT('Ctrl Pts',(46.8473376351276,31.2099145951219,-39.4030579681171));
#270056=CARTESIAN_POINT('Ctrl Pts',(46.8244864012849,31.100491008194,-39.3802058007947));
#270057=CARTESIAN_POINT('Ctrl Pts',(46.8159835841289,31.0642007181343,-39.3724617791813));
#270058=CARTESIAN_POINT('Ctrl Pts',(46.7971994340653,30.9919902985873,-39.3567184316147));
#270059=CARTESIAN_POINT('Ctrl Pts',(46.7869180143304,30.9560697430251,-39.348719018068));
#270060=CARTESIAN_POINT('Ctrl Pts',(46.7645577831729,30.8846047089445,-39.3324614852073));
#270061=CARTESIAN_POINT('Ctrl Pts',(46.7524740398656,30.8490466964409,-39.3242001616755));
#270062=CARTESIAN_POINT('Ctrl Pts',(46.7264943732153,30.7783632709098,-39.3074248358622));
#270063=CARTESIAN_POINT('Ctrl Pts',(46.7127058271388,30.7435263364611,-39.2989795362367));
#270064=CARTESIAN_POINT('Ctrl Pts',(46.6981266907859,30.7091523367251,-39.2904704536276));
#270065=CARTESIAN_POINT('Ctrl Pts',(46.3487330454107,30.7584586806226,-39.6906893116447));
#270066=CARTESIAN_POINT('Ctrl Pts',(46.3360438872384,30.7285888871829,-39.6821802290355));
#270067=CARTESIAN_POINT('Ctrl Pts',(46.3226713842648,30.6991295511679,-39.6736097631786));
#270068=CARTESIAN_POINT('Ctrl Pts',(46.2945825861103,30.6410182279319,-39.6563473395677));
#270069=CARTESIAN_POINT('Ctrl Pts',(46.2798662162942,30.6123662852523,-39.64765537635));
#270070=CARTESIAN_POINT('Ctrl Pts',(46.2337210871567,30.527609915333,-39.6213979762735));
#270071=CARTESIAN_POINT('Ctrl Pts',(46.2003005032305,30.4727024332251,-39.6036513777721));
#270072=CARTESIAN_POINT('Ctrl Pts',(46.1461777229336,30.3927408835902,-39.5766649735353));
#270073=CARTESIAN_POINT('Ctrl Pts',(46.1274704458576,30.3664875975353,-39.5676083375096));
#270074=CARTESIAN_POINT('Ctrl Pts',(46.0887077763598,30.3147915248746,-39.5493708740563));
#270075=CARTESIAN_POINT('Ctrl Pts',(46.0686648791047,30.2893638816766,-39.5401956278259));
#270076=CARTESIAN_POINT('Ctrl Pts',(46.0271562868518,30.2392734556588,-39.5216959947856));
#270077=CARTESIAN_POINT('Ctrl Pts',(46.0058148371699,30.2147663918631,-39.5124281109973));
#270078=CARTESIAN_POINT('Ctrl Pts',(45.9621731101223,30.167034895406,-39.4939415032943));
#270079=CARTESIAN_POINT('Ctrl Pts',(45.9398338756316,30.1437634024636,-39.4847054081427));
#270080=CARTESIAN_POINT('Ctrl Pts',(45.8713217104267,30.0757495650345,-39.4570347710093));
#270081=CARTESIAN_POINT('Ctrl Pts',(45.8236322612105,30.0327740175956,-39.4386265854377));
#270082=CARTESIAN_POINT('Ctrl Pts',(45.7491121861247,29.9718412271654,-39.4110765633066));
#270083=CARTESIAN_POINT('Ctrl Pts',(45.7237731661291,29.9521190412175,-39.4019033918271));
#270084=CARTESIAN_POINT('Ctrl Pts',(45.6720909021616,29.9138594468863,-39.3835777110047));
#270085=CARTESIAN_POINT('Ctrl Pts',(45.6457477019571,29.8953219871642,-39.3744251999072));
#270086=CARTESIAN_POINT('Ctrl Pts',(45.5920438586766,29.85944733933,-39.3561414140728));
#270087=CARTESIAN_POINT('Ctrl Pts',(45.5646902588189,29.8421147384108,-39.3470125137204));
#270088=CARTESIAN_POINT('Ctrl Pts',(45.5228600486148,29.8170205763042,-39.3333286037734));
#270089=CARTESIAN_POINT('Ctrl Pts',(45.5087785426461,29.8088053710447,-39.3287676189716));
#270090=CARTESIAN_POINT('Ctrl Pts',(45.4804993011169,29.7927664789577,-39.3196980033327));
#270091=CARTESIAN_POINT('Ctrl Pts',(45.4662788414783,29.7849278840232,-39.3151816892667));
#270092=CARTESIAN_POINT('Ctrl Pts',(45.3948322071948,29.7466787770249,-39.2927130701762));
#270093=CARTESIAN_POINT('Ctrl Pts',(45.336485100633,29.7190029057417,-39.2750621485905));
#270094=CARTESIAN_POINT('Ctrl Pts',(45.2174821634192,29.6694332894901,-39.2404159866344));
#270095=CARTESIAN_POINT('Ctrl Pts',(45.1568212895685,29.647533012283,-39.2234183942954));
#270096=CARTESIAN_POINT('Ctrl Pts',(45.0640714235939,29.619055039813,-39.1984205234013));
#270097=CARTESIAN_POINT('Ctrl Pts',(45.032861270908,29.6102922086151,-39.1901711169105));
#270098=CARTESIAN_POINT('Ctrl Pts',(44.9698441198096,29.5942499980371,-39.1738424433647));
#270099=CARTESIAN_POINT('Ctrl Pts',(44.9380562327559,29.5869745020916,-39.1657679316868));
#270100=CARTESIAN_POINT('Ctrl Pts',(44.8737931083252,29.573925804024,-39.149775035991));
#270101=CARTESIAN_POINT('Ctrl Pts',(44.8415208853874,29.5681974475295,-39.1419079029737));
#270102=CARTESIAN_POINT('Ctrl Pts',(44.776970845224,29.5583613251754,-39.1264966011694));
#270103=CARTESIAN_POINT('Ctrl Pts',(44.7446379778246,29.554242349424,-39.1189387253041));
#270104=CARTESIAN_POINT('Ctrl Pts',(44.6475178199358,29.5442689888186,-39.0967183333452));
#270105=CARTESIAN_POINT('Ctrl Pts',(44.5825753395907,29.5407861890414,-39.0824996206453));
#270106=CARTESIAN_POINT('Ctrl Pts',(44.4523137000486,29.5401680254183,-39.0552681967223));
#270107=CARTESIAN_POINT('Ctrl Pts',(44.3869794861938,29.5430364177713,-39.042253099238));
#270108=CARTESIAN_POINT('Ctrl Pts',(44.3050948879356,29.5506999745547,-39.0267708676041));
#270109=CARTESIAN_POINT('Ctrl Pts',(44.2886956677166,29.5524407317244,-39.0237122163303));
#270110=CARTESIAN_POINT('Ctrl Pts',(44.2558932837023,29.5563326981298,-39.0176779775804));
#270111=CARTESIAN_POINT('Ctrl Pts',(44.2394573135744,29.5584895570295,-39.0146967151644));
#270112=CARTESIAN_POINT('Ctrl Pts',(44.1902801628687,29.5655670337388,-39.0059044369212));
#270113=CARTESIAN_POINT('Ctrl Pts',(44.1577489684097,29.5710783602803,-39.0002581196331));
#270114=CARTESIAN_POINT('Ctrl Pts',(44.0930902099635,29.5836780129281,-38.9893737660692));
#270115=CARTESIAN_POINT('Ctrl Pts',(44.0609787624772,29.5907638288663,-38.9841385716989));
#270116=CARTESIAN_POINT('Ctrl Pts',(43.9971881707919,29.6064950769681,-38.9740800966435));
#270117=CARTESIAN_POINT('Ctrl Pts',(43.9655090304771,29.6151405228279,-38.969256818787));
#270118=CARTESIAN_POINT('Ctrl Pts',(43.9025826910914,29.6339901792778,-38.9600230993416));
#270119=CARTESIAN_POINT('Ctrl Pts',(43.8713354893841,29.6441943800886,-38.9556126545029));
#270120=CARTESIAN_POINT('Ctrl Pts',(43.8092758314442,29.6661720973477,-38.9472084833648));
#270121=CARTESIAN_POINT('Ctrl Pts',(43.7784633658234,29.6779455796926,-38.9432147474799));
#270122=CARTESIAN_POINT('Ctrl Pts',(43.7172792568189,29.7030842010437,-38.9356509496391));
#270123=CARTESIAN_POINT('Ctrl Pts',(43.6869070838288,29.7164504701877,-38.9320810127575));
#270124=CARTESIAN_POINT('Ctrl Pts',(43.6266151921457,29.7448048716196,-38.9253745061563));
#270125=CARTESIAN_POINT('Ctrl Pts',(43.5966493659251,29.7598259498784,-38.9222351635375));
#270126=CARTESIAN_POINT('Ctrl Pts',(43.5379112806659,29.7911336867559,-38.9164715361192));
#270127=CARTESIAN_POINT('Ctrl Pts',(43.5089941631931,29.8074860237238,-38.9138306268446));
#270128=CARTESIAN_POINT('Ctrl Pts',(43.4521388277713,29.8415269250742,-38.9090343829106));
#270129=CARTESIAN_POINT('Ctrl Pts',(43.4241857920873,29.8592223311679,-38.9068773722382));
#270130=CARTESIAN_POINT('Ctrl Pts',(43.3417400360357,29.9143184778597,-38.9011252479271));
#270131=CARTESIAN_POINT('Ctrl Pts',(43.2886573738269,29.9537246686422,-38.8982474648125));
#270132=CARTESIAN_POINT('Ctrl Pts',(43.1862838907427,30.0379288436163,-38.8944239449498));
#270133=CARTESIAN_POINT('Ctrl Pts',(43.136983004927,30.0827355501013,-38.893477927521));
#270134=CARTESIAN_POINT('Ctrl Pts',(43.0423554365792,30.1779102993728,-38.893593096851));
#270135=CARTESIAN_POINT('Ctrl Pts',(42.9978715396443,30.2274270793998,-38.8946524983587));
#270136=CARTESIAN_POINT('Ctrl Pts',(42.9143010667291,30.3302227545307,-38.8986981279734));
#270137=CARTESIAN_POINT('Ctrl Pts',(42.8752237175721,30.3834938975299,-38.9016846639526));
#270138=CARTESIAN_POINT('Ctrl Pts',(42.8024397261494,30.4937517735858,-38.9095657636758));
#270139=CARTESIAN_POINT('Ctrl Pts',(42.7687347167421,30.5507433047372,-38.9144616840886));
#270140=CARTESIAN_POINT('Ctrl Pts',(42.7300278300793,30.6243427738123,-38.9217927993296));
#270141=CARTESIAN_POINT('Ctrl Pts',(42.7224591498617,30.6391844010125,-38.9233206679252));
#270142=CARTESIAN_POINT('Ctrl Pts',(42.7076683020993,30.6691039109109,-38.9264983150556));
#270143=CARTESIAN_POINT('Ctrl Pts',(42.7004432835422,30.6841920440013,-38.9281496447495));
#270144=CARTESIAN_POINT('Ctrl Pts',(42.6794143353072,30.7295580738094,-38.9332597737812));
#270145=CARTESIAN_POINT('Ctrl Pts',(42.6662166357692,30.7600070397506,-38.9368809290395));
#270146=CARTESIAN_POINT('Ctrl Pts',(42.6414216277427,30.8213220567451,-38.9445436541549));
#270147=CARTESIAN_POINT('Ctrl Pts',(42.6298250815994,30.8521852903658,-38.9485847931962));
#270148=CARTESIAN_POINT('Ctrl Pts',(42.6082082262651,30.9143167270108,-38.9570788827674));
#270149=CARTESIAN_POINT('Ctrl Pts',(42.5981879579414,30.9455849404748,-38.9615318444951));
#270150=CARTESIAN_POINT('Ctrl Pts',(42.5797100543851,31.0085229640247,-38.9708449417209));
#270151=CARTESIAN_POINT('Ctrl Pts',(42.5712524352517,31.0401927781745,-38.9757050820557));
#270152=CARTESIAN_POINT('Ctrl Pts',(42.5558976643663,31.1039335760284,-38.9858308250948));
#270153=CARTESIAN_POINT('Ctrl Pts',(42.5490005053429,31.1360045577763,-38.9910964266694));
#270154=CARTESIAN_POINT('Ctrl Pts',(42.5367758515694,31.2005501914637,-39.0020342749577));
#270155=CARTESIAN_POINT('Ctrl Pts',(42.5314471712796,31.2330404201865,-39.007709523219));
#270156=CARTESIAN_POINT('Ctrl Pts',(42.5223849923266,31.2983677257365,-39.0194587805602));
#270157=CARTESIAN_POINT('Ctrl Pts',(42.5186403552644,31.3313583601098,-39.0255624829972));
#270158=CARTESIAN_POINT('Ctrl Pts',(42.5128293460636,31.3970657507066,-39.038055061464));
#270159=CARTESIAN_POINT('Ctrl Pts',(42.5107468075751,31.4298508641049,-39.0444548642532));
#270160=CARTESIAN_POINT('Ctrl Pts',(42.5081970620853,31.4952703256329,-39.0575511235813));
#270161=CARTESIAN_POINT('Ctrl Pts',(42.5077288537135,31.5279075248247,-39.0642479703919));
#270162=CARTESIAN_POINT('Ctrl Pts',(42.5087067479981,31.6256052084393,-39.0847758818791));
#270163=CARTESIAN_POINT('Ctrl Pts',(42.5125304809965,31.6904522179578,-39.0990434188884));
#270164=CARTESIAN_POINT('Ctrl Pts',(42.5229811189973,31.7873005996235,-39.1213030342398));
#270165=CARTESIAN_POINT('Ctrl Pts',(42.5272518260001,31.8195129184735,-39.1288662059234));
#270166=CARTESIAN_POINT('Ctrl Pts',(42.5373776944208,31.883795893367,-39.1442798245848));
#270167=CARTESIAN_POINT('Ctrl Pts',(42.5432345666966,31.9158715468512,-39.1521316546249));
#270168=CARTESIAN_POINT('Ctrl Pts',(42.5565470612704,31.979859498611,-39.168119763369));
#270169=CARTESIAN_POINT('Ctrl Pts',(42.5640260671368,32.0118444622012,-39.1762758410947));
#270170=CARTESIAN_POINT('Ctrl Pts',(42.5804532704541,32.0750557648418,-39.1927214573391));
#270171=CARTESIAN_POINT('Ctrl Pts',(42.5894227227712,32.106396161248,-39.2010390020672));
#270172=CARTESIAN_POINT('Ctrl Pts',(42.6088418543565,32.1684870422805,-39.2178439045483));
#270173=CARTESIAN_POINT('Ctrl Pts',(42.6192936389916,32.1992486628788,-39.226334003443));
#270174=CARTESIAN_POINT('Ctrl Pts',(42.6416735245966,32.2602075594843,-39.2434876394842));
#270175=CARTESIAN_POINT('Ctrl Pts',(42.6536016315145,32.290404833084,-39.2521511779583));
#270176=CARTESIAN_POINT('Ctrl Pts',(42.6789366404289,32.3502342598595,-39.2696511714811));
#270177=CARTESIAN_POINT('Ctrl Pts',(42.6923367443656,32.3798518740678,-39.2784832479687));
#270178=CARTESIAN_POINT('Ctrl Pts',(42.7206559859697,32.4385753054162,-39.2963386321761));
#270179=CARTESIAN_POINT('Ctrl Pts',(42.7355220126264,32.4675648427258,-39.3053271639861));
#270180=CARTESIAN_POINT('Ctrl Pts',(42.7819686876355,32.5529513552204,-39.3323236941673));
#270181=CARTESIAN_POINT('Ctrl Pts',(42.8154843714806,32.6080042266715,-39.350429376845));
#270182=CARTESIAN_POINT('Ctrl Pts',(42.8874714697309,32.7144015518502,-39.3868314468607));
#270183=CARTESIAN_POINT('Ctrl Pts',(42.9259451142984,32.7657569305986,-39.405130570804));
#270184=CARTESIAN_POINT('Ctrl Pts',(42.9873802660617,32.8400220747848,-39.4327251562925));
#270185=CARTESIAN_POINT('Ctrl Pts',(43.0084803849644,32.8643150897193,-39.4419477180718));
#270186=CARTESIAN_POINT('Ctrl Pts',(43.0519381822279,32.911966602613,-39.460442053495));
#270187=CARTESIAN_POINT('Ctrl Pts',(43.0742932293765,32.9353217065842,-39.4697125999696));
#270188=CARTESIAN_POINT('Ctrl Pts',(43.1202941152109,32.9810940910691,-39.4883087327733));
#270189=CARTESIAN_POINT('Ctrl Pts',(43.1439529159728,33.0035126604972,-39.4976371211004));
#270190=CARTESIAN_POINT('Ctrl Pts',(43.1920211429799,33.0468913167546,-39.5161342576841));
#270191=CARTESIAN_POINT('Ctrl Pts',(43.2165352643027,33.0679574354316,-39.5253457202097));
#270192=CARTESIAN_POINT('Ctrl Pts',(43.2913474244647,33.1291646243131,-39.5528104082097));
#270193=CARTESIAN_POINT('Ctrl Pts',(43.3430301425081,33.1674361598715,-39.5709418650873));
#270194=CARTESIAN_POINT('Ctrl Pts',(43.4231858671606,33.2210184664833,-39.5978530872083));
#270195=CARTESIAN_POINT('Ctrl Pts',(43.4503469560668,33.2382438729789,-39.6067770568578));
#270196=CARTESIAN_POINT('Ctrl Pts',(43.5055597590889,33.2714157254684,-39.6245320627911));
#270197=CARTESIAN_POINT('Ctrl Pts',(43.5336114345675,33.2873622273092,-39.6333631021097));
#270198=CARTESIAN_POINT('Ctrl Pts',(43.5906171763999,33.3179591419151,-39.6509316376977));
#270199=CARTESIAN_POINT('Ctrl Pts',(43.6195686807026,33.3326076488467,-39.6596682334695));
#270200=CARTESIAN_POINT('Ctrl Pts',(43.6784027873839,33.3605894168931,-39.6770502813188));
#270201=CARTESIAN_POINT('Ctrl Pts',(43.7083065099628,33.3739233472053,-39.6857000236169));
#270202=CARTESIAN_POINT('Ctrl Pts',(43.7683635828038,33.3989600904335,-39.7027096012684));
#270203=CARTESIAN_POINT('Ctrl Pts',(43.7986441240576,33.410725045928,-39.7111073577373));
#270204=CARTESIAN_POINT('Ctrl Pts',(43.8596239235883,33.4327283064733,-39.7276688298622));
#270205=CARTESIAN_POINT('Ctrl Pts',(43.8903364640963,33.4429729918037,-39.7358364820756));
#270206=CARTESIAN_POINT('Ctrl Pts',(43.9831381693492,33.4714483547834,-39.760003404431));
#270207=CARTESIAN_POINT('Ctrl Pts',(44.0458899425586,33.4874253805623,-39.7756673535664));
#270208=CARTESIAN_POINT('Ctrl Pts',(44.1413568263141,33.5068320087337,-39.7984910804967));
#270209=CARTESIAN_POINT('Ctrl Pts',(44.1734026620325,33.512539916883,-39.8059867898386));
#270210=CARTESIAN_POINT('Ctrl Pts',(44.2379485985024,33.5224086377434,-39.8207511924796));
#270211=CARTESIAN_POINT('Ctrl Pts',(44.2704344157376,33.5265678396433,-39.8280167344336));
#270212=CARTESIAN_POINT('Ctrl Pts',(44.31955450659,33.5316239864186,-39.8387510991363));
#270213=CARTESIAN_POINT('Ctrl Pts',(44.3359803233845,33.5331096864767,-39.8422988490203));
#270214=CARTESIAN_POINT('Ctrl Pts',(44.3687702925121,33.5356678958833,-39.8492980293521));
#270215=CARTESIAN_POINT('Ctrl Pts',(44.3851668896783,33.5367439047296,-39.8527565827752));
#270216=CARTESIAN_POINT('Ctrl Pts',(44.4343055941691,33.5393615686568,-39.8629980872985));
#270217=CARTESIAN_POINT('Ctrl Pts',(44.467043811667,33.5402980820414,-39.8696572702326));
#270218=CARTESIAN_POINT('Ctrl Pts',(44.5651280609268,33.5407002285591,-39.8891214986439));
#270219=CARTESIAN_POINT('Ctrl Pts',(44.6303961191261,33.5377689750917,-39.9014257084291));
#270220=CARTESIAN_POINT('Ctrl Pts',(44.7606551553719,33.5254981705544,-39.9246908296974));
#270221=CARTESIAN_POINT('Ctrl Pts',(44.8256640685817,33.5161533726516,-39.9356542165744));
#270222=CARTESIAN_POINT('Ctrl Pts',(44.906721867411,33.5003619888654,-39.9484974119658));
#270223=CARTESIAN_POINT('Ctrl Pts',(44.9229346750623,33.4969927872433,-39.9510241738426));
#270224=CARTESIAN_POINT('Ctrl Pts',(44.9553219764425,33.4898425172325,-39.9559880147365));
#270225=CARTESIAN_POINT('Ctrl Pts',(44.9715284344022,33.4860526078472,-39.958429637772));
#270226=CARTESIAN_POINT('Ctrl Pts',(45.0199627900161,33.4740854281601,-39.9655990795304));
#270227=CARTESIAN_POINT('Ctrl Pts',(45.0519106460378,33.4653389646544,-39.9701583622527));
#270228=CARTESIAN_POINT('Ctrl Pts',(45.1152342592699,33.4463085275747,-39.9788590382424));
#270229=CARTESIAN_POINT('Ctrl Pts',(45.1465931161906,33.4360289026411,-39.9829979637287));
#270230=CARTESIAN_POINT('Ctrl Pts',(45.2087103117349,33.4139546170134,-39.9908577188348));
#270231=CARTESIAN_POINT('Ctrl Pts',(45.2394686437959,33.4021599396053,-39.9945785431013));
#270232=CARTESIAN_POINT('Ctrl Pts',(45.3003857153532,33.3770580671335,-40.0016036322017));
#270233=CARTESIAN_POINT('Ctrl Pts',(45.3305444573974,33.3637508783763,-40.0049078982014));
#270234=CARTESIAN_POINT('Ctrl Pts',(45.390258886243,33.3356154142248,-40.011098275424));
#270235=CARTESIAN_POINT('Ctrl Pts',(45.4198145849242,33.3207871687102,-40.0139843944556));
#270236=CARTESIAN_POINT('Ctrl Pts',(45.4783149483493,33.2895896149825,-40.01933367126));
#270237=CARTESIAN_POINT('Ctrl Pts',(45.507262517348,33.2732175573309,-40.0217968588865));
#270238=CARTESIAN_POINT('Ctrl Pts',(45.5645222978915,33.2389114608181,-40.0262919941319));
#270239=CARTESIAN_POINT('Ctrl Pts',(45.5928960780074,33.2209281679648,-40.0283263501325));
#270240=CARTESIAN_POINT('Ctrl Pts',(45.6483112696052,33.1838254126132,-40.0319112250503));
#270241=CARTESIAN_POINT('Ctrl Pts',(45.6754897776133,33.1646269393907,-40.033473120182));
#270242=CARTESIAN_POINT('Ctrl Pts',(45.7287236826122,33.1250040552468,-40.0361368706617));
#270243=CARTESIAN_POINT('Ctrl Pts',(45.7547928320097,33.1045715914186,-40.0372398412512));
#270244=CARTESIAN_POINT('Ctrl Pts',(45.8313713764485,33.0414275867026,-40.0398685197573));
#270245=CARTESIAN_POINT('Ctrl Pts',(45.8802555440049,32.9968736013142,-40.0407155796136));
#270246=CARTESIAN_POINT('Ctrl Pts',(45.9503135478119,32.9263375747907,-40.0406220600909));
#270247=CARTESIAN_POINT('Ctrl Pts',(45.9731206268418,32.9022070589556,-40.0403631547939));
#270248=CARTESIAN_POINT('Ctrl Pts',(46.0176283770391,32.8526917463635,-40.0393834530318));
#270249=CARTESIAN_POINT('Ctrl Pts',(46.0393233161468,32.8273141108128,-40.0386629364799));
#270250=CARTESIAN_POINT('Ctrl Pts',(46.0816063372946,32.7752494087917,-40.0367489513753));
#270251=CARTESIAN_POINT('Ctrl Pts',(46.1020200031328,32.7487743967956,-40.0355628438162));
#270252=CARTESIAN_POINT('Ctrl Pts',(46.1413455248285,32.6950606561891,-40.0327468789706));
#270253=CARTESIAN_POINT('Ctrl Pts',(46.1602720912561,32.6678035871797,-40.0311163104268));
#270254=CARTESIAN_POINT('Ctrl Pts',(46.2148746530555,32.5848590029048,-40.0255677342833));
#270255=CARTESIAN_POINT('Ctrl Pts',(46.2483818229377,32.5279958230559,-40.0209940857161));
#270256=CARTESIAN_POINT('Ctrl Pts',(46.3096688668557,32.4111729744312,-40.0101125434596));
#270257=CARTESIAN_POINT('Ctrl Pts',(46.3374502738645,32.3511989868894,-40.0038021480578));
#270258=CARTESIAN_POINT('Ctrl Pts',(46.368527809654,32.2742945109209,-39.99481246295));
#270259=CARTESIAN_POINT('Ctrl Pts',(46.3745625031242,32.2588039482195,-39.9929572402591));
#270260=CARTESIAN_POINT('Ctrl Pts',(46.3862570590194,32.2276457996089,-39.9891378326849));
#270261=CARTESIAN_POINT('Ctrl Pts',(46.3919277006514,32.2119441234091,-39.9871690698157));
#270262=CARTESIAN_POINT('Ctrl Pts',(46.4083204627969,32.1647096562841,-39.9811146940715));
#270263=CARTESIAN_POINT('Ctrl Pts',(46.4183992792463,32.1331328020619,-39.9768930221268));
#270264=CARTESIAN_POINT('Ctrl Pts',(46.4369323752314,32.0697100737179,-39.9680740796957));
#270265=CARTESIAN_POINT('Ctrl Pts',(46.4453810238695,32.0378809710586,-39.9634789966875));
#270266=CARTESIAN_POINT('Ctrl Pts',(46.4606707140735,31.9739914674526,-39.9539230277982));
#270267=CARTESIAN_POINT('Ctrl Pts',(46.4675116609156,31.9419310527617,-39.9489621213728));
#270268=CARTESIAN_POINT('Ctrl Pts',(46.4856471656838,31.8454065140233,-39.9335346428238));
#270269=CARTESIAN_POINT('Ctrl Pts',(46.4945595050313,31.7805939086316,-39.9225233405268));
#270270=CARTESIAN_POINT('Ctrl Pts',(46.5031525845005,31.682706857495,-39.9049137240114));
#270271=CARTESIAN_POINT('Ctrl Pts',(46.5052196048422,31.6499521123145,-39.8988586119036));
#270272=CARTESIAN_POINT('Ctrl Pts',(46.5071100859963,31.6006666000752,-39.8895013323517));
#270273=CARTESIAN_POINT('Ctrl Pts',(46.5075383370072,31.5841997621947,-39.8863338999606));
#270274=CARTESIAN_POINT('Ctrl Pts',(46.5079880490572,31.5512292566173,-39.8799094799294));
#270275=CARTESIAN_POINT('Ctrl Pts',(46.5080089473365,31.5346906881349,-39.8766454813005));
#270276=CARTESIAN_POINT('Ctrl Pts',(46.5074573980809,31.4851841124548,-39.8667505882022));
#270277=CARTESIAN_POINT('Ctrl Pts',(46.5062766666147,31.4523784018193,-39.8600285058855));
#270278=CARTESIAN_POINT('Ctrl Pts',(46.5023268283512,31.3870651032717,-39.8463202210145));
#270279=CARTESIAN_POINT('Ctrl Pts',(46.4995580430915,31.3545727204625,-39.8393370895085));
#270280=CARTESIAN_POINT('Ctrl Pts',(46.4889122836107,31.2575799370501,-39.8180059067137));
#270281=CARTESIAN_POINT('Ctrl Pts',(46.4787005768383,31.1935629350167,-39.8032768261342));
#270282=CARTESIAN_POINT('Ctrl Pts',(46.4587745183326,31.098492744583,-39.7804246588118));
#270283=CARTESIAN_POINT('Ctrl Pts',(46.4513631036993,31.0669621704925,-39.7726806371984));
#270284=CARTESIAN_POINT('Ctrl Pts',(46.4349953704741,31.0042214510855,-39.7569372896318));
#270285=CARTESIAN_POINT('Ctrl Pts',(46.426038976159,30.973010935597,-39.7489378760851));
#270286=CARTESIAN_POINT('Ctrl Pts',(46.4065648883721,30.9109154529952,-39.7326803432244));
#270287=CARTESIAN_POINT('Ctrl Pts',(46.3960429010861,30.8800187258512,-39.7244190196926));
#270288=CARTESIAN_POINT('Ctrl Pts',(46.3734248182074,30.8185999023854,-39.7076436938793));
#270289=CARTESIAN_POINT('Ctrl Pts',(46.3614222035831,30.7883284740624,-39.6991983942538));
#270290=CARTESIAN_POINT('Ctrl Pts',(46.3487330454107,30.7584586806226,-39.6906893116447));
#270291=CARTESIAN_POINT('Ctrl Pts',(44.6028102757013,33.538203052834,-39.8960581756957));
#270292=CARTESIAN_POINT('Ctrl Pts',(44.5684884519592,33.5398325791396,-39.8896053029486));
#270293=CARTESIAN_POINT('Ctrl Pts',(44.5341306228379,33.5405765787541,-39.8829664139251));
#270294=CARTESIAN_POINT('Ctrl Pts',(44.4997391850464,33.5404355737569,-39.8761416497953));
#270295=CARTESIAN_POINT('Ctrl Pts',(44.4670443896497,33.5403015249987,-39.8696535736582));
#270296=CARTESIAN_POINT('Ctrl Pts',(44.4343061264537,33.5393650105759,-39.8629943907241));
#270297=CARTESIAN_POINT('Ctrl Pts',(44.4015469444054,33.5376198991251,-39.8561667210419));
#270298=CARTESIAN_POINT('Ctrl Pts',(44.3851673533813,33.5367473433996,-39.8527528862008));
#270299=CARTESIAN_POINT('Ctrl Pts',(44.3687707333322,33.5356713331865,-39.8492943327777));
#270300=CARTESIAN_POINT('Ctrl Pts',(44.3523757258895,33.5343922268333,-39.8457947426118));
#270301=CARTESIAN_POINT('Ctrl Pts',(44.3359807184467,33.53311312048,-39.8422951524459));
#270302=CARTESIAN_POINT('Ctrl Pts',(44.3195548787318,33.5316274184839,-39.8387474025619));
#270303=CARTESIAN_POINT('Ctrl Pts',(44.3031814922686,33.5299420340084,-39.8351692809943));
#270304=CARTESIAN_POINT('Ctrl Pts',(44.2704347193421,33.5265712650576,-39.8280130378592));
#270305=CARTESIAN_POINT('Ctrl Pts',(44.2379488567859,33.5224120576217,-39.8207474959053));
#270306=CARTESIAN_POINT('Ctrl Pts',(44.2056758435329,33.5174776905724,-39.8133652945847));
#270307=CARTESIAN_POINT('Ctrl Pts',(44.1734028307723,33.5125433235984,-39.8059830933769));
#270308=CARTESIAN_POINT('Ctrl Pts',(44.1413569694056,33.506835411636,-39.7984873881882));
#270309=CARTESIAN_POINT('Ctrl Pts',(44.1095346139294,33.5003666523966,-39.7908793336944));
#270310=CARTESIAN_POINT('Ctrl Pts',(44.0458899015202,33.4874291336216,-39.7756632243584));
#270311=CARTESIAN_POINT('Ctrl Pts',(43.9831381149063,33.471452179088,-39.759999220822));
#270312=CARTESIAN_POINT('Ctrl Pts',(43.9212701806475,33.4524682573117,-39.7438882601));
#270313=CARTESIAN_POINT('Ctrl Pts',(43.8903362137541,33.4429762964961,-39.7358327798005));
#270314=CARTESIAN_POINT('Ctrl Pts',(43.8596236543864,33.432731604347,-39.7276651332879));
#270315=CARTESIAN_POINT('Ctrl Pts',(43.8291337121394,33.421729958977,-39.7193843972254));
#270316=CARTESIAN_POINT('Ctrl Pts',(43.7986437698924,33.4107283136069,-39.7111036611629));
#270317=CARTESIAN_POINT('Ctrl Pts',(43.7683631864552,33.3989633419485,-39.7027059046941));
#270318=CARTESIAN_POINT('Ctrl Pts',(43.7383346082092,33.3864449531174,-39.6942011158683));
#270319=CARTESIAN_POINT('Ctrl Pts',(43.7083060299631,33.3739265642863,-39.6856963270425));
#270320=CARTESIAN_POINT('Ctrl Pts',(43.6784022657394,33.3605926156183,-39.6770465847445));
#270321=CARTESIAN_POINT('Ctrl Pts',(43.6489851714386,33.3466017123189,-39.6683555608198));
#270322=CARTESIAN_POINT('Ctrl Pts',(43.6195680771379,33.3326108090195,-39.6596645368951));
#270323=CARTESIAN_POINT('Ctrl Pts',(43.5906156336918,33.3179617994446,-39.6509276635309));
#270324=CARTESIAN_POINT('Ctrl Pts',(43.5621135894733,33.3026639516225,-39.6421434977462));
#270325=CARTESIAN_POINT('Ctrl Pts',(43.5336113200827,33.2873659829441,-39.6333592625648));
#270326=CARTESIAN_POINT('Ctrl Pts',(43.5055593687618,33.2714193184022,-39.6245281992176));
#270327=CARTESIAN_POINT('Ctrl Pts',(43.4779525093745,33.2548330333127,-39.6156506437734));
#270328=CARTESIAN_POINT('Ctrl Pts',(43.4503460861836,33.2382470102913,-39.6067732285971));
#270329=CARTESIAN_POINT('Ctrl Pts',(43.4231847792171,33.2210213314943,-39.5978493197658));
#270330=CARTESIAN_POINT('Ctrl Pts',(43.3964663782543,33.2031606790307,-39.5888789832603));
#270331=CARTESIAN_POINT('Ctrl Pts',(43.3430291541635,33.1674390918953,-39.5709381685129));
#270332=CARTESIAN_POINT('Ctrl Pts',(43.2913463642683,33.129167503371,-39.5528067116353));
#270333=CARTESIAN_POINT('Ctrl Pts',(43.2414715215205,33.088362654268,-39.5344969196353));
#270334=CARTESIAN_POINT('Ctrl Pts',(43.2165341001466,33.0679602297166,-39.5253420236353));
#270335=CARTESIAN_POINT('Ctrl Pts',(43.1920199447671,33.0468940818524,-39.5161305611097));
#270336=CARTESIAN_POINT('Ctrl Pts',(43.1679857978823,33.0252047236631,-39.5068819928179));
#270337=CARTESIAN_POINT('Ctrl Pts',(43.1439516509975,33.0035153654738,-39.497633424526));
#270338=CARTESIAN_POINT('Ctrl Pts',(43.1202928173846,32.9810967649645,-39.4883050361989));
#270339=CARTESIAN_POINT('Ctrl Pts',(43.0972923425396,32.9582105409828,-39.4790069697971));
#270340=CARTESIAN_POINT('Ctrl Pts',(43.0742918676945,32.9353243170012,-39.4697089033952));
#270341=CARTESIAN_POINT('Ctrl Pts',(43.0519360617005,32.9119683859121,-39.460438038431));
#270342=CARTESIAN_POINT('Ctrl Pts',(43.0302080409885,32.8881435936574,-39.451191262225));
#270343=CARTESIAN_POINT('Ctrl Pts',(43.0084800202764,32.8643188014027,-39.4419444860189));
#270344=CARTESIAN_POINT('Ctrl Pts',(42.9873794912476,32.8400253900556,-39.4327217732547));
#270345=CARTESIAN_POINT('Ctrl Pts',(42.9669007794172,32.8152701048891,-39.4235233479461));
#270346=CARTESIAN_POINT('Ctrl Pts',(42.9259433557564,32.7657595345561,-39.4051264973289));
#270347=CARTESIAN_POINT('Ctrl Pts',(42.8874698490093,32.7144038555933,-39.3868277502863));
#270348=CARTESIAN_POINT('Ctrl Pts',(42.8514762500672,32.661205119079,-39.3686267152785));
#270349=CARTESIAN_POINT('Ctrl Pts',(42.8154826511251,32.6080063825646,-39.3504256802706));
#270350=CARTESIAN_POINT('Ctrl Pts',(42.7819669209395,32.5529534345799,-39.332319997593));
#270351=CARTESIAN_POINT('Ctrl Pts',(42.7510024281725,32.4960290137494,-39.3143223108055));
#270352=CARTESIAN_POINT('Ctrl Pts',(42.735520181789,32.4675668033342,-39.3053234674117));
#270353=CARTESIAN_POINT('Ctrl Pts',(42.7206541346169,32.4385772256996,-39.2963349356017));
#270354=CARTESIAN_POINT('Ctrl Pts',(42.7064944942894,32.4092154691749,-39.287407243498));
#270355=CARTESIAN_POINT('Ctrl Pts',(42.6923348539619,32.3798537126501,-39.2784795513943));
#270356=CARTESIAN_POINT('Ctrl Pts',(42.678934731563,32.3502360572277,-39.2696474749068));
#270357=CARTESIAN_POINT('Ctrl Pts',(42.6662672096693,32.3203213022045,-39.2608974781453));
#270358=CARTESIAN_POINT('Ctrl Pts',(46.6981266849492,30.7091523375488,-39.2904704603133));
#270359=CARTESIAN_POINT('Ctrl Pts',(46.6689684123063,30.6404043382273,-39.273452295095));
#270360=CARTESIAN_POINT('Ctrl Pts',(46.6043681216411,30.5066861069553,-39.238925705885));
#270361=CARTESIAN_POINT('Ctrl Pts',(46.5083209189471,30.3487389562033,-39.1945593129175));
#270362=CARTESIAN_POINT('Ctrl Pts',(46.4437937583117,30.2581216171786,-39.1673894861782));
#270363=CARTESIAN_POINT('Ctrl Pts',(46.3992224148768,30.1986447451181,-39.1491520227249));
#270364=CARTESIAN_POINT('Ctrl Pts',(46.3761748773305,30.1693908446446,-39.1399767764946));
#270365=CARTESIAN_POINT('Ctrl Pts',(46.3284414024809,30.1117648114071,-39.1214771434543));
#270366=CARTESIAN_POINT('Ctrl Pts',(46.3038983378397,30.083571828401,-39.112209259666));
#270367=CARTESIAN_POINT('Ctrl Pts',(46.253707387608,30.0286632749651,-39.0937226519629));
#270368=CARTESIAN_POINT('Ctrl Pts',(46.2280147026909,30.001893564456,-39.0844865568113));
#270369=CARTESIAN_POINT('Ctrl Pts',(46.1492148010453,29.9236586721517,-39.0568159196779));
#270370=CARTESIAN_POINT('Ctrl Pts',(46.0669347173688,29.8495134741745,-39.0292038481275));
#270371=CARTESIAN_POINT('Ctrl Pts',(45.9503410384262,29.7587889734315,-38.9925114043613));
#270372=CARTESIAN_POINT('Ctrl Pts',(45.8594191065401,29.6948377475824,-38.9650526418885));
#270373=CARTESIAN_POINT('Ctrl Pts',(45.7964751089327,29.6549785818455,-38.9467936623891));
#270374=CARTESIAN_POINT('Ctrl Pts',(45.748348603817,29.6261284949947,-38.9331097524421));
#270375=CARTESIAN_POINT('Ctrl Pts',(45.7321473284057,29.616684052073,-38.9285487676403));
#270376=CARTESIAN_POINT('Ctrl Pts',(45.6996106203311,29.5982459977232,-38.9194791520014));
#270377=CARTESIAN_POINT('Ctrl Pts',(45.683249044345,29.5892352448745,-38.9149628379356));
#270378=CARTESIAN_POINT('Ctrl Pts',(45.6010439155842,29.5452684013657,-38.8924942188443));
#270379=CARTESIAN_POINT('Ctrl Pts',(45.4667739830181,29.4816584171599,-38.8571935516581));
#270380=CARTESIAN_POINT('Ctrl Pts',(45.2922645146651,29.4187721922835,-38.8147007629208));
#270381=CARTESIAN_POINT('Ctrl Pts',(45.184512437616,29.3885937253944,-38.7899522655792));
#270382=CARTESIAN_POINT('Ctrl Pts',(45.1119891467798,29.3701842541612,-38.7736235920333));
#270383=CARTESIAN_POINT('Ctrl Pts',(45.0754052578815,29.3618381514785,-38.7655490803555));
#270384=CARTESIAN_POINT('Ctrl Pts',(45.0014447932705,29.3468760834356,-38.7495561846596));
#270385=CARTESIAN_POINT('Ctrl Pts',(44.964301863367,29.3403115562353,-38.7416890516424));
#270386=CARTESIAN_POINT('Ctrl Pts',(44.8900079594565,29.3290481892184,-38.726277749838));
#270387=CARTESIAN_POINT('Ctrl Pts',(44.8527936282157,29.324336495618,-38.7187198739728));
#270388=CARTESIAN_POINT('Ctrl Pts',(44.7410083373266,29.3129455735289,-38.6964994820139));
#270389=CARTESIAN_POINT('Ctrl Pts',(44.6662563757167,29.3089967422249,-38.6822807693139));
#270390=CARTESIAN_POINT('Ctrl Pts',(44.516312468428,29.3084067934202,-38.6550493453909));
#270391=CARTESIAN_POINT('Ctrl Pts',(44.441103189525,29.3117700143417,-38.6420342479066));
#270392=CARTESIAN_POINT('Ctrl Pts',(44.3468378615956,29.3206690055189,-38.6265520162729));
#270393=CARTESIAN_POINT('Ctrl Pts',(44.3279589148655,29.3226883315868,-38.6234933649988));
#270394=CARTESIAN_POINT('Ctrl Pts',(44.2901960653062,29.3271995080042,-38.6174591262491));
#270395=CARTESIAN_POINT('Ctrl Pts',(44.271274393292,29.329697893027,-38.614477863833));
#270396=CARTESIAN_POINT('Ctrl Pts',(44.2146592782019,29.3378915995821,-38.60568558559));
#270397=CARTESIAN_POINT('Ctrl Pts',(44.1772069502033,29.344266758826,-38.6000392683017));
#270398=CARTESIAN_POINT('Ctrl Pts',(44.0655444875092,29.3661148598052,-38.5837127379559));
#270399=CARTESIAN_POINT('Ctrl Pts',(43.9553791862171,29.3933792052515,-38.5686255047386));
#270400=CARTESIAN_POINT('Ctrl Pts',(43.8114622524781,29.4404829778103,-38.5509833019505));
#270401=CARTESIAN_POINT('Ctrl Pts',(43.705021834675,29.481230340464,-38.5390021142185));
#270402=CARTESIAN_POINT('Ctrl Pts',(43.6350719757086,29.512061063653,-38.5318621614261));
#270403=CARTESIAN_POINT('Ctrl Pts',(43.5656410085295,29.5447591316771,-38.525155654825));
#270404=CARTESIAN_POINT('Ctrl Pts',(43.5311320054746,29.5620794464364,-38.5220163122062));
#270405=CARTESIAN_POINT('Ctrl Pts',(43.4634866412134,29.5981758355574,-38.5162526847879));
#270406=CARTESIAN_POINT('Ctrl Pts',(43.4301834663392,29.6170276546,-38.5136117755133));
#270407=CARTESIAN_POINT('Ctrl Pts',(43.3647025891651,29.6562685687332,-38.5088155315793));
#270408=CARTESIAN_POINT('Ctrl Pts',(43.2681192378476,29.7174608121974,-38.5023448938576));
#270409=CARTESIAN_POINT('Ctrl Pts',(43.1764049274077,29.7855824582168,-38.4980286134812));
#270410=CARTESIAN_POINT('Ctrl Pts',(43.0584774180437,29.8826126224142,-38.4942050936184));
#270411=CARTESIAN_POINT('Ctrl Pts',(43.001681818637,29.9342392650769,-38.4932590761897));
#270412=CARTESIAN_POINT('Ctrl Pts',(42.8926599718677,30.0438904492243,-38.4933742455196));
#270413=CARTESIAN_POINT('Ctrl Pts',(42.8414047150844,30.1009342501745,-38.4944336470273));
#270414=CARTESIAN_POINT('Ctrl Pts',(42.7451036203247,30.2193471227021,-38.498479276642));
#270415=CARTESIAN_POINT('Ctrl Pts',(42.6550322643363,30.3420646399833,-38.5044516702661));
#270416=CARTESIAN_POINT('Ctrl Pts',(42.5773225406025,30.4733365238586,-38.5142428327574));
#270417=CARTESIAN_POINT('Ctrl Pts',(42.5326943378214,30.5580963840027,-38.5215739479982));
#270418=CARTESIAN_POINT('Ctrl Pts',(42.5239673850246,30.5751883092729,-38.5231018165939));
#270419=CARTESIAN_POINT('Ctrl Pts',(42.5069121510755,30.60964376351,-38.5262794637242));
#270420=CARTESIAN_POINT('Ctrl Pts',(42.4985805781952,30.627019094627,-38.5279307934181));
#270421=CARTESIAN_POINT('Ctrl Pts',(42.4743295471271,30.6792614198295,-38.5330409224498));
#270422=CARTESIAN_POINT('Ctrl Pts',(42.4438856226513,30.7493896366731,-38.5402834483744));
#270423=CARTESIAN_POINT('Ctrl Pts',(42.4037483179465,30.8560072598611,-38.5524071291592));
#270424=CARTESIAN_POINT('Ctrl Pts',(42.3690543371876,30.9640160484273,-38.5657659376104));
#270425=CARTESIAN_POINT('Ctrl Pts',(42.3397558527982,31.0734075527136,-38.5803463747351));
#270426=CARTESIAN_POINT('Ctrl Pts',(42.3238156343608,31.1472555030051,-38.5908775753381));
#270427=CARTESIAN_POINT('Ctrl Pts',(42.3096820427396,31.2215665449467,-38.6018154236264));
#270428=CARTESIAN_POINT('Ctrl Pts',(42.3035171869091,31.2589715314082,-38.6074906718877));
#270429=CARTESIAN_POINT('Ctrl Pts',(42.2930235524414,31.3341791410138,-38.6192399292287));
#270430=CARTESIAN_POINT('Ctrl Pts',(42.2886818075092,31.3721585359098,-38.6253436316658));
#270431=CARTESIAN_POINT('Ctrl Pts',(42.281930630611,31.4478003630713,-38.6378362101326));
#270432=CARTESIAN_POINT('Ctrl Pts',(42.277074994566,31.5232809912004,-38.6506356205751));
#270433=CARTESIAN_POINT('Ctrl Pts',(42.2747992363309,31.6735553614761,-38.6774229397946));
#270434=CARTESIAN_POINT('Ctrl Pts',(42.2834818483937,31.8228397562226,-38.7059581415094));
#270435=CARTESIAN_POINT('Ctrl Pts',(42.3030248127084,31.9711385758679,-38.7362097844166));
#270436=CARTESIAN_POINT('Ctrl Pts',(42.3164494406915,32.0449687602614,-38.7519128032936));
#270437=CARTESIAN_POINT('Ctrl Pts',(42.3317154579634,32.1186122141692,-38.7679009120377));
#270438=CARTESIAN_POINT('Ctrl Pts',(42.3402956643805,32.1554227583218,-38.7760569897633));
#270439=CARTESIAN_POINT('Ctrl Pts',(42.3591481714288,32.228169160774,-38.7925026060078));
#270440=CARTESIAN_POINT('Ctrl Pts',(42.3694448348212,32.2642362896146,-38.8008201507359));
#270441=CARTESIAN_POINT('Ctrl Pts',(42.4028917825415,32.3714169561226,-38.8260275044574));
#270442=CARTESIAN_POINT('Ctrl Pts',(42.428602574983,32.4415633880281,-38.8431823298655));
#270443=CARTESIAN_POINT('Ctrl Pts',(42.4722685042023,32.5448307979217,-38.8694323201497));
#270444=CARTESIAN_POINT('Ctrl Pts',(42.4876674804306,32.5789105800712,-38.8782643966373));
#270445=CARTESIAN_POINT('Ctrl Pts',(42.5202146590728,32.6464795812123,-38.8961197808447));
#270446=CARTESIAN_POINT('Ctrl Pts',(42.5373018269229,32.6798350022668,-38.9051083126545));
#270447=CARTESIAN_POINT('Ctrl Pts',(42.5906929412925,32.7780783962456,-38.9321048428364));
#270448=CARTESIAN_POINT('Ctrl Pts',(42.629225789877,32.8414173722334,-38.9502105255135));
#270449=CARTESIAN_POINT('Ctrl Pts',(42.7120000069194,32.9638220552461,-38.9866125955294));
#270450=CARTESIAN_POINT('Ctrl Pts',(42.7783647966162,33.0524402968179,-39.0140612314234));
#270451=CARTESIAN_POINT('Ctrl Pts',(42.8754380724448,33.1642175243331,-39.0509520337677));
#270452=CARTESIAN_POINT('Ctrl Pts',(42.9268673384212,33.2179450225078,-39.0694937486382));
#270453=CARTESIAN_POINT('Ctrl Pts',(42.9797817061918,33.2705900457306,-39.088089881442));
#270454=CARTESIAN_POINT('Ctrl Pts',(43.0069972096607,33.2963736994336,-39.097418269769));
#270455=CARTESIAN_POINT('Ctrl Pts',(43.0622936398443,33.3462615369726,-39.1159154063528));
#270456=CARTESIAN_POINT('Ctrl Pts',(43.0904949946047,33.3704876748183,-39.1251268688783));
#270457=CARTESIAN_POINT('Ctrl Pts',(43.176562606447,33.4408730143712,-39.1525915568785));
#270458=CARTESIAN_POINT('Ctrl Pts',(43.2360245534179,33.4848790444095,-39.1707230137558));
#270459=CARTESIAN_POINT('Ctrl Pts',(43.358992255749,33.5670176609587,-39.2066046432507));
#270460=CARTESIAN_POINT('Ctrl Pts',(43.4542745623933,33.6242424638975,-39.233238623837));
#270461=CARTESIAN_POINT('Ctrl Pts',(43.5542222374601,33.6747516510336,-39.2594493821381));
#270462=CARTESIAN_POINT('Ctrl Pts',(43.6219256430316,33.7069073870393,-39.2768314299875));
#270463=CARTESIAN_POINT('Ctrl Pts',(43.6563381479934,33.7222286468184,-39.2854811722856));
#270464=CARTESIAN_POINT('Ctrl Pts',(43.7254519170511,33.7509934760635,-39.3024907499371));
#270465=CARTESIAN_POINT('Ctrl Pts',(43.7602995448845,33.7645084608315,-39.3108885064059));
#270466=CARTESIAN_POINT('Ctrl Pts',(43.8304781084082,33.789780836939,-39.3274499785309));
#270467=CARTESIAN_POINT('Ctrl Pts',(43.9365171946568,33.8250735562425,-39.3519527568515));
#270468=CARTESIAN_POINT('Ctrl Pts',(44.0809642638621,33.8617420360433,-39.3832806139221));
#270469=CARTESIAN_POINT('Ctrl Pts',(44.1916183723467,33.8813683146414,-39.4057679385072));
#270470=CARTESIAN_POINT('Ctrl Pts',(44.2659122959159,33.8926702964892,-39.4205323411483));
#270471=CARTESIAN_POINT('Ctrl Pts',(44.3033049221432,33.8974288658374,-39.4277978831022));
#270472=CARTESIAN_POINT('Ctrl Pts',(44.3598453576919,33.9032050944765,-39.4385322478049));
#270473=CARTESIAN_POINT('Ctrl Pts',(44.3787527158677,33.9049006163346,-39.4420799976889));
#270474=CARTESIAN_POINT('Ctrl Pts',(44.4164967874688,33.9078161173588,-39.4490791780208));
#270475=CARTESIAN_POINT('Ctrl Pts',(44.4353708468856,33.9090400957878,-39.4525377314439));
#270476=CARTESIAN_POINT('Ctrl Pts',(44.4919347179527,33.9120095261765,-39.462779235967));
#270477=CARTESIAN_POINT('Ctrl Pts',(44.52962054914,33.9130584408517,-39.4694384189012));
#270478=CARTESIAN_POINT('Ctrl Pts',(44.6425299001817,33.9134342925821,-39.4889026473125));
#270479=CARTESIAN_POINT('Ctrl Pts',(44.7176656228988,33.9100023852834,-39.5012068570978));
#270480=CARTESIAN_POINT('Ctrl Pts',(44.867623327666,33.8957625538083,-39.524471978366));
#270481=CARTESIAN_POINT('Ctrl Pts',(44.9424659600731,33.8849485744664,-39.5354353652432));
#270482=CARTESIAN_POINT('Ctrl Pts',(45.0357885152669,33.8666999843662,-39.5482785606344));
#270483=CARTESIAN_POINT('Ctrl Pts',(45.0544546343785,33.8628074782943,-39.5508053225112));
#270484=CARTESIAN_POINT('Ctrl Pts',(45.091743102575,33.8545484160302,-39.5557691634051));
#270485=CARTESIAN_POINT('Ctrl Pts',(45.1104022544846,33.850171655015,-39.5582107864407));
#270486=CARTESIAN_POINT('Ctrl Pts',(45.1661672125598,33.8363538303533,-39.5653802281989));
#270487=CARTESIAN_POINT('Ctrl Pts',(45.2029511118778,33.8262578362557,-39.5699395109212));
#270488=CARTESIAN_POINT('Ctrl Pts',(45.312316831343,33.7933159380614,-39.582990524906));
#270489=CARTESIAN_POINT('Ctrl Pts',(45.4195983160475,33.7551076509549,-39.5947758536238));
#270490=CARTESIAN_POINT('Ctrl Pts',(45.5585113890164,33.6937328563153,-39.6079933748399));
#270491=CARTESIAN_POINT('Ctrl Pts',(45.6606150024606,33.6424505696195,-39.6166516297843));
#270492=CARTESIAN_POINT('Ctrl Pts',(45.7272860947277,33.6047101271221,-39.6215780075552));
#270493=CARTESIAN_POINT('Ctrl Pts',(45.7932287365117,33.5651705839516,-39.6260731428005));
#270494=CARTESIAN_POINT('Ctrl Pts',(45.8259059249178,33.5444453395394,-39.6281074988013));
#270495=CARTESIAN_POINT('Ctrl Pts',(45.8897275017006,33.5016881508368,-39.6316923737189));
#270496=CARTESIAN_POINT('Ctrl Pts',(45.9210297733036,33.4795651380848,-39.6332542688506));
#270497=CARTESIAN_POINT('Ctrl Pts',(45.9823424846244,33.4339088874735,-39.6359180193303));
#270498=CARTESIAN_POINT('Ctrl Pts',(46.0724202597563,33.3632801300718,-39.6392265347984));
#270499=CARTESIAN_POINT('Ctrl Pts',(46.1850394564173,33.2606222983665,-39.6409205727319));
#270500=CARTESIAN_POINT('Ctrl Pts',(46.2638636333332,33.1772336958075,-39.6401443034625));
#270501=CARTESIAN_POINT('Ctrl Pts',(46.3151397511292,33.1201974856456,-39.6391646017005));
#270502=CARTESIAN_POINT('Ctrl Pts',(46.3401349353408,33.0909661742941,-39.6384440851485));
#270503=CARTESIAN_POINT('Ctrl Pts',(46.3888523044997,33.0309971480077,-39.6365301000439));
#270504=CARTESIAN_POINT('Ctrl Pts',(46.4123735341802,33.0005036828642,-39.6353439924849));
#270505=CARTESIAN_POINT('Ctrl Pts',(46.4576879006691,32.9386388625828,-39.6325280276393));
#270506=CARTESIAN_POINT('Ctrl Pts',(46.52311576659,32.8444620833496,-39.6276360146217));
#270507=CARTESIAN_POINT('Ctrl Pts',(46.5810426872604,32.7462345994881,-39.6207752343847));
#270508=CARTESIAN_POINT('Ctrl Pts',(46.6516918187307,32.6117039458857,-39.6098936921283));
#270509=CARTESIAN_POINT('Ctrl Pts',(46.683723185051,32.5426422373878,-39.6035832967262));
#270510=CARTESIAN_POINT('Ctrl Pts',(46.7195635412788,32.4540883209461,-39.5945936116187));
#270511=CARTESIAN_POINT('Ctrl Pts',(46.7265235775841,32.4362514419463,-39.5927383889278));
#270512=CARTESIAN_POINT('Ctrl Pts',(46.7400123459627,32.4003742100513,-39.5889189813535));
#270513=CARTESIAN_POINT('Ctrl Pts',(46.7465535157541,32.3822946053341,-39.5869502184844));
#270514=CARTESIAN_POINT('Ctrl Pts',(46.7654644360989,32.3279072933142,-39.5808958427402));
#270515=CARTESIAN_POINT('Ctrl Pts',(46.7770937339888,32.2915493874551,-39.5766741707955));
#270516=CARTESIAN_POINT('Ctrl Pts',(46.8091770518909,32.182013131159,-39.5634457571489));
#270517=CARTESIAN_POINT('Ctrl Pts',(46.8444383818759,32.034891308334,-39.5443264312115));
#270518=CARTESIAN_POINT('Ctrl Pts',(46.8650708643864,31.8856621776612,-39.5223044891954));
#270519=CARTESIAN_POINT('Ctrl Pts',(46.8750487417844,31.7729724844591,-39.50469487268));
#270520=CARTESIAN_POINT('Ctrl Pts',(46.8774570362353,31.7352651712118,-39.4986397605723));
#270521=CARTESIAN_POINT('Ctrl Pts',(46.8796767940079,31.6785286095959,-39.4892824810203));
#270522=CARTESIAN_POINT('Ctrl Pts',(46.8801843407089,31.6595724593507,-39.4861150486293));
#270523=CARTESIAN_POINT('Ctrl Pts',(46.8807312344332,31.6216180949417,-39.479690628598));
#270524=CARTESIAN_POINT('Ctrl Pts',(46.8807699646674,31.6025797052015,-39.4764266299692));
#270525=CARTESIAN_POINT('Ctrl Pts',(46.8801790388754,31.5455906639181,-39.4665317368708));
#270526=CARTESIAN_POINT('Ctrl Pts',(46.8788490796135,31.5078273383739,-39.4598096545541));
#270527=CARTESIAN_POINT('Ctrl Pts',(46.874360617844,31.4326451774338,-39.4461013696832));
#270528=CARTESIAN_POINT('Ctrl Pts',(46.864884835636,31.320441459725,-39.4251517854185));
#270529=CARTESIAN_POINT('Ctrl Pts',(46.8414902947658,31.1730719473388,-39.3956936109857));
#270530=CARTESIAN_POINT('Ctrl Pts',(46.8074810934279,31.0279105813681,-39.364717848004));
#270531=CARTESIAN_POINT('Ctrl Pts',(46.7869180083019,30.9560697433081,-39.3487190247537));
#270532=CARTESIAN_POINT('Ctrl Pts',(46.7645577771926,30.884604709384,-39.332461491893));
#270533=CARTESIAN_POINT('Ctrl Pts',(46.7524740339114,30.8490466969583,-39.3242001683612));
#270534=CARTESIAN_POINT('Ctrl Pts',(46.7264943673172,30.7783632715819,-39.3074248425479));
#270535=CARTESIAN_POINT('Ctrl Pts',(46.7127058212706,30.7435263372096,-39.2989795429224));
#270536=CARTESIAN_POINT('Ctrl Pts',(46.6981266849492,30.7091523375488,-39.2904704603133));
#270537=CARTESIAN_POINT('Ctrl Pts',(44.7926621173534,30.9780510210195,-41.4731170634489));
#270538=CARTESIAN_POINT('Ctrl Pts',(44.7841183378731,30.958431594105,-41.4560988982307));
#270539=CARTESIAN_POINT('Ctrl Pts',(44.7652574387158,30.9202429989855,-41.4215723090211));
#270540=CARTESIAN_POINT('Ctrl Pts',(44.7373647422364,30.8750641226134,-41.3772059160528));
#270541=CARTESIAN_POINT('Ctrl Pts',(44.7186826069414,30.8491098680677,-41.3500360893141));
#270542=CARTESIAN_POINT('Ctrl Pts',(44.7057896374646,30.8320666178198,-41.3317986258606));
#270543=CARTESIAN_POINT('Ctrl Pts',(44.6991283043737,30.8236797190306,-41.3226233796301));
#270544=CARTESIAN_POINT('Ctrl Pts',(44.6853430526266,30.8071501195218,-41.3041237465898));
#270545=CARTESIAN_POINT('Ctrl Pts',(44.6782604199269,30.7990587859436,-41.2948558628018));
#270546=CARTESIAN_POINT('Ctrl Pts',(44.6637865272211,30.7832912649286,-41.2763692550984));
#270547=CARTESIAN_POINT('Ctrl Pts',(44.65638232911,30.7755995480316,-41.2671331599469));
#270548=CARTESIAN_POINT('Ctrl Pts',(44.6336879630273,30.7531065345255,-41.2394625228135));
#270549=CARTESIAN_POINT('Ctrl Pts',(44.6100194582072,30.7317609779911,-41.211850451263));
#270550=CARTESIAN_POINT('Ctrl Pts',(44.5765344835469,30.7055824366946,-41.1751580074971));
#270551=CARTESIAN_POINT('Ctrl Pts',(44.5504480754,30.6870962504203,-41.147699245024));
#270552=CARTESIAN_POINT('Ctrl Pts',(44.5324056777293,30.6755504391987,-41.1294402655247));
#270553=CARTESIAN_POINT('Ctrl Pts',(44.5186168522497,30.6671837862428,-41.1157563555777));
#270554=CARTESIAN_POINT('Ctrl Pts',(44.5139760207251,30.6644431539959,-41.1111953707762));
#270555=CARTESIAN_POINT('Ctrl Pts',(44.5046579712977,30.6590892493455,-41.102125755137));
#270556=CARTESIAN_POINT('Ctrl Pts',(44.4999732573772,30.6564710151932,-41.0976094410703));
#270557=CARTESIAN_POINT('Ctrl Pts',(44.4764410055871,30.6436866063214,-41.0751408219827));
#270558=CARTESIAN_POINT('Ctrl Pts',(44.4380363426647,30.6251318507397,-41.0398401547925));
#270559=CARTESIAN_POINT('Ctrl Pts',(44.3881999640401,30.6066279457426,-40.9973473660572));
#270560=CARTESIAN_POINT('Ctrl Pts',(44.3574626802754,30.5976558165788,-40.9725988687145));
#270561=CARTESIAN_POINT('Ctrl Pts',(44.3367823836873,30.5921565153947,-40.9562701951691));
#270562=CARTESIAN_POINT('Ctrl Pts',(44.3263541271388,30.5896491085923,-40.9481956834911));
#270563=CARTESIAN_POINT('Ctrl Pts',(44.3052793937559,30.5851218575581,-40.9322027877955));
#270564=CARTESIAN_POINT('Ctrl Pts',(44.2946995104909,30.5831174982377,-40.924335654778));
#270565=CARTESIAN_POINT('Ctrl Pts',(44.2735450602529,30.5796377993431,-40.9089243529734));
#270566=CARTESIAN_POINT('Ctrl Pts',(44.2629524396991,30.5781585711684,-40.9013664771085));
#270567=CARTESIAN_POINT('Ctrl Pts',(44.2311453972639,30.5744985086998,-40.8791460851492));
#270568=CARTESIAN_POINT('Ctrl Pts',(44.2098907431643,30.5730912421562,-40.8649273724495));
#270569=CARTESIAN_POINT('Ctrl Pts',(44.1672866942957,30.5723474200962,-40.8376959485268));
#270570=CARTESIAN_POINT('Ctrl Pts',(44.1459323927671,30.5730120277702,-40.8246808510428));
#270571=CARTESIAN_POINT('Ctrl Pts',(44.1191870166623,30.5751734135742,-40.8091986194082));
#270572=CARTESIAN_POINT('Ctrl Pts',(44.1138315874482,30.5756735271978,-40.806139968135));
#270573=CARTESIAN_POINT('Ctrl Pts',(44.1031212948485,30.5768077596639,-40.8001057293845));
#270574=CARTESIAN_POINT('Ctrl Pts',(44.0977557278508,30.5774435866632,-40.7971244669688));
#270575=CARTESIAN_POINT('Ctrl Pts',(44.0817045383335,30.5795497856634,-40.7883321887253));
#270576=CARTESIAN_POINT('Ctrl Pts',(44.0710902649836,30.5812139186595,-40.7826858714375));
#270577=CARTESIAN_POINT('Ctrl Pts',(44.0394561806682,30.5869813183234,-40.7663593410916));
#270578=CARTESIAN_POINT('Ctrl Pts',(44.0082701709188,30.5942909050994,-40.7512721078743));
#270579=CARTESIAN_POINT('Ctrl Pts',(43.9675777996734,30.6070988998346,-40.7336299050859));
#270580=CARTESIAN_POINT('Ctrl Pts',(43.9375066395073,30.6182485087226,-40.721648717354));
#270581=CARTESIAN_POINT('Ctrl Pts',(43.917761614853,30.626725808719,-40.7145087645619));
#270582=CARTESIAN_POINT('Ctrl Pts',(43.8981718083816,30.6357351147044,-40.7078022579606));
#270583=CARTESIAN_POINT('Ctrl Pts',(43.8884396229394,30.6405162381665,-40.7046629153417));
#270584=CARTESIAN_POINT('Ctrl Pts',(43.8693712864522,30.6504970769624,-40.6988992879235));
#270585=CARTESIAN_POINT('Ctrl Pts',(43.8599880575193,30.6557176389023,-40.6962583786489));
#270586=CARTESIAN_POINT('Ctrl Pts',(43.8415477166501,30.6665995934339,-40.6914621347147));
#270587=CARTESIAN_POINT('Ctrl Pts',(43.8143622090585,30.6835906587784,-40.6849914969931));
#270588=CARTESIAN_POINT('Ctrl Pts',(43.7885885365895,30.7025683103525,-40.6806752166169));
#270589=CARTESIAN_POINT('Ctrl Pts',(43.7554869731093,30.7296502406846,-40.676851696754));
#270590=CARTESIAN_POINT('Ctrl Pts',(43.7395647886014,30.744083456595,-40.6759056793254));
#270591=CARTESIAN_POINT('Ctrl Pts',(43.7090440489059,30.7747854825451,-40.6760208486551));
#270592=CARTESIAN_POINT('Ctrl Pts',(43.6947173014185,30.7907796762741,-40.6770802501629));
#270593=CARTESIAN_POINT('Ctrl Pts',(43.6678443418708,30.8240220908504,-40.6811258797777));
#270594=CARTESIAN_POINT('Ctrl Pts',(43.6427576069985,30.8585127548254,-40.687098273402));
#270595=CARTESIAN_POINT('Ctrl Pts',(43.6212142380078,30.8954846730083,-40.6968894358922));
#270596=CARTESIAN_POINT('Ctrl Pts',(43.6088787182641,30.9193798597989,-40.7042205511341));
#270597=CARTESIAN_POINT('Ctrl Pts',(43.6064685586478,30.9241994859948,-40.7057484197296));
#270598=CARTESIAN_POINT('Ctrl Pts',(43.6017624551859,30.9339175659931,-40.70892606686));
#270599=CARTESIAN_POINT('Ctrl Pts',(43.5994656231147,30.9388193592268,-40.7105773965538));
#270600=CARTESIAN_POINT('Ctrl Pts',(43.5927866482525,30.953560895212,-40.7156875255853));
#270601=CARTESIAN_POINT('Ctrl Pts',(43.5844198153918,30.9733582110501,-40.72293005151));
#270602=CARTESIAN_POINT('Ctrl Pts',(43.5734440082896,31.0034822735469,-40.7350537322951));
#270603=CARTESIAN_POINT('Ctrl Pts',(43.5640181327981,31.0340244080827,-40.7484125407461));
#270604=CARTESIAN_POINT('Ctrl Pts',(43.5561284133843,31.0649820306433,-40.7629929778707));
#270605=CARTESIAN_POINT('Ctrl Pts',(43.5518912037438,31.0858969805267,-40.7735241784737));
#270606=CARTESIAN_POINT('Ctrl Pts',(43.5481682579358,31.1069510729684,-40.7844620267622));
#270607=CARTESIAN_POINT('Ctrl Pts',(43.5465635963524,31.1175527760565,-40.7901372750232));
#270608=CARTESIAN_POINT('Ctrl Pts',(43.5438765944467,31.1388768366658,-40.8018865323646));
#270609=CARTESIAN_POINT('Ctrl Pts',(43.5427912565025,31.1496493641875,-40.8079902348016));
#270610=CARTESIAN_POINT('Ctrl Pts',(43.5411674088753,31.1711124235333,-40.8204828132684));
#270611=CARTESIAN_POINT('Ctrl Pts',(43.5400805588778,31.19253758885,-40.8332822237109));
#270612=CARTESIAN_POINT('Ctrl Pts',(43.5400129658238,31.2352236668913,-40.8600695429299));
#270613=CARTESIAN_POINT('Ctrl Pts',(43.5430492497798,31.2776738375434,-40.8886047446452));
#270614=CARTESIAN_POINT('Ctrl Pts',(43.5491614319672,31.3198884817001,-40.918856387552));
#270615=CARTESIAN_POINT('Ctrl Pts',(43.5532522131496,31.3409199794841,-40.9345594064291));
#270616=CARTESIAN_POINT('Ctrl Pts',(43.5578644352119,31.361905871423,-40.9505475151733));
#270617=CARTESIAN_POINT('Ctrl Pts',(43.560439098329,31.3723994717644,-40.9587035928991));
#270618=CARTESIAN_POINT('Ctrl Pts',(43.5660648897127,31.3931449423641,-40.9751492091434));
#270619=CARTESIAN_POINT('Ctrl Pts',(43.5691234314236,31.4034342087731,-40.9834667538713));
#270620=CARTESIAN_POINT('Ctrl Pts',(43.5790202279964,31.4340221767704,-41.0086741075936));
#270621=CARTESIAN_POINT('Ctrl Pts',(43.5865808644402,31.4540562960243,-41.0258289330007));
#270622=CARTESIAN_POINT('Ctrl Pts',(43.5993606039644,31.4835727602996,-41.0520789232858));
#270623=CARTESIAN_POINT('Ctrl Pts',(43.6038584649574,31.4933175175814,-41.0609109997729));
#270624=CARTESIAN_POINT('Ctrl Pts',(43.6133480280387,31.5126460303085,-41.0787663839806));
#270625=CARTESIAN_POINT('Ctrl Pts',(43.6183219077102,31.5221915251339,-41.0877549157913));
#270626=CARTESIAN_POINT('Ctrl Pts',(43.6338406007018,31.5503182102049,-41.1147514459697));
#270627=CARTESIAN_POINT('Ctrl Pts',(43.6450116757484,31.5684678157769,-41.13285712865));
#270628=CARTESIAN_POINT('Ctrl Pts',(43.6689569093208,31.6035742491305,-41.1692591986645));
#270629=CARTESIAN_POINT('Ctrl Pts',(43.6881189975485,31.6290150958394,-41.1967078345595));
#270630=CARTESIAN_POINT('Ctrl Pts',(43.7160805799803,31.6611548911343,-41.2335986369031));
#270631=CARTESIAN_POINT('Ctrl Pts',(43.7308739938731,31.6766212732249,-41.2521403517739));
#270632=CARTESIAN_POINT('Ctrl Pts',(43.7460847706871,31.6917854492915,-41.2707364845776));
#270633=CARTESIAN_POINT('Ctrl Pts',(43.7539033240721,31.6992171694526,-41.2800648729051));
#270634=CARTESIAN_POINT('Ctrl Pts',(43.7697797892606,31.7136063232936,-41.298562009488));
#270635=CARTESIAN_POINT('Ctrl Pts',(43.7778723272806,31.7205988773597,-41.3077734720143));
#270636=CARTESIAN_POINT('Ctrl Pts',(43.8025568401133,31.7409299545529,-41.3352381600133));
#270637=CARTESIAN_POINT('Ctrl Pts',(43.8195937300504,31.7536621581445,-41.353369616892));
#270638=CARTESIAN_POINT('Ctrl Pts',(43.8547939251157,31.7774712224987,-41.3892512463859));
#270639=CARTESIAN_POINT('Ctrl Pts',(43.8820456950658,31.7940939723408,-41.4158852269725));
#270640=CARTESIAN_POINT('Ctrl Pts',(43.9105977352555,31.8088239425505,-41.4420959852738));
#270641=CARTESIAN_POINT('Ctrl Pts',(43.9299312426308,31.8182163905263,-41.4594780331231));
#270642=CARTESIAN_POINT('Ctrl Pts',(43.9397545046832,31.8226994853967,-41.4681277754213));
#270643=CARTESIAN_POINT('Ctrl Pts',(43.959476379363,31.8311327029401,-41.4851373530728));
#270644=CARTESIAN_POINT('Ctrl Pts',(43.969416794615,31.835103670887,-41.4935351095415));
#270645=CARTESIAN_POINT('Ctrl Pts',(43.9894286782948,31.8425474915593,-41.5100965816665));
#270646=CARTESIAN_POINT('Ctrl Pts',(44.0196562937352,31.8529720625538,-41.5345993599874));
#270647=CARTESIAN_POINT('Ctrl Pts',(44.0607928561344,31.8639280327151,-41.5659272170578));
#270648=CARTESIAN_POINT('Ctrl Pts',(44.0922765794535,31.8699137146658,-41.5884145416429));
#270649=CARTESIAN_POINT('Ctrl Pts',(44.1134085621028,31.8733992175668,-41.6031789442838));
#270650=CARTESIAN_POINT('Ctrl Pts',(44.1240412545,31.8748890570172,-41.6104444862381));
#270651=CARTESIAN_POINT('Ctrl Pts',(44.1401138557838,31.8767382236783,-41.6211788509405));
#270652=CARTESIAN_POINT('Ctrl Pts',(44.1454877988083,31.8772894545129,-41.6247266008247));
#270653=CARTESIAN_POINT('Ctrl Pts',(44.1562140153048,31.878256418298,-41.6317257811562));
#270654=CARTESIAN_POINT('Ctrl Pts',(44.161576905651,31.8786734249769,-41.6351843345794));
#270655=CARTESIAN_POINT('Ctrl Pts',(44.1776466456902,31.8797244502982,-41.6454258391029));
#270656=CARTESIAN_POINT('Ctrl Pts',(44.1883500092183,31.8801603696231,-41.6520850220369));
#270657=CARTESIAN_POINT('Ctrl Pts',(44.2204087008324,31.8806796234647,-41.671549250448));
#270658=CARTESIAN_POINT('Ctrl Pts',(44.2417298059497,31.8799780982567,-41.6838534602333));
#270659=CARTESIAN_POINT('Ctrl Pts',(44.2842582084951,31.8764766164199,-41.7071185815018));
#270660=CARTESIAN_POINT('Ctrl Pts',(44.3054713486111,31.8736750129732,-41.7180819683776));
#270661=CARTESIAN_POINT('Ctrl Pts',(44.3319064277948,31.8688271235064,-41.7309251637703));
#270662=CARTESIAN_POINT('Ctrl Pts',(44.3371930873745,31.8677885276791,-41.7334519256467));
#270663=CARTESIAN_POINT('Ctrl Pts',(44.3477523920959,31.8655764110726,-41.7384157665409));
#270664=CARTESIAN_POINT('Ctrl Pts',(44.353035452149,31.8644001232798,-41.7408573895762));
#270665=CARTESIAN_POINT('Ctrl Pts',(44.368821997144,31.8606750365135,-41.7480268313348));
#270666=CARTESIAN_POINT('Ctrl Pts',(44.3792318927429,31.8579388865424,-41.752586114057));
#270667=CARTESIAN_POINT('Ctrl Pts',(44.4101727404,31.8489724804825,-41.7656371280416));
#270668=CARTESIAN_POINT('Ctrl Pts',(44.4405041748167,31.8385015328462,-41.7774224567595));
#270669=CARTESIAN_POINT('Ctrl Pts',(44.4797386522914,31.8215610256552,-41.7906399779756));
#270670=CARTESIAN_POINT('Ctrl Pts',(44.5085558494592,31.8073558935676,-41.7992982329201));
#270671=CARTESIAN_POINT('Ctrl Pts',(44.5273583247585,31.7968714183439,-41.8042246106906));
#270672=CARTESIAN_POINT('Ctrl Pts',(44.5459478308046,31.7858731708475,-41.8087197459362));
#270673=CARTESIAN_POINT('Ctrl Pts',(44.5551558111633,31.7801015230391,-41.8107541019367));
#270674=CARTESIAN_POINT('Ctrl Pts',(44.5731320510561,31.7681815367951,-41.814338976855));
#270675=CARTESIAN_POINT('Ctrl Pts',(44.5819448307914,31.7620078883687,-41.8159008719862));
#270676=CARTESIAN_POINT('Ctrl Pts',(44.5991987000126,31.7492554022398,-41.8185646224661));
#270677=CARTESIAN_POINT('Ctrl Pts',(44.6245350600795,31.7295108031857,-41.8218731379338));
#270678=CARTESIAN_POINT('Ctrl Pts',(44.6561620699444,31.7007477525095,-41.8235671758672));
#270679=CARTESIAN_POINT('Ctrl Pts',(44.6782580742923,31.6773394437008,-41.8227909065983));
#270680=CARTESIAN_POINT('Ctrl Pts',(44.6926220014235,31.6613194462407,-41.8218112048364));
#270681=CARTESIAN_POINT('Ctrl Pts',(44.6996188611148,31.6531046671394,-41.8210906882841));
#270682=CARTESIAN_POINT('Ctrl Pts',(44.7132456597446,31.6362429219073,-41.8191767031797));
#270683=CARTESIAN_POINT('Ctrl Pts',(44.7198193777268,31.627664624135,-41.8179905956202));
#270684=CARTESIAN_POINT('Ctrl Pts',(44.7324727845908,31.610252798272,-41.8151746307749));
#270685=CARTESIAN_POINT('Ctrl Pts',(44.7507253937504,31.5837345714901,-41.8102826177571));
#270686=CARTESIAN_POINT('Ctrl Pts',(44.7668325292565,31.5560404782777,-41.8034218375205));
#270687=CARTESIAN_POINT('Ctrl Pts',(44.7864242741839,31.5180816884312,-41.7925402952635));
#270688=CARTESIAN_POINT('Ctrl Pts',(44.7952779235527,31.4985810718442,-41.7862298998632));
#270689=CARTESIAN_POINT('Ctrl Pts',(44.8051436066325,31.4735589245645,-41.777240214754));
#270690=CARTESIAN_POINT('Ctrl Pts',(44.8070571630202,31.4685179927861,-41.7753849920635));
#270691=CARTESIAN_POINT('Ctrl Pts',(44.8107609555809,31.4583769076679,-41.7715655844892));
#270692=CARTESIAN_POINT('Ctrl Pts',(44.8125545845603,31.4532656516023,-41.76959682162));
#270693=CARTESIAN_POINT('Ctrl Pts',(44.8177323950795,31.4378873281915,-41.7635424458753));
#270694=CARTESIAN_POINT('Ctrl Pts',(44.8209059367305,31.4276035217402,-41.7593207739311));
#270695=CARTESIAN_POINT('Ctrl Pts',(44.8296276705658,31.3966113763671,-41.7460923602843));
#270696=CARTESIAN_POINT('Ctrl Pts',(44.8391161742293,31.3549585404116,-41.7269730343471));
#270697=CARTESIAN_POINT('Ctrl Pts',(44.8444380100638,31.312658433005,-41.7049510923314));
#270698=CARTESIAN_POINT('Ctrl Pts',(44.8468637082338,31.2806969121874,-41.6873414758157));
#270699=CARTESIAN_POINT('Ctrl Pts',(44.8474108190536,31.2699990859542,-41.6812863637077));
#270700=CARTESIAN_POINT('Ctrl Pts',(44.8478348231013,31.2538978106508,-41.671929084156));
#270701=CARTESIAN_POINT('Ctrl Pts',(44.8479099202363,31.2485174556463,-41.6687616517648));
#270702=CARTESIAN_POINT('Ctrl Pts',(44.8479268208064,31.2377432265879,-41.6623372317338));
#270703=CARTESIAN_POINT('Ctrl Pts',(44.8478683021095,31.2323379437313,-41.6590732331048));
#270704=CARTESIAN_POINT('Ctrl Pts',(44.8474921214824,31.2161555213209,-41.6491783400064));
#270705=CARTESIAN_POINT('Ctrl Pts',(44.8469759958029,31.2054292064128,-41.6424562576898));
#270706=CARTESIAN_POINT('Ctrl Pts',(44.8454249887827,31.1840681958411,-41.6287479728186));
#270707=CARTESIAN_POINT('Ctrl Pts',(44.8423204600693,31.1521790951542,-41.6077983885548));
#270708=CARTESIAN_POINT('Ctrl Pts',(44.8351290816859,31.1102584040656,-41.5783402141209));
#270709=CARTESIAN_POINT('Ctrl Pts',(44.8249268329474,31.0689281614894,-41.54736445114));
#270710=CARTESIAN_POINT('Ctrl Pts',(44.8188163283608,31.0484607830594,-41.5313656278891));
#270711=CARTESIAN_POINT('Ctrl Pts',(44.8121960627665,31.028093840338,-41.5151080950287));
#270712=CARTESIAN_POINT('Ctrl Pts',(44.808629563005,31.0179567656131,-41.5068467714969));
#270713=CARTESIAN_POINT('Ctrl Pts',(44.8009827391877,30.9977990758989,-41.4900714456835));
#270714=CARTESIAN_POINT('Ctrl Pts',(44.7969340070935,30.9878607344767,-41.4816261460579));
#270715=CARTESIAN_POINT('Ctrl Pts',(44.7926621173534,30.9780510210195,-41.4731170634489));
#270716=CARTESIAN_POINT('Ctrl Pts',(46.6981266849492,30.7091523375488,-39.2904704603133));
#270717=CARTESIAN_POINT('Ctrl Pts',(46.6689684123063,30.6404043382273,-39.273452295095));
#270718=CARTESIAN_POINT('Ctrl Pts',(46.6043681216411,30.5066861069553,-39.238925705885));
#270719=CARTESIAN_POINT('Ctrl Pts',(46.5083209189471,30.3487389562033,-39.1945593129175));
#270720=CARTESIAN_POINT('Ctrl Pts',(46.4437937583117,30.2581216171786,-39.1673894861782));
#270721=CARTESIAN_POINT('Ctrl Pts',(46.3992224148768,30.1986447451181,-39.1491520227249));
#270722=CARTESIAN_POINT('Ctrl Pts',(46.3761748773305,30.1693908446446,-39.1399767764946));
#270723=CARTESIAN_POINT('Ctrl Pts',(46.3284414024809,30.1117648114071,-39.1214771434543));
#270724=CARTESIAN_POINT('Ctrl Pts',(46.3038983378397,30.083571828401,-39.112209259666));
#270725=CARTESIAN_POINT('Ctrl Pts',(46.253707387608,30.0286632749651,-39.0937226519629));
#270726=CARTESIAN_POINT('Ctrl Pts',(46.2280147026909,30.001893564456,-39.0844865568113));
#270727=CARTESIAN_POINT('Ctrl Pts',(46.1492148010453,29.9236586721517,-39.0568159196779));
#270728=CARTESIAN_POINT('Ctrl Pts',(46.0669347173688,29.8495134741745,-39.0292038481275));
#270729=CARTESIAN_POINT('Ctrl Pts',(45.9503410384262,29.7587889734315,-38.9925114043613));
#270730=CARTESIAN_POINT('Ctrl Pts',(45.8594191065401,29.6948377475824,-38.9650526418885));
#270731=CARTESIAN_POINT('Ctrl Pts',(45.7964751089327,29.6549785818455,-38.9467936623891));
#270732=CARTESIAN_POINT('Ctrl Pts',(45.748348603817,29.6261284949947,-38.9331097524421));
#270733=CARTESIAN_POINT('Ctrl Pts',(45.7321473284057,29.616684052073,-38.9285487676403));
#270734=CARTESIAN_POINT('Ctrl Pts',(45.6996106203311,29.5982459977232,-38.9194791520014));
#270735=CARTESIAN_POINT('Ctrl Pts',(45.683249044345,29.5892352448745,-38.9149628379356));
#270736=CARTESIAN_POINT('Ctrl Pts',(45.6010439155842,29.5452684013657,-38.8924942188443));
#270737=CARTESIAN_POINT('Ctrl Pts',(45.4667739830181,29.4816584171599,-38.8571935516581));
#270738=CARTESIAN_POINT('Ctrl Pts',(45.2922645146651,29.4187721922835,-38.8147007629208));
#270739=CARTESIAN_POINT('Ctrl Pts',(45.184512437616,29.3885937253944,-38.7899522655792));
#270740=CARTESIAN_POINT('Ctrl Pts',(45.1119891467798,29.3701842541612,-38.7736235920333));
#270741=CARTESIAN_POINT('Ctrl Pts',(45.0754052578815,29.3618381514785,-38.7655490803555));
#270742=CARTESIAN_POINT('Ctrl Pts',(45.0014447932705,29.3468760834356,-38.7495561846596));
#270743=CARTESIAN_POINT('Ctrl Pts',(44.964301863367,29.3403115562353,-38.7416890516424));
#270744=CARTESIAN_POINT('Ctrl Pts',(44.8900079594565,29.3290481892184,-38.726277749838));
#270745=CARTESIAN_POINT('Ctrl Pts',(44.8527936282157,29.324336495618,-38.7187198739728));
#270746=CARTESIAN_POINT('Ctrl Pts',(44.7410083373266,29.3129455735289,-38.6964994820139));
#270747=CARTESIAN_POINT('Ctrl Pts',(44.6662563757167,29.3089967422249,-38.6822807693139));
#270748=CARTESIAN_POINT('Ctrl Pts',(44.516312468428,29.3084067934202,-38.6550493453909));
#270749=CARTESIAN_POINT('Ctrl Pts',(44.441103189525,29.3117700143417,-38.6420342479066));
#270750=CARTESIAN_POINT('Ctrl Pts',(44.3468378615956,29.3206690055189,-38.6265520162729));
#270751=CARTESIAN_POINT('Ctrl Pts',(44.3279589148655,29.3226883315868,-38.6234933649988));
#270752=CARTESIAN_POINT('Ctrl Pts',(44.2901960653062,29.3271995080042,-38.6174591262491));
#270753=CARTESIAN_POINT('Ctrl Pts',(44.271274393292,29.329697893027,-38.614477863833));
#270754=CARTESIAN_POINT('Ctrl Pts',(44.2146592782019,29.3378915995821,-38.60568558559));
#270755=CARTESIAN_POINT('Ctrl Pts',(44.1772069502033,29.344266758826,-38.6000392683017));
#270756=CARTESIAN_POINT('Ctrl Pts',(44.0655444875092,29.3661148598052,-38.5837127379559));
#270757=CARTESIAN_POINT('Ctrl Pts',(43.9553791862171,29.3933792052515,-38.5686255047386));
#270758=CARTESIAN_POINT('Ctrl Pts',(43.8114622524781,29.4404829778103,-38.5509833019505));
#270759=CARTESIAN_POINT('Ctrl Pts',(43.705021834675,29.481230340464,-38.5390021142185));
#270760=CARTESIAN_POINT('Ctrl Pts',(43.6350719757086,29.512061063653,-38.5318621614261));
#270761=CARTESIAN_POINT('Ctrl Pts',(43.5656410085295,29.5447591316771,-38.525155654825));
#270762=CARTESIAN_POINT('Ctrl Pts',(43.5311320054746,29.5620794464364,-38.5220163122062));
#270763=CARTESIAN_POINT('Ctrl Pts',(43.4634866412134,29.5981758355574,-38.5162526847879));
#270764=CARTESIAN_POINT('Ctrl Pts',(43.4301834663392,29.6170276546,-38.5136117755133));
#270765=CARTESIAN_POINT('Ctrl Pts',(43.3647025891651,29.6562685687332,-38.5088155315793));
#270766=CARTESIAN_POINT('Ctrl Pts',(43.2681192378476,29.7174608121974,-38.5023448938576));
#270767=CARTESIAN_POINT('Ctrl Pts',(43.1764049274077,29.7855824582168,-38.4980286134812));
#270768=CARTESIAN_POINT('Ctrl Pts',(43.0584774180437,29.8826126224142,-38.4942050936184));
#270769=CARTESIAN_POINT('Ctrl Pts',(43.001681818637,29.9342392650769,-38.4932590761897));
#270770=CARTESIAN_POINT('Ctrl Pts',(42.8926599718677,30.0438904492243,-38.4933742455196));
#270771=CARTESIAN_POINT('Ctrl Pts',(42.8414047150844,30.1009342501745,-38.4944336470273));
#270772=CARTESIAN_POINT('Ctrl Pts',(42.7451036203247,30.2193471227021,-38.498479276642));
#270773=CARTESIAN_POINT('Ctrl Pts',(42.6550322643363,30.3420646399833,-38.5044516702661));
#270774=CARTESIAN_POINT('Ctrl Pts',(42.5773225406025,30.4733365238586,-38.5142428327574));
#270775=CARTESIAN_POINT('Ctrl Pts',(42.5326943378214,30.5580963840027,-38.5215739479982));
#270776=CARTESIAN_POINT('Ctrl Pts',(42.5239673850246,30.5751883092729,-38.5231018165939));
#270777=CARTESIAN_POINT('Ctrl Pts',(42.5069121510755,30.60964376351,-38.5262794637242));
#270778=CARTESIAN_POINT('Ctrl Pts',(42.4985805781952,30.627019094627,-38.5279307934181));
#270779=CARTESIAN_POINT('Ctrl Pts',(42.4743295471271,30.6792614198295,-38.5330409224498));
#270780=CARTESIAN_POINT('Ctrl Pts',(42.4438856226513,30.7493896366731,-38.5402834483744));
#270781=CARTESIAN_POINT('Ctrl Pts',(42.4037483179465,30.8560072598611,-38.5524071291592));
#270782=CARTESIAN_POINT('Ctrl Pts',(42.3690543371876,30.9640160484273,-38.5657659376104));
#270783=CARTESIAN_POINT('Ctrl Pts',(42.3397558527982,31.0734075527136,-38.5803463747351));
#270784=CARTESIAN_POINT('Ctrl Pts',(42.3238156343608,31.1472555030051,-38.5908775753381));
#270785=CARTESIAN_POINT('Ctrl Pts',(42.3096820427396,31.2215665449467,-38.6018154236264));
#270786=CARTESIAN_POINT('Ctrl Pts',(42.3035171869091,31.2589715314082,-38.6074906718877));
#270787=CARTESIAN_POINT('Ctrl Pts',(42.2930235524414,31.3341791410138,-38.6192399292287));
#270788=CARTESIAN_POINT('Ctrl Pts',(42.2886818075092,31.3721585359098,-38.6253436316658));
#270789=CARTESIAN_POINT('Ctrl Pts',(42.281930630611,31.4478003630713,-38.6378362101326));
#270790=CARTESIAN_POINT('Ctrl Pts',(42.277074994566,31.5232809912004,-38.6506356205751));
#270791=CARTESIAN_POINT('Ctrl Pts',(42.2747992363309,31.6735553614761,-38.6774229397946));
#270792=CARTESIAN_POINT('Ctrl Pts',(42.2834818483937,31.8228397562226,-38.7059581415094));
#270793=CARTESIAN_POINT('Ctrl Pts',(42.3030248127084,31.9711385758679,-38.7362097844166));
#270794=CARTESIAN_POINT('Ctrl Pts',(42.3164494406915,32.0449687602614,-38.7519128032936));
#270795=CARTESIAN_POINT('Ctrl Pts',(42.3317154579634,32.1186122141692,-38.7679009120377));
#270796=CARTESIAN_POINT('Ctrl Pts',(42.3402956643805,32.1554227583218,-38.7760569897633));
#270797=CARTESIAN_POINT('Ctrl Pts',(42.3591481714288,32.228169160774,-38.7925026060078));
#270798=CARTESIAN_POINT('Ctrl Pts',(42.3694448348212,32.2642362896146,-38.8008201507359));
#270799=CARTESIAN_POINT('Ctrl Pts',(42.4028917825415,32.3714169561226,-38.8260275044574));
#270800=CARTESIAN_POINT('Ctrl Pts',(42.428602574983,32.4415633880281,-38.8431823298655));
#270801=CARTESIAN_POINT('Ctrl Pts',(42.4722685042023,32.5448307979217,-38.8694323201497));
#270802=CARTESIAN_POINT('Ctrl Pts',(42.4876674804306,32.5789105800712,-38.8782643966373));
#270803=CARTESIAN_POINT('Ctrl Pts',(42.5202146590728,32.6464795812123,-38.8961197808447));
#270804=CARTESIAN_POINT('Ctrl Pts',(42.5373018269229,32.6798350022668,-38.9051083126545));
#270805=CARTESIAN_POINT('Ctrl Pts',(42.5906929412925,32.7780783962456,-38.9321048428364));
#270806=CARTESIAN_POINT('Ctrl Pts',(42.629225789877,32.8414173722334,-38.9502105255135));
#270807=CARTESIAN_POINT('Ctrl Pts',(42.7120000069194,32.9638220552461,-38.9866125955294));
#270808=CARTESIAN_POINT('Ctrl Pts',(42.7783647966162,33.0524402968179,-39.0140612314234));
#270809=CARTESIAN_POINT('Ctrl Pts',(42.8754380724448,33.1642175243331,-39.0509520337677));
#270810=CARTESIAN_POINT('Ctrl Pts',(42.9268673384212,33.2179450225078,-39.0694937486382));
#270811=CARTESIAN_POINT('Ctrl Pts',(42.9797817061918,33.2705900457306,-39.088089881442));
#270812=CARTESIAN_POINT('Ctrl Pts',(43.0069972096607,33.2963736994336,-39.097418269769));
#270813=CARTESIAN_POINT('Ctrl Pts',(43.0622936398443,33.3462615369726,-39.1159154063528));
#270814=CARTESIAN_POINT('Ctrl Pts',(43.0904949946047,33.3704876748183,-39.1251268688783));
#270815=CARTESIAN_POINT('Ctrl Pts',(43.176562606447,33.4408730143712,-39.1525915568785));
#270816=CARTESIAN_POINT('Ctrl Pts',(43.2360245534179,33.4848790444095,-39.1707230137558));
#270817=CARTESIAN_POINT('Ctrl Pts',(43.358992255749,33.5670176609587,-39.2066046432507));
#270818=CARTESIAN_POINT('Ctrl Pts',(43.4542745623933,33.6242424638975,-39.233238623837));
#270819=CARTESIAN_POINT('Ctrl Pts',(43.5542222374601,33.6747516510336,-39.2594493821381));
#270820=CARTESIAN_POINT('Ctrl Pts',(43.6219256430316,33.7069073870393,-39.2768314299875));
#270821=CARTESIAN_POINT('Ctrl Pts',(43.6563381479934,33.7222286468184,-39.2854811722856));
#270822=CARTESIAN_POINT('Ctrl Pts',(43.7254519170511,33.7509934760635,-39.3024907499371));
#270823=CARTESIAN_POINT('Ctrl Pts',(43.7602995448845,33.7645084608315,-39.3108885064059));
#270824=CARTESIAN_POINT('Ctrl Pts',(43.8304781084082,33.789780836939,-39.3274499785309));
#270825=CARTESIAN_POINT('Ctrl Pts',(43.9365171946568,33.8250735562425,-39.3519527568515));
#270826=CARTESIAN_POINT('Ctrl Pts',(44.0809642638621,33.8617420360433,-39.3832806139221));
#270827=CARTESIAN_POINT('Ctrl Pts',(44.1916183723467,33.8813683146414,-39.4057679385072));
#270828=CARTESIAN_POINT('Ctrl Pts',(44.2659122959159,33.8926702964892,-39.4205323411483));
#270829=CARTESIAN_POINT('Ctrl Pts',(44.3033049221432,33.8974288658374,-39.4277978831022));
#270830=CARTESIAN_POINT('Ctrl Pts',(44.3598453576919,33.9032050944765,-39.4385322478049));
#270831=CARTESIAN_POINT('Ctrl Pts',(44.3787527158677,33.9049006163346,-39.4420799976889));
#270832=CARTESIAN_POINT('Ctrl Pts',(44.4164967874688,33.9078161173588,-39.4490791780208));
#270833=CARTESIAN_POINT('Ctrl Pts',(44.4353708468856,33.9090400957878,-39.4525377314439));
#270834=CARTESIAN_POINT('Ctrl Pts',(44.4919347179527,33.9120095261765,-39.462779235967));
#270835=CARTESIAN_POINT('Ctrl Pts',(44.52962054914,33.9130584408517,-39.4694384189012));
#270836=CARTESIAN_POINT('Ctrl Pts',(44.6425299001817,33.9134342925821,-39.4889026473125));
#270837=CARTESIAN_POINT('Ctrl Pts',(44.7176656228988,33.9100023852834,-39.5012068570978));
#270838=CARTESIAN_POINT('Ctrl Pts',(44.867623327666,33.8957625538083,-39.524471978366));
#270839=CARTESIAN_POINT('Ctrl Pts',(44.9424659600731,33.8849485744664,-39.5354353652432));
#270840=CARTESIAN_POINT('Ctrl Pts',(45.0357885152669,33.8666999843662,-39.5482785606344));
#270841=CARTESIAN_POINT('Ctrl Pts',(45.0544546343785,33.8628074782943,-39.5508053225112));
#270842=CARTESIAN_POINT('Ctrl Pts',(45.091743102575,33.8545484160302,-39.5557691634051));
#270843=CARTESIAN_POINT('Ctrl Pts',(45.1104022544846,33.850171655015,-39.5582107864407));
#270844=CARTESIAN_POINT('Ctrl Pts',(45.1661672125598,33.8363538303533,-39.5653802281989));
#270845=CARTESIAN_POINT('Ctrl Pts',(45.2029511118778,33.8262578362557,-39.5699395109212));
#270846=CARTESIAN_POINT('Ctrl Pts',(45.312316831343,33.7933159380614,-39.582990524906));
#270847=CARTESIAN_POINT('Ctrl Pts',(45.4195983160475,33.7551076509549,-39.5947758536238));
#270848=CARTESIAN_POINT('Ctrl Pts',(45.5585113890164,33.6937328563153,-39.6079933748399));
#270849=CARTESIAN_POINT('Ctrl Pts',(45.6606150024606,33.6424505696195,-39.6166516297843));
#270850=CARTESIAN_POINT('Ctrl Pts',(45.7272860947277,33.6047101271221,-39.6215780075552));
#270851=CARTESIAN_POINT('Ctrl Pts',(45.7932287365117,33.5651705839516,-39.6260731428005));
#270852=CARTESIAN_POINT('Ctrl Pts',(45.8259059249178,33.5444453395394,-39.6281074988013));
#270853=CARTESIAN_POINT('Ctrl Pts',(45.8897275017006,33.5016881508368,-39.6316923737189));
#270854=CARTESIAN_POINT('Ctrl Pts',(45.9210297733036,33.4795651380848,-39.6332542688506));
#270855=CARTESIAN_POINT('Ctrl Pts',(45.9823424846244,33.4339088874735,-39.6359180193303));
#270856=CARTESIAN_POINT('Ctrl Pts',(46.0724202597563,33.3632801300718,-39.6392265347984));
#270857=CARTESIAN_POINT('Ctrl Pts',(46.1850394564173,33.2606222983665,-39.6409205727319));
#270858=CARTESIAN_POINT('Ctrl Pts',(46.2638636333332,33.1772336958075,-39.6401443034625));
#270859=CARTESIAN_POINT('Ctrl Pts',(46.3151397511292,33.1201974856456,-39.6391646017005));
#270860=CARTESIAN_POINT('Ctrl Pts',(46.3401349353408,33.0909661742941,-39.6384440851485));
#270861=CARTESIAN_POINT('Ctrl Pts',(46.3888523044997,33.0309971480077,-39.6365301000439));
#270862=CARTESIAN_POINT('Ctrl Pts',(46.4123735341802,33.0005036828642,-39.6353439924849));
#270863=CARTESIAN_POINT('Ctrl Pts',(46.4576879006691,32.9386388625828,-39.6325280276393));
#270864=CARTESIAN_POINT('Ctrl Pts',(46.52311576659,32.8444620833496,-39.6276360146217));
#270865=CARTESIAN_POINT('Ctrl Pts',(46.5810426872604,32.7462345994881,-39.6207752343847));
#270866=CARTESIAN_POINT('Ctrl Pts',(46.6516918187307,32.6117039458857,-39.6098936921283));
#270867=CARTESIAN_POINT('Ctrl Pts',(46.683723185051,32.5426422373878,-39.6035832967262));
#270868=CARTESIAN_POINT('Ctrl Pts',(46.7195635412788,32.4540883209461,-39.5945936116187));
#270869=CARTESIAN_POINT('Ctrl Pts',(46.7265235775841,32.4362514419463,-39.5927383889278));
#270870=CARTESIAN_POINT('Ctrl Pts',(46.7400123459627,32.4003742100513,-39.5889189813535));
#270871=CARTESIAN_POINT('Ctrl Pts',(46.7465535157541,32.3822946053341,-39.5869502184844));
#270872=CARTESIAN_POINT('Ctrl Pts',(46.7654644360989,32.3279072933142,-39.5808958427402));
#270873=CARTESIAN_POINT('Ctrl Pts',(46.7770937339888,32.2915493874551,-39.5766741707955));
#270874=CARTESIAN_POINT('Ctrl Pts',(46.8091770518909,32.182013131159,-39.5634457571489));
#270875=CARTESIAN_POINT('Ctrl Pts',(46.8444383818759,32.034891308334,-39.5443264312115));
#270876=CARTESIAN_POINT('Ctrl Pts',(46.8650708643864,31.8856621776612,-39.5223044891954));
#270877=CARTESIAN_POINT('Ctrl Pts',(46.8750487417844,31.7729724844591,-39.50469487268));
#270878=CARTESIAN_POINT('Ctrl Pts',(46.8774570362353,31.7352651712118,-39.4986397605723));
#270879=CARTESIAN_POINT('Ctrl Pts',(46.8796767940079,31.6785286095959,-39.4892824810203));
#270880=CARTESIAN_POINT('Ctrl Pts',(46.8801843407089,31.6595724593507,-39.4861150486293));
#270881=CARTESIAN_POINT('Ctrl Pts',(46.8807312344332,31.6216180949417,-39.479690628598));
#270882=CARTESIAN_POINT('Ctrl Pts',(46.8807699646674,31.6025797052015,-39.4764266299692));
#270883=CARTESIAN_POINT('Ctrl Pts',(46.8801790388754,31.5455906639181,-39.4665317368708));
#270884=CARTESIAN_POINT('Ctrl Pts',(46.8788490796135,31.5078273383739,-39.4598096545541));
#270885=CARTESIAN_POINT('Ctrl Pts',(46.874360617844,31.4326451774338,-39.4461013696832));
#270886=CARTESIAN_POINT('Ctrl Pts',(46.864884835636,31.320441459725,-39.4251517854185));
#270887=CARTESIAN_POINT('Ctrl Pts',(46.8414902947658,31.1730719473388,-39.3956936109857));
#270888=CARTESIAN_POINT('Ctrl Pts',(46.8074810934279,31.0279105813681,-39.364717848004));
#270889=CARTESIAN_POINT('Ctrl Pts',(46.7869180083019,30.9560697433081,-39.3487190247537));
#270890=CARTESIAN_POINT('Ctrl Pts',(46.7645577771926,30.884604709384,-39.332461491893));
#270891=CARTESIAN_POINT('Ctrl Pts',(46.7524740339114,30.8490466969583,-39.3242001683612));
#270892=CARTESIAN_POINT('Ctrl Pts',(46.7264943673172,30.7783632715819,-39.3074248425479));
#270893=CARTESIAN_POINT('Ctrl Pts',(46.7127058212706,30.7435263372096,-39.2989795429224));
#270894=CARTESIAN_POINT('Ctrl Pts',(46.6981266849492,30.7091523375488,-39.2904704603133));
#270895=CARTESIAN_POINT('Ctrl Pts',(44.7926621173534,30.9780510210195,-41.4731170634489));
#270896=CARTESIAN_POINT('Ctrl Pts',(44.7841183378731,30.958431594105,-41.4560988982307));
#270897=CARTESIAN_POINT('Ctrl Pts',(44.7652574387158,30.9202429989855,-41.4215723090211));
#270898=CARTESIAN_POINT('Ctrl Pts',(44.7373647422364,30.8750641226134,-41.3772059160528));
#270899=CARTESIAN_POINT('Ctrl Pts',(44.7186826069414,30.8491098680677,-41.3500360893141));
#270900=CARTESIAN_POINT('Ctrl Pts',(44.7057896374646,30.8320666178198,-41.3317986258606));
#270901=CARTESIAN_POINT('Ctrl Pts',(44.6991283043737,30.8236797190306,-41.3226233796301));
#270902=CARTESIAN_POINT('Ctrl Pts',(44.6853430526266,30.8071501195218,-41.3041237465898));
#270903=CARTESIAN_POINT('Ctrl Pts',(44.6782604199269,30.7990587859436,-41.2948558628018));
#270904=CARTESIAN_POINT('Ctrl Pts',(44.6637865272211,30.7832912649286,-41.2763692550984));
#270905=CARTESIAN_POINT('Ctrl Pts',(44.65638232911,30.7755995480316,-41.2671331599469));
#270906=CARTESIAN_POINT('Ctrl Pts',(44.6336879630273,30.7531065345255,-41.2394625228135));
#270907=CARTESIAN_POINT('Ctrl Pts',(44.6100194582072,30.7317609779911,-41.211850451263));
#270908=CARTESIAN_POINT('Ctrl Pts',(44.5765344835469,30.7055824366946,-41.1751580074971));
#270909=CARTESIAN_POINT('Ctrl Pts',(44.5504480754,30.6870962504203,-41.147699245024));
#270910=CARTESIAN_POINT('Ctrl Pts',(44.5324056777293,30.6755504391987,-41.1294402655247));
#270911=CARTESIAN_POINT('Ctrl Pts',(44.5186168522497,30.6671837862428,-41.1157563555777));
#270912=CARTESIAN_POINT('Ctrl Pts',(44.5139760207251,30.6644431539959,-41.1111953707762));
#270913=CARTESIAN_POINT('Ctrl Pts',(44.5046579712977,30.6590892493455,-41.102125755137));
#270914=CARTESIAN_POINT('Ctrl Pts',(44.4999732573772,30.6564710151932,-41.0976094410703));
#270915=CARTESIAN_POINT('Ctrl Pts',(44.4764410055871,30.6436866063214,-41.0751408219827));
#270916=CARTESIAN_POINT('Ctrl Pts',(44.4380363426647,30.6251318507397,-41.0398401547925));
#270917=CARTESIAN_POINT('Ctrl Pts',(44.3881999640401,30.6066279457426,-40.9973473660572));
#270918=CARTESIAN_POINT('Ctrl Pts',(44.3574626802754,30.5976558165788,-40.9725988687145));
#270919=CARTESIAN_POINT('Ctrl Pts',(44.3367823836873,30.5921565153947,-40.9562701951691));
#270920=CARTESIAN_POINT('Ctrl Pts',(44.3263541271388,30.5896491085923,-40.9481956834911));
#270921=CARTESIAN_POINT('Ctrl Pts',(44.3052793937559,30.5851218575581,-40.9322027877955));
#270922=CARTESIAN_POINT('Ctrl Pts',(44.2946995104909,30.5831174982377,-40.924335654778));
#270923=CARTESIAN_POINT('Ctrl Pts',(44.2735450602529,30.5796377993431,-40.9089243529734));
#270924=CARTESIAN_POINT('Ctrl Pts',(44.2629524396991,30.5781585711684,-40.9013664771085));
#270925=CARTESIAN_POINT('Ctrl Pts',(44.2311453972639,30.5744985086998,-40.8791460851492));
#270926=CARTESIAN_POINT('Ctrl Pts',(44.2098907431643,30.5730912421562,-40.8649273724495));
#270927=CARTESIAN_POINT('Ctrl Pts',(44.1672866942957,30.5723474200962,-40.8376959485268));
#270928=CARTESIAN_POINT('Ctrl Pts',(44.1459323927671,30.5730120277702,-40.8246808510428));
#270929=CARTESIAN_POINT('Ctrl Pts',(44.1191870166623,30.5751734135742,-40.8091986194082));
#270930=CARTESIAN_POINT('Ctrl Pts',(44.1138315874482,30.5756735271978,-40.806139968135));
#270931=CARTESIAN_POINT('Ctrl Pts',(44.1031212948485,30.5768077596639,-40.8001057293845));
#270932=CARTESIAN_POINT('Ctrl Pts',(44.0977557278508,30.5774435866632,-40.7971244669688));
#270933=CARTESIAN_POINT('Ctrl Pts',(44.0817045383335,30.5795497856634,-40.7883321887253));
#270934=CARTESIAN_POINT('Ctrl Pts',(44.0710902649836,30.5812139186595,-40.7826858714375));
#270935=CARTESIAN_POINT('Ctrl Pts',(44.0394561806682,30.5869813183234,-40.7663593410916));
#270936=CARTESIAN_POINT('Ctrl Pts',(44.0082701709188,30.5942909050994,-40.7512721078743));
#270937=CARTESIAN_POINT('Ctrl Pts',(43.9675777996734,30.6070988998346,-40.7336299050859));
#270938=CARTESIAN_POINT('Ctrl Pts',(43.9375066395073,30.6182485087226,-40.721648717354));
#270939=CARTESIAN_POINT('Ctrl Pts',(43.917761614853,30.626725808719,-40.7145087645619));
#270940=CARTESIAN_POINT('Ctrl Pts',(43.8981718083816,30.6357351147044,-40.7078022579606));
#270941=CARTESIAN_POINT('Ctrl Pts',(43.8884396229394,30.6405162381665,-40.7046629153417));
#270942=CARTESIAN_POINT('Ctrl Pts',(43.8693712864522,30.6504970769624,-40.6988992879235));
#270943=CARTESIAN_POINT('Ctrl Pts',(43.8599880575193,30.6557176389023,-40.6962583786489));
#270944=CARTESIAN_POINT('Ctrl Pts',(43.8415477166501,30.6665995934339,-40.6914621347147));
#270945=CARTESIAN_POINT('Ctrl Pts',(43.8143622090585,30.6835906587784,-40.6849914969931));
#270946=CARTESIAN_POINT('Ctrl Pts',(43.7885885365895,30.7025683103525,-40.6806752166169));
#270947=CARTESIAN_POINT('Ctrl Pts',(43.7554869731093,30.7296502406846,-40.676851696754));
#270948=CARTESIAN_POINT('Ctrl Pts',(43.7395647886014,30.744083456595,-40.6759056793254));
#270949=CARTESIAN_POINT('Ctrl Pts',(43.7090440489059,30.7747854825451,-40.6760208486551));
#270950=CARTESIAN_POINT('Ctrl Pts',(43.6947173014185,30.7907796762741,-40.6770802501629));
#270951=CARTESIAN_POINT('Ctrl Pts',(43.6678443418708,30.8240220908504,-40.6811258797777));
#270952=CARTESIAN_POINT('Ctrl Pts',(43.6427576069985,30.8585127548254,-40.687098273402));
#270953=CARTESIAN_POINT('Ctrl Pts',(43.6212142380078,30.8954846730083,-40.6968894358922));
#270954=CARTESIAN_POINT('Ctrl Pts',(43.6088787182641,30.9193798597989,-40.7042205511341));
#270955=CARTESIAN_POINT('Ctrl Pts',(43.6064685586478,30.9241994859948,-40.7057484197296));
#270956=CARTESIAN_POINT('Ctrl Pts',(43.6017624551859,30.9339175659931,-40.70892606686));
#270957=CARTESIAN_POINT('Ctrl Pts',(43.5994656231147,30.9388193592268,-40.7105773965538));
#270958=CARTESIAN_POINT('Ctrl Pts',(43.5927866482525,30.953560895212,-40.7156875255853));
#270959=CARTESIAN_POINT('Ctrl Pts',(43.5844198153918,30.9733582110501,-40.72293005151));
#270960=CARTESIAN_POINT('Ctrl Pts',(43.5734440082896,31.0034822735469,-40.7350537322951));
#270961=CARTESIAN_POINT('Ctrl Pts',(43.5640181327981,31.0340244080827,-40.7484125407461));
#270962=CARTESIAN_POINT('Ctrl Pts',(43.5561284133843,31.0649820306433,-40.7629929778707));
#270963=CARTESIAN_POINT('Ctrl Pts',(43.5518912037438,31.0858969805267,-40.7735241784737));
#270964=CARTESIAN_POINT('Ctrl Pts',(43.5481682579358,31.1069510729684,-40.7844620267622));
#270965=CARTESIAN_POINT('Ctrl Pts',(43.5465635963524,31.1175527760565,-40.7901372750232));
#270966=CARTESIAN_POINT('Ctrl Pts',(43.5438765944467,31.1388768366658,-40.8018865323646));
#270967=CARTESIAN_POINT('Ctrl Pts',(43.5427912565025,31.1496493641875,-40.8079902348016));
#270968=CARTESIAN_POINT('Ctrl Pts',(43.5411674088753,31.1711124235333,-40.8204828132684));
#270969=CARTESIAN_POINT('Ctrl Pts',(43.5400805588778,31.19253758885,-40.8332822237109));
#270970=CARTESIAN_POINT('Ctrl Pts',(43.5400129658238,31.2352236668913,-40.8600695429299));
#270971=CARTESIAN_POINT('Ctrl Pts',(43.5430492497798,31.2776738375434,-40.8886047446452));
#270972=CARTESIAN_POINT('Ctrl Pts',(43.5491614319672,31.3198884817001,-40.918856387552));
#270973=CARTESIAN_POINT('Ctrl Pts',(43.5532522131496,31.3409199794841,-40.9345594064291));
#270974=CARTESIAN_POINT('Ctrl Pts',(43.5578644352119,31.361905871423,-40.9505475151733));
#270975=CARTESIAN_POINT('Ctrl Pts',(43.560439098329,31.3723994717644,-40.9587035928991));
#270976=CARTESIAN_POINT('Ctrl Pts',(43.5660648897127,31.3931449423641,-40.9751492091434));
#270977=CARTESIAN_POINT('Ctrl Pts',(43.5691234314236,31.4034342087731,-40.9834667538713));
#270978=CARTESIAN_POINT('Ctrl Pts',(43.5790202279964,31.4340221767704,-41.0086741075936));
#270979=CARTESIAN_POINT('Ctrl Pts',(43.5865808644402,31.4540562960243,-41.0258289330007));
#270980=CARTESIAN_POINT('Ctrl Pts',(43.5993606039644,31.4835727602996,-41.0520789232858));
#270981=CARTESIAN_POINT('Ctrl Pts',(43.6038584649574,31.4933175175814,-41.0609109997729));
#270982=CARTESIAN_POINT('Ctrl Pts',(43.6133480280387,31.5126460303085,-41.0787663839806));
#270983=CARTESIAN_POINT('Ctrl Pts',(43.6183219077102,31.5221915251339,-41.0877549157913));
#270984=CARTESIAN_POINT('Ctrl Pts',(43.6338406007018,31.5503182102049,-41.1147514459697));
#270985=CARTESIAN_POINT('Ctrl Pts',(43.6450116757484,31.5684678157769,-41.13285712865));
#270986=CARTESIAN_POINT('Ctrl Pts',(43.6689569093208,31.6035742491305,-41.1692591986645));
#270987=CARTESIAN_POINT('Ctrl Pts',(43.6881189975485,31.6290150958394,-41.1967078345595));
#270988=CARTESIAN_POINT('Ctrl Pts',(43.7160805799803,31.6611548911343,-41.2335986369031));
#270989=CARTESIAN_POINT('Ctrl Pts',(43.7308739938731,31.6766212732249,-41.2521403517739));
#270990=CARTESIAN_POINT('Ctrl Pts',(43.7460847706871,31.6917854492915,-41.2707364845776));
#270991=CARTESIAN_POINT('Ctrl Pts',(43.7539033240721,31.6992171694526,-41.2800648729051));
#270992=CARTESIAN_POINT('Ctrl Pts',(43.7697797892606,31.7136063232936,-41.298562009488));
#270993=CARTESIAN_POINT('Ctrl Pts',(43.7778723272806,31.7205988773597,-41.3077734720143));
#270994=CARTESIAN_POINT('Ctrl Pts',(43.8025568401133,31.7409299545529,-41.3352381600133));
#270995=CARTESIAN_POINT('Ctrl Pts',(43.8195937300504,31.7536621581445,-41.353369616892));
#270996=CARTESIAN_POINT('Ctrl Pts',(43.8547939251157,31.7774712224987,-41.3892512463859));
#270997=CARTESIAN_POINT('Ctrl Pts',(43.8820456950658,31.7940939723408,-41.4158852269725));
#270998=CARTESIAN_POINT('Ctrl Pts',(43.9105977352555,31.8088239425505,-41.4420959852738));
#270999=CARTESIAN_POINT('Ctrl Pts',(43.9299312426308,31.8182163905263,-41.4594780331231));
#271000=CARTESIAN_POINT('Ctrl Pts',(43.9397545046832,31.8226994853967,-41.4681277754213));
#271001=CARTESIAN_POINT('Ctrl Pts',(43.959476379363,31.8311327029401,-41.4851373530728));
#271002=CARTESIAN_POINT('Ctrl Pts',(43.969416794615,31.835103670887,-41.4935351095415));
#271003=CARTESIAN_POINT('Ctrl Pts',(43.9894286782948,31.8425474915593,-41.5100965816665));
#271004=CARTESIAN_POINT('Ctrl Pts',(44.0196562937352,31.8529720625538,-41.5345993599874));
#271005=CARTESIAN_POINT('Ctrl Pts',(44.0607928561344,31.8639280327151,-41.5659272170578));
#271006=CARTESIAN_POINT('Ctrl Pts',(44.0922765794535,31.8699137146658,-41.5884145416429));
#271007=CARTESIAN_POINT('Ctrl Pts',(44.1134085621028,31.8733992175668,-41.6031789442838));
#271008=CARTESIAN_POINT('Ctrl Pts',(44.1240412545,31.8748890570172,-41.6104444862381));
#271009=CARTESIAN_POINT('Ctrl Pts',(44.1401138557838,31.8767382236783,-41.6211788509405));
#271010=CARTESIAN_POINT('Ctrl Pts',(44.1454877988083,31.8772894545129,-41.6247266008247));
#271011=CARTESIAN_POINT('Ctrl Pts',(44.1562140153048,31.878256418298,-41.6317257811562));
#271012=CARTESIAN_POINT('Ctrl Pts',(44.161576905651,31.8786734249769,-41.6351843345794));
#271013=CARTESIAN_POINT('Ctrl Pts',(44.1776466456902,31.8797244502982,-41.6454258391029));
#271014=CARTESIAN_POINT('Ctrl Pts',(44.1883500092183,31.8801603696231,-41.6520850220369));
#271015=CARTESIAN_POINT('Ctrl Pts',(44.2204087008324,31.8806796234647,-41.671549250448));
#271016=CARTESIAN_POINT('Ctrl Pts',(44.2417298059497,31.8799780982567,-41.6838534602333));
#271017=CARTESIAN_POINT('Ctrl Pts',(44.2842582084951,31.8764766164199,-41.7071185815018));
#271018=CARTESIAN_POINT('Ctrl Pts',(44.3054713486111,31.8736750129732,-41.7180819683776));
#271019=CARTESIAN_POINT('Ctrl Pts',(44.3319064277948,31.8688271235064,-41.7309251637703));
#271020=CARTESIAN_POINT('Ctrl Pts',(44.3371930873745,31.8677885276791,-41.7334519256467));
#271021=CARTESIAN_POINT('Ctrl Pts',(44.3477523920959,31.8655764110726,-41.7384157665409));
#271022=CARTESIAN_POINT('Ctrl Pts',(44.353035452149,31.8644001232798,-41.7408573895762));
#271023=CARTESIAN_POINT('Ctrl Pts',(44.368821997144,31.8606750365135,-41.7480268313348));
#271024=CARTESIAN_POINT('Ctrl Pts',(44.3792318927429,31.8579388865424,-41.752586114057));
#271025=CARTESIAN_POINT('Ctrl Pts',(44.4101727404,31.8489724804825,-41.7656371280416));
#271026=CARTESIAN_POINT('Ctrl Pts',(44.4405041748167,31.8385015328462,-41.7774224567595));
#271027=CARTESIAN_POINT('Ctrl Pts',(44.4797386522914,31.8215610256552,-41.7906399779756));
#271028=CARTESIAN_POINT('Ctrl Pts',(44.5085558494592,31.8073558935676,-41.7992982329201));
#271029=CARTESIAN_POINT('Ctrl Pts',(44.5273583247585,31.7968714183439,-41.8042246106906));
#271030=CARTESIAN_POINT('Ctrl Pts',(44.5459478308046,31.7858731708475,-41.8087197459362));
#271031=CARTESIAN_POINT('Ctrl Pts',(44.5551558111633,31.7801015230391,-41.8107541019367));
#271032=CARTESIAN_POINT('Ctrl Pts',(44.5731320510561,31.7681815367951,-41.814338976855));
#271033=CARTESIAN_POINT('Ctrl Pts',(44.5819448307914,31.7620078883687,-41.8159008719862));
#271034=CARTESIAN_POINT('Ctrl Pts',(44.5991987000126,31.7492554022398,-41.8185646224661));
#271035=CARTESIAN_POINT('Ctrl Pts',(44.6245350600795,31.7295108031857,-41.8218731379338));
#271036=CARTESIAN_POINT('Ctrl Pts',(44.6561620699444,31.7007477525095,-41.8235671758672));
#271037=CARTESIAN_POINT('Ctrl Pts',(44.6782580742923,31.6773394437008,-41.8227909065983));
#271038=CARTESIAN_POINT('Ctrl Pts',(44.6926220014235,31.6613194462407,-41.8218112048364));
#271039=CARTESIAN_POINT('Ctrl Pts',(44.6996188611148,31.6531046671394,-41.8210906882841));
#271040=CARTESIAN_POINT('Ctrl Pts',(44.7132456597446,31.6362429219073,-41.8191767031797));
#271041=CARTESIAN_POINT('Ctrl Pts',(44.7198193777268,31.627664624135,-41.8179905956202));
#271042=CARTESIAN_POINT('Ctrl Pts',(44.7324727845908,31.610252798272,-41.8151746307749));
#271043=CARTESIAN_POINT('Ctrl Pts',(44.7507253937504,31.5837345714901,-41.8102826177571));
#271044=CARTESIAN_POINT('Ctrl Pts',(44.7668325292565,31.5560404782777,-41.8034218375205));
#271045=CARTESIAN_POINT('Ctrl Pts',(44.7864242741839,31.5180816884312,-41.7925402952635));
#271046=CARTESIAN_POINT('Ctrl Pts',(44.7952779235527,31.4985810718442,-41.7862298998632));
#271047=CARTESIAN_POINT('Ctrl Pts',(44.8051436066325,31.4735589245645,-41.777240214754));
#271048=CARTESIAN_POINT('Ctrl Pts',(44.8070571630202,31.4685179927861,-41.7753849920635));
#271049=CARTESIAN_POINT('Ctrl Pts',(44.8107609555809,31.4583769076679,-41.7715655844892));
#271050=CARTESIAN_POINT('Ctrl Pts',(44.8125545845603,31.4532656516023,-41.76959682162));
#271051=CARTESIAN_POINT('Ctrl Pts',(44.8177323950795,31.4378873281915,-41.7635424458753));
#271052=CARTESIAN_POINT('Ctrl Pts',(44.8209059367305,31.4276035217402,-41.7593207739311));
#271053=CARTESIAN_POINT('Ctrl Pts',(44.8296276705658,31.3966113763671,-41.7460923602843));
#271054=CARTESIAN_POINT('Ctrl Pts',(44.8391161742293,31.3549585404116,-41.7269730343471));
#271055=CARTESIAN_POINT('Ctrl Pts',(44.8444380100638,31.312658433005,-41.7049510923314));
#271056=CARTESIAN_POINT('Ctrl Pts',(44.8468637082338,31.2806969121874,-41.6873414758157));
#271057=CARTESIAN_POINT('Ctrl Pts',(44.8474108190536,31.2699990859542,-41.6812863637077));
#271058=CARTESIAN_POINT('Ctrl Pts',(44.8478348231013,31.2538978106508,-41.671929084156));
#271059=CARTESIAN_POINT('Ctrl Pts',(44.8479099202363,31.2485174556463,-41.6687616517648));
#271060=CARTESIAN_POINT('Ctrl Pts',(44.8479268208064,31.2377432265879,-41.6623372317338));
#271061=CARTESIAN_POINT('Ctrl Pts',(44.8478683021095,31.2323379437313,-41.6590732331048));
#271062=CARTESIAN_POINT('Ctrl Pts',(44.8474921214824,31.2161555213209,-41.6491783400064));
#271063=CARTESIAN_POINT('Ctrl Pts',(44.8469759958029,31.2054292064128,-41.6424562576898));
#271064=CARTESIAN_POINT('Ctrl Pts',(44.8454249887827,31.1840681958411,-41.6287479728186));
#271065=CARTESIAN_POINT('Ctrl Pts',(44.8423204600693,31.1521790951542,-41.6077983885548));
#271066=CARTESIAN_POINT('Ctrl Pts',(44.8351290816859,31.1102584040656,-41.5783402141209));
#271067=CARTESIAN_POINT('Ctrl Pts',(44.8249268329474,31.0689281614894,-41.54736445114));
#271068=CARTESIAN_POINT('Ctrl Pts',(44.8188163283608,31.0484607830594,-41.5313656278891));
#271069=CARTESIAN_POINT('Ctrl Pts',(44.8121960627665,31.028093840338,-41.5151080950287));
#271070=CARTESIAN_POINT('Ctrl Pts',(44.808629563005,31.0179567656131,-41.5068467714969));
#271071=CARTESIAN_POINT('Ctrl Pts',(44.8009827391877,30.9977990758989,-41.4900714456835));
#271072=CARTESIAN_POINT('Ctrl Pts',(44.7969340070935,30.9878607344767,-41.4816261460579));
#271073=CARTESIAN_POINT('Ctrl Pts',(44.7926621173534,30.9780510210195,-41.4731170634489));
#271074=CARTESIAN_POINT('Origin',(-52.7694692252869,296.281453912738,10.95005));
#271075=CARTESIAN_POINT('Origin',(0.,0.,153.53805));
#271076=CARTESIAN_POINT('',(-63.0894692252869,-82.5030998968147,153.53805));
#271077=CARTESIAN_POINT('',(-63.0894692252869,-92.5030998968147,153.53805));
#271078=CARTESIAN_POINT('',(73.0894692252869,-82.5030998968147,153.53805));
#271079=CARTESIAN_POINT('Origin',(-73.0894692252869,-82.5030998968147,-17.14995));
#271080=CARTESIAN_POINT('Origin',(5.38401031719611,-82.5030998968147,-17.14995));
#271081=CARTESIAN_POINT('Ctrl Pts',(-0.169874834567261,-85.851674811826,
-27.1502359615018));
#271082=CARTESIAN_POINT('Ctrl Pts',(-0.145946434383659,-92.5030998968192,
-24.7866082076174));
#271083=CARTESIAN_POINT('Ctrl Pts',(-0.0748618073283795,-92.5030998968147,
-17.7280551702244));
#271084=CARTESIAN_POINT('Ctrl Pts',(0.394610061152761,-85.8685073521107,
-27.1502371407667));
#271085=CARTESIAN_POINT('Ctrl Pts',(0.338716347147105,-92.5030998968009,
-24.7784666680916));
#271086=CARTESIAN_POINT('Ctrl Pts',(0.173920958628183,-92.5030998968147,
-17.7306509939903));
#271087=CARTESIAN_POINT('Ctrl Pts',(0.962014587078309,-85.8002834495678,
-27.1502324270453));
#271088=CARTESIAN_POINT('Ctrl Pts',(0.828565975978851,-92.5030998968164,
-24.8114183373701));
#271089=CARTESIAN_POINT('Ctrl Pts',(0.422955977429241,-92.5030998968147,
-17.7201896452643));
#271090=CARTESIAN_POINT('Ctrl Pts',(1.93889369920201,-85.552294476256,-27.1502147670435));
#271091=CARTESIAN_POINT('Ctrl Pts',(1.69546368882409,-92.5030998968131,
-24.9368559750962));
#271092=CARTESIAN_POINT('Ctrl Pts',(0.896430364579228,-92.5030998968147,
-17.6799095294768));
#271093=CARTESIAN_POINT('Ctrl Pts',(2.35718494292016,-85.3865396246594,
-27.1502028196572));
#271094=CARTESIAN_POINT('Ctrl Pts',(2.08121842339136,-92.5030998968131,
-25.0233036000206));
#271095=CARTESIAN_POINT('Ctrl Pts',(1.12083047611226,-92.5030998968147,
-17.6522940965419));
#271096=CARTESIAN_POINT('Ctrl Pts',(3.0780812402123,-85.0202717903424,-27.1501754494839));
#271097=CARTESIAN_POINT('Ctrl Pts',(2.77549818896186,-92.5030998968163,
-25.2259546915078));
#271098=CARTESIAN_POINT('Ctrl Pts',(1.56980869024178,-92.5030998968147,
-17.5876430272881));
#271099=CARTESIAN_POINT('Ctrl Pts',(3.38194948801199,-84.8206163093558,
-27.1501601110217));
#271100=CARTESIAN_POINT('Ctrl Pts',(3.08467361627495,-92.5030998968131,
-25.3424934416491));
#271101=CARTESIAN_POINT('Ctrl Pts',(1.79438464918826,-92.5030998968147,
-17.5507208438431));
#271102=CARTESIAN_POINT('Ctrl Pts',(3.89377079482511,-84.4303577244072,
-27.1501289936074));
#271103=CARTESIAN_POINT('Ctrl Pts',(3.62855575415517,-92.5030998968163,
-25.5852049434394));
#271104=CARTESIAN_POINT('Ctrl Pts',(2.24356700539472,-92.5030998968147,
-17.4752655247545));
#271105=CARTESIAN_POINT('Ctrl Pts',(4.10257681992759,-84.2394549664702,
-27.1501132274934));
#271106=CARTESIAN_POINT('Ctrl Pts',(3.86265300096946,-92.5030998968147,
-25.711554223593));
#271107=CARTESIAN_POINT('Ctrl Pts',(2.46817300837612,-92.5030998968147,
-17.436753256288));
#271108=CARTESIAN_POINT('Ctrl Pts',(4.45337763448428,-83.8827081815476,
-27.1500827415735));
#271109=CARTESIAN_POINT('Ctrl Pts',(4.26906742896229,-92.5030998968147,
-25.9620711921812));
#271110=CARTESIAN_POINT('Ctrl Pts',(2.91730945232171,-92.5030998968147,
-17.3637278504744));
#271111=CARTESIAN_POINT('Ctrl Pts',(4.59558320478324,-83.716482094176,-27.1500680141482));
#271112=CARTESIAN_POINT('Ctrl Pts',(4.4403397493691,-92.5030998968132,-26.0861356446505));
#271113=CARTESIAN_POINT('Ctrl Pts',(3.14184022161926,-92.5030998968147,
-17.3291973359009));
#271114=CARTESIAN_POINT('Ctrl Pts',(4.83597577945107,-83.410864072468,-27.1500401253627));
#271115=CARTESIAN_POINT('Ctrl Pts',(4.73445387257387,-92.5030998968163,
-26.3263362157338));
#271116=CARTESIAN_POINT('Ctrl Pts',(3.59075876905671,-92.5030998968147,
-17.2677041352167));
#271117=CARTESIAN_POINT('Ctrl Pts',(4.93413245371605,-83.2712700024158,
-27.1500269570775));
#271118=CARTESIAN_POINT('Ctrl Pts',(4.85635963295471,-92.5030998968147,
-26.4422106175989));
#271119=CARTESIAN_POINT('Ctrl Pts',(3.81514693917863,-92.5030998968147,
-17.2407207033043));
#271120=CARTESIAN_POINT('Ctrl Pts',(5.19470999992647,-82.8737477208187,
-27.1499885377058));
#271121=CARTESIAN_POINT('Ctrl Pts',(5.17979449445077,-92.5030998968147,
-26.7890797663465));
#271122=CARTESIAN_POINT('Ctrl Pts',(4.5130376946388,-92.5030998968147,-17.171964762087));
#271123=CARTESIAN_POINT('Ctrl Pts',(5.30881834285142,-82.6567298213553,
-27.1499661445796));
#271124=CARTESIAN_POINT('Ctrl Pts',(5.31191864255755,-92.5030998968147,
-26.997459926319));
#271125=CARTESIAN_POINT('Ctrl Pts',(4.98621969734588,-92.5030998968147,
-17.1472825822804));
#271126=CARTESIAN_POINT('Ctrl Pts',(5.39841089769199,-82.472613872288,-27.1499468655863));
#271127=CARTESIAN_POINT('Ctrl Pts',(5.39819317091255,-92.5030998968147,
-27.1804541962469));
#271128=CARTESIAN_POINT('Ctrl Pts',(5.45887555911843,-92.5030998968147,
-17.150178956551));
#271129=CARTESIAN_POINT('Origin',(1.41042477321282E-15,-82.5030998968147,
-17.7284445206843));
#271130=CARTESIAN_POINT('Ctrl Pts',(-5.39809669430894,-82.4732737992708,
-27.1499469787481));
#271131=CARTESIAN_POINT('Ctrl Pts',(-5.39788655217846,-92.5030998968165,
-27.1797930106087));
#271132=CARTESIAN_POINT('Ctrl Pts',(-5.45726577017968,-92.5030998968147,
-17.1501706266968));
#271133=CARTESIAN_POINT('Ctrl Pts',(-5.30886063243231,-82.6566303581222,
-27.1499658967189));
#271134=CARTESIAN_POINT('Ctrl Pts',(-5.31191862612171,-92.5030998968037,
-26.9975597293636));
#271135=CARTESIAN_POINT('Ctrl Pts',(-4.98640454681432,-92.5030998968147,
-17.1473282668043));
#271136=CARTESIAN_POINT('Ctrl Pts',(-5.19437641593366,-82.8743413684576,
-27.1499880308083));
#271137=CARTESIAN_POINT('Ctrl Pts',(-5.17939033909145,-92.5030998968214,
-26.7885311413234));
#271138=CARTESIAN_POINT('Ctrl Pts',(-4.5118874940125,-92.5030998968147,
-17.1720464128354));
#271139=CARTESIAN_POINT('Ctrl Pts',(-4.93363058595232,-83.2720169605468,
-27.1500258986046));
#271140=CARTESIAN_POINT('Ctrl Pts',(-4.85573761804792,-92.5030998968116,
-26.4415790974878));
#271141=CARTESIAN_POINT('Ctrl Pts',(-3.81392533048433,-92.5030998968147,
-17.2408561198441));
#271142=CARTESIAN_POINT('Ctrl Pts',(-4.83539590630493,-83.4116638334138,
-27.1500388770639));
#271143=CARTESIAN_POINT('Ctrl Pts',(-4.73373456567037,-92.5030998968163,
-26.3256849257087));
#271144=CARTESIAN_POINT('Ctrl Pts',(-3.58954505611625,-92.5030998968147,
-17.2678587127851));
#271145=CARTESIAN_POINT('Ctrl Pts',(-4.5950226526386,-83.7171602823886,
-27.150066343477));
#271146=CARTESIAN_POINT('Ctrl Pts',(-4.43965961273775,-92.5030998968131,
-26.0856204646364));
#271147=CARTESIAN_POINT('Ctrl Pts',(-3.14092565857454,-92.5030998968147,
-17.3293343467266));
#271148=CARTESIAN_POINT('Ctrl Pts',(-4.4529164758076,-83.8832078848245,
-27.1500808379342));
#271149=CARTESIAN_POINT('Ctrl Pts',(-4.26852102169272,-92.5030998968131,
-25.9617090677426));
#271150=CARTESIAN_POINT('Ctrl Pts',(-2.91668691778663,-92.5030998968147,
-17.3638276255333));
#271151=CARTESIAN_POINT('Ctrl Pts',(-4.10263735547408,-84.2393897958904,
-27.1501108287274));
#271152=CARTESIAN_POINT('Ctrl Pts',(-3.86272243617917,-92.5030998968163,
-25.711600464872));
#271153=CARTESIAN_POINT('Ctrl Pts',(-2.46828355116468,-92.5030998968147,
-17.4367367279748));
#271154=CARTESIAN_POINT('Ctrl Pts',(-3.89426477057059,-84.4299010626526,
-27.1501263322654));
#271155=CARTESIAN_POINT('Ctrl Pts',(-3.62910775040391,-92.5030998968131,
-25.5855037071153));
#271156=CARTESIAN_POINT('Ctrl Pts',(-2.24411925992876,-92.5030998968147,
-17.4751702604172));
#271157=CARTESIAN_POINT('Ctrl Pts',(-3.38365208284729,-84.8194236006233,
-27.1501569388914));
#271158=CARTESIAN_POINT('Ctrl Pts',(-3.08643540678968,-92.5030998968163,
-25.3432079853536));
#271159=CARTESIAN_POINT('Ctrl Pts',(-1.79576147994535,-92.5030998968147,
-17.5504920425344));
#271160=CARTESIAN_POINT('Ctrl Pts',(-3.08057929275139,-85.0187465574387,
-27.1501720300308));
#271161=CARTESIAN_POINT('Ctrl Pts',(-2.77799526160932,-92.5030998968131,
-25.2268269826121));
#271162=CARTESIAN_POINT('Ctrl Pts',(-1.57156765625021,-92.5030998968147,
-17.5873625651759));
#271163=CARTESIAN_POINT('Ctrl Pts',(-2.36100384729412,-85.3848777755655,
-27.150198993857));
#271164=CARTESIAN_POINT('Ctrl Pts',(-2.08479461247351,-92.5030998968162,
-25.0241879469932));
#271165=CARTESIAN_POINT('Ctrl Pts',(-1.12300814069231,-92.5030998968147,
-17.6520074619466));
#271166=CARTESIAN_POINT('Ctrl Pts',(-1.94321144755505,-85.5508732644712,
-27.1502107853729));
#271167=CARTESIAN_POINT('Ctrl Pts',(-1.69937754472461,-92.5030998968131,
-24.9375848748653));
#271168=CARTESIAN_POINT('Ctrl Pts',(-0.898640395518054,-92.5030998968147,
-17.6796731644661));
#271169=CARTESIAN_POINT('Ctrl Pts',(-0.966563031715962,-85.7995116268941,
-27.1502282342258));
#271170=CARTESIAN_POINT('Ctrl Pts',(-0.832525978497703,-92.5030998968165,
-24.8117943080671));
#271171=CARTESIAN_POINT('Ctrl Pts',(-0.425031788870384,-92.5030998968147,
-17.7200662512515));
#271172=CARTESIAN_POINT('Ctrl Pts',(-0.398829554477319,-85.8683863875495,
-27.150232923976));
#271173=CARTESIAN_POINT('Ctrl Pts',(-0.342329126887928,-92.5030998968067,
-24.7785206905936));
#271174=CARTESIAN_POINT('Ctrl Pts',(-0.175752411133516,-92.5030998968147,
-17.7306309540816));
#271175=CARTESIAN_POINT('Ctrl Pts',(0.167436639224824,-85.8517605842216,
-27.1502317757357));
#271176=CARTESIAN_POINT('Ctrl Pts',(0.143847524607735,-92.5030998968173,
-24.7865630937963));
#271177=CARTESIAN_POINT('Ctrl Pts',(0.0737804994758404,-92.5030998968147,
-17.7280665405117));
#271178=CARTESIAN_POINT('Origin',(-5.38401031719611,-82.5030998968147,-17.14995));
#271179=CARTESIAN_POINT('Origin',(0.,-82.5030998968147,143.53805));
#271180=CARTESIAN_POINT('Origin',(-63.0894692252869,-82.5030998968147,143.53805));
#271181=CARTESIAN_POINT('Origin',(-63.0894692252869,-82.5030998968147,178.93805));
#271182=CARTESIAN_POINT('Origin',(-63.0894692252869,-82.5030998968147,-17.14995));
#271183=CARTESIAN_POINT('Origin',(-63.0894692252869,-82.5030998968147,143.53805));
#271184=CARTESIAN_POINT('Origin',(-73.0894692252869,-82.5030998968147,-17.14995));
#271185=CARTESIAN_POINT('Origin',(-63.0894692252869,-82.5030998968147,-17.14995));
#271186=CARTESIAN_POINT('Origin',(-63.0894692252869,-82.5030998968147,143.53805));
#271187=CARTESIAN_POINT('Origin',(-63.0894692252869,-82.5030998968147,143.53805));
#271188=CARTESIAN_POINT('Origin',(-63.0894692252869,-82.5030998968147,-17.14995));
#271189=CARTESIAN_POINT('Origin',(-63.0894692252869,-82.5030998968147,-17.14995));
#271190=CARTESIAN_POINT('Origin',(-63.0894692252869,0.,143.53805));
#271191=CARTESIAN_POINT('Origin',(-63.0894692252885,54.390525141761,143.538050000002));
#271192=CARTESIAN_POINT('Origin',(-63.0894692252869,-64.3905251417593,-17.14995));
#271193=CARTESIAN_POINT('Origin',(-63.0894692252876,54.39052514176,-17.1499500000007));
#271194=CARTESIAN_POINT('Origin',(-63.0894692252869,54.3905251417593,178.93805));
#310583=UNCERTAINTY_MEASURE_WITH_UNIT(LENGTH_MEASURE(0.01),#310624,
'DISTANCE_ACCURACY_VALUE',
'Maximum model space distance between geometric entities at asserted c
onnectivities');
#310601=UNCERTAINTY_MEASURE_WITH_UNIT(LENGTH_MEASURE(0.01),#310624,
'DISTANCE_ACCURACY_VALUE',
'Maximum model space distance between geometric entities at asserted c
onnectivities');
#310605=(
GEOMETRIC_REPRESENTATION_CONTEXT(3)
GLOBAL_UNCERTAINTY_ASSIGNED_CONTEXT((#310583))
GLOBAL_UNIT_ASSIGNED_CONTEXT((#310624,#310626,#310627))
REPRESENTATION_CONTEXT('','3D')
);
#310623=(
GEOMETRIC_REPRESENTATION_CONTEXT(3)
GLOBAL_UNCERTAINTY_ASSIGNED_CONTEXT((#310601))
GLOBAL_UNIT_ASSIGNED_CONTEXT((#310624,#310626,#310627))
REPRESENTATION_CONTEXT('','3D')
);
#310624=(
LENGTH_UNIT()
NAMED_UNIT(*)
SI_UNIT(.MILLI.,.METRE.)
);
#310626=(
NAMED_UNIT(*)
PLANE_ANGLE_UNIT()
SI_UNIT($,.RADIAN.)
);
#310627=(
NAMED_UNIT(*)
SI_UNIT($,.STERADIAN.)
SOLID_ANGLE_UNIT()
);
#310631=SHAPE_DEFINITION_REPRESENTATION(#310652,#310896);
#310652=PRODUCT_DEFINITION_SHAPE('',$,#310918);
#310896=SHAPE_REPRESENTATION('',(#94082),#310605);
#310914=PRODUCT_DEFINITION_CONTEXT('part definition',#310979,'design');
#310918=PRODUCT_DEFINITION('Motor with Mount Bracket',
'Motor with Mount Bracket',#310939,#310914);
#310939=PRODUCT_DEFINITION_FORMATION('',$,#310984);
#310979=APPLICATION_CONTEXT(
'Core Data for Automotive Mechanical Design Process');
#310980=PRODUCT_CONTEXT('part definition',#310979,'mechanical');
#310984=PRODUCT('Motor with Mount Bracket','Motor with Mount Bracket',$,
(#310980));
#311005=PRESENTATION_STYLE_ASSIGNMENT((#311012));
#311012=SURFACE_STYLE_USAGE(.BOTH.,#311019);
#311019=SURFACE_SIDE_STYLE('',(#311026));
#311026=SURFACE_STYLE_FILL_AREA(#311033);
#311033=FILL_AREA_STYLE('Opaque(20,51,87)',(#311040));
#311040=FILL_AREA_STYLE_COLOUR('Opaque(20,51,87)',#311047);
#311047=COLOUR_RGB('Opaque(20,51,87)',0.0784313725490196,0.2,0.341176470588235);
ENDSEC;
END-ISO-10303-21;
